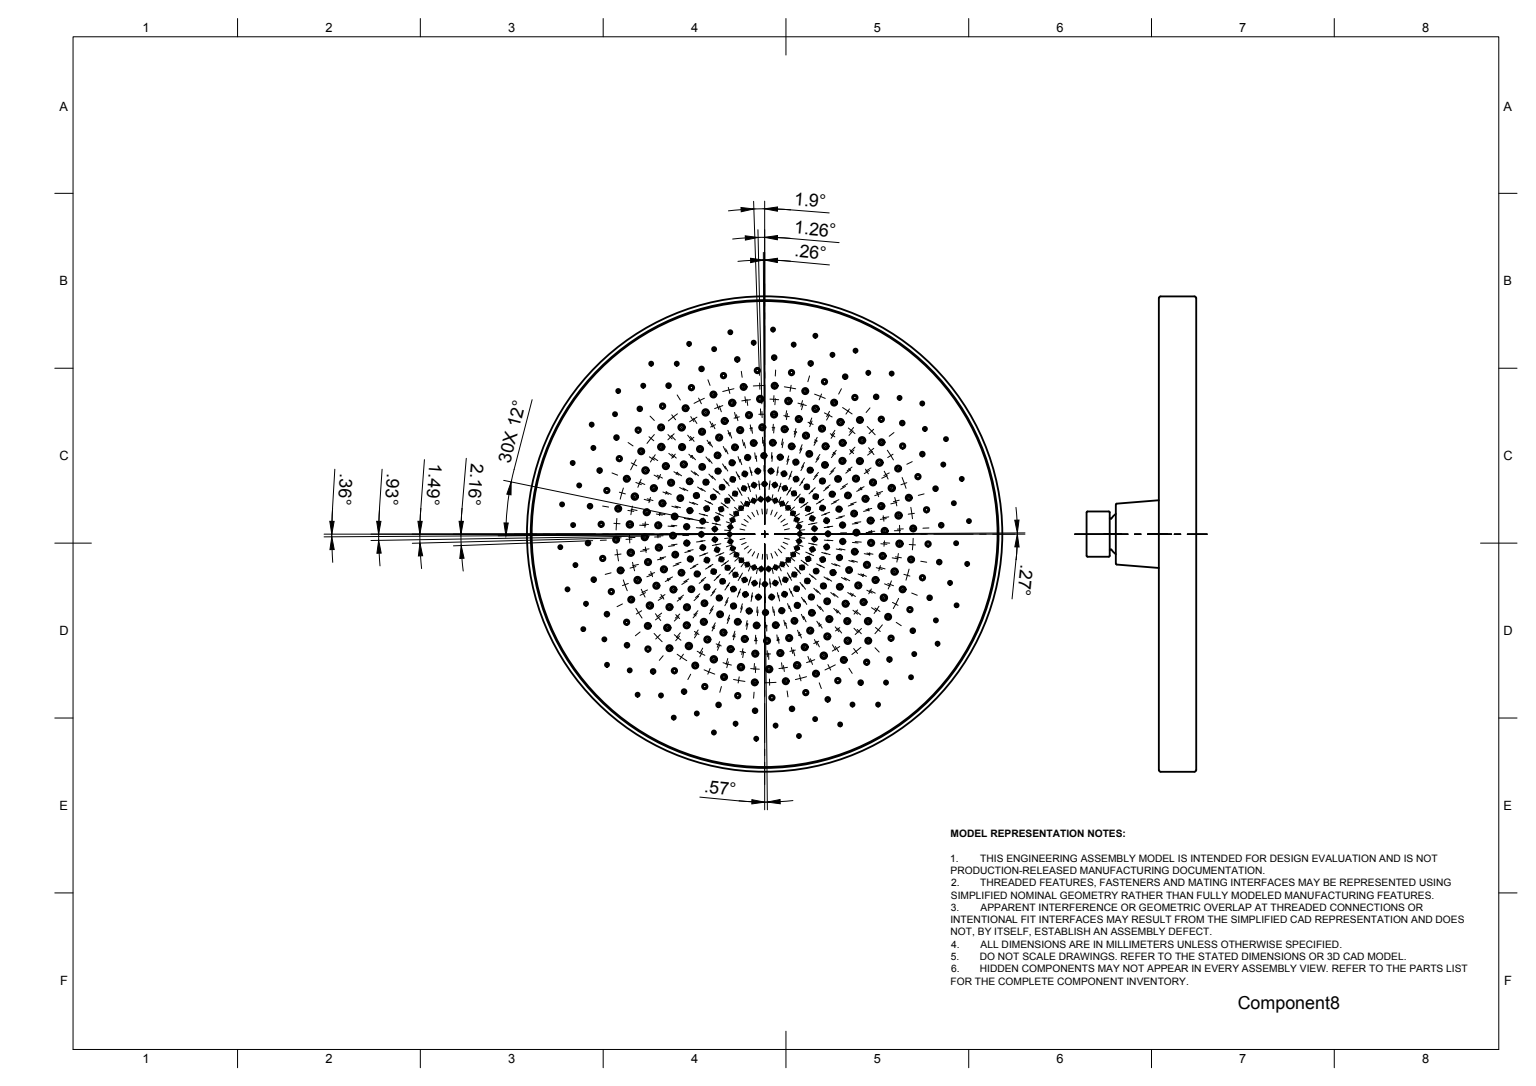
ISO-10303-21;
HEADER;
/* Generated by software containing ST-Developer
 * from STEP Tools, Inc. (www.steptools.com) 
 */

FILE_DESCRIPTION(
/* description */ ('STEP AP214'),
/* implementation_level */ '2;1');

FILE_NAME(
/* name */ 'Component8.step',
/* time_stamp */ '2026-10-06T11:02:40-07:00',
/* author */ (''),
/* organization */ (''),
/* preprocessor_version */ 'ST-DEVELOPER v20.2',
/* originating_system */ 'Autodesk Translation Framework v15.15.0.0',
/* authorisation */ '');

FILE_SCHEMA (('AUTOMOTIVE_DESIGN { 1 0 10303 214 3 1 1 }'));
ENDSEC;

DATA;
#10=MECHANICAL_DESIGN_GEOMETRIC_PRESENTATION_REPRESENTATION('',(#2943),#130910);
#70=SPHERICAL_SURFACE('',#50902,14.1583614602198);
#82=CONICAL_SURFACE('',#50915,18.5103550292801,0.080595262641945);
#732=FACE_BOUND('',#15338,.T.);
#733=FACE_BOUND('',#15339,.T.);
#734=FACE_BOUND('',#15340,.T.);
#735=FACE_BOUND('',#15341,.T.);
#736=FACE_BOUND('',#15342,.T.);
#737=FACE_BOUND('',#15343,.T.);
#738=FACE_BOUND('',#15344,.T.);
#739=FACE_BOUND('',#15345,.T.);
#740=FACE_BOUND('',#15346,.T.);
#741=FACE_BOUND('',#15347,.T.);
#742=FACE_BOUND('',#15348,.T.);
#743=FACE_BOUND('',#15349,.T.);
#744=FACE_BOUND('',#15350,.T.);
#745=FACE_BOUND('',#15351,.T.);
#746=FACE_BOUND('',#15352,.T.);
#747=FACE_BOUND('',#15353,.T.);
#748=FACE_BOUND('',#15354,.T.);
#749=FACE_BOUND('',#15355,.T.);
#750=FACE_BOUND('',#15356,.T.);
#751=FACE_BOUND('',#15357,.T.);
#752=FACE_BOUND('',#15358,.T.);
#753=FACE_BOUND('',#15359,.T.);
#754=FACE_BOUND('',#15360,.T.);
#755=FACE_BOUND('',#15361,.T.);
#756=FACE_BOUND('',#15362,.T.);
#757=FACE_BOUND('',#15363,.T.);
#758=FACE_BOUND('',#15364,.T.);
#759=FACE_BOUND('',#15365,.T.);
#760=FACE_BOUND('',#15366,.T.);
#761=FACE_BOUND('',#15367,.T.);
#762=FACE_BOUND('',#15368,.T.);
#763=FACE_BOUND('',#15369,.T.);
#764=FACE_BOUND('',#15370,.T.);
#765=FACE_BOUND('',#15371,.T.);
#766=FACE_BOUND('',#15372,.T.);
#767=FACE_BOUND('',#15373,.T.);
#768=FACE_BOUND('',#15374,.T.);
#769=FACE_BOUND('',#15375,.T.);
#770=FACE_BOUND('',#15376,.T.);
#771=FACE_BOUND('',#15377,.T.);
#772=FACE_BOUND('',#15378,.T.);
#773=FACE_BOUND('',#15379,.T.);
#774=FACE_BOUND('',#15380,.T.);
#775=FACE_BOUND('',#15381,.T.);
#776=FACE_BOUND('',#15382,.T.);
#777=FACE_BOUND('',#15383,.T.);
#778=FACE_BOUND('',#15384,.T.);
#779=FACE_BOUND('',#15385,.T.);
#780=FACE_BOUND('',#15386,.T.);
#781=FACE_BOUND('',#15387,.T.);
#782=FACE_BOUND('',#15388,.T.);
#783=FACE_BOUND('',#15389,.T.);
#784=FACE_BOUND('',#15390,.T.);
#785=FACE_BOUND('',#15391,.T.);
#786=FACE_BOUND('',#15392,.T.);
#787=FACE_BOUND('',#15393,.T.);
#788=FACE_BOUND('',#15394,.T.);
#789=FACE_BOUND('',#15395,.T.);
#790=FACE_BOUND('',#15396,.T.);
#791=FACE_BOUND('',#15397,.T.);
#792=FACE_BOUND('',#16183,.T.);
#793=FACE_BOUND('',#16193,.T.);
#794=FACE_BOUND('',#16196,.T.);
#795=FACE_BOUND('',#16198,.T.);
#796=FACE_BOUND('',#16200,.T.);
#797=FACE_BOUND('',#16203,.T.);
#798=FACE_BOUND('',#16205,.T.);
#799=FACE_BOUND('',#16206,.T.);
#800=FACE_BOUND('',#16207,.T.);
#801=FACE_BOUND('',#16208,.T.);
#802=FACE_BOUND('',#16209,.T.);
#803=FACE_BOUND('',#16210,.T.);
#804=FACE_BOUND('',#16211,.T.);
#805=FACE_BOUND('',#16212,.T.);
#806=FACE_BOUND('',#16213,.T.);
#807=FACE_BOUND('',#16214,.T.);
#808=FACE_BOUND('',#16215,.T.);
#809=FACE_BOUND('',#16216,.T.);
#810=FACE_BOUND('',#16217,.T.);
#811=FACE_BOUND('',#16218,.T.);
#812=FACE_BOUND('',#16219,.T.);
#813=FACE_BOUND('',#16220,.T.);
#814=FACE_BOUND('',#16221,.T.);
#815=FACE_BOUND('',#16222,.T.);
#816=FACE_BOUND('',#16223,.T.);
#817=FACE_BOUND('',#16224,.T.);
#818=FACE_BOUND('',#16225,.T.);
#819=FACE_BOUND('',#16226,.T.);
#820=FACE_BOUND('',#16227,.T.);
#821=FACE_BOUND('',#16228,.T.);
#822=FACE_BOUND('',#16229,.T.);
#823=FACE_BOUND('',#16230,.T.);
#824=FACE_BOUND('',#16231,.T.);
#825=FACE_BOUND('',#16232,.T.);
#826=FACE_BOUND('',#16233,.T.);
#827=FACE_BOUND('',#16234,.T.);
#828=FACE_BOUND('',#16235,.T.);
#829=FACE_BOUND('',#16236,.T.);
#830=FACE_BOUND('',#16237,.T.);
#831=FACE_BOUND('',#16238,.T.);
#832=FACE_BOUND('',#16239,.T.);
#833=FACE_BOUND('',#16240,.T.);
#834=FACE_BOUND('',#16241,.T.);
#835=FACE_BOUND('',#16242,.T.);
#836=FACE_BOUND('',#16243,.T.);
#837=FACE_BOUND('',#16244,.T.);
#838=FACE_BOUND('',#16245,.T.);
#839=FACE_BOUND('',#16246,.T.);
#840=FACE_BOUND('',#16247,.T.);
#841=FACE_BOUND('',#16248,.T.);
#842=FACE_BOUND('',#16249,.T.);
#843=FACE_BOUND('',#16250,.T.);
#844=FACE_BOUND('',#16251,.T.);
#845=FACE_BOUND('',#16252,.T.);
#846=FACE_BOUND('',#16253,.T.);
#847=FACE_BOUND('',#16254,.T.);
#848=FACE_BOUND('',#16255,.T.);
#849=FACE_BOUND('',#16256,.T.);
#850=FACE_BOUND('',#16257,.T.);
#851=FACE_BOUND('',#16258,.T.);
#852=FACE_BOUND('',#16259,.T.);
#853=FACE_BOUND('',#16260,.T.);
#854=FACE_BOUND('',#16261,.T.);
#855=FACE_BOUND('',#16262,.T.);
#856=FACE_BOUND('',#16263,.T.);
#857=FACE_BOUND('',#16264,.T.);
#858=FACE_BOUND('',#16265,.T.);
#859=FACE_BOUND('',#16266,.T.);
#860=FACE_BOUND('',#16267,.T.);
#861=FACE_BOUND('',#16268,.T.);
#862=FACE_BOUND('',#16269,.T.);
#863=FACE_BOUND('',#16270,.T.);
#864=FACE_BOUND('',#16271,.T.);
#865=FACE_BOUND('',#16272,.T.);
#866=FACE_BOUND('',#16273,.T.);
#867=FACE_BOUND('',#16274,.T.);
#868=FACE_BOUND('',#16275,.T.);
#869=FACE_BOUND('',#16276,.T.);
#870=FACE_BOUND('',#16277,.T.);
#871=FACE_BOUND('',#16278,.T.);
#872=FACE_BOUND('',#16279,.T.);
#873=FACE_BOUND('',#16280,.T.);
#874=FACE_BOUND('',#16281,.T.);
#875=FACE_BOUND('',#16282,.T.);
#876=FACE_BOUND('',#16283,.T.);
#877=FACE_BOUND('',#16284,.T.);
#878=FACE_BOUND('',#16285,.T.);
#879=FACE_BOUND('',#16286,.T.);
#880=FACE_BOUND('',#16287,.T.);
#881=FACE_BOUND('',#16288,.T.);
#882=FACE_BOUND('',#16289,.T.);
#883=FACE_BOUND('',#16290,.T.);
#884=FACE_BOUND('',#16291,.T.);
#885=FACE_BOUND('',#16292,.T.);
#886=FACE_BOUND('',#16293,.T.);
#887=FACE_BOUND('',#16294,.T.);
#888=FACE_BOUND('',#16295,.T.);
#889=FACE_BOUND('',#16296,.T.);
#890=FACE_BOUND('',#16297,.T.);
#891=FACE_BOUND('',#16298,.T.);
#892=FACE_BOUND('',#16299,.T.);
#893=FACE_BOUND('',#16300,.T.);
#894=FACE_BOUND('',#16301,.T.);
#895=FACE_BOUND('',#16302,.T.);
#896=FACE_BOUND('',#16303,.T.);
#897=FACE_BOUND('',#16304,.T.);
#898=FACE_BOUND('',#16305,.T.);
#899=FACE_BOUND('',#16306,.T.);
#900=FACE_BOUND('',#16307,.T.);
#901=FACE_BOUND('',#16308,.T.);
#902=FACE_BOUND('',#16309,.T.);
#903=FACE_BOUND('',#16310,.T.);
#904=FACE_BOUND('',#16311,.T.);
#905=FACE_BOUND('',#16312,.T.);
#906=FACE_BOUND('',#16313,.T.);
#907=FACE_BOUND('',#16314,.T.);
#908=FACE_BOUND('',#16315,.T.);
#909=FACE_BOUND('',#16316,.T.);
#910=FACE_BOUND('',#16317,.T.);
#911=FACE_BOUND('',#16318,.T.);
#912=FACE_BOUND('',#16319,.T.);
#913=FACE_BOUND('',#16320,.T.);
#914=FACE_BOUND('',#16321,.T.);
#915=FACE_BOUND('',#16322,.T.);
#916=FACE_BOUND('',#16323,.T.);
#917=FACE_BOUND('',#16324,.T.);
#918=FACE_BOUND('',#16325,.T.);
#919=FACE_BOUND('',#16326,.T.);
#920=FACE_BOUND('',#16327,.T.);
#921=FACE_BOUND('',#16328,.T.);
#922=FACE_BOUND('',#16329,.T.);
#923=FACE_BOUND('',#16330,.T.);
#924=FACE_BOUND('',#16331,.T.);
#925=FACE_BOUND('',#16332,.T.);
#926=FACE_BOUND('',#16333,.T.);
#927=FACE_BOUND('',#16334,.T.);
#928=FACE_BOUND('',#16335,.T.);
#929=FACE_BOUND('',#16336,.T.);
#930=FACE_BOUND('',#16337,.T.);
#931=FACE_BOUND('',#16338,.T.);
#932=FACE_BOUND('',#16339,.T.);
#933=FACE_BOUND('',#16340,.T.);
#934=FACE_BOUND('',#16341,.T.);
#935=FACE_BOUND('',#16342,.T.);
#936=FACE_BOUND('',#16343,.T.);
#937=FACE_BOUND('',#16344,.T.);
#938=FACE_BOUND('',#16345,.T.);
#939=FACE_BOUND('',#16346,.T.);
#940=FACE_BOUND('',#16347,.T.);
#941=FACE_BOUND('',#16348,.T.);
#942=FACE_BOUND('',#16349,.T.);
#943=FACE_BOUND('',#16350,.T.);
#944=FACE_BOUND('',#16351,.T.);
#945=FACE_BOUND('',#16352,.T.);
#946=FACE_BOUND('',#16353,.T.);
#947=FACE_BOUND('',#16354,.T.);
#948=FACE_BOUND('',#16355,.T.);
#949=FACE_BOUND('',#16356,.T.);
#950=FACE_BOUND('',#16357,.T.);
#951=FACE_BOUND('',#16358,.T.);
#952=FACE_BOUND('',#16359,.T.);
#953=FACE_BOUND('',#16360,.T.);
#954=FACE_BOUND('',#16361,.T.);
#955=FACE_BOUND('',#16362,.T.);
#956=FACE_BOUND('',#16363,.T.);
#957=FACE_BOUND('',#16364,.T.);
#958=FACE_BOUND('',#16365,.T.);
#959=FACE_BOUND('',#16366,.T.);
#960=FACE_BOUND('',#16367,.T.);
#961=FACE_BOUND('',#16368,.T.);
#962=FACE_BOUND('',#16369,.T.);
#963=FACE_BOUND('',#16370,.T.);
#964=FACE_BOUND('',#16371,.T.);
#965=FACE_BOUND('',#16372,.T.);
#966=FACE_BOUND('',#16373,.T.);
#967=FACE_BOUND('',#16374,.T.);
#968=FACE_BOUND('',#16375,.T.);
#969=FACE_BOUND('',#16376,.T.);
#970=FACE_BOUND('',#16377,.T.);
#971=FACE_BOUND('',#16378,.T.);
#972=FACE_BOUND('',#16379,.T.);
#973=FACE_BOUND('',#16380,.T.);
#974=FACE_BOUND('',#16381,.T.);
#975=FACE_BOUND('',#16382,.T.);
#976=FACE_BOUND('',#16383,.T.);
#977=FACE_BOUND('',#16384,.T.);
#978=FACE_BOUND('',#16385,.T.);
#979=FACE_BOUND('',#16386,.T.);
#980=FACE_BOUND('',#16387,.T.);
#981=FACE_BOUND('',#16388,.T.);
#982=FACE_BOUND('',#16389,.T.);
#983=FACE_BOUND('',#16390,.T.);
#984=FACE_BOUND('',#16391,.T.);
#985=FACE_BOUND('',#16392,.T.);
#986=FACE_BOUND('',#16393,.T.);
#987=FACE_BOUND('',#16394,.T.);
#988=FACE_BOUND('',#16395,.T.);
#989=FACE_BOUND('',#16396,.T.);
#990=FACE_BOUND('',#16397,.T.);
#991=FACE_BOUND('',#16398,.T.);
#992=FACE_BOUND('',#16399,.T.);
#993=FACE_BOUND('',#16400,.T.);
#994=FACE_BOUND('',#16401,.T.);
#995=FACE_BOUND('',#16402,.T.);
#996=FACE_BOUND('',#16403,.T.);
#997=FACE_BOUND('',#16404,.T.);
#998=FACE_BOUND('',#16405,.T.);
#999=FACE_BOUND('',#16406,.T.);
#1000=FACE_BOUND('',#16407,.T.);
#1001=FACE_BOUND('',#16408,.T.);
#1002=FACE_BOUND('',#16409,.T.);
#1003=FACE_BOUND('',#16410,.T.);
#1004=FACE_BOUND('',#16411,.T.);
#1005=FACE_BOUND('',#16412,.T.);
#1006=FACE_BOUND('',#16413,.T.);
#1007=FACE_BOUND('',#16414,.T.);
#1008=FACE_BOUND('',#16415,.T.);
#1009=FACE_BOUND('',#16416,.T.);
#1010=FACE_BOUND('',#16417,.T.);
#1011=FACE_BOUND('',#16418,.T.);
#1012=FACE_BOUND('',#16419,.T.);
#1013=FACE_BOUND('',#16420,.T.);
#1014=FACE_BOUND('',#16421,.T.);
#1015=FACE_BOUND('',#16422,.T.);
#1016=FACE_BOUND('',#16423,.T.);
#1017=FACE_BOUND('',#16424,.T.);
#1018=FACE_BOUND('',#16425,.T.);
#1019=FACE_BOUND('',#16426,.T.);
#1020=FACE_BOUND('',#16427,.T.);
#1021=FACE_BOUND('',#16428,.T.);
#1022=FACE_BOUND('',#16429,.T.);
#1023=FACE_BOUND('',#16430,.T.);
#1024=FACE_BOUND('',#16431,.T.);
#1025=FACE_BOUND('',#16432,.T.);
#1026=FACE_BOUND('',#16433,.T.);
#1027=FACE_BOUND('',#16434,.T.);
#1028=FACE_BOUND('',#16435,.T.);
#1029=FACE_BOUND('',#16436,.T.);
#1030=FACE_BOUND('',#16437,.T.);
#1031=FACE_BOUND('',#16438,.T.);
#1032=FACE_BOUND('',#16439,.T.);
#1033=FACE_BOUND('',#16440,.T.);
#1034=FACE_BOUND('',#16441,.T.);
#1035=FACE_BOUND('',#16442,.T.);
#1036=FACE_BOUND('',#16443,.T.);
#1037=FACE_BOUND('',#16444,.T.);
#1038=FACE_BOUND('',#16445,.T.);
#1039=FACE_BOUND('',#16446,.T.);
#1040=FACE_BOUND('',#16447,.T.);
#1041=FACE_BOUND('',#16448,.T.);
#1042=FACE_BOUND('',#16449,.T.);
#1043=FACE_BOUND('',#16450,.T.);
#1044=FACE_BOUND('',#16451,.T.);
#1045=FACE_BOUND('',#16452,.T.);
#1046=FACE_BOUND('',#16453,.T.);
#1047=FACE_BOUND('',#16454,.T.);
#1048=FACE_BOUND('',#16455,.T.);
#1049=FACE_BOUND('',#16456,.T.);
#1050=FACE_BOUND('',#16457,.T.);
#1051=FACE_BOUND('',#16458,.T.);
#1052=FACE_BOUND('',#16459,.T.);
#1053=FACE_BOUND('',#16460,.T.);
#1054=FACE_BOUND('',#16461,.T.);
#1055=FACE_BOUND('',#16462,.T.);
#1056=FACE_BOUND('',#16463,.T.);
#1057=FACE_BOUND('',#16464,.T.);
#1058=FACE_BOUND('',#16465,.T.);
#1059=FACE_BOUND('',#16466,.T.);
#1060=FACE_BOUND('',#16467,.T.);
#1061=FACE_BOUND('',#16468,.T.);
#1062=FACE_BOUND('',#16469,.T.);
#1063=FACE_BOUND('',#16470,.T.);
#1064=FACE_BOUND('',#16471,.T.);
#1065=FACE_BOUND('',#16472,.T.);
#1066=FACE_BOUND('',#16473,.T.);
#1067=FACE_BOUND('',#16474,.T.);
#1068=FACE_BOUND('',#16476,.T.);
#1069=FACE_BOUND('',#16477,.T.);
#1070=FACE_BOUND('',#16478,.T.);
#1071=FACE_BOUND('',#16479,.T.);
#1072=FACE_BOUND('',#16480,.T.);
#1073=FACE_BOUND('',#16481,.T.);
#1074=FACE_BOUND('',#16482,.T.);
#1075=FACE_BOUND('',#16483,.T.);
#1076=FACE_BOUND('',#16484,.T.);
#1077=FACE_BOUND('',#16485,.T.);
#1078=FACE_BOUND('',#16486,.T.);
#1079=FACE_BOUND('',#16487,.T.);
#1080=FACE_BOUND('',#16488,.T.);
#1081=FACE_BOUND('',#16489,.T.);
#1082=FACE_BOUND('',#16490,.T.);
#1083=FACE_BOUND('',#16491,.T.);
#1084=FACE_BOUND('',#16492,.T.);
#1085=FACE_BOUND('',#16493,.T.);
#1086=FACE_BOUND('',#16494,.T.);
#1087=FACE_BOUND('',#16495,.T.);
#1088=FACE_BOUND('',#16496,.T.);
#1089=FACE_BOUND('',#16497,.T.);
#1090=FACE_BOUND('',#16498,.T.);
#1091=FACE_BOUND('',#16499,.T.);
#1092=FACE_BOUND('',#16500,.T.);
#1093=FACE_BOUND('',#16501,.T.);
#1094=FACE_BOUND('',#16502,.T.);
#1095=FACE_BOUND('',#16503,.T.);
#1096=FACE_BOUND('',#16504,.T.);
#1097=FACE_BOUND('',#16505,.T.);
#1098=FACE_BOUND('',#16506,.T.);
#1099=FACE_BOUND('',#16507,.T.);
#1100=FACE_BOUND('',#16508,.T.);
#1101=FACE_BOUND('',#16509,.T.);
#1102=FACE_BOUND('',#16510,.T.);
#1103=FACE_BOUND('',#16511,.T.);
#1104=FACE_BOUND('',#16512,.T.);
#1105=FACE_BOUND('',#16513,.T.);
#1106=FACE_BOUND('',#16514,.T.);
#1107=FACE_BOUND('',#16515,.T.);
#1108=FACE_BOUND('',#16516,.T.);
#1109=FACE_BOUND('',#16517,.T.);
#1110=FACE_BOUND('',#16518,.T.);
#1111=FACE_BOUND('',#16519,.T.);
#1112=FACE_BOUND('',#16520,.T.);
#1113=FACE_BOUND('',#16521,.T.);
#1114=FACE_BOUND('',#16522,.T.);
#1115=FACE_BOUND('',#16523,.T.);
#1116=FACE_BOUND('',#16524,.T.);
#1117=FACE_BOUND('',#16525,.T.);
#1118=FACE_BOUND('',#16526,.T.);
#1119=FACE_BOUND('',#16527,.T.);
#1120=FACE_BOUND('',#16528,.T.);
#1121=FACE_BOUND('',#16529,.T.);
#1122=FACE_BOUND('',#16530,.T.);
#1123=FACE_BOUND('',#16531,.T.);
#1124=FACE_BOUND('',#16532,.T.);
#1125=FACE_BOUND('',#16533,.T.);
#1126=FACE_BOUND('',#16534,.T.);
#1127=FACE_BOUND('',#16535,.T.);
#1128=FACE_BOUND('',#16538,.T.);
#1129=FACE_BOUND('',#16541,.T.);
#1130=FACE_BOUND('',#16544,.T.);
#1131=FACE_BOUND('',#16547,.T.);
#1132=FACE_BOUND('',#16550,.T.);
#1133=FACE_BOUND('',#16553,.T.);
#1134=FACE_BOUND('',#16556,.T.);
#1135=FACE_BOUND('',#16559,.T.);
#1136=FACE_BOUND('',#16562,.T.);
#1137=FACE_BOUND('',#16565,.T.);
#1138=FACE_BOUND('',#16568,.T.);
#1139=FACE_BOUND('',#16571,.T.);
#1140=FACE_BOUND('',#16574,.T.);
#1141=FACE_BOUND('',#16577,.T.);
#1142=FACE_BOUND('',#16580,.T.);
#1143=FACE_BOUND('',#16583,.T.);
#1144=FACE_BOUND('',#16586,.T.);
#1145=FACE_BOUND('',#16589,.T.);
#1146=FACE_BOUND('',#16592,.T.);
#1147=FACE_BOUND('',#16595,.T.);
#1148=FACE_BOUND('',#16598,.T.);
#1149=FACE_BOUND('',#16601,.T.);
#1150=FACE_BOUND('',#16604,.T.);
#1151=FACE_BOUND('',#16607,.T.);
#1152=FACE_BOUND('',#16610,.T.);
#1153=FACE_BOUND('',#16613,.T.);
#1154=FACE_BOUND('',#16616,.T.);
#1155=FACE_BOUND('',#16619,.T.);
#1156=FACE_BOUND('',#16622,.T.);
#1157=FACE_BOUND('',#16625,.T.);
#1158=FACE_BOUND('',#16628,.T.);
#1159=FACE_BOUND('',#16631,.T.);
#1160=FACE_BOUND('',#16634,.T.);
#1161=FACE_BOUND('',#16637,.T.);
#1162=FACE_BOUND('',#16640,.T.);
#1163=FACE_BOUND('',#16643,.T.);
#1164=FACE_BOUND('',#16646,.T.);
#1165=FACE_BOUND('',#16649,.T.);
#1166=FACE_BOUND('',#16652,.T.);
#1167=FACE_BOUND('',#16655,.T.);
#1168=FACE_BOUND('',#16658,.T.);
#1169=FACE_BOUND('',#16661,.T.);
#1170=FACE_BOUND('',#16664,.T.);
#1171=FACE_BOUND('',#16667,.T.);
#1172=FACE_BOUND('',#16670,.T.);
#1173=FACE_BOUND('',#16673,.T.);
#1174=FACE_BOUND('',#16676,.T.);
#1175=FACE_BOUND('',#16679,.T.);
#1176=FACE_BOUND('',#16682,.T.);
#1177=FACE_BOUND('',#16685,.T.);
#1178=FACE_BOUND('',#16688,.T.);
#1179=FACE_BOUND('',#16691,.T.);
#1180=FACE_BOUND('',#16694,.T.);
#1181=FACE_BOUND('',#16697,.T.);
#1182=FACE_BOUND('',#16700,.T.);
#1183=FACE_BOUND('',#16703,.T.);
#1184=FACE_BOUND('',#16706,.T.);
#1185=FACE_BOUND('',#16709,.T.);
#1186=FACE_BOUND('',#16712,.T.);
#1187=FACE_BOUND('',#16715,.T.);
#1188=FACE_BOUND('',#16718,.T.);
#1189=FACE_BOUND('',#16721,.T.);
#1190=FACE_BOUND('',#16724,.T.);
#1191=FACE_BOUND('',#16727,.T.);
#1192=FACE_BOUND('',#16730,.T.);
#1193=FACE_BOUND('',#16733,.T.);
#1194=FACE_BOUND('',#16736,.T.);
#1195=FACE_BOUND('',#16739,.T.);
#1196=FACE_BOUND('',#16742,.T.);
#1197=FACE_BOUND('',#16745,.T.);
#1198=FACE_BOUND('',#16748,.T.);
#1199=FACE_BOUND('',#16751,.T.);
#1200=FACE_BOUND('',#16754,.T.);
#1201=FACE_BOUND('',#16757,.T.);
#1202=FACE_BOUND('',#16760,.T.);
#1203=FACE_BOUND('',#16763,.T.);
#1204=FACE_BOUND('',#16766,.T.);
#1205=FACE_BOUND('',#16769,.T.);
#1206=FACE_BOUND('',#16772,.T.);
#1207=FACE_BOUND('',#16775,.T.);
#1208=FACE_BOUND('',#16778,.T.);
#1209=FACE_BOUND('',#16781,.T.);
#1210=FACE_BOUND('',#16784,.T.);
#1211=FACE_BOUND('',#16787,.T.);
#1212=FACE_BOUND('',#16790,.T.);
#1213=FACE_BOUND('',#16793,.T.);
#1214=FACE_BOUND('',#16796,.T.);
#1215=FACE_BOUND('',#16799,.T.);
#1216=FACE_BOUND('',#16802,.T.);
#1217=FACE_BOUND('',#16805,.T.);
#1218=FACE_BOUND('',#16808,.T.);
#1219=FACE_BOUND('',#16811,.T.);
#1220=FACE_BOUND('',#16814,.T.);
#1221=FACE_BOUND('',#16817,.T.);
#1222=FACE_BOUND('',#16820,.T.);
#1223=FACE_BOUND('',#16823,.T.);
#1224=FACE_BOUND('',#16826,.T.);
#1225=FACE_BOUND('',#16829,.T.);
#1226=FACE_BOUND('',#16832,.T.);
#1227=FACE_BOUND('',#16835,.T.);
#1228=FACE_BOUND('',#16838,.T.);
#1229=FACE_BOUND('',#16841,.T.);
#1230=FACE_BOUND('',#16844,.T.);
#1231=FACE_BOUND('',#16847,.T.);
#1232=FACE_BOUND('',#16850,.T.);
#1233=FACE_BOUND('',#16853,.T.);
#1234=FACE_BOUND('',#16856,.T.);
#1235=FACE_BOUND('',#16859,.T.);
#1236=FACE_BOUND('',#16862,.T.);
#1237=FACE_BOUND('',#16865,.T.);
#1238=FACE_BOUND('',#16868,.T.);
#1239=FACE_BOUND('',#16871,.T.);
#1240=FACE_BOUND('',#16874,.T.);
#1241=FACE_BOUND('',#16877,.T.);
#1242=FACE_BOUND('',#16880,.T.);
#1243=FACE_BOUND('',#16883,.T.);
#1244=FACE_BOUND('',#16886,.T.);
#1245=FACE_BOUND('',#16889,.T.);
#1246=FACE_BOUND('',#16892,.T.);
#1247=FACE_BOUND('',#16895,.T.);
#1248=FACE_BOUND('',#16898,.T.);
#1249=FACE_BOUND('',#16901,.T.);
#1250=FACE_BOUND('',#16904,.T.);
#1251=FACE_BOUND('',#16907,.T.);
#1252=FACE_BOUND('',#16910,.T.);
#1253=FACE_BOUND('',#16913,.T.);
#1254=FACE_BOUND('',#16916,.T.);
#1255=FACE_BOUND('',#16919,.T.);
#1256=FACE_BOUND('',#16922,.T.);
#1257=FACE_BOUND('',#16925,.T.);
#1258=FACE_BOUND('',#16928,.T.);
#1259=FACE_BOUND('',#16931,.T.);
#1260=FACE_BOUND('',#16934,.T.);
#1261=FACE_BOUND('',#16937,.T.);
#1262=FACE_BOUND('',#16940,.T.);
#1263=FACE_BOUND('',#16943,.T.);
#1264=FACE_BOUND('',#16946,.T.);
#1265=FACE_BOUND('',#16949,.T.);
#1266=FACE_BOUND('',#16952,.T.);
#1267=FACE_BOUND('',#16955,.T.);
#1268=FACE_BOUND('',#16958,.T.);
#1269=FACE_BOUND('',#16961,.T.);
#1270=FACE_BOUND('',#16964,.T.);
#1271=FACE_BOUND('',#16967,.T.);
#1272=FACE_BOUND('',#16970,.T.);
#1273=FACE_BOUND('',#16973,.T.);
#1274=FACE_BOUND('',#16976,.T.);
#1275=FACE_BOUND('',#16979,.T.);
#1276=FACE_BOUND('',#16982,.T.);
#1277=FACE_BOUND('',#16985,.T.);
#1278=FACE_BOUND('',#16988,.T.);
#1279=FACE_BOUND('',#16991,.T.);
#1280=FACE_BOUND('',#16994,.T.);
#1281=FACE_BOUND('',#16997,.T.);
#1282=FACE_BOUND('',#17000,.T.);
#1283=FACE_BOUND('',#17003,.T.);
#1284=FACE_BOUND('',#17006,.T.);
#1285=FACE_BOUND('',#17009,.T.);
#1286=FACE_BOUND('',#17012,.T.);
#1287=FACE_BOUND('',#17015,.T.);
#1288=FACE_BOUND('',#17018,.T.);
#1289=FACE_BOUND('',#17021,.T.);
#1290=FACE_BOUND('',#17024,.T.);
#1291=FACE_BOUND('',#17027,.T.);
#1292=FACE_BOUND('',#17030,.T.);
#1293=FACE_BOUND('',#17033,.T.);
#1294=FACE_BOUND('',#17036,.T.);
#1295=FACE_BOUND('',#17039,.T.);
#1296=FACE_BOUND('',#17042,.T.);
#1297=FACE_BOUND('',#17045,.T.);
#1298=FACE_BOUND('',#17048,.T.);
#1299=FACE_BOUND('',#17051,.T.);
#1300=FACE_BOUND('',#17054,.T.);
#1301=FACE_BOUND('',#17057,.T.);
#1302=FACE_BOUND('',#17060,.T.);
#1303=FACE_BOUND('',#17063,.T.);
#1304=FACE_BOUND('',#17066,.T.);
#1305=FACE_BOUND('',#17069,.T.);
#1306=FACE_BOUND('',#17072,.T.);
#1307=FACE_BOUND('',#17075,.T.);
#1308=FACE_BOUND('',#17078,.T.);
#1309=FACE_BOUND('',#17081,.T.);
#1310=FACE_BOUND('',#17084,.T.);
#1311=FACE_BOUND('',#17087,.T.);
#1312=FACE_BOUND('',#17090,.T.);
#1313=FACE_BOUND('',#17093,.T.);
#1314=FACE_BOUND('',#17096,.T.);
#1315=FACE_BOUND('',#17099,.T.);
#1316=FACE_BOUND('',#17102,.T.);
#1317=FACE_BOUND('',#17105,.T.);
#1318=FACE_BOUND('',#17108,.T.);
#1319=FACE_BOUND('',#17111,.T.);
#1320=FACE_BOUND('',#17114,.T.);
#1321=FACE_BOUND('',#17117,.T.);
#1322=FACE_BOUND('',#17120,.T.);
#1323=FACE_BOUND('',#17123,.T.);
#1324=FACE_BOUND('',#17126,.T.);
#1325=FACE_BOUND('',#17129,.T.);
#1326=FACE_BOUND('',#17132,.T.);
#1327=FACE_BOUND('',#17135,.T.);
#1328=FACE_BOUND('',#17138,.T.);
#1329=FACE_BOUND('',#17141,.T.);
#1330=FACE_BOUND('',#17144,.T.);
#1331=FACE_BOUND('',#17147,.T.);
#1332=FACE_BOUND('',#17150,.T.);
#1333=FACE_BOUND('',#17153,.T.);
#1334=FACE_BOUND('',#17156,.T.);
#1335=FACE_BOUND('',#17159,.T.);
#1336=FACE_BOUND('',#17162,.T.);
#1337=FACE_BOUND('',#17165,.T.);
#1338=FACE_BOUND('',#17168,.T.);
#1339=FACE_BOUND('',#17171,.T.);
#1340=FACE_BOUND('',#17174,.T.);
#1341=FACE_BOUND('',#17177,.T.);
#1342=FACE_BOUND('',#17180,.T.);
#1343=FACE_BOUND('',#17183,.T.);
#1344=FACE_BOUND('',#17186,.T.);
#1345=FACE_BOUND('',#17189,.T.);
#1346=FACE_BOUND('',#17192,.T.);
#1347=FACE_BOUND('',#17195,.T.);
#1348=FACE_BOUND('',#17198,.T.);
#1349=FACE_BOUND('',#17201,.T.);
#1350=FACE_BOUND('',#17204,.T.);
#1351=FACE_BOUND('',#17207,.T.);
#1352=FACE_BOUND('',#17210,.T.);
#1353=FACE_BOUND('',#17213,.T.);
#1354=FACE_BOUND('',#17216,.T.);
#1355=FACE_BOUND('',#17219,.T.);
#1356=FACE_BOUND('',#17222,.T.);
#1357=FACE_BOUND('',#17225,.T.);
#1358=FACE_BOUND('',#17228,.T.);
#1359=FACE_BOUND('',#17231,.T.);
#1360=FACE_BOUND('',#17234,.T.);
#1361=FACE_BOUND('',#17237,.T.);
#1362=FACE_BOUND('',#17240,.T.);
#1363=FACE_BOUND('',#17243,.T.);
#1364=FACE_BOUND('',#17246,.T.);
#1365=FACE_BOUND('',#17249,.T.);
#1366=FACE_BOUND('',#17252,.T.);
#1367=FACE_BOUND('',#17255,.T.);
#1368=FACE_BOUND('',#17258,.T.);
#1369=FACE_BOUND('',#17261,.T.);
#1370=FACE_BOUND('',#17264,.T.);
#1371=FACE_BOUND('',#17267,.T.);
#1372=FACE_BOUND('',#17270,.T.);
#1373=FACE_BOUND('',#17273,.T.);
#1374=FACE_BOUND('',#17276,.T.);
#1375=FACE_BOUND('',#17279,.T.);
#1376=FACE_BOUND('',#17282,.T.);
#1377=FACE_BOUND('',#17285,.T.);
#1378=FACE_BOUND('',#17288,.T.);
#1379=FACE_BOUND('',#17291,.T.);
#1380=FACE_BOUND('',#17294,.T.);
#1381=FACE_BOUND('',#17297,.T.);
#1382=FACE_BOUND('',#17300,.T.);
#1383=FACE_BOUND('',#17303,.T.);
#1384=FACE_BOUND('',#17306,.T.);
#1385=FACE_BOUND('',#17309,.T.);
#1386=FACE_BOUND('',#17312,.T.);
#1387=FACE_BOUND('',#17315,.T.);
#1388=FACE_BOUND('',#17318,.T.);
#1389=FACE_BOUND('',#17321,.T.);
#1390=FACE_BOUND('',#17324,.T.);
#1391=FACE_BOUND('',#17327,.T.);
#1392=FACE_BOUND('',#17330,.T.);
#1393=FACE_BOUND('',#17333,.T.);
#1394=FACE_BOUND('',#17336,.T.);
#1395=FACE_BOUND('',#17339,.T.);
#1396=FACE_BOUND('',#17342,.T.);
#1397=FACE_BOUND('',#17345,.T.);
#1398=FACE_BOUND('',#17348,.T.);
#1399=FACE_BOUND('',#17351,.T.);
#1400=FACE_BOUND('',#17354,.T.);
#1401=FACE_BOUND('',#17357,.T.);
#1402=FACE_BOUND('',#17360,.T.);
#1403=FACE_BOUND('',#17363,.T.);
#1404=FACE_BOUND('',#17366,.T.);
#1405=FACE_BOUND('',#17369,.T.);
#1406=FACE_BOUND('',#17372,.T.);
#1407=FACE_BOUND('',#17375,.T.);
#1408=FACE_BOUND('',#17378,.T.);
#1409=FACE_BOUND('',#17381,.T.);
#1410=FACE_BOUND('',#17384,.T.);
#1411=FACE_BOUND('',#17387,.T.);
#1412=FACE_BOUND('',#17390,.T.);
#1413=FACE_BOUND('',#17393,.T.);
#1414=FACE_BOUND('',#17396,.T.);
#1415=FACE_BOUND('',#17399,.T.);
#1416=FACE_BOUND('',#17402,.T.);
#1417=FACE_BOUND('',#17405,.T.);
#1418=FACE_BOUND('',#17408,.T.);
#1419=FACE_BOUND('',#17411,.T.);
#1420=FACE_BOUND('',#17414,.T.);
#1421=FACE_BOUND('',#17417,.T.);
#1422=FACE_BOUND('',#17420,.T.);
#1423=FACE_BOUND('',#17423,.T.);
#1424=FACE_BOUND('',#17426,.T.);
#1425=FACE_BOUND('',#17429,.T.);
#1426=FACE_BOUND('',#17432,.T.);
#1427=FACE_BOUND('',#17435,.T.);
#1428=FACE_BOUND('',#17438,.T.);
#1429=FACE_BOUND('',#17441,.T.);
#1430=FACE_BOUND('',#17444,.T.);
#1431=FACE_BOUND('',#17447,.T.);
#1432=FACE_BOUND('',#17450,.T.);
#1433=FACE_BOUND('',#17453,.T.);
#1434=FACE_BOUND('',#17456,.T.);
#1435=FACE_BOUND('',#17459,.T.);
#1436=FACE_BOUND('',#17462,.T.);
#1437=FACE_BOUND('',#17465,.T.);
#1438=FACE_BOUND('',#17468,.T.);
#1439=FACE_BOUND('',#17471,.T.);
#1440=FACE_BOUND('',#17474,.T.);
#1441=FACE_BOUND('',#17477,.T.);
#1442=FACE_BOUND('',#17480,.T.);
#1443=FACE_BOUND('',#17483,.T.);
#1444=FACE_BOUND('',#17486,.T.);
#1445=FACE_BOUND('',#17489,.T.);
#1446=FACE_BOUND('',#17492,.T.);
#1447=FACE_BOUND('',#17495,.T.);
#1448=FACE_BOUND('',#17498,.T.);
#1449=FACE_BOUND('',#17501,.T.);
#1450=FACE_BOUND('',#17504,.T.);
#1451=FACE_BOUND('',#17507,.T.);
#1452=FACE_BOUND('',#17510,.T.);
#1453=FACE_BOUND('',#17513,.T.);
#1454=FACE_BOUND('',#17516,.T.);
#1455=FACE_BOUND('',#17519,.T.);
#1456=FACE_BOUND('',#17522,.T.);
#1457=FACE_BOUND('',#17525,.T.);
#1458=FACE_BOUND('',#17528,.T.);
#1459=FACE_BOUND('',#17531,.T.);
#1460=FACE_BOUND('',#17534,.T.);
#1461=FACE_BOUND('',#17537,.T.);
#1462=FACE_BOUND('',#17540,.T.);
#1463=FACE_BOUND('',#17543,.T.);
#1464=FACE_BOUND('',#17546,.T.);
#1465=FACE_BOUND('',#17549,.T.);
#1466=FACE_BOUND('',#17552,.T.);
#1467=FACE_BOUND('',#17555,.T.);
#1468=FACE_BOUND('',#17558,.T.);
#1469=FACE_BOUND('',#17561,.T.);
#1470=FACE_BOUND('',#17564,.T.);
#1471=FACE_BOUND('',#17567,.T.);
#1472=FACE_BOUND('',#17570,.T.);
#1473=FACE_BOUND('',#17573,.T.);
#1474=FACE_BOUND('',#17576,.T.);
#1475=FACE_BOUND('',#17579,.T.);
#1476=FACE_BOUND('',#17582,.T.);
#1477=FACE_BOUND('',#17585,.T.);
#1478=FACE_BOUND('',#17588,.T.);
#1479=FACE_BOUND('',#17591,.T.);
#1480=FACE_BOUND('',#17594,.T.);
#1481=FACE_BOUND('',#17597,.T.);
#1482=FACE_BOUND('',#17600,.T.);
#1483=FACE_BOUND('',#17603,.T.);
#1484=FACE_BOUND('',#17606,.T.);
#1485=FACE_BOUND('',#17609,.T.);
#1486=FACE_BOUND('',#17612,.T.);
#1487=FACE_BOUND('',#17615,.T.);
#1488=FACE_BOUND('',#17618,.T.);
#1489=FACE_BOUND('',#17621,.T.);
#1490=FACE_BOUND('',#17624,.T.);
#1491=FACE_BOUND('',#17627,.T.);
#1492=FACE_BOUND('',#17630,.T.);
#1493=FACE_BOUND('',#17633,.T.);
#1494=FACE_BOUND('',#17636,.T.);
#1495=FACE_BOUND('',#17639,.T.);
#1496=FACE_BOUND('',#17642,.T.);
#1497=FACE_BOUND('',#17645,.T.);
#1498=FACE_BOUND('',#17648,.T.);
#1499=FACE_BOUND('',#17651,.T.);
#1500=FACE_BOUND('',#17654,.T.);
#1501=FACE_BOUND('',#17657,.T.);
#1502=FACE_BOUND('',#17660,.T.);
#1503=FACE_BOUND('',#17663,.T.);
#1504=FACE_BOUND('',#17666,.T.);
#1505=FACE_BOUND('',#17669,.T.);
#1506=FACE_BOUND('',#17672,.T.);
#1507=FACE_BOUND('',#17675,.T.);
#1508=FACE_BOUND('',#17678,.T.);
#1509=FACE_BOUND('',#17681,.T.);
#1510=FACE_BOUND('',#17684,.T.);
#1511=FACE_BOUND('',#17687,.T.);
#1512=FACE_BOUND('',#17690,.T.);
#1513=FACE_BOUND('',#17693,.T.);
#1514=FACE_BOUND('',#17696,.T.);
#1515=FACE_BOUND('',#17699,.T.);
#1516=FACE_BOUND('',#17702,.T.);
#1686=(
BOUNDED_SURFACE()
B_SPLINE_SURFACE(2,3,((#106592,#106593,#106594,#106595),(#106596,#106597,
#106598,#106599),(#106600,#106601,#106602,#106603)),.UNSPECIFIED.,.F.,.F.,
 .F.)
B_SPLINE_SURFACE_WITH_KNOTS((3,3),(4,4),(0.,0.976475345222878),(0.,1.),
 .UNSPECIFIED.)
GEOMETRIC_REPRESENTATION_ITEM()
RATIONAL_B_SPLINE_SURFACE(((1.,0.333333333333333,0.333333333333333,1.),
(1.,0.333333333333333,0.333333333333333,1.),(1.,0.333333333333333,0.333333333333333,
1.)))
REPRESENTATION_ITEM('')
SURFACE()
);
#1687=(
BOUNDED_SURFACE()
B_SPLINE_SURFACE(3,3,((#128284,#128285,#128286,#128287),(#128288,#128289,
#128290,#128291),(#128292,#128293,#128294,#128295),(#128296,#128297,#128298,
#128299)),.UNSPECIFIED.,.F.,.F.,.F.)
B_SPLINE_SURFACE_WITH_KNOTS((4,4),(4,4),(0.847987177476328,0.924268857153948),
(0.,1.),.UNSPECIFIED.)
GEOMETRIC_REPRESENTATION_ITEM()
RATIONAL_B_SPLINE_SURFACE(((1.,0.999906698612453,0.999906698612453,1.),
(1.,0.999906698612453,0.999906698612453,1.),(1.,0.999906698612453,0.999906698612453,
1.),(1.,0.999906698612453,0.999906698612453,1.)))
REPRESENTATION_ITEM('')
SURFACE()
);
#1688=(
BOUNDED_SURFACE()
B_SPLINE_SURFACE(2,3,((#128308,#128309,#128310,#128311),(#128312,#128313,
#128314,#128315),(#128316,#128317,#128318,#128319)),.UNSPECIFIED.,.F.,.F.,
 .F.)
B_SPLINE_SURFACE_WITH_KNOTS((3,3),(4,4),(0.,0.976475345222877),(0.,1.),
 .UNSPECIFIED.)
GEOMETRIC_REPRESENTATION_ITEM()
RATIONAL_B_SPLINE_SURFACE(((1.,0.333333333333333,0.333333333333333,1.),
(1.,0.333333333333333,0.333333333333333,1.),(1.,0.333333333333333,0.333333333333333,
1.)))
REPRESENTATION_ITEM('')
SURFACE()
);
#1689=(
BOUNDED_SURFACE()
B_SPLINE_SURFACE(3,3,((#128861,#128862,#128863,#128864),(#128865,#128866,
#128867,#128868),(#128869,#128870,#128871,#128872),(#128873,#128874,#128875,
#128876)),.UNSPECIFIED.,.F.,.F.,.F.)
B_SPLINE_SURFACE_WITH_KNOTS((4,4),(4,4),(0.485044458534508,0.53777950288349),
(0.,1.),.UNSPECIFIED.)
GEOMETRIC_REPRESENTATION_ITEM()
RATIONAL_B_SPLINE_SURFACE(((1.,0.999962226576742,0.999962226576742,1.),
(1.,0.999962226576742,0.999962226576742,1.),(1.,0.999962226576742,0.999962226576742,
1.),(1.,0.999962226576742,0.999962226576742,1.)))
REPRESENTATION_ITEM('')
SURFACE()
);
#1690=(
BOUNDED_SURFACE()
B_SPLINE_SURFACE(3,3,((#128878,#128879,#128880,#128881),(#128882,#128883,
#128884,#128885),(#128886,#128887,#128888,#128889),(#128890,#128891,#128892,
#128893)),.UNSPECIFIED.,.F.,.F.,.F.)
B_SPLINE_SURFACE_WITH_KNOTS((4,4),(4,4),(0.320611406771219,0.371419418548152),
(0.,1.),.UNSPECIFIED.)
GEOMETRIC_REPRESENTATION_ITEM()
RATIONAL_B_SPLINE_SURFACE(((1.,0.999967235134602,0.999967235134602,1.),
(1.,0.999967235134602,0.999967235134602,1.),(1.,0.999967235134602,0.999967235134602,
1.),(1.,0.999967235134602,0.999967235134602,1.)))
REPRESENTATION_ITEM('')
SURFACE()
);
#1691=(
BOUNDED_SURFACE()
B_SPLINE_SURFACE(3,3,((#128895,#128896,#128897,#128898),(#128899,#128900,
#128901,#128902),(#128903,#128904,#128905,#128906),(#128907,#128908,#128909,
#128910)),.UNSPECIFIED.,.F.,.F.,.F.)
B_SPLINE_SURFACE_WITH_KNOTS((4,4),(4,4),(0.675456663809549,0.739075881246651),
(0.,1.),.UNSPECIFIED.)
GEOMETRIC_REPRESENTATION_ITEM()
RATIONAL_B_SPLINE_SURFACE(((1.,0.999940066556315,0.999940066556315,1.),
(1.,0.999940066556315,0.999940066556315,1.),(1.,0.999940066556315,0.999940066556315,
1.),(1.,0.999940066556315,0.999940066556315,1.)))
REPRESENTATION_ITEM('')
SURFACE()
);
#1692=(
BOUNDED_SURFACE()
B_SPLINE_SURFACE(3,3,((#128912,#128913,#128914,#128915),(#128916,#128917,
#128918,#128919),(#128920,#128921,#128922,#128923),(#128924,#128925,#128926,
#128927)),.UNSPECIFIED.,.F.,.F.,.F.)
B_SPLINE_SURFACE_WITH_KNOTS((4,4),(4,4),(0.848056712870581,0.924286002747189),
(0.,1.),.UNSPECIFIED.)
GEOMETRIC_REPRESENTATION_ITEM()
RATIONAL_B_SPLINE_SURFACE(((1.,0.999906141303136,0.999906141303136,1.),
(1.,0.999906141303136,0.999906141303136,1.),(1.,0.999906141303136,0.999906141303136,
1.),(1.,0.999906141303136,0.999906141303136,1.)))
REPRESENTATION_ITEM('')
SURFACE()
);
#1693=(
BOUNDED_SURFACE()
B_SPLINE_SURFACE(3,3,((#128929,#128930,#128931,#128932),(#128933,#128934,
#128935,#128936),(#128937,#128938,#128939,#128940),(#128941,#128942,#128943,
#128944)),.UNSPECIFIED.,.F.,.F.,.F.)
B_SPLINE_SURFACE_WITH_KNOTS((4,4),(4,4),(0.320500925502344,0.371279762151148),
(0.,1.),.UNSPECIFIED.)
GEOMETRIC_REPRESENTATION_ITEM()
RATIONAL_B_SPLINE_SURFACE(((1.,0.999967409032415,0.999967409032415,1.),
(1.,0.999967409032415,0.999967409032415,1.),(1.,0.999967409032415,0.999967409032415,
1.),(1.,0.999967409032415,0.999967409032415,1.)))
REPRESENTATION_ITEM('')
SURFACE()
);
#1694=(
BOUNDED_SURFACE()
B_SPLINE_SURFACE(3,3,((#128946,#128947,#128948,#128949),(#128950,#128951,
#128952,#128953),(#128954,#128955,#128956,#128957),(#128958,#128959,#128960,
#128961)),.UNSPECIFIED.,.F.,.F.,.F.)
B_SPLINE_SURFACE_WITH_KNOTS((4,4),(4,4),(0.485038746158877,0.537899824885899),
(0.,1.),.UNSPECIFIED.)
GEOMETRIC_REPRESENTATION_ITEM()
RATIONAL_B_SPLINE_SURFACE(((1.,0.999962208905504,0.999962208905504,1.),
(1.,0.999962208905504,0.999962208905504,1.),(1.,0.999962208905504,0.999962208905504,
1.),(1.,0.999962208905504,0.999962208905504,1.)))
REPRESENTATION_ITEM('')
SURFACE()
);
#1695=(
BOUNDED_SURFACE()
B_SPLINE_SURFACE(3,3,((#128963,#128964,#128965,#128966),(#128967,#128968,
#128969,#128970),(#128971,#128972,#128973,#128974),(#128975,#128976,#128977,
#128978)),.UNSPECIFIED.,.F.,.F.,.F.)
B_SPLINE_SURFACE_WITH_KNOTS((4,4),(4,4),(0.675591945838646,0.739081108319602),
(0.,1.),.UNSPECIFIED.)
GEOMETRIC_REPRESENTATION_ITEM()
RATIONAL_B_SPLINE_SURFACE(((1.,0.999939919244887,0.999939919244887,1.),
(1.,0.999939919244887,0.999939919244887,1.),(1.,0.999939919244887,0.999939919244887,
1.),(1.,0.999939919244887,0.999939919244887,1.)))
REPRESENTATION_ITEM('')
SURFACE()
);
#1696=(
BOUNDED_SURFACE()
B_SPLINE_SURFACE(3,3,((#128980,#128981,#128982,#128983),(#128984,#128985,
#128986,#128987),(#128988,#128989,#128990,#128991),(#128992,#128993,#128994,
#128995)),.UNSPECIFIED.,.F.,.F.,.F.)
B_SPLINE_SURFACE_WITH_KNOTS((4,4),(4,4),(0.847948073492975,0.924101847380027),
(0.,1.),.UNSPECIFIED.)
GEOMETRIC_REPRESENTATION_ITEM()
RATIONAL_B_SPLINE_SURFACE(((1.,0.999906397449935,0.999906397449935,1.),
(1.,0.999906397449935,0.999906397449935,1.),(1.,0.999906397449935,0.999906397449935,
1.),(1.,0.999906397449935,0.999906397449935,1.)))
REPRESENTATION_ITEM('')
SURFACE()
);
#1697=(
BOUNDED_SURFACE()
B_SPLINE_SURFACE(3,3,((#128997,#128998,#128999,#129000),(#129001,#129002,
#129003,#129004),(#129005,#129006,#129007,#129008),(#129009,#129010,#129011,
#129012)),.UNSPECIFIED.,.F.,.F.,.F.)
B_SPLINE_SURFACE_WITH_KNOTS((4,4),(4,4),(0.320502373890073,0.371416725883164),
(0.,1.),.UNSPECIFIED.)
GEOMETRIC_REPRESENTATION_ITEM()
RATIONAL_B_SPLINE_SURFACE(((1.,0.999967412958646,0.999967412958646,1.),
(1.,0.999967412958646,0.999967412958646,1.),(1.,0.999967412958646,0.999967412958646,
1.),(1.,0.999967412958646,0.999967412958646,1.)))
REPRESENTATION_ITEM('')
SURFACE()
);
#1698=(
BOUNDED_SURFACE()
B_SPLINE_SURFACE(3,3,((#129014,#129015,#129016,#129017),(#129018,#129019,
#129020,#129021),(#129022,#129023,#129024,#129025),(#129026,#129027,#129028,
#129029)),.UNSPECIFIED.,.F.,.F.,.F.)
B_SPLINE_SURFACE_WITH_KNOTS((4,4),(4,4),(0.485176572716987,0.537896306928668),
(0.,1.),.UNSPECIFIED.)
GEOMETRIC_REPRESENTATION_ITEM()
RATIONAL_B_SPLINE_SURFACE(((1.,0.999962047914293,0.999962047914293,1.),
(1.,0.999962047914293,0.999962047914293,1.),(1.,0.999962047914293,0.999962047914293,
1.),(1.,0.999962047914293,0.999962047914293,1.)))
REPRESENTATION_ITEM('')
SURFACE()
);
#1699=(
BOUNDED_SURFACE()
B_SPLINE_SURFACE(3,3,((#129031,#129032,#129033,#129034),(#129035,#129036,
#129037,#129038),(#129039,#129040,#129041,#129042),(#129043,#129044,#129045,
#129046)),.UNSPECIFIED.,.F.,.F.,.F.)
B_SPLINE_SURFACE_WITH_KNOTS((4,4),(4,4),(0.675443757413942,0.738914540526937),
(0.,1.),.UNSPECIFIED.)
GEOMETRIC_REPRESENTATION_ITEM()
RATIONAL_B_SPLINE_SURFACE(((1.,0.999940218802441,0.999940218802441,1.),
(1.,0.999940218802441,0.999940218802441,1.),(1.,0.999940218802441,0.999940218802441,
1.),(1.,0.999940218802441,0.999940218802441,1.)))
REPRESENTATION_ITEM('')
SURFACE()
);
#1700=(
BOUNDED_SURFACE()
B_SPLINE_SURFACE(3,3,((#129048,#129049,#129050,#129051),(#129052,#129053,
#129054,#129055),(#129056,#129057,#129058,#129059),(#129060,#129061,#129062,
#129063)),.UNSPECIFIED.,.F.,.F.,.F.)
B_SPLINE_SURFACE_WITH_KNOTS((4,4),(4,4),(0.847942166937427,0.924299897199325),
(0.,1.),.UNSPECIFIED.)
GEOMETRIC_REPRESENTATION_ITEM()
RATIONAL_B_SPLINE_SURFACE(((1.,0.999906256993129,0.999906256993129,1.),
(1.,0.999906256993129,0.999906256993129,1.),(1.,0.999906256993129,0.999906256993129,
1.),(1.,0.999906256993129,0.999906256993129,1.)))
REPRESENTATION_ITEM('')
SURFACE()
);
#1701=(
BOUNDED_SURFACE()
B_SPLINE_SURFACE(3,3,((#129065,#129066,#129067,#129068),(#129069,#129070,
#129071,#129072),(#129073,#129074,#129075,#129076),(#129077,#129078,#129079,
#129080)),.UNSPECIFIED.,.F.,.F.,.F.)
B_SPLINE_SURFACE_WITH_KNOTS((4,4),(4,4),(0.320591553275913,0.371408509515467),
(0.,1.),.UNSPECIFIED.)
GEOMETRIC_REPRESENTATION_ITEM()
RATIONAL_B_SPLINE_SURFACE(((1.,0.999967222717093,0.999967222717093,1.),
(1.,0.999967222717093,0.999967222717093,1.),(1.,0.999967222717093,0.999967222717093,
1.),(1.,0.999967222717093,0.999967222717093,1.)))
REPRESENTATION_ITEM('')
SURFACE()
);
#1702=(
BOUNDED_SURFACE()
B_SPLINE_SURFACE(3,3,((#129082,#129083,#129084,#129085),(#129086,#129087,
#129088,#129089),(#129090,#129091,#129092,#129093),(#129094,#129095,#129096,
#129097)),.UNSPECIFIED.,.F.,.F.,.F.)
B_SPLINE_SURFACE_WITH_KNOTS((4,4),(4,4),(0.485044526648914,0.537808799135296),
(0.,1.),.UNSPECIFIED.)
GEOMETRIC_REPRESENTATION_ITEM()
RATIONAL_B_SPLINE_SURFACE(((1.,0.999962197880072,0.999962197880072,1.),
(1.,0.999962197880072,0.999962197880072,1.),(1.,0.999962197880072,0.999962197880072,
1.),(1.,0.999962197880072,0.999962197880072,1.)))
REPRESENTATION_ITEM('')
SURFACE()
);
#1703=(
BOUNDED_SURFACE()
B_SPLINE_SURFACE(3,3,((#129099,#129100,#129101,#129102),(#129103,#129104,
#129105,#129106),(#129107,#129108,#129109,#129110),(#129111,#129112,#129113,
#129114)),.UNSPECIFIED.,.F.,.F.,.F.)
B_SPLINE_SURFACE_WITH_KNOTS((4,4),(4,4),(0.675446956850003,0.739072743686735),
(0.,1.),.UNSPECIFIED.)
GEOMETRIC_REPRESENTATION_ITEM()
RATIONAL_B_SPLINE_SURFACE(((1.,0.999940262362188,0.999940262362188,1.),
(1.,0.999940262362188,0.999940262362188,1.),(1.,0.999940262362188,0.999940262362188,
1.),(1.,0.999940262362188,0.999940262362188,1.)))
REPRESENTATION_ITEM('')
SURFACE()
);
#1704=(
BOUNDED_SURFACE()
B_SPLINE_SURFACE(3,3,((#129116,#129117,#129118,#129119),(#129120,#129121,
#129122,#129123),(#129124,#129125,#129126,#129127),(#129128,#129129,#129130,
#129131)),.UNSPECIFIED.,.F.,.F.,.F.)
B_SPLINE_SURFACE_WITH_KNOTS((4,4),(4,4),(0.848119490523076,0.924292153421624),
(0.,1.),.UNSPECIFIED.)
GEOMETRIC_REPRESENTATION_ITEM()
RATIONAL_B_SPLINE_SURFACE(((1.,0.999905838370628,0.999905838370628,1.),
(1.,0.999905838370628,0.999905838370628,1.),(1.,0.999905838370628,0.999905838370628,
1.),(1.,0.999905838370628,0.999905838370628,1.)))
REPRESENTATION_ITEM('')
SURFACE()
);
#1705=(
BOUNDED_SURFACE()
B_SPLINE_SURFACE(3,3,((#129133,#129134,#129135,#129136),(#129137,#129138,
#129139,#129140),(#129141,#129142,#129143,#129144),(#129145,#129146,#129147,
#129148)),.UNSPECIFIED.,.F.,.F.,.F.)
B_SPLINE_SURFACE_WITH_KNOTS((4,4),(4,4),(0.320518889190736,0.371365428236457),
(0.,1.),.UNSPECIFIED.)
GEOMETRIC_REPRESENTATION_ITEM()
RATIONAL_B_SPLINE_SURFACE(((1.,0.999967318979484,0.999967318979484,1.),
(1.,0.999967318979484,0.999967318979484,1.),(1.,0.999967318979484,0.999967318979484,
1.),(1.,0.999967318979484,0.999967318979484,1.)))
REPRESENTATION_ITEM('')
SURFACE()
);
#1706=(
BOUNDED_SURFACE()
B_SPLINE_SURFACE(3,3,((#129150,#129151,#129152,#129153),(#129154,#129155,
#129156,#129157),(#129158,#129159,#129160,#129161),(#129162,#129163,#129164,
#129165)),.UNSPECIFIED.,.F.,.F.,.F.)
B_SPLINE_SURFACE_WITH_KNOTS((4,4),(4,4),(0.485053151926106,0.537874785203655),
(0.,1.),.UNSPECIFIED.)
GEOMETRIC_REPRESENTATION_ITEM()
RATIONAL_B_SPLINE_SURFACE(((1.,0.999962225139893,0.999962225139893,1.),
(1.,0.999962225139893,0.999962225139893,1.),(1.,0.999962225139893,0.999962225139893,
1.),(1.,0.999962225139893,0.999962225139893,1.)))
REPRESENTATION_ITEM('')
SURFACE()
);
#1707=(
BOUNDED_SURFACE()
B_SPLINE_SURFACE(3,3,((#129167,#129168,#129169,#129170),(#129171,#129172,
#129173,#129174),(#129175,#129176,#129177,#129178),(#129179,#129180,#129181,
#129182)),.UNSPECIFIED.,.F.,.F.,.F.)
B_SPLINE_SURFACE_WITH_KNOTS((4,4),(4,4),(0.675540106157524,0.739058970060862),
(0.,1.),.UNSPECIFIED.)
GEOMETRIC_REPRESENTATION_ITEM()
RATIONAL_B_SPLINE_SURFACE(((1.,0.999939959405442,0.999939959405442,1.),
(1.,0.999939959405442,0.999939959405442,1.),(1.,0.999939959405442,0.999939959405442,
1.),(1.,0.999939959405442,0.999939959405442,1.)))
REPRESENTATION_ITEM('')
SURFACE()
);
#1708=(
BOUNDED_SURFACE()
B_SPLINE_SURFACE(3,3,((#129184,#129185,#129186,#129187),(#129188,#129189,
#129190,#129191),(#129192,#129193,#129194,#129195),(#129196,#129197,#129198,
#129199)),.UNSPECIFIED.,.F.,.F.,.F.)
B_SPLINE_SURFACE_WITH_KNOTS((4,4),(4,4),(0.847959162456777,0.924189890634277),
(0.,1.),.UNSPECIFIED.)
GEOMETRIC_REPRESENTATION_ITEM()
RATIONAL_B_SPLINE_SURFACE(((1.,0.999906054677511,0.999906054677511,1.),
(1.,0.999906054677511,0.999906054677511,1.),(1.,0.999906054677511,0.999906054677511,
1.),(1.,0.999906054677511,0.999906054677511,1.)))
REPRESENTATION_ITEM('')
SURFACE()
);
#1709=(
BOUNDED_SURFACE()
B_SPLINE_SURFACE(3,3,((#129201,#129202,#129203,#129204),(#129205,#129206,
#129207,#129208),(#129209,#129210,#129211,#129212),(#129213,#129214,#129215,
#129216)),.UNSPECIFIED.,.F.,.F.,.F.)
B_SPLINE_SURFACE_WITH_KNOTS((4,4),(4,4),(0.320639964684793,0.371314507617759),
(0.,1.),.UNSPECIFIED.)
GEOMETRIC_REPRESENTATION_ITEM()
RATIONAL_B_SPLINE_SURFACE(((1.,0.999967350702174,0.999967350702174,1.),
(1.,0.999967350702174,0.999967350702174,1.),(1.,0.999967350702174,0.999967350702174,
1.),(1.,0.999967350702174,0.999967350702174,1.)))
REPRESENTATION_ITEM('')
SURFACE()
);
#1710=(
BOUNDED_SURFACE()
B_SPLINE_SURFACE(3,3,((#129218,#129219,#129220,#129221),(#129222,#129223,
#129224,#129225),(#129226,#129227,#129228,#129229),(#129230,#129231,#129232,
#129233)),.UNSPECIFIED.,.F.,.F.,.F.)
B_SPLINE_SURFACE_WITH_KNOTS((4,4),(4,4),(0.485088192372813,0.537796433966225),
(0.,1.),.UNSPECIFIED.)
GEOMETRIC_REPRESENTATION_ITEM()
RATIONAL_B_SPLINE_SURFACE(((1.,0.999962120409815,0.999962120409815,1.),
(1.,0.999962120409815,0.999962120409815,1.),(1.,0.999962120409815,0.999962120409815,
1.),(1.,0.999962120409815,0.999962120409815,1.)))
REPRESENTATION_ITEM('')
SURFACE()
);
#1711=(
BOUNDED_SURFACE()
B_SPLINE_SURFACE(3,3,((#129235,#129236,#129237,#129238),(#129239,#129240,
#129241,#129242),(#129243,#129244,#129245,#129246),(#129247,#129248,#129249,
#129250)),.UNSPECIFIED.,.F.,.F.,.F.)
B_SPLINE_SURFACE_WITH_KNOTS((4,4),(4,4),(0.675478450031988,0.739029557635334),
(0.,1.),.UNSPECIFIED.)
GEOMETRIC_REPRESENTATION_ITEM()
RATIONAL_B_SPLINE_SURFACE(((1.,0.999940036715462,0.999940036715462,1.),
(1.,0.999940036715462,0.999940036715462,1.),(1.,0.999940036715462,0.999940036715462,
1.),(1.,0.999940036715462,0.999940036715462,1.)))
REPRESENTATION_ITEM('')
SURFACE()
);
#1712=(
BOUNDED_SURFACE()
B_SPLINE_SURFACE(3,3,((#129252,#129253,#129254,#129255),(#129256,#129257,
#129258,#129259),(#129260,#129261,#129262,#129263),(#129264,#129265,#129266,
#129267)),.UNSPECIFIED.,.F.,.F.,.F.)
B_SPLINE_SURFACE_WITH_KNOTS((4,4),(4,4),(0.847977146575099,0.924247070973153),
(0.,1.),.UNSPECIFIED.)
GEOMETRIC_REPRESENTATION_ITEM()
RATIONAL_B_SPLINE_SURFACE(((1.,0.9999062633542,0.9999062633542,1.),(1.,
0.9999062633542,0.9999062633542,1.),(1.,0.9999062633542,0.9999062633542,
1.),(1.,0.9999062633542,0.9999062633542,1.)))
REPRESENTATION_ITEM('')
SURFACE()
);
#1713=(
BOUNDED_SURFACE()
B_SPLINE_SURFACE(3,3,((#129269,#129270,#129271,#129272),(#129273,#129274,
#129275,#129276),(#129277,#129278,#129279,#129280),(#129281,#129282,#129283,
#129284)),.UNSPECIFIED.,.F.,.F.,.F.)
B_SPLINE_SURFACE_WITH_KNOTS((4,4),(4,4),(0.320583334123496,0.371380663507137),
(0.,1.),.UNSPECIFIED.)
GEOMETRIC_REPRESENTATION_ITEM()
RATIONAL_B_SPLINE_SURFACE(((1.,0.99996730938274,0.99996730938274,1.),(1.,
0.99996730938274,0.99996730938274,1.),(1.,0.99996730938274,0.99996730938274,
1.),(1.,0.99996730938274,0.99996730938274,1.)))
REPRESENTATION_ITEM('')
SURFACE()
);
#1714=(
BOUNDED_SURFACE()
B_SPLINE_SURFACE(3,3,((#129286,#129287,#129288,#129289),(#129290,#129291,
#129292,#129293),(#129294,#129295,#129296,#129297),(#129298,#129299,#129300,
#129301)),.UNSPECIFIED.,.F.,.F.,.F.)
B_SPLINE_SURFACE_WITH_KNOTS((4,4),(4,4),(0.485126102700377,0.537860300944991),
(0.,1.),.UNSPECIFIED.)
GEOMETRIC_REPRESENTATION_ITEM()
RATIONAL_B_SPLINE_SURFACE(((1.,0.999962137299808,0.999962137299808,1.),
(1.,0.999962137299808,0.999962137299808,1.),(1.,0.999962137299808,0.999962137299808,
1.),(1.,0.999962137299808,0.999962137299808,1.)))
REPRESENTATION_ITEM('')
SURFACE()
);
#1715=(
BOUNDED_SURFACE()
B_SPLINE_SURFACE(3,3,((#129303,#129304,#129305,#129306),(#129307,#129308,
#129309,#129310),(#129311,#129312,#129313,#129314),(#129315,#129316,#129317,
#129318)),.UNSPECIFIED.,.F.,.F.,.F.)
B_SPLINE_SURFACE_WITH_KNOTS((4,4),(4,4),(0.675620555481706,0.738956525898373),
(0.,1.),.UNSPECIFIED.)
GEOMETRIC_REPRESENTATION_ITEM()
RATIONAL_B_SPLINE_SURFACE(((1.,0.999940072974474,0.999940072974474,1.),
(1.,0.999940072974474,0.999940072974474,1.),(1.,0.999940072974474,0.999940072974474,
1.),(1.,0.999940072974474,0.999940072974474,1.)))
REPRESENTATION_ITEM('')
SURFACE()
);
#1716=(
BOUNDED_SURFACE()
B_SPLINE_SURFACE(3,3,((#129320,#129321,#129322,#129323),(#129324,#129325,
#129326,#129327),(#129328,#129329,#129330,#129331),(#129332,#129333,#129334,
#129335)),.UNSPECIFIED.,.F.,.F.,.F.)
B_SPLINE_SURFACE_WITH_KNOTS((4,4),(4,4),(0.84799244392776,0.924142505922786),
(0.,1.),.UNSPECIFIED.)
GEOMETRIC_REPRESENTATION_ITEM()
RATIONAL_B_SPLINE_SURFACE(((1.,0.999906153501141,0.999906153501141,1.),
(1.,0.999906153501141,0.999906153501141,1.),(1.,0.999906153501141,0.999906153501141,
1.),(1.,0.999906153501141,0.999906153501141,1.)))
REPRESENTATION_ITEM('')
SURFACE()
);
#1717=(
BOUNDED_SURFACE()
B_SPLINE_SURFACE(3,3,((#129337,#129338,#129339,#129340),(#129341,#129342,
#129343,#129344),(#129345,#129346,#129347,#129348),(#129349,#129350,#129351,
#129352)),.UNSPECIFIED.,.F.,.F.,.F.)
B_SPLINE_SURFACE_WITH_KNOTS((4,4),(4,4),(0.320518100436019,0.371362835533565),
(0.,1.),.UNSPECIFIED.)
GEOMETRIC_REPRESENTATION_ITEM()
RATIONAL_B_SPLINE_SURFACE(((1.,0.999967298407033,0.999967298407033,1.),
(1.,0.999967298407033,0.999967298407033,1.),(1.,0.999967298407033,0.999967298407033,
1.),(1.,0.999967298407033,0.999967298407033,1.)))
REPRESENTATION_ITEM('')
SURFACE()
);
#1718=(
BOUNDED_SURFACE()
B_SPLINE_SURFACE(3,3,((#129354,#129355,#129356,#129357),(#129358,#129359,
#129360,#129361),(#129362,#129363,#129364,#129365),(#129366,#129367,#129368,
#129369)),.UNSPECIFIED.,.F.,.F.,.F.)
B_SPLINE_SURFACE_WITH_KNOTS((4,4),(4,4),(0.485111695336929,0.537875420193652),
(0.,1.),.UNSPECIFIED.)
GEOMETRIC_REPRESENTATION_ITEM()
RATIONAL_B_SPLINE_SURFACE(((1.,0.999962111917502,0.999962111917502,1.),
(1.,0.999962111917502,0.999962111917502,1.),(1.,0.999962111917502,0.999962111917502,
1.),(1.,0.999962111917502,0.999962111917502,1.)))
REPRESENTATION_ITEM('')
SURFACE()
);
#1719=(
BOUNDED_SURFACE()
B_SPLINE_SURFACE(3,3,((#129371,#129372,#129373,#129374),(#129375,#129376,
#129377,#129378),(#129379,#129380,#129381,#129382),(#129383,#129384,#129385,
#129386)),.UNSPECIFIED.,.F.,.F.,.F.)
B_SPLINE_SURFACE_WITH_KNOTS((4,4),(4,4),(0.67554330969252,0.739050792335592),
(0.,1.),.UNSPECIFIED.)
GEOMETRIC_REPRESENTATION_ITEM()
RATIONAL_B_SPLINE_SURFACE(((1.,0.999940183216014,0.999940183216014,1.),
(1.,0.999940183216014,0.999940183216014,1.),(1.,0.999940183216014,0.999940183216014,
1.),(1.,0.999940183216014,0.999940183216014,1.)))
REPRESENTATION_ITEM('')
SURFACE()
);
#1720=(
BOUNDED_SURFACE()
B_SPLINE_SURFACE(3,3,((#129388,#129389,#129390,#129391),(#129392,#129393,
#129394,#129395),(#129396,#129397,#129398,#129399),(#129400,#129401,#129402,
#129403)),.UNSPECIFIED.,.F.,.F.,.F.)
B_SPLINE_SURFACE_WITH_KNOTS((4,4),(4,4),(0.848082295900864,0.924212909944339),
(0.,1.),.UNSPECIFIED.)
GEOMETRIC_REPRESENTATION_ITEM()
RATIONAL_B_SPLINE_SURFACE(((1.,0.999906015094081,0.999906015094081,1.),
(1.,0.999906015094081,0.999906015094081,1.),(1.,0.999906015094081,0.999906015094081,
1.),(1.,0.999906015094081,0.999906015094081,1.)))
REPRESENTATION_ITEM('')
SURFACE()
);
#1721=(
BOUNDED_SURFACE()
B_SPLINE_SURFACE(3,3,((#129405,#129406,#129407,#129408),(#129409,#129410,
#129411,#129412),(#129413,#129414,#129415,#129416),(#129417,#129418,#129419,
#129420)),.UNSPECIFIED.,.F.,.F.,.F.)
B_SPLINE_SURFACE_WITH_KNOTS((4,4),(4,4),(0.320600960423681,0.371411458072819),
(0.,1.),.UNSPECIFIED.)
GEOMETRIC_REPRESENTATION_ITEM()
RATIONAL_B_SPLINE_SURFACE(((1.,0.999967243891018,0.999967243891018,1.),
(1.,0.999967243891018,0.999967243891018,1.),(1.,0.999967243891018,0.999967243891018,
1.),(1.,0.999967243891018,0.999967243891018,1.)))
REPRESENTATION_ITEM('')
SURFACE()
);
#1722=(
BOUNDED_SURFACE()
B_SPLINE_SURFACE(3,3,((#129422,#129423,#129424,#129425),(#129426,#129427,
#129428,#129429),(#129430,#129431,#129432,#129433),(#129434,#129435,#129436,
#129437)),.UNSPECIFIED.,.F.,.F.,.F.)
B_SPLINE_SURFACE_WITH_KNOTS((4,4),(4,4),(0.48504256867854,0.537887934754555),
(0.,1.),.UNSPECIFIED.)
GEOMETRIC_REPRESENTATION_ITEM()
RATIONAL_B_SPLINE_SURFACE(((1.,0.999962231855016,0.999962231855016,1.),
(1.,0.999962231855016,0.999962231855016,1.),(1.,0.999962231855016,0.999962231855016,
1.),(1.,0.999962231855016,0.999962231855016,1.)))
REPRESENTATION_ITEM('')
SURFACE()
);
#1723=(
BOUNDED_SURFACE()
B_SPLINE_SURFACE(3,3,((#129439,#129440,#129441,#129442),(#129443,#129444,
#129445,#129446),(#129447,#129448,#129449,#129450),(#129451,#129452,#129453,
#129454)),.UNSPECIFIED.,.F.,.F.,.F.)
B_SPLINE_SURFACE_WITH_KNOTS((4,4),(4,4),(0.675450724081424,0.73897092350891),
(0.,1.),.UNSPECIFIED.)
GEOMETRIC_REPRESENTATION_ITEM()
RATIONAL_B_SPLINE_SURFACE(((1.,0.99994009649207,0.99994009649207,1.),(1.,
0.99994009649207,0.99994009649207,1.),(1.,0.99994009649207,0.99994009649207,
1.),(1.,0.99994009649207,0.99994009649207,1.)))
REPRESENTATION_ITEM('')
SURFACE()
);
#1724=(
BOUNDED_SURFACE()
B_SPLINE_SURFACE(3,3,((#129456,#129457,#129458,#129459),(#129460,#129461,
#129462,#129463),(#129464,#129465,#129466,#129467),(#129468,#129469,#129470,
#129471)),.UNSPECIFIED.,.F.,.F.,.F.)
B_SPLINE_SURFACE_WITH_KNOTS((4,4),(4,4),(0.848090733102027,0.924284397580542),
(0.,1.),.UNSPECIFIED.)
GEOMETRIC_REPRESENTATION_ITEM()
RATIONAL_B_SPLINE_SURFACE(((1.,0.999905868674041,0.999905868674041,1.),
(1.,0.999905868674041,0.999905868674041,1.),(1.,0.999905868674041,0.999905868674041,
1.),(1.,0.999905868674041,0.999905868674041,1.)))
REPRESENTATION_ITEM('')
SURFACE()
);
#1725=(
BOUNDED_SURFACE()
B_SPLINE_SURFACE(3,3,((#129473,#129474,#129475,#129476),(#129477,#129478,
#129479,#129480),(#129481,#129482,#129483,#129484),(#129485,#129486,#129487,
#129488)),.UNSPECIFIED.,.F.,.F.,.F.)
B_SPLINE_SURFACE_WITH_KNOTS((4,4),(4,4),(0.320500281417297,0.37141920772819),
(0.,1.),.UNSPECIFIED.)
GEOMETRIC_REPRESENTATION_ITEM()
RATIONAL_B_SPLINE_SURFACE(((1.,0.999967398958956,0.999967398958956,1.),
(1.,0.999967398958956,0.999967398958956,1.),(1.,0.999967398958956,0.999967398958956,
1.),(1.,0.999967398958956,0.999967398958956,1.)))
REPRESENTATION_ITEM('')
SURFACE()
);
#1726=(
BOUNDED_SURFACE()
B_SPLINE_SURFACE(3,3,((#129490,#129491,#129492,#129493),(#129494,#129495,
#129496,#129497),(#129498,#129499,#129500,#129501),(#129502,#129503,#129504,
#129505)),.UNSPECIFIED.,.F.,.F.,.F.)
B_SPLINE_SURFACE_WITH_KNOTS((4,4),(4,4),(0.485039113478553,0.537770836541586),
(0.,1.),.UNSPECIFIED.)
GEOMETRIC_REPRESENTATION_ITEM()
RATIONAL_B_SPLINE_SURFACE(((1.,0.999962216400084,0.999962216400084,1.),
(1.,0.999962216400084,0.999962216400084,1.),(1.,0.999962216400084,0.999962216400084,
1.),(1.,0.999962216400084,0.999962216400084,1.)))
REPRESENTATION_ITEM('')
SURFACE()
);
#1727=(
BOUNDED_SURFACE()
B_SPLINE_SURFACE(3,3,((#129507,#129508,#129509,#129510),(#129511,#129512,
#129513,#129514),(#129515,#129516,#129517,#129518),(#129519,#129520,#129521,
#129522)),.UNSPECIFIED.,.F.,.F.,.F.)
B_SPLINE_SURFACE_WITH_KNOTS((4,4),(4,4),(0.675616885244456,0.739079678101414),
(0.,1.),.UNSPECIFIED.)
GEOMETRIC_REPRESENTATION_ITEM()
RATIONAL_B_SPLINE_SURFACE(((1.,0.999939908563371,0.999939908563371,1.),
(1.,0.999939908563371,0.999939908563371,1.),(1.,0.999939908563371,0.999939908563371,
1.),(1.,0.999939908563371,0.999939908563371,1.)))
REPRESENTATION_ITEM('')
SURFACE()
);
#1728=(
BOUNDED_SURFACE()
B_SPLINE_SURFACE(3,3,((#129524,#129525,#129526,#129527),(#129528,#129529,
#129530,#129531),(#129532,#129533,#129534,#129535),(#129536,#129537,#129538,
#129539)),.UNSPECIFIED.,.F.,.F.,.F.)
B_SPLINE_SURFACE_WITH_KNOTS((4,4),(4,4),(0.847942523738152,0.924296420006828),
(0.,1.),.UNSPECIFIED.)
GEOMETRIC_REPRESENTATION_ITEM()
RATIONAL_B_SPLINE_SURFACE(((1.,0.999906356251184,0.999906356251184,1.),
(1.,0.999906356251184,0.999906356251184,1.),(1.,0.999906356251184,0.999906356251184,
1.),(1.,0.999906356251184,0.999906356251184,1.)))
REPRESENTATION_ITEM('')
SURFACE()
);
#1729=(
BOUNDED_SURFACE()
B_SPLINE_SURFACE(3,3,((#129541,#129542,#129543,#129544),(#129545,#129546,
#129547,#129548),(#129549,#129550,#129551,#129552),(#129553,#129554,#129555,
#129556)),.UNSPECIFIED.,.F.,.F.,.F.)
B_SPLINE_SURFACE_WITH_KNOTS((4,4),(4,4),(0.320503220290746,0.371278341845292),
(0.,1.),.UNSPECIFIED.)
GEOMETRIC_REPRESENTATION_ITEM()
RATIONAL_B_SPLINE_SURFACE(((1.,0.999967413248699,0.999967413248699,1.),
(1.,0.999967413248699,0.999967413248699,1.),(1.,0.999967413248699,0.999967413248699,
1.),(1.,0.999967413248699,0.999967413248699,1.)))
REPRESENTATION_ITEM('')
SURFACE()
);
#1730=(
BOUNDED_SURFACE()
B_SPLINE_SURFACE(3,3,((#129558,#129559,#129560,#129561),(#129562,#129563,
#129564,#129565),(#129566,#129567,#129568,#129569),(#129570,#129571,#129572,
#129573)),.UNSPECIFIED.,.F.,.F.,.F.)
B_SPLINE_SURFACE_WITH_KNOTS((4,4),(4,4),(0.485167461585208,0.537898795794421),
(0.,1.),.UNSPECIFIED.)
GEOMETRIC_REPRESENTATION_ITEM()
RATIONAL_B_SPLINE_SURFACE(((1.,0.999962048910248,0.999962048910248,1.),
(1.,0.999962048910248,0.999962048910248,1.),(1.,0.999962048910248,0.999962048910248,
1.),(1.,0.999962048910248,0.999962048910248,1.)))
REPRESENTATION_ITEM('')
SURFACE()
);
#1731=(
BOUNDED_SURFACE()
B_SPLINE_SURFACE(3,3,((#129575,#129576,#129577,#129578),(#129579,#129580,
#129581,#129582),(#129583,#129584,#129585,#129586),(#129587,#129588,#129589,
#129590)),.UNSPECIFIED.,.F.,.F.,.F.)
B_SPLINE_SURFACE_WITH_KNOTS((4,4),(4,4),(0.675444558331159,0.739082790885492),
(0.,1.),.UNSPECIFIED.)
GEOMETRIC_REPRESENTATION_ITEM()
RATIONAL_B_SPLINE_SURFACE(((1.,0.999940167892219,0.999940167892219,1.),
(1.,0.999940167892219,0.999940167892219,1.),(1.,0.999940167892219,0.999940167892219,
1.),(1.,0.999940167892219,0.999940167892219,1.)))
REPRESENTATION_ITEM('')
SURFACE()
);
#1732=(
BOUNDED_SURFACE()
B_SPLINE_SURFACE(3,3,((#129592,#129593,#129594,#129595),(#129596,#129597,
#129598,#129599),(#129600,#129601,#129602,#129603),(#129604,#129605,#129606,
#129607)),.UNSPECIFIED.,.F.,.F.,.F.)
B_SPLINE_SURFACE_WITH_KNOTS((4,4),(4,4),(0.847944615083763,0.924067134683459),
(0.,1.),.UNSPECIFIED.)
GEOMETRIC_REPRESENTATION_ITEM()
RATIONAL_B_SPLINE_SURFACE(((1.,0.999906379098947,0.999906379098947,1.),
(1.,0.999906379098947,0.999906379098947,1.),(1.,0.999906379098947,0.999906379098947,
1.),(1.,0.999906379098947,0.999906379098947,1.)))
REPRESENTATION_ITEM('')
SURFACE()
);
#1733=(
BOUNDED_SURFACE()
B_SPLINE_SURFACE(3,3,((#129609,#129610,#129611,#129612),(#129613,#129614,
#129615,#129616),(#129617,#129618,#129619,#129620),(#129621,#129622,#129623,
#129624)),.UNSPECIFIED.,.F.,.F.,.F.)
B_SPLINE_SURFACE_WITH_KNOTS((4,4),(4,4),(0.320579981379885,0.371413971104649),
(0.,1.),.UNSPECIFIED.)
GEOMETRIC_REPRESENTATION_ITEM()
RATIONAL_B_SPLINE_SURFACE(((1.,0.999967229881466,0.999967229881466,1.),
(1.,0.999967229881466,0.999967229881466,1.),(1.,0.999967229881466,0.999967229881466,
1.),(1.,0.999967229881466,0.999967229881466,1.)))
REPRESENTATION_ITEM('')
SURFACE()
);
#1734=(
BOUNDED_SURFACE()
B_SPLINE_SURFACE(3,3,((#129626,#129627,#129628,#129629),(#129630,#129631,
#129632,#129633),(#129634,#129635,#129636,#129637),(#129638,#129639,#129640,
#129641)),.UNSPECIFIED.,.F.,.F.,.F.)
B_SPLINE_SURFACE_WITH_KNOTS((4,4),(4,4),(0.485048076032685,0.537894489611572),
(0.,1.),.UNSPECIFIED.)
GEOMETRIC_REPRESENTATION_ITEM()
RATIONAL_B_SPLINE_SURFACE(((1.,0.999962180624942,0.999962180624942,1.),
(1.,0.999962180624942,0.999962180624942,1.),(1.,0.999962180624942,0.999962180624942,
1.),(1.,0.999962180624942,0.999962180624942,1.)))
REPRESENTATION_ITEM('')
SURFACE()
);
#1735=(
BOUNDED_SURFACE()
B_SPLINE_SURFACE(3,3,((#129643,#129644,#129645,#129646),(#129647,#129648,
#129649,#129650),(#129651,#129652,#129653,#129654),(#129655,#129656,#129657,
#129658)),.UNSPECIFIED.,.F.,.F.,.F.)
B_SPLINE_SURFACE_WITH_KNOTS((4,4),(4,4),(0.675453398131279,0.738944677678275),
(0.,1.),.UNSPECIFIED.)
GEOMETRIC_REPRESENTATION_ITEM()
RATIONAL_B_SPLINE_SURFACE(((1.,0.9999402244459,0.9999402244459,1.),(1.,
0.9999402244459,0.9999402244459,1.),(1.,0.9999402244459,0.9999402244459,
1.),(1.,0.9999402244459,0.9999402244459,1.)))
REPRESENTATION_ITEM('')
SURFACE()
);
#1736=(
BOUNDED_SURFACE()
B_SPLINE_SURFACE(3,3,((#129660,#129661,#129662,#129663),(#129664,#129665,
#129666,#129667),(#129668,#129669,#129670,#129671),(#129672,#129673,#129674,
#129675)),.UNSPECIFIED.,.F.,.F.,.F.)
B_SPLINE_SURFACE_WITH_KNOTS((4,4),(4,4),(0.848081923661779,0.924293307560431),
(0.,1.),.UNSPECIFIED.)
GEOMETRIC_REPRESENTATION_ITEM()
RATIONAL_B_SPLINE_SURFACE(((1.,0.999905876932681,0.999905876932681,1.),
(1.,0.999905876932681,0.999905876932681,1.),(1.,0.999905876932681,0.999905876932681,
1.),(1.,0.999905876932681,0.999905876932681,1.)))
REPRESENTATION_ITEM('')
SURFACE()
);
#1737=(
BOUNDED_SURFACE()
B_SPLINE_SURFACE(3,3,((#129677,#129678,#129679,#129680),(#129681,#129682,
#129683,#129684),(#129685,#129686,#129687,#129688),(#129689,#129690,#129691,
#129692)),.UNSPECIFIED.,.F.,.F.,.F.)
B_SPLINE_SURFACE_WITH_KNOTS((4,4),(4,4),(0.320532095739598,0.371399682963038),
(0.,1.),.UNSPECIFIED.)
GEOMETRIC_REPRESENTATION_ITEM()
RATIONAL_B_SPLINE_SURFACE(((1.,0.999967407141921,0.999967407141921,1.),
(1.,0.999967407141921,0.999967407141921,1.),(1.,0.999967407141921,0.999967407141921,
1.),(1.,0.999967407141921,0.999967407141921,1.)))
REPRESENTATION_ITEM('')
SURFACE()
);
#1738=(
BOUNDED_SURFACE()
B_SPLINE_SURFACE(3,3,((#129694,#129695,#129696,#129697),(#129698,#129699,
#129700,#129701),(#129702,#129703,#129704,#129705),(#129706,#129707,#129708,
#129709)),.UNSPECIFIED.,.F.,.F.,.F.)
B_SPLINE_SURFACE_WITH_KNOTS((4,4),(4,4),(0.485063242836078,0.537827571850851),
(0.,1.),.UNSPECIFIED.)
GEOMETRIC_REPRESENTATION_ITEM()
RATIONAL_B_SPLINE_SURFACE(((1.,0.999962210107628,0.999962210107628,1.),
(1.,0.999962210107628,0.999962210107628,1.),(1.,0.999962210107628,0.999962210107628,
1.),(1.,0.999962210107628,0.999962210107628,1.)))
REPRESENTATION_ITEM('')
SURFACE()
);
#1739=(
BOUNDED_SURFACE()
B_SPLINE_SURFACE(3,3,((#129711,#129712,#129713,#129714),(#129715,#129716,
#129717,#129718),(#129719,#129720,#129721,#129722),(#129723,#129724,#129725,
#129726)),.UNSPECIFIED.,.F.,.F.,.F.)
B_SPLINE_SURFACE_WITH_KNOTS((4,4),(4,4),(0.675517041172354,0.739061923565337),
(0.,1.),.UNSPECIFIED.)
GEOMETRIC_REPRESENTATION_ITEM()
RATIONAL_B_SPLINE_SURFACE(((1.,0.999940001666099,0.999940001666099,1.),
(1.,0.999940001666099,0.999940001666099,1.),(1.,0.999940001666099,0.999940001666099,
1.),(1.,0.999940001666099,0.999940001666099,1.)))
REPRESENTATION_ITEM('')
SURFACE()
);
#1740=(
BOUNDED_SURFACE()
B_SPLINE_SURFACE(3,3,((#129728,#129729,#129730,#129731),(#129732,#129733,
#129734,#129735),(#129736,#129737,#129738,#129739),(#129740,#129741,#129742,
#129743)),.UNSPECIFIED.,.F.,.F.,.F.)
B_SPLINE_SURFACE_WITH_KNOTS((4,4),(4,4),(0.847973179754561,0.924280871374564),
(0.,1.),.UNSPECIFIED.)
GEOMETRIC_REPRESENTATION_ITEM()
RATIONAL_B_SPLINE_SURFACE(((1.,0.999906008444178,0.999906008444178,1.),
(1.,0.999906008444178,0.999906008444178,1.),(1.,0.999906008444178,0.999906008444178,
1.),(1.,0.999906008444178,0.999906008444178,1.)))
REPRESENTATION_ITEM('')
SURFACE()
);
#1741=(
BOUNDED_SURFACE()
B_SPLINE_SURFACE(3,3,((#129745,#129746,#129747,#129748),(#129749,#129750,
#129751,#129752),(#129753,#129754,#129755,#129756),(#129757,#129758,#129759,
#129760)),.UNSPECIFIED.,.F.,.F.,.F.)
B_SPLINE_SURFACE_WITH_KNOTS((4,4),(4,4),(0.320557075856707,0.371389535077562),
(0.,1.),.UNSPECIFIED.)
GEOMETRIC_REPRESENTATION_ITEM()
RATIONAL_B_SPLINE_SURFACE(((1.,0.999967354745893,0.999967354745893,1.),
(1.,0.999967354745893,0.999967354745893,1.),(1.,0.999967354745893,0.999967354745893,
1.),(1.,0.999967354745893,0.999967354745893,1.)))
REPRESENTATION_ITEM('')
SURFACE()
);
#1742=(
BOUNDED_SURFACE()
B_SPLINE_SURFACE(3,3,((#129762,#129763,#129764,#129765),(#129766,#129767,
#129768,#129769),(#129770,#129771,#129772,#129773),(#129774,#129775,#129776,
#129777)),.UNSPECIFIED.,.F.,.F.,.F.)
B_SPLINE_SURFACE_WITH_KNOTS((4,4),(4,4),(0.485068338493211,0.537857806791834),
(0.,1.),.UNSPECIFIED.)
GEOMETRIC_REPRESENTATION_ITEM()
RATIONAL_B_SPLINE_SURFACE(((1.,0.999962427563455,0.999962427563455,1.),
(1.,0.999962427563455,0.999962427563455,1.),(1.,0.999962427563455,0.999962427563455,
1.),(1.,0.999962427563455,0.999962427563455,1.)))
REPRESENTATION_ITEM('')
SURFACE()
);
#1743=(
BOUNDED_SURFACE()
B_SPLINE_SURFACE(3,3,((#129779,#129780,#129781,#129782),(#129783,#129784,
#129785,#129786),(#129787,#129788,#129789,#129790),(#129791,#129792,#129793,
#129794)),.UNSPECIFIED.,.F.,.F.,.F.)
B_SPLINE_SURFACE_WITH_KNOTS((4,4),(4,4),(0.675489981246965,0.739042440925566),
(0.,1.),.UNSPECIFIED.)
GEOMETRIC_REPRESENTATION_ITEM()
RATIONAL_B_SPLINE_SURFACE(((1.,0.999940192796421,0.999940192796421,1.),
(1.,0.999940192796421,0.999940192796421,1.),(1.,0.999940192796421,0.999940192796421,
1.),(1.,0.999940192796421,0.999940192796421,1.)))
REPRESENTATION_ITEM('')
SURFACE()
);
#1744=(
BOUNDED_SURFACE()
B_SPLINE_SURFACE(3,3,((#129796,#129797,#129798,#129799),(#129800,#129801,
#129802,#129803),(#129804,#129805,#129806,#129807),(#129808,#129809,#129810,
#129811)),.UNSPECIFIED.,.F.,.F.,.F.)
B_SPLINE_SURFACE_WITH_KNOTS((4,4),(4,4),(0.847997664137825,0.924222883197149),
(0.,1.),.UNSPECIFIED.)
GEOMETRIC_REPRESENTATION_ITEM()
RATIONAL_B_SPLINE_SURFACE(((1.,0.999906130607457,0.999906130607457,1.),
(1.,0.999906130607457,0.999906130607457,1.),(1.,0.999906130607457,0.999906130607457,
1.),(1.,0.999906130607457,0.999906130607457,1.)))
REPRESENTATION_ITEM('')
SURFACE()
);
#1745=(
BOUNDED_SURFACE()
B_SPLINE_SURFACE(3,3,((#129813,#129814,#129815,#129816),(#129817,#129818,
#129819,#129820),(#129821,#129822,#129823,#129824),(#129825,#129826,#129827,
#129828)),.UNSPECIFIED.,.F.,.F.,.F.)
B_SPLINE_SURFACE_WITH_KNOTS((4,4),(4,4),(0.320507814263771,0.371406373023686),
(0.,1.),.UNSPECIFIED.)
GEOMETRIC_REPRESENTATION_ITEM()
RATIONAL_B_SPLINE_SURFACE(((1.,0.999967375144329,0.999967375144329,1.),
(1.,0.999967375144329,0.999967375144329,1.),(1.,0.999967375144329,0.999967375144329,
1.),(1.,0.999967375144329,0.999967375144329,1.)))
REPRESENTATION_ITEM('')
SURFACE()
);
#1746=(
BOUNDED_SURFACE()
B_SPLINE_SURFACE(3,3,((#129830,#129831,#129832,#129833),(#129834,#129835,
#129836,#129837),(#129838,#129839,#129840,#129841),(#129842,#129843,#129844,
#129845)),.UNSPECIFIED.,.F.,.F.,.F.)
B_SPLINE_SURFACE_WITH_KNOTS((4,4),(4,4),(0.485052737431369,0.53783191570572),
(0.,1.),.UNSPECIFIED.)
GEOMETRIC_REPRESENTATION_ITEM()
RATIONAL_B_SPLINE_SURFACE(((1.,0.999962226594182,0.999962226594182,1.),
(1.,0.999962226594182,0.999962226594182,1.),(1.,0.999962226594182,0.999962226594182,
1.),(1.,0.999962226594182,0.999962226594182,1.)))
REPRESENTATION_ITEM('')
SURFACE()
);
#1747=(
BOUNDED_SURFACE()
B_SPLINE_SURFACE(3,3,((#129847,#129848,#129849,#129850),(#129851,#129852,
#129853,#129854),(#129855,#129856,#129857,#129858),(#129859,#129860,#129861,
#129862)),.UNSPECIFIED.,.F.,.F.,.F.)
B_SPLINE_SURFACE_WITH_KNOTS((4,4),(4,4),(0.675526759490361,0.739051034903929),
(0.,1.),.UNSPECIFIED.)
GEOMETRIC_REPRESENTATION_ITEM()
RATIONAL_B_SPLINE_SURFACE(((1.,0.999940214293996,0.999940214293996,1.),
(1.,0.999940214293996,0.999940214293996,1.),(1.,0.999940214293996,0.999940214293996,
1.),(1.,0.999940214293996,0.999940214293996,1.)))
REPRESENTATION_ITEM('')
SURFACE()
);
#1748=(
BOUNDED_SURFACE()
B_SPLINE_SURFACE(3,3,((#129864,#129865,#129866,#129867),(#129868,#129869,
#129870,#129871),(#129872,#129873,#129874,#129875),(#129876,#129877,#129878,
#129879)),.UNSPECIFIED.,.F.,.F.,.F.)
B_SPLINE_SURFACE_WITH_KNOTS((4,4),(4,4),(0.847972351420996,0.924252627795196),
(0.,1.),.UNSPECIFIED.)
GEOMETRIC_REPRESENTATION_ITEM()
RATIONAL_B_SPLINE_SURFACE(((1.,0.999906726046663,0.999906726046663,1.),
(1.,0.999906726046663,0.999906726046663,1.),(1.,0.999906726046663,0.999906726046663,
1.),(1.,0.999906726046663,0.999906726046663,1.)))
REPRESENTATION_ITEM('')
SURFACE()
);
#1749=(
BOUNDED_SURFACE()
B_SPLINE_SURFACE(3,3,((#129881,#129882,#129883,#129884),(#129885,#129886,
#129887,#129888),(#129889,#129890,#129891,#129892),(#129893,#129894,#129895,
#129896)),.UNSPECIFIED.,.F.,.F.,.F.)
B_SPLINE_SURFACE_WITH_KNOTS((4,4),(4,4),(0.320502655600432,0.371307521287429),
(0.,1.),.UNSPECIFIED.)
GEOMETRIC_REPRESENTATION_ITEM()
RATIONAL_B_SPLINE_SURFACE(((1.,0.999967242859915,0.999967242859915,1.),
(1.,0.999967242859915,0.999967242859915,1.),(1.,0.999967242859915,0.999967242859915,
1.),(1.,0.999967242859915,0.999967242859915,1.)))
REPRESENTATION_ITEM('')
SURFACE()
);
#1750=(
BOUNDED_SURFACE()
B_SPLINE_SURFACE(3,3,((#129898,#129899,#129900,#129901),(#129902,#129903,
#129904,#129905),(#129906,#129907,#129908,#129909),(#129910,#129911,#129912,
#129913)),.UNSPECIFIED.,.F.,.F.,.F.)
B_SPLINE_SURFACE_WITH_KNOTS((4,4),(4,4),(0.485155008733541,0.537892550151409),
(0.,1.),.UNSPECIFIED.)
GEOMETRIC_REPRESENTATION_ITEM()
RATIONAL_B_SPLINE_SURFACE(((1.,0.999962141529141,0.999962141529141,1.),
(1.,0.999962141529141,0.999962141529141,1.),(1.,0.999962141529141,0.999962141529141,
1.),(1.,0.999962141529141,0.999962141529141,1.)))
REPRESENTATION_ITEM('')
SURFACE()
);
#1751=(
BOUNDED_SURFACE()
B_SPLINE_SURFACE(3,3,((#129915,#129916,#129917,#129918),(#129919,#129920,
#129921,#129922),(#129923,#129924,#129925,#129926),(#129927,#129928,#129929,
#129930)),.UNSPECIFIED.,.F.,.F.,.F.)
B_SPLINE_SURFACE_WITH_KNOTS((4,4),(4,4),(0.675449354058364,0.739068188298896),
(0.,1.),.UNSPECIFIED.)
GEOMETRIC_REPRESENTATION_ITEM()
RATIONAL_B_SPLINE_SURFACE(((1.,0.999940252055417,0.999940252055417,1.),
(1.,0.999940252055417,0.999940252055417,1.),(1.,0.999940252055417,0.999940252055417,
1.),(1.,0.999940252055417,0.999940252055417,1.)))
REPRESENTATION_ITEM('')
SURFACE()
);
#1752=(
BOUNDED_SURFACE()
B_SPLINE_SURFACE(3,3,((#129932,#129933,#129934,#129935),(#129936,#129937,
#129938,#129939),(#129940,#129941,#129942,#129943),(#129944,#129945,#129946,
#129947)),.UNSPECIFIED.,.F.,.F.,.F.)
B_SPLINE_SURFACE_WITH_KNOTS((4,4),(4,4),(0.847955892602436,0.924180945781555),
(0.,1.),.UNSPECIFIED.)
GEOMETRIC_REPRESENTATION_ITEM()
RATIONAL_B_SPLINE_SURFACE(((1.,0.999906284659141,0.999906284659141,1.),
(1.,0.999906284659141,0.999906284659141,1.),(1.,0.999906284659141,0.999906284659141,
1.),(1.,0.999906284659141,0.999906284659141,1.)))
REPRESENTATION_ITEM('')
SURFACE()
);
#1753=(
BOUNDED_SURFACE()
B_SPLINE_SURFACE(3,3,((#129949,#129950,#129951,#129952),(#129953,#129954,
#129955,#129956),(#129957,#129958,#129959,#129960),(#129961,#129962,#129963,
#129964)),.UNSPECIFIED.,.F.,.F.,.F.)
B_SPLINE_SURFACE_WITH_KNOTS((4,4),(4,4),(0.320636407294544,0.371421293305274),
(0.,1.),.UNSPECIFIED.)
GEOMETRIC_REPRESENTATION_ITEM()
RATIONAL_B_SPLINE_SURFACE(((1.,0.999967341957925,0.999967341957925,1.),
(1.,0.999967341957925,0.999967341957925,1.),(1.,0.999967341957925,0.999967341957925,
1.),(1.,0.999967341957925,0.999967341957925,1.)))
REPRESENTATION_ITEM('')
SURFACE()
);
#1754=(
BOUNDED_SURFACE()
B_SPLINE_SURFACE(3,3,((#129966,#129967,#129968,#129969),(#129970,#129971,
#129972,#129973),(#129974,#129975,#129976,#129977),(#129978,#129979,#129980,
#129981)),.UNSPECIFIED.,.F.,.F.,.F.)
B_SPLINE_SURFACE_WITH_KNOTS((4,4),(4,4),(0.485037430561784,0.537898553504801),
(0.,1.),.UNSPECIFIED.)
GEOMETRIC_REPRESENTATION_ITEM()
RATIONAL_B_SPLINE_SURFACE(((1.,0.999962289386236,0.999962289386236,1.),
(1.,0.999962289386236,0.999962289386236,1.),(1.,0.999962289386236,0.999962289386236,
1.),(1.,0.999962289386236,0.999962289386236,1.)))
REPRESENTATION_ITEM('')
SURFACE()
);
#1755=(
BOUNDED_SURFACE()
B_SPLINE_SURFACE(3,3,((#129983,#129984,#129985,#129986),(#129987,#129988,
#129989,#129990),(#129991,#129992,#129993,#129994),(#129995,#129996,#129997,
#129998)),.UNSPECIFIED.,.F.,.F.,.F.)
B_SPLINE_SURFACE_WITH_KNOTS((4,4),(4,4),(0.675444462502036,0.738927835629777),
(0.,1.),.UNSPECIFIED.)
GEOMETRIC_REPRESENTATION_ITEM()
RATIONAL_B_SPLINE_SURFACE(((1.,0.999939938463589,0.999939938463589,1.),
(1.,0.999939938463589,0.999939938463589,1.),(1.,0.999939938463589,0.999939938463589,
1.),(1.,0.999939938463589,0.999939938463589,1.)))
REPRESENTATION_ITEM('')
SURFACE()
);
#1756=(
BOUNDED_SURFACE()
B_SPLINE_SURFACE(3,3,((#130000,#130001,#130002,#130003),(#130004,#130005,
#130006,#130007),(#130008,#130009,#130010,#130011),(#130012,#130013,#130014,
#130015)),.UNSPECIFIED.,.F.,.F.,.F.)
B_SPLINE_SURFACE_WITH_KNOTS((4,4),(4,4),(0.848132173016768,0.924294320658525),
(0.,1.),.UNSPECIFIED.)
GEOMETRIC_REPRESENTATION_ITEM()
RATIONAL_B_SPLINE_SURFACE(((1.,0.999906066464898,0.999906066464898,1.),
(1.,0.999906066464898,0.999906066464898,1.),(1.,0.999906066464898,0.999906066464898,
1.),(1.,0.999906066464898,0.999906066464898,1.)))
REPRESENTATION_ITEM('')
SURFACE()
);
#1757=(
BOUNDED_SURFACE()
B_SPLINE_SURFACE(3,3,((#130017,#130018,#130019,#130020),(#130021,#130022,
#130023,#130024),(#130025,#130026,#130027,#130028),(#130029,#130030,#130031,
#130032)),.UNSPECIFIED.,.F.,.F.,.F.)
B_SPLINE_SURFACE_WITH_KNOTS((4,4),(4,4),(0.320505725021218,0.371419722674487),
(0.,1.),.UNSPECIFIED.)
GEOMETRIC_REPRESENTATION_ITEM()
RATIONAL_B_SPLINE_SURFACE(((1.,0.999967360975282,0.999967360975282,1.),
(1.,0.999967360975282,0.999967360975282,1.),(1.,0.999967360975282,0.999967360975282,
1.),(1.,0.999967360975282,0.999967360975282,1.)))
REPRESENTATION_ITEM('')
SURFACE()
);
#1758=(
BOUNDED_SURFACE()
B_SPLINE_SURFACE(3,3,((#130034,#130035,#130036,#130037),(#130038,#130039,
#130040,#130041),(#130042,#130043,#130044,#130045),(#130046,#130047,#130048,
#130049)),.UNSPECIFIED.,.F.,.F.,.F.)
B_SPLINE_SURFACE_WITH_KNOTS((4,4),(4,4),(0.485041236272929,0.537757161067977),
(0.,1.),.UNSPECIFIED.)
GEOMETRIC_REPRESENTATION_ITEM()
RATIONAL_B_SPLINE_SURFACE(((1.,0.999962057900831,0.999962057900831,1.),
(1.,0.999962057900831,0.999962057900831,1.),(1.,0.999962057900831,0.999962057900831,
1.),(1.,0.999962057900831,0.999962057900831,1.)))
REPRESENTATION_ITEM('')
SURFACE()
);
#1759=(
BOUNDED_SURFACE()
B_SPLINE_SURFACE(3,3,((#130051,#130052,#130053,#130054),(#130055,#130056,
#130057,#130058),(#130059,#130060,#130061,#130062),(#130063,#130064,#130065,
#130066)),.UNSPECIFIED.,.F.,.F.,.F.)
B_SPLINE_SURFACE_WITH_KNOTS((4,4),(4,4),(0.675602722634434,0.739081859127056),
(0.,1.),.UNSPECIFIED.)
GEOMETRIC_REPRESENTATION_ITEM()
RATIONAL_B_SPLINE_SURFACE(((1.,0.99994018156245,0.99994018156245,1.),(1.,
0.99994018156245,0.99994018156245,1.),(1.,0.99994018156245,0.99994018156245,
1.),(1.,0.99994018156245,0.99994018156245,1.)))
REPRESENTATION_ITEM('')
SURFACE()
);
#1760=(
BOUNDED_SURFACE()
B_SPLINE_SURFACE(3,3,((#130068,#130069,#130070,#130071),(#130072,#130073,
#130074,#130075),(#130076,#130077,#130078,#130079),(#130080,#130081,#130082,
#130083)),.UNSPECIFIED.,.F.,.F.,.F.)
B_SPLINE_SURFACE_WITH_KNOTS((4,4),(4,4),(0.847942716817777,0.924300472680093),
(0.,1.),.UNSPECIFIED.)
GEOMETRIC_REPRESENTATION_ITEM()
RATIONAL_B_SPLINE_SURFACE(((1.,0.99990624222844,0.99990624222844,1.),(1.,
0.99990624222844,0.99990624222844,1.),(1.,0.99990624222844,0.99990624222844,
1.),(1.,0.99990624222844,0.99990624222844,1.)))
REPRESENTATION_ITEM('')
SURFACE()
);
#1761=(
BOUNDED_SURFACE()
B_SPLINE_SURFACE(3,3,((#130085,#130086,#130087,#130088),(#130089,#130090,
#130091,#130092),(#130093,#130094,#130095,#130096),(#130097,#130098,#130099,
#130100)),.UNSPECIFIED.,.F.,.F.,.F.)
B_SPLINE_SURFACE_WITH_KNOTS((4,4),(4,4),(0.320514009564598,0.371328550441877),
(0.,1.),.UNSPECIFIED.)
GEOMETRIC_REPRESENTATION_ITEM()
RATIONAL_B_SPLINE_SURFACE(((1.,0.999967231313903,0.999967231313903,1.),
(1.,0.999967231313903,0.999967231313903,1.),(1.,0.999967231313903,0.999967231313903,
1.),(1.,0.999967231313903,0.999967231313903,1.)))
REPRESENTATION_ITEM('')
SURFACE()
);
#1762=(
BOUNDED_SURFACE()
B_SPLINE_SURFACE(3,3,((#130102,#130103,#130104,#130105),(#130106,#130107,
#130108,#130109),(#130110,#130111,#130112,#130113),(#130114,#130115,#130116,
#130117)),.UNSPECIFIED.,.F.,.F.,.F.)
B_SPLINE_SURFACE_WITH_KNOTS((4,4),(4,4),(0.48512402908949,0.537892318607367),
(0.,1.),.UNSPECIFIED.)
GEOMETRIC_REPRESENTATION_ITEM()
RATIONAL_B_SPLINE_SURFACE(((1.,0.999962289571751,0.999962289571751,1.),
(1.,0.999962289571751,0.999962289571751,1.),(1.,0.999962289571751,0.999962289571751,
1.),(1.,0.999962289571751,0.999962289571751,1.)))
REPRESENTATION_ITEM('')
SURFACE()
);
#1763=(
BOUNDED_SURFACE()
B_SPLINE_SURFACE(3,3,((#130119,#130120,#130121,#130122),(#130123,#130124,
#130125,#130126),(#130127,#130128,#130129,#130130),(#130131,#130132,#130133,
#130134)),.UNSPECIFIED.,.F.,.F.,.F.)
B_SPLINE_SURFACE_WITH_KNOTS((4,4),(4,4),(0.675452991908006,0.739078420574732),
(0.,1.),.UNSPECIFIED.)
GEOMETRIC_REPRESENTATION_ITEM()
RATIONAL_B_SPLINE_SURFACE(((1.,0.999940089902897,0.999940089902897,1.),
(1.,0.999940089902897,0.999940089902897,1.),(1.,0.999940089902897,0.999940089902897,
1.),(1.,0.999940089902897,0.999940089902897,1.)))
REPRESENTATION_ITEM('')
SURFACE()
);
#1764=(
BOUNDED_SURFACE()
B_SPLINE_SURFACE(3,3,((#130136,#130137,#130138,#130139),(#130140,#130141,
#130142,#130143),(#130144,#130145,#130146,#130147),(#130148,#130149,#130150,
#130151)),.UNSPECIFIED.,.F.,.F.,.F.)
B_SPLINE_SURFACE_WITH_KNOTS((4,4),(4,4),(0.847950520319574,0.924115043194035),
(0.,1.),.UNSPECIFIED.)
GEOMETRIC_REPRESENTATION_ITEM()
RATIONAL_B_SPLINE_SURFACE(((1.,0.999905876767882,0.999905876767882,1.),
(1.,0.999905876767882,0.999905876767882,1.),(1.,0.999905876767882,0.999905876767882,
1.),(1.,0.999905876767882,0.999905876767882,1.)))
REPRESENTATION_ITEM('')
SURFACE()
);
#1765=(
BOUNDED_SURFACE()
B_SPLINE_SURFACE(3,3,((#130153,#130154,#130155,#130156),(#130157,#130158,
#130159,#130160),(#130161,#130162,#130163,#130164),(#130165,#130166,#130167,
#130168)),.UNSPECIFIED.,.F.,.F.,.F.)
B_SPLINE_SURFACE_WITH_KNOTS((4,4),(4,4),(0.320554317164351,0.371402703199328),
(0.,1.),.UNSPECIFIED.)
GEOMETRIC_REPRESENTATION_ITEM()
RATIONAL_B_SPLINE_SURFACE(((1.,0.999967393810812,0.999967393810812,1.),
(1.,0.999967393810812,0.999967393810812,1.),(1.,0.999967393810812,0.999967393810812,
1.),(1.,0.999967393810812,0.999967393810812,1.)))
REPRESENTATION_ITEM('')
SURFACE()
);
#1766=(
BOUNDED_SURFACE()
B_SPLINE_SURFACE(3,3,((#130170,#130171,#130172,#130173),(#130174,#130175,
#130176,#130177),(#130178,#130179,#130180,#130181),(#130182,#130183,#130184,
#130185)),.UNSPECIFIED.,.F.,.F.,.F.)
B_SPLINE_SURFACE_WITH_KNOTS((4,4),(4,4),(0.485062342489115,0.537883560988347),
(0.,1.),.UNSPECIFIED.)
GEOMETRIC_REPRESENTATION_ITEM()
RATIONAL_B_SPLINE_SURFACE(((1.,0.999962138574809,0.999962138574809,1.),
(1.,0.999962138574809,0.999962138574809,1.),(1.,0.999962138574809,0.999962138574809,
1.),(1.,0.999962138574809,0.999962138574809,1.)))
REPRESENTATION_ITEM('')
SURFACE()
);
#1767=(
BOUNDED_SURFACE()
B_SPLINE_SURFACE(3,3,((#130187,#130188,#130189,#130190),(#130191,#130192,
#130193,#130194),(#130195,#130196,#130197,#130198),(#130199,#130200,#130201,
#130202)),.UNSPECIFIED.,.F.,.F.,.F.)
B_SPLINE_SURFACE_WITH_KNOTS((4,4),(4,4),(0.675466656549766,0.738982296165968),
(0.,1.),.UNSPECIFIED.)
GEOMETRIC_REPRESENTATION_ITEM()
RATIONAL_B_SPLINE_SURFACE(((1.,0.999939980433748,0.999939980433748,1.),
(1.,0.999939980433748,0.999939980433748,1.),(1.,0.999939980433748,0.999939980433748,
1.),(1.,0.999939980433748,0.999939980433748,1.)))
REPRESENTATION_ITEM('')
SURFACE()
);
#1768=(
BOUNDED_SURFACE()
B_SPLINE_SURFACE(3,3,((#130204,#130205,#130206,#130207),(#130208,#130209,
#130210,#130211),(#130212,#130213,#130214,#130215),(#130216,#130217,#130218,
#130219)),.UNSPECIFIED.,.F.,.F.,.F.)
B_SPLINE_SURFACE_WITH_KNOTS((4,4),(4,4),(0.84804648712844,0.924282372382723),
(0.,1.),.UNSPECIFIED.)
GEOMETRIC_REPRESENTATION_ITEM()
RATIONAL_B_SPLINE_SURFACE(((1.,0.999906415714148,0.999906415714148,1.),
(1.,0.999906415714148,0.999906415714148,1.),(1.,0.999906415714148,0.999906415714148,
1.),(1.,0.999906415714148,0.999906415714148,1.)))
REPRESENTATION_ITEM('')
SURFACE()
);
#1769=(
BOUNDED_SURFACE()
B_SPLINE_SURFACE(3,3,((#130221,#130222,#130223,#130224),(#130225,#130226,
#130227,#130228),(#130229,#130230,#130231,#130232),(#130233,#130234,#130235,
#130236)),.UNSPECIFIED.,.F.,.F.,.F.)
B_SPLINE_SURFACE_WITH_KNOTS((4,4),(4,4),(0.320604734130633,0.371278297272317),
(0.,1.),.UNSPECIFIED.)
GEOMETRIC_REPRESENTATION_ITEM()
RATIONAL_B_SPLINE_SURFACE(((1.,0.999967281636602,0.999967281636602,1.),
(1.,0.999967281636602,0.999967281636602,1.),(1.,0.999967281636602,0.999967281636602,
1.),(1.,0.999967281636602,0.999967281636602,1.)))
REPRESENTATION_ITEM('')
SURFACE()
);
#1770=(
BOUNDED_SURFACE()
B_SPLINE_SURFACE(3,3,((#130238,#130239,#130240,#130241),(#130242,#130243,
#130244,#130245),(#130246,#130247,#130248,#130249),(#130250,#130251,#130252,
#130253)),.UNSPECIFIED.,.F.,.F.,.F.)
B_SPLINE_SURFACE_WITH_KNOTS((4,4),(4,4),(0.485137973433402,0.537847298674517),
(0.,1.),.UNSPECIFIED.)
GEOMETRIC_REPRESENTATION_ITEM()
RATIONAL_B_SPLINE_SURFACE(((1.,0.99996212094789,0.99996212094789,1.),(1.,
0.99996212094789,0.99996212094789,1.),(1.,0.99996212094789,0.99996212094789,
1.),(1.,0.99996212094789,0.99996212094789,1.)))
REPRESENTATION_ITEM('')
SURFACE()
);
#1771=(
BOUNDED_SURFACE()
B_SPLINE_SURFACE(3,3,((#130255,#130256,#130257,#130258),(#130259,#130260,
#130261,#130262),(#130263,#130264,#130265,#130266),(#130267,#130268,#130269,
#130270)),.UNSPECIFIED.,.F.,.F.,.F.)
B_SPLINE_SURFACE_WITH_KNOTS((4,4),(4,4),(0.675493277798674,0.739045612587958),
(0.,1.),.UNSPECIFIED.)
GEOMETRIC_REPRESENTATION_ITEM()
RATIONAL_B_SPLINE_SURFACE(((1.,0.999940222070666,0.999940222070666,1.),
(1.,0.999940222070666,0.999940222070666,1.),(1.,0.999940222070666,0.999940222070666,
1.),(1.,0.999940222070666,0.999940222070666,1.)))
REPRESENTATION_ITEM('')
SURFACE()
);
#1772=(
BOUNDED_SURFACE()
B_SPLINE_SURFACE(3,3,((#130272,#130273,#130274,#130275),(#130276,#130277,
#130278,#130279),(#130280,#130281,#130282,#130283),(#130284,#130285,#130286,
#130287)),.UNSPECIFIED.,.F.,.F.,.F.)
B_SPLINE_SURFACE_WITH_KNOTS((4,4),(4,4),(0.84799348482738,0.92426372810007),
(0.,1.),.UNSPECIFIED.)
GEOMETRIC_REPRESENTATION_ITEM()
RATIONAL_B_SPLINE_SURFACE(((1.,0.999905944721945,0.999905944721945,1.),
(1.,0.999905944721945,0.999905944721945,1.),(1.,0.999905944721945,0.999905944721945,
1.),(1.,0.999905944721945,0.999905944721945,1.)))
REPRESENTATION_ITEM('')
SURFACE()
);
#1773=(
BOUNDED_SURFACE()
B_SPLINE_SURFACE(3,3,((#130289,#130290,#130291,#130292),(#130293,#130294,
#130295,#130296),(#130297,#130298,#130299,#130300),(#130301,#130302,#130303,
#130304)),.UNSPECIFIED.,.F.,.F.,.F.)
B_SPLINE_SURFACE_WITH_KNOTS((4,4),(4,4),(0.3205402280231,0.371335872514157),
(0.,1.),.UNSPECIFIED.)
GEOMETRIC_REPRESENTATION_ITEM()
RATIONAL_B_SPLINE_SURFACE(((1.,0.99996727377962,0.99996727377962,1.),(1.,
0.99996727377962,0.99996727377962,1.),(1.,0.99996727377962,0.99996727377962,
1.),(1.,0.99996727377962,0.99996727377962,1.)))
REPRESENTATION_ITEM('')
SURFACE()
);
#1774=(
BOUNDED_SURFACE()
B_SPLINE_SURFACE(3,3,((#130306,#130307,#130308,#130309),(#130310,#130311,
#130312,#130313),(#130314,#130315,#130316,#130317),(#130318,#130319,#130320,
#130321)),.UNSPECIFIED.,.F.,.F.,.F.)
B_SPLINE_SURFACE_WITH_KNOTS((4,4),(4,4),(0.485075837246189,0.537808186355769),
(0.,1.),.UNSPECIFIED.)
GEOMETRIC_REPRESENTATION_ITEM()
RATIONAL_B_SPLINE_SURFACE(((1.,0.999962230795869,0.999962230795869,1.),
(1.,0.999962230795869,0.999962230795869,1.),(1.,0.999962230795869,0.999962230795869,
1.),(1.,0.999962230795869,0.999962230795869,1.)))
REPRESENTATION_ITEM('')
SURFACE()
);
#1775=(
BOUNDED_SURFACE()
B_SPLINE_SURFACE(3,3,((#130323,#130324,#130325,#130326),(#130327,#130328,
#130329,#130330),(#130331,#130332,#130333,#130334),(#130335,#130336,#130337,
#130338)),.UNSPECIFIED.,.F.,.F.,.F.)
B_SPLINE_SURFACE_WITH_KNOTS((4,4),(4,4),(0.675564486464684,0.738898139890546),
(0.,1.),.UNSPECIFIED.)
GEOMETRIC_REPRESENTATION_ITEM()
RATIONAL_B_SPLINE_SURFACE(((1.,0.999939996666824,0.999939996666824,1.),
(1.,0.999939996666824,0.999939996666824,1.),(1.,0.999939996666824,0.999939996666824,
1.),(1.,0.999939996666824,0.999939996666824,1.)))
REPRESENTATION_ITEM('')
SURFACE()
);
#1776=(
BOUNDED_SURFACE()
B_SPLINE_SURFACE(3,3,((#130340,#130341,#130342,#130343),(#130344,#130345,
#130346,#130347),(#130348,#130349,#130350,#130351),(#130352,#130353,#130354,
#130355)),.UNSPECIFIED.,.F.,.F.,.F.)
B_SPLINE_SURFACE_WITH_KNOTS((4,4),(4,4),(0.84809304582895,0.924247716835722),
(0.,1.),.UNSPECIFIED.)
GEOMETRIC_REPRESENTATION_ITEM()
RATIONAL_B_SPLINE_SURFACE(((1.,0.999905933509504,0.999905933509504,1.),
(1.,0.999905933509504,0.999905933509504,1.),(1.,0.999905933509504,0.999905933509504,
1.),(1.,0.999905933509504,0.999905933509504,1.)))
REPRESENTATION_ITEM('')
SURFACE()
);
#1777=(
BOUNDED_SURFACE()
B_SPLINE_SURFACE(3,3,((#130357,#130358,#130359,#130360),(#130361,#130362,
#130363,#130364),(#130365,#130366,#130367,#130368),(#130369,#130370,#130371,
#130372)),.UNSPECIFIED.,.F.,.F.,.F.)
B_SPLINE_SURFACE_WITH_KNOTS((4,4),(4,4),(0.320557294445702,0.371402834588606),
(0.,1.),.UNSPECIFIED.)
GEOMETRIC_REPRESENTATION_ITEM()
RATIONAL_B_SPLINE_SURFACE(((1.,0.999967373265669,0.999967373265669,1.),
(1.,0.999967373265669,0.999967373265669,1.),(1.,0.999967373265669,0.999967373265669,
1.),(1.,0.999967373265669,0.999967373265669,1.)))
REPRESENTATION_ITEM('')
SURFACE()
);
#1778=(
BOUNDED_SURFACE()
B_SPLINE_SURFACE(3,3,((#130374,#130375,#130376,#130377),(#130378,#130379,
#130380,#130381),(#130382,#130383,#130384,#130385),(#130386,#130387,#130388,
#130389)),.UNSPECIFIED.,.F.,.F.,.F.)
B_SPLINE_SURFACE_WITH_KNOTS((4,4),(4,4),(0.485061470768506,0.537824685725865),
(0.,1.),.UNSPECIFIED.)
GEOMETRIC_REPRESENTATION_ITEM()
RATIONAL_B_SPLINE_SURFACE(((1.,0.999962123207486,0.999962123207486,1.),
(1.,0.999962123207486,0.999962123207486,1.),(1.,0.999962123207486,0.999962123207486,
1.),(1.,0.999962123207486,0.999962123207486,1.)))
REPRESENTATION_ITEM('')
SURFACE()
);
#1779=(
BOUNDED_SURFACE()
B_SPLINE_SURFACE(3,3,((#130391,#130392,#130393,#130394),(#130395,#130396,
#130397,#130398),(#130399,#130400,#130401,#130402),(#130403,#130404,#130405,
#130406)),.UNSPECIFIED.,.F.,.F.,.F.)
B_SPLINE_SURFACE_WITH_KNOTS((4,4),(4,4),(0.675473799809187,0.738977929617164),
(0.,1.),.UNSPECIFIED.)
GEOMETRIC_REPRESENTATION_ITEM()
RATIONAL_B_SPLINE_SURFACE(((1.,0.999940012441812,0.999940012441812,1.),
(1.,0.999940012441812,0.999940012441812,1.),(1.,0.999940012441812,0.999940012441812,
1.),(1.,0.999940012441812,0.999940012441812,1.)))
REPRESENTATION_ITEM('')
SURFACE()
);
#1780=(
BOUNDED_SURFACE()
B_SPLINE_SURFACE(3,3,((#130408,#130409,#130410,#130411),(#130412,#130413,
#130414,#130415),(#130416,#130417,#130418,#130419),(#130420,#130421,#130422,
#130423)),.UNSPECIFIED.,.F.,.F.,.F.)
B_SPLINE_SURFACE_WITH_KNOTS((4,4),(4,4),(0.848025753359781,0.924153418178438),
(0.,1.),.UNSPECIFIED.)
GEOMETRIC_REPRESENTATION_ITEM()
RATIONAL_B_SPLINE_SURFACE(((1.,0.99990637728161,0.99990637728161,1.),(1.,
0.99990637728161,0.99990637728161,1.),(1.,0.99990637728161,0.99990637728161,
1.),(1.,0.99990637728161,0.99990637728161,1.)))
REPRESENTATION_ITEM('')
SURFACE()
);
#1781=(
BOUNDED_SURFACE()
B_SPLINE_SURFACE(3,3,((#130425,#130426,#130427,#130428),(#130429,#130430,
#130431,#130432),(#130433,#130434,#130435,#130436),(#130437,#130438,#130439,
#130440)),.UNSPECIFIED.,.F.,.F.,.F.)
B_SPLINE_SURFACE_WITH_KNOTS((4,4),(4,4),(0.320510703809115,0.371320148131838),
(0.,1.),.UNSPECIFIED.)
GEOMETRIC_REPRESENTATION_ITEM()
RATIONAL_B_SPLINE_SURFACE(((1.,0.999967253008905,0.999967253008905,1.),
(1.,0.999967253008905,0.999967253008905,1.),(1.,0.999967253008905,0.999967253008905,
1.),(1.,0.999967253008905,0.999967253008905,1.)))
REPRESENTATION_ITEM('')
SURFACE()
);
#1782=(
BOUNDED_SURFACE()
B_SPLINE_SURFACE(3,3,((#130442,#130443,#130444,#130445),(#130446,#130447,
#130448,#130449),(#130450,#130451,#130452,#130453),(#130454,#130455,#130456,
#130457)),.UNSPECIFIED.,.F.,.F.,.F.)
B_SPLINE_SURFACE_WITH_KNOTS((4,4),(4,4),(0.485049233505636,0.537894115044618),
(0.,1.),.UNSPECIFIED.)
GEOMETRIC_REPRESENTATION_ITEM()
RATIONAL_B_SPLINE_SURFACE(((1.,0.999962145144179,0.999962145144179,1.),
(1.,0.999962145144179,0.999962145144179,1.),(1.,0.999962145144179,0.999962145144179,
1.),(1.,0.999962145144179,0.999962145144179,1.)))
REPRESENTATION_ITEM('')
SURFACE()
);
#1783=(
BOUNDED_SURFACE()
B_SPLINE_SURFACE(3,3,((#130459,#130460,#130461,#130462),(#130463,#130464,
#130465,#130466),(#130467,#130468,#130469,#130470),(#130471,#130472,#130473,
#130474)),.UNSPECIFIED.,.F.,.F.,.F.)
B_SPLINE_SURFACE_WITH_KNOTS((4,4),(4,4),(0.67554993384203,0.739074174432657),
(0.,1.),.UNSPECIFIED.)
GEOMETRIC_REPRESENTATION_ITEM()
RATIONAL_B_SPLINE_SURFACE(((1.,0.999940279534679,0.999940279534679,1.),
(1.,0.999940279534679,0.999940279534679,1.),(1.,0.999940279534679,0.999940279534679,
1.),(1.,0.999940279534679,0.999940279534679,1.)))
REPRESENTATION_ITEM('')
SURFACE()
);
#1784=(
BOUNDED_SURFACE()
B_SPLINE_SURFACE(3,3,((#130476,#130477,#130478,#130479),(#130480,#130481,
#130482,#130483),(#130484,#130485,#130486,#130487),(#130488,#130489,#130490,
#130491)),.UNSPECIFIED.,.F.,.F.,.F.)
B_SPLINE_SURFACE_WITH_KNOTS((4,4),(4,4),(0.847957765543921,0.924145861363742),
(0.,1.),.UNSPECIFIED.)
GEOMETRIC_REPRESENTATION_ITEM()
RATIONAL_B_SPLINE_SURFACE(((1.,0.9999059073186,0.9999059073186,1.),(1.,
0.9999059073186,0.9999059073186,1.),(1.,0.9999059073186,0.9999059073186,
1.),(1.,0.9999059073186,0.9999059073186,1.)))
REPRESENTATION_ITEM('')
SURFACE()
);
#1785=(
BOUNDED_SURFACE()
B_SPLINE_SURFACE(3,3,((#130493,#130494,#130495,#130496),(#130497,#130498,
#130499,#130500),(#130501,#130502,#130503,#130504),(#130505,#130506,#130507,
#130508)),.UNSPECIFIED.,.F.,.F.,.F.)
B_SPLINE_SURFACE_WITH_KNOTS((4,4),(4,4),(0.320502991162247,0.371421831902603),
(0.,1.),.UNSPECIFIED.)
GEOMETRIC_REPRESENTATION_ITEM()
RATIONAL_B_SPLINE_SURFACE(((1.,0.999967329307079,0.999967329307079,1.),
(1.,0.999967329307079,0.999967329307079,1.),(1.,0.999967329307079,0.999967329307079,
1.),(1.,0.999967329307079,0.999967329307079,1.)))
REPRESENTATION_ITEM('')
SURFACE()
);
#1786=(
BOUNDED_SURFACE()
B_SPLINE_SURFACE(3,3,((#130510,#130511,#130512,#130513),(#130514,#130515,
#130516,#130517),(#130518,#130519,#130520,#130521),(#130522,#130523,#130524,
#130525)),.UNSPECIFIED.,.F.,.F.,.F.)
B_SPLINE_SURFACE_WITH_KNOTS((4,4),(4,4),(0.485162005966803,0.537898074092653),
(0.,1.),.UNSPECIFIED.)
GEOMETRIC_REPRESENTATION_ITEM()
RATIONAL_B_SPLINE_SURFACE(((1.,0.999962283120094,0.999962283120094,1.),
(1.,0.999962283120094,0.999962283120094,1.),(1.,0.999962283120094,0.999962283120094,
1.),(1.,0.999962283120094,0.999962283120094,1.)))
REPRESENTATION_ITEM('')
SURFACE()
);
#1787=(
BOUNDED_SURFACE()
B_SPLINE_SURFACE(3,3,((#130527,#130528,#130529,#130530),(#130531,#130532,
#130533,#130534),(#130535,#130536,#130537,#130538),(#130539,#130540,#130541,
#130542)),.UNSPECIFIED.,.F.,.F.,.F.)
B_SPLINE_SURFACE_WITH_KNOTS((4,4),(4,4),(0.675446019028147,0.738904200659153),
(0.,1.),.UNSPECIFIED.)
GEOMETRIC_REPRESENTATION_ITEM()
RATIONAL_B_SPLINE_SURFACE(((1.,0.999939928462316,0.999939928462316,1.),
(1.,0.999939928462316,0.999939928462316,1.),(1.,0.999939928462316,0.999939928462316,
1.),(1.,0.999939928462316,0.999939928462316,1.)))
REPRESENTATION_ITEM('')
SURFACE()
);
#1788=(
BOUNDED_SURFACE()
B_SPLINE_SURFACE(3,3,((#130544,#130545,#130546,#130547),(#130548,#130549,
#130550,#130551),(#130552,#130553,#130554,#130555),(#130556,#130557,#130558,
#130559)),.UNSPECIFIED.,.F.,.F.,.F.)
B_SPLINE_SURFACE_WITH_KNOTS((4,4),(4,4),(0.847946092181821,0.924299972364549),
(0.,1.),.UNSPECIFIED.)
GEOMETRIC_REPRESENTATION_ITEM()
RATIONAL_B_SPLINE_SURFACE(((1.,0.999906151714093,0.999906151714093,1.),
(1.,0.999906151714093,0.999906151714093,1.),(1.,0.999906151714093,0.999906151714093,
1.),(1.,0.999906151714093,0.999906151714093,1.)))
REPRESENTATION_ITEM('')
SURFACE()
);
#1789=(
BOUNDED_SURFACE()
B_SPLINE_SURFACE(3,3,((#130561,#130562,#130563,#130564),(#130565,#130566,
#130567,#130568),(#130569,#130570,#130571,#130572),(#130573,#130574,#130575,
#130576)),.UNSPECIFIED.,.F.,.F.,.F.)
B_SPLINE_SURFACE_WITH_KNOTS((4,4),(4,4),(0.320639346010966,0.371419107445367),
(0.,1.),.UNSPECIFIED.)
GEOMETRIC_REPRESENTATION_ITEM()
RATIONAL_B_SPLINE_SURFACE(((1.,0.999967363082376,0.999967363082376,1.),
(1.,0.999967363082376,0.999967363082376,1.),(1.,0.999967363082376,0.999967363082376,
1.),(1.,0.999967363082376,0.999967363082376,1.)))
REPRESENTATION_ITEM('')
SURFACE()
);
#1790=(
BOUNDED_SURFACE()
B_SPLINE_SURFACE(3,3,((#130578,#130579,#130580,#130581),(#130582,#130583,
#130584,#130585),(#130586,#130587,#130588,#130589),(#130590,#130591,#130592,
#130593)),.UNSPECIFIED.,.F.,.F.,.F.)
B_SPLINE_SURFACE_WITH_KNOTS((4,4),(4,4),(0.485038469133326,0.53776448421819),
(0.,1.),.UNSPECIFIED.)
GEOMETRIC_REPRESENTATION_ITEM()
RATIONAL_B_SPLINE_SURFACE(((1.,0.999962058707067,0.999962058707067,1.),
(1.,0.999962058707067,0.999962058707067,1.),(1.,0.999962058707067,0.999962058707067,
1.),(1.,0.999962058707067,0.999962058707067,1.)))
REPRESENTATION_ITEM('')
SURFACE()
);
#1791=(
BOUNDED_SURFACE()
B_SPLINE_SURFACE(3,3,((#130595,#130596,#130597,#130598),(#130599,#130600,
#130601,#130602),(#130603,#130604,#130605,#130606),(#130607,#130608,#130609,
#130610)),.UNSPECIFIED.,.F.,.F.,.F.)
B_SPLINE_SURFACE_WITH_KNOTS((4,4),(4,4),(0.675442877290701,0.739081132522842),
(0.,1.),.UNSPECIFIED.)
GEOMETRIC_REPRESENTATION_ITEM()
RATIONAL_B_SPLINE_SURFACE(((1.,0.999940234359194,0.999940234359194,1.),
(1.,0.999940234359194,0.999940234359194,1.),(1.,0.999940234359194,0.999940234359194,
1.),(1.,0.999940234359194,0.999940234359194,1.)))
REPRESENTATION_ITEM('')
SURFACE()
);
#1792=(
BOUNDED_SURFACE()
B_SPLINE_SURFACE(3,3,((#130612,#130613,#130614,#130615),(#130616,#130617,
#130618,#130619),(#130620,#130621,#130622,#130623),(#130624,#130625,#130626,
#130627)),.UNSPECIFIED.,.F.,.F.,.F.)
B_SPLINE_SURFACE_WITH_KNOTS((4,4),(4,4),(0.848165051389747,0.924298160543409),
(0.,1.),.UNSPECIFIED.)
GEOMETRIC_REPRESENTATION_ITEM()
RATIONAL_B_SPLINE_SURFACE(((1.,0.999906139404426,0.999906139404426,1.),
(1.,0.999906139404426,0.999906139404426,1.),(1.,0.999906139404426,0.999906139404426,
1.),(1.,0.999906139404426,0.999906139404426,1.)))
REPRESENTATION_ITEM('')
SURFACE()
);
#1793=(
BOUNDED_SURFACE()
B_SPLINE_SURFACE(3,3,((#130629,#130630,#130631,#130632),(#130633,#130634,
#130635,#130636),(#130637,#130638,#130639,#130640),(#130641,#130642,#130643,
#130644)),.UNSPECIFIED.,.F.,.F.,.F.)
B_SPLINE_SURFACE_WITH_KNOTS((4,4),(4,4),(0.32050822714455,0.371339675656775),
(0.,1.),.UNSPECIFIED.)
GEOMETRIC_REPRESENTATION_ITEM()
RATIONAL_B_SPLINE_SURFACE(((1.,0.999967238121568,0.999967238121568,1.),
(1.,0.999967238121568,0.999967238121568,1.),(1.,0.999967238121568,0.999967238121568,
1.),(1.,0.999967238121568,0.999967238121568,1.)))
REPRESENTATION_ITEM('')
SURFACE()
);
#1794=(
BOUNDED_SURFACE()
B_SPLINE_SURFACE(3,3,((#130646,#130647,#130648,#130649),(#130650,#130651,
#130652,#130653),(#130654,#130655,#130656,#130657),(#130658,#130659,#130660,
#130661)),.UNSPECIFIED.,.F.,.F.,.F.)
B_SPLINE_SURFACE_WITH_KNOTS((4,4),(4,4),(0.48504281620503,0.537888955734494),
(0.,1.),.UNSPECIFIED.)
GEOMETRIC_REPRESENTATION_ITEM()
RATIONAL_B_SPLINE_SURFACE(((1.,0.999962273981182,0.999962273981182,1.),
(1.,0.999962273981182,0.999962273981182,1.),(1.,0.999962273981182,0.999962273981182,
1.),(1.,0.999962273981182,0.999962273981182,1.)))
REPRESENTATION_ITEM('')
SURFACE()
);
#1795=(
BOUNDED_SURFACE()
B_SPLINE_SURFACE(3,3,((#130663,#130664,#130665,#130666),(#130667,#130668,
#130669,#130670),(#130671,#130672,#130673,#130674),(#130675,#130676,#130677,
#130678)),.UNSPECIFIED.,.F.,.F.,.F.)
B_SPLINE_SURFACE_WITH_KNOTS((4,4),(4,4),(0.675575393990298,0.739072202256826),
(0.,1.),.UNSPECIFIED.)
GEOMETRIC_REPRESENTATION_ITEM()
RATIONAL_B_SPLINE_SURFACE(((1.,0.999940054601015,0.999940054601015,1.),
(1.,0.999940054601015,0.999940054601015,1.),(1.,0.999940054601015,0.999940054601015,
1.),(1.,0.999940054601015,0.999940054601015,1.)))
REPRESENTATION_ITEM('')
SURFACE()
);
#1796=(
BOUNDED_SURFACE()
B_SPLINE_SURFACE(3,3,((#130680,#130681,#130682,#130683),(#130684,#130685,
#130686,#130687),(#130688,#130689,#130690,#130691),(#130692,#130693,#130694,
#130695)),.UNSPECIFIED.,.F.,.F.,.F.)
B_SPLINE_SURFACE_WITH_KNOTS((4,4),(4,4),(0.847948974964019,0.924153056993776),
(0.,1.),.UNSPECIFIED.)
GEOMETRIC_REPRESENTATION_ITEM()
RATIONAL_B_SPLINE_SURFACE(((1.,0.999905914043422,0.999905914043422,1.),
(1.,0.999905914043422,0.999905914043422,1.),(1.,0.999905914043422,0.999905914043422,
1.),(1.,0.999905914043422,0.999905914043422,1.)))
REPRESENTATION_ITEM('')
SURFACE()
);
#1797=(
BOUNDED_SURFACE()
B_SPLINE_SURFACE(3,3,((#130697,#130698,#130699,#130700),(#130701,#130702,
#130703,#130704),(#130705,#130706,#130707,#130708),(#130709,#130710,#130711,
#130712)),.UNSPECIFIED.,.F.,.F.,.F.)
B_SPLINE_SURFACE_WITH_KNOTS((4,4),(4,4),(0.320522498194537,0.37138906164921),
(0.,1.),.UNSPECIFIED.)
GEOMETRIC_REPRESENTATION_ITEM()
RATIONAL_B_SPLINE_SURFACE(((1.,0.999967455651376,0.999967455651376,1.),
(1.,0.999967455651376,0.999967455651376,1.),(1.,0.999967455651376,0.999967455651376,
1.),(1.,0.999967455651376,0.999967455651376,1.)))
REPRESENTATION_ITEM('')
SURFACE()
);
#1798=(
BOUNDED_SURFACE()
B_SPLINE_SURFACE(3,3,((#130714,#130715,#130716,#130717),(#130718,#130719,
#130720,#130721),(#130722,#130723,#130724,#130725),(#130726,#130727,#130728,
#130729)),.UNSPECIFIED.,.F.,.F.,.F.)
B_SPLINE_SURFACE_WITH_KNOTS((4,4),(4,4),(0.485106664599375,0.537873353821538),
(0.,1.),.UNSPECIFIED.)
GEOMETRIC_REPRESENTATION_ITEM()
RATIONAL_B_SPLINE_SURFACE(((1.,0.999962124007028,0.999962124007028,1.),
(1.,0.999962124007028,0.999962124007028,1.),(1.,0.999962124007028,0.999962124007028,
1.),(1.,0.999962124007028,0.999962124007028,1.)))
REPRESENTATION_ITEM('')
SURFACE()
);
#1799=(
BOUNDED_SURFACE()
B_SPLINE_SURFACE(3,3,((#130731,#130732,#130733,#130734),(#130735,#130736,
#130737,#130738),(#130739,#130740,#130741,#130742),(#130743,#130744,#130745,
#130746)),.UNSPECIFIED.,.F.,.F.,.F.)
B_SPLINE_SURFACE_WITH_KNOTS((4,4),(4,4),(0.675463196603712,0.739005452081438),
(0.,1.),.UNSPECIFIED.)
GEOMETRIC_REPRESENTATION_ITEM()
RATIONAL_B_SPLINE_SURFACE(((1.,0.999940012325831,0.999940012325831,1.),
(1.,0.999940012325831,0.999940012325831,1.),(1.,0.999940012325831,0.999940012325831,
1.),(1.,0.999940012325831,0.999940012325831,1.)))
REPRESENTATION_ITEM('')
SURFACE()
);
#1800=(
BOUNDED_SURFACE()
B_SPLINE_SURFACE(3,3,((#130748,#130749,#130750,#130751),(#130752,#130753,
#130754,#130755),(#130756,#130757,#130758,#130759),(#130760,#130761,#130762,
#130763)),.UNSPECIFIED.,.F.,.F.,.F.)
B_SPLINE_SURFACE_WITH_KNOTS((4,4),(4,4),(0.847961069051777,0.924267936729202),
(0.,1.),.UNSPECIFIED.)
GEOMETRIC_REPRESENTATION_ITEM()
RATIONAL_B_SPLINE_SURFACE(((1.,0.999906371282588,0.999906371282588,1.),
(1.,0.999906371282588,0.999906371282588,1.),(1.,0.999906371282588,0.999906371282588,
1.),(1.,0.999906371282588,0.999906371282588,1.)))
REPRESENTATION_ITEM('')
SURFACE()
);
#1801=(
BOUNDED_SURFACE()
B_SPLINE_SURFACE(3,3,((#130765,#130766,#130767,#130768),(#130769,#130770,
#130771,#130772),(#130773,#130774,#130775,#130776),(#130777,#130778,#130779,
#130780)),.UNSPECIFIED.,.F.,.F.,.F.)
B_SPLINE_SURFACE_WITH_KNOTS((4,4),(4,4),(0.320531188332224,0.371363614789913),
(0.,1.),.UNSPECIFIED.)
GEOMETRIC_REPRESENTATION_ITEM()
RATIONAL_B_SPLINE_SURFACE(((1.,0.999967376576078,0.999967376576078,1.),
(1.,0.999967376576078,0.999967376576078,1.),(1.,0.999967376576078,0.999967376576078,
1.),(1.,0.999967376576078,0.999967376576078,1.)))
REPRESENTATION_ITEM('')
SURFACE()
);
#1802=(
BOUNDED_SURFACE()
B_SPLINE_SURFACE(3,3,((#130782,#130783,#130784,#130785),(#130786,#130787,
#130788,#130789),(#130790,#130791,#130792,#130793),(#130794,#130795,#130796,
#130797)),.UNSPECIFIED.,.F.,.F.,.F.)
B_SPLINE_SURFACE_WITH_KNOTS((4,4),(4,4),(0.485078772666084,0.537867979489318),
(0.,1.),.UNSPECIFIED.)
GEOMETRIC_REPRESENTATION_ITEM()
RATIONAL_B_SPLINE_SURFACE(((1.,0.999962406883938,0.999962406883938,1.),
(1.,0.999962406883938,0.999962406883938,1.),(1.,0.999962406883938,0.999962406883938,
1.),(1.,0.999962406883938,0.999962406883938,1.)))
REPRESENTATION_ITEM('')
SURFACE()
);
#1803=(
BOUNDED_SURFACE()
B_SPLINE_SURFACE(3,3,((#130799,#130800,#130801,#130802),(#130803,#130804,
#130805,#130806),(#130807,#130808,#130809,#130810),(#130811,#130812,#130813,
#130814)),.UNSPECIFIED.,.F.,.F.,.F.)
B_SPLINE_SURFACE_WITH_KNOTS((4,4),(4,4),(0.675482427883467,0.739033730461373),
(0.,1.),.UNSPECIFIED.)
GEOMETRIC_REPRESENTATION_ITEM()
RATIONAL_B_SPLINE_SURFACE(((1.,0.999940312318114,0.999940312318114,1.),
(1.,0.999940312318114,0.999940312318114,1.),(1.,0.999940312318114,0.999940312318114,
1.),(1.,0.999940312318114,0.999940312318114,1.)))
REPRESENTATION_ITEM('')
SURFACE()
);
#1804=(
BOUNDED_SURFACE()
B_SPLINE_SURFACE(3,3,((#130816,#130817,#130818,#130819),(#130820,#130821,
#130822,#130823),(#130824,#130825,#130826,#130827),(#130828,#130829,#130830,
#130831)),.UNSPECIFIED.,.F.,.F.,.F.)
B_SPLINE_SURFACE_WITH_KNOTS((4,4),(4,4),(0.848015663369457,0.924242408791934),
(0.,1.),.UNSPECIFIED.)
GEOMETRIC_REPRESENTATION_ITEM()
RATIONAL_B_SPLINE_SURFACE(((1.,0.999905933188592,0.999905933188592,1.),
(1.,0.999905933188592,0.999905933188592,1.),(1.,0.999905933188592,0.999905933188592,
1.),(1.,0.999905933188592,0.999905933188592,1.)))
REPRESENTATION_ITEM('')
SURFACE()
);
#1805=(
BOUNDED_SURFACE()
B_SPLINE_SURFACE(3,3,((#130833,#130834,#130835,#130836),(#130837,#130838,
#130839,#130840),(#130841,#130842,#130843,#130844),(#130845,#130846,#130847,
#130848)),.UNSPECIFIED.,.F.,.F.,.F.)
B_SPLINE_SURFACE_WITH_KNOTS((4,4),(4,4),(0.320515186267197,0.371414001692915),
(0.,1.),.UNSPECIFIED.)
GEOMETRIC_REPRESENTATION_ITEM()
RATIONAL_B_SPLINE_SURFACE(((1.,0.999967299513002,0.999967299513002,1.),
(1.,0.999967299513002,0.999967299513002,1.),(1.,0.999967299513002,0.999967299513002,
1.),(1.,0.999967299513002,0.999967299513002,1.)))
REPRESENTATION_ITEM('')
SURFACE()
);
#1806=(
BOUNDED_SURFACE()
B_SPLINE_SURFACE(3,3,((#130850,#130851,#130852,#130853),(#130854,#130855,
#130856,#130857),(#130858,#130859,#130860,#130861),(#130862,#130863,#130864,
#130865)),.UNSPECIFIED.,.F.,.F.,.F.)
B_SPLINE_SURFACE_WITH_KNOTS((4,4),(4,4),(0.485104001865671,0.537883970557087),
(0.,1.),.UNSPECIFIED.)
GEOMETRIC_REPRESENTATION_ITEM()
RATIONAL_B_SPLINE_SURFACE(((1.,0.999962204175861,0.999962204175861,1.),
(1.,0.999962204175861,0.999962204175861,1.),(1.,0.999962204175861,0.999962204175861,
1.),(1.,0.999962204175861,0.999962204175861,1.)))
REPRESENTATION_ITEM('')
SURFACE()
);
#1807=(
BOUNDED_SURFACE()
B_SPLINE_SURFACE(3,3,((#130867,#130868,#130869,#130870),(#130871,#130872,
#130873,#130874),(#130875,#130876,#130877,#130878),(#130879,#130880,#130881,
#130882)),.UNSPECIFIED.,.F.,.F.,.F.)
B_SPLINE_SURFACE_WITH_KNOTS((4,4),(4,4),(0.675472893615401,0.738995723881163),
(0.,1.),.UNSPECIFIED.)
GEOMETRIC_REPRESENTATION_ITEM()
RATIONAL_B_SPLINE_SURFACE(((1.,0.999940268417788,0.999940268417788,1.),
(1.,0.999940268417788,0.999940268417788,1.),(1.,0.999940268417788,0.999940268417788,
1.),(1.,0.999940268417788,0.999940268417788,1.)))
REPRESENTATION_ITEM('')
SURFACE()
);
#2361=B_SPLINE_CURVE_WITH_KNOTS('',2,(#106608,#106609,#106610),
 .UNSPECIFIED.,.F.,.F.,(3,3),(0.,0.976475345222877),.UNSPECIFIED.);
#2362=B_SPLINE_CURVE_WITH_KNOTS('',2,(#106613,#106614,#106615),
 .UNSPECIFIED.,.F.,.F.,(3,3),(0.,0.976475345222875),.UNSPECIFIED.);
#2363=B_SPLINE_CURVE_WITH_KNOTS('',3,(#106618,#106619,#106620,#106621,#106622,
#106623,#106624,#106625,#106626,#106627,#106628,#106629,#106630,#106631,
#106632,#106633,#106634,#106635,#106636,#106637,#106638,#106639,#106640,
#106641,#106642,#106643,#106644,#106645,#106646,#106647),.UNSPECIFIED.,
 .F.,.F.,(4,2,2,2,2,2,2,2,2,2,2,2,2,2,4),(0.344961523665507,0.345864796648895,
0.383397870327102,0.424095939866412,0.467988143099323,0.511077186362632,
0.54898968974865,0.584500295299886,0.594525424662999,0.600320181695393,
0.604744384514621,0.610406509282569,0.620117456540854,0.65644704575773,
0.689892766641171),.UNSPECIFIED.);
#2364=B_SPLINE_CURVE_WITH_KNOTS('',3,(#106648,#106649,#106650,#106651,#106652,
#106653,#106654,#106655,#106656,#106657,#106658,#106659,#106660,#106661,
#106662,#106663,#106664,#106665,#106666,#106667,#106668,#106669,#106670,
#106671,#106672,#106673,#106674,#106675,#106676,#106677,#106678),
 .UNSPECIFIED.,.F.,.F.,(4,3,2,2,2,2,2,2,2,2,2,2,2,2,4),(0.689892766641171,
0.689896902267116,0.727453888182981,0.768250651128135,0.812331190066408,
0.855408230286001,0.893310548156423,0.92927077257846,0.939389872106851,
0.945235691660359,0.949698027562582,0.955408685939896,0.965204348659296,
1.00190831825778,1.03485842593262),.UNSPECIFIED.);
#2365=B_SPLINE_CURVE_WITH_KNOTS('',3,(#106681,#106682,#106683,#106684,#106685,
#106686,#106687,#106688,#106689,#106690,#106691,#106692,#106693,#106694,
#106695,#106696,#106697,#106698,#106699,#106700,#106701,#106702,#106703,
#106704,#106705,#106706,#106707,#106708,#106709,#106710),.UNSPECIFIED.,
 .F.,.F.,(4,2,2,2,2,2,2,2,2,2,2,2,2,2,4),(0.345009231853205,0.378244613783399,
0.420328023332794,0.464149227428814,0.506016437255813,0.543856281234535,
0.565813314722034,0.573688761513894,0.578687760592208,0.583312543899507,
0.589347859881529,0.601974028845171,0.645360854368571,0.669727951332881,
0.689924578750462),.UNSPECIFIED.);
#2366=B_SPLINE_CURVE_WITH_KNOTS('',3,(#106711,#106712,#106713,#106714,#106715,
#106716,#106717,#106718,#106719,#106720,#106721,#106722,#106723,#106724,
#106725,#106726,#106727,#106728,#106729,#106730,#106731,#106732,#106733,
#106734,#106735,#106736,#106737,#106738,#106739,#106740,#106741,#106742,
#106743),.UNSPECIFIED.,.F.,.F.,(4,3,2,2,2,2,2,2,2,2,2,2,2,2,2,4),(0.689924578750462,
0.68993991408243,0.729536128270215,0.772335318064264,0.815994793172523,
0.857023119234385,0.897080615078242,0.913006093260828,0.919873093228367,
0.924198675336843,0.928927860867944,0.935400644318752,0.950143092826215,
0.993632031191612,1.02921319219025,1.03494914593564),.UNSPECIFIED.);
#2367=B_SPLINE_CURVE_WITH_KNOTS('',3,(#106746,#106747,#106748,#106749,#106750,
#106751,#106752,#106753,#106754,#106755,#106756,#106757,#106758,#106759,
#106760,#106761,#106762,#106763,#106764,#106765,#106766,#106767,#106768,
#106769,#106770,#106771,#106772,#106773,#106774,#106775),.UNSPECIFIED.,
 .F.,.F.,(4,2,2,2,2,2,2,2,2,2,2,2,2,2,4),(0.346938551924172,0.378440651179373,
0.421240632795595,0.464958543144959,0.506100204098339,0.54769824656266,
0.561705730881516,0.567440855372351,0.572216908670401,0.577088174639597,
0.584110215881562,0.601759745786392,0.645470178035154,0.67174709596461,
0.693868053317107),.UNSPECIFIED.);
#2368=B_SPLINE_CURVE_WITH_KNOTS('',3,(#106776,#106777,#106778,#106779,#106780,
#106781,#106782,#106783,#106784,#106785,#106786,#106787,#106788,#106789,
#106790,#106791,#106792,#106793,#106794,#106795,#106796,#106797,#106798,
#106799,#106800,#106801,#106802,#106803,#106804,#106805,#106806,#106807,
#106808),.UNSPECIFIED.,.F.,.F.,(4,3,2,2,2,2,2,2,2,2,2,2,2,2,2,4),(0.693868053317107,
0.693886488938521,0.734477998053822,0.778249159437278,0.82165549791726,
0.860952275386496,0.900557922887624,0.9098397687485,0.915807211744923,0.920529512902708,
0.925787413564647,0.934409438144411,0.963342903225506,0.99595895476539,
1.03255538373466,1.04082504086269),.UNSPECIFIED.);
#2369=B_SPLINE_CURVE_WITH_KNOTS('',3,(#106811,#106812,#106813,#106814,#106815,
#106816,#106817,#106818,#106819,#106820,#106821,#106822,#106823,#106824,
#106825,#106826,#106827,#106828,#106829,#106830,#106831,#106832,#106833,
#106834,#106835,#106836,#106837,#106838,#106839,#106840),.UNSPECIFIED.,
 .F.,.F.,(4,2,2,2,2,2,2,2,2,2,2,2,2,2,4),(0.40209989847735,0.40660288487618,
0.45450907004254,0.50530634558164,0.554814904564047,0.59717232465397,0.631280174008838,
0.641914587848182,0.648218209580416,0.653710157873207,0.660536877518756,
0.673512975029444,0.724577287352579,0.76556777577582,0.80412687291917),
 .UNSPECIFIED.);
#2370=B_SPLINE_CURVE_WITH_KNOTS('',3,(#106841,#106842,#106843,#106844,#106845,
#106846,#106847,#106848,#106849,#106850,#106851,#106852,#106853,#106854,
#106855,#106856,#106857,#106858,#106859,#106860,#106861,#106862,#106863,
#106864,#106865,#106866,#106867,#106868,#106869,#106870,#106871),
 .UNSPECIFIED.,.F.,.F.,(4,3,2,2,2,2,2,2,2,2,2,2,2,2,4),(0.80412687291917,
0.804148773323481,0.852022764489678,0.902845917375077,0.952486292226827,
0.993805484048557,1.03219252264168,1.04331428445352,1.04983910175525,1.0553827665417,
1.06210101783198,1.07437911638428,1.12547022180492,1.16619918742605,1.20624867180083),
 .UNSPECIFIED.);
#2371=B_SPLINE_CURVE_WITH_KNOTS('',3,(#106874,#106875,#106876,#106877,#106878,
#106879,#106880,#106881,#106882,#106883,#106884,#106885,#106886,#106887,
#106888,#106889,#106890,#106891,#106892,#106893,#106894,#106895,#106896,
#106897,#106898,#106899,#106900,#106901,#106902,#106903),.UNSPECIFIED.,
 .F.,.F.,(4,2,2,2,2,2,2,2,2,2,2,2,2,2,4),(0.465633214662796,0.465954622179084,
0.521966589812807,0.580586441169497,0.637296003323887,0.689137640373933,
0.718928717554103,0.730000425807782,0.737142867836688,0.743827353101546,
0.75265656150245,0.771478832925962,0.830418451259722,0.87860301952136,0.931247240689163),
 .UNSPECIFIED.);
#2372=B_SPLINE_CURVE_WITH_KNOTS('',3,(#106904,#106905,#106906,#106907,#106908,
#106909,#106910,#106911,#106912,#106913,#106914,#106915,#106916,#106917,
#106918,#106919,#106920,#106921,#106922,#106923,#106924,#106925,#106926,
#106927,#106928,#106929,#106930,#106931,#106932,#106933,#106934),
 .UNSPECIFIED.,.F.,.F.,(4,3,2,2,2,2,2,2,2,2,2,2,2,2,4),(0.931247240689163,
0.931260314529748,0.987731629074412,1.04629867668198,1.1027854627381,1.15459842582523,
1.18443011275622,1.19558842708719,1.20281567458219,1.20960223615331,1.21860242711111,
1.23793740883115,1.29692637503074,1.34499044045235,1.39689352919254),
 .UNSPECIFIED.);
#2373=B_SPLINE_CURVE_WITH_KNOTS('',3,(#106937,#106938,#106939,#106940,#106941,
#106942,#106943,#106944,#106945,#106946,#106947,#106948,#106949,#106950,
#106951,#106952,#106953,#106954,#106955,#106956,#106957,#106958,#106959,
#106960,#106961,#106962,#106963,#106964,#106965,#106966),.UNSPECIFIED.,
 .F.,.F.,(4,2,2,2,2,2,2,2,2,2,2,2,2,2,4),(0.465633282607765,0.476375394601976,
0.528663123786714,0.584725991294486,0.64333981569091,0.700032605532688,
0.75318841685325,0.780812469598235,0.792201294755606,0.799151250192924,
0.806562525317479,0.816363786652937,0.837233438559275,0.896272823761712,
0.931207257834669),.UNSPECIFIED.);
#2374=B_SPLINE_CURVE_WITH_KNOTS('',3,(#106967,#106968,#106969,#106970,#106971,
#106972,#106973,#106974,#106975,#106976,#106977,#106978,#106979,#106980,
#106981,#106982,#106983,#106984,#106985,#106986,#106987,#106988,#106989,
#106990,#106991,#106992,#106993,#106994,#106995,#106996,#106997),
 .UNSPECIFIED.,.F.,.F.,(4,3,2,2,2,2,2,2,2,2,2,2,2,2,4),(0.931207257834669,
0.931212131173444,0.982986506311894,1.03869641281129,1.09737760956241,1.15460057349639,
1.20473347532919,1.24264303882272,1.25581895302213,1.26401634376283,1.27147456569156,
1.28101576638611,1.3002403817436,1.35942112225154,1.39684541378121),
 .UNSPECIFIED.);
#2375=B_SPLINE_CURVE_WITH_KNOTS('',3,(#107000,#107001,#107002,#107003,#107004,
#107005,#107006,#107007,#107008,#107009,#107010,#107011,#107012,#107013,
#107014,#107015,#107016,#107017,#107018,#107019,#107020,#107021,#107022,
#107023,#107024,#107025,#107026,#107027,#107028,#107029),.UNSPECIFIED.,
 .F.,.F.,(4,2,2,2,2,2,2,2,2,2,2,2,2,2,4),(0.402110712104017,0.41872237939637,
0.463540332761411,0.511693032899096,0.562458220229975,0.611784757547159,
0.655989679395872,0.685075113511474,0.695759884692332,0.702594719239558,
0.708942989788131,0.717248297339878,0.734614608729777,0.757078010388911,
0.804098343149695),.UNSPECIFIED.);
#2376=B_SPLINE_CURVE_WITH_KNOTS('',3,(#107030,#107031,#107032,#107033,#107034,
#107035,#107036,#107037,#107038,#107039,#107040,#107041,#107042,#107043,
#107044,#107045,#107046,#107047,#107048,#107049,#107050,#107051,#107052,
#107053,#107054,#107055,#107056,#107057,#107058,#107059,#107060),
 .UNSPECIFIED.,.F.,.F.,(4,3,2,2,2,2,2,2,2,2,2,2,2,2,4),(0.804098343149695,
0.804102668688614,0.84772337182573,0.894852633655198,0.945590312254206,
0.995686686428953,1.04088233415374,1.08317466217842,1.0957257184503,1.10311305075802,
1.10939434530366,1.11700267358253,1.1308607530412,1.18173687996318,1.20621338079263),
 .UNSPECIFIED.);
#2377=B_SPLINE_CURVE_WITH_KNOTS('',3,(#107063,#107064,#107065,#107066,#107067,
#107068,#107069,#107070,#107071,#107072,#107073,#107074,#107075,#107076,
#107077,#107078,#107079,#107080,#107081,#107082,#107083,#107084,#107085,
#107086,#107087,#107088,#107089,#107090,#107091,#107092),.UNSPECIFIED.,
 .F.,.F.,(4,2,2,2,2,2,2,2,2,2,2,2,2,2,4),(0.346992260168847,0.349530800286321,
0.38627866048027,0.426164077376898,0.469071116498728,0.512754181117553,
0.553769559902602,0.597242326448665,0.60786359204204,0.614714583583491,
0.620138976121923,0.626171706766658,0.636023024924637,0.668251949000156,
0.693906585258332),.UNSPECIFIED.);
#2378=B_SPLINE_CURVE_WITH_KNOTS('',3,(#107093,#107094,#107095,#107096,#107097,
#107098,#107099,#107100,#107101,#107102,#107103,#107104,#107105,#107106,
#107107,#107108,#107109,#107110,#107111,#107112,#107113,#107114,#107115,
#107116,#107117,#107118,#107119,#107120,#107121,#107122,#107123),
 .UNSPECIFIED.,.F.,.F.,(4,3,2,2,2,2,2,2,2,2,2,2,2,2,4),(0.693906585258332,
0.693912249614694,0.730513622803473,0.770348783422489,0.813285096596775,
0.857012732304838,0.898242274447473,0.940578720860681,0.953105519851957,
0.959832426695438,0.965425958564593,0.971115461808322,0.979275907192453,
0.999461241194498,1.04090450978354),.UNSPECIFIED.);
#2379=B_SPLINE_CURVE_WITH_KNOTS('',3,(#107126,#107127,#107128,#107129,#107130,
#107131,#107132,#107133,#107134,#107135,#107136,#107137,#107138,#107139,
#107140,#107141,#107142,#107143,#107144,#107145,#107146,#107147,#107148,
#107149,#107150,#107151,#107152,#107153,#107154,#107155),.UNSPECIFIED.,
 .F.,.F.,(4,2,2,2,2,2,2,2,2,2,2,2,2,2,4),(0.344951413336473,0.351263812252431,
0.387082240635607,0.426231505582015,0.468477015007063,0.512252444209689,
0.553957162909252,0.593842901031732,0.61206567233696,0.620069861726783,
0.62514830287496,0.630721476371493,0.638371191430603,0.655771612190609,
0.689837953066993),.UNSPECIFIED.);
#2380=B_SPLINE_CURVE_WITH_KNOTS('',3,(#107156,#107157,#107158,#107159,#107160,
#107161,#107162,#107163,#107164,#107165,#107166,#107167,#107168,#107169,
#107170,#107171,#107172,#107173,#107174,#107175,#107176,#107177,#107178,
#107179,#107180,#107181,#107182,#107183,#107184,#107185,#107186),
 .UNSPECIFIED.,.F.,.F.,(4,3,2,2,2,2,2,2,2,2,2,2,2,2,4),(0.689837953066993,
0.689842314231483,0.725044567858473,0.763732437183778,0.805601673607611,
0.849510712956202,0.891773097528399,0.92955257745313,0.954274008555207,
0.963486286429678,0.969426005177119,0.974977209335325,0.982290928535058,
0.997772229719781,1.03479372756796),.UNSPECIFIED.);
#2381=B_SPLINE_CURVE_WITH_KNOTS('',3,(#107189,#107190,#107191,#107192,#107193,
#107194,#107195,#107196,#107197,#107198,#107199,#107200,#107201,#107202,
#107203,#107204,#107205,#107206,#107207,#107208,#107209,#107210,#107211,
#107212,#107213,#107214,#107215,#107216,#107217,#107218),.UNSPECIFIED.,
 .F.,.F.,(4,2,2,2,2,2,2,2,2,2,2,2,2,2,4),(0.465611109415691,0.467801168335867,
0.521727320971316,0.579585905539099,0.637746437962676,0.691244410595713,
0.743421186764121,0.756490984203512,0.765054461682126,0.771929024386779,
0.779678856588505,0.792584330974367,0.837109914470849,0.88241247221796,
0.931180169103219),.UNSPECIFIED.);
#2382=B_SPLINE_CURVE_WITH_KNOTS('',3,(#107219,#107220,#107221,#107222,#107223,
#107224,#107225,#107226,#107227,#107228,#107229,#107230,#107231,#107232,
#107233,#107234,#107235,#107236,#107237,#107238,#107239,#107240,#107241,
#107242,#107243,#107244,#107245,#107246,#107247,#107248,#107249),
 .UNSPECIFIED.,.F.,.F.,(4,3,2,2,2,2,2,2,2,2,2,2,2,2,4),(0.931180169103219,
0.931190700960073,0.985359391461488,1.04360629966377,1.1017009783728,1.15517235673943,
1.20857836605825,1.22186490429068,1.23055817840862,1.23753111124902,1.24538769484831,
1.25846672994737,1.30364877307048,1.34893703322522,1.39680181037576),
 .UNSPECIFIED.);
#2383=B_SPLINE_CURVE_WITH_KNOTS('',3,(#107252,#107253,#107254,#107255,#107256,
#107257,#107258,#107259,#107260,#107261,#107262,#107263,#107264,#107265,
#107266,#107267,#107268,#107269,#107270,#107271,#107272,#107273,#107274,
#107275,#107276,#107277,#107278,#107279,#107280,#107281),.UNSPECIFIED.,
 .F.,.F.,(4,2,2,2,2,2,2,2,2,2,2,2,2,2,4),(0.402104921302211,0.40543549785947,
0.451285049701036,0.500507144213953,0.551060081418048,0.599064996386686,
0.647473246556257,0.664439861589408,0.672224467659491,0.678150589012572,
0.684415149542514,0.693989426680647,0.721067191394358,0.757870178076073,
0.804134169471361),.UNSPECIFIED.);
#2384=B_SPLINE_CURVE_WITH_KNOTS('',3,(#107282,#107283,#107284,#107285,#107286,
#107287,#107288,#107289,#107290,#107291,#107292,#107293,#107294,#107295,
#107296,#107297,#107298,#107299,#107300,#107301,#107302,#107303,#107304,
#107305,#107306,#107307,#107308,#107309,#107310,#107311,#107312),
 .UNSPECIFIED.,.F.,.F.,(4,3,2,2,2,2,2,2,2,2,2,2,2,2,4),(0.804134169471361,
0.804148839679616,0.849980894175911,0.899293831723779,0.949871636716832,
0.998054666218493,1.04512970460772,1.06464658368308,1.07326751351405,1.07931411697895,
1.08546450846965,1.09429459053202,1.11625370584153,1.16727831526251,1.20625376098183),
 .UNSPECIFIED.);
#2385=B_SPLINE_CURVE_WITH_KNOTS('',3,(#107315,#107316,#107317,#107318,#107319,
#107320,#107321,#107322,#107323,#107324,#107325,#107326,#107327,#107328,
#107329,#107330,#107331,#107332,#107333,#107334,#107335,#107336,#107337,
#107338,#107339,#107340,#107341,#107342,#107343,#107344,#107345,#107346),
 .UNSPECIFIED.,.F.,.F.,(4,2,2,2,2,2,2,2,2,2,2,2,2,2,2,4),(0.346968393948669,
0.349681440565168,0.38848093502615,0.43028464532601,0.474246146607666,0.516732383605594,
0.554321336137149,0.579626948171219,0.588407112189454,0.593879794000829,
0.598870391068503,0.605276295008421,0.618284444515363,0.634910302035259,
0.666887126081608,0.693786984354256),.UNSPECIFIED.);
#2386=B_SPLINE_CURVE_WITH_KNOTS('',3,(#107347,#107348,#107349,#107350,#107351,
#107352,#107353,#107354,#107355,#107356,#107357,#107358,#107359,#107360,
#107361,#107362,#107363,#107364,#107365,#107366,#107367,#107368,#107369,
#107370,#107371,#107372,#107373,#107374,#107375,#107376,#107377),
 .UNSPECIFIED.,.F.,.F.,(4,3,2,2,2,2,2,2,2,2,2,2,2,2,4),(0.693786984354256,
0.693797831240842,0.732509231161277,0.774310918514032,0.818303801091492,
0.860899596877086,0.89782782159184,0.925658037889556,0.934852364047167,
0.940451300977366,0.945471484446629,0.951800265319109,0.964281244127681,
1.00801838154444,1.04076622518951),.UNSPECIFIED.);
#2387=B_SPLINE_CURVE_WITH_KNOTS('',3,(#107380,#107381,#107382,#107383,#107384,
#107385,#107386,#107387,#107388,#107389,#107390,#107391,#107392,#107393,
#107394,#107395,#107396,#107397,#107398,#107399,#107400,#107401,#107402,
#107403,#107404,#107405,#107406,#107407,#107408,#107409),.UNSPECIFIED.,
 .F.,.F.,(4,2,2,2,2,2,2,2,2,2,2,2,2,2,4),(0.235057050857596,0.292167847167887,
0.348533232507195,0.401524038651083,0.427641552568632,0.43803416448635,
0.444965886579442,0.451624678980447,0.460685531955045,0.481055806932457,
0.540180732620175,0.588617276937645,0.641338245174112,0.698017197142133,
0.700679974573688),.UNSPECIFIED.);
#2388=B_SPLINE_CURVE_WITH_KNOTS('',3,(#107410,#107411,#107412,#107413,#107414,
#107415,#107416,#107417,#107418,#107419,#107420,#107421,#107422,#107423,
#107424,#107425,#107426,#107427,#107428,#107429,#107430,#107431,#107432,
#107433,#107434,#107435,#107436,#107437,#107438,#107439,#107440,#107441,
#107442),.UNSPECIFIED.,.F.,.F.,(4,2,2,2,2,2,2,2,2,3,2,2,2,2,2,4),(0.700679974573688,
0.75654544780487,0.81278852129577,0.865332254711976,0.892716069810879,0.903401685258624,
0.910463492023461,0.917199943822292,0.92629568345056,0.93118074096206,0.964614669288399,
1.00756753716764,1.05596925831,1.1084746812396,1.1647789115579,1.16623779181966),
 .UNSPECIFIED.);
#2389=B_SPLINE_CURVE_WITH_KNOTS('',3,(#107445,#107446,#107447,#107448,#107449,
#107450,#107451,#107452,#107453,#107454,#107455,#107456,#107457,#107458,
#107459,#107460,#107461,#107462,#107463,#107464,#107465,#107466,#107467,
#107468,#107469,#107470,#107471,#107472),.UNSPECIFIED.,.F.,.F.,(4,2,2,2,
2,2,2,2,2,2,2,2,2,4),(0.402076330997609,0.452506126987892,0.501960460596592,
0.544174046662978,0.578024001620107,0.588408509033419,0.594526453801688,
0.599886720261833,0.606484916474157,0.61902420194864,0.670057777031238,
0.710940214646799,0.755738002101945,0.804142170440177),.UNSPECIFIED.);
#2390=B_SPLINE_CURVE_WITH_KNOTS('',3,(#107473,#107474,#107475,#107476,#107477,
#107478,#107479,#107480,#107481,#107482,#107483,#107484,#107485,#107486,
#107487,#107488,#107489,#107490,#107491,#107492,#107493,#107494,#107495,
#107496,#107497,#107498,#107499,#107500,#107501,#107502,#107503,#107504,
#107505),.UNSPECIFIED.,.F.,.F.,(4,3,2,2,2,2,2,2,2,2,2,2,2,2,2,4),(0.804142170440177,
0.80418148149889,0.854955500213731,0.904274720656576,0.946542921138172,
0.980094405895,0.990499100597637,0.996663986623071,1.0020365722695,1.00872009768154,
1.02145302090351,1.07252538866429,1.11332010049143,1.15793086937237,1.20589739254531,
1.2062578124965),.UNSPECIFIED.);
#2391=B_SPLINE_CURVE_WITH_KNOTS('',3,(#107508,#107509,#107510,#107511,#107512,
#107513,#107514,#107515,#107516,#107517,#107518,#107519,#107520,#107521,
#107522,#107523,#107524,#107525,#107526,#107527,#107528,#107529,#107530,
#107531,#107532,#107533,#107534,#107535,#107536,#107537),.UNSPECIFIED.,
 .F.,.F.,(4,2,2,2,2,2,2,2,2,2,2,2,2,2,4),(0.346941605198609,0.373567910257419,
0.417315713383248,0.458600424228201,0.499168359176905,0.514509718036955,
0.521095418591649,0.525235214587882,0.529755122461575,0.535931877421553,
0.549970599447536,0.593803901426271,0.629554481206799,0.663265304325165,
0.693877848521967),.UNSPECIFIED.);
#2392=B_SPLINE_CURVE_WITH_KNOTS('',3,(#107538,#107539,#107540,#107541,#107542,
#107543,#107544,#107545,#107546,#107547,#107548,#107549,#107550,#107551,
#107552,#107553,#107554,#107555,#107556,#107557,#107558,#107559,#107560,
#107561,#107562,#107563,#107564,#107565,#107566,#107567,#107568,#107569,
#107570),.UNSPECIFIED.,.F.,.F.,(4,3,2,2,2,2,2,2,2,2,2,2,2,2,2,4),(0.693877848521967,
0.693902648209849,0.738154480356306,0.781315453318249,0.81887107307235,
0.855429713474733,0.86408961971932,0.869698324340631,0.874166418409527,
0.879174671198948,0.887469616252308,0.916149834072149,0.948595112072686,
0.985080349849095,1.02476161037089,1.04084425340846),.UNSPECIFIED.);
#2393=B_SPLINE_CURVE_WITH_KNOTS('',3,(#107573,#107574,#107575,#107576,#107577,
#107578,#107579,#107580,#107581,#107582,#107583,#107584,#107585,#107586,
#107587,#107588,#107589,#107590,#107591,#107592,#107593,#107594,#107595,
#107596,#107597,#107598,#107599,#107600,#107601,#107602),.UNSPECIFIED.,
 .F.,.F.,(4,2,2,2,2,2,2,2,2,2,2,2,2,2,4),(0.345013218218888,0.376774001203925,
0.42054829328545,0.462160314370201,0.500129576849606,0.520667701551143,
0.52798814139206,0.532626762104135,0.536915397032792,0.542511761139062,
0.554238383666024,0.597657877890008,0.632740518823297,0.662888343785372,
0.689951584416554),.UNSPECIFIED.);
#2394=B_SPLINE_CURVE_WITH_KNOTS('',3,(#107603,#107604,#107605,#107606,#107607,
#107608,#107609,#107610,#107611,#107612,#107613,#107614,#107615,#107616,
#107617,#107618,#107619,#107620,#107621,#107622,#107623,#107624,#107625,
#107626,#107627,#107628,#107629,#107630,#107631,#107632,#107633,#107634,
#107635),.UNSPECIFIED.,.F.,.F.,(4,3,2,2,2,2,2,2,2,2,2,2,2,2,2,4),(0.689951584416554,
0.690031175819254,0.733367493896147,0.77682341922442,0.816779853506336,
0.859352194286298,0.869120219591277,0.874371575626691,0.878753589986668,
0.883235408613554,0.889725075757398,0.906246615748049,0.949592112952706,
0.985377265897947,1.02453248644676,1.03504439403814),.UNSPECIFIED.);
#2395=B_SPLINE_CURVE_WITH_KNOTS('',3,(#107638,#107639,#107640,#107641,#107642,
#107643,#107644,#107645,#107646,#107647,#107648,#107649,#107650,#107651,
#107652,#107653,#107654,#107655,#107656,#107657,#107658,#107659,#107660,
#107661,#107662,#107663,#107664,#107665,#107666,#107667),.UNSPECIFIED.,
 .F.,.F.,(4,2,2,2,2,2,2,2,2,2,2,2,2,2,4),(0.465678353925176,0.47947283256797,
0.538189478865465,0.595588351848854,0.645484311587241,0.685163547761563,
0.697581925416736,0.704952011159827,0.711377663530687,0.719369776764823,
0.734570748252662,0.793813012992343,0.841382671384268,0.888689663004795,
0.931208999842379),.UNSPECIFIED.);
#2396=B_SPLINE_CURVE_WITH_KNOTS('',3,(#107668,#107669,#107670,#107671,#107672,
#107673,#107674,#107675,#107676,#107677,#107678,#107679,#107680,#107681,
#107682,#107683,#107684,#107685,#107686,#107687,#107688,#107689,#107690,
#107691,#107692,#107693,#107694,#107695,#107696,#107697,#107698),
 .UNSPECIFIED.,.F.,.F.,(4,3,2,2,2,2,2,2,2,2,2,2,2,2,4),(0.931208999842379,
0.931226011304187,0.990115852016496,1.04793975658026,1.09935327814772,1.14838855309107,
1.16193535150595,1.16970866979478,1.17627256265779,1.18405220552771,1.19799767304289,
1.25690684108002,1.30400469548165,1.35545656622951,1.39690436522936),
 .UNSPECIFIED.);
#2397=B_SPLINE_CURVE_WITH_KNOTS('',3,(#107701,#107702,#107703,#107704,#107705,
#107706,#107707,#107708,#107709,#107710,#107711,#107712,#107713,#107714,
#107715,#107716,#107717,#107718,#107719,#107720,#107721,#107722,#107723,
#107724,#107725,#107726,#107727,#107728,#107729,#107730),.UNSPECIFIED.,
 .F.,.F.,(4,2,2,2,2,2,2,2,2,2,2,2,2,2,4),(0.345014549679634,0.386080567219748,
0.430067136651455,0.472735539508552,0.507148500076332,0.54032355653713,
0.549335158653087,0.554493138732614,0.558409474651096,0.563401158008921,
0.571922511028402,0.603836011650846,0.636683621167115,0.665362157489524,
0.689861699781107),.UNSPECIFIED.);
#2398=B_SPLINE_CURVE_WITH_KNOTS('',3,(#107731,#107732,#107733,#107734,#107735,
#107736,#107737,#107738,#107739,#107740,#107741,#107742,#107743,#107744,
#107745,#107746,#107747,#107748,#107749,#107750,#107751,#107752,#107753,
#107754,#107755,#107756,#107757,#107758,#107759,#107760,#107761,#107762,
#107763),.UNSPECIFIED.,.F.,.F.,(4,3,2,2,2,2,2,2,2,2,2,2,2,2,2,4),(0.689861699781107,
0.689885375867946,0.731365309643938,0.775350418287857,0.81793713912826,
0.854547668609502,0.885597013512973,0.894397666004993,0.899531658955586,
0.903879917755934,0.909136579589272,0.918721215817642,0.961979632551239,
0.996553294581035,1.0346901002883,1.03489992554758),.UNSPECIFIED.);
#2399=B_SPLINE_CURVE_WITH_KNOTS('',3,(#107766,#107767,#107768,#107769,#107770,
#107771,#107772,#107773,#107774,#107775,#107776,#107777,#107778,#107779,
#107780,#107781,#107782,#107783,#107784,#107785,#107786,#107787,#107788,
#107789,#107790,#107791,#107792,#107793,#107794,#107795),.UNSPECIFIED.,
 .F.,.F.,(4,2,2,2,2,2,2,2,2,2,2,2,2,2,4),(0.346984223850431,0.383731720043479,
0.427698885613696,0.470189395445113,0.506972584188474,0.533779035203666,
0.542258080208027,0.547330337125225,0.551374818695336,0.556768695551526,
0.566676832623525,0.610454623908707,0.645453349283034,0.670975380391931,
0.693877493439465),.UNSPECIFIED.);
#2400=B_SPLINE_CURVE_WITH_KNOTS('',3,(#107796,#107797,#107798,#107799,#107800,
#107801,#107802,#107803,#107804,#107805,#107806,#107807,#107808,#107809,
#107810,#107811,#107812,#107813,#107814,#107815,#107816,#107817,#107818,
#107819,#107820,#107821,#107822,#107823,#107824,#107825,#107826,#107827,
#107828),.UNSPECIFIED.,.F.,.F.,(4,3,2,2,2,2,2,2,2,2,2,2,2,2,2,4),(0.693877493439465,
0.693901141466938,0.73629287301764,0.780170172633046,0.82212462450606,0.860287561330358,
0.882073393862794,0.889866480431594,0.894811040195521,0.899385691506485,
0.905358118387944,0.917873381778568,0.961665207927685,0.997075301414317,
1.03584749510858,1.04088536531737),.UNSPECIFIED.);
#2401=B_SPLINE_CURVE_WITH_KNOTS('',3,(#107831,#107832,#107833,#107834,#107835,
#107836,#107837,#107838,#107839,#107840,#107841,#107842,#107843,#107844,
#107845,#107846,#107847,#107848,#107849,#107850,#107851,#107852,#107853,
#107854,#107855,#107856,#107857,#107858,#107859,#107860),.UNSPECIFIED.,
 .F.,.F.,(4,2,2,2,2,2,2,2,2,2,2,2,2,2,4),(0.402049162873731,0.433559116857739,
0.484300694332918,0.533445518859648,0.576861073004399,0.606036271221772,
0.615810656424386,0.621810686769589,0.627224521241337,0.634098780951983,
0.64782988545491,0.698680764045257,0.739769115378164,0.773562070585536,
0.804032136336491),.UNSPECIFIED.);
#2402=B_SPLINE_CURVE_WITH_KNOTS('',3,(#107861,#107862,#107863,#107864,#107865,
#107866,#107867,#107868,#107869,#107870,#107871,#107872,#107873,#107874,
#107875,#107876,#107877,#107878,#107879,#107880,#107881,#107882,#107883,
#107884,#107885,#107886,#107887,#107888,#107889,#107890,#107891,#107892,
#107893),.UNSPECIFIED.,.F.,.F.,(4,3,2,2,2,2,2,2,2,2,2,2,2,2,2,4),(0.804032136336491,
0.804062641115949,0.85398261454777,0.904386995172918,0.951492381667235,
1.00139949755574,1.01359242137182,1.02087251185226,1.02641430638157,1.03227768692638,
1.04126037251219,1.06694413485489,1.1031299344385,1.14435539546706,1.18931296399841,
1.20611180398968),.UNSPECIFIED.);
#2403=B_SPLINE_CURVE_WITH_KNOTS('',3,(#107896,#107897,#107898,#107899,#107900,
#107901,#107902,#107903,#107904,#107905,#107906,#107907,#107908,#107909,
#107910,#107911,#107912,#107913,#107914,#107915,#107916,#107917,#107918,
#107919,#107920,#107921,#107922,#107923),.UNSPECIFIED.,.F.,.F.,(4,2,2,2,
2,2,2,2,2,2,2,2,2,4),(0.346923834548804,0.347492471562536,0.358682387319118,
0.381656594144265,0.4255057126124,0.463082280883045,0.503624903071197,0.547176174235262,
0.590646242398574,0.630908946566644,0.663727463065525,0.677240358541954,
0.686199062140188,0.693838455970793),.UNSPECIFIED.);
#2404=B_SPLINE_CURVE_WITH_KNOTS('',3,(#107924,#107925,#107926,#107927,#107928,
#107929,#107930,#107931,#107932,#107933,#107934,#107935,#107936,#107937,
#107938,#107939,#107940,#107941,#107942,#107943,#107944,#107945,#107946,
#107947,#107948,#107949),.UNSPECIFIED.,.F.,.F.,(4,2,2,2,2,2,2,2,2,2,2,2,
4),(0.693839419404206,0.704606750411996,0.725889158263226,0.769735770694385,
0.807180923266053,0.847680428772612,0.891263177530282,0.934787064816284,
0.975315507846382,1.00980363380315,1.02369855675641,1.03279737143398,1.0407622905196),
 .UNSPECIFIED.);
#2405=B_SPLINE_CURVE_WITH_KNOTS('',3,(#107952,#107953,#107954,#107955,#107956,
#107957,#107958,#107959,#107960,#107961,#107962,#107963,#107964,#107965,
#107966,#107967,#107968,#107969,#107970,#107971,#107972,#107973,#107974,
#107975,#107976,#107977,#107978,#107979),.UNSPECIFIED.,.F.,.F.,(4,2,2,2,
2,2,2,2,2,2,2,2,2,4),(0.402045801646055,0.426921368863666,0.477783146629179,
0.521019108342606,0.567585276430284,0.617510190643648,0.66788189707345,
0.715127898259456,0.756057910476084,0.771905472506671,0.782049634113368,
0.791401874899713,0.803445023961482,0.804097435867718),.UNSPECIFIED.);
#2406=B_SPLINE_CURVE_WITH_KNOTS('',3,(#107980,#107981,#107982,#107983,#107984,
#107985,#107986,#107987,#107988,#107989,#107990,#107991,#107992,#107993,
#107994,#107995,#107996,#107997,#107998,#107999,#108000,#108001,#108002,
#108003,#108004,#108005,#108006,#108007,#108008,#108009,#108010),
 .UNSPECIFIED.,.F.,.F.,(4,3,2,2,2,2,2,2,2,2,2,2,2,2,4),(0.804097435867718,
0.804103776346135,0.829254561954751,0.880091094347011,0.923508652442152,
0.970360729707258,1.02070692826603,1.07099893487689,1.11789119350307,1.1582226578329,
1.17400850621127,1.18420897271328,1.19368863158308,1.20600944477179,1.20614957799219),
 .UNSPECIFIED.);
#2407=B_SPLINE_CURVE_WITH_KNOTS('',3,(#108013,#108014,#108015,#108016,#108017,
#108018,#108019,#108020,#108021,#108022,#108023,#108024,#108025,#108026,
#108027,#108028,#108029,#108030,#108031,#108032,#108033,#108034,#108035,
#108036,#108037,#108038,#108039,#108040,#108041,#108042,#108043),
 .UNSPECIFIED.,.F.,.F.,(4,2,2,2,2,2,2,2,2,2,2,2,2,3,4),(0.465705745830445,
0.470774723111983,0.52973002499315,0.578949941471191,0.632027677515685,
0.688850530102868,0.747336217373916,0.803360293533464,0.858785062007324,
0.878232653829143,0.889966032860068,0.900224687334042,0.912925016678726,
0.931340862153995,0.931356284564515),.UNSPECIFIED.);
#2408=B_SPLINE_CURVE_WITH_KNOTS('',3,(#108044,#108045,#108046,#108047,#108048,
#108049,#108050,#108051,#108052,#108053,#108054,#108055,#108056,#108057,
#108058,#108059,#108060,#108061,#108062,#108063,#108064,#108065,#108066,
#108067,#108068,#108069),.UNSPECIFIED.,.F.,.F.,(4,2,2,2,2,2,2,2,2,2,2,2,
4),(0.931356284564515,0.99029013163098,1.03925563042585,1.09229320421292,
1.1492159206642,1.20771402926609,1.26396011211653,1.32304991410423,1.34320598478706,
1.35520274265849,1.3656980982517,1.37850099915017,1.39704660798444),
 .UNSPECIFIED.);
#2409=B_SPLINE_CURVE_WITH_KNOTS('',3,(#108072,#108073,#108074,#108075,#108076,
#108077,#108078,#108079,#108080,#108081,#108082,#108083,#108084,#108085,
#108086,#108087,#108088,#108089,#108090,#108091,#108092,#108093,#108094,
#108095,#108096,#108097,#108098,#108099,#108100,#108101,#108102),
 .UNSPECIFIED.,.F.,.F.,(4,2,2,2,2,2,2,2,2,2,2,2,2,3,4),(0.465625642587795,
0.46963582819796,0.486523139143415,0.521324663550571,0.580567805094179,
0.631598103689096,0.68626244179692,0.744842955132037,0.802806095596914,
0.856101750172039,0.894199625898987,0.912116560013009,0.92483196746483,
0.93121746950414,0.931219179268937),.UNSPECIFIED.);
#2410=B_SPLINE_CURVE_WITH_KNOTS('',3,(#108103,#108104,#108105,#108106,#108107,
#108108,#108109,#108110,#108111,#108112,#108113,#108114,#108115,#108116,
#108117,#108118,#108119,#108120,#108121,#108122,#108123,#108124,#108125,
#108126,#108127,#108128),.UNSPECIFIED.,.F.,.F.,(4,2,2,2,2,2,2,2,2,2,2,2,
4),(0.931219179268937,0.945898873169598,0.971610242714637,1.03089218876425,
1.08093500745788,1.13484629914441,1.19265752748803,1.25095610952642,1.30630408366767,
1.3543436424464,1.37459191685001,1.38807682528934,1.39684311209194),
 .UNSPECIFIED.);
#2411=B_SPLINE_CURVE_WITH_KNOTS('',3,(#108131,#108132,#108133,#108134,#108135,
#108136,#108137,#108138,#108139,#108140,#108141,#108142,#108143,#108144,
#108145,#108146,#108147,#108148,#108149,#108150,#108151,#108152,#108153,
#108154,#108155,#108156,#108157,#108158,#108159,#108160),.UNSPECIFIED.,
 .F.,.F.,(4,2,2,2,2,2,2,2,2,2,2,2,2,2,4),(0.344929353748955,0.356066387985214,
0.389855717107168,0.427273389355083,0.46783456176705,0.511548842370844,
0.554747413930576,0.593618559643077,0.627942429506497,0.63944129776671,
0.646393342871627,0.651954413439602,0.659369265155035,0.672885808948647,
0.689779825813832),.UNSPECIFIED.);
#2412=B_SPLINE_CURVE_WITH_KNOTS('',3,(#108161,#108162,#108163,#108164,#108165,
#108166,#108167,#108168,#108169,#108170,#108171,#108172,#108173,#108174,
#108175,#108176,#108177,#108178,#108179,#108180,#108181,#108182,#108183,
#108184,#108185,#108186,#108187,#108188,#108189,#108190,#108191),
 .UNSPECIFIED.,.F.,.F.,(4,3,2,2,2,2,2,2,2,2,2,2,2,2,4),(0.689779825813832,
0.689781272935385,0.722061177204161,0.758341904221671,0.797942076641633,
0.840714760187093,0.884384308283039,0.925587030298816,0.968028390553152,
0.980740789559616,0.988792848857853,0.995059183993389,1.00190661459628,
1.01279771322258,1.03471062668434),.UNSPECIFIED.);
#2413=B_SPLINE_CURVE_WITH_KNOTS('',3,(#108194,#108195,#108196,#108197,#108198,
#108199,#108200,#108201,#108202,#108203,#108204,#108205,#108206,#108207,
#108208,#108209,#108210,#108211,#108212,#108213,#108214,#108215,#108216,
#108217,#108218,#108219,#108220,#108221,#108222,#108223),.UNSPECIFIED.,
 .F.,.F.,(4,2,2,2,2,2,2,2,2,2,2,2,2,2,4),(0.346946091970032,0.362169661154315,
0.397913330429784,0.436911788404973,0.478890702759673,0.522820047512213,
0.565181015061556,0.604959042354894,0.625937529042244,0.635004093110909,
0.640690484113908,0.646869824701532,0.655230741674527,0.673680600425937,
0.693804801232447),.UNSPECIFIED.);
#2414=B_SPLINE_CURVE_WITH_KNOTS('',3,(#108224,#108225,#108226,#108227,#108228,
#108229,#108230,#108231,#108232,#108233,#108234,#108235,#108236,#108237,
#108238,#108239,#108240,#108241,#108242,#108243,#108244,#108245,#108246,
#108247,#108248,#108249,#108250,#108251,#108252,#108253,#108254),
 .UNSPECIFIED.,.F.,.F.,(4,3,2,2,2,2,2,2,2,2,2,2,2,2,4),(0.693804801232447,
0.693806115099353,0.727855665576057,0.765538671741975,0.806334052799794,
0.850308183137197,0.893628499506294,0.932649719620875,0.967659922220942,
0.979166044414383,0.986074731355195,0.991577842716568,0.998889785880524,
1.01215643999181,1.04075220706938),.UNSPECIFIED.);
#2415=B_SPLINE_CURVE_WITH_KNOTS('',3,(#108257,#108258,#108259,#108260,#108261,
#108262,#108263,#108264,#108265,#108266,#108267,#108268,#108269,#108270,
#108271,#108272,#108273,#108274,#108275,#108276,#108277,#108278,#108279,
#108280,#108281,#108282,#108283,#108284,#108285,#108286),.UNSPECIFIED.,
 .F.,.F.,(4,2,2,2,2,2,2,2,2,2,2,2,2,2,4),(0.402056392934123,0.415725541001598,
0.458014623602486,0.503818281659996,0.552968951849433,0.603544598861705,
0.651759339635257,0.701442307487862,0.717795138271998,0.726389516260717,
0.733336281403097,0.741203550532206,0.754346536834056,0.799145653455496,
0.804125925786716),.UNSPECIFIED.);
#2416=B_SPLINE_CURVE_WITH_KNOTS('',3,(#108287,#108288,#108289,#108290,#108291,
#108292,#108293,#108294,#108295,#108296,#108297,#108298,#108299,#108300,
#108301,#108302,#108303,#108304,#108305,#108306,#108307,#108308,#108309,
#108310,#108311,#108312,#108313,#108314,#108315,#108316,#108317),
 .UNSPECIFIED.,.F.,.F.,(4,3,2,2,2,2,2,2,2,2,2,2,2,2,4),(0.804125925786716,
0.804128615238701,0.845155185705043,0.890014570959388,0.93831179499375,
0.989084952746491,1.03844854652443,1.08299792990404,1.11259388513163,1.12407593396706,
1.13161574664347,1.13875379755981,1.14828275904418,1.16884243501129,1.20618500817282),
 .UNSPECIFIED.);
#2417=B_SPLINE_CURVE_WITH_KNOTS('',3,(#108320,#108321,#108322,#108323,#108324,
#108325,#108326,#108327,#108328,#108329,#108330,#108331,#108332,#108333,
#108334,#108335,#108336,#108337,#108338,#108339,#108340,#108341,#108342,
#108343,#108344,#108345,#108346,#108347,#108348,#108349),.UNSPECIFIED.,
 .F.,.F.,(4,2,2,2,2,2,2,2,2,2,2,2,2,2,4),(0.465633555653808,0.48902304098224,
0.539900733776193,0.594559743378545,0.653268263770176,0.711087177306013,
0.762115182186353,0.805365665617788,0.820017835174731,0.828957198199194,
0.836960392683509,0.847007604204608,0.866574886846893,0.891177068870352,
0.931115281912586),.UNSPECIFIED.);
#2418=B_SPLINE_CURVE_WITH_KNOTS('',3,(#108350,#108351,#108352,#108353,#108354,
#108355,#108356,#108357,#108358,#108359,#108360,#108361,#108362,#108363,
#108364,#108365,#108366,#108367,#108368,#108369,#108370,#108371,#108372,
#108373,#108374,#108375,#108376,#108377,#108378,#108379,#108380),
 .UNSPECIFIED.,.F.,.F.,(4,3,2,2,2,2,2,2,2,2,2,2,2,2,4),(0.931115281912586,
0.931118834265423,0.980185404156724,1.03339735797292,1.09056474151636,1.14899276356096,
1.20469552616681,1.26194703525585,1.28158858556552,1.29173091397475,1.29984279634438,
1.30894160242414,1.32394974737251,1.3737045459604,1.39675238991923),
 .UNSPECIFIED.);
#2419=B_SPLINE_CURVE_WITH_KNOTS('',3,(#108383,#108384,#108385,#108386,#108387,
#108388,#108389,#108390,#108391,#108392,#108393,#108394,#108395,#108396,
#108397,#108398,#108399,#108400,#108401,#108402,#108403,#108404,#108405,
#108406,#108407,#108408,#108409,#108410,#108411,#108412,#108413),
 .UNSPECIFIED.,.F.,.F.,(4,2,2,2,2,2,2,2,2,2,2,2,2,3,4),(0.465589681684986,
0.496128546877633,0.544999613356941,0.597826659970873,0.65441740735428,
0.712942957110809,0.769128685328421,0.827041610036713,0.844828954473707,
0.856270447579278,0.865269152346198,0.875183138738762,0.891087651752675,
0.931218391145373,0.931220143022425),.UNSPECIFIED.);
#2420=B_SPLINE_CURVE_WITH_KNOTS('',3,(#108414,#108415,#108416,#108417,#108418,
#108419,#108420,#108421,#108422,#108423,#108424,#108425,#108426,#108427,
#108428,#108429,#108430,#108431,#108432,#108433,#108434,#108435,#108436,
#108437,#108438,#108439,#108440,#108441),.UNSPECIFIED.,.F.,.F.,(4,2,2,2,
2,2,2,2,2,2,2,2,2,4),(0.931220143022425,0.976984089799801,1.02746543549214,
1.08190728792339,1.14042373752107,1.19843917110758,1.25168121512924,1.29873019007383,
1.31517435472236,1.3252999622728,1.33441215374149,1.34589730846604,1.36832488468541,
1.39680807283036),.UNSPECIFIED.);
#2421=B_SPLINE_CURVE_WITH_KNOTS('',3,(#108444,#108445,#108446,#108447,#108448,
#108449,#108450,#108451,#108452,#108453,#108454,#108455,#108456,#108457,
#108458,#108459,#108460,#108461,#108462,#108463,#108464,#108465,#108466,
#108467,#108468,#108469,#108470,#108471),.UNSPECIFIED.,.F.,.F.,(4,2,2,2,
2,2,2,2,2,2,2,2,2,4),(0.402063646876575,0.441646596742676,0.483924716415397,
0.529687053017377,0.578771335705642,0.62936790151733,0.677767564968129,
0.728753561348022,0.744574570083672,0.753834238490205,0.760926103248254,
0.769993393033367,0.785403526963908,0.804156206519059),.UNSPECIFIED.);
#2422=B_SPLINE_CURVE_WITH_KNOTS('',3,(#108472,#108473,#108474,#108475,#108476,
#108477,#108478,#108479,#108480,#108481,#108482,#108483,#108484,#108485,
#108486,#108487,#108488,#108489,#108490,#108491,#108492,#108493,#108494,
#108495,#108496,#108497,#108498,#108499,#108500,#108501,#108502),
 .UNSPECIFIED.,.F.,.F.,(4,3,2,2,2,2,2,2,2,2,2,2,2,2,4),(0.804156206519059,
0.804157258093312,0.854950961196192,0.898407721114375,0.945342475157257,
0.995820010661875,1.0460439587594,1.0923382436039,1.13368877110193,1.14817489104761,
1.15708729909082,1.16509903970329,1.17518134959325,1.19480243396671,1.20622090496989),
 .UNSPECIFIED.);
#2423=B_SPLINE_CURVE_WITH_KNOTS('',3,(#108505,#108506,#108507,#108508,#108509,
#108510,#108511,#108512,#108513,#108514,#108515,#108516,#108517,#108518,
#108519,#108520,#108521,#108522,#108523,#108524,#108525,#108526,#108527,
#108528,#108529,#108530,#108531,#108532),.UNSPECIFIED.,.F.,.F.,(4,2,2,2,
2,2,2,2,2,2,2,2,2,4),(0.346979838988578,0.389336004351652,0.425577187134249,
0.46496713826328,0.507320727156668,0.55117060783772,0.593174276350411,0.635676681418817,
0.651757495702357,0.660344238561706,0.667330683117476,0.675272687128708,
0.688553176936598,0.693939839454841),.UNSPECIFIED.);
#2424=B_SPLINE_CURVE_WITH_KNOTS('',3,(#108533,#108534,#108535,#108536,#108537,
#108538,#108539,#108540,#108541,#108542,#108543,#108544,#108545,#108546,
#108547,#108548,#108549,#108550,#108551,#108552,#108553,#108554,#108555,
#108556,#108557,#108558,#108559,#108560),.UNSPECIFIED.,.F.,.F.,(4,2,2,2,
2,2,2,2,2,2,2,2,2,4),(0.693940241893941,0.737947156937577,0.774444412995097,
0.814135349753758,0.856885167708674,0.900674824035094,0.942337766572511,
0.986246565510725,1.00029536137702,1.0084596027801,1.01549910539396,1.02397712029396,
1.03938606723986,1.04092008088252),.UNSPECIFIED.);
#2425=B_SPLINE_CURVE_WITH_KNOTS('',3,(#108563,#108564,#108565,#108566,#108567,
#108568,#108569,#108570,#108571,#108572,#108573,#108574,#108575,#108576,
#108577,#108578,#108579,#108580,#108581,#108582,#108583,#108584,#108585,
#108586,#108587,#108588,#108589,#108590),.UNSPECIFIED.,.F.,.F.,(4,2,2,2,
2,2,2,2,2,2,2,2,2,4),(0.344885080154984,0.354876053781735,0.398358879728667,
0.434465989334581,0.473802837102125,0.516196923660638,0.55993729649274,
0.601593803249262,0.644356926525559,0.659194193979544,0.667768322580426,
0.674987214089382,0.683465605510929,0.689844673350394),.UNSPECIFIED.);
#2426=B_SPLINE_CURVE_WITH_KNOTS('',3,(#108591,#108592,#108593,#108594,#108595,
#108596,#108597,#108598,#108599,#108600,#108601,#108602,#108603,#108604,
#108605,#108606,#108607,#108608,#108609,#108610,#108611,#108612,#108613,
#108614,#108615,#108616,#108617,#108618,#108619,#108620,#108621),
 .UNSPECIFIED.,.F.,.F.,(4,3,2,2,2,2,2,2,2,2,2,2,2,2,4),(0.689844673350394,
0.689846634861934,0.715465196018713,0.748402202680178,0.785108152470509,
0.825054217672711,0.868162581283261,0.911721478265126,0.952519282856293,
0.99187467863693,1.00547719556773,1.01371135701474,1.02028401069715,1.02900997080457,
1.03473171501692),.UNSPECIFIED.);
#2427=B_SPLINE_CURVE_WITH_KNOTS('',3,(#108624,#108625,#108626,#108627,#108628,
#108629,#108630,#108631,#108632,#108633,#108634,#108635,#108636,#108637,
#108638,#108639,#108640,#108641,#108642,#108643,#108644,#108645,#108646,
#108647,#108648,#108649,#108650,#108651,#108652,#108653),.UNSPECIFIED.,
 .F.,.F.,(4,2,2,2,2,2,2,2,2,2,2,2,2,2,4),(0.23513087161813,0.257665545269238,
0.314319195769947,0.366535179018702,0.395398201653438,0.406406232789782,
0.413600810132003,0.42040112084831,0.429482432095946,0.449207525765485,
0.508236859979792,0.556589804879141,0.609236088900844,0.665834302352657,
0.700744682332408),.UNSPECIFIED.);
#2428=B_SPLINE_CURVE_WITH_KNOTS('',3,(#108654,#108655,#108656,#108657,#108658,
#108659,#108660,#108661,#108662,#108663,#108664,#108665,#108666,#108667,
#108668,#108669,#108670,#108671,#108672,#108673,#108674,#108675,#108676,
#108677,#108678,#108679,#108680,#108681,#108682,#108683,#108684,#108685,
#108686),.UNSPECIFIED.,.F.,.F.,(4,2,2,2,2,2,2,2,2,2,3,2,2,2,2,4),(0.700744682332408,
0.724377815208848,0.780725936511176,0.833217266124318,0.86120641695614,
0.872169246047208,0.879420403240007,0.886340189619999,0.895684963280036,
0.916407130769888,0.931141466796302,0.973719157965918,1.02185187591133,
1.07413019711891,1.13019606874401,1.16627233841443),.UNSPECIFIED.);
#2429=B_SPLINE_CURVE_WITH_KNOTS('',3,(#108689,#108690,#108691,#108692,#108693,
#108694,#108695,#108696,#108697,#108698,#108699,#108700,#108701,#108702,
#108703,#108704,#108705,#108706,#108707,#108708,#108709,#108710,#108711,
#108712,#108713,#108714,#108715,#108716,#108717,#108718),.UNSPECIFIED.,
 .F.,.F.,(4,2,2,2,2,2,2,2,2,2,2,2,2,2,4),(0.402049576064962,0.442924940773306,
0.490985398883326,0.538391239477101,0.556366477228441,0.564315810841895,
0.569899087317611,0.575587236270038,0.583774297354325,0.604278587837761,
0.655331441968366,0.69752209930774,0.743402415341105,0.773581410804251,
0.804039827553986),.UNSPECIFIED.);
#2430=B_SPLINE_CURVE_WITH_KNOTS('',3,(#108719,#108720,#108721,#108722,#108723,
#108724,#108725,#108726,#108727,#108728,#108729,#108730,#108731,#108732,
#108733,#108734,#108735,#108736,#108737,#108738,#108739,#108740,#108741,
#108742,#108743,#108744,#108745,#108746,#108747,#108748,#108749,#108750,
#108751),.UNSPECIFIED.,.F.,.F.,(4,3,2,2,2,2,2,2,2,2,2,2,2,2,2,4),(0.804039827553986,
0.804063550621079,0.854373442811622,0.900881225382939,0.949678790887404,
0.96080284686332,0.967871450737339,0.973410881050953,0.979522490884367,
0.989418941157237,1.02159380938173,1.05923062921021,1.10145952242515,1.14725276098453,
1.19642197418901,1.20611312668604),.UNSPECIFIED.);
#2431=B_SPLINE_CURVE_WITH_KNOTS('',3,(#108754,#108755,#108756,#108757,#108758,
#108759,#108760,#108761,#108762,#108763,#108764,#108765,#108766,#108767,
#108768,#108769,#108770,#108771,#108772,#108773,#108774,#108775,#108776,
#108777,#108778,#108779,#108780,#108781,#108782,#108783),.UNSPECIFIED.,
 .F.,.F.,(4,2,2,2,2,2,2,2,2,2,2,2,2,2,4),(0.346993950805442,0.380996151679775,
0.423508224638363,0.460147398068903,0.487374610716494,0.495858524682818,
0.500900558944594,0.505305062634139,0.51079885501452,0.52131419844937,0.565233428154864,
0.600368372516561,0.638991123740337,0.66668600193962,0.693883548523562),
 .UNSPECIFIED.);
#2432=B_SPLINE_CURVE_WITH_KNOTS('',3,(#108784,#108785,#108786,#108787,#108788,
#108789,#108790,#108791,#108792,#108793,#108794,#108795,#108796,#108797,
#108798,#108799,#108800,#108801,#108802,#108803,#108804,#108805,#108806,
#108807,#108808,#108809,#108810,#108811,#108812,#108813,#108814,#108815,
#108816),.UNSPECIFIED.,.F.,.F.,(4,3,2,2,2,2,2,2,2,2,2,2,2,2,2,4),(0.693883548523562,
0.693911449692292,0.737714685061078,0.779272180174301,0.818589460670165,
0.836942720435357,0.844132912473772,0.848432810651463,0.852961474627973,
0.858870645041464,0.871244658654114,0.915042137758771,0.950422336714534,
0.989171528292634,1.03093524701467,1.04090540049773),.UNSPECIFIED.);
#2433=B_SPLINE_CURVE_WITH_KNOTS('',3,(#108819,#108820,#108821,#108822,#108823,
#108824,#108825,#108826,#108827,#108828,#108829,#108830,#108831,#108832,
#108833,#108834,#108835,#108836,#108837,#108838,#108839,#108840,#108841,
#108842,#108843,#108844,#108845,#108846,#108847,#108848),.UNSPECIFIED.,
 .F.,.F.,(4,2,2,2,2,2,2,2,2,2,2,2,2,2,4),(0.3449473234351,0.383972379609475,
0.426630739903034,0.463495506028656,0.49478654096451,0.503410679492906,
0.508385006664272,0.512183429878956,0.517050806941317,0.525433985800617,
0.557706502535248,0.590555291519674,0.627396944749139,0.659553333722666,
0.68982195704123),.UNSPECIFIED.);
#2434=B_SPLINE_CURVE_WITH_KNOTS('',3,(#108849,#108850,#108851,#108852,#108853,
#108854,#108855,#108856,#108857,#108858,#108859,#108860,#108861,#108862,
#108863,#108864,#108865,#108866,#108867,#108868,#108869,#108870,#108871,
#108872,#108873,#108874,#108875,#108876,#108877,#108878,#108879,#108880,
#108881),.UNSPECIFIED.,.F.,.F.,(4,3,2,2,2,2,2,2,2,2,2,2,2,2,2,4),(0.68982195704123,
0.689915857735377,0.733838749870872,0.776100520611407,0.811923867201258,
0.840265609412777,0.848576158635835,0.853501218510488,0.857761720827947,
0.862941916004609,0.872615795928119,0.915883691423952,0.950464809790433,
0.988612423914805,1.02990109317486,1.03486318117048),.UNSPECIFIED.);
#2435=B_SPLINE_CURVE_WITH_KNOTS('',3,(#108884,#108885,#108886,#108887,#108888,
#108889,#108890,#108891,#108892,#108893,#108894,#108895,#108896,#108897,
#108898,#108899,#108900,#108901,#108902,#108903,#108904,#108905,#108906,
#108907,#108908,#108909,#108910,#108911,#108912,#108913,#108914),
 .UNSPECIFIED.,.F.,.F.,(4,2,2,2,2,2,2,2,2,2,2,2,2,3,4),(0.344948818872903,
0.34648558610318,0.35379420124694,0.363486809549799,0.380807029707963,0.424289830006885,
0.460871612859494,0.500666448418649,0.543589083599318,0.587222639540401,
0.628438882135512,0.668029692054682,0.682703378839969,0.689884357221945,
0.689885383506442),.UNSPECIFIED.);
#2436=B_SPLINE_CURVE_WITH_KNOTS('',3,(#108915,#108916,#108917,#108918,#108919,
#108920,#108921,#108922,#108923,#108924,#108925,#108926,#108927,#108928,
#108929,#108930,#108931,#108932,#108933,#108934,#108935,#108936,#108937,
#108938,#108939,#108940),.UNSPECIFIED.,.F.,.F.,(4,2,2,2,2,2,2,2,2,2,2,2,
4),(0.689885383506442,0.698053478442917,0.707526032156531,0.723721892194936,
0.767089663931964,0.803365942675116,0.842817653261609,0.885307866396609,
0.929024686839016,0.970639482202589,1.01223872953034,1.02722931611229,1.03483317609485),
 .UNSPECIFIED.);
#2437=B_SPLINE_CURVE_WITH_KNOTS('',3,(#108943,#108944,#108945,#108946,#108947,
#108948,#108949,#108950,#108951,#108952,#108953,#108954,#108955,#108956,
#108957,#108958,#108959,#108960,#108961,#108962,#108963,#108964,#108965,
#108966,#108967,#108968,#108969,#108970),.UNSPECIFIED.,.F.,.F.,(4,2,2,2,
2,2,2,2,2,2,2,2,2,4),(0.344882043626189,0.352989105107807,0.363926627501424,
0.3711716185643,0.378060236624948,0.387276828919064,0.407094714992322,0.450659584359954,
0.487474857318371,0.527535978355668,0.570775578744059,0.614277204715927,
0.65477324729973,0.689797023258215),.UNSPECIFIED.);
#2438=B_SPLINE_CURVE_WITH_KNOTS('',3,(#108971,#108972,#108973,#108974,#108975,
#108976,#108977,#108978,#108979,#108980,#108981,#108982,#108983,#108984,
#108985,#108986,#108987,#108988,#108989,#108990,#108991,#108992,#108993,
#108994,#108995,#108996,#108997,#108998),.UNSPECIFIED.,.F.,.F.,(4,2,2,2,
2,2,2,2,2,2,2,2,2,4),(0.689797333961378,0.703450158460547,0.71220221069754,
0.719066574503029,0.726610076636724,0.738671816952097,0.775294349047951,
0.80986862415414,0.847901887648394,0.889027092265501,0.933366718957538,
0.976197876803047,1.01535724395698,1.0346790668844),.UNSPECIFIED.);
#2439=B_SPLINE_CURVE_WITH_KNOTS('',3,(#109001,#109002,#109003,#109004,#109005,
#109006,#109007,#109008,#109009,#109010,#109011,#109012,#109013,#109014,
#109015,#109016,#109017,#109018,#109019,#109020,#109021,#109022,#109023,
#109024,#109025,#109026,#109027,#109028),.UNSPECIFIED.,.F.,.F.,(4,2,2,2,
2,2,2,2,2,2,2,2,2,4),(0.346869666639179,0.354370653515026,0.362541062299255,
0.370355651574061,0.38085124734922,0.403385681755292,0.447233199907815,
0.484762146264627,0.52536318975603,0.569075144213089,0.612537491684678,
0.652657149294534,0.687070443946799,0.693791313456527),.UNSPECIFIED.);
#2440=B_SPLINE_CURVE_WITH_KNOTS('',3,(#109029,#109030,#109031,#109032,#109033,
#109034,#109035,#109036,#109037,#109038,#109039,#109040,#109041,#109042,
#109043,#109044,#109045,#109046,#109047,#109048,#109049,#109050,#109051,
#109052,#109053,#109054,#109055,#109056,#109057,#109058,#109059),
 .UNSPECIFIED.,.F.,.F.,(4,3,2,2,2,2,2,2,2,2,2,2,2,2,4),(0.693791313456527,
0.693794119363892,0.704023311866356,0.711876653713803,0.720190462252714,
0.732808907987192,0.766691935276412,0.80138404315909,0.839422665010973,
0.880425923133339,0.924528249546443,0.967721377887932,1.00633946370428,
1.03596310622201,1.04066378600307),.UNSPECIFIED.);
#2441=B_SPLINE_CURVE_WITH_KNOTS('',3,(#109062,#109063,#109064,#109065,#109066,
#109067,#109068,#109069,#109070,#109071,#109072,#109073,#109074,#109075,
#109076,#109077,#109078,#109079,#109080,#109081,#109082,#109083,#109084,
#109085,#109086,#109087,#109088,#109089,#109090,#109091,#109092),
 .UNSPECIFIED.,.F.,.F.,(4,2,2,2,2,2,2,2,2,2,2,2,2,3,4),(0.402095295909212,
0.405579891764716,0.415766170466332,0.4284730590739,0.45249443113515,0.503327000412256,
0.546700481715136,0.593473225181061,0.643696040678488,0.694046096415582,
0.741373026361261,0.781608430858166,0.798286582163595,0.804144678533662,
0.804146349058566),.UNSPECIFIED.);
#2442=B_SPLINE_CURVE_WITH_KNOTS('',3,(#109093,#109094,#109095,#109096,#109097,
#109098,#109099,#109100,#109101,#109102,#109103,#109104,#109105,#109106,
#109107,#109108,#109109,#109110,#109111,#109112,#109113,#109114,#109115,
#109116,#109117,#109118),.UNSPECIFIED.,.F.,.F.,(4,2,2,2,2,2,2,2,2,2,2,2,
4),(0.804146349058566,0.814450657715169,0.825919625880521,0.844245346091432,
0.89509135649372,0.937392406014544,0.983081672039519,1.03202864527732,1.0826698233326,
1.13145421224722,1.18006724600391,1.19837326252841,1.20623997444287),
 .UNSPECIFIED.);
#2443=B_SPLINE_CURVE_WITH_KNOTS('',3,(#109121,#109122,#109123,#109124,#109125,
#109126,#109127,#109128,#109129,#109130,#109131,#109132,#109133,#109134,
#109135,#109136,#109137,#109138,#109139,#109140,#109141,#109142,#109143,
#109144,#109145,#109146,#109147,#109148,#109149,#109150),.UNSPECIFIED.,
 .F.,.F.,(4,2,2,2,2,2,2,2,2,2,2,2,2,2,4),(0.465630957639009,0.481933210616303,
0.535242614313078,0.563024946110058,0.574648402499332,0.581809656529143,
0.589496546094033,0.599743139456495,0.621829787220229,0.680864997484433,
0.729716870256327,0.782756962199145,0.83974870019235,0.881827618684303,
0.931138912205881),.UNSPECIFIED.);
#2444=B_SPLINE_CURVE_WITH_KNOTS('',3,(#109151,#109152,#109153,#109154,#109155,
#109156,#109157,#109158,#109159,#109160,#109161,#109162,#109163,#109164,
#109165,#109166,#109167,#109168,#109169,#109170,#109171,#109172,#109173,
#109174,#109175,#109176,#109177,#109178,#109179,#109180,#109181),
 .UNSPECIFIED.,.F.,.F.,(4,3,2,2,2,2,2,2,2,2,2,2,2,2,4),(0.931138912205881,
0.931141638331543,0.980504007870222,1.02323155336671,1.0374278068647,1.0460417539728,
1.05373254085545,1.06337028302394,1.08213318737524,1.14131516052482,1.18943829620451,
1.24168287524649,1.29769743121417,1.35631949893545,1.39677259597055),
 .UNSPECIFIED.);
#2445=B_SPLINE_CURVE_WITH_KNOTS('',3,(#109184,#109185,#109186,#109187,#109188,
#109189,#109190,#109191,#109192,#109193,#109194,#109195,#109196,#109197,
#109198,#109199,#109200,#109201,#109202,#109203,#109204,#109205,#109206,
#109207,#109208,#109209,#109210,#109211,#109212,#109213),.UNSPECIFIED.,
 .F.,.F.,(4,2,2,2,2,2,2,2,2,2,2,2,2,2,4),(0.402124309272361,0.421627341777243,
0.464872714227461,0.496765510113577,0.507624575968613,0.514319250314185,
0.520371390461007,0.528062884199748,0.543405344995164,0.594209088483205,
0.635662749000266,0.680906583862294,0.729607600766311,0.764590820032904,
0.804073160672369),.UNSPECIFIED.);
#2446=B_SPLINE_CURVE_WITH_KNOTS('',3,(#109214,#109215,#109216,#109217,#109218,
#109219,#109220,#109221,#109222,#109223,#109224,#109225,#109226,#109227,
#109228,#109229,#109230,#109231,#109232,#109233,#109234,#109235,#109236,
#109237,#109238,#109239,#109240,#109241,#109242,#109243,#109244),
 .UNSPECIFIED.,.F.,.F.,(4,3,2,2,2,2,2,2,2,2,2,2,2,2,4),(0.804073160672369,
0.804085254144401,0.850050308649933,0.895243952982647,0.907843732340252,
0.915061602581693,0.921143593411249,0.928331556329836,0.94114401239225,
0.991985862136534,1.0328415254673,1.0774801344348,1.12546183964273,1.17625016754876,
1.20620956341676),.UNSPECIFIED.);
#2447=B_SPLINE_CURVE_WITH_KNOTS('',3,(#109247,#109248,#109249,#109250,#109251,
#109252,#109253,#109254,#109255,#109256,#109257,#109258,#109259,#109260,
#109261,#109262,#109263,#109264,#109265,#109266,#109267,#109268,#109269,
#109270,#109271,#109272,#109273,#109274,#109275,#109276),.UNSPECIFIED.,
 .F.,.F.,(4,2,2,2,2,2,2,2,2,2,2,2,2,2,4),(0.346994532186391,0.382164652532166,
0.420784033011186,0.442103361704628,0.45010253341702,0.455291674197675,
0.460170465296368,0.466649939984645,0.480606624884645,0.524360787319406,
0.560151349727645,0.599306476742075,0.64155218827536,0.666590950965648,
0.693872421523419),.UNSPECIFIED.);
#2448=B_SPLINE_CURVE_WITH_KNOTS('',3,(#109277,#109278,#109279,#109280,#109281,
#109282,#109283,#109284,#109285,#109286,#109287,#109288,#109289,#109290,
#109291,#109292,#109293,#109294,#109295,#109296,#109297,#109298,#109299,
#109300,#109301,#109302,#109303,#109304,#109305,#109306,#109307,#109308,
#109309),.UNSPECIFIED.,.F.,.F.,(4,3,2,2,2,2,2,2,2,2,2,2,2,2,2,4),(0.693872421523419,
0.693884091081668,0.7351695103979,0.776128574475123,0.791745968454944,0.797891390586484,
0.802453862835923,0.807407685914084,0.814124184856907,0.829141438103611,
0.872882271954203,0.908751433499746,0.947896971802218,0.990049089273971,
1.03394297490375,1.04087862326806),.UNSPECIFIED.);
#2449=B_SPLINE_CURVE_WITH_KNOTS('',3,(#109312,#109313,#109314,#109315,#109316,
#109317,#109318,#109319,#109320,#109321,#109322,#109323,#109324,#109325,
#109326,#109327,#109328,#109329,#109330,#109331,#109332,#109333,#109334,
#109335,#109336,#109337,#109338,#109339,#109340,#109341),.UNSPECIFIED.,
 .F.,.F.,(4,2,2,2,2,2,2,2,2,2,2,2,2,2,4),(0.344999942815522,0.381943582058605,
0.418154029345294,0.44831722446467,0.45712008470837,0.462312727341851,0.46678675019175,
0.472201183473186,0.482227764720134,0.525498069008382,0.560258776784043,
0.598611000252602,0.640171561678573,0.664290716544723,0.68990424298228),
 .UNSPECIFIED.);
#2450=B_SPLINE_CURVE_WITH_KNOTS('',3,(#109342,#109343,#109344,#109345,#109346,
#109347,#109348,#109349,#109350,#109351,#109352,#109353,#109354,#109355,
#109356,#109357,#109358,#109359,#109360,#109361,#109362,#109363,#109364,
#109365,#109366,#109367,#109368,#109369,#109370,#109371,#109372,#109373,
#109374),.UNSPECIFIED.,.F.,.F.,(4,3,2,2,2,2,2,2,2,2,2,2,2,2,2,4),(0.68990424298228,
0.689921489597089,0.732017271454668,0.768741909879443,0.794320223466152,
0.802659448183967,0.807720878420951,0.811799401099935,0.817294338043404,
0.827565067504058,0.870910623355331,0.90565267068528,0.943924419349473,
0.985327674934479,1.0292961171375,1.03492143241261),.UNSPECIFIED.);
#2451=B_SPLINE_CURVE_WITH_KNOTS('',3,(#109377,#109378,#109379,#109380,#109381,
#109382,#109383,#109384,#109385,#109386,#109387,#109388,#109389,#109390,
#109391,#109392,#109393,#109394,#109395,#109396,#109397,#109398,#109399,
#109400,#109401,#109402,#109403,#109404,#109405,#109406),.UNSPECIFIED.,
 .F.,.F.,(4,2,2,2,2,2,2,2,2,2,2,2,2,2,4),(0.235147519047353,0.270079203343737,
0.321248161065438,0.360484158913179,0.373462373146903,0.381345721820111,
0.388394617326011,0.397247094673285,0.414563352645265,0.473778780166836,
0.521797219958211,0.574157167267294,0.630455746779035,0.689053581599555,
0.700757096167161),.UNSPECIFIED.);
#2452=B_SPLINE_CURVE_WITH_KNOTS('',3,(#109407,#109408,#109409,#109410,#109411,
#109412,#109413,#109414,#109415,#109416,#109417,#109418,#109419,#109420,
#109421,#109422,#109423,#109424,#109425,#109426,#109427,#109428,#109429,
#109430,#109431,#109432,#109433,#109434,#109435,#109436,#109437),
 .UNSPECIFIED.,.F.,.F.,(4,2,2,2,2,2,2,2,2,3,2,2,2,2,4),(0.700757096167161,
0.74574592571697,0.797562147829136,0.828614623243329,0.840400148080654,
0.848080143967425,0.855320592607384,0.864958909385184,0.885761885582985,
0.931172598139542,0.978100519054367,1.02940050406239,1.0844850950303,1.1437492669342,
1.16632011718689),.UNSPECIFIED.);
#2453=B_SPLINE_CURVE_WITH_KNOTS('',3,(#109440,#109441,#109442,#109443,#109444,
#109445,#109446,#109447,#109448,#109449,#109450,#109451,#109452,#109453,
#109454,#109455,#109456,#109457,#109458,#109459,#109460,#109461,#109462,
#109463,#109464,#109465,#109466,#109467,#109468,#109469),.UNSPECIFIED.,
 .F.,.F.,(4,2,2,2,2,2,2,2,2,2,2,2,2,2,4),(0.402068706671266,0.403065557403745,
0.452265829927698,0.495942952564712,0.525036207784967,0.535088757160506,
0.541344128236347,0.547042238725329,0.554348485704057,0.569162218753928,
0.619983909342393,0.661298627530047,0.706438874571811,0.755042332304185,
0.804117029823683),.UNSPECIFIED.);
#2454=B_SPLINE_CURVE_WITH_KNOTS('',3,(#109470,#109471,#109472,#109473,#109474,
#109475,#109476,#109477,#109478,#109479,#109480,#109481,#109482,#109483,
#109484,#109485,#109486,#109487,#109488,#109489,#109490,#109491,#109492,
#109493,#109494,#109495,#109496,#109497,#109498,#109499,#109500),
 .UNSPECIFIED.,.F.,.F.,(4,3,2,2,2,2,2,2,2,2,2,2,2,2,4),(0.804117029823683,
0.804148478785509,0.853289954180878,0.89669726254831,0.926741624702312,
0.936995948249101,0.943342218262998,0.949101125759267,0.956456433532982,
0.971280891051743,1.02210639107617,1.06328898116581,1.10820381165191,1.15646537383303,
1.20621718545677),.UNSPECIFIED.);
#2455=B_SPLINE_CURVE_WITH_KNOTS('',3,(#109503,#109504,#109505,#109506,#109507,
#109508,#109509,#109510,#109511,#109512,#109513,#109514,#109515,#109516,
#109517,#109518,#109519,#109520,#109521,#109522,#109523,#109524,#109525,
#109526,#109527,#109528,#109529,#109530,#109531,#109532,#109533,#109534),
 .UNSPECIFIED.,.F.,.F.,(4,2,2,2,2,2,2,2,2,2,2,2,2,2,2,4),(0.347000201591407,
0.349957219711082,0.39293291266258,0.428785611965772,0.46239565443992,0.47172731156569,
0.477108289343941,0.481213483526896,0.486467015331691,0.495487378786048,
0.529647560730359,0.56320586320055,0.600581178594504,0.641128658155968,
0.667016278770337,0.69380582230332),.UNSPECIFIED.);
#2456=B_SPLINE_CURVE_WITH_KNOTS('',3,(#109535,#109536,#109537,#109538,#109539,
#109540,#109541,#109542,#109543,#109544,#109545,#109546,#109547,#109548,
#109549,#109550,#109551,#109552,#109553,#109554,#109555,#109556,#109557,
#109558,#109559,#109560,#109561,#109562,#109563,#109564,#109565),
 .UNSPECIFIED.,.F.,.F.,(4,3,2,2,2,2,2,2,2,2,2,2,2,2,4),(0.69380582230332,
0.693823417159995,0.736887921450666,0.77375096897562,0.8088488216942,0.818398781231576,
0.823859998204031,0.828463261660433,0.833911929852199,0.843668681036052,
0.885405269817422,0.920052462661799,0.958204970860161,0.99939121812381,
1.0408236187514),.UNSPECIFIED.);
#2457=B_SPLINE_CURVE_WITH_KNOTS('',3,(#109568,#109569,#109570,#109571,#109572,
#109573,#109574,#109575,#109576,#109577,#109578,#109579,#109580,#109581,
#109582,#109583,#109584,#109585,#109586,#109587,#109588,#109589,#109590,
#109591,#109592,#109593,#109594,#109595,#109596,#109597),.UNSPECIFIED.,
 .F.,.F.,(4,2,2,2,2,2,2,2,2,2,2,2,2,2,4),(0.344994788972036,0.371998850508981,
0.41383828389175,0.451257335147389,0.473742260370782,0.481413353641608,
0.486172059564842,0.490502237936666,0.496054570065859,0.50734469069417,
0.5507443601542,0.585751946465345,0.624314672083482,0.657180388120093,0.689930754578743),
 .UNSPECIFIED.);
#2458=B_SPLINE_CURVE_WITH_KNOTS('',3,(#109598,#109599,#109600,#109601,#109602,
#109603,#109604,#109605,#109606,#109607,#109608,#109609,#109610,#109611,
#109612,#109613,#109614,#109615,#109616,#109617,#109618,#109619,#109620,
#109621,#109622,#109623,#109624,#109625,#109626,#109627,#109628,#109629,
#109630),.UNSPECIFIED.,.F.,.F.,(4,3,2,2,2,2,2,2,2,2,2,2,2,2,2,4),(0.689930754578743,
0.68995605109708,0.733315175883505,0.772752808703065,0.814476102512377,
0.823487197603381,0.829129592965408,0.833502545720314,0.838281230189835,
0.845927355678044,0.870210369956026,0.901450945282902,0.937040898848585,
0.976028236344697,1.01813254197155,1.03495084006912),.UNSPECIFIED.);
#2459=B_SPLINE_CURVE_WITH_KNOTS('',3,(#109633,#109634,#109635,#109636,#109637,
#109638,#109639,#109640,#109641,#109642,#109643,#109644,#109645,#109646,
#109647,#109648,#109649,#109650,#109651,#109652,#109653,#109654,#109655,
#109656,#109657,#109658,#109659,#109660,#109661,#109662,#109663,#109664),
 .UNSPECIFIED.,.F.,.F.,(4,2,2,2,2,2,2,2,2,2,2,2,2,2,2,4),(0.344971545335952,
0.345545647028644,0.384764681179798,0.40424327008886,0.412309880833698,
0.417253957091865,0.422545454073276,0.429579981909098,0.444717699179436,
0.488060634823621,0.523877930949446,0.563102095839794,0.605510165502449,
0.643225963532927,0.664545274820508,0.689824776316506),.UNSPECIFIED.);
#2460=B_SPLINE_CURVE_WITH_KNOTS('',3,(#109665,#109666,#109667,#109668,#109669,
#109670,#109671,#109672,#109673,#109674,#109675,#109676,#109677,#109678,
#109679,#109680,#109681,#109682,#109683,#109684,#109685,#109686,#109687,
#109688,#109689,#109690,#109691,#109692,#109693,#109694,#109695),
 .UNSPECIFIED.,.F.,.F.,(4,3,2,2,2,2,2,2,2,2,2,2,2,2,4),(0.689824776316506,
0.689830282259499,0.728867836398559,0.74884817389962,0.757049758657684,
0.762048740226498,0.767378328492543,0.77442980694277,0.789487509518511,
0.832830212937649,0.868546979352336,0.907616287512977,0.949786922410696,
0.993585378979441,1.03480182759545),.UNSPECIFIED.);
#2461=B_SPLINE_CURVE_WITH_KNOTS('',3,(#109698,#109699,#109700,#109701,#109702,
#109703,#109704,#109705,#109706,#109707,#109708,#109709,#109710,#109711,
#109712,#109713,#109714,#109715,#109716,#109717,#109718,#109719,#109720,
#109721,#109722,#109723,#109724,#109725,#109726,#109727),.UNSPECIFIED.,
 .F.,.F.,(4,2,2,2,2,2,2,2,2,2,2,2,2,2,4),(0.346991000077703,0.369652304047158,
0.393534285289892,0.402847338016846,0.408986699981362,0.414819000879822,
0.422638624902608,0.439658747555291,0.483358554520194,0.51977654113599,
0.559441391326081,0.602191731812778,0.641992454894118,0.665097906765919,
0.693832015935598),.UNSPECIFIED.);
#2462=B_SPLINE_CURVE_WITH_KNOTS('',3,(#109728,#109729,#109730,#109731,#109732,
#109733,#109734,#109735,#109736,#109737,#109738,#109739,#109740,#109741,
#109742,#109743,#109744,#109745,#109746,#109747,#109748,#109749,#109750,
#109751,#109752,#109753,#109754,#109755,#109756,#109757,#109758),
 .UNSPECIFIED.,.F.,.F.,(4,3,2,2,2,2,2,2,2,2,2,2,2,2,4),(0.693832015935598,
0.693838450061331,0.735157906153247,0.747030826425598,0.753866318900802,
0.759637840977357,0.766464847112779,0.778622940969573,0.82230777596829,
0.857791368445199,0.896584070116107,0.938366691203684,0.982333997742008,
1.02487382026543,1.04082945013903),.UNSPECIFIED.);
#2463=B_SPLINE_CURVE_WITH_KNOTS('',3,(#109761,#109762,#109763,#109764,#109765,
#109766,#109767,#109768,#109769,#109770,#109771,#109772,#109773,#109774,
#109775,#109776,#109777,#109778,#109779,#109780,#109781,#109782,#109783,
#109784,#109785,#109786,#109787,#109788,#109789,#109790),.UNSPECIFIED.,
 .F.,.F.,(4,2,2,2,2,2,2,2,2,2,2,2,2,2,4),(0.402070660444346,0.430721222203059,
0.448436737907617,0.457639121252569,0.465012884527248,0.473287523239665,
0.486915648254195,0.531388130722923,0.571962836637525,0.616435337523612,
0.664342021409311,0.715164441118493,0.752777285105839,0.775342417317356,
0.803996534145188),.UNSPECIFIED.);
#2464=B_SPLINE_CURVE_WITH_KNOTS('',3,(#109791,#109792,#109793,#109794,#109795,
#109796,#109797,#109798,#109799,#109800,#109801,#109802,#109803,#109804,
#109805,#109806,#109807,#109808,#109809,#109810,#109811,#109812,#109813,
#109814,#109815,#109816,#109817,#109818),.UNSPECIFIED.,.F.,.F.,(4,2,2,2,
2,2,2,2,2,2,2,2,2,4),(0.80399666330925,0.840948073023333,0.85411547906342,
0.862340222843209,0.869827285138543,0.879389422933621,0.898503079269372,
0.949541782070688,0.991673901808353,1.03732980012108,1.08631662695951,1.13693275473247,
1.18540913330378,1.20606719458953),.UNSPECIFIED.);
#2465=B_SPLINE_CURVE_WITH_KNOTS('',3,(#109821,#109822,#109823,#109824,#109825,
#109826,#109827,#109828,#109829,#109830,#109831,#109832,#109833,#109834,
#109835,#109836,#109837,#109838,#109839,#109840,#109841,#109842,#109843,
#109844,#109845,#109846,#109847,#109848,#109849,#109850,#109851),
 .UNSPECIFIED.,.F.,.F.,(4,2,2,2,2,2,2,2,2,2,2,2,2,3,4),(0.46556985358348,
0.477882011556651,0.488346204604764,0.499686903254209,0.514866865476111,
0.547047227056689,0.606163109414153,0.656953163861814,0.711606625070641,
0.770301819100196,0.828283906607871,0.881749498431883,0.924288167774753,
0.931164974956878,0.931170439482049),.UNSPECIFIED.);
#2466=B_SPLINE_CURVE_WITH_KNOTS('',3,(#109852,#109853,#109854,#109855,#109856,
#109857,#109858,#109859,#109860,#109861,#109862,#109863,#109864,#109865,
#109866,#109867,#109868,#109869,#109870,#109871,#109872,#109873,#109874,
#109875,#109876,#109877,#109878,#109879),.UNSPECIFIED.,.F.,.F.,(4,2,2,2,
2,2,2,2,2,2,2,2,2,4),(0.931170439482049,0.946077334530951,0.957538186455137,
0.969659736733055,0.987988431122021,1.03634818069539,1.08369048993003,1.13512985187121,
1.19024389724709,1.24943791437987,1.30707512832393,1.36096869048164,1.39504142334864,
1.39673482854036),.UNSPECIFIED.);
#2467=B_SPLINE_CURVE_WITH_KNOTS('',3,(#109882,#109883,#109884,#109885,#109886,
#109887,#109888,#109889,#109890,#109891,#109892,#109893,#109894,#109895,
#109896,#109897,#109898,#109899,#109900,#109901,#109902,#109903,#109904,
#109905,#109906,#109907,#109908,#109909),.UNSPECIFIED.,.F.,.F.,(4,2,2,2,
2,2,2,2,2,2,2,2,2,4),(0.402035858284301,0.415800106188637,0.426509562079159,
0.43449821732174,0.44316499473855,0.454821097473714,0.479978494161069,0.530831774585308,
0.574142313470446,0.620921348665322,0.671202766396292,0.721509774951859,
0.768376054624899,0.804067995108011),.UNSPECIFIED.);
#2468=B_SPLINE_CURVE_WITH_KNOTS('',3,(#109910,#109911,#109912,#109913,#109914,
#109915,#109916,#109917,#109918,#109919,#109920,#109921,#109922,#109923,
#109924,#109925,#109926,#109927,#109928,#109929,#109930,#109931,#109932,
#109933,#109934,#109935,#109936,#109937),.UNSPECIFIED.,.F.,.F.,(4,2,2,2,
2,2,2,2,2,2,2,2,2,4),(0.804068015337196,0.820830037169018,0.831725865127309,
0.840355281596958,0.849911251608451,0.865314090182635,0.912359544350536,
0.953570658305018,0.998400421083362,1.04651355615953,1.09728907212346,1.14674897700792,
1.19347446440925,1.20610385339231),.UNSPECIFIED.);
#2469=B_SPLINE_CURVE_WITH_KNOTS('',3,(#109940,#109941,#109942,#109943,#109944,
#109945,#109946,#109947,#109948,#109949,#109950,#109951,#109952,#109953,
#109954,#109955,#109956,#109957,#109958,#109959,#109960,#109961,#109962,
#109963,#109964,#109965,#109966,#109967,#109968,#109969),.UNSPECIFIED.,
 .F.,.F.,(4,2,2,2,2,2,2,2,2,2,2,2,2,2,4),(0.34693956539501,0.36351871144698,
0.376402246255229,0.383922554697919,0.390434897410649,0.398320444565317,
0.41279772900145,0.456696958114542,0.492818163098098,0.532197319465947,
0.574634286636639,0.61850585479356,0.649183604204981,0.668216244832537,
0.693788573117956),.UNSPECIFIED.);
#2470=B_SPLINE_CURVE_WITH_KNOTS('',3,(#109970,#109971,#109972,#109973,#109974,
#109975,#109976,#109977,#109978,#109979,#109980,#109981,#109982,#109983,
#109984,#109985,#109986,#109987,#109988,#109989,#109990,#109991,#109992,
#109993,#109994,#109995,#109996,#109997),.UNSPECIFIED.,.F.,.F.,(4,2,2,2,
2,2,2,2,2,2,2,2,2,4),(0.693788666223921,0.716636792221272,0.726516620727249,
0.732704302176124,0.739415944795447,0.748466294242799,0.768259990862704,
0.812205377250718,0.849077532443543,0.88904156018983,0.932010512859336,
0.975680172894089,1.01671881686369,1.04072813851297),.UNSPECIFIED.);
#2471=B_SPLINE_CURVE_WITH_KNOTS('',3,(#110000,#110001,#110002,#110003,#110004,
#110005,#110006,#110007,#110008,#110009,#110010,#110011,#110012,#110013,
#110014,#110015,#110016,#110017,#110018,#110019,#110020,#110021,#110022,
#110023,#110024,#110025,#110026,#110027,#110028,#110029),.UNSPECIFIED.,
 .F.,.F.,(4,2,2,2,2,2,2,2,2,2,2,2,2,2,4),(0.344949052494914,0.36277009235622,
0.381467624672727,0.388884092762833,0.394389517740211,0.400354875245585,
0.408399545858477,0.426069166833454,0.469389147836557,0.505710222697627,
0.545356716966147,0.588183386073944,0.630668972094002,0.656032036251321,
0.6898186201039),.UNSPECIFIED.);
#2472=B_SPLINE_CURVE_WITH_KNOTS('',3,(#110030,#110031,#110032,#110033,#110034,
#110035,#110036,#110037,#110038,#110039,#110040,#110041,#110042,#110043,
#110044,#110045,#110046,#110047,#110048,#110049,#110050,#110051,#110052,
#110053,#110054,#110055,#110056,#110057,#110058,#110059,#110060),
 .UNSPECIFIED.,.F.,.F.,(4,3,2,2,2,2,2,2,2,2,2,2,2,2,4),(0.6898186201039,
0.689820287363217,0.720993326898501,0.731680371989911,0.738253283448811,
0.744176013144634,0.751666615512782,0.766445212379684,0.809788249849371,
0.845546547900242,0.884630535928773,0.926803266506532,0.970599772849603,
1.01242230839075,1.03476933985813),.UNSPECIFIED.);
#2473=B_SPLINE_CURVE_WITH_KNOTS('',3,(#110063,#110064,#110065,#110066,#110067,
#110068,#110069,#110070,#110071,#110072,#110073,#110074,#110075,#110076,
#110077,#110078,#110079,#110080,#110081,#110082,#110083,#110084,#110085,
#110086,#110087,#110088,#110089,#110090,#110091,#110092),.UNSPECIFIED.,
 .F.,.F.,(4,2,2,2,2,2,2,2,2,2,2,2,2,2,4),(0.344940008736965,0.378978791644863,
0.42186508520073,0.431590749918263,0.437742985858769,0.442544553022841,
0.44782033022748,0.456311381108014,0.48343211103597,0.515569701577298,0.551845082220461,
0.591482902943101,0.634321511103674,0.660439052235908,0.689822751077019),
 .UNSPECIFIED.);
#2474=B_SPLINE_CURVE_WITH_KNOTS('',3,(#110093,#110094,#110095,#110096,#110097,
#110098,#110099,#110100,#110101,#110102,#110103,#110104,#110105,#110106,
#110107,#110108,#110109,#110110,#110111,#110112,#110113,#110114,#110115,
#110116,#110117,#110118,#110119,#110120,#110121,#110122,#110123,#110124,
#110125),.UNSPECIFIED.,.F.,.F.,(4,3,2,2,2,2,2,2,2,2,2,2,2,2,2,4),(0.689822751077019,
0.689835002982984,0.728744495340446,0.76747936074641,0.776814384144543,
0.782869367749044,0.787694633017288,0.793101248828574,0.802041370620515,
0.832608555074118,0.865362173435765,0.902043132002549,0.941969769687353,
0.985027673395759,1.02852816507098,1.03477501171995),.UNSPECIFIED.);
#2475=B_SPLINE_CURVE_WITH_KNOTS('',3,(#110128,#110129,#110130,#110131,#110132,
#110133,#110134,#110135,#110136,#110137,#110138,#110139,#110140,#110141,
#110142,#110143,#110144,#110145,#110146,#110147,#110148,#110149,#110150,
#110151,#110152,#110153,#110154,#110155,#110156,#110157,#110158,#110159,
#110160),.UNSPECIFIED.,.F.,.F.,(4,2,2,2,2,2,2,2,2,2,2,2,2,2,3,4),(0.347023138138081,
0.354237651152506,0.392088742983375,0.417111712806915,0.426077762137051,
0.43174994473942,0.436977598867684,0.44376256853267,0.45778036032763,0.501521672898848,
0.537374603000262,0.576570640714205,0.618850505784507,0.653291130836709,
0.693855228776299,0.693903487772775),.UNSPECIFIED.);
#2476=B_SPLINE_CURVE_WITH_KNOTS('',3,(#110161,#110162,#110163,#110164,#110165,
#110166,#110167,#110168,#110169,#110170,#110171,#110172,#110173,#110174,
#110175,#110176,#110177,#110178,#110179,#110180,#110181,#110182,#110183,
#110184,#110185,#110186,#110187,#110188),.UNSPECIFIED.,.F.,.F.,(4,2,2,2,
2,2,2,2,2,2,2,2,2,4),(0.693903487772775,0.729687754639204,0.761874414282563,
0.771942093684843,0.777899539963646,0.783079765382483,0.789502118333581,
0.801642899823187,0.845596548586892,0.881045805067327,0.91982886691259,
0.961612807804786,1.00557856818985,1.04087836691438),.UNSPECIFIED.);
#2477=B_SPLINE_CURVE_WITH_KNOTS('',3,(#110191,#110192,#110193,#110194,#110195,
#110196,#110197,#110198,#110199,#110200,#110201,#110202,#110203,#110204,
#110205,#110206,#110207,#110208,#110209,#110210,#110211,#110212,#110213,
#110214,#110215,#110216,#110217,#110218,#110219,#110220),.UNSPECIFIED.,
 .F.,.F.,(4,2,2,2,2,2,2,2,2,2,2,2,2,2,4),(0.402082644734097,0.408816886367671,
0.457317700146456,0.475413758181528,0.484000465094417,0.490648854483846,
0.497776850058018,0.508849809023471,0.540995027585967,0.579223696731807,
0.621922224793676,0.668212867966239,0.718001195146057,0.756613895926381,
0.804035907610257),.UNSPECIFIED.);
#2478=B_SPLINE_CURVE_WITH_KNOTS('',3,(#110221,#110222,#110223,#110224,#110225,
#110226,#110227,#110228,#110229,#110230,#110231,#110232,#110233,#110234,
#110235,#110236,#110237,#110238,#110239,#110240,#110241,#110242,#110243,
#110244,#110245,#110246,#110247,#110248,#110249,#110250,#110251),
 .UNSPECIFIED.,.F.,.F.,(4,3,2,2,2,2,2,2,2,2,2,2,2,2,4),(0.804035907610257,
0.804040984651415,0.850086369432104,0.873922371268176,0.884014085041587,
0.89028098025585,0.897048185533734,0.906140890385097,0.926032251354922,
0.977055761637495,1.0191917936117,1.06487574383506,1.11390884249085,1.16451044494518,
1.20612362938551),.UNSPECIFIED.);
#2479=B_SPLINE_CURVE_WITH_KNOTS('',3,(#110254,#110255,#110256,#110257,#110258,
#110259,#110260,#110261,#110262,#110263,#110264,#110265,#110266,#110267,
#110268,#110269,#110270,#110271,#110272,#110273,#110274,#110275,#110276,
#110277,#110278,#110279,#110280,#110281,#110282,#110283,#110284,#110285,
#110286),.UNSPECIFIED.,.F.,.F.,(4,2,2,2,2,2,2,2,2,2,2,2,2,2,3,4),(0.465697318151285,
0.500096550816189,0.530152083768842,0.542887027000964,0.550777921662509,
0.55927272797757,0.570621274065763,0.595067159352315,0.65402940437608,0.703342238243548,
0.756754657905659,0.814127098826639,0.865095529254773,0.894692705834994,
0.931141236328648,0.931163109251236),.UNSPECIFIED.);
#2480=B_SPLINE_CURVE_WITH_KNOTS('',3,(#110287,#110288,#110289,#110290,#110291,
#110292,#110293,#110294,#110295,#110296,#110297,#110298,#110299,#110300,
#110301,#110302,#110303,#110304,#110305,#110306,#110307,#110308,#110309,
#110310,#110311,#110312,#110313,#110314),.UNSPECIFIED.,.F.,.F.,(4,2,2,2,
2,2,2,2,2,2,2,2,2,4),(0.931163109251236,0.986893757473382,1.00378700412891,
1.01368892697709,1.02129904029214,1.03107558281521,1.04786913337837,1.10678708647645,
1.15462078504369,1.20659986804395,1.26232717177621,1.32099255779553,1.37806644213216,
1.39683855447993),.UNSPECIFIED.);
#2481=B_SPLINE_CURVE_WITH_KNOTS('',3,(#110317,#110318,#110319,#110320,#110321,
#110322,#110323,#110324,#110325,#110326,#110327,#110328,#110329,#110330,
#110331,#110332,#110333,#110334,#110335,#110336,#110337,#110338,#110339,
#110340,#110341,#110342,#110343,#110344),.UNSPECIFIED.,.F.,.F.,(4,2,2,2,
2,2,2,2,2,2,2,2,2,4),(0.4655389112447,0.488133130774159,0.506318884175181,
0.517142152662043,0.526626059065126,0.538230532411421,0.559797581148832,
0.618783918753435,0.667805538713148,0.720924860650082,0.777953615959564,
0.83642444066412,0.875349746240229,0.93113996876562),.UNSPECIFIED.);
#2482=B_SPLINE_CURVE_WITH_KNOTS('',3,(#110345,#110346,#110347,#110348,#110349,
#110350,#110351,#110352,#110353,#110354,#110355,#110356,#110357,#110358,
#110359,#110360,#110361,#110362,#110363,#110364,#110365,#110366,#110367,
#110368,#110369,#110370,#110371,#110372),.UNSPECIFIED.,.F.,.F.,(4,2,2,2,
2,2,2,2,2,2,2,2,2,4),(0.93113999918218,0.963154453507864,0.977016717729584,
0.986854762909184,0.996911582350658,1.01135266092654,1.04654269594155,1.09119591127059,
1.14061195756702,1.19389677378683,1.25097456683904,1.30939222705096,1.3649241947938,
1.39667888001032),.UNSPECIFIED.);
#2483=B_SPLINE_CURVE_WITH_KNOTS('',3,(#110382,#110383,#110384,#110385,#110386,
#110387,#110388,#110389,#110390,#110391,#110392,#110393,#110394,#110395,
#110396,#110397,#110398,#110399,#110400,#110401,#110402,#110403,#110404,
#110405,#110406,#110407,#110408,#110409,#110410,#110411,#110412,#110413,
#110414,#110415,#110416,#110417,#110418,#110419),.UNSPECIFIED.,.T.,.F.,
(4,2,2,2,2,2,2,2,2,2,2,2,2,2,2,2,2,2,4),(0.,0.0253587207966879,0.0757398285085816,
0.126070132097997,0.176266080606921,0.226299383634684,0.276249073740046,
0.326254642699978,0.376402382431699,0.401502370508004,0.426571573512854,
0.477394582349303,0.528028902540467,0.57881116631453,0.629741966063948,
0.68057107151679,0.731217559248426,0.7819629019431,0.804608887664541),
 .UNSPECIFIED.);
#2484=B_SPLINE_CURVE_WITH_KNOTS('',3,(#110423,#110424,#110425,#110426,#110427,
#110428,#110429,#110430,#110431,#110432,#110433,#110434,#110435,#110436,
#110437,#110438,#110439,#110440,#110441,#110442,#110443,#110444,#110445),
 .UNSPECIFIED.,.F.,.F.,(4,2,2,2,2,2,2,2,2,3,4),(0.213085231160066,0.229427465846964,
0.256360845004798,0.282978089057426,0.309527611387396,0.336016212989723,
0.362490334276596,0.389007528718512,0.415593427837248,0.42617576632081,
0.42617835082105),.UNSPECIFIED.);
#2485=B_SPLINE_CURVE_WITH_KNOTS('',3,(#110449,#110450,#110451,#110452,#110453,
#110454,#110455,#110456,#110457,#110458,#110459,#110460,#110461,#110462,
#110463,#110464,#110465,#110466,#110467,#110468),.UNSPECIFIED.,.F.,.F.,
(4,2,2,2,2,2,2,2,2,4),(0.42617835082105,0.439441496185428,0.466455555306613,
0.493421519222728,0.520432879955794,0.547485339174318,0.574506555632534,
0.6014753733821,0.628473697232218,0.639260997480876),.UNSPECIFIED.);
#2486=B_SPLINE_CURVE_WITH_KNOTS('',3,(#110472,#110473,#110474,#110475,#110476,
#110477,#110478,#110479,#110480,#110481,#110482,#110483,#110484,#110485,
#110486,#110487,#110488,#110489,#110490,#110491,#110492,#110493,#110494,
#110495,#110496,#110497,#110498,#110499,#110500,#110501,#110502,#110503,
#110504,#110505,#110506,#110507,#110508,#110509),.UNSPECIFIED.,.T.,.F.,
(4,2,2,2,2,2,2,2,2,2,2,2,2,2,2,2,2,2,4),(0.,0.0215934538029461,0.0661140688763958,
0.109673264959663,0.152976786454784,0.196013449229872,0.238933453610375,
0.281964346413397,0.325260417404302,0.347000989066419,0.368728099328494,
0.412825446316775,0.456665802011567,0.500491031429621,0.544396329252895,
0.587414183713088,0.631225382181991,0.675103653567844,0.694395412341892),
 .UNSPECIFIED.);
#2487=B_SPLINE_CURVE_WITH_KNOTS('',3,(#110513,#110514,#110515,#110516,#110517,
#110518,#110519,#110520,#110521,#110522,#110523,#110524,#110525,#110526,
#110527,#110528,#110529,#110530,#110531,#110532,#110533,#110534),
 .UNSPECIFIED.,.F.,.F.,(4,2,2,2,2,2,2,2,2,2,4),(0.157591377093445,0.158341318200066,
0.16816064064739,0.188318306898892,0.2082429048757,0.227875908952582,0.247403814330963,
0.266900129823757,0.28645832978064,0.306134210260318,0.315207466804691),
 .UNSPECIFIED.);
#2488=B_SPLINE_CURVE_WITH_KNOTS('',3,(#110538,#110539,#110540,#110541,#110542,
#110543,#110544,#110545,#110546,#110547,#110548,#110549,#110550,#110551,
#110552,#110553,#110554,#110555,#110556,#110557,#110558,#110559,#110560),
 .UNSPECIFIED.,.F.,.F.,(4,3,2,2,2,2,2,2,2,2,4),(0.315207466804691,0.315229215381257,
0.325074413465618,0.345142403734454,0.36514541055531,0.385129442882843,
0.404649613884746,0.424165788062158,0.443755125331743,0.463768996929674,
0.472820592474702),.UNSPECIFIED.);
#2489=B_SPLINE_CURVE_WITH_KNOTS('',3,(#110564,#110565,#110566,#110567,#110568,
#110569,#110570,#110571,#110572,#110573,#110574,#110575,#110576,#110577,
#110578,#110579,#110580,#110581,#110582,#110583,#110584,#110585,#110586,
#110587,#110588,#110589,#110590,#110591,#110592,#110593,#110594,#110595,
#110596,#110597,#110598,#110599,#110600,#110601),.UNSPECIFIED.,.T.,.F.,
(4,2,2,2,2,2,2,2,2,2,2,2,2,2,2,2,2,2,4),(0.,0.0214612457013718,0.0430041716204019,
0.0873575122693011,0.130712730392479,0.173621420731722,0.2161633020124,
0.258638327861848,0.301388430216311,0.344585415156887,0.366255653226389,
0.387851313185509,0.431696072327512,0.475306021742627,0.518888272730588,
0.561418888334619,0.604005607771101,0.647584473031916,0.690474393099494),
 .UNSPECIFIED.);
#2490=B_SPLINE_CURVE_WITH_KNOTS('',3,(#110605,#110606,#110607,#110608,#110609,
#110610,#110611,#110612,#110613,#110614,#110615,#110616,#110617,#110618,
#110619,#110620,#110621,#110622,#110623,#110624,#110625,#110626,#110627,
#110628,#110629),.UNSPECIFIED.,.F.,.F.,(4,2,2,2,2,2,2,2,2,2,3,4),(0.155294477826636,
0.155659400125146,0.165338299598688,0.175034361113789,0.194920097606448,
0.214541319872842,0.233821348963659,0.252953941695607,0.272074687541761,
0.29132605951052,0.310584998214978,0.310589086453876),.UNSPECIFIED.);
#2491=B_SPLINE_CURVE_WITH_KNOTS('',3,(#110633,#110634,#110635,#110636,#110637,
#110638,#110639,#110640,#110641,#110642,#110643,#110644,#110645,#110646,
#110647,#110648,#110649,#110650,#110651,#110652),.UNSPECIFIED.,.F.,.F.,
(4,2,2,2,2,2,2,2,2,4),(0.310589086453876,0.320305218454811,0.330010867645859,
0.349792458885214,0.369503570696552,0.388938417010325,0.408070037520553,
0.427213089555852,0.446492546606876,0.465879476041615),.UNSPECIFIED.);
#2492=B_SPLINE_CURVE_WITH_KNOTS('',3,(#110656,#110657,#110658,#110659,#110660,
#110661,#110662,#110663,#110664,#110665,#110666,#110667,#110668,#110669,
#110670,#110671,#110672,#110673,#110674,#110675,#110676,#110677,#110678,
#110679,#110680,#110681,#110682,#110683,#110684,#110685,#110686,#110687,
#110688,#110689,#110690,#110691,#110692,#110693),.UNSPECIFIED.,.T.,.F.,
(4,2,2,2,2,2,2,2,2,2,2,2,2,2,2,2,2,2,4),(0.,0.0582499854078214,0.116522238011401,
0.174719222883445,0.232763101450122,0.290685326407376,0.348596993560137,
0.406576740290978,0.435566714351364,0.494495631365087,0.552987315365781,
0.611558833999642,0.670345355331475,0.729066826381109,0.78756171029075,
0.846156998753239,0.874931172542359,0.903174012205886,0.93172187928848),
 .UNSPECIFIED.);
#2493=B_SPLINE_CURVE_WITH_KNOTS('',3,(#110697,#110698,#110699,#110700,#110701,
#110702,#110703,#110704,#110705,#110706,#110707,#110708,#110709,#110710,
#110711,#110712,#110713,#110714,#110715,#110716,#110717,#110718),
 .UNSPECIFIED.,.F.,.F.,(4,2,2,2,2,2,2,2,2,2,4),(0.276825859161365,0.297043390131478,
0.331626580694953,0.366194217943258,0.400710187129129,0.435170426794847,
0.469611031748545,0.504073425287484,0.521299803107865,0.537372852441424,
0.55357036764084),.UNSPECIFIED.);
#2494=B_SPLINE_CURVE_WITH_KNOTS('',3,(#110722,#110723,#110724,#110725,#110726,
#110727,#110728,#110729,#110730,#110731,#110732,#110733,#110734,#110735,
#110736,#110737,#110738,#110739,#110740,#110741),.UNSPECIFIED.,.F.,.F.,
(4,2,2,2,2,2,2,2,2,4),(0.553570660833043,0.588585516849723,0.623535548686362,
0.658551470263866,0.693596719240443,0.728577625844064,0.763532714810859,
0.798639038192274,0.816043463348951,0.830396226802205),.UNSPECIFIED.);
#2495=B_SPLINE_CURVE_WITH_KNOTS('',3,(#110745,#110746,#110747,#110748,#110749,
#110750,#110751,#110752,#110753,#110754,#110755,#110756,#110757,#110758,
#110759,#110760,#110761,#110762,#110763,#110764,#110765,#110766,#110767,
#110768,#110769,#110770,#110771,#110772,#110773,#110774,#110775,#110776,
#110777,#110778,#110779,#110780),.UNSPECIFIED.,.T.,.F.,(4,2,2,2,2,2,2,2,
2,2,2,2,2,2,2,2,2,4),(0.,0.0503768236674881,0.100697265705858,0.150882364943078,
0.200910039641612,0.250863071799662,0.300878991841609,0.351037208469142,
0.376138911045814,0.401180140933725,0.45196140826745,0.502592407894745,
0.553406592994723,0.60437887729313,0.655232719281932,0.70587844620255,0.756604415957716,
0.804713332817945),.UNSPECIFIED.);
#2496=B_SPLINE_CURVE_WITH_KNOTS('',3,(#110784,#110785,#110786,#110787,#110788,
#110789,#110790,#110791,#110792,#110793,#110794,#110795,#110796,#110797,
#110798,#110799,#110800,#110801,#110802,#110803,#110804,#110805,#110806,
#110807,#110808),.UNSPECIFIED.,.F.,.F.,(4,2,2,2,2,2,2,2,2,2,3,4),(0.213125454324095,
0.215371214439484,0.242304080051861,0.26891712435903,0.295463050658844,
0.321950717827531,0.348427104398956,0.374948460855996,0.401537986608032,
0.413805283512627,0.426168952202461,0.426174000047882),.UNSPECIFIED.);
#2497=B_SPLINE_CURVE_WITH_KNOTS('',3,(#110812,#110813,#110814,#110815,#110816,
#110817,#110818,#110819,#110820,#110821,#110822,#110823,#110824,#110825,
#110826,#110827,#110828,#110829),.UNSPECIFIED.,.F.,.F.,(4,2,2,2,2,2,2,2,
4),(0.426174000047882,0.453163023079439,0.480127907810925,0.507155788480461,
0.533952061349386,0.560478308801999,0.587447628308409,0.614431474663807,
0.639294406526556),.UNSPECIFIED.);
#2498=B_SPLINE_CURVE_WITH_KNOTS('',3,(#110833,#110834,#110835,#110836,#110837,
#110838,#110839,#110840,#110841,#110842,#110843,#110844,#110845,#110846,
#110847,#110848,#110849,#110850,#110851,#110852,#110853,#110854,#110855,
#110856,#110857,#110858,#110859,#110860,#110861,#110862,#110863,#110864,
#110865,#110866,#110867,#110868,#110869,#110870),.UNSPECIFIED.,.T.,.F.,
(4,2,2,2,2,2,2,2,2,2,2,2,2,2,2,2,2,2,4),(0.,0.0444221121400932,0.0879541817963996,
0.131227015999418,0.174246979918824,0.217174048974236,0.260231920457301,
0.303559228338858,0.325306871790306,0.346970541213297,0.390946973288773,
0.434747171355873,0.478633478836622,0.521609326830897,0.564635515872938,
0.608480355472813,0.652299252145619,0.673231330408672,0.694389830450528),
 .UNSPECIFIED.);
#2499=B_SPLINE_CURVE_WITH_KNOTS('',3,(#110874,#110875,#110876,#110877,#110878,
#110879,#110880,#110881,#110882,#110883,#110884,#110885,#110886,#110887,
#110888,#110889,#110890,#110891,#110892,#110893,#110894,#110895),
 .UNSPECIFIED.,.F.,.F.,(4,2,2,2,2,2,2,2,2,2,4),(0.157589267359033,0.158005279271924,
0.178114857305211,0.198037545113508,0.217659078264535,0.237181560870524,
0.256681548189167,0.276250496936562,0.295938152700304,0.305537860047768,
0.315206514186509),.UNSPECIFIED.);
#2500=B_SPLINE_CURVE_WITH_KNOTS('',3,(#110899,#110900,#110901,#110902,#110903,
#110904,#110905,#110906,#110907,#110908,#110909,#110910,#110911,#110912,
#110913,#110914,#110915,#110916,#110917,#110918,#110919,#110920,#110921),
 .UNSPECIFIED.,.F.,.F.,(4,3,2,2,2,2,2,2,2,2,4),(0.315206514186509,0.315228106062157,
0.335243855233202,0.355229872898987,0.375034891987949,0.39454965103334,
0.414070002826143,0.43367079485033,0.453658486096216,0.463440026256045,
0.472817373421189),.UNSPECIFIED.);
#2501=B_SPLINE_CURVE_WITH_KNOTS('',3,(#110925,#110926,#110927,#110928,#110929,
#110930,#110931,#110932,#110933,#110934,#110935,#110936,#110937,#110938,
#110939,#110940,#110941,#110942,#110943,#110944,#110945,#110946,#110947,
#110948,#110949,#110950,#110951,#110952,#110953,#110954,#110955,#110956,
#110957,#110958,#110959,#110960,#110961,#110962),.UNSPECIFIED.,.T.,.F.,
(4,2,2,2,2,2,2,2,2,2,2,2,2,2,2,2,2,2,4),(0.,0.0215520464773449,0.065916778292889,
0.109258524694745,0.152151785274527,0.194685629726144,0.237165327483375,
0.279930295138766,0.323143228583621,0.344811565913954,0.366403507243528,
0.410241083863158,0.453847992476275,0.497429011858637,0.539957033885482,
0.582551741103232,0.626132369502366,0.6698761895927,0.69048940316824),
 .UNSPECIFIED.);
#2502=B_SPLINE_CURVE_WITH_KNOTS('',3,(#110966,#110967,#110968,#110969,#110970,
#110971,#110972,#110973,#110974,#110975,#110976,#110977,#110978,#110979,
#110980,#110981,#110982,#110983,#110984,#110985,#110986,#110987),
 .UNSPECIFIED.,.F.,.F.,(4,2,2,2,2,2,2,2,2,2,4),(0.15527235737458,0.15562510787596,
0.165323609967748,0.185212103287073,0.204826616573261,0.224100586518285,
0.243230509120738,0.26235370154504,0.28161134459152,0.30106539687992,0.31057081404642),
 .UNSPECIFIED.);
#2503=B_SPLINE_CURVE_WITH_KNOTS('',3,(#110991,#110992,#110993,#110994,#110995,
#110996,#110997,#110998,#110999,#111000,#111001,#111002,#111003,#111004,
#111005,#111006,#111007,#111008,#111009,#111010,#111011,#111012,#111013),
 .UNSPECIFIED.,.F.,.F.,(4,3,2,2,2,2,2,2,2,2,4),(0.31057081404642,0.310589850236165,
0.32029547338224,0.340076326550382,0.359786151240218,0.379216021927432,
0.398345929856394,0.417491927740968,0.436777439352559,0.456533677744053,
0.465862207610745),.UNSPECIFIED.);
#2504=B_SPLINE_CURVE_WITH_KNOTS('',3,(#111017,#111018,#111019,#111020,#111021,
#111022,#111023,#111024,#111025,#111026,#111027,#111028,#111029,#111030,
#111031,#111032,#111033,#111034,#111035,#111036,#111037,#111038,#111039,
#111040,#111041,#111042,#111043,#111044,#111045,#111046,#111047,#111048,
#111049,#111050,#111051,#111052,#111053,#111054),.UNSPECIFIED.,.T.,.F.,
(4,2,2,2,2,2,2,2,2,2,2,2,2,2,2,2,2,2,4),(0.,0.0582371853616322,0.116450034307396,
0.174555153981211,0.23253603852723,0.290470301636954,0.348447688277155,
0.377437572006861,0.406430276039093,0.465167898343824,0.523607434262112,
0.582288349171024,0.641268831623812,0.700144809512642,0.758670415181914,
0.817168437078618,0.845875575798632,0.875163161983379,0.931710252415266),
 .UNSPECIFIED.);
#2505=B_SPLINE_CURVE_WITH_KNOTS('',3,(#111058,#111059,#111060,#111061,#111062,
#111063,#111064,#111065,#111066,#111067,#111068,#111069,#111070,#111071,
#111072,#111073,#111074,#111075,#111076,#111077,#111078,#111079,#111080,
#111081,#111082),.UNSPECIFIED.,.F.,.F.,(4,2,2,2,2,2,2,2,2,2,3,4),(0.276799012407407,
0.279373782652995,0.313936794852817,0.348484301688893,0.382991613305011,
0.417459748808092,0.45192017602727,0.48640262407376,0.50363241062791,0.520852093736164,
0.553556515029853,0.55355923315894),.UNSPECIFIED.);
#2506=B_SPLINE_CURVE_WITH_KNOTS('',3,(#111086,#111087,#111088,#111089,#111090,
#111091,#111092,#111093,#111094,#111095,#111096,#111097,#111098,#111099,
#111100,#111101,#111102,#111103,#111104,#111105),.UNSPECIFIED.,.F.,.F.,
(4,2,2,2,2,2,2,2,2,4),(0.55355923315894,0.588486820049772,0.623528572740515,
0.658687237671087,0.693800354600396,0.728770060347164,0.763712953575019,
0.780829430331441,0.798001660236641,0.83035552743726),.UNSPECIFIED.);
#2507=B_SPLINE_CURVE_WITH_KNOTS('',3,(#111109,#111110,#111111,#111112,#111113,
#111114,#111115,#111116,#111117,#111118,#111119,#111120,#111121,#111122,
#111123,#111124,#111125,#111126,#111127,#111128,#111129,#111130,#111131,
#111132,#111133,#111134,#111135,#111136,#111137,#111138,#111139,#111140,
#111141,#111142,#111143,#111144),.UNSPECIFIED.,.T.,.F.,(4,2,2,2,2,2,2,2,
2,2,2,2,2,2,2,2,2,4),(0.,0.0503765293579072,0.100656386784499,0.150767302359921,
0.200734910020674,0.250685919670086,0.300751653603399,0.35095811132866,
0.376056517716232,0.426926457491189,0.477568603688572,0.528302799585843,
0.579143561840979,0.629894549187007,0.680535051806248,0.73136306480552,
0.782694491287284,0.80473018173603),.UNSPECIFIED.);
#2508=B_SPLINE_CURVE_WITH_KNOTS('',3,(#111148,#111149,#111150,#111151,#111152,
#111153,#111154,#111155,#111156,#111157,#111158,#111159,#111160,#111161,
#111162,#111163,#111164,#111165,#111166,#111167),.UNSPECIFIED.,.F.,.F.,
(4,2,2,2,2,2,2,2,2,4),(0.213098726156546,0.215970507757757,0.242617902005601,
0.269207806476468,0.295724361337248,0.322195200337876,0.348679383881839,
0.375225908894206,0.401835845995312,0.426189984379948),.UNSPECIFIED.);
#2509=B_SPLINE_CURVE_WITH_KNOTS('',3,(#111171,#111172,#111173,#111174,#111175,
#111176,#111177,#111178,#111179,#111180,#111181,#111182,#111183,#111184,
#111185,#111186,#111187,#111188,#111189,#111190,#111191),.UNSPECIFIED.,
 .F.,.F.,(4,3,2,2,2,2,2,2,2,4),(0.426189984379948,0.426215668917109,0.453208711882292,
0.480176759933483,0.507173805734186,0.534171874901274,0.561140699681476,
0.588130649676459,0.615239336311902,0.639314395073655),.UNSPECIFIED.);
#2510=B_SPLINE_CURVE_WITH_KNOTS('',3,(#111195,#111196,#111197,#111198,#111199,
#111200,#111201,#111202,#111203,#111204,#111205,#111206,#111207,#111208,
#111209,#111210,#111211,#111212,#111213,#111214,#111215,#111216,#111217,
#111218,#111219,#111220,#111221,#111222,#111223,#111224,#111225,#111226,
#111227,#111228,#111229,#111230,#111231,#111232),.UNSPECIFIED.,.T.,.F.,
(4,2,2,2,2,2,2,2,2,2,2,2,2,2,2,2,2,2,4),(0.,0.0436396354015875,0.0870799379946624,
0.130235175112472,0.173181603494129,0.216128697217889,0.259286147781706,
0.302719831957823,0.324465331746154,0.368595894415476,0.412446137360158,
0.456247245545887,0.500100201234702,0.543937122812399,0.58773303976263,
0.63165494060563,0.653207446330335,0.673701504443971,0.694392975330147),
 .UNSPECIFIED.);
#2511=B_SPLINE_CURVE_WITH_KNOTS('',3,(#111236,#111237,#111238,#111239,#111240,
#111241,#111242,#111243,#111244,#111245,#111246,#111247,#111248,#111249,
#111250,#111251,#111252,#111253,#111254,#111255,#111256,#111257),
 .UNSPECIFIED.,.F.,.F.,(4,2,2,2,2,2,2,2,2,2,4),(0.157608270286503,0.168928237568431,
0.188674330321961,0.208302465762515,0.227826612069672,0.247322672121388,
0.266884223982705,0.286564705052486,0.296430638563966,0.305790479364867,
0.315202716294224),.UNSPECIFIED.);
#2512=B_SPLINE_CURVE_WITH_KNOTS('',3,(#111261,#111262,#111263,#111264,#111265,
#111266,#111267,#111268,#111269,#111270,#111271,#111272,#111273,#111274,
#111275,#111276,#111277,#111278,#111279,#111280,#111281,#111282,#111283),
 .UNSPECIFIED.,.F.,.F.,(4,3,2,2,2,2,2,2,2,2,4),(0.315202716294224,0.315228523372249,
0.335270894652026,0.355254388730732,0.375013449023108,0.394520810149056,
0.414067151678346,0.434066258167069,0.454138928812652,0.463973627677658,
0.472836793658752),.UNSPECIFIED.);
#2513=B_SPLINE_CURVE_WITH_KNOTS('',3,(#111287,#111288,#111289,#111290,#111291,
#111292,#111293,#111294,#111295,#111296,#111297,#111298,#111299,#111300,
#111301,#111302,#111303,#111304,#111305,#111306,#111307,#111308,#111309,
#111310,#111311,#111312,#111313,#111314,#111315,#111316,#111317,#111318,
#111319,#111320,#111321,#111322,#111323,#111324),.UNSPECIFIED.,.T.,.F.,
(4,2,2,2,2,2,2,2,2,2,2,2,2,2,2,2,2,2,4),(0.,0.044308474695846,0.0876221732407881,
0.13048794984384,0.173010584725196,0.215501776298411,0.258294467524509,
0.301535055508773,0.323165493512123,0.34471113614295,0.38847500202065,0.432069843045601,
0.475261647497953,0.517783869440572,0.560390231176503,0.603979847218741,
0.647677207401233,0.668966276445715,0.690485997484513),.UNSPECIFIED.);
#2514=B_SPLINE_CURVE_WITH_KNOTS('',3,(#111328,#111329,#111330,#111331,#111332,
#111333,#111334,#111335,#111336,#111337,#111338,#111339,#111340,#111341,
#111342,#111343,#111344,#111345,#111346,#111347,#111348,#111349),
 .UNSPECIFIED.,.F.,.F.,(4,2,2,2,2,2,2,2,2,2,4),(0.155266549715351,0.155540359583602,
0.175401508132681,0.195010291008741,0.214273102592753,0.233399032217858,
0.252527597849283,0.271796998188979,0.291262445086705,0.300880271086537,
0.310565043388772),.UNSPECIFIED.);
#2515=B_SPLINE_CURVE_WITH_KNOTS('',3,(#111353,#111354,#111355,#111356,#111357,
#111358,#111359,#111360,#111361,#111362,#111363,#111364,#111365,#111366,
#111367,#111368,#111369,#111370,#111371,#111372,#111373,#111374,#111375),
 .UNSPECIFIED.,.F.,.F.,(4,3,2,2,2,2,2,2,2,2,4),(0.310565043388772,0.310589642487775,
0.330339397260518,0.350044366011474,0.369470075015529,0.388596515754746,
0.407748711655326,0.427046686185302,0.446782028837706,0.456448834828453,
0.465856192203126),.UNSPECIFIED.);
#2516=B_SPLINE_CURVE_WITH_KNOTS('',3,(#111379,#111380,#111381,#111382,#111383,
#111384,#111385,#111386,#111387,#111388,#111389,#111390,#111391,#111392,
#111393,#111394,#111395,#111396,#111397,#111398,#111399,#111400,#111401,
#111402,#111403,#111404,#111405,#111406,#111407,#111408,#111409,#111410,
#111411,#111412,#111413,#111414,#111415,#111416),.UNSPECIFIED.,.T.,.F.,
(4,2,2,2,2,2,2,2,2,2,2,2,2,2,2,2,2,2,4),(0.,0.0582746652411334,0.116465563883562,
0.174498657639209,0.232413193768181,0.290323519241188,0.348304847203968,
0.37729479476534,0.436198928686154,0.49468657172654,0.553261258987217,0.612031433556264,
0.670719397047039,0.729201952557845,0.787836578600544,0.816640912143595,
0.845923968771257,0.90415568160122,0.931717558493197),.UNSPECIFIED.);
#2517=B_SPLINE_CURVE_WITH_KNOTS('',3,(#111420,#111421,#111422,#111423,#111424,
#111425,#111426,#111427,#111428,#111429,#111430,#111431,#111432,#111433,
#111434,#111435,#111436,#111437,#111438,#111439,#111440,#111441),
 .UNSPECIFIED.,.F.,.F.,(4,2,2,2,2,2,2,2,2,2,4),(0.276824259036896,0.296611116807084,
0.331178721594792,0.365691854475663,0.400148469904013,0.434586793442788,
0.469048541672308,0.486274882510752,0.503503889308575,0.53860420639192,
0.553568065350035),.UNSPECIFIED.);
#2518=B_SPLINE_CURVE_WITH_KNOTS('',3,(#111445,#111446,#111447,#111448,#111449,
#111450,#111451,#111452,#111453,#111454,#111455,#111456,#111457,#111458,
#111459,#111460,#111461,#111462,#111463,#111464),.UNSPECIFIED.,.F.,.F.,
(4,2,2,2,2,2,2,2,2,4),(0.553568655458047,0.588517511821428,0.623525749772073,
0.658555918364597,0.693525509166112,0.728486932769869,0.763618198128497,
0.781022020612757,0.815594259375338,0.830392914494943),.UNSPECIFIED.);
#2519=B_SPLINE_CURVE_WITH_KNOTS('',3,(#111468,#111469,#111470,#111471,#111472,
#111473,#111474,#111475,#111476,#111477,#111478,#111479,#111480,#111481,
#111482,#111483,#111484,#111485,#111486,#111487,#111488,#111489,#111490,
#111491,#111492,#111493,#111494,#111495,#111496,#111497,#111498,#111499,
#111500,#111501,#111502,#111503),.UNSPECIFIED.,.T.,.F.,(4,2,2,2,2,2,2,2,
2,2,2,2,2,2,2,2,2,4),(0.,0.0503397569852893,0.100535814375046,0.150559311436999,
0.20049644388078,0.250492956056916,0.300635695532588,0.325734796020786,
0.350832855894969,0.401702116132417,0.452343313876895,0.503069511784625,
0.553891621921385,0.60462388767292,0.655263863923187,0.706116496828786,
0.757483229007975,0.804696187913725),.UNSPECIFIED.);
#2520=B_SPLINE_CURVE_WITH_KNOTS('',3,(#111507,#111508,#111509,#111510,#111511,
#111512,#111513,#111514,#111515,#111516,#111517,#111518,#111519,#111520,
#111521,#111522,#111523,#111524,#111525,#111526,#111527,#111528,#111529),
 .UNSPECIFIED.,.F.,.F.,(4,2,2,2,2,2,2,2,2,3,4),(0.213084510884075,0.228781186975439,
0.255371494150004,0.281887710763666,0.308357606751256,0.334840690693978,
0.361386330906224,0.387995767314121,0.41510213099284,0.426162916715676,
0.426168100816612),.UNSPECIFIED.);
#2521=B_SPLINE_CURVE_WITH_KNOTS('',3,(#111533,#111534,#111535,#111536,#111537,
#111538,#111539,#111540,#111541,#111542,#111543,#111544,#111545,#111546,
#111547,#111548,#111549,#111550,#111551,#111552),.UNSPECIFIED.,.F.,.F.,
(4,2,2,2,2,2,2,2,2,4),(0.426168100816612,0.453130885029272,0.480106246397837,
0.507100150030191,0.53407533862366,0.561043554729105,0.588091928815527,
0.601349529885376,0.628296013507661,0.639247427599751),.UNSPECIFIED.);
#2522=B_SPLINE_CURVE_WITH_KNOTS('',3,(#111556,#111557,#111558,#111559,#111560,
#111561,#111562,#111563,#111564,#111565,#111566,#111567,#111568,#111569,
#111570,#111571,#111572,#111573,#111574,#111575,#111576,#111577,#111578,
#111579,#111580,#111581,#111582,#111583,#111584,#111585,#111586,#111587,
#111588,#111589,#111590,#111591,#111592,#111593),.UNSPECIFIED.,.T.,.F.,
(4,2,2,2,2,2,2,2,2,2,2,2,2,2,2,2,2,2,4),(0.,0.0435250099426588,0.0867875676414407,
0.129798831049099,0.172723528677881,0.215785743787518,0.259119343545877,
0.280868720015448,0.302536290796754,0.346522406274042,0.390327377842269,
0.434204529765891,0.477178955585274,0.520208273340797,0.564038055478109,
0.607876492390102,0.6293685607735,0.650934887956273,0.694354039347353),
 .UNSPECIFIED.);
#2523=B_SPLINE_CURVE_WITH_KNOTS('',3,(#111597,#111598,#111599,#111600,#111601,
#111602,#111603,#111604,#111605,#111606,#111607,#111608,#111609,#111610,
#111611,#111612,#111613,#111614,#111615,#111616,#111617,#111618,#111619,
#111620,#111621),.UNSPECIFIED.,.F.,.F.,(4,2,2,2,2,2,2,2,2,2,3,4),(0.157609960982023,
0.158131914212271,0.178047596316255,0.197664157824957,0.21718321769825,
0.236683024193072,0.256254661663229,0.275945553163195,0.2857852745923,0.295605663211171,
0.315211906754256,0.315215197496655),.UNSPECIFIED.);
#2524=B_SPLINE_CURVE_WITH_KNOTS('',3,(#111625,#111626,#111627,#111628,#111629,
#111630,#111631,#111632,#111633,#111634,#111635,#111636,#111637,#111638,
#111639,#111640,#111641,#111642,#111643,#111644),.UNSPECIFIED.,.F.,.F.,
(4,2,2,2,2,2,2,2,2,4),(0.315215197496655,0.335200466876354,0.354999433605467,
0.374512449736718,0.394033699253622,0.413636951394353,0.433631734481444,
0.443418967878,0.453219950155937,0.472821867736279),.UNSPECIFIED.);
#2525=B_SPLINE_CURVE_WITH_KNOTS('',3,(#111648,#111649,#111650,#111651,#111652,
#111653,#111654,#111655,#111656,#111657,#111658,#111659,#111660,#111661,
#111662,#111663,#111664,#111665,#111666,#111667,#111668,#111669,#111670,
#111671,#111672,#111673,#111674,#111675,#111676,#111677,#111678,#111679,
#111680,#111681,#111682,#111683,#111684,#111685),.UNSPECIFIED.,.T.,.F.,
(4,2,2,2,2,2,2,2,2,2,2,2,2,2,2,2,2,2,4),(0.,0.0435158903681535,0.0866337303822979,
0.129311950410083,0.17176772862335,0.214353892471028,0.257343254730134,
0.300752733852546,0.322381697566155,0.366274614380129,0.409883810353136,
0.453406609581401,0.495934191090317,0.538530090897993,0.582105934721859,
0.625923161624818,0.64744336097096,0.66884623605417,0.69046738873967),
 .UNSPECIFIED.);
#2526=B_SPLINE_CURVE_WITH_KNOTS('',3,(#111689,#111690,#111691,#111692,#111693,
#111694,#111695,#111696,#111697,#111698,#111699,#111700,#111701,#111702,
#111703,#111704,#111705,#111706,#111707,#111708,#111709,#111710,#111711,
#111712,#111713),.UNSPECIFIED.,.F.,.F.,(4,2,2,2,2,2,2,2,2,2,3,4),(0.15531487351589,
0.166145970728797,0.185609441146789,0.204874632650298,0.223999607628438,
0.243124535499743,0.262389220003626,0.281850923436399,0.291587450265206,
0.301045446444696,0.310583538395292,0.310587695933181),.UNSPECIFIED.);
#2527=B_SPLINE_CURVE_WITH_KNOTS('',3,(#111717,#111718,#111719,#111720,#111721,
#111722,#111723,#111724,#111725,#111726,#111727,#111728,#111729,#111730,
#111731,#111732,#111733,#111734,#111735,#111736),.UNSPECIFIED.,.F.,.F.,
(4,2,2,2,2,2,2,2,2,4),(0.310587695933181,0.330338548490155,0.35001160002629,
0.36918336873163,0.388303018538272,0.407509226017143,0.427247589363119,
0.447088430248727,0.456810155929384,0.465898411911182),.UNSPECIFIED.);
#2528=B_SPLINE_CURVE_WITH_KNOTS('',3,(#111740,#111741,#111742,#111743,#111744,
#111745,#111746,#111747,#111748,#111749,#111750,#111751,#111752,#111753,
#111754,#111755,#111756,#111757,#111758,#111759,#111760,#111761,#111762,
#111763,#111764,#111765,#111766,#111767,#111768,#111769,#111770,#111771,
#111772,#111773,#111774,#111775,#111776,#111777),.UNSPECIFIED.,.T.,.F.,
(4,2,2,2,2,2,2,2,2,2,2,2,2,2,2,2,2,2,4),(0.,0.0579456402909644,0.0869299048751541,
0.115920063309306,0.174806990420041,0.233290522899272,0.291875001059739,
0.350660758745357,0.409359852180272,0.467844120994597,0.526472280441444,
0.555272349874393,0.584555610575361,0.642786260517934,0.701059261140235,
0.759300709458156,0.817409370762721,0.875368479051853,0.931707159703552),
 .UNSPECIFIED.);
#2529=B_SPLINE_CURVE_WITH_KNOTS('',3,(#111781,#111782,#111783,#111784,#111785,
#111786,#111787,#111788,#111789,#111790,#111791,#111792,#111793,#111794,
#111795,#111796,#111797,#111798,#111799,#111800),.UNSPECIFIED.,.F.,.F.,
(4,2,2,2,2,2,2,2,2,4),(1.00000028111068E-6,0.0347832075796592,0.0692716651495764,
0.103819772803296,0.13840130343469,0.172863389577014,0.190089620355572,
0.207318502211029,0.242417063886181,0.276778761880576),.UNSPECIFIED.);
#2530=B_SPLINE_CURVE_WITH_KNOTS('',3,(#111804,#111805,#111806,#111807,#111808,
#111809,#111810,#111811,#111812,#111813,#111814,#111815,#111816,#111817,
#111818,#111819,#111820,#111821,#111822,#111823,#111824,#111825,#111826,
#111827,#111828,#111829,#111830,#111831,#111832,#111833,#111834,#111835,
#111836,#111837,#111838,#111839,#111840,#111841,#111842,#111843,#111844,
#111845,#111846,#111847,#111848,#111849,#111850,#111851,#111852,#111853,
#111854,#111855,#111856,#111857,#111858,#111859,#111860,#111861,#111862,
#111863,#111864,#111865,#111866,#111867,#111868,#111869,#111870,#111871,
#111872,#111873,#111874,#111875,#111876,#111877,#111878,#111879,#111880,
#111881,#111882),.UNSPECIFIED.,.F.,.F.,(4,3,3,3,3,3,3,3,3,3,3,3,3,3,3,3,
3,3,3,3,3,3,3,3,3,3,4),(0.00274647550789723,0.00284764836235053,0.00294876159984055,
0.00304994614202459,0.00308970325655458,0.00318942908487613,0.00328907626887442,
0.00338877449852303,0.00343293100521208,0.00354315533571446,0.00365327844248592,
0.00376338004483701,0.00377615875386958,0.0039686408465685,0.00411938650252707,
0.00426424510927638,0.00441595944867224,0.00446261425118457,0.00458541711012655,
0.00470860724668196,0.00480584199984207,0.00493281230714532,0.00505965424824699,
0.00518600265972549,0.00531190386550827,0.00543695346148025,0.00549229749715719),
 .UNSPECIFIED.);
#2531=B_SPLINE_CURVE_WITH_KNOTS('',3,(#111886,#111887,#111888,#111889,#111890,
#111891,#111892,#111893,#111894,#111895,#111896,#111897,#111898,#111899,
#111900,#111901,#111902,#111903,#111904,#111905,#111906,#111907,#111908,
#111909,#111910,#111911,#111912,#111913,#111914,#111915,#111916,#111917,
#111918,#111919,#111920,#111921),.UNSPECIFIED.,.T.,.F.,(4,2,2,2,2,2,2,2,
2,2,2,2,2,2,2,2,2,4),(0.,0.050238053143519,0.100318703593234,0.150284930734814,
0.200263745526201,0.250367992087392,0.30059723478709,0.351510110444586,
0.402132532931605,0.452865784267353,0.503834596479786,0.554795405381783,
0.605516639507723,0.656143227180573,0.680951395143589,0.705853156657982,
0.756739251203461,0.804680497302985),.UNSPECIFIED.);
#2532=B_SPLINE_CURVE_WITH_KNOTS('',3,(#111925,#111926,#111927,#111928,#111929,
#111930,#111931,#111932,#111933,#111934,#111935,#111936,#111937,#111938,
#111939,#111940,#111941,#111942,#111943,#111944,#111945,#111946,#111947),
 .UNSPECIFIED.,.F.,.F.,(4,2,2,2,2,2,2,2,2,3,4),(0.2131238921346,0.214468422234068,
0.241041142260569,0.267548108379182,0.294021969529815,0.320519566555282,
0.347081755444668,0.373699970899426,0.400716003372662,0.426139175217478,
0.426214998931696),.UNSPECIFIED.);
#2533=B_SPLINE_CURVE_WITH_KNOTS('',3,(#111951,#111952,#111953,#111954,#111955,
#111956,#111957,#111958,#111959,#111960,#111961,#111962,#111963,#111964,
#111965,#111966,#111967,#111968,#111969,#111970),.UNSPECIFIED.,.F.,.F.,
(4,2,2,2,2,2,2,2,2,4),(0.426214998931696,0.453141486117911,0.479941628222141,
0.506446749253699,0.533446181809698,0.560399835109198,0.573588277851575,
0.586799440471832,0.61397554918602,0.639263067352078),.UNSPECIFIED.);
#2534=B_SPLINE_CURVE_WITH_KNOTS('',3,(#111974,#111975,#111976,#111977,#111978,
#111979,#111980,#111981,#111982,#111983,#111984,#111985,#111986,#111987,
#111988,#111989,#111990,#111991,#111992,#111993,#111994,#111995,#111996,
#111997,#111998,#111999,#112000,#112001,#112002,#112003,#112004,#112005,
#112006,#112007,#112008,#112009,#112010,#112011),.UNSPECIFIED.,.T.,.F.,
(4,2,2,2,2,2,2,2,2,2,2,2,2,2,2,2,2,2,4),(0.,0.0434332594561585,0.0865773364499496,
0.129513968405876,0.17245727714254,0.215616554324647,0.259052653928386,
0.280820020239544,0.324985455094301,0.368839855016106,0.412603610869772,
0.456387211561026,0.500159730990598,0.543941426909056,0.587917004107691,
0.609507132339805,0.631194826658406,0.675273884169567,0.694350838467621),
 .UNSPECIFIED.);
#2535=B_SPLINE_CURVE_WITH_KNOTS('',3,(#112015,#112016,#112017,#112018,#112019,
#112020,#112021,#112022,#112023,#112024,#112025,#112026,#112027,#112028,
#112029,#112030,#112031,#112032,#112033,#112034,#112035,#112036),
 .UNSPECIFIED.,.F.,.F.,(4,2,2,2,2,2,2,2,2,2,4),(0.157597789128493,0.169083802496607,
0.18870673517436,0.208226233094476,0.227720441582404,0.247283245699002,
0.266966206820028,0.276841811354643,0.286707833757665,0.306807298818768,
0.315181555765077),.UNSPECIFIED.);
#2536=B_SPLINE_CURVE_WITH_KNOTS('',3,(#112040,#112041,#112042,#112043,#112044,
#112045,#112046,#112047,#112048,#112049,#112050,#112051,#112052,#112053,
#112054,#112055,#112056,#112057,#112058,#112059,#112060,#112061,#112062),
 .UNSPECIFIED.,.F.,.F.,(4,3,2,2,2,2,2,2,2,2,4),(0.315181555765077,0.315211081404571,
0.335185778257555,0.355123769487627,0.374629687959294,0.394580515763128,
0.414589339174075,0.43469511893165,0.44454832600833,0.46455224696731,0.472808870533064),
 .UNSPECIFIED.);
#2537=B_SPLINE_CURVE_WITH_KNOTS('',3,(#112066,#112067,#112068,#112069,#112070,
#112071,#112072,#112073,#112074,#112075,#112076,#112077,#112078,#112079,
#112080,#112081,#112082,#112083,#112084,#112085,#112086,#112087,#112088,
#112089,#112090,#112091,#112092,#112093,#112094,#112095,#112096,#112097,
#112098,#112099,#112100,#112101),.UNSPECIFIED.,.T.,.F.,(4,2,2,2,2,2,2,2,
2,2,2,2,2,2,2,2,2,4),(0.,0.0433164111904613,0.0861802904256355,0.128695730684266,
0.17117710467452,0.213959992111218,0.257192364442634,0.278872188929985,
0.300475215881829,0.344325448282991,0.387923981596494,0.43146876574843,
0.473989434020882,0.516592272710811,0.560170910964625,0.603968557707506,
0.648131236112833,0.690514011068081),.UNSPECIFIED.);
#2538=B_SPLINE_CURVE_WITH_KNOTS('',3,(#112105,#112106,#112107,#112108,#112109,
#112110,#112111,#112112,#112113,#112114,#112115,#112116,#112117,#112118,
#112119,#112120,#112121,#112122,#112123,#112124,#112125,#112126),
 .UNSPECIFIED.,.F.,.F.,(4,2,2,2,2,2,2,2,2,2,4),(0.155287089809751,0.156239702321605,
0.175693722579379,0.194950054784518,0.214071007842835,0.233198182186066,
0.252469243668368,0.271936827701031,0.281664497015936,0.291376767571409,
0.310561645694942),.UNSPECIFIED.);
#2539=B_SPLINE_CURVE_WITH_KNOTS('',3,(#112130,#112131,#112132,#112133,#112134,
#112135,#112136,#112137,#112138,#112139,#112140,#112141,#112142,#112143,
#112144,#112145,#112146,#112147,#112148,#112149,#112150),.UNSPECIFIED.,
 .F.,.F.,(4,3,2,2,2,2,2,2,2,4),(0.310561645694942,0.310600891687435,0.330305486834909,
0.349720687016697,0.368845270661463,0.387995078999074,0.40729029280085,
0.427067810869433,0.446935487204266,0.465887981497185),.UNSPECIFIED.);
#2540=B_SPLINE_CURVE_WITH_KNOTS('',3,(#112154,#112155,#112156,#112157,#112158,
#112159,#112160,#112161,#112162,#112163,#112164,#112165,#112166,#112167,
#112168,#112169,#112170,#112171,#112172,#112173,#112174,#112175,#112176,
#112177,#112178,#112179,#112180,#112181,#112182,#112183,#112184,#112185,
#112186,#112187,#112188,#112189,#112190,#112191),.UNSPECIFIED.,.T.,.F.,
(4,2,2,2,2,2,2,2,2,2,2,2,2,2,2,2,2,2,4),(0.,0.0580082234967378,0.0870003549736756,
0.145722824454584,0.204170932747089,0.262860983195594,0.32181813325465,
0.380645368506535,0.439147647867318,0.497686767907287,0.526427549115819,
0.555714243195097,0.61393184666816,0.672175661372658,0.730386137666084,
0.78847933364516,0.846448163441301,0.904377989258386,0.93172076410077),
 .UNSPECIFIED.);
#2541=B_SPLINE_CURVE_WITH_KNOTS('',3,(#112195,#112196,#112197,#112198,#112199,
#112200,#112201,#112202,#112203,#112204,#112205,#112206,#112207,#112208,
#112209,#112210,#112211,#112212,#112213,#112214,#112215,#112216),
 .UNSPECIFIED.,.F.,.F.,(4,2,2,2,2,2,2,2,2,2,4),(0.276825419382499,0.296324142535683,
0.330827915139416,0.365291806459535,0.399749802742698,0.434231353821986,
0.451460874855943,0.468676585515715,0.503676193620126,0.538615895182268,
0.553565879266481),.UNSPECIFIED.);
#2542=B_SPLINE_CURVE_WITH_KNOTS('',3,(#112220,#112221,#112222,#112223,#112224,
#112225,#112226,#112227,#112228,#112229,#112230,#112231,#112232,#112233,
#112234,#112235,#112236,#112237,#112238,#112239),.UNSPECIFIED.,.F.,.F.,
(4,2,2,2,2,2,2,2,2,4),(0.553566629579059,0.588673847195773,0.623808685061497,
0.658827117911204,0.693760556057172,0.728808292162389,0.74621422278564,
0.780776959390752,0.815342636920125,0.830391298648981),.UNSPECIFIED.);
#2543=B_SPLINE_CURVE_WITH_KNOTS('',3,(#112243,#112244,#112245,#112246,#112247,
#112248,#112249,#112250,#112251,#112252,#112253,#112254,#112255,#112256,
#112257,#112258,#112259,#112260,#112261,#112262,#112263,#112264,#112265,
#112266,#112267,#112268,#112269,#112270,#112271,#112272,#112273,#112274,
#112275,#112276,#112277,#112278),.UNSPECIFIED.,.T.,.F.,(4,2,2,2,2,2,2,2,
2,2,2,2,2,2,2,2,2,4),(0.,0.0501941079062752,0.100208029985453,0.150133961016788,
0.200122562975031,0.250261040409613,0.300503454318807,0.351402927886362,
0.402040021073659,0.452714837694694,0.503452587635481,0.55411839025828,
0.604764231782756,0.655704733278668,0.681060469351491,0.731450356759017,
0.781833273489143,0.804680564507272),.UNSPECIFIED.);
#2544=B_SPLINE_CURVE_WITH_KNOTS('',3,(#112282,#112283,#112284,#112285,#112286,
#112287,#112288,#112289,#112290,#112291,#112292,#112293,#112294,#112295,
#112296,#112297,#112298,#112299,#112300,#112301,#112302,#112303,#112304,
#112305,#112306),.UNSPECIFIED.,.F.,.F.,(4,2,2,2,2,2,2,2,2,2,3,4),(0.213115940430313,
0.228240783603859,0.25475654265634,0.281222254477514,0.307699372237131,
0.334239639354176,0.347526280393058,0.360821523860804,0.387448044952019,
0.41444762115626,0.42607809063124,0.426122798621427),.UNSPECIFIED.);
#2545=B_SPLINE_CURVE_WITH_KNOTS('',3,(#112310,#112311,#112312,#112313,#112314,
#112315,#112316,#112317,#112318,#112319,#112320,#112321,#112322,#112323,
#112324,#112325,#112326,#112327,#112328,#112329),.UNSPECIFIED.,.F.,.F.,
(4,2,2,2,2,2,2,2,2,4),(0.426122798621427,0.453022011122751,0.479971032167598,
0.506914688870937,0.533886525204312,0.560974013753547,0.574405821463177,
0.601073035300724,0.627725348855489,0.639194031061553),.UNSPECIFIED.);
#2546=B_SPLINE_CURVE_WITH_KNOTS('',3,(#112333,#112334,#112335,#112336,#112337,
#112338,#112339,#112340,#112341,#112342,#112343,#112344,#112345,#112346,
#112347,#112348,#112349,#112350,#112351,#112352,#112353,#112354,#112355,
#112356,#112357,#112358,#112359,#112360,#112361,#112362,#112363,#112364,
#112365,#112366,#112367,#112368,#112369,#112370),.UNSPECIFIED.,.T.,.F.,
(4,2,2,2,2,2,2,2,2,2,2,2,2,2,2,2,2,2,4),(0.,0.0432546244612286,0.086255807439944,
0.129173083664551,0.172232566355353,0.215565601873972,0.23731502413423,
0.259009358276642,0.30304397619408,0.346860989813651,0.390696968675583,
0.434168192850255,0.477198720502358,0.521002216775895,0.564898011457953,
0.586432590869027,0.608052372281735,0.652125519462753,0.694293106594506),
 .UNSPECIFIED.);
#2547=B_SPLINE_CURVE_WITH_KNOTS('',3,(#112374,#112375,#112376,#112377,#112378,
#112379,#112380,#112381,#112382,#112383,#112384,#112385,#112386,#112387,
#112388,#112389,#112390,#112391,#112392,#112393,#112394,#112395),
 .UNSPECIFIED.,.F.,.F.,(4,2,2,2,2,2,2,2,2,2,4),(0.157571090181139,0.158533388827235,
0.178145141731992,0.197659871594592,0.217157670328134,0.236729740971422,
0.256421770612226,0.266273321120224,0.276108275501286,0.296155698892633,
0.315156398956201),.UNSPECIFIED.);
#2548=B_SPLINE_CURVE_WITH_KNOTS('',3,(#112399,#112400,#112401,#112402,#112403,
#112404,#112405,#112406,#112407,#112408,#112409,#112410,#112411,#112412,
#112413,#112414,#112415,#112416,#112417,#112418,#112419,#112420,#112421),
 .UNSPECIFIED.,.F.,.F.,(4,3,2,2,2,2,2,2,2,2,4),(0.315156398956201,0.315184248085558,
0.33516826884962,0.354679961794265,0.37420007938843,0.394184451236293,0.414202323850884,
0.4240062685368,0.433828109433089,0.453986817846637,0.472755338266697),
 .UNSPECIFIED.);
#2549=B_SPLINE_CURVE_WITH_KNOTS('',3,(#112425,#112426,#112427,#112428,#112429,
#112430,#112431,#112432,#112433,#112434,#112435,#112436,#112437,#112438,
#112439,#112440,#112441,#112442,#112443,#112444,#112445,#112446,#112447,
#112448,#112449,#112450,#112451,#112452,#112453,#112454,#112455,#112456,
#112457,#112458,#112459,#112460),.UNSPECIFIED.,.T.,.F.,(4,2,2,2,2,2,2,2,
2,2,2,2,2,2,2,2,2,4),(0.,0.0430585199525399,0.0856946946073311,0.128146367850984,
0.170765293674358,0.21380192121876,0.258059130523452,0.279602698825103,
0.32336245007672,0.366948239185581,0.41010425798879,0.452616352668395,0.495235832149333,
0.53881891492568,0.582560673493689,0.626639303656973,0.670992351859876,
0.690486283458249),.UNSPECIFIED.);
#2550=B_SPLINE_CURVE_WITH_KNOTS('',3,(#112464,#112465,#112466,#112467,#112468,
#112469,#112470,#112471,#112472,#112473,#112474,#112475,#112476,#112477,
#112478,#112479,#112480,#112481,#112482,#112483,#112484,#112485,#112486),
 .UNSPECIFIED.,.F.,.F.,(4,2,2,2,2,2,2,2,2,3,4),(0.15531757295188,0.156219469888912,
0.175559071474778,0.194724030140012,0.21382905049678,0.233024066023952,
0.252406525118312,0.272263835569533,0.292052092223187,0.310621714473832,
0.310623433033234),.UNSPECIFIED.);
#2551=B_SPLINE_CURVE_WITH_KNOTS('',3,(#112490,#112491,#112492,#112493,#112494,
#112495,#112496,#112497,#112498,#112499,#112500,#112501,#112502,#112503,
#112504,#112505,#112506,#112507),.UNSPECIFIED.,.F.,.F.,(4,2,2,2,2,2,2,2,
4),(0.310623433033234,0.330112775227974,0.349270594235827,0.36839029551999,
0.387608771293272,0.407326728692038,0.42711301933763,0.446969017839007,
0.465939287425712),.UNSPECIFIED.);
#2552=B_SPLINE_CURVE_WITH_KNOTS('',3,(#112511,#112512,#112513,#112514,#112515,
#112516,#112517,#112518,#112519,#112520,#112521,#112522,#112523,#112524,
#112525,#112526,#112527,#112528,#112529,#112530,#112531,#112532,#112533,
#112534,#112535,#112536,#112537,#112538,#112539,#112540,#112541,#112542,
#112543,#112544,#112545,#112546),.UNSPECIFIED.,.T.,.F.,(4,2,2,2,2,2,2,2,
2,2,2,2,2,2,2,2,2,4),(0.,0.0580987417317566,0.116047179752343,0.173942504194012,
0.231890034901526,0.260874895236775,0.289864886177479,0.348715623176785,
0.40719421054338,0.465783055157053,0.524545288006566,0.583199724794616,
0.641672766601171,0.700361462609497,0.759142645252055,0.817380642606661,
0.875659937599892,0.931838431390136),.UNSPECIFIED.);
#2553=B_SPLINE_CURVE_WITH_KNOTS('',3,(#112550,#112551,#112552,#112553,#112554,
#112555,#112556,#112557,#112558,#112559,#112560,#112561,#112562,#112563,
#112564,#112565,#112566,#112567,#112568,#112569,#112570,#112571),
 .UNSPECIFIED.,.F.,.F.,(4,2,2,2,2,2,2,2,2,2,4),(0.139807847310764,0.172892344288993,
0.207349020107777,0.241786047442339,0.276246202522754,0.293472315492746,
0.31070131942903,0.345811547283687,0.380767382220101,0.41573982156058,0.416591164797455),
 .UNSPECIFIED.);
#2554=B_SPLINE_CURVE_WITH_KNOTS('',3,(#112575,#112576,#112577,#112578,#112579,
#112580,#112581,#112582,#112583,#112584,#112585,#112586,#112587,#112588,
#112589,#112590,#112591,#112592,#112593,#112594,#112595,#112596,#112597),
 .UNSPECIFIED.,.F.,.F.,(4,2,2,2,3,2,2,2,2,2,4),(0.416591164797455,0.450764532772226,
0.485758661251731,0.52070521808968,0.553554982405065,0.570960064057211,
0.588202925424454,0.622775829172639,0.657363001084429,0.691932699501471,
0.69336282971583),.UNSPECIFIED.);
#2555=B_SPLINE_CURVE_WITH_KNOTS('',3,(#112601,#112602,#112603,#112604,#112605,
#112606,#112607,#112608,#112609,#112610,#112611,#112612,#112613,#112614,
#112615,#112616,#112617,#112618,#112619,#112620,#112621,#112622,#112623,
#112624,#112625,#112626,#112627,#112628,#112629,#112630,#112631,#112632,
#112633,#112634,#112635,#112636),.UNSPECIFIED.,.T.,.F.,(4,2,2,2,2,2,2,2,
2,2,2,2,2,2,2,2,2,4),(0.,0.0500751837172648,0.100032835755184,0.150004622813311,
0.200104477996478,0.250330155712872,0.301275718890895,0.351916973449905,
0.402634777221146,0.453544462099944,0.504429457760046,0.555113620900938,
0.605779259382996,0.630621781652347,0.655571265702426,0.706455348933985,
0.756802298634988,0.804652792367142),.UNSPECIFIED.);
#2556=B_SPLINE_CURVE_WITH_KNOTS('',3,(#112640,#112641,#112642,#112643,#112644,
#112645,#112646,#112647,#112648,#112649,#112650,#112651,#112652,#112653,
#112654,#112655,#112656,#112657,#112658,#112659,#112660,#112661,#112662,
#112663,#112664),.UNSPECIFIED.,.F.,.F.,(4,2,2,2,2,2,2,2,2,2,3,4),(0.213076432906529,
0.214625312887961,0.241130224916482,0.267600798364176,0.294095401469753,
0.320655354479264,0.333945803383919,0.347229432506566,0.374268970490067,
0.401233145512626,0.426062397290551,0.426094069355307),.UNSPECIFIED.);
#2557=B_SPLINE_CURVE_WITH_KNOTS('',3,(#112668,#112669,#112670,#112671,#112672,
#112673,#112674,#112675,#112676,#112677,#112678,#112679,#112680,#112681,
#112682,#112683,#112684,#112685,#112686,#112687),.UNSPECIFIED.,.F.,.F.,
(4,2,2,2,2,2,2,2,2,4),(0.426094069355307,0.453108809523285,0.480148392673564,
0.507128954570031,0.534100718191605,0.547305148979544,0.560538665060336,
0.58748104776454,0.614114710291041,0.63913883019708),.UNSPECIFIED.);
#2558=B_SPLINE_CURVE_WITH_KNOTS('',3,(#112691,#112692,#112693,#112694,#112695,
#112696,#112697,#112698,#112699,#112700,#112701,#112702,#112703,#112704,
#112705,#112706,#112707,#112708,#112709,#112710,#112711,#112712,#112713,
#112714,#112715,#112716,#112717,#112718,#112719,#112720,#112721,#112722,
#112723,#112724,#112725,#112726,#112727,#112728),.UNSPECIFIED.,.T.,.F.,
(4,2,2,2,2,2,2,2,2,2,2,2,2,2,2,2,2,2,4),(0.,0.0431036505402475,0.086030227698429,
0.12899757453654,0.172198322896197,0.215665127366231,0.237347439199144,
0.28136115483838,0.325171935923412,0.369015030741623,0.412483731024054,
0.455518305292952,0.499321306509743,0.54321713079997,0.564752036213917,
0.58637219462266,0.63043986218883,0.673944869558154,0.694276631667984),
 .UNSPECIFIED.);
#2559=B_SPLINE_CURVE_WITH_KNOTS('',3,(#112732,#112733,#112734,#112735,#112736,
#112737,#112738,#112739,#112740,#112741,#112742,#112743,#112744,#112745,
#112746,#112747,#112748,#112749,#112750,#112751,#112752,#112753),
 .UNSPECIFIED.,.F.,.F.,(4,2,2,2,2,2,2,2,2,2,4),(0.157610394168263,0.167948182018796,
0.187461103302467,0.206959039117144,0.226532732494941,0.246226517887538,
0.256075595964361,0.265907492794962,0.285949702319035,0.305941086537169,
0.315175721481595),.UNSPECIFIED.);
#2560=B_SPLINE_CURVE_WITH_KNOTS('',3,(#112757,#112758,#112759,#112760,#112761,
#112762,#112763,#112764,#112765,#112766,#112767,#112768,#112769,#112770,
#112771,#112772,#112773,#112774,#112775,#112776),.UNSPECIFIED.,.F.,.F.,
(4,2,2,2,2,2,2,2,2,4),(0.315176131159691,0.334712905302903,0.354217365440266,
0.373772274158537,0.393765409621518,0.413813284197024,0.423632882046344,
0.443787520663527,0.46351526610713,0.472786115649858),.UNSPECIFIED.);
#2561=B_SPLINE_CURVE_WITH_KNOTS('',3,(#112780,#112781,#112782,#112783,#112784,
#112785,#112786,#112787,#112788,#112789,#112790,#112791,#112792,#112793,
#112794,#112795,#112796,#112797,#112798,#112799,#112800,#112801,#112802,
#112803,#112804,#112805,#112806,#112807,#112808,#112809,#112810,#112811,
#112812,#112813,#112814,#112815,#112816,#112817),.UNSPECIFIED.,.T.,.F.,
(4,2,2,2,2,2,2,2,2,2,2,2,2,2,2,2,2,2,4),(0.,0.0428352656493673,0.0853323262706088,
0.12781305629003,0.170609089855836,0.213855236814163,0.23554467169079,0.257156357809307,
0.301012526245623,0.344596881047352,0.388103409972812,0.43061567105667,
0.473223348968646,0.51680383210501,0.56065107298488,0.582188244212754,0.626563562308793,
0.67003492597377,0.69032599641099),.UNSPECIFIED.);
#2562=B_SPLINE_CURVE_WITH_KNOTS('',3,(#112821,#112822,#112823,#112824,#112825,
#112826,#112827,#112828,#112829,#112830,#112831,#112832,#112833,#112834,
#112835,#112836,#112837,#112838,#112839,#112840),.UNSPECIFIED.,.F.,.F.,
(4,2,2,2,2,2,2,2,2,4),(0.155279913630204,0.16580783098891,0.184973337282856,
0.204075159603871,0.223264401799693,0.242640837393322,0.262555404900247,
0.282398648796319,0.3021371068126,0.310566010568874),.UNSPECIFIED.);
#2563=B_SPLINE_CURVE_WITH_KNOTS('',3,(#112844,#112845,#112846,#112847,#112848,
#112849,#112850,#112851,#112852,#112853,#112854,#112855,#112856,#112857,
#112858,#112859,#112860,#112861,#112862,#112863),.UNSPECIFIED.,.F.,.F.,
(4,2,2,2,2,2,2,2,2,4),(0.31056680619282,0.329971810180022,0.349091924172357,
0.368241538651675,0.387939228916316,0.407735663979358,0.417440913787486,
0.437356634777529,0.457031325949547,0.465846719823024),.UNSPECIFIED.);
#2564=B_SPLINE_CURVE_WITH_KNOTS('',3,(#112868,#112869,#112870,#112871,#112872,
#112873,#112874,#112875,#112876,#112877,#112878,#112879,#112880,#112881,
#112882,#112883,#112884,#112885,#112886,#112887,#112888,#112889,#112890,
#112891,#112892,#112893,#112894,#112895,#112896,#112897,#112898,#112899,
#112900,#112901,#112902,#112903,#112904,#112905,#112906,#112907,#112908,
#112909,#112910,#112911,#112912,#112913,#112914,#112915,#112916,#112917,
#112918,#112919,#112920,#112921,#112922,#112923,#112924,#112925,#112926,
#112927,#112928,#112929,#112930,#112931,#112932,#112933,#112934,#112935,
#112936,#112937,#112938,#112939,#112940,#112941,#112942,#112943,#112944,
#112945,#112946,#112947,#112948,#112949,#112950,#112951,#112952,#112953,
#112954,#112955,#112956,#112957,#112958,#112959,#112960,#112961,#112962,
#112963,#112964,#112965,#112966,#112967,#112968,#112969,#112970,#112971,
#112972,#112973,#112974,#112975,#112976,#112977,#112978,#112979,#112980,
#112981,#112982,#112983,#112984,#112985,#112986,#112987,#112988,#112989,
#112990,#112991),.UNSPECIFIED.,.F.,.F.,(4,3,3,3,3,3,3,3,3,3,3,3,3,3,3,3,
3,3,3,3,3,3,3,3,3,3,3,3,3,3,3,3,3,3,3,3,3,3,3,3,3,4),(0.,0.000132727827510117,
0.000266773740721149,0.000288916803381741,0.000405384809022413,0.000521742841023505,
0.000577833606763482,0.000712486468141431,0.000847464610128366,0.000866750410145223,
0.000975173680697608,0.00108362607993552,0.00115566721352696,0.00130437632058373,
0.00145300072902973,0.00160173866912145,0.00173350082029021,0.0018816218515353,
0.00202963491476389,0.00217772706204638,0.00231133442705345,0.00242041547284975,
0.0025294417699843,0.00260025123043525,0.0027352309774238,0.00287005073028349,
0.00288916803381705,0.00300322542298272,0.00311737920790335,0.00317808483719885,
0.00331233809713726,0.00344542767765184,0.00346700164058064,0.00367446908522699,
0.00389243458456527,0.00404483524734448,0.00417937562109319,0.00431434174898983,
0.00433375205072634,0.00444167959104199,0.00454961794032719,0.00462266885410819),
 .UNSPECIFIED.);
#2565=B_SPLINE_CURVE_WITH_KNOTS('',3,(#112992,#112993,#112994,#112995,#112996,
#112997,#112998,#112999,#113000,#113001,#113002,#113003,#113004,#113005,
#113006,#113007,#113008,#113009,#113010,#113011,#113012,#113013),
 .UNSPECIFIED.,.F.,.F.,(4,2,2,2,2,2,2,2,2,2,4),(1.00000008493243E-6,0.029653429365995,
0.0602604700157899,0.11533078437385,0.17381113667683,0.232718531946666,
0.29151133439998,0.349760765588745,0.405060944992747,0.435860211986261,
0.465679959802954),.UNSPECIFIED.);
#2566=B_SPLINE_CURVE_WITH_KNOTS('',3,(#113017,#113018,#113019,#113020,#113021,
#113022,#113023,#113024,#113025,#113026,#113027,#113028,#113029,#113030,
#113031,#113032,#113033,#113034,#113035,#113036,#113037,#113038),
 .UNSPECIFIED.,.F.,.F.,(4,2,2,2,2,2,2,2,2,2,4),(0.139778603637599,0.155618232301033,
0.190078361151525,0.224525782933454,0.258996784686075,0.276224747417236,
0.293454286943181,0.328509035327943,0.363455338377977,0.398466352212045,
0.416560896929866),.UNSPECIFIED.);
#2567=B_SPLINE_CURVE_WITH_KNOTS('',3,(#113042,#113043,#113044,#113045,#113046,
#113047,#113048,#113049,#113050,#113051,#113052,#113053,#113054,#113055,
#113056,#113057,#113058,#113059,#113060,#113061,#113062,#113063,#113064),
 .UNSPECIFIED.,.F.,.F.,(4,2,2,2,2,3,2,2,2,2,4),(0.416560896929866,0.433550062973671,
0.468586736901151,0.503537705167099,0.538545078807563,0.553571177289101,
0.5709760822326,0.605544501529132,0.640121440384529,0.674680233623428,0.6933497809267),
 .UNSPECIFIED.);
#2568=B_SPLINE_CURVE_WITH_KNOTS('',3,(#113068,#113069,#113070,#113071,#113072,
#113073,#113074,#113075,#113076,#113077,#113078,#113079,#113080,#113081,
#113082,#113083,#113084,#113085,#113086,#113087,#113088,#113089,#113090,
#113091,#113092,#113093,#113094,#113095,#113096,#113097,#113098,#113099,
#113100,#113101,#113102,#113103),.UNSPECIFIED.,.T.,.F.,(4,2,2,2,2,2,2,2,
2,2,2,2,2,2,2,2,2,4),(0.,0.0500013751008811,0.0999335696666295,0.149942216996394,
0.200099464079681,0.250344942531881,0.301166873531067,0.35180215134918,
0.402535817466994,0.453341707681982,0.504043858657694,0.554688223342568,
0.605603037386339,0.630958857926489,0.681344686655627,0.731710165394641,
0.781959095477368,0.8046581519998),.UNSPECIFIED.);
#2569=B_SPLINE_CURVE_WITH_KNOTS('',3,(#113107,#113108,#113109,#113110,#113111,
#113112,#113113,#113114,#113115,#113116,#113117,#113118,#113119,#113120,
#113121,#113122,#113123,#113124,#113125,#113126,#113127,#113128,#113129,
#113130,#113131),.UNSPECIFIED.,.F.,.F.,(4,2,2,2,2,2,2,2,2,2,3,4),(0.21306639715026,
0.227818517188535,0.254284620692242,0.280769692590348,0.307320004030579,
0.320608781865553,0.333904721980843,0.360999127823795,0.387980630115309,
0.414943709069341,0.426070661041189,0.426071735170524),.UNSPECIFIED.);
#2570=B_SPLINE_CURVE_WITH_KNOTS('',3,(#113135,#113136,#113137,#113138,#113139,
#113140,#113141,#113142,#113143,#113144,#113145,#113146,#113147,#113148,
#113149,#113150,#113151,#113152,#113153,#113154),.UNSPECIFIED.,.F.,.F.,
(4,2,2,2,2,2,2,2,2,4),(0.426071735170524,0.453056419326165,0.480023136717187,
0.506993993658203,0.534059802781662,0.547491641042938,0.574156120741799,
0.600799182590686,0.627381165688696,0.639137058191448),.UNSPECIFIED.);
#2571=B_SPLINE_CURVE_WITH_KNOTS('',3,(#113158,#113159,#113160,#113161,#113162,
#113163,#113164,#113165,#113166,#113167,#113168,#113169,#113170,#113171,
#113172,#113173,#113174,#113175,#113176,#113177,#113178,#113179,#113180,
#113181,#113182,#113183,#113184,#113185,#113186,#113187,#113188,#113189,
#113190,#113191,#113192,#113193,#113194,#113195),.UNSPECIFIED.,.T.,.F.,
(4,2,2,2,2,2,2,2,2,2,2,2,2,2,2,2,2,2,4),(0.,0.0429891853374796,0.0859005999535319,
0.128961697155561,0.172298985504059,0.194049435970534,0.215763342582676,
0.259828801018375,0.30364808584257,0.34744608553005,0.391291350030285,0.435107609405515,
0.478899297207649,0.522858735862178,0.544436771053145,0.566107742248526,
0.610164662353544,0.653665850718197,0.694242334530551),.UNSPECIFIED.);
#2572=B_SPLINE_CURVE_WITH_KNOTS('',3,(#113199,#113200,#113201,#113202,#113203,
#113204,#113205,#113206,#113207,#113208,#113209,#113210,#113211,#113212,
#113213,#113214,#113215,#113216,#113217,#113218,#113219,#113220),
 .UNSPECIFIED.,.F.,.F.,(4,2,2,2,2,2,2,2,2,2,4),(0.157585769628841,0.158225301867115,
0.177736895355939,0.197232454756444,0.216803549637752,0.236495203073658,
0.246357547652047,0.256205161209479,0.276272029703586,0.296265613933276,
0.315159925279468),.UNSPECIFIED.);
#2573=B_SPLINE_CURVE_WITH_KNOTS('',3,(#113224,#113225,#113226,#113227,#113228,
#113229,#113230,#113231,#113232,#113233,#113234,#113235,#113236,#113237,
#113238,#113239,#113240,#113241,#113242,#113243),.UNSPECIFIED.,.F.,.F.,
(4,2,2,2,2,2,2,2,2,4),(0.315160050285981,0.334670430203605,0.354189141254802,
0.374168068425965,0.394206586146733,0.404024624906889,0.413863252447633,
0.434047259293593,0.453776342647583,0.47274569490831),.UNSPECIFIED.);
#2574=B_SPLINE_CURVE_WITH_KNOTS('',3,(#113247,#113248,#113249,#113250,#113251,
#113252,#113253,#113254,#113255,#113256,#113257,#113258,#113259,#113260,
#113261,#113262,#113263,#113264,#113265,#113266,#113267,#113268,#113269,
#113270,#113271,#113272,#113273,#113274,#113275,#113276,#113277,#113278,
#113279,#113280,#113281,#113282),.UNSPECIFIED.,.T.,.F.,(4,2,2,2,2,2,2,2,
2,2,2,2,2,2,2,2,2,4),(0.,0.0426100058611737,0.0850537338212922,0.127683673144397,
0.170738592765703,0.21499975720634,0.258917600876533,0.302551931591063,
0.346114098909498,0.388667892881555,0.431196440879394,0.473979898101083,
0.517628800858337,0.539043319669517,0.560533654325841,0.604811095552307,
0.648250315521968,0.690350009265023),.UNSPECIFIED.);
#2575=B_SPLINE_CURVE_WITH_KNOTS('',3,(#113286,#113287,#113288,#113289,#113290,
#113291,#113292,#113293,#113294,#113295,#113296,#113297,#113298,#113299,
#113300,#113301,#113302,#113303,#113304,#113305),.UNSPECIFIED.,.F.,.F.,
(4,2,2,2,2,2,2,2,2,4),(0.155247189447164,0.15543816107154,0.174597755768616,
0.193700166759114,0.212895298509184,0.232278832018566,0.252145502041954,
0.271941852319901,0.291661619042685,0.310534450795838),.UNSPECIFIED.);
#2576=B_SPLINE_CURVE_WITH_KNOTS('',3,(#113309,#113310,#113311,#113312,#113313,
#113314,#113315,#113316,#113317,#113318,#113319,#113320,#113321,#113322,
#113323,#113324,#113325,#113326,#113327,#113328),.UNSPECIFIED.,.F.,.F.,
(4,2,2,2,2,2,2,2,2,4),(0.310534954456055,0.329684905209518,0.348803441508971,
0.368026285193018,0.387750202801044,0.397415039714546,0.407097339812214,
0.426966474822227,0.446639471435926,0.465781640243002),.UNSPECIFIED.);
#2577=B_SPLINE_CURVE_WITH_KNOTS('',3,(#113331,#113332,#113333,#113334,#113335,
#113336,#113337,#113338,#113339,#113340,#113341,#113342,#113343,#113344,
#113345,#113346,#113347,#113348,#113349,#113350,#113351,#113352,#113353,
#113354,#113355,#113356,#113357,#113358,#113359,#113360,#113361,#113362,
#113363,#113364,#113365,#113366,#113367,#113368,#113369,#113370,#113371,
#113372,#113373,#113374,#113375,#113376,#113377,#113378,#113379,#113380,
#113381,#113382),.UNSPECIFIED.,.T.,.F.,(4,2,2,2,2,2,2,2,2,2,2,2,2,2,2,2,
2,2,2,2,2,2,2,2,2,4),(0.,0.0149121900649762,0.0263730121522091,0.0384946282833061,
0.0568236080976033,0.105185035310543,0.15252757552285,0.203967129899997,
0.259081364502726,0.318275621652717,0.375912708112063,0.429806971717993,
0.463877271061734,0.477882387809619,0.488346463978146,0.499687248960309,
0.514867691809364,0.547050340458692,0.606166413599678,0.656956780260717,
0.711610535401277,0.770306075356335,0.828288024650288,0.881752841068639,
0.924288918494816,0.931164985314503),.UNSPECIFIED.);
#2578=B_SPLINE_CURVE_WITH_KNOTS('',3,(#113385,#113386,#113387,#113388,#113389,
#113390,#113391,#113392,#113393,#113394,#113395,#113396,#113397,#113398,
#113399,#113400,#113401,#113402,#113403,#113404,#113405,#113406,#113407,
#113408,#113409,#113410,#113411,#113412,#113413,#113414,#113415,#113416,
#113417,#113418,#113419,#113420),.UNSPECIFIED.,.T.,.F.,(4,2,2,2,2,2,2,2,
2,2,2,2,2,2,2,2,2,4),(0.,0.0579392178980262,0.115832358242759,0.173782569200263,
0.202768105596445,0.231758126402807,0.290580147948642,0.349055239233202,
0.407648475424486,0.466395965739747,0.525022431850849,0.583492702203568,
0.642227911139218,0.701011634440832,0.759255031074558,0.817537947627413,
0.875769434518001,0.931837689371155),.UNSPECIFIED.);
#2579=B_SPLINE_CURVE_WITH_KNOTS('',3,(#113424,#113425,#113426,#113427,#113428,
#113429,#113430,#113431,#113432,#113433,#113434,#113435,#113436,#113437,
#113438,#113439,#113440,#113441,#113442,#113443,#113444,#113445),
 .UNSPECIFIED.,.F.,.F.,(4,2,2,2,2,2,2,2,2,2,4),(0.139755173621917,0.172696789744073,
0.207132505990929,0.241593382301936,0.258819812106426,0.276048929239917,
0.311151713616841,0.346105311669953,0.381075529717181,0.41609094289428,
0.416542789415429),.UNSPECIFIED.);
#2580=B_SPLINE_CURVE_WITH_KNOTS('',3,(#113449,#113450,#113451,#113452,#113453,
#113454,#113455,#113456,#113457,#113458,#113459,#113460,#113461,#113462,
#113463,#113464,#113465,#113466,#113467,#113468,#113469),.UNSPECIFIED.,
 .F.,.F.,(4,2,2,2,3,2,2,2,2,4),(0.416542789415429,0.451073116937688,0.486019624601739,
0.521078658759031,0.553639441035905,0.588214628645733,0.622803758665613,
0.657372419330951,0.691883255250138,0.693394614657822),.UNSPECIFIED.);
#2581=B_SPLINE_CURVE_WITH_KNOTS('',3,(#113472,#113473,#113474,#113475,#113476,
#113477,#113478,#113479,#113480,#113481,#113482,#113483,#113484,#113485,
#113486,#113487,#113488,#113489,#113490,#113491,#113492,#113493,#113494,
#113495,#113496,#113497,#113498,#113499,#113500,#113501,#113502,#113503,
#113504,#113505,#113506,#113507,#113508,#113509,#113510,#113511,#113512,
#113513,#113514,#113515,#113516,#113517,#113518,#113519,#113520,#113521),
 .UNSPECIFIED.,.T.,.F.,(4,2,2,2,2,2,2,2,2,2,2,2,2,2,2,2,2,2,2,2,2,2,2,2,
4),(0.,0.0103059827755144,0.021774930988132,0.0401005683710028,0.090946545392836,
0.133247576820222,0.17893682677858,0.227883783029288,0.278524964641298,
0.327309372403573,0.37592257094133,0.394228620230764,0.40557993585886,0.415766213194267,
0.428473089004967,0.452494405415434,0.503326975354497,0.546700448497774,
0.593473184390451,0.643695991372201,0.694046049974661,0.741372994330537,
0.781608468235862,0.798286634292714,0.804144679584088),.UNSPECIFIED.);
#2582=B_SPLINE_CURVE_WITH_KNOTS('',3,(#113524,#113525,#113526,#113527,#113528,
#113529,#113530,#113531,#113532,#113533,#113534,#113535,#113536,#113537,
#113538,#113539,#113540,#113541,#113542,#113543,#113544,#113545,#113546,
#113547,#113548,#113549,#113550,#113551,#113552,#113553,#113554,#113555,
#113556,#113557,#113558,#113559,#113560,#113561),.UNSPECIFIED.,.T.,.F.,
(4,2,2,2,2,2,2,2,2,2,2,2,2,2,2,2,2,2,4),(0.,0.0499381989460856,0.0998725123828674,
0.149935465327738,0.175016839438851,0.20011500129057,0.250360066695874,
0.301079010812412,0.351683677823475,0.402342546584077,0.452986451623471,
0.503593628908851,0.55440362747551,0.579355474490794,0.604708961736832,
0.655104047538882,0.705491754668316,0.755762117527372,0.80452176568964),
 .UNSPECIFIED.);
#2583=B_SPLINE_CURVE_WITH_KNOTS('',3,(#113565,#113566,#113567,#113568,#113569,
#113570,#113571,#113572,#113573,#113574,#113575,#113576,#113577,#113578,
#113579,#113580,#113581,#113582,#113583,#113584,#113585,#113586),
 .UNSPECIFIED.,.F.,.F.,(4,2,2,2,2,2,2,2,2,2,4),(0.213036061661774,0.214062815800093,
0.240524020727665,0.266997646133557,0.29353628989623,0.306823019148326,
0.320117997400603,0.346744786261035,0.373746339552302,0.400671850422301,
0.426054641361433),.UNSPECIFIED.);
#2584=B_SPLINE_CURVE_WITH_KNOTS('',3,(#113590,#113591,#113592,#113593,#113594,
#113595,#113596,#113597,#113598,#113599,#113600,#113601,#113602,#113603,
#113604,#113605,#113606,#113607,#113608,#113609),.UNSPECIFIED.,.F.,.F.,
(4,2,2,2,2,2,2,2,2,4),(0.426054687950607,0.452967716227119,0.479908637510472,
0.506954984943613,0.520385011281766,0.533687129977179,0.560356541301992,
0.587011391805014,0.613604928441249,0.639090749612381),.UNSPECIFIED.);
#2585=B_SPLINE_CURVE_WITH_KNOTS('',3,(#113613,#113614,#113615,#113616,#113617,
#113618,#113619,#113620,#113621,#113622,#113623,#113624,#113625,#113626,
#113627,#113628,#113629,#113630,#113631,#113632,#113633,#113634,#113635,
#113636,#113637,#113638,#113639,#113640,#113641,#113642,#113643,#113644,
#113645,#113646,#113647,#113648,#113649,#113650),.UNSPECIFIED.,.T.,.F.,
(4,2,2,2,2,2,2,2,2,2,2,2,2,2,2,2,2,2,4),(0.,0.0429187561003746,0.0858896515884315,
0.129100841751142,0.172575064704186,0.194263906971067,0.238287259078713,
0.282096822611242,0.325917945154874,0.369798678855887,0.413639582963019,
0.457434972396386,0.501380295514906,0.52294868181926,0.544607783282859,
0.588658005732957,0.63214369771093,0.675352452131438,0.694246639445642),
 .UNSPECIFIED.);
#2586=B_SPLINE_CURVE_WITH_KNOTS('',3,(#113654,#113655,#113656,#113657,#113658,
#113659,#113660,#113661,#113662,#113663,#113664,#113665,#113666,#113667,
#113668,#113669,#113670,#113671,#113672,#113673,#113674,#113675),
 .UNSPECIFIED.,.F.,.F.,(4,2,2,2,2,2,2,2,2,2,4),(0.157602878251341,0.167966818930531,
0.187464755105539,0.207042369642738,0.226740593720201,0.236595153449156,
0.246433052495769,0.266483796840619,0.286473869825833,0.306251221539351,
0.31516019215871),.UNSPECIFIED.);
#2587=B_SPLINE_CURVE_WITH_KNOTS('',3,(#113679,#113680,#113681,#113682,#113683,
#113684,#113685,#113686,#113687,#113688,#113689,#113690,#113691,#113692,
#113693,#113694,#113695,#113696,#113697,#113698),.UNSPECIFIED.,.F.,.F.,
(4,2,2,2,2,2,2,2,2,4),(0.315160208779593,0.334664476111517,0.354222134261767,
0.374222014056629,0.394291801029766,0.40412343171917,0.424295177671824,
0.44401709971294,0.463618758444822,0.472763087030934),.UNSPECIFIED.);
#2588=B_SPLINE_CURVE_WITH_KNOTS('',3,(#113702,#113703,#113704,#113705,#113706,
#113707,#113708,#113709,#113710,#113711,#113712,#113713,#113714,#113715,
#113716,#113717,#113718,#113719,#113720,#113721,#113722,#113723,#113724,
#113725,#113726,#113727,#113728,#113729,#113730,#113731,#113732,#113733,
#113734,#113735,#113736,#113737),.UNSPECIFIED.,.T.,.F.,(4,2,2,2,2,2,2,2,
2,2,2,2,2,2,2,2,2,4),(0.,0.0424789666300493,0.0849679774709149,0.127790667162137,
0.171061745642256,0.215259555594848,0.259077282811308,0.302642339527092,
0.346144078161022,0.38864715447244,0.431272128189375,0.474862210112901,
0.518734949851575,0.54028507684164,0.584672370605554,0.628106698383023,
0.671112016502596,0.690344504645899),.UNSPECIFIED.);
#2589=B_SPLINE_CURVE_WITH_KNOTS('',3,(#113741,#113742,#113743,#113744,#113745,
#113746,#113747,#113748,#113749,#113750,#113751,#113752,#113753,#113754,
#113755,#113756,#113757,#113758,#113759,#113760,#113761,#113762),
 .UNSPECIFIED.,.F.,.F.,(4,2,2,2,2,2,2,2,2,2,4),(0.155262427717209,0.165532373530381,
0.184632674841114,0.203829217875136,0.223215778643951,0.232952142141799,
0.24268393600619,0.262519622819918,0.282251093096163,0.301905988234787,
0.310480476684161),.UNSPECIFIED.);
#2590=B_SPLINE_CURVE_WITH_KNOTS('',3,(#113766,#113767,#113768,#113769,#113770,
#113771,#113772,#113773,#113774,#113775,#113776,#113777,#113778,#113779,
#113780,#113781,#113782,#113783,#113784,#113785),.UNSPECIFIED.,.F.,.F.,
(4,2,2,2,2,2,2,2,2,4),(0.310481108556768,0.329596553706086,0.348750568027949,
0.368451085094143,0.388251140444173,0.39795747456272,0.417871174091899,
0.437531059277961,0.456858480786928,0.465742904401369),.UNSPECIFIED.);
#2591=B_SPLINE_CURVE_WITH_KNOTS('',3,(#113788,#113789,#113790,#113791,#113792,
#113793,#113794,#113795,#113796,#113797,#113798,#113799,#113800,#113801,
#113802,#113803,#113804,#113805,#113806,#113807,#113808,#113809,#113810,
#113811,#113812,#113813,#113814,#113815,#113816,#113817,#113818,#113819,
#113820,#113821,#113822,#113823,#113824,#113825,#113826,#113827,#113828,
#113829,#113830,#113831,#113832,#113833,#113834,#113835,#113836,#113837,
#113838,#113839),.UNSPECIFIED.,.T.,.F.,(4,2,2,2,2,2,2,2,2,2,2,2,2,2,2,2,
2,2,2,2,2,2,2,2,2,4),(0.,0.0320144497702016,0.0458767136401181,0.0557147592155635,
0.0657715796145349,0.0802126605367964,0.115402705682847,0.160055925397762,
0.209471976042195,0.262756796732718,0.319834594604882,0.378252258368803,
0.433784228024685,0.488133124396683,0.506318876043764,0.517142144121038,
0.526626050564159,0.538230524464352,0.559797575654237,0.61878391320983,
0.667805533571324,0.720924855856359,0.777953611535871,0.836424436159223,
0.875349742476717,0.931139968817718),.UNSPECIFIED.);
#2592=B_SPLINE_CURVE_WITH_KNOTS('',3,(#113842,#113843,#113844,#113845,#113846,
#113847,#113848,#113849,#113850,#113851,#113852,#113853,#113854,#113855,
#113856,#113857,#113858,#113859,#113860,#113861,#113862,#113863,#113864,
#113865,#113866,#113867,#113868,#113869,#113870,#113871,#113872,#113873,
#113874,#113875,#113876,#113877),.UNSPECIFIED.,.T.,.F.,(4,2,2,2,2,2,2,2,
2,2,2,2,2,2,2,2,2,4),(0.,0.057912290383271,0.115844267345691,0.173845899019275,
0.202836343323089,0.261569328211721,0.320036860000859,0.378698392235191,
0.437537296788471,0.496221105841023,0.554691820018049,0.613381775757485,
0.672164534867042,0.730400175357851,0.788666822605191,0.846880699532441,
0.904953792012004,0.931852649550286),.UNSPECIFIED.);
#2593=B_SPLINE_CURVE_WITH_KNOTS('',3,(#113881,#113882,#113883,#113884,#113885,
#113886,#113887,#113888,#113889,#113890,#113891,#113892,#113893,#113894,
#113895,#113896,#113897,#113898,#113899,#113900),.UNSPECIFIED.,.F.,.F.,
(4,2,2,2,2,2,2,2,2,4),(0.139754715013795,0.172609259421165,0.207064650854054,
0.24155037115346,0.258779798092583,0.293833199650583,0.328780765782036,
0.363788421544044,0.398858105741495,0.416586635623603),.UNSPECIFIED.);
#2594=B_SPLINE_CURVE_WITH_KNOTS('',3,(#113904,#113905,#113906,#113907,#113908,
#113909,#113910,#113911,#113912,#113913,#113914,#113915,#113916,#113917,
#113918,#113919,#113920,#113921,#113922,#113923,#113924,#113925,#113926),
 .UNSPECIFIED.,.F.,.F.,(4,2,2,2,2,3,2,2,2,2,4),(0.416586635623603,0.433877760225201,
0.468826219581986,0.503854463105767,0.538780024933523,0.553655470180159,
0.588232581400899,0.6228064666686,0.657341280871621,0.691819483465528,0.693410185193954),
 .UNSPECIFIED.);
#2595=B_SPLINE_CURVE_WITH_KNOTS('',3,(#113929,#113930,#113931,#113932,#113933,
#113934,#113935,#113936,#113937,#113938,#113939,#113940,#113941,#113942,
#113943,#113944,#113945,#113946,#113947,#113948,#113949,#113950,#113951,
#113952,#113953,#113954,#113955,#113956,#113957,#113958,#113959,#113960,
#113961,#113962,#113963,#113964,#113965,#113966,#113967,#113968,#113969,
#113970,#113971,#113972,#113973,#113974,#113975,#113976,#113977,#113978,
#113979,#113980),.UNSPECIFIED.,.T.,.F.,(4,2,2,2,2,2,2,2,2,2,2,2,2,2,2,2,
2,2,2,2,2,2,2,2,2,4),(0.,0.0167619929348656,0.0276578117894851,0.0362872275608602,
0.0458432035478929,0.061246066336341,0.108291688612086,0.149502826269685,
0.194332609410432,0.242445764956923,0.293221281057508,0.342681173875022,
0.389406729870615,0.415800156239406,0.426509574580191,0.434498220080772,
0.44316500485031,0.454821148519414,0.479978746987761,0.530832024838283,
0.57414259102436,0.620921651218219,0.671203097113141,0.72151009555737,0.768376318472014,
0.804067995997234),.UNSPECIFIED.);
#2596=B_SPLINE_CURVE_WITH_KNOTS('',3,(#113983,#113984,#113985,#113986,#113987,
#113988,#113989,#113990,#113991,#113992,#113993,#113994,#113995,#113996,
#113997,#113998,#113999,#114000,#114001,#114002,#114003,#114004,#114005,
#114006,#114007,#114008,#114009,#114010,#114011,#114012,#114013,#114014,
#114015,#114016,#114017,#114018,#114019,#114020),.UNSPECIFIED.,.T.,.F.,
(4,2,2,2,2,2,2,2,2,2,2,2,2,2,2,2,2,2,4),(0.,0.0499483525656873,0.099989590289901,
0.150174211793659,0.175276943687537,0.226175081735644,0.276808377411066,
0.32754657529046,0.378464849820159,0.429330158496053,0.479996567083159,
0.530683580160234,0.5555461562912,0.580523336179942,0.631403252897784,0.681741873714619,
0.731957307096482,0.782008216404938,0.804543742961689),.UNSPECIFIED.);
#2597=B_SPLINE_CURVE_WITH_KNOTS('',3,(#114024,#114025,#114026,#114027,#114028,
#114029,#114030,#114031,#114032,#114033,#114034,#114035,#114036,#114037,
#114038,#114039,#114040,#114041,#114042,#114043,#114044,#114045),
 .UNSPECIFIED.,.F.,.F.,(4,2,2,2,2,2,2,2,2,2,4),(0.21306486411963,0.227332866823859,
0.253831618810689,0.280397178858473,0.293689043125694,0.306966278490336,
0.33399561376579,0.360958674455788,0.387958258092557,0.415007997854744,
0.426072187027784),.UNSPECIFIED.);
#2598=B_SPLINE_CURVE_WITH_KNOTS('',3,(#114049,#114050,#114051,#114052,#114053,
#114054,#114055,#114056,#114057,#114058,#114059,#114060,#114061,#114062,
#114063,#114064,#114065,#114066,#114067,#114068),.UNSPECIFIED.,.F.,.F.,
(4,2,2,2,2,2,2,2,2,4),(0.426072562334217,0.453077952711787,0.480040917586814,
0.507059803852167,0.520299739781239,0.547239747248079,0.573869121368994,
0.600435778555616,0.62693553674137,0.639137426453847),.UNSPECIFIED.);
#2599=B_SPLINE_CURVE_WITH_KNOTS('',3,(#114071,#114072,#114073,#114074,#114075,
#114076,#114077,#114078,#114079,#114080,#114081,#114082,#114083,#114084,
#114085,#114086,#114087,#114088,#114089,#114090,#114091,#114092,#114093,
#114094,#114095,#114096,#114097,#114098,#114099,#114100,#114101,#114102,
#114103,#114104,#114105,#114106,#114107,#114108,#114109,#114110,#114111,
#114112,#114113,#114114,#114115,#114116,#114117,#114118,#114119,#114120,
#114121,#114122),.UNSPECIFIED.,.T.,.F.,(4,2,2,2,2,2,2,2,2,2,2,2,2,2,2,2,
2,2,2,2,2,2,2,2,2,4),(0.,0.0102292473935223,0.018082598833696,0.0263963859846061,
0.0390147385032582,0.0728971977507561,0.107589219061119,0.145627768693997,
0.186630958119302,0.230733204186149,0.273926375893012,0.312544707081939,
0.342168896043744,0.354370671563563,0.362541105016026,0.370355680991137,
0.380851202731197,0.403385275933281,0.447232798198564,0.484761694810815,
0.525362691985882,0.569074594761023,0.612536964225629,0.652656732784191,
0.687070434853681,0.693794119617982),.UNSPECIFIED.);
#2600=B_SPLINE_CURVE_WITH_KNOTS('',3,(#114125,#114126,#114127,#114128,#114129,
#114130,#114131,#114132,#114133,#114134,#114135,#114136,#114137,#114138,
#114139,#114140,#114141,#114142,#114143,#114144,#114145,#114146,#114147,
#114148,#114149,#114150,#114151,#114152,#114153,#114154,#114155,#114156,
#114157,#114158,#114159,#114160),.UNSPECIFIED.,.T.,.F.,(4,2,2,2,2,2,2,2,
2,2,2,2,2,2,2,2,2,4),(0.,0.0429106502366654,0.0859817598443145,0.129331618969271,
0.151085232625045,0.172807852044397,0.21688288321358,0.260697808811353,
0.304470070080087,0.348270726520065,0.392048555605167,0.435841729163604,
0.479853272526997,0.524250865104275,0.567905223640583,0.611392741401498,
0.654598658582422,0.694333300491708),.UNSPECIFIED.);
#2601=B_SPLINE_CURVE_WITH_KNOTS('',3,(#114164,#114165,#114166,#114167,#114168,
#114169,#114170,#114171,#114172,#114173,#114174,#114175,#114176,#114177,
#114178,#114179,#114180,#114181,#114182,#114183,#114184,#114185),
 .UNSPECIFIED.,.F.,.F.,(4,2,2,2,2,2,2,2,2,2,4),(0.157555629279167,0.158070011383171,
0.177565895247574,0.197140695879063,0.216836715527659,0.226706323780034,
0.236561509314436,0.256637830271492,0.276629064151961,0.296577893477034,
0.315128960060253),.UNSPECIFIED.);
#2602=B_SPLINE_CURVE_WITH_KNOTS('',3,(#114189,#114190,#114191,#114192,#114193,
#114194,#114195,#114196,#114197,#114198,#114199,#114200,#114201,#114202,
#114203,#114204,#114205,#114206,#114207,#114208,#114209,#114210,#114211),
 .UNSPECIFIED.,.F.,.F.,(4,3,2,2,2,2,2,2,2,2,4),(0.315128960060253,0.31515595446884,
0.334676647783077,0.354656565529836,0.374714656610475,0.384544781031409,
0.394396710796161,0.41438903597914,0.434114151291953,0.453717853798424,
0.472711583748007),.UNSPECIFIED.);
#2603=B_SPLINE_CURVE_WITH_KNOTS('',3,(#114214,#114215,#114216,#114217,#114218,
#114219,#114220,#114221,#114222,#114223,#114224,#114225,#114226,#114227,
#114228,#114229,#114230,#114231,#114232,#114233,#114234,#114235,#114236,
#114237,#114238,#114239,#114240,#114241,#114242,#114243,#114244,#114245,
#114246,#114247,#114248,#114249,#114250,#114251,#114252,#114253,#114254,
#114255,#114256,#114257,#114258,#114259,#114260,#114261,#114262,#114263),
 .UNSPECIFIED.,.T.,.F.,(4,2,2,2,2,2,2,2,2,2,2,2,2,2,2,2,2,2,2,2,2,2,2,2,
4),(0.,0.00816912193231024,0.0176416594614524,0.0338374510674327,0.0772052149196674,
0.113481480317982,0.152933178844101,0.195423379618985,0.239140203807657,
0.28075501503573,0.3223543759762,0.3373449838732,0.346485616157516,0.353794230672201,
0.363486832242064,0.380807023601717,0.424289821313145,0.460871598877258,
0.500666429588826,0.54358905970758,0.587222617397712,0.628438867274253,
0.668029721109657,0.682703416332507,0.689884358287045),.UNSPECIFIED.);
#2604=B_SPLINE_CURVE_WITH_KNOTS('',3,(#114266,#114267,#114268,#114269,#114270,
#114271,#114272,#114273,#114274,#114275,#114276,#114277,#114278,#114279,
#114280,#114281,#114282,#114283,#114284,#114285,#114286,#114287,#114288,
#114289,#114290,#114291,#114292,#114293,#114294,#114295,#114296,#114297,
#114298,#114299,#114300,#114301,#114302,#114303),.UNSPECIFIED.,.T.,.F.,
(4,2,2,2,2,2,2,2,2,2,2,2,2,2,2,2,2,2,4),(0.,0.0424329954915689,0.0850548921633571,
0.128105489804561,0.149803496669879,0.171520604045967,0.215603286957798,
0.259291508388645,0.302760327587543,0.3461701106744,0.388697344372228,0.432199116431131,
0.47596752314268,0.497471190734652,0.519075683971176,0.563108028735137,
0.606545409681133,0.649549890723535,0.690224907908624),.UNSPECIFIED.);
#2605=B_SPLINE_CURVE_WITH_KNOTS('',3,(#114307,#114308,#114309,#114310,#114311,
#114312,#114313,#114314,#114315,#114316,#114317,#114318,#114319,#114320,
#114321,#114322,#114323,#114324,#114325,#114326,#114327,#114328),
 .UNSPECIFIED.,.F.,.F.,(4,2,2,2,2,2,2,2,2,2,4),(0.155239472480513,0.155629710387306,
0.174728016684647,0.193920885494023,0.213303831703006,0.223055692389348,
0.23280748114644,0.252679804558889,0.272421255492315,0.292053011218848,
0.310471145323146),.UNSPECIFIED.);
#2606=B_SPLINE_CURVE_WITH_KNOTS('',3,(#114332,#114333,#114334,#114335,#114336,
#114337,#114338,#114339,#114340,#114341,#114342,#114343,#114344,#114345,
#114346,#114347,#114348,#114349,#114350,#114351),.UNSPECIFIED.,.F.,.F.,
(4,2,2,2,2,2,2,2,2,4),(0.310471318769338,0.329587743034597,0.348807224721795,
0.368577426857687,0.378277472762051,0.388005564817206,0.407959259227537,
0.427615216256153,0.44694589841925,0.465710791249851),.UNSPECIFIED.);
#2607=B_SPLINE_CURVE_WITH_KNOTS('',3,(#114354,#114355,#114356,#114357,#114358,
#114359,#114360,#114361,#114362,#114363,#114364,#114365,#114366,#114367,
#114368,#114369,#114370,#114371,#114372,#114373,#114374,#114375,#114376,
#114377,#114378,#114379,#114380,#114381,#114382,#114383,#114384,#114385,
#114386,#114387,#114388,#114389,#114390,#114391,#114392,#114393,#114394,
#114395,#114396,#114397,#114398,#114399,#114400,#114401,#114402,#114403,
#114404,#114405),.UNSPECIFIED.,.T.,.F.,(4,2,2,2,2,2,2,2,2,2,2,2,2,2,2,2,
2,2,2,2,2,2,2,2,2,4),(0.,0.0525083345848551,0.108779286030152,0.167362101081689,
0.223884663346406,0.279431074018823,0.303364169525237,0.314486881214728,
0.322976133922097,0.331946667594864,0.345595995515426,0.383174082493277,
0.427903989648404,0.477632626158776,0.531410548614856,0.589183859623761,
0.647452074973242,0.702210239020413,0.756794536135306,0.773516436584552,
0.783377035922492,0.791753189623331,0.801870707780898,0.820156312424674,
0.879246497783655,0.931260216792454),.UNSPECIFIED.);
#2608=B_SPLINE_CURVE_WITH_KNOTS('',3,(#114408,#114409,#114410,#114411,#114412,
#114413,#114414,#114415,#114416,#114417,#114418,#114419,#114420,#114421,
#114422,#114423,#114424,#114425,#114426,#114427,#114428,#114429,#114430,
#114431,#114432,#114433,#114434,#114435,#114436,#114437,#114438,#114439,
#114440,#114441),.UNSPECIFIED.,.T.,.F.,(4,2,2,2,2,2,2,2,2,2,2,2,2,2,2,2,
4),(0.,0.0579319231973149,0.115920382400655,0.17394883011719,0.232575230845978,
0.29104002295107,0.349793697557817,0.408751929036138,0.467508142527154,
0.525973906050046,0.58459684254218,0.643901563943303,0.702126116460104,
0.760371269954299,0.818562878710026,0.876625675277847,0.931980461253038),
 .UNSPECIFIED.);
#2609=B_SPLINE_CURVE_WITH_KNOTS('',3,(#114445,#114446,#114447,#114448,#114449,
#114450,#114451,#114452,#114453,#114454,#114455,#114456,#114457,#114458,
#114459,#114460,#114461,#114462,#114463,#114464),.UNSPECIFIED.,.F.,.F.,
(4,2,2,2,2,2,2,2,2,4),(0.139799730781408,0.172534688541551,0.20701737584227,
0.224247110424717,0.241456599860779,0.27645017850127,0.311393660872747,
0.346452033300128,0.381592642182531,0.416592031663367),.UNSPECIFIED.);
#2610=B_SPLINE_CURVE_WITH_KNOTS('',3,(#114468,#114469,#114470,#114471,#114472,
#114473,#114474,#114475,#114476,#114477,#114478,#114479,#114480,#114481,
#114482,#114483,#114484,#114485,#114486,#114487,#114488,#114489,#114490),
 .UNSPECIFIED.,.F.,.F.,(4,2,2,2,2,3,2,2,2,2,4),(0.416592031663367,0.416659563180101,
0.451607079053152,0.486590699737675,0.521807059609053,0.553638721576443,
0.588205308843122,0.62275164209292,0.657252949664438,0.691715150272187,
0.693438452357851),.UNSPECIFIED.);
#2611=B_SPLINE_CURVE_WITH_KNOTS('',3,(#114493,#114494,#114495,#114496,#114497,
#114498,#114499,#114500,#114501,#114502,#114503,#114504,#114505,#114506,
#114507,#114508,#114509,#114510,#114511,#114512,#114513,#114514,#114515,
#114516,#114517,#114518,#114519,#114520,#114521,#114522,#114523,#114524,
#114525,#114526,#114527,#114528,#114529,#114530,#114531,#114532,#114533,
#114534,#114535,#114536,#114537,#114538,#114539,#114540,#114541,#114542,
#114543,#114544,#114545,#114546),.UNSPECIFIED.,.T.,.F.,(4,2,2,2,2,2,2,2,
2,2,2,2,2,2,2,2,2,2,2,2,2,2,2,2,2,2,4),(0.,0.0369491160369705,0.0501161427537167,
0.0583408003539779,0.0658278867613358,0.0753901969450591,0.0945046567240877,
0.145543352718396,0.187675607865597,0.233331625629896,0.282318578506677,
0.332934697685839,0.381410945852096,0.430720162800404,0.448434472729937,
0.45763659248232,0.465010329741499,0.473285136007353,0.486913981469558,
0.531392119941888,0.57196763051739,0.616440783205194,0.66434809866151,0.715170452984358,
0.752780603211039,0.775344267167268,0.803996562106116),.UNSPECIFIED.);
#2612=B_SPLINE_CURVE_WITH_KNOTS('',3,(#114549,#114550,#114551,#114552,#114553,
#114554,#114555,#114556,#114557,#114558,#114559,#114560,#114561,#114562,
#114563,#114564,#114565,#114566,#114567,#114568,#114569,#114570,#114571,
#114572,#114573,#114574,#114575,#114576,#114577,#114578,#114579,#114580,
#114581,#114582,#114583,#114584,#114585,#114586),.UNSPECIFIED.,.T.,.F.,
(4,2,2,2,2,2,2,2,2,2,2,2,2,2,2,2,2,2,4),(0.,0.0499637560937677,0.100062844084125,
0.125152294272686,0.150253945446171,0.201248481135741,0.251911968622351,
0.30259118437123,0.353387136819273,0.404139339396542,0.454777727746519,
0.505547296964785,0.530469187635523,0.555824699095162,0.606213141707336,
0.656572148122596,0.706804639103619,0.75685973914386,0.804538060714784),
 .UNSPECIFIED.);
#2613=B_SPLINE_CURVE_WITH_KNOTS('',3,(#114590,#114591,#114592,#114593,#114594,
#114595,#114596,#114597,#114598,#114599,#114600,#114601,#114602,#114603,
#114604,#114605,#114606,#114607,#114608,#114609,#114610,#114611),
 .UNSPECIFIED.,.F.,.F.,(4,2,2,2,2,2,2,2,2,2,4),(0.213035334055591,0.213498058337152,
0.239986509786572,0.266541736009027,0.279831953885245,0.293128400800926,
0.320214748878366,0.347192802047242,0.374155977515257,0.401138870741644,
0.42606188797298),.UNSPECIFIED.);
#2614=B_SPLINE_CURVE_WITH_KNOTS('',3,(#114615,#114616,#114617,#114618,#114619,
#114620,#114621,#114622,#114623,#114624,#114625,#114626,#114627,#114628,
#114629,#114630,#114631,#114632,#114633,#114634),.UNSPECIFIED.,.F.,.F.,
(4,2,2,2,2,2,2,2,2,4),(0.42606268775071,0.453023220919234,0.480038654483965,
0.493275670389338,0.506707490462197,0.533372517385062,0.560013344973749,
0.586590984961471,0.613095139159837,0.639098021806301),.UNSPECIFIED.);
#2615=B_SPLINE_CURVE_WITH_KNOTS('',3,(#114637,#114638,#114639,#114640,#114641,
#114642,#114643,#114644,#114645,#114646,#114647,#114648,#114649,#114650,
#114651,#114652,#114653,#114654,#114655,#114656,#114657,#114658,#114659,
#114660,#114661,#114662,#114663,#114664,#114665,#114666,#114667,#114668,
#114669,#114670,#114671,#114672,#114673,#114674,#114675,#114676,#114677,
#114678,#114679,#114680,#114681,#114682,#114683,#114684,#114685,#114686,
#114687,#114688,#114689,#114690),.UNSPECIFIED.,.T.,.F.,(4,2,2,2,2,2,2,2,
2,2,2,2,2,2,2,2,2,2,2,2,2,2,2,2,2,2,4),(0.,0.0228480468435155,0.0327278613357826,
0.0389155412692941,0.0456271880868092,0.0546775533820688,0.0744713233992156,
0.118416720185575,0.155288894882617,0.195252941934963,0.238221915332059,
0.281891583999893,0.322930222568161,0.363518611295154,0.3764021328255,0.383922438192359,
0.390434781093071,0.398320332011738,0.412797633133752,0.456696864945195,
0.492818073211253,0.532197232422632,0.574634202506513,0.618505769963775,
0.64918353719598,0.668216196324756,0.693788572706354),.UNSPECIFIED.);
#2616=B_SPLINE_CURVE_WITH_KNOTS('',3,(#114693,#114694,#114695,#114696,#114697,
#114698,#114699,#114700,#114701,#114702,#114703,#114704,#114705,#114706,
#114707,#114708,#114709,#114710,#114711,#114712,#114713,#114714,#114715,
#114716,#114717,#114718,#114719,#114720,#114721,#114722,#114723,#114724,
#114725,#114726,#114727,#114728),.UNSPECIFIED.,.T.,.F.,(4,2,2,2,2,2,2,2,
2,2,2,2,2,2,2,2,2,4),(0.,0.0429881271999506,0.0862259450153807,0.12971880175422,
0.151383394484505,0.195368245878792,0.239171549410387,0.283012428053759,
0.32647532705118,0.370326496748914,0.414125196034328,0.458075699664007,
0.502382022531898,0.546417694371204,0.589878387317715,0.633059308295633,
0.676015445526238,0.694361023560929),.UNSPECIFIED.);
#2617=B_SPLINE_CURVE_WITH_KNOTS('',3,(#114732,#114733,#114734,#114735,#114736,
#114737,#114738,#114739,#114740,#114741,#114742,#114743,#114744,#114745,
#114746,#114747,#114748,#114749,#114750,#114751,#114752,#114753),
 .UNSPECIFIED.,.F.,.F.,(4,2,2,2,2,2,2,2,2,2,4),(0.157606273259384,0.167943647681616,
0.187531534785128,0.207239841218768,0.217088558581301,0.226918881348354,
0.246957240578774,0.266944508893794,0.286716039025147,0.306221084842367,
0.315164770989864),.UNSPECIFIED.);
#2618=B_SPLINE_CURVE_WITH_KNOTS('',3,(#114757,#114758,#114759,#114760,#114761,
#114762,#114763,#114764,#114765,#114766,#114767,#114768,#114769,#114770,
#114771,#114772,#114773,#114774,#114775,#114776),.UNSPECIFIED.,.F.,.F.,
(4,2,2,2,2,2,2,2,2,4),(0.315165008584859,0.33473120703126,0.354732300285761,
0.374800531585434,0.384630520973591,0.404797893462523,0.42451030767009,
0.444102244164262,0.463606440620998,0.472771281844243),.UNSPECIFIED.);
#2619=B_SPLINE_CURVE_WITH_KNOTS('',3,(#114779,#114780,#114781,#114782,#114783,
#114784,#114785,#114786,#114787,#114788,#114789,#114790,#114791,#114792,
#114793,#114794,#114795,#114796,#114797,#114798,#114799,#114800,#114801,
#114802,#114803,#114804,#114805,#114806,#114807,#114808,#114809,#114810,
#114811,#114812,#114813,#114814,#114815,#114816,#114817,#114818,#114819,
#114820,#114821,#114822,#114823,#114824,#114825,#114826,#114827,#114828,
#114829,#114830),.UNSPECIFIED.,.T.,.F.,(4,2,2,2,2,2,2,2,2,2,2,2,2,2,2,2,
2,2,2,2,2,2,2,2,2,4),(0.,0.0136527846687363,0.0224048280718145,0.0292691959298057,
0.0368127137003927,0.0488745028759635,0.085497339849254,0.12007168662968,
0.158105018498429,0.199230292707366,0.243569997033518,0.286401168138391,
0.325560442066355,0.352989103119234,0.363926580530411,0.371171561415239,
0.378060184528038,0.387276805864347,0.407094836053811,0.450659703174363,
0.487474997610149,0.527536138269538,0.570775759477264,0.614277377050491,
0.654773380862052,0.689797023507),.UNSPECIFIED.);
#2620=B_SPLINE_CURVE_WITH_KNOTS('',3,(#114833,#114834,#114835,#114836,#114837,
#114838,#114839,#114840,#114841,#114842,#114843,#114844,#114845,#114846,
#114847,#114848,#114849,#114850,#114851,#114852,#114853,#114854,#114855,
#114856,#114857,#114858,#114859,#114860,#114861,#114862,#114863,#114864,
#114865,#114866,#114867,#114868,#114869,#114870),.UNSPECIFIED.,.T.,.F.,
(4,2,2,2,2,2,2,2,2,2,2,2,2,2,2,2,2,2,4),(0.,0.0425200356386948,0.0854005081350503,
0.128721173636264,0.150328968556923,0.194198532515018,0.237811372563917,
0.281382187239665,0.323917849204456,0.36645979650346,0.41002400041801,0.45368714777466,
0.475110659146658,0.496611135342448,0.540900250276031,0.584295227160176,
0.627255306982154,0.669821335667285,0.690233235741649),.UNSPECIFIED.);
#2621=B_SPLINE_CURVE_WITH_KNOTS('',3,(#114874,#114875,#114876,#114877,#114878,
#114879,#114880,#114881,#114882,#114883,#114884,#114885,#114886,#114887,
#114888,#114889,#114890,#114891,#114892,#114893,#114894,#114895),
 .UNSPECIFIED.,.F.,.F.,(4,2,2,2,2,2,2,2,2,2,4),(0.155262278701396,0.165381853607852,
0.184598949561035,0.204009403841683,0.213725435380747,0.223428918096119,
0.243208588599942,0.262918832679783,0.282370974502219,0.301506216814708,
0.310476735734228),.UNSPECIFIED.);
#2622=B_SPLINE_CURVE_WITH_KNOTS('',3,(#114899,#114900,#114901,#114902,#114903,
#114904,#114905,#114906,#114907,#114908,#114909,#114910,#114911,#114912,
#114913,#114914,#114915,#114916,#114917,#114918),.UNSPECIFIED.,.F.,.F.,
(4,2,2,2,2,2,2,2,2,4),(0.310476868687956,0.329646504529723,0.349347797550038,
0.369112205680196,0.378795195849324,0.3986619979492,0.418308071473111,0.437611587488503,
0.456753059132737,0.465739147389351),.UNSPECIFIED.);
#2623=B_SPLINE_CURVE_WITH_KNOTS('',3,(#114921,#114922,#114923,#114924,#114925,
#114926,#114927,#114928,#114929,#114930,#114931,#114932,#114933,#114934,
#114935,#114936,#114937,#114938,#114939,#114940,#114941,#114942,#114943,
#114944,#114945,#114946,#114947,#114948,#114949,#114950,#114951,#114952,
#114953,#114954,#114955,#114956,#114957,#114958,#114959,#114960,#114961,
#114962,#114963,#114964,#114965,#114966,#114967,#114968,#114969,#114970,
#114971,#114972,#114973,#114974),.UNSPECIFIED.,.T.,.F.,(4,2,2,2,2,2,2,2,
2,2,2,2,2,2,2,2,2,2,2,2,2,2,2,2,2,2,4),(0.,0.0493622911687678,0.0920897389128855,
0.106285977716751,0.114899921438983,0.122590708880221,0.132228456506715,
0.150991386280156,0.210173358576881,0.25829649839813,0.310541080858129,
0.366555640333151,0.425177707499093,0.481933053819406,0.535242472646899,
0.563024761787985,0.574648209252878,0.581809461553343,0.589496352209351,
0.59974295206476,0.621829632667757,0.680864842162272,0.729716719843076,
0.782756815964081,0.839748558376594,0.881827529122477,0.931141638313032),
 .UNSPECIFIED.);
#2624=B_SPLINE_CURVE_WITH_KNOTS('',3,(#114977,#114978,#114979,#114980,#114981,
#114982,#114983,#114984,#114985,#114986,#114987,#114988,#114989,#114990,
#114991,#114992,#114993,#114994,#114995,#114996,#114997,#114998,#114999,
#115000,#115001,#115002,#115003,#115004,#115005,#115006,#115007,#115008,
#115009,#115010,#115011,#115012),.UNSPECIFIED.,.T.,.F.,(4,2,2,2,2,2,2,2,
2,2,2,2,2,2,2,2,2,4),(0.,0.0579192164299872,0.115915121999537,0.173939752951927,
0.232491074358606,0.290999738521068,0.349702831816148,0.408399067865895,
0.466900664533333,0.525466259798678,0.554212336114783,0.612999379812414,
0.671249213282526,0.729534399890861,0.787757602555752,0.845825377259922,
0.903751470504909,0.931850859346782),.UNSPECIFIED.);
#2625=B_SPLINE_CURVE_WITH_KNOTS('',3,(#115016,#115017,#115018,#115019,#115020,
#115021,#115022,#115023,#115024,#115025,#115026,#115027,#115028,#115029,
#115030,#115031,#115032,#115033,#115034,#115035),.UNSPECIFIED.,.F.,.F.,
(4,2,2,2,2,2,2,2,2,4),(0.139799547746219,0.172474352311618,0.206955199528419,
0.241453517992284,0.276447794358104,0.311395446051869,0.346393507325481,
0.381392485264966,0.416340784159462,0.416668190260015),.UNSPECIFIED.);
#2626=B_SPLINE_CURVE_WITH_KNOTS('',3,(#115039,#115040,#115041,#115042,#115043,
#115044,#115045,#115046,#115047,#115048,#115049,#115050,#115051,#115052,
#115053,#115054,#115055,#115056,#115057,#115058,#115059),.UNSPECIFIED.,
 .F.,.F.,(4,2,2,2,3,2,2,2,2,4),(0.416668190260015,0.451332143736155,0.486542632424401,
0.521110864132053,0.553717878818723,0.588300910930042,0.622838001130257,
0.657310553681014,0.691745956896247,0.693517426564942),.UNSPECIFIED.);
#2627=B_SPLINE_CURVE_WITH_KNOTS('',3,(#115062,#115063,#115064,#115065,#115066,
#115067,#115068,#115069,#115070,#115071,#115072,#115073,#115074,#115075,
#115076,#115077,#115078,#115079,#115080,#115081,#115082,#115083,#115084,
#115085,#115086,#115087,#115088,#115089,#115090,#115091,#115092,#115093,
#115094,#115095,#115096,#115097,#115098,#115099,#115100,#115101,#115102,
#115103,#115104,#115105,#115106,#115107,#115108,#115109,#115110,#115111,
#115112,#115113,#115114,#115115),.UNSPECIFIED.,.T.,.F.,(4,2,2,2,2,2,2,2,
2,2,2,2,2,2,2,2,2,2,2,2,2,2,2,2,2,2,4),(0.,0.0460454477309475,0.0698812709915654,
0.0799729491598215,0.0862398375617845,0.0930070476114817,0.102099779915382,
0.12199128194129,0.173014803100763,0.21515085683549,0.260834825677685,0.309867943965691,
0.360469541845697,0.408816940310194,0.457317861799748,0.475413690833949,
0.484000351732,0.490648733697361,0.497776749178407,0.508849795549764,0.540995625074898,
0.579224411541502,0.621923026586917,0.668213746346409,0.718002156860292,
0.756614424716887,0.804040984351295),.UNSPECIFIED.);
#2628=B_SPLINE_CURVE_WITH_KNOTS('',3,(#115118,#115119,#115120,#115121,#115122,
#115123,#115124,#115125,#115126,#115127,#115128,#115129,#115130,#115131,
#115132,#115133,#115134,#115135,#115136,#115137,#115138,#115139,#115140,
#115141,#115142,#115143,#115144,#115145,#115146,#115147,#115148,#115149,
#115150,#115151,#115152,#115153,#115154,#115155),.UNSPECIFIED.,.T.,.F.,
(4,2,2,2,2,2,2,2,2,2,2,2,2,2,2,2,2,2,4),(0.,0.0500536302415826,0.100248886721465,
0.125348489355815,0.176214379653189,0.226845565123319,0.277601849505133,
0.328529501083987,0.379384828230058,0.430042925474586,0.480747127831807,
0.505624113439625,0.530982199089092,0.581360554251538,0.631694084279792,
0.681899084709615,0.731940525776284,0.781889300824048,0.804562731596483),
 .UNSPECIFIED.);
#2629=B_SPLINE_CURVE_WITH_KNOTS('',3,(#115159,#115160,#115161,#115162,#115163,
#115164,#115165,#115166,#115167,#115168,#115169,#115170,#115171,#115172,
#115173,#115174,#115175,#115176,#115177,#115178,#115179,#115180),
 .UNSPECIFIED.,.F.,.F.,(4,2,2,2,2,2,2,2,2,2,4),(0.21303360006203,0.226832685951809,
0.253402905279486,0.266696066155347,0.279968866775037,0.306991635605764,
0.333954950569698,0.360959243335334,0.388011844627178,0.415040640294028,
0.426047300578329),.UNSPECIFIED.);
#2630=B_SPLINE_CURVE_WITH_KNOTS('',3,(#115184,#115185,#115186,#115187,#115188,
#115189,#115190,#115191,#115192,#115193,#115194,#115195,#115196,#115197,
#115198,#115199,#115200,#115201,#115202,#115203,#115204,#115205,#115206),
 .UNSPECIFIED.,.F.,.F.,(4,3,2,2,2,2,2,2,2,2,4),(0.426047300578329,0.426084033079102,
0.453047560010972,0.4800723465664,0.493315909525459,0.520255179816914,0.5468823927282,
0.573445726460533,0.599943230326549,0.626413995982194,0.639117633141133),
 .UNSPECIFIED.);
#2631=B_SPLINE_CURVE_WITH_KNOTS('',3,(#115209,#115210,#115211,#115212,#115213,
#115214,#115215,#115216,#115217,#115218,#115219,#115220,#115221,#115222,
#115223,#115224,#115225,#115226,#115227,#115228,#115229,#115230,#115231,
#115232,#115233,#115234,#115235,#115236,#115237,#115238,#115239,#115240,
#115241,#115242,#115243,#115244,#115245,#115246,#115247,#115248,#115249,
#115250,#115251,#115252,#115253,#115254,#115255,#115256,#115257,#115258,
#115259,#115260,#115261,#115262),.UNSPECIFIED.,.T.,.F.,(4,2,2,2,2,2,2,2,
2,2,2,2,2,2,2,2,2,2,2,2,2,2,2,2,2,2,4),(0.,0.0413227067380907,0.0531960655412227,
0.060031662678502,0.0658031849778232,0.07263008717472,0.0847877219638444,
0.128472435213838,0.163955924831537,0.202748540799982,0.24453107733556,
0.288498399386162,0.331038302481138,0.369654939117629,0.393537949750696,
0.40285118334134,0.408990585916016,0.414822866875922,0.422642375189097,
0.439661907426131,0.483361718793369,0.519779614744175,0.559444385853513,
0.602194643829491,0.641994578407272,0.665099346451145,0.693838467012807),
 .UNSPECIFIED.);
#2632=B_SPLINE_CURVE_WITH_KNOTS('',3,(#115265,#115266,#115267,#115268,#115269,
#115270,#115271,#115272,#115273,#115274,#115275,#115276,#115277,#115278,
#115279,#115280,#115281,#115282,#115283,#115284,#115285,#115286,#115287,
#115288,#115289,#115290,#115291,#115292,#115293,#115294,#115295,#115296,
#115297,#115298,#115299,#115300),.UNSPECIFIED.,.T.,.F.,(4,2,2,2,2,2,2,2,
2,2,2,2,2,2,2,2,2,4),(0.,0.0431187333258002,0.0865147403830464,0.108243472874369,
0.12987976773851,0.173823473750012,0.217625265484648,0.261500895168154,
0.30446942925918,0.347533682276283,0.391335394292735,0.435259987839497,
0.479528027047697,0.523564188295094,0.567017611697541,0.610192543513944,
0.65314862373146,0.69437312784443),.UNSPECIFIED.);
#2633=B_SPLINE_CURVE_WITH_KNOTS('',3,(#115304,#115305,#115306,#115307,#115308,
#115309,#115310,#115311,#115312,#115313,#115314,#115315,#115316,#115317,
#115318,#115319,#115320,#115321,#115322,#115323,#115324,#115325,#115326),
 .UNSPECIFIED.,.F.,.F.,(4,2,2,2,2,2,2,2,2,3,4),(0.157667239710267,0.158554027511542,
0.17815254113598,0.1978706695312,0.217965348217132,0.237985776857621,0.257972625908517,
0.277739830800538,0.297244191330894,0.315264873286815,0.315290356393478),
 .UNSPECIFIED.);
#2634=B_SPLINE_CURVE_WITH_KNOTS('',3,(#115330,#115331,#115332,#115333,#115334,
#115335,#115336,#115337,#115338,#115339,#115340,#115341,#115342,#115343,
#115344,#115345,#115346,#115347),.UNSPECIFIED.,.F.,.F.,(4,2,2,2,2,2,2,2,
4),(0.315290356393478,0.335251799150366,0.35527186304086,0.37536599132469,
0.395521932534894,0.415225521851564,0.434809279024896,0.454311174901168,
0.472932112997082),.UNSPECIFIED.);
#2635=B_SPLINE_CURVE_WITH_KNOTS('',3,(#115350,#115351,#115352,#115353,#115354,
#115355,#115356,#115357,#115358,#115359,#115360,#115361,#115362,#115363,
#115364,#115365,#115366,#115367,#115368,#115369,#115370,#115371,#115372,
#115373,#115374,#115375,#115376,#115377,#115378,#115379,#115380,#115381,
#115382,#115383,#115384,#115385,#115386,#115387,#115388,#115389,#115390,
#115391,#115392,#115393,#115394,#115395,#115396,#115397,#115398,#115399,
#115400,#115401,#115402,#115403),.UNSPECIFIED.,.T.,.F.,(4,2,2,2,2,2,2,2,
2,2,2,2,2,2,2,2,2,2,2,2,2,2,2,2,2,2,4),(0.,0.0311731506870284,0.0418602132086393,
0.048433128696634,0.0543558575881586,0.0618464529327373,0.0766250168557595,
0.119968052551404,0.155726344679955,0.19481032757455,0.236983053010675,
0.280779560740691,0.322602102638611,0.362770152170366,0.381467742535013,
0.388884220477945,0.394389648003183,0.400355003625582,0.408399663589159,
0.426069229886513,0.469389210961475,0.505710277303957,0.545356763992023,
0.588183425258028,0.630669016411542,0.656032073470706,0.689820287540479),
 .UNSPECIFIED.);
#2636=B_SPLINE_CURVE_WITH_KNOTS('',3,(#115406,#115407,#115408,#115409,#115410,
#115411,#115412,#115413,#115414,#115415,#115416,#115417,#115418,#115419,
#115420,#115421,#115422,#115423,#115424,#115425,#115426,#115427,#115428,
#115429,#115430,#115431,#115432,#115433,#115434,#115435,#115436,#115437,
#115438,#115439,#115440,#115441,#115442,#115443),.UNSPECIFIED.,.T.,.F.,
(4,2,2,2,2,2,2,2,2,2,2,2,2,2,2,2,2,2,4),(0.,0.0426685344635419,0.0857754965458324,
0.107489611928664,0.129156562111911,0.173132822929053,0.216777258109929,
0.260284069552824,0.303288551242756,0.345834109097685,0.389370602799947,
0.433121652565274,0.454607365601712,0.476184832899817,0.520605100709639,
0.564002866904102,0.606959572147738,0.649520039161279,0.690276797053979),
 .UNSPECIFIED.);
#2637=B_SPLINE_CURVE_WITH_KNOTS('',3,(#115447,#115448,#115449,#115450,#115451,
#115452,#115453,#115454,#115455,#115456,#115457,#115458,#115459,#115460,
#115461,#115462,#115463,#115464,#115465,#115466,#115467,#115468,#115469,
#115470,#115471),.UNSPECIFIED.,.F.,.F.,(4,2,2,2,2,2,2,2,2,2,3,4),(0.155275981907625,
0.155530727882454,0.174743293281782,0.194149185772797,0.203888255648882,
0.213620765996803,0.233452450372135,0.253177159350054,0.272625126802198,
0.29176374553163,0.310495193130836,0.310519740065872),.UNSPECIFIED.);
#2638=B_SPLINE_CURVE_WITH_KNOTS('',3,(#115475,#115476,#115477,#115478,#115479,
#115480,#115481,#115482,#115483,#115484,#115485,#115486,#115487,#115488,
#115489,#115490,#115491,#115492,#115493,#115494),.UNSPECIFIED.,.F.,.F.,
(4,2,2,2,2,2,2,2,2,4),(0.310519740065872,0.329735065471992,0.349497188529111,
0.359187916628613,0.368901622450452,0.388823108609513,0.408466318982931,
0.427776988505657,0.446921682939557,0.465771175038461),.UNSPECIFIED.);
#2639=B_SPLINE_CURVE_WITH_KNOTS('',3,(#115497,#115498,#115499,#115500,#115501,
#115502,#115503,#115504,#115505,#115506,#115507,#115508,#115509,#115510,
#115511,#115512,#115513,#115514,#115515,#115516,#115517,#115518,#115519,
#115520,#115521,#115522,#115523,#115524,#115525,#115526,#115527,#115528,
#115529,#115530,#115531,#115532,#115533,#115534,#115535,#115536,#115537,
#115538,#115539,#115540,#115541,#115542,#115543,#115544,#115545,#115546,
#115547,#115548,#115549,#115550,#115551,#115552),.UNSPECIFIED.,.T.,.F.,
(4,2,2,2,2,2,2,2,2,2,2,2,2,2,2,2,2,2,2,2,2,2,2,2,2,2,2,4),(0.,0.0556753555883514,
0.111295357417788,0.132652566908597,0.14142414914753,0.1487293705942,0.156174104643047,
0.166882176783822,0.193563212831233,0.2306943281175,0.277656076892647,0.328982761782772,
0.384093225685445,0.443390367350251,0.500873838595757,0.551867915029868,
0.590932224647382,0.603885289668247,0.611762893866178,0.618812845921861,
0.627674925944102,0.645036014643981,0.704250219211749,0.752276706881969,
0.804643362721499,0.860948773120595,0.894503008286371,0.931042954406025),
 .UNSPECIFIED.);
#2640=B_SPLINE_CURVE_WITH_KNOTS('',3,(#115555,#115556,#115557,#115558,#115559,
#115560,#115561,#115562,#115563,#115564,#115565,#115566,#115567,#115568,
#115569,#115570,#115571,#115572,#115573,#115574,#115575,#115576,#115577,
#115578,#115579,#115580,#115581,#115582,#115583,#115584,#115585,#115586,
#115587,#115588,#115589,#115590),.UNSPECIFIED.,.T.,.F.,(4,2,2,2,2,2,2,2,
2,2,2,2,2,2,2,2,2,4),(0.,0.0579994311336097,0.116029404790947,0.174596164903087,
0.233073341184589,0.291880997534754,0.350877078588918,0.409632811124117,
0.468086866237769,0.526716683879389,0.555532242001599,0.614327126259762,
0.672562416696001,0.730782847087877,0.788903549501615,0.84689624499945,
0.904830147920778,0.931861761959869),.UNSPECIFIED.);
#2641=B_SPLINE_CURVE_WITH_KNOTS('',3,(#115594,#115595,#115596,#115597,#115598,
#115599,#115600,#115601,#115602,#115603,#115604,#115605,#115606,#115607,
#115608,#115609,#115610,#115611),.UNSPECIFIED.,.F.,.F.,(4,2,2,2,2,2,2,2,
4),(0.139799327221814,0.172451176872989,0.206950960902435,0.241917535014109,
0.276864920489073,0.311948417753927,0.347111913059652,0.382185271834272,
0.416673693505186),.UNSPECIFIED.);
#2642=B_SPLINE_CURVE_WITH_KNOTS('',3,(#115615,#115616,#115617,#115618,#115619,
#115620,#115621,#115622,#115623,#115624,#115625,#115626,#115627,#115628,
#115629,#115630,#115631,#115632,#115633,#115634,#115635,#115636,#115637,
#115638,#115639),.UNSPECIFIED.,.F.,.F.,(4,2,2,2,2,2,3,2,2,2,2,4),(0.416673693505186,
0.417127062322145,0.452103545097567,0.469249909212646,0.504177842204279,
0.538741036337965,0.553651070766805,0.588191271421502,0.622688360343799,
0.657151199404152,0.691614448294263,0.693450397988619),.UNSPECIFIED.);
#2643=B_SPLINE_CURVE_WITH_KNOTS('',3,(#115642,#115643,#115644,#115645,#115646,
#115647,#115648,#115649,#115650,#115651,#115652,#115653,#115654,#115655,
#115656,#115657,#115658,#115659,#115660,#115661,#115662,#115663,#115664,
#115665,#115666,#115667,#115668,#115669,#115670,#115671,#115672,#115673,
#115674,#115675,#115676,#115677,#115678,#115679,#115680,#115681,#115682,
#115683,#115684,#115685,#115686,#115687,#115688,#115689,#115690,#115691,
#115692,#115693,#115694,#115695),.UNSPECIFIED.,.T.,.F.,(4,2,2,2,2,2,2,2,
2,2,2,2,2,2,2,2,2,2,2,2,2,2,2,2,2,2,4),(0.,0.0459650663680729,0.0911587487632471,
0.103758532892469,0.11097640426392,0.117058395098765,0.124246356906787,
0.137058808038479,0.187900652546287,0.228756314324871,0.273394922041315,
0.32137662602244,0.372164954082387,0.421627383459268,0.464872751605755,
0.4967655638021,0.507624632110352,0.514319307018795,0.520371447043926,0.528062939766105,
0.543405395719753,0.594209139288907,0.635662798972432,0.680906633143842,
0.729607649348098,0.764590848895352,0.804085254219191),.UNSPECIFIED.);
#2644=B_SPLINE_CURVE_WITH_KNOTS('',3,(#115698,#115699,#115700,#115701,#115702,
#115703,#115704,#115705,#115706,#115707,#115708,#115709,#115710,#115711,
#115712,#115713,#115714,#115715,#115716,#115717,#115718,#115719,#115720,
#115721,#115722,#115723,#115724,#115725,#115726,#115727,#115728,#115729,
#115730,#115731,#115732,#115733,#115734,#115735),.UNSPECIFIED.,.T.,.F.,
(4,2,2,2,2,2,2,2,2,2,2,2,2,2,2,2,2,2,4),(0.,0.050121484155583,0.075216166844529,
0.100319777381396,0.151235204038981,0.20188109216132,0.252602851798492,
0.30345847426458,0.3542470207301,0.404892138611418,0.455654054509687,0.480571332706012,
0.505928132668391,0.556314256329173,0.606659368692688,0.656872239708216,
0.706914001750365,0.756857068749588,0.804567373387168),.UNSPECIFIED.);
#2645=B_SPLINE_CURVE_WITH_KNOTS('',3,(#115739,#115740,#115741,#115742,#115743,
#115744,#115745,#115746,#115747,#115748,#115749,#115750,#115751,#115752,
#115753,#115754,#115755,#115756,#115757,#115758,#115759,#115760),
 .UNSPECIFIED.,.F.,.F.,(4,2,2,2,2,2,2,2,2,2,4),(0.213043644044945,0.213108864360279,
0.23967407776299,0.252966657113423,0.266258274056565,0.293313125821752,
0.320284000338968,0.347266237832029,0.374279444703112,0.401275655429572,
0.426078427446025),.UNSPECIFIED.);
#2646=B_SPLINE_CURVE_WITH_KNOTS('',3,(#115764,#115765,#115766,#115767,#115768,
#115769,#115770,#115771,#115772,#115773,#115774,#115775,#115776,#115777,
#115778,#115779,#115780,#115781,#115782,#115783),.UNSPECIFIED.,.F.,.F.,
(4,2,2,2,2,2,2,2,2,4),(0.426078993093609,0.453084151464664,0.466313597304974,
0.479578787641244,0.506518893015236,0.533152886075883,0.559722291205634,
0.586222004888706,0.612690373328852,0.639122637138555),.UNSPECIFIED.);
#2647=B_SPLINE_CURVE_WITH_KNOTS('',3,(#115786,#115787,#115788,#115789,#115790,
#115791,#115792,#115793,#115794,#115795,#115796,#115797,#115798,#115799,
#115800,#115801,#115802,#115803,#115804,#115805,#115806,#115807,#115808,
#115809,#115810,#115811,#115812,#115813,#115814,#115815,#115816,#115817,
#115818,#115819,#115820,#115821,#115822,#115823,#115824,#115825,#115826,
#115827,#115828,#115829,#115830,#115831,#115832,#115833,#115834,#115835,
#115836,#115837,#115838,#115839),.UNSPECIFIED.,.T.,.F.,(4,2,2,2,2,2,2,2,
2,2,2,2,2,2,2,2,2,2,2,2,2,2,2,2,2,2,4),(0.,0.0358323773236018,0.0680188975168841,
0.0780865576065245,0.0840439994585673,0.0892242253478545,0.0956465843966478,
0.107787393851632,0.151741050997288,0.187190313612102,0.225973380531026,
0.267757326418516,0.311723085858284,0.354237392706437,0.392088501575104,
0.417111408422495,0.426077447776635,0.431749628100514,0.436977282925462,
0.443762257478613,0.457780073244758,0.501521385415829,0.537374319538356,
0.576570360647237,0.618850229147283,0.653290957580071,0.693855228535154),
 .UNSPECIFIED.);
#2648=B_SPLINE_CURVE_WITH_KNOTS('',3,(#115842,#115843,#115844,#115845,#115846,
#115847,#115848,#115849,#115850,#115851,#115852,#115853,#115854,#115855,
#115856,#115857,#115858,#115859,#115860,#115861,#115862,#115863,#115864,
#115865,#115866,#115867,#115868,#115869,#115870,#115871,#115872,#115873,
#115874,#115875,#115876,#115877),.UNSPECIFIED.,.T.,.F.,(4,2,2,2,2,2,2,2,
2,2,2,2,2,2,2,2,2,4),(0.,0.0432393772392339,0.0867357606147896,0.108454670231706,
0.152516802376092,0.196322221380555,0.240080495751704,0.283855323105076,
0.327612995695394,0.371423848910237,0.415499999521694,0.437148924076865,
0.481248840441568,0.524832181184604,0.568165199922297,0.611217062785529,
0.654126345857691,0.694403285213169),.UNSPECIFIED.);
#2649=B_SPLINE_CURVE_WITH_KNOTS('',3,(#115881,#115882,#115883,#115884,#115885,
#115886,#115887,#115888,#115889,#115890,#115891,#115892,#115893,#115894,
#115895,#115896,#115897,#115898,#115899,#115900),.UNSPECIFIED.,.F.,.F.,
(4,2,2,2,2,2,2,2,2,4),(0.157626892744907,0.158356648238268,0.178006478909925,
0.197765608415954,0.217893227495238,0.237918399467858,0.257873965262179,
0.277802919510397,0.297312155754085,0.315258042050784),.UNSPECIFIED.);
#2650=B_SPLINE_CURVE_WITH_KNOTS('',3,(#115904,#115905,#115906,#115907,#115908,
#115909,#115910,#115911,#115912,#115913,#115914,#115915,#115916,#115917,
#115918,#115919,#115920,#115921,#115922,#115923,#115924),.UNSPECIFIED.,
 .F.,.F.,(4,3,2,2,2,2,2,2,2,4),(0.315258042050784,0.315279326727019,0.335308798957692,
0.35544106154069,0.375647730314253,0.395414743460894,0.415069475378914,
0.434609381924642,0.454099654500455,0.472906219471926),.UNSPECIFIED.);
#2651=B_SPLINE_CURVE_WITH_KNOTS('',3,(#115927,#115928,#115929,#115930,#115931,
#115932,#115933,#115934,#115935,#115936,#115937,#115938,#115939,#115940,
#115941,#115942,#115943,#115944,#115945,#115946,#115947,#115948,#115949,
#115950,#115951,#115952,#115953,#115954,#115955,#115956,#115957,#115958,
#115959,#115960,#115961,#115962,#115963,#115964,#115965,#115966,#115967,
#115968,#115969,#115970,#115971,#115972,#115973,#115974,#115975,#115976,
#115977,#115978,#115979,#115980,#115981,#115982),.UNSPECIFIED.,.T.,.F.,
(4,2,2,2,2,2,2,2,2,2,2,2,2,2,2,2,2,2,2,2,2,2,2,2,2,2,2,4),(0.,0.0390375792045744,
0.0590178458522155,0.0672194166711689,0.0722183955160815,0.0775479853100994,
0.0845994732587413,0.0996572237805605,0.14299992688214,0.178716701234394,
0.217786016234129,0.259956657972089,0.303755112722266,0.345545654433592,
0.38476471673647,0.404243229009083,0.412309823986064,0.417253897181447,
0.422545396002088,0.429579934992201,0.444717708915258,0.488060644137423,
0.523877949673102,0.563102122736068,0.605510200655335,0.643225976330391,
0.664545279498856,0.689830282636683),.UNSPECIFIED.);
#2652=B_SPLINE_CURVE_WITH_KNOTS('',3,(#115985,#115986,#115987,#115988,#115989,
#115990,#115991,#115992,#115993,#115994,#115995,#115996,#115997,#115998,
#115999,#116000,#116001,#116002,#116003,#116004,#116005,#116006,#116007,
#116008,#116009,#116010,#116011,#116012,#116013,#116014,#116015,#116016,
#116017,#116018,#116019,#116020,#116021,#116022),.UNSPECIFIED.,.T.,.F.,
(4,2,2,2,2,2,2,2,2,2,2,2,2,2,2,2,2,2,4),(0.,0.0429286760162795,0.0862893470429538,
0.107869956323031,0.15168893150141,0.195288381210701,0.238885645590843,
0.281412823568044,0.323975646504692,0.367552260777747,0.411219341914282,
0.432643267861024,0.454142634616226,0.498425946874695,0.541789855901478,
0.584712513093188,0.627258856393838,0.669718871101792,0.69031086887045),
 .UNSPECIFIED.);
#2653=B_SPLINE_CURVE_WITH_KNOTS('',3,(#116026,#116027,#116028,#116029,#116030,
#116031,#116032,#116033,#116034,#116035,#116036,#116037,#116038,#116039,
#116040,#116041,#116042,#116043,#116044,#116045,#116046,#116047),
 .UNSPECIFIED.,.F.,.F.,(4,2,2,2,2,2,2,2,2,2,4),(0.155281525707715,0.165407413678005,
0.184837154921267,0.194547083649518,0.204241569791125,0.224004541735763,
0.243710040103625,0.263152667016854,0.282283166620068,0.301416643807714,
0.310510623695354),.UNSPECIFIED.);
#2654=B_SPLINE_CURVE_WITH_KNOTS('',3,(#116051,#116052,#116053,#116054,#116055,
#116056,#116057,#116058,#116059,#116060,#116061,#116062,#116063,#116064,
#116065,#116066,#116067,#116068,#116069,#116070),.UNSPECIFIED.,.F.,.F.,
(4,2,2,2,2,2,2,2,2,4),(0.310510783932394,0.33021534549801,0.349975556798286,
0.359654748676357,0.37951365110717,0.399147572564983,0.418436153684863,
0.43757097487398,0.456683395879265,0.465792149403069),.UNSPECIFIED.);
#2655=B_SPLINE_CURVE_WITH_KNOTS('',3,(#116073,#116074,#116075,#116076,#116077,
#116078,#116079,#116080,#116081,#116082,#116083,#116084,#116085,#116086,
#116087,#116088,#116089,#116090,#116091,#116092,#116093,#116094,#116095,
#116096,#116097,#116098,#116099,#116100,#116101,#116102,#116103,#116104,
#116105,#116106,#116107,#116108,#116109,#116110,#116111,#116112,#116113,
#116114,#116115,#116116,#116117,#116118,#116119,#116120,#116121,#116122,
#116123,#116124,#116125,#116126),.UNSPECIFIED.,.T.,.F.,(4,2,2,2,2,2,2,2,
2,2,2,2,2,2,2,2,2,2,2,2,2,2,2,2,2,2,4),(0.,0.0577066589623385,0.108220241511108,
0.155025064619134,0.168566924488323,0.176486388257448,0.183196502035754,
0.19130287220519,0.206035894029007,0.26494305616825,0.312215986498219,0.36379987608317,
0.419167761629723,0.477871964115765,0.535180527979754,0.584787120836968,
0.622981568939877,0.63542970577016,0.642952510898312,0.648987621127709,
0.657075914044929,0.672025070963926,0.731047633253834,0.778568461524894,
0.83053501913079,0.880505757758383,0.931203521812045),.UNSPECIFIED.);
#2656=B_SPLINE_CURVE_WITH_KNOTS('',3,(#116129,#116130,#116131,#116132,#116133,
#116134,#116135,#116136,#116137,#116138,#116139,#116140,#116141,#116142,
#116143,#116144,#116145,#116146,#116147,#116148,#116149,#116150,#116151,
#116152,#116153,#116154,#116155,#116156,#116157,#116158,#116159,#116160,
#116161,#116162,#116163,#116164),.UNSPECIFIED.,.T.,.F.,(4,2,2,2,2,2,2,2,
2,2,2,2,2,2,2,2,2,4),(0.,0.0580062210999761,0.116027500581797,0.174539501268387,
0.233085095091822,0.291851800270691,0.350586183609165,0.4090941168664,0.467658902805053,
0.496406714569538,0.525691391466127,0.583914495393509,0.642183460479962,
0.700438611055605,0.758574908135443,0.816555683924175,0.874457701625133,
0.931848830026075),.UNSPECIFIED.);
#2657=B_SPLINE_CURVE_WITH_KNOTS('',3,(#116168,#116169,#116170,#116171,#116172,
#116173,#116174,#116175,#116176,#116177,#116178,#116179,#116180,#116181,
#116182,#116183,#116184,#116185),.UNSPECIFIED.,.F.,.F.,(4,2,2,2,2,2,2,2,
4),(0.139756359393238,0.172379146205813,0.206875888117782,0.241848498189916,
0.276811650419912,0.311843728956546,0.346869648108179,0.381826442196638,
0.416625798777337),.UNSPECIFIED.);
#2658=B_SPLINE_CURVE_WITH_KNOTS('',3,(#116189,#116190,#116191,#116192,#116193,
#116194,#116195,#116196,#116197,#116198,#116199,#116200,#116201,#116202,
#116203,#116204,#116205,#116206,#116207,#116208,#116209,#116210,#116211,
#116212,#116213),.UNSPECIFIED.,.F.,.F.,(4,2,2,2,2,2,3,2,2,2,2,4),(0.416625798777337,
0.416811988200141,0.433955298027859,0.4513600485358,0.48592734829649,0.520509887106317,
0.553630915158508,0.588160307888751,0.622630239726201,0.657069905215908,
0.69152400979313,0.693387274551746),.UNSPECIFIED.);
#2659=B_SPLINE_CURVE_WITH_KNOTS('',3,(#116216,#116217,#116218,#116219,#116220,
#116221,#116222,#116223,#116224,#116225,#116226,#116227,#116228,#116229,
#116230,#116231,#116232,#116233,#116234,#116235,#116236,#116237,#116238,
#116239,#116240,#116241,#116242,#116243,#116244,#116245,#116246,#116247,
#116248,#116249,#116250,#116251,#116252,#116253,#116254,#116255,#116256,
#116257,#116258,#116259,#116260,#116261,#116262,#116263,#116264,#116265,
#116266,#116267,#116268,#116269),.UNSPECIFIED.,.T.,.F.,(4,2,2,2,2,2,2,2,
2,2,2,2,2,2,2,2,2,2,2,2,2,2,2,2,2,2,4),(0.,0.0491414753089632,0.0925487839832437,
0.122593144975948,0.132847468349746,0.139193738324383,0.14495264583004,
0.152307953678182,0.167132411558137,0.217957911591671,0.25914050175531,
0.304055332305895,0.35231689455287,0.403065556918838,0.452265829412814,
0.495942952242087,0.525036206824292,0.535088756106163,0.54134412715987,
0.547042237653256,0.554348484673671,0.56916221793295,0.619983908515213,
0.661298626737727,0.706438873808049,0.755042331569686,0.804148478915545),
 .UNSPECIFIED.);
#2660=B_SPLINE_CURVE_WITH_KNOTS('',3,(#116272,#116273,#116274,#116275,#116276,
#116277,#116278,#116279,#116280,#116281,#116282,#116283,#116284,#116285,
#116286,#116287,#116288,#116289,#116290,#116291,#116292,#116293,#116294,
#116295,#116296,#116297,#116298,#116299,#116300,#116301,#116302,#116303,
#116304,#116305,#116306,#116307,#116308,#116309),.UNSPECIFIED.,.T.,.F.,
(4,2,2,2,2,2,2,2,2,2,2,2,2,2,2,2,2,2,4),(0.,0.0501833807776728,0.0752864723656921,
0.12626759651476,0.176927418053835,0.227597522568229,0.278358481987529,
0.329065980432407,0.379699791417318,0.430534861965737,0.455501787095014,
0.480856165965872,0.531251764035078,0.581611739513776,0.63183513372458,
0.681877255988317,0.731811481032622,0.781785602018675,0.804591288052395),
 .UNSPECIFIED.);
#2661=B_SPLINE_CURVE_WITH_KNOTS('',3,(#116313,#116314,#116315,#116316,#116317,
#116318,#116319,#116320,#116321,#116322,#116323,#116324,#116325,#116326,
#116327,#116328,#116329,#116330,#116331,#116332,#116333,#116334),
 .UNSPECIFIED.,.F.,.F.,(4,2,2,2,2,2,2,2,2,2,4),(0.213057265421291,0.226444841366151,
0.239736816501714,0.253034106200005,0.280126668221598,0.3071042938041,0.334056714793563,
0.36101913045305,0.387974252130544,0.414936420729693,0.42607613571615),
 .UNSPECIFIED.);
#2662=B_SPLINE_CURVE_WITH_KNOTS('',3,(#116338,#116339,#116340,#116341,#116342,
#116343,#116344,#116345,#116346,#116347,#116348,#116349,#116350,#116351,
#116352,#116353,#116354,#116355,#116356,#116357,#116358,#116359,#116360),
 .UNSPECIFIED.,.F.,.F.,(4,3,2,2,2,2,2,2,2,2,4),(0.42607613571615,0.426097060646127,
0.453209656703842,0.466641094363468,0.493308893322814,0.519950454049193,
0.546525916596096,0.57302682164241,0.599491300460783,0.625982272547063,
0.639154326067418),.UNSPECIFIED.);
#2663=B_SPLINE_CURVE_WITH_KNOTS('',3,(#116363,#116364,#116365,#116366,#116367,
#116368,#116369,#116370,#116371,#116372,#116373,#116374,#116375,#116376,
#116377,#116378,#116379,#116380,#116381,#116382,#116383,#116384,#116385,
#116386,#116387,#116388,#116389,#116390,#116391,#116392,#116393,#116394,
#116395,#116396,#116397,#116398,#116399,#116400,#116401,#116402,#116403,
#116404,#116405,#116406,#116407,#116408,#116409,#116410,#116411,#116412,
#116413,#116414,#116415,#116416,#116417,#116418),.UNSPECIFIED.,.T.,.F.,
(4,2,2,2,2,2,2,2,2,2,2,2,2,2,2,2,2,2,2,2,2,2,2,2,2,2,2,4),(0.,0.041285253628399,
0.0822448660680709,0.0978610724808867,0.10400629769675,0.108568719624014,
0.113522581485496,0.120239297953382,0.13525770505281,0.178998524482636,
0.214867867279051,0.254013558218206,0.296165829644769,0.340059680648694,
0.382165264453309,0.420785265606447,0.442102674108075,0.450101530221598,
0.455290600040355,0.460169421252104,0.466649080514575,0.480606708590981,
0.524360856110365,0.560151574991358,0.599306833792761,0.6415526782016,0.666591170965427,
0.693884097625634),.UNSPECIFIED.);
#2664=B_SPLINE_CURVE_WITH_KNOTS('',3,(#116421,#116422,#116423,#116424,#116425,
#116426,#116427,#116428,#116429,#116430,#116431,#116432,#116433,#116434,
#116435,#116436,#116437,#116438,#116439,#116440,#116441,#116442,#116443,
#116444,#116445,#116446,#116447,#116448,#116449,#116450,#116451,#116452,
#116453,#116454,#116455,#116456),.UNSPECIFIED.,.T.,.F.,(4,2,2,2,2,2,2,2,
2,2,2,2,2,2,2,2,2,4),(0.,0.043430317645468,0.0876189818453222,0.131490406017855,
0.17529842262449,0.219243734427261,0.262215746345614,0.305308136875401,
0.34910933896524,0.393004507675874,0.414540236113842,0.45894962553968,0.502489821198032,
0.545774652003282,0.588801627501863,0.63172385035613,0.674765513237447,
0.694442278112711),.UNSPECIFIED.);
#2665=B_SPLINE_CURVE_WITH_KNOTS('',3,(#116460,#116461,#116462,#116463,#116464,
#116465,#116466,#116467,#116468,#116469,#116470,#116471,#116472,#116473,
#116474,#116475,#116476,#116477,#116478,#116479),.UNSPECIFIED.,.F.,.F.,
(4,2,2,2,2,2,2,2,2,4),(0.157627193529841,0.167716827321412,0.187814282331985,
0.207836144110288,0.227821673078062,0.247827083298905,0.267342985260238,
0.28685856777808,0.306450487286998,0.315250728700652),.UNSPECIFIED.);
#2666=B_SPLINE_CURVE_WITH_KNOTS('',3,(#116483,#116484,#116485,#116486,#116487,
#116488,#116489,#116490,#116491,#116492,#116493,#116494,#116495,#116496,
#116497,#116498,#116499,#116500,#116501,#116502,#116503,#116504,#116505),
 .UNSPECIFIED.,.F.,.F.,(4,3,2,2,2,2,2,2,2,2,4),(0.315250728700652,0.315252659637721,
0.335252771579398,0.345044128740003,0.365147854527748,0.385081661646758,
0.404715888785962,0.424245396326341,0.443741595607751,0.463297264804012,
0.472879853167562),.UNSPECIFIED.);
#2667=B_SPLINE_CURVE_WITH_KNOTS('',3,(#116508,#116509,#116510,#116511,#116512,
#116513,#116514,#116515,#116516,#116517,#116518,#116519,#116520,#116521,
#116522,#116523,#116524,#116525,#116526,#116527,#116528,#116529,#116530,
#116531,#116532,#116533,#116534,#116535,#116536,#116537,#116538,#116539,
#116540,#116541,#116542,#116543,#116544,#116545,#116546,#116547,#116548,
#116549,#116550,#116551,#116552,#116553,#116554,#116555,#116556,#116557,
#116558,#116559,#116560,#116561,#116562,#116563),.UNSPECIFIED.,.T.,.F.,
(4,2,2,2,2,2,2,2,2,2,2,2,2,2,2,2,2,2,2,2,2,2,2,2,2,2,2,4),(0.,0.0389094768208776,
0.077644299909024,0.0869793188239608,0.0930343010064621,0.0978595661268027,
0.103266182813461,0.112206308441846,0.142773526660472,0.175527151159333,
0.212208114415353,0.252134756286138,0.29519266441111,0.338693154248625,
0.378978774214529,0.421865026269376,0.431590686763012,0.437742921379179,
0.442544488371915,0.447820266261681,0.456311320145132,0.483432074234788,
0.51556966970483,0.551845054032032,0.591482878005452,0.63432148952688,0.660439037839305,
0.689835002387049),.UNSPECIFIED.);
#2668=B_SPLINE_CURVE_WITH_KNOTS('',3,(#116566,#116567,#116568,#116569,#116570,
#116571,#116572,#116573,#116574,#116575,#116576,#116577,#116578,#116579,
#116580,#116581,#116582,#116583,#116584,#116585,#116586,#116587,#116588,
#116589,#116590,#116591,#116592,#116593,#116594,#116595,#116596,#116597,
#116598,#116599,#116600,#116601,#116602,#116603),.UNSPECIFIED.,.T.,.F.,
(4,2,2,2,2,2,2,2,2,2,2,2,2,2,2,2,2,2,4),(0.,0.0431561762404372,0.0648561590452176,
0.0864916690642867,0.130405697248895,0.174030302676733,0.217566990876258,
0.260102189498512,0.302668301258938,0.346227368299971,0.389977906413364,
0.411459041889591,0.433027647489369,0.477425144947406,0.520797890347173,
0.563724989172446,0.606272249689026,0.648733187794411,0.690383069014513),
 .UNSPECIFIED.);
#2669=B_SPLINE_CURVE_WITH_KNOTS('',3,(#116607,#116608,#116609,#116610,#116611,
#116612,#116613,#116614,#116615,#116616,#116617,#116618,#116619,#116620,
#116621,#116622,#116623,#116624,#116625,#116626,#116627,#116628),
 .UNSPECIFIED.,.F.,.F.,(4,2,2,2,2,2,2,2,2,2,4),(0.155275319539932,0.155472519940377,
0.174899463638446,0.184631482355954,0.194352939394403,0.214162137141302,
0.233879076545751,0.253319079372333,0.272453534450712,0.291587356219028,
0.310541455171113),.UNSPECIFIED.);
#2670=B_SPLINE_CURVE_WITH_KNOTS('',3,(#116632,#116633,#116634,#116635,#116636,
#116637,#116638,#116639,#116640,#116641,#116642,#116643,#116644,#116645,
#116646,#116647,#116648,#116649,#116650,#116651,#116652,#116653,#116654),
 .UNSPECIFIED.,.F.,.F.,(4,3,2,2,2,2,2,2,2,2,4),(0.310541455171113,0.310542742432682,
0.330303977577274,0.339991361015711,0.349699012642844,0.369606133275464,
0.389237991660081,0.408533484226866,0.42767172155954,0.446783628648094,
0.465818061972614),.UNSPECIFIED.);
#2671=B_SPLINE_CURVE_WITH_KNOTS('',3,(#116657,#116658,#116659,#116660,#116661,
#116662,#116663,#116664,#116665,#116666,#116667,#116668,#116669,#116670,
#116671,#116672,#116673,#116674,#116675,#116676,#116677,#116678,#116679,
#116680,#116681,#116682,#116683,#116684,#116685,#116686,#116687,#116688,
#116689,#116690,#116691,#116692,#116693,#116694,#116695,#116696,#116697,
#116698,#116699,#116700,#116701,#116702,#116703,#116704,#116705,#116706,
#116707,#116708,#116709,#116710,#116711,#116712),.UNSPECIFIED.,.T.,.F.,
(4,2,2,2,2,2,2,2,2,2,2,2,2,2,2,2,2,2,2,2,2,2,2,2,2,2,2,4),(0.,0.0584891512695919,
0.114492542178861,0.167895255153171,0.192926962144756,0.203201312515091,
0.209475661727826,0.216178889385321,0.225078797588162,0.244244249149783,
0.303228610481566,0.351253205348421,0.40344779802583,0.459430920400994,
0.518055048404651,0.574790904207356,0.626379818080268,0.656739046234691,
0.667820528375868,0.674906502512356,0.681494594812286,0.690134018443859,
0.708330275060749,0.767556059783576,0.81565597509107,0.86809846809008,0.89975349026725,
0.931147159319543),.UNSPECIFIED.);
#2672=B_SPLINE_CURVE_WITH_KNOTS('',3,(#116715,#116716,#116717,#116718,#116719,
#116720,#116721,#116722,#116723,#116724,#116725,#116726,#116727,#116728,
#116729,#116730,#116731,#116732,#116733,#116734,#116735,#116736,#116737,
#116738,#116739,#116740,#116741,#116742,#116743,#116744,#116745,#116746,
#116747,#116748,#116749,#116750),.UNSPECIFIED.,.T.,.F.,(4,2,2,2,2,2,2,2,
2,2,2,2,2,2,2,2,2,4),(0.,0.0580273876658578,0.116624709778379,0.175109980248094,
0.233875067237791,0.292781005354475,0.351458258505243,0.409917402953638,
0.468652301333266,0.497938514908916,0.556156374039708,0.614407784487279,
0.672639310224047,0.730758072220705,0.788738683692563,0.846658543028034,
0.904617546167748,0.931861050654944),.UNSPECIFIED.);
#2673=B_SPLINE_CURVE_WITH_KNOTS('',3,(#116754,#116755,#116756,#116757,#116758,
#116759,#116760,#116761,#116762,#116763,#116764,#116765,#116766,#116767,
#116768,#116769,#116770,#116771),.UNSPECIFIED.,.F.,.F.,(4,2,2,2,2,2,2,2,
4),(0.13975667624528,0.172385107747455,0.207377997148642,0.242328900489864,
0.277382835898854,0.312493359299448,0.347523544103189,0.382466335247368,
0.416631398225218),.UNSPECIFIED.);
#2674=B_SPLINE_CURVE_WITH_KNOTS('',3,(#116775,#116776,#116777,#116778,#116779,
#116780,#116781,#116782,#116783,#116784,#116785,#116786,#116787,#116788,
#116789,#116790,#116791,#116792,#116793,#116794,#116795,#116796,#116797,
#116798,#116799),.UNSPECIFIED.,.F.,.F.,(4,2,2,2,2,2,3,2,2,2,2,4),(0.416631398225218,
0.417494170154389,0.434899729575189,0.469463645133473,0.504035272545212,
0.538595601414024,0.55364530802227,0.588140235067004,0.6225958952251,0.657050905834583,
0.691532621286376,0.69340198426755),.UNSPECIFIED.);
#2675=B_SPLINE_CURVE_WITH_KNOTS('',3,(#116802,#116803,#116804,#116805,#116806,
#116807,#116808,#116809,#116810,#116811,#116812,#116813,#116814,#116815,
#116816,#116817,#116818,#116819,#116820,#116821,#116822,#116823,#116824,
#116825,#116826,#116827,#116828,#116829,#116830,#116831,#116832,#116833,
#116834,#116835,#116836,#116837,#116838,#116839,#116840,#116841,#116842,
#116843,#116844,#116845,#116846,#116847,#116848,#116849,#116850,#116851,
#116852,#116853,#116854,#116855,#116856,#116857),.UNSPECIFIED.,.T.,.F.,
(4,2,2,2,2,2,2,2,2,2,2,2,2,2,2,2,2,2,2,2,2,2,2,2,2,2,2,4),(0.,0.050309885077182,
0.0968176213990348,0.14561500811571,0.156739046106578,0.163807644338246,
0.16934707395481,0.175458686824546,0.185355150398173,0.217530128519313,
0.25516696991148,0.297395878474636,0.343189130145614,0.392358357282366,
0.442924870955592,0.490985306930195,0.538391227704406,0.55636629273847,
0.564315592840812,0.569898862718201,0.575587019218597,0.583774116525507,
0.604278624054994,0.655331471969062,0.697522159209062,0.743402500798943,
0.773581445154641,0.804063549998697),.UNSPECIFIED.);
#2676=B_SPLINE_CURVE_WITH_KNOTS('',3,(#116860,#116861,#116862,#116863,#116864,
#116865,#116866,#116867,#116868,#116869,#116870,#116871,#116872,#116873,
#116874,#116875,#116876,#116877,#116878,#116879,#116880,#116881,#116882,
#116883,#116884,#116885,#116886,#116887,#116888,#116889,#116890,#116891,
#116892,#116893,#116894,#116895),.UNSPECIFIED.,.T.,.F.,(4,2,2,2,2,2,2,2,
2,2,2,2,2,2,2,2,2,4),(0.,0.0251012805543509,0.0501415752591219,0.100917082239335,
0.151542035486755,0.202362336623636,0.253360602597951,0.304245574169001,
0.354898572509294,0.405593370032142,0.45672129467809,0.507094850947286,
0.557408623612551,0.607586772950294,0.657611039698548,0.707566257516175,
0.757588498528219,0.804710998356802),.UNSPECIFIED.);
#2677=B_SPLINE_CURVE_WITH_KNOTS('',3,(#116899,#116900,#116901,#116902,#116903,
#116904,#116905,#116906,#116907,#116908,#116909,#116910,#116911,#116912,
#116913,#116914,#116915,#116916,#116917,#116918),.UNSPECIFIED.,.F.,.F.,
(4,2,2,2,2,2,2,2,2,4),(0.213045309439027,0.225903171160768,0.23915487036106,
0.266145051380448,0.293105692945154,0.320136249990941,0.34662148809123,
0.373143786348127,0.400118964953456,0.426087518215633),.UNSPECIFIED.);
#2678=B_SPLINE_CURVE_WITH_KNOTS('',3,(#116922,#116923,#116924,#116925,#116926,
#116927,#116928,#116929,#116930,#116931,#116932,#116933,#116934,#116935,
#116936,#116937,#116938,#116939,#116940,#116941,#116942,#116943,#116944,
#116945,#116946),.UNSPECIFIED.,.F.,.F.,(4,3,2,2,2,2,2,2,2,2,2,4),(0.426087518215633,
0.426092043059227,0.439294541944362,0.452527327986773,0.479465410345481,
0.506084663851214,0.532639176079408,0.559132814855581,0.58560811112673,
0.612122033742717,0.638703850902336,0.639137352498254),.UNSPECIFIED.);
#2679=B_SPLINE_CURVE_WITH_KNOTS('',3,(#116949,#116950,#116951,#116952,#116953,
#116954,#116955,#116956,#116957,#116958,#116959,#116960,#116961,#116962,
#116963,#116964,#116965,#116966,#116967,#116968,#116969,#116970,#116971,
#116972,#116973,#116974,#116975,#116976,#116977,#116978,#116979,#116980,
#116981,#116982,#116983,#116984,#116985,#116986,#116987,#116988,#116989,
#116990,#116991,#116992,#116993,#116994,#116995,#116996,#116997,#116998,
#116999,#117000,#117001,#117002,#117003,#117004),.UNSPECIFIED.,.T.,.F.,
(4,2,2,2,2,2,2,2,2,2,2,2,2,2,2,2,2,2,2,2,2,2,2,2,2,2,2,4),(0.,0.04306450588528,
0.0799275659781319,0.115025434929688,0.124575396355486,0.130036613772263,
0.134639877230734,0.140088544983391,0.149845294197815,0.191581859546887,
0.22622904912325,0.264381554721172,0.305567799522646,0.349957215317373,
0.392932910186313,0.428785627015779,0.462395684866412,0.471727343819009,
0.477108322028563,0.481213516207419,0.486467047619745,0.495487409345996,
0.529647573843035,0.563205873397388,0.600581186566829,0.641128664104466,
0.667016282704079,0.693823417143794),.UNSPECIFIED.);
#2680=B_SPLINE_CURVE_WITH_KNOTS('',3,(#117007,#117008,#117009,#117010,#117011,
#117012,#117013,#117014,#117015,#117016,#117017,#117018,#117019,#117020,
#117021,#117022,#117023,#117024,#117025,#117026,#117027,#117028,#117029,
#117030,#117031,#117032,#117033,#117034,#117035,#117036,#117037,#117038,
#117039,#117040,#117041,#117042),.UNSPECIFIED.,.T.,.F.,(4,2,2,2,2,2,2,2,
2,2,2,2,2,2,2,2,2,4),(0.,0.0435201388237783,0.0876896865062443,0.131556050902525,
0.175347888012368,0.219184263957841,0.263011932322101,0.306802442037427,
0.350712621875749,0.372257866489833,0.393892414057866,0.437988072782709,
0.481550707432859,0.524854944245018,0.567888576652302,0.610803761428183,
0.653830385515191,0.69446576879133),.UNSPECIFIED.);
#2681=B_SPLINE_CURVE_WITH_KNOTS('',3,(#117046,#117047,#117048,#117049,#117050,
#117051,#117052,#117053,#117054,#117055,#117056,#117057,#117058,#117059,
#117060,#117061,#117062,#117063,#117064,#117065,#117066),.UNSPECIFIED.,
 .F.,.F.,(4,2,2,2,2,2,2,2,3,4),(0.157656823790096,0.177236697355346,0.197336849182283,
0.217351967607823,0.237321518579206,0.256846128436631,0.276358786518457,
0.296332744546969,0.315265150459455,0.315307705902751),.UNSPECIFIED.);
#2682=B_SPLINE_CURVE_WITH_KNOTS('',3,(#117070,#117071,#117072,#117073,#117074,
#117075,#117076,#117077,#117078,#117079,#117080,#117081,#117082,#117083,
#117084,#117085,#117086,#117087,#117088,#117089,#117090,#117091),
 .UNSPECIFIED.,.F.,.F.,(4,2,2,2,2,2,2,2,2,2,4),(0.315307705902751,0.325075072158519,
0.33490628806666,0.355089026447615,0.374851285877192,0.394499906238306,
0.4140370791025,0.433530763726022,0.453075863775059,0.472735940924408,0.472921974249551),
 .UNSPECIFIED.);
#2683=B_SPLINE_CURVE_WITH_KNOTS('',3,(#117094,#117095,#117096,#117097,#117098,
#117099,#117100,#117101,#117102,#117103,#117104,#117105,#117106,#117107,
#117108,#117109,#117110,#117111,#117112,#117113,#117114,#117115,#117116,
#117117,#117118,#117119,#117120,#117121,#117122,#117123,#117124,#117125,
#117126,#117127,#117128,#117129,#117130,#117131,#117132,#117133,#117134,
#117135,#117136,#117137,#117138,#117139,#117140,#117141,#117142,#117143,
#117144,#117145,#117146,#117147,#117148,#117149),.UNSPECIFIED.,.T.,.F.,
(4,2,2,2,2,2,2,2,2,2,2,2,2,2,2,2,2,2,2,2,2,2,2,2,2,2,2,4),(0.,0.0420957482556104,
0.0788204825590171,0.10439842115468,0.112737593521854,0.117799011810767,
0.121877536406845,0.127372490945778,0.137643300991004,0.180988892763695,
0.215730960955723,0.25400272679975,0.295405998843111,0.339374438240802,
0.381943378576841,0.418153695727972,0.448316824505312,0.457119676510764,
0.462312317182371,0.466786340130831,0.472200775743362,0.482227367612323,
0.525497676632813,0.560258387201869,0.598610612973799,0.640171176621586,
0.664290506141458,0.689921488883007),.UNSPECIFIED.);
#2684=B_SPLINE_CURVE_WITH_KNOTS('',3,(#117152,#117153,#117154,#117155,#117156,
#117157,#117158,#117159,#117160,#117161,#117162,#117163,#117164,#117165,
#117166,#117167,#117168,#117169,#117170,#117171,#117172,#117173,#117174,
#117175,#117176,#117177,#117178,#117179,#117180,#117181,#117182,#117183,
#117184,#117185,#117186,#117187,#117188,#117189),.UNSPECIFIED.,.T.,.F.,
(4,2,2,2,2,2,2,2,2,2,2,2,2,2,2,2,2,2,4),(0.,0.0433710488880423,0.0650253824547739,
0.108968254486875,0.152596643322638,0.196107206689574,0.238642946636128,
0.281214225978943,0.32477135649117,0.368564045409551,0.390072545346376,
0.411672777792178,0.455677790431156,0.499049066862304,0.541971910087472,
0.584515751159163,0.626977488416304,0.669703944754416,0.690418361534604),
 .UNSPECIFIED.);
#2685=B_SPLINE_CURVE_WITH_KNOTS('',3,(#117193,#117194,#117195,#117196,#117197,
#117198,#117199,#117200,#117201,#117202,#117203,#117204,#117205,#117206,
#117207,#117208,#117209,#117210,#117211,#117212,#117213,#117214),
 .UNSPECIFIED.,.F.,.F.,(4,2,2,2,2,2,2,2,2,2,4),(0.155304109067118,0.165313690891263,
0.175054466501976,0.184785723582231,0.204609586111903,0.224327485013603,
0.243761651045815,0.262895169247043,0.282030889979258,0.301296683977728,
0.310555525369536),.UNSPECIFIED.);
#2686=B_SPLINE_CURVE_WITH_KNOTS('',3,(#117218,#117219,#117220,#117221,#117222,
#117223,#117224,#117225,#117226,#117227,#117228,#117229,#117230,#117231,
#117232,#117233,#117234,#117235,#117236,#117237,#117238,#117239,#117240),
 .UNSPECIFIED.,.F.,.F.,(4,3,2,2,2,2,2,2,2,2,4),(0.310555525369536,0.31055833948538,
0.330390740094614,0.340111031893878,0.360037161153345,0.37966238872268,
0.398954774450647,0.418091310700888,0.437204580349564,0.456440316485847,
0.465862448552498),.UNSPECIFIED.);
#2687=B_SPLINE_CURVE_WITH_KNOTS('',3,(#117243,#117244,#117245,#117246,#117247,
#117248,#117249,#117250,#117251,#117252,#117253,#117254,#117255,#117256,
#117257,#117258,#117259,#117260,#117261,#117262,#117263,#117264,#117265,
#117266,#117267,#117268,#117269,#117270,#117271,#117272,#117273,#117274,
#117275,#117276,#117277,#117278,#117279,#117280,#117281,#117282,#117283,
#117284,#117285,#117286,#117287,#117288,#117289,#117290,#117291,#117292,
#117293,#117294,#117295,#117296),.UNSPECIFIED.,.T.,.F.,(4,2,2,2,2,2,2,2,
2,2,2,2,2,2,2,2,2,2,2,2,2,2,2,2,2,2,4),(0.,0.0588899148675681,0.116713784598351,
0.168127032983557,0.217161756198921,0.230708488164785,0.238481790712691,
0.245045683531671,0.252825342057254,0.266770879667179,0.325680310196297,
0.372778207213426,0.424230111324823,0.479472421391073,0.538189063657707,
0.59558791103362,0.645483611950939,0.685162679203097,0.697581033759298,
0.704951114140878,0.711376767007497,0.719368887500008,0.734569892864707,
0.793812168199268,0.841381833347496,0.888689256421084,0.931225999577531),
 .UNSPECIFIED.);
#2688=B_SPLINE_CURVE_WITH_KNOTS('',3,(#117299,#117300,#117301,#117302,#117303,
#117304,#117305,#117306,#117307,#117308,#117309,#117310,#117311,#117312,
#117313,#117314,#117315,#117316,#117317,#117318,#117319,#117320,#117321,
#117322,#117323,#117324,#117325,#117326,#117327,#117328,#117329,#117330,
#117331,#117332,#117333,#117334,#117335,#117336),.UNSPECIFIED.,.T.,.F.,
(4,2,2,2,2,2,2,2,2,2,2,2,2,2,2,2,2,2,4),(0.,0.0586869128804075,0.117101756083158,
0.175809300555675,0.234870079029752,0.293836105351144,0.352394127952532,
0.410832470887651,0.439493106921451,0.468301655288093,0.527096860275995,
0.585318822752492,0.643517734326523,0.701618600084167,0.759606971398693,
0.817555987879628,0.875547839400924,0.903528726059672,0.931729138475359),
 .UNSPECIFIED.);
#2689=B_SPLINE_CURVE_WITH_KNOTS('',3,(#117340,#117341,#117342,#117343,#117344,
#117345,#117346,#117347,#117348,#117349,#117350,#117351,#117352,#117353,
#117354,#117355,#117356,#117357,#117358,#117359),.UNSPECIFIED.,.F.,.F.,
(4,2,2,2,2,2,2,2,2,4),(0.139842570142282,0.172920078696101,0.207831273050215,
0.242880597158898,0.278083844108549,0.3132558378693,0.348251982782376,0.383159208999535,
0.400246012749396,0.416635718978169),.UNSPECIFIED.);
#2690=B_SPLINE_CURVE_WITH_KNOTS('',3,(#117363,#117364,#117365,#117366,#117367,
#117368,#117369,#117370,#117371,#117372,#117373,#117374,#117375,#117376,
#117377,#117378,#117379,#117380,#117381,#117382,#117383,#117384,#117385),
 .UNSPECIFIED.,.F.,.F.,(4,2,2,2,2,3,2,2,2,2,4),(0.416635718978169,0.417378505027386,
0.45230554511966,0.486859439730073,0.521400572944025,0.553633145844837,
0.588108965928037,0.622576103225218,0.657062747984201,0.691566133172587,
0.69347571598712),.UNSPECIFIED.);
#2691=B_SPLINE_CURVE_WITH_KNOTS('',3,(#117388,#117389,#117390,#117391,#117392,
#117393,#117394,#117395,#117396,#117397,#117398,#117399,#117400,#117401,
#117402,#117403,#117404,#117405,#117406,#117407,#117408,#117409,#117410,
#117411,#117412,#117413,#117414,#117415,#117416,#117417,#117418,#117419,
#117420,#117421,#117422,#117423,#117424,#117425,#117426,#117427,#117428,
#117429,#117430,#117431,#117432,#117433,#117434,#117435,#117436,#117437,
#117438,#117439,#117440,#117441),.UNSPECIFIED.,.T.,.F.,(4,2,2,2,2,2,2,2,
2,2,2,2,2,2,2,2,2,2,2,2,2,2,2,2,2,2,4),(0.,0.0507741420462431,0.100094123453666,
0.142359412560989,0.175922593461849,0.186328843425225,0.19249408395989,
0.197866628454765,0.204549652896258,0.217280256032914,0.268351707683292,
0.309145879302129,0.353756216170168,0.401722317023322,0.45251258636343,
0.501967269874822,0.544179399225482,0.578035171108809,0.588420444970115,
0.594538564389574,0.599898813169662,0.60649676894749,0.619034943707488,
0.670068082662381,0.710950255764047,0.755747830094524,0.804181423392594),
 .UNSPECIFIED.);
#2692=B_SPLINE_CURVE_WITH_KNOTS('',3,(#117444,#117445,#117446,#117447,#117448,
#117449,#117450,#117451,#117452,#117453,#117454,#117455,#117456,#117457,
#117458,#117459,#117460,#117461,#117462,#117463,#117464,#117465,#117466,
#117467,#117468,#117469,#117470,#117471,#117472,#117473,#117474,#117475,
#117476,#117477,#117478,#117479),.UNSPECIFIED.,.T.,.F.,(4,2,2,2,2,2,2,2,
2,2,2,2,2,2,2,2,2,4),(0.,0.0250756242963306,0.0759095369482803,0.126546430158223,
0.177318372769854,0.228228295543835,0.279038395635305,0.329682630992297,
0.380447242003444,0.431684110304875,0.482066275987924,0.532392855418118,
0.582579304112608,0.632602831630785,0.68254973102261,0.73256082187328,0.782716074484924,
0.804734027170493),.UNSPECIFIED.);
#2693=B_SPLINE_CURVE_WITH_KNOTS('',3,(#117483,#117484,#117485,#117486,#117487,
#117488,#117489,#117490,#117491,#117492,#117493,#117494,#117495,#117496,
#117497,#117498,#117499,#117500,#117501,#117502),.UNSPECIFIED.,.F.,.F.,
(4,2,2,2,2,2,2,2,2,4),(0.213048682846188,0.226000664813719,0.253024885755239,
0.279991915565222,0.306995259686518,0.334036256070164,0.361049651624042,
0.388018253154667,0.415023294971757,0.426106451248178),.UNSPECIFIED.);
#2694=B_SPLINE_CURVE_WITH_KNOTS('',3,(#117506,#117507,#117508,#117509,#117510,
#117511,#117512,#117513,#117514,#117515,#117516,#117517,#117518,#117519,
#117520,#117521,#117522,#117523,#117524,#117525,#117526,#117527,#117528,
#117529,#117530),.UNSPECIFIED.,.F.,.F.,(4,3,2,2,2,2,2,2,2,2,2,4),(0.426106451248178,
0.426109299341064,0.43936868528645,0.466306397762246,0.492932086443071,
0.519491619644926,0.545986019938596,0.57245772480979,0.598965803631853,
0.625542456621915,0.638837591160798,0.639157982187252),.UNSPECIFIED.);
#2695=B_SPLINE_CURVE_WITH_KNOTS('',3,(#117533,#117534,#117535,#117536,#117537,
#117538,#117539,#117540,#117541,#117542,#117543,#117544,#117545,#117546,
#117547,#117548,#117549,#117550,#117551,#117552,#117553,#117554,#117555,
#117556,#117557,#117558,#117559,#117560,#117561,#117562,#117563,#117564,
#117565,#117566,#117567,#117568,#117569,#117570,#117571,#117572,#117573,
#117574,#117575,#117576,#117577,#117578,#117579,#117580,#117581,#117582,
#117583,#117584,#117585,#117586,#117587,#117588),.UNSPECIFIED.,.T.,.F.,
(4,2,2,2,2,2,2,2,2,2,2,2,2,2,2,2,2,2,2,2,2,2,2,2,2,2,2,4),(0.,0.0438032399281999,
0.0853607593781,0.124677963323405,0.143031430545011,0.150221652844284,0.154521557014495,
0.159050218307573,0.16495937041696,0.17733329248977,0.221130773605562,0.256510956710958,
0.295260135268376,0.337023841203116,0.380996197810603,0.423508283158955,
0.460147416455634,0.487374794940251,0.495858730912228,0.500900770187446,
0.505305273252891,0.510799058391344,0.521314368148725,0.565233583186423,
0.600368519153137,0.638991263532745,0.66668607501751,0.693911448956519),
 .UNSPECIFIED.);
#2696=B_SPLINE_CURVE_WITH_KNOTS('',3,(#117591,#117592,#117593,#117594,#117595,
#117596,#117597,#117598,#117599,#117600,#117601,#117602,#117603,#117604,
#117605,#117606,#117607,#117608,#117609,#117610,#117611,#117612,#117613,
#117614,#117615,#117616,#117617,#117618,#117619,#117620,#117621,#117622,
#117623,#117624,#117625,#117626,#117627,#117628),.UNSPECIFIED.,.T.,.F.,
(4,2,2,2,2,2,2,2,2,2,2,2,2,2,2,2,2,2,4),(0.,0.021720404281955,0.0658046663067377,
0.109640478743245,0.153471770102935,0.196955906477114,0.239974074579092,
0.283788922227855,0.327660640057054,0.349176397554091,0.370772527384884,
0.415295853168791,0.458843328684095,0.502130984362252,0.545156609874512,
0.588077379151349,0.631120466938282,0.674432102515339,0.694392108277034),
 .UNSPECIFIED.);
#2697=B_SPLINE_CURVE_WITH_KNOTS('',3,(#117632,#117633,#117634,#117635,#117636,
#117637,#117638,#117639,#117640,#117641,#117642,#117643,#117644,#117645,
#117646,#117647,#117648,#117649,#117650,#117651,#117652,#117653,#117654,
#117655,#117656),.UNSPECIFIED.,.F.,.F.,(4,2,2,2,2,2,2,2,2,2,3,4),(0.157639235373943,
0.157642233535094,0.167484880448895,0.187547965451918,0.207549295069419,
0.227535872366622,0.24705560360124,0.266571987452983,0.286162045201152,
0.306173181062702,0.315228898222867,0.315250512378167),.UNSPECIFIED.);
#2698=B_SPLINE_CURVE_WITH_KNOTS('',3,(#117660,#117661,#117662,#117663,#117664,
#117665,#117666,#117667,#117668,#117669,#117670,#117671,#117672,#117673,
#117674,#117675,#117676,#117677,#117678,#117679),.UNSPECIFIED.,.F.,.F.,
(4,2,2,2,2,2,2,2,2,4),(0.315250512378167,0.325044189685063,0.345194921525286,
0.365124037617517,0.38476096157514,0.404291501464033,0.423787526395124,
0.443342675224153,0.463014699867811,0.47286813359681),.UNSPECIFIED.);
#2699=B_SPLINE_CURVE_WITH_KNOTS('',3,(#117682,#117683,#117684,#117685,#117686,
#117687,#117688,#117689,#117690,#117691,#117692,#117693,#117694,#117695,
#117696,#117697,#117698,#117699,#117700,#117701,#117702,#117703,#117704,
#117705,#117706,#117707,#117708,#117709,#117710,#117711,#117712,#117713,
#117714,#117715,#117716,#117717,#117718,#117719,#117720,#117721,#117722,
#117723,#117724,#117725,#117726,#117727,#117728,#117729,#117730,#117731,
#117732,#117733,#117734,#117735,#117736,#117737),.UNSPECIFIED.,.T.,.F.,
(4,2,2,2,2,2,2,2,2,2,2,2,2,2,2,2,2,2,2,2,2,2,2,2,2,2,2,4),(0.,0.043359114946712,
0.0827966930249876,0.124519807183276,0.133530885608685,0.139173275794822,
0.143546227845922,0.14832491485639,0.155971051546056,0.180254156404085,
0.211494752418665,0.247084720750642,0.286072070810718,0.328176388927468,
0.371998745260341,0.413838162940434,0.451257260030457,0.473742030125035,
0.481413100726095,0.486171801486404,0.490501981131898,0.496054323204978,
0.5073444923318,0.550744168012344,0.585751764291186,0.624314498227347,0.65718029277283,
0.689956049972293),.UNSPECIFIED.);
#2700=B_SPLINE_CURVE_WITH_KNOTS('',3,(#117740,#117741,#117742,#117743,#117744,
#117745,#117746,#117747,#117748,#117749,#117750,#117751,#117752,#117753,
#117754,#117755,#117756,#117757,#117758,#117759,#117760,#117761,#117762,
#117763,#117764,#117765,#117766,#117767,#117768,#117769,#117770,#117771,
#117772,#117773,#117774,#117775,#117776,#117777),.UNSPECIFIED.,.T.,.F.,
(4,2,2,2,2,2,2,2,2,2,2,2,2,2,2,2,2,2,4),(0.,0.0216485531474219,0.0432173037461375,
0.0870175786107822,0.130618682039334,0.174231294254911,0.216757996492257,
0.259351610024986,0.30293769448103,0.34664050390938,0.368085861126179,0.389609200257064,
0.433928919817407,0.477263108896134,0.520150204902444,0.562682206963715,
0.605164701416418,0.64793524162617,0.690474681070088),.UNSPECIFIED.);
#2701=B_SPLINE_CURVE_WITH_KNOTS('',3,(#117781,#117782,#117783,#117784,#117785,
#117786,#117787,#117788,#117789,#117790,#117791,#117792,#117793,#117794,
#117795,#117796,#117797,#117798,#117799,#117800),.UNSPECIFIED.,.F.,.F.,
(4,2,2,2,2,2,2,2,2,4),(0.155292405987498,0.164791612401374,0.174486676683334,
0.194251067647735,0.213959456186071,0.233396530522292,0.252527635537242,
0.271671379434195,0.290952375222479,0.310581312971656),.UNSPECIFIED.);
#2702=B_SPLINE_CURVE_WITH_KNOTS('',3,(#117804,#117805,#117806,#117807,#117808,
#117809,#117810,#117811,#117812,#117813,#117814,#117815,#117816,#117817,
#117818,#117819,#117820,#117821,#117822,#117823,#117824,#117825,#117826,
#117827,#117828),.UNSPECIFIED.,.F.,.F.,(4,3,2,2,2,2,2,2,2,2,2,4),(0.310581312971656,
0.310585453103689,0.320254584528652,0.329939011021033,0.349806464126837,
0.369431787280329,0.38871220797298,0.407845471371859,0.426966696725866,
0.446218186332258,0.465665653817226,0.465877859091187),.UNSPECIFIED.);
#2703=B_SPLINE_CURVE_WITH_KNOTS('',3,(#117831,#117832,#117833,#117834,#117835,
#117836,#117837,#117838,#117839,#117840,#117841,#117842,#117843,#117844,
#117845,#117846,#117847,#117848,#117849,#117850,#117851,#117852,#117853,
#117854,#117855,#117856,#117857,#117858,#117859,#117860,#117861,#117862,
#117863,#117864,#117865,#117866,#117867,#117868,#117869,#117870,#117871,
#117872,#117873,#117874,#117875,#117876,#117877,#117878,#117879,#117880,
#117881,#117882,#117883,#117884),.UNSPECIFIED.,.T.,.F.,(4,2,2,2,2,2,2,2,
2,2,2,2,2,2,2,2,2,2,2,2,2,2,2,2,2,2,4),(0.,0.0564712967416743,0.115038347531717,
0.171525153227716,0.223338045127873,0.253169957371529,0.264328308664071,
0.271555564478627,0.278342122584976,0.287342292159235,0.306677164918464,
0.365666117627072,0.413730164621536,0.465954645778289,0.521966597945684,
0.580586451721482,0.637296030517189,0.689137603931885,0.718928884525764,
0.730000625988998,0.737143075518541,0.743827557819252,0.752656747560013,
0.771478924689879,0.830418531004859,0.878603082634546,0.931260313331436),
 .UNSPECIFIED.);
#2704=B_SPLINE_CURVE_WITH_KNOTS('',3,(#117888,#117889,#117890,#117891,#117892,
#117893,#117894,#117895,#117896,#117897,#117898,#117899,#117900,#117901,
#117902,#117903,#117904,#117905,#117906,#117907,#117908,#117909,#117910,
#117911,#117912,#117913,#117914,#117915,#117916,#117917,#117918,#117919,
#117920,#117921,#117922,#117923,#117924,#117925,#117926,#117927,#117928,
#117929,#117930,#117931,#117932,#117933,#117934,#117935,#117936,#117937,
#117938,#117939,#117940,#117941,#117942,#117943,#117944,#117945,#117946,
#117947,#117948,#117949,#117950,#117951,#117952,#117953,#117954,#117955,
#117956,#117957,#117958,#117959,#117960,#117961,#117962,#117963,#117964,
#117965,#117966,#117967,#117968,#117969,#117970,#117971,#117972,#117973,
#117974,#117975,#117976,#117977,#117978,#117979,#117980,#117981,#117982,
#117983,#117984,#117985,#117986,#117987,#117988,#117989,#117990,#117991,
#117992,#117993,#117994,#117995,#117996,#117997,#117998,#117999,#118000,
#118001,#118002,#118003,#118004,#118005,#118006,#118007,#118008,#118009,
#118010,#118011),.UNSPECIFIED.,.F.,.F.,(4,3,3,3,3,3,3,3,3,3,3,3,3,3,3,3,
3,3,3,3,3,3,3,3,3,3,3,3,3,3,3,3,3,3,3,3,3,3,3,3,3,4),(0.,0.000132780866822235,
0.000266873743469484,0.000288904340061033,0.000405509517205523,0.000522002177348785,
0.000577808680122067,0.000712482869108472,0.00084747631154527,0.0008667130201831,
0.000975050275463839,0.00108341287396082,0.00115561736024413,0.00130428113167908,
0.00145285915006363,0.00160154905450121,0.00173342604036622,0.00188138755364419,
0.00202924107209608,0.00217717427357142,0.00231123472048831,0.00242030735385376,
0.0025293260926867,0.00260013906054927,0.00273508332987814,0.00286987804292202,
0.00288904340061024,0.00300313603185183,0.0031173273659021,0.0031779477406712,
0.00331220596338911,0.00344530795511321,0.00346685208073216,0.00367373680256345,
0.00389128296162316,0.004044660760854,0.00417924015261657,0.00431424687026292,
0.00433356510091496,0.00444155537662282,0.00454955744617284,0.00462246944097592),
 .UNSPECIFIED.);
#2705=B_SPLINE_CURVE_WITH_KNOTS('',3,(#118012,#118013,#118014,#118015,#118016,
#118017,#118018,#118019,#118020,#118021,#118022,#118023,#118024,#118025,
#118026,#118027,#118028,#118029,#118030,#118031),.UNSPECIFIED.,.F.,.F.,
(4,2,2,2,2,2,2,2,2,4),(1.00000017144998E-6,0.0589091086023463,0.116821182098481,
0.174782248585886,0.232882215848222,0.290811365541089,0.348733625156973,
0.406721474339845,0.436820554289351,0.465866613116424),.UNSPECIFIED.);
#2706=B_SPLINE_CURVE_WITH_KNOTS('',3,(#118035,#118036,#118037,#118038,#118039,
#118040,#118041,#118042,#118043,#118044,#118045,#118046,#118047,#118048,
#118049,#118050,#118051,#118052,#118053,#118054,#118055,#118056),
 .UNSPECIFIED.,.F.,.F.,(4,2,2,2,2,2,2,2,2,2,4),(0.139811245314732,0.155709821294679,
0.1906606447556,0.225651069631098,0.260726976222177,0.295779710904132,0.330740401449915,
0.365720622817098,0.38286162399923,0.4002666603197,0.416590733425148),
 .UNSPECIFIED.);
#2707=B_SPLINE_CURVE_WITH_KNOTS('',3,(#118060,#118061,#118062,#118063,#118064,
#118065,#118066,#118067,#118068,#118069,#118070,#118071,#118072,#118073,
#118074,#118075,#118076,#118077,#118078,#118079,#118080,#118081,#118082),
 .UNSPECIFIED.,.F.,.F.,(4,2,2,2,2,3,2,2,2,2,4),(0.416590733425148,0.434833062902334,
0.469409572199181,0.503972722175614,0.538489176242052,0.553563397262184,
0.588014339663571,0.62246556895172,0.656945200368898,0.674174237448786,
0.693374642576916),.UNSPECIFIED.);
#2708=B_SPLINE_CURVE_WITH_KNOTS('',3,(#118085,#118086,#118087,#118088,#118089,
#118090,#118091,#118092,#118093,#118094,#118095,#118096,#118097,#118098,
#118099,#118100,#118101,#118102,#118103,#118104,#118105,#118106,#118107,
#118108,#118109,#118110,#118111,#118112,#118113,#118114,#118115,#118116,
#118117,#118118,#118119,#118120,#118121,#118122,#118123,#118124,#118125,
#118126,#118127,#118128,#118129,#118130,#118131,#118132,#118133,#118134,
#118135,#118136,#118137,#118138,#118139,#118140),.UNSPECIFIED.,.T.,.F.,
(4,2,2,2,2,2,2,2,2,2,2,2,2,2,2,2,2,2,2,2,2,2,2,2,2,2,2,4),(0.,0.0499191511799086,
0.100323798483693,0.147430853941386,0.19733219387334,0.209533422841237,
0.21681600564989,0.222358234196958,0.228220671789085,0.23719913857369,0.262853256702964,
0.299031751002697,0.340252278981359,0.385205828086949,0.433510601774857,
0.484252817009215,0.533401629552871,0.576802914325161,0.606031391015876,
0.615813482963946,0.621815274859459,0.627228741894021,0.63409986671774,
0.647815955990171,0.69869320668563,0.739781768645123,0.773567944088127,
0.804062709433453),.UNSPECIFIED.);
#2709=B_SPLINE_CURVE_WITH_KNOTS('',3,(#118143,#118144,#118145,#118146,#118147,
#118148,#118149,#118150,#118151,#118152,#118153,#118154,#118155,#118156,
#118157,#118158,#118159,#118160,#118161,#118162,#118163,#118164,#118165,
#118166,#118167,#118168,#118169,#118170,#118171,#118172,#118173,#118174,
#118175,#118176,#118177,#118178),.UNSPECIFIED.,.T.,.F.,(4,2,2,2,2,2,2,2,
2,2,2,2,2,2,2,2,2,4),(0.,0.0508102428370469,0.101446446049902,0.15223400388986,
0.203157794195011,0.253970631498262,0.304612808351331,0.355379759922047,
0.406622741889554,0.45700292782468,0.507323471911212,0.557501934458369,
0.607520193736365,0.657468271381405,0.707486102342854,0.75764833283291,
0.781103021944058,0.80473316872163),.UNSPECIFIED.);
#2710=B_SPLINE_CURVE_WITH_KNOTS('',3,(#118182,#118183,#118184,#118185,#118186,
#118187,#118188,#118189,#118190,#118191,#118192,#118193,#118194,#118195,
#118196,#118197,#118198,#118199,#118200,#118201,#118202),.UNSPECIFIED.,
 .F.,.F.,(4,2,2,2,2,2,2,2,3,4),(0.213076350460928,0.239748662991589,0.266715218453498,
0.293725024577096,0.32077322414254,0.347789969932072,0.37475820239879,0.401761549963476,
0.426157396856437,0.426182397841807),.UNSPECIFIED.);
#2711=B_SPLINE_CURVE_WITH_KNOTS('',3,(#118206,#118207,#118208,#118209,#118210,
#118211,#118212,#118213,#118214,#118215,#118216,#118217,#118218,#118219,
#118220,#118221,#118222,#118223,#118224,#118225,#118226,#118227),
 .UNSPECIFIED.,.F.,.F.,(4,2,2,2,2,2,2,2,2,2,4),(0.426182397841807,0.453093828382958,
0.479716429177484,0.506272416039609,0.532764847505401,0.559237494928504,
0.585748871646683,0.612328914248202,0.625624663661876,0.638890854983996,
0.639233747317365),.UNSPECIFIED.);
#2712=B_SPLINE_CURVE_WITH_KNOTS('',3,(#118230,#118231,#118232,#118233,#118234,
#118235,#118236,#118237,#118238,#118239,#118240,#118241,#118242,#118243,
#118244,#118245,#118246,#118247,#118248,#118249,#118250,#118251,#118252,
#118253,#118254,#118255,#118256,#118257,#118258,#118259,#118260,#118261,
#118262,#118263,#118264,#118265,#118266,#118267,#118268,#118269,#118270,
#118271,#118272,#118273,#118274,#118275,#118276,#118277,#118278,#118279,
#118280,#118281,#118282,#118283,#118284,#118285),.UNSPECIFIED.,.T.,.F.,
(4,2,2,2,2,2,2,2,2,2,2,2,2,2,2,2,2,2,2,2,2,2,2,2,2,2,2,4),(0.,0.0442480422944534,
0.0874111550741445,0.124982769447723,0.161567305412722,0.17022981975583,
0.175839348378204,0.18030752670857,0.185315270085969,0.193607980645255,
0.222268058354423,0.254709421019499,0.291191815675512,0.330870616067579,
0.373576985297977,0.417325574307142,0.458614686770495,0.499167985772272,
0.514540802408916,0.521132469232114,0.525273371147843,0.529792346622681,
0.535963995927171,0.549975098997772,0.593804620572848,0.629550277964284,
0.663265595848305,0.693902648410645),.UNSPECIFIED.);
#2713=B_SPLINE_CURVE_WITH_KNOTS('',3,(#118288,#118289,#118290,#118291,#118292,
#118293,#118294,#118295,#118296,#118297,#118298,#118299,#118300,#118301,
#118302,#118303,#118304,#118305,#118306,#118307,#118308,#118309,#118310,
#118311,#118312,#118313,#118314,#118315,#118316,#118317,#118318,#118319,
#118320,#118321,#118322,#118323,#118324,#118325),.UNSPECIFIED.,.T.,.F.,
(4,2,2,2,2,2,2,2,2,2,2,2,2,2,2,2,2,2,4),(0.,0.0439639503368589,0.0877604826916409,
0.131653516194325,0.174628164548689,0.217655865061386,0.261503244306837,
0.305316782533662,0.326788961668223,0.348329007627559,0.39274923929494,
0.436273490381119,0.479536625012623,0.522550458846832,0.565478794845261,
0.608544620564116,0.651881382844738,0.673041580934267,0.69438925335854),
 .UNSPECIFIED.);
#2714=B_SPLINE_CURVE_WITH_KNOTS('',3,(#118329,#118330,#118331,#118332,#118333,
#118334,#118335,#118336,#118337,#118338,#118339,#118340,#118341,#118342,
#118343,#118344,#118345,#118346,#118347,#118348),.UNSPECIFIED.,.F.,.F.,
(4,2,2,2,2,2,2,2,2,4),(0.157613569881594,0.177590621004305,0.197575064366368,
0.21738044374067,0.236894863818513,0.256415359500327,0.276016696532489,
0.296001655089685,0.305565247158479,0.315223462967867),.UNSPECIFIED.);
#2715=B_SPLINE_CURVE_WITH_KNOTS('',3,(#118352,#118353,#118354,#118355,#118356,
#118357,#118358,#118359,#118360,#118361,#118362,#118363,#118364,#118365,
#118366,#118367,#118368,#118369,#118370,#118371,#118372,#118373,#118374,
#118375,#118376),.UNSPECIFIED.,.F.,.F.,(4,3,2,2,2,2,2,2,2,2,2,4),(0.315223462967867,
0.315228090781128,0.335331383930744,0.355256493204118,0.374879646147263,
0.394403179322639,0.413902980207927,0.433470625988996,0.453156745636569,
0.462992521725115,0.472807666153366,0.472841660662722),.UNSPECIFIED.);
#2716=B_SPLINE_CURVE_WITH_KNOTS('',3,(#118379,#118380,#118381,#118382,#118383,
#118384,#118385,#118386,#118387,#118388,#118389,#118390,#118391,#118392,
#118393,#118394,#118395,#118396,#118397,#118398,#118399,#118400,#118401,
#118402,#118403,#118404,#118405,#118406,#118407,#118408,#118409,#118410,
#118411,#118412,#118413,#118414,#118415,#118416,#118417,#118418,#118419,
#118420,#118421,#118422,#118423,#118424,#118425,#118426,#118427,#118428,
#118429,#118430,#118431,#118432,#118433,#118434),.UNSPECIFIED.,.T.,.F.,
(4,2,2,2,2,2,2,2,2,2,2,2,2,2,2,2,2,2,2,2,2,2,2,2,2,2,2,4),(0.,0.0439238371863919,
0.0861902321541546,0.122000766940326,0.150399248999695,0.158716774702034,
0.16364349810409,0.167903904328712,0.173082066416487,0.182746594055837,
0.22600984128997,0.260588517680107,0.298734181935875,0.340021026144596,
0.384008664161648,0.426668835524534,0.460906519679387,0.494393680768921,
0.502475247123739,0.507752815267995,0.511987106073311,0.516766095538759,
0.524760138175885,0.553180307333632,0.585302647338573,0.621597531052235,
0.656973501569907,0.689916370643902),.UNSPECIFIED.);
#2717=B_SPLINE_CURVE_WITH_KNOTS('',3,(#118437,#118438,#118439,#118440,#118441,
#118442,#118443,#118444,#118445,#118446,#118447,#118448,#118449,#118450,
#118451,#118452,#118453,#118454,#118455,#118456,#118457,#118458,#118459,
#118460,#118461,#118462,#118463,#118464,#118465,#118466,#118467,#118468,
#118469,#118470,#118471,#118472,#118473,#118474),.UNSPECIFIED.,.T.,.F.,
(4,2,2,2,2,2,2,2,2,2,2,2,2,2,2,2,2,2,4),(0.,0.0215971103688694,0.0654425307483053,
0.109049877051987,0.152622345814217,0.195150110292293,0.237745904043596,
0.28132562175596,0.325081612743124,0.346562119435945,0.368126525189833,
0.412507376679562,0.455838675269931,0.498719845806797,0.54124703606024,
0.583729631416507,0.626505135491807,0.669729282213455,0.690488132151514),
 .UNSPECIFIED.);
#2718=B_SPLINE_CURVE_WITH_KNOTS('',3,(#118478,#118479,#118480,#118481,#118482,
#118483,#118484,#118485,#118486,#118487,#118488,#118489,#118490,#118491,
#118492,#118493,#118494,#118495,#118496,#118497,#118498,#118499,#118500),
 .UNSPECIFIED.,.F.,.F.,(4,2,2,2,2,2,2,2,2,3,4),(0.155318197570125,0.164879844339497,
0.184666529440326,0.204377543531482,0.223808485417644,0.242939179394705,
0.262083926601905,0.281366837067981,0.301126438334268,0.310590172209869,
0.310609150032715),.UNSPECIFIED.);
#2719=B_SPLINE_CURVE_WITH_KNOTS('',3,(#118504,#118505,#118506,#118507,#118508,
#118509,#118510,#118511,#118512,#118513,#118514,#118515,#118516,#118517,
#118518,#118519,#118520,#118521,#118522,#118523,#118524,#118525),
 .UNSPECIFIED.,.F.,.F.,(4,2,2,2,2,2,2,2,2,2,4),(0.310609150032715,0.320291308615886,
0.340184624148909,0.359802870962863,0.379081454733931,0.398213338810906,
0.417334739031231,0.436587884463708,0.456037397362742,0.46576085708419,
0.465908369779994),.UNSPECIFIED.);
#2720=B_SPLINE_CURVE_WITH_KNOTS('',3,(#118528,#118529,#118530,#118531,#118532,
#118533,#118534,#118535,#118536,#118537,#118538,#118539,#118540,#118541,
#118542,#118543,#118544,#118545,#118546,#118547,#118548,#118549,#118550,
#118551,#118552,#118553,#118554,#118555,#118556,#118557,#118558,#118559,
#118560,#118561,#118562,#118563,#118564,#118565,#118566,#118567,#118568,
#118569,#118570,#118571,#118572,#118573,#118574,#118575,#118576,#118577,
#118578,#118579,#118580,#118581),.UNSPECIFIED.,.T.,.F.,(4,2,2,2,2,2,2,2,
2,2,2,2,2,2,2,2,2,2,2,2,2,2,2,2,2,2,4),(0.,0.0541686820922835,0.112415580690374,
0.170510262941422,0.223981665771125,0.277387759445974,0.290674307093365,
0.299367584212841,0.306340517334599,0.31419709898001,0.327276125557507,
0.372458093488531,0.417746341578146,0.467801168688974,0.521727313250452,
0.579585888464177,0.637746424232553,0.691244422142438,0.743421281273534,
0.756491088086435,0.765054568557719,0.771929131539263,0.77967896178005,
0.792584427627161,0.837109936091434,0.882412481374293,0.931190701269262),
 .UNSPECIFIED.);
#2721=B_SPLINE_CURVE_WITH_KNOTS('',3,(#118585,#118586,#118587,#118588,#118589,
#118590,#118591,#118592,#118593,#118594,#118595,#118596,#118597,#118598,
#118599,#118600,#118601,#118602,#118603,#118604,#118605,#118606,#118607,
#118608,#118609,#118610,#118611,#118612,#118613,#118614,#118615,#118616,
#118617,#118618,#118619,#118620,#118621,#118622,#118623,#118624,#118625,
#118626,#118627,#118628,#118629,#118630,#118631,#118632,#118633,#118634,
#118635,#118636,#118637,#118638,#118639,#118640,#118641,#118642,#118643,
#118644,#118645,#118646,#118647,#118648,#118649,#118650,#118651,#118652,
#118653,#118654,#118655,#118656,#118657,#118658,#118659,#118660,#118661,
#118662,#118663,#118664,#118665,#118666,#118667,#118668,#118669,#118670,
#118671,#118672,#118673,#118674,#118675,#118676,#118677,#118678,#118679,
#118680,#118681,#118682,#118683,#118684,#118685,#118686,#118687,#118688,
#118689,#118690,#118691,#118692,#118693,#118694,#118695,#118696,#118697,
#118698,#118699,#118700,#118701,#118702,#118703,#118704,#118705,#118706,
#118707,#118708),.UNSPECIFIED.,.F.,.F.,(4,3,3,3,3,3,3,3,3,3,3,3,3,3,3,3,
3,3,3,3,3,3,3,3,3,3,3,3,3,3,3,3,3,3,3,3,3,3,3,3,3,4),(0.,0.00013277251793653,
0.000266857202581178,0.000288907094292459,0.000405479252460701,0.000521939192059059,
0.000577814188584917,0.000712479190419921,0.000847463317123744,0.000866721282877376,
0.00097506874242616,0.00108344212283471,0.00115562837716983,0.00130427764647303,
0.00145284128808089,0.00160151709564146,0.00173344256575487,0.00188142671647943,
0.00202930303207845,0.00217725917594754,0.0023112567543399,0.00242030890240509,
0.00252930785338822,0.00260016384863234,0.0027351175251363,0.00286991989522071,
0.00288907094292478,0.00300323587270697,0.00311750014522043,0.00317797803721722,
0.00331224152428824,0.00344534695923621,0.00346688513150965,0.00367342646213443,
0.00389049440139844,0.00404469932009453,0.00417928189170992,0.00431428786646436,
0.00433360641438694,0.00444159423475505,0.00454959321591867,0.00462251350867935),
 .UNSPECIFIED.);
#2722=B_SPLINE_CURVE_WITH_KNOTS('',3,(#118709,#118710,#118711,#118712,#118713,
#118714,#118715,#118716,#118717,#118718,#118719,#118720,#118721,#118722,
#118723,#118724,#118725,#118726,#118727,#118728),.UNSPECIFIED.,.F.,.F.,
(4,2,2,2,2,2,2,2,2,4),(1.0000001659162E-6,0.0587516845672802,0.116678515181389,
0.174707853111328,0.232881544735254,0.29079726537627,0.3487559236141,0.377742355197926,
0.423463627058049,0.465815224763171),.UNSPECIFIED.);
#2723=B_SPLINE_CURVE_WITH_KNOTS('',3,(#118732,#118733,#118734,#118735,#118736,
#118737,#118738,#118739,#118740,#118741,#118742,#118743,#118744,#118745,
#118746,#118747,#118748,#118749,#118750,#118751),.UNSPECIFIED.,.F.,.F.,
(4,2,2,2,2,2,2,2,2,4),(0.139779656786197,0.173396151004641,0.208397696003322,
0.243489615098716,0.27855188804276,0.313513313892874,0.348489752671695,
0.365628705522415,0.383033972564603,0.416570719226277),.UNSPECIFIED.);
#2724=B_SPLINE_CURVE_WITH_KNOTS('',3,(#118755,#118756,#118757,#118758,#118759,
#118760,#118761,#118762,#118763,#118764,#118765,#118766,#118767,#118768,
#118769,#118770,#118771,#118772,#118773,#118774,#118775,#118776,#118777,
#118778,#118779),.UNSPECIFIED.,.F.,.F.,(4,2,2,2,2,3,2,2,2,2,2,4),(0.416570719226277,
0.417599765181018,0.45217391626731,0.486733498952397,0.521247003328364,
0.553550457873372,0.587998762871438,0.622466686453937,0.639693726684147,
0.656923100441351,0.692000901398468,0.69333011465957),.UNSPECIFIED.);
#2725=B_SPLINE_CURVE_WITH_KNOTS('',3,(#118782,#118783,#118784,#118785,#118786,
#118787,#118788,#118789,#118790,#118791,#118792,#118793,#118794,#118795,
#118796,#118797,#118798,#118799,#118800,#118801,#118802,#118803,#118804,
#118805,#118806,#118807,#118808,#118809,#118810,#118811,#118812,#118813,
#118814,#118815,#118816,#118817,#118818,#118819,#118820,#118821,#118822,
#118823,#118824,#118825,#118826,#118827,#118828,#118829,#118830,#118831,
#118832,#118833,#118834,#118835),.UNSPECIFIED.,.T.,.F.,(4,2,2,2,2,2,2,2,
2,2,2,2,2,2,2,2,2,2,2,2,2,2,2,2,2,2,4),(0.,0.0478739945692769,0.0986971471010809,
0.148337519565137,0.189656688812435,0.228043708382913,0.239165467815064,
0.245690284550349,0.251233949360227,0.25795220129384,0.270230302745385,
0.321321411721412,0.362050378315662,0.406602849867675,0.454509035792872,
0.505306311247286,0.554814869634011,0.597172283297015,0.631280129484872,
0.641914542897276,0.648218164531197,0.653710112834502,0.660536832617733,
0.673512930764169,0.724577243318909,0.765567731891649,0.804148773373606),
 .UNSPECIFIED.);
#2726=B_SPLINE_CURVE_WITH_KNOTS('',3,(#118838,#118839,#118840,#118841,#118842,
#118843,#118844,#118845,#118846,#118847,#118848,#118849,#118850,#118851,
#118852,#118853,#118854,#118855,#118856,#118857,#118858,#118859,#118860,
#118861,#118862,#118863,#118864,#118865,#118866,#118867,#118868,#118869,
#118870,#118871),.UNSPECIFIED.,.T.,.F.,(4,2,2,2,2,2,2,2,2,2,2,2,2,2,2,2,
4),(0.,0.0507036982380927,0.101367967769165,0.15217435009708,0.202988254858527,
0.253660615022253,0.304349675621658,0.355417624755026,0.406309245550189,
0.456681959570615,0.506950514497502,0.557047627860013,0.607008171588907,
0.65696367342519,0.707040719162867,0.757254767928788,0.80482271556345),
 .UNSPECIFIED.);
#2727=B_SPLINE_CURVE_WITH_KNOTS('',3,(#118875,#118876,#118877,#118878,#118879,
#118880,#118881,#118882,#118883,#118884,#118885,#118886,#118887,#118888,
#118889,#118890,#118891,#118892,#118893,#118894,#118895,#118896,#118897),
 .UNSPECIFIED.,.F.,.F.,(4,2,2,2,2,2,2,2,2,3,4),(0.213107054482159,0.226203862898588,
0.253173118245501,0.28015352143344,0.307156285370326,0.334139138956564,
0.361106824850293,0.38814457612529,0.415330879616146,0.42617130555841,0.426197129198138),
 .UNSPECIFIED.);
#2728=B_SPLINE_CURVE_WITH_KNOTS('',3,(#118901,#118902,#118903,#118904,#118905,
#118906,#118907,#118908,#118909,#118910,#118911,#118912,#118913,#118914,
#118915,#118916,#118917,#118918,#118919,#118920),.UNSPECIFIED.,.F.,.F.,
(4,2,2,2,2,2,2,2,2,4),(0.426197129198138,0.452822943590338,0.479420811937044,
0.505945019640447,0.532418265293895,0.558897919334064,0.58543642024838,
0.612041061741514,0.625328210873673,0.639278360040569),.UNSPECIFIED.);
#2729=B_SPLINE_CURVE_WITH_KNOTS('',3,(#118923,#118924,#118925,#118926,#118927,
#118928,#118929,#118930,#118931,#118932,#118933,#118934,#118935,#118936,
#118937,#118938,#118939,#118940,#118941,#118942,#118943,#118944,#118945,
#118946,#118947,#118948,#118949,#118950,#118951,#118952,#118953,#118954,
#118955,#118956,#118957,#118958,#118959,#118960,#118961,#118962,#118963,
#118964,#118965,#118966,#118967,#118968,#118969,#118970,#118971,#118972,
#118973,#118974,#118975,#118976,#118977,#118978),.UNSPECIFIED.,.T.,.F.,
(4,2,2,2,2,2,2,2,2,2,2,2,2,2,2,2,2,2,2,2,2,2,2,2,2,2,2,4),(0.,0.0423917071008588,
0.0862690124816813,0.128223494874909,0.166386336836243,0.188172470137429,
0.195965603192946,0.200910173484711,0.205484821318604,0.211457224587722,
0.223972369869265,0.267764198510775,0.303174271614316,0.341946448532938,
0.383731798431802,0.42769896692924,0.470189492903271,0.506972629115825,
0.533779293250024,0.542258367054284,0.547330630539367,0.55137511128395,
0.556768979326987,0.566677076478627,0.610454812685682,0.645453523164812,
0.670975464062507,0.69390114019026),.UNSPECIFIED.);
#2730=B_SPLINE_CURVE_WITH_KNOTS('',3,(#118981,#118982,#118983,#118984,#118985,
#118986,#118987,#118988,#118989,#118990,#118991,#118992,#118993,#118994,
#118995,#118996,#118997,#118998,#118999,#119000,#119001,#119002,#119003,
#119004,#119005,#119006,#119007,#119008,#119009,#119010,#119011,#119012,
#119013,#119014,#119015,#119016,#119017,#119018),.UNSPECIFIED.,.T.,.F.,
(4,2,2,2,2,2,2,2,2,2,2,2,2,2,2,2,2,2,4),(0.,0.0439285969839785,0.0877338055835913,
0.131600288228661,0.174581723094377,0.218417405783077,0.262237812383161,
0.306273059701853,0.327893564393435,0.371979478856129,0.415515580695926,
0.458786565242884,0.501799585059231,0.544720010296071,0.587775168317762,
0.631102572848802,0.652852121001093,0.673538591001646,0.694388197397481),
 .UNSPECIFIED.);
#2731=B_SPLINE_CURVE_WITH_KNOTS('',3,(#119022,#119023,#119024,#119025,#119026,
#119027,#119028,#119029,#119030,#119031,#119032,#119033,#119034,#119035,
#119036,#119037,#119038,#119039,#119040,#119041,#119042,#119043,#119044,
#119045,#119046),.UNSPECIFIED.,.F.,.F.,(4,2,2,2,2,2,2,2,2,2,3,4),(0.157664314186863,
0.167520999539812,0.187522964929857,0.207504733138004,0.227022893262324,
0.246540738053684,0.266134356212337,0.286153085842429,0.295957890558149,
0.30554520497725,0.315225351986019,0.315251153228398),.UNSPECIFIED.);
#2732=B_SPLINE_CURVE_WITH_KNOTS('',3,(#119050,#119051,#119052,#119053,#119054,
#119055,#119056,#119057,#119058,#119059,#119060,#119061,#119062,#119063,
#119064,#119065,#119066,#119067,#119068,#119069),.UNSPECIFIED.,.F.,.F.,
(4,2,2,2,2,2,2,2,2,4),(0.315251153228398,0.335201080329252,0.354894727899546,
0.374468684471932,0.393968635000947,0.413485447868118,0.433100328931788,
0.452833383067246,0.462678741523263,0.472889666172882),.UNSPECIFIED.);
#2733=B_SPLINE_CURVE_WITH_KNOTS('',3,(#119072,#119073,#119074,#119075,#119076,
#119077,#119078,#119079,#119080,#119081,#119082,#119083,#119084,#119085,
#119086,#119087,#119088,#119089,#119090,#119091,#119092,#119093,#119094,
#119095,#119096,#119097,#119098,#119099,#119100,#119101,#119102,#119103,
#119104,#119105,#119106,#119107,#119108,#119109,#119110,#119111,#119112,
#119113,#119114,#119115,#119116,#119117,#119118,#119119,#119120,#119121,
#119122,#119123,#119124,#119125,#119126,#119127),.UNSPECIFIED.,.T.,.F.,
(4,2,2,2,2,2,2,2,2,2,2,2,2,2,2,2,2,2,2,2,2,2,2,2,2,2,2,4),(0.,0.0433357033279547,
0.0867918942096803,0.12674974376004,0.169317740075874,0.179091766390012,
0.184344749294548,0.188727191507819,0.193208494521891,0.199695700510524,
0.216202111608105,0.259547133084174,0.295329969828243,0.334483203156315,
0.376753899026277,0.420528758464677,0.462143525407209,0.500104687054551,
0.520667413014844,0.527991625556146,0.532631100199553,0.536919456730402,
0.542513918627149,0.554231014573357,0.597650721490353,0.632731625953485,
0.662884793490238,0.690031112817339),.UNSPECIFIED.);
#2734=B_SPLINE_CURVE_WITH_KNOTS('',3,(#119130,#119131,#119132,#119133,#119134,
#119135,#119136,#119137,#119138,#119139,#119140,#119141,#119142,#119143,
#119144,#119145,#119146,#119147,#119148,#119149,#119150,#119151,#119152,
#119153,#119154,#119155,#119156,#119157,#119158,#119159,#119160,#119161,
#119162,#119163,#119164,#119165,#119166,#119167),.UNSPECIFIED.,.T.,.F.,
(4,2,2,2,2,2,2,2,2,2,2,2,2,2,2,2,2,2,4),(0.,0.0437846598539115,0.0873818383118426,
0.130569174600926,0.173091910935896,0.215698254859366,0.25928498636956,
0.303005395562776,0.324461683296978,0.345997226871332,0.390332486539213,
0.433644313592107,0.476506969627738,0.519027119267212,0.561518089693932,
0.604312670966229,0.647555474893121,0.668924190877181,0.690483896486725),
 .UNSPECIFIED.);
#2735=B_SPLINE_CURVE_WITH_KNOTS('',3,(#119171,#119172,#119173,#119174,#119175,
#119176,#119177,#119178,#119179,#119180,#119181,#119182,#119183,#119184,
#119185,#119186,#119187,#119188,#119189,#119190,#119191,#119192,#119193),
 .UNSPECIFIED.,.F.,.F.,(4,2,2,2,2,2,2,2,2,3,4),(0.155323839065176,0.174895282975292,
0.194601807476139,0.214028772431744,0.233156373086578,0.252306343141429,
0.271599920800694,0.291343602566944,0.300917682052659,0.310590124203141,
0.310614889159676),.UNSPECIFIED.);
#2736=B_SPLINE_CURVE_WITH_KNOTS('',3,(#119197,#119198,#119199,#119200,#119201,
#119202,#119203,#119204,#119205,#119206,#119207,#119208,#119209,#119210,
#119211,#119212,#119213,#119214,#119215,#119216,#119217,#119218),
 .UNSPECIFIED.,.F.,.F.,(4,2,2,2,2,2,2,2,2,2,4),(0.310614889159676,0.330461615882692,
0.350073356350718,0.369341148381857,0.38846889618466,0.407595133318853,
0.426859384772424,0.446319865203601,0.45603054018867,0.465724013336885,
0.465913963268316),.UNSPECIFIED.);
#2737=B_SPLINE_CURVE_WITH_KNOTS('',3,(#119222,#119223,#119224,#119225,#119226,
#119227,#119228,#119229,#119230,#119231,#119232,#119233,#119234,#119235,
#119236,#119237,#119238,#119239,#119240,#119241,#119242,#119243,#119244,
#119245,#119246,#119247,#119248,#119249,#119250,#119251),.UNSPECIFIED.,
 .F.,.F.,(4,2,2,2,2,2,2,2,2,2,2,2,2,2,4),(1.00000010940975E-6,0.0384609387804645,
0.0726049480932644,0.12998621409426,0.183385238805886,0.232646795046144,
0.285302749131523,0.314403553947751,0.326074174045375,0.333858467758951,
0.341326316436165,0.351457949388285,0.37402026617642,0.433053304401173,
0.465421514323042),.UNSPECIFIED.);
#2738=B_SPLINE_CURVE_WITH_KNOTS('',3,(#119255,#119256,#119257,#119258,#119259,
#119260,#119261,#119262,#119263,#119264,#119265,#119266,#119267,#119268,
#119269,#119270,#119271,#119272,#119273,#119274,#119275,#119276,#119277,
#119278,#119279,#119280,#119281,#119282,#119283,#119284,#119285,#119286,
#119287,#119288,#119289,#119290,#119291,#119292,#119293,#119294,#119295,
#119296,#119297,#119298,#119299,#119300,#119301,#119302,#119303,#119304,
#119305,#119306,#119307,#119308,#119309,#119310,#119311,#119312,#119313,
#119314,#119315,#119316,#119317,#119318,#119319,#119320,#119321,#119322,
#119323,#119324,#119325,#119326,#119327,#119328,#119329,#119330,#119331,
#119332,#119333,#119334,#119335,#119336,#119337,#119338,#119339,#119340,
#119341,#119342,#119343,#119344,#119345,#119346,#119347,#119348,#119349,
#119350,#119351,#119352,#119353,#119354,#119355,#119356,#119357,#119358,
#119359,#119360,#119361,#119362,#119363,#119364,#119365,#119366,#119367,
#119368,#119369,#119370,#119371,#119372,#119373,#119374,#119375,#119376,
#119377,#119378),.UNSPECIFIED.,.F.,.F.,(4,3,3,3,3,3,3,3,3,3,3,3,3,3,3,3,
3,3,3,3,3,3,3,3,3,3,3,3,3,3,3,3,3,3,3,3,3,3,3,3,3,4),(0.,0.00013276129913434,
0.000266835524831858,0.000288910361442746,0.00040545879614334,0.000521895356260907,
0.000577820722885491,0.00071247778923503,0.000847454257176977,0.000866731084328237,
0.000975087715605292,0.00108347076913653,0.00115564144577098,0.00130428008995543,
0.00145283323966009,0.00160149883572666,0.00173346216865647,0.00188146410637275,
0.00202935838489384,0.00217733269970768,0.00231128289154197,0.00242032515157694,
0.00252931477079484,0.00260019325298471,0.00273515651973894,0.00286996752096618,
0.00288910361442745,0.0030033190459749,0.00311763416070541,0.00317801397587019,
0.00331228109060909,0.00344538869240954,0.00346692433731293,0.00367323273482719,
0.00388991397652125,0.00404474506019841,0.00417932605144588,0.00431432738910213,
0.00433365542164112,0.00444162789512621,0.0045496106988975,0.00462256578308383),
 .UNSPECIFIED.);
#2739=B_SPLINE_CURVE_WITH_KNOTS('',3,(#119379,#119380,#119381,#119382,#119383,
#119384,#119385,#119386,#119387,#119388,#119389,#119390,#119391,#119392,
#119393,#119394,#119395,#119396,#119397,#119398),.UNSPECIFIED.,.F.,.F.,
(4,2,2,2,2,2,2,2,2,4),(1.00000016868767E-6,0.0585541366944336,0.116515904932218,
0.174631749418359,0.232879705095392,0.290789101013029,0.348769985500845,
0.377759774398062,0.42345230050058,0.465809052198513),.UNSPECIFIED.);
#2740=B_SPLINE_CURVE_WITH_KNOTS('',3,(#119399,#119400,#119401,#119402,#119403,
#119404,#119405,#119406,#119407,#119408,#119409,#119410,#119411,#119412,
#119413,#119414,#119415,#119416,#119417,#119418,#119419,#119420,#119421,
#119422,#119423,#119424,#119425,#119426,#119427,#119428,#119429,#119430,
#119431,#119432,#119433,#119434,#119435,#119436,#119437,#119438,#119439,
#119440,#119441,#119442,#119443,#119444,#119445,#119446,#119447,#119448,
#119449,#119450,#119451,#119452,#119453,#119454,#119455,#119456,#119457,
#119458,#119459,#119460,#119461,#119462,#119463,#119464,#119465,#119466,
#119467,#119468,#119469,#119470,#119471,#119472,#119473,#119474,#119475,
#119476,#119477,#119478,#119479,#119480,#119481,#119482,#119483,#119484,
#119485,#119486,#119487,#119488,#119489,#119490,#119491,#119492,#119493,
#119494,#119495,#119496,#119497,#119498,#119499,#119500,#119501,#119502,
#119503,#119504,#119505,#119506,#119507,#119508,#119509,#119510,#119511,
#119512,#119513,#119514,#119515,#119516,#119517,#119518,#119519,#119520,
#119521,#119522),.UNSPECIFIED.,.F.,.F.,(4,3,3,3,3,3,3,3,3,3,3,3,3,3,3,3,
3,3,3,3,3,3,3,3,3,3,3,3,3,3,3,3,3,3,3,3,3,3,3,3,3,4),(0.,0.000132745935003127,
0.000266814935045813,0.000288919615584892,0.000405543240980673,0.00052205660558132,
0.000577839231169785,0.000712522167078833,0.000847534928045407,0.000866758846754677,
0.00097514847331441,0.00108356503212164,0.00115567846233957,0.00130446679715503,
0.00145316983239142,0.00160198502321772,0.00173351769350932,0.00188149019865714,
0.00202935391483387,0.0021772961594043,0.00231135692467908,0.00242052512897724,
0.00252963569872571,0.00260027654026395,0.00273521641874506,0.00287000951803308,
0.00288919615584882,0.00300295417106767,0.00311680707883515,0.00317811577143369,
0.00331235835362441,0.00344545082104483,0.00346703538701856,0.003675605881335,
0.0038952874317491,0.0040448746181883,0.00417940787509396,0.00431437880260212,
0.00433379423377317,0.0044417693386194,0.00454975693031286,0.00462271384935804),
 .UNSPECIFIED.);
#2741=B_SPLINE_CURVE_WITH_KNOTS('',3,(#119526,#119527,#119528,#119529,#119530,
#119531,#119532,#119533,#119534,#119535,#119536,#119537,#119538,#119539,
#119540,#119541,#119542,#119543,#119544,#119545,#119546,#119547),
 .UNSPECIFIED.,.F.,.F.,(4,2,2,2,2,2,2,2,2,2,4),(0.139827597716775,0.156235126594654,
0.191204336808387,0.226231673968276,0.261235307761556,0.296182933144171,
0.33120275340376,0.34837260812873,0.365776511367808,0.400348110030799,0.41660864742562),
 .UNSPECIFIED.);
#2742=B_SPLINE_CURVE_WITH_KNOTS('',3,(#119551,#119552,#119553,#119554,#119555,
#119556,#119557,#119558,#119559,#119560,#119561,#119562,#119563,#119564,
#119565,#119566,#119567,#119568,#119569,#119570,#119571,#119572,#119573),
 .UNSPECIFIED.,.F.,.F.,(4,2,2,2,2,3,2,2,2,2,4),(0.41660864742562,0.434934002630221,
0.469503712280229,0.504019646860705,0.538477704551985,0.553565728510636,
0.588009075052285,0.622483929180438,0.639712551567059,0.67484049808458,
0.69339332622741),.UNSPECIFIED.);
#2743=B_SPLINE_CURVE_WITH_KNOTS('',3,(#119576,#119577,#119578,#119579,#119580,
#119581,#119582,#119583,#119584,#119585,#119586,#119587,#119588,#119589,
#119590,#119591,#119592,#119593,#119594,#119595,#119596,#119597,#119598,
#119599,#119600,#119601,#119602,#119603,#119604,#119605,#119606,#119607,
#119608,#119609,#119610,#119611,#119612,#119613,#119614,#119615,#119616,
#119617,#119618,#119619,#119620,#119621,#119622,#119623,#119624,#119625,
#119626,#119627,#119628,#119629),.UNSPECIFIED.,.T.,.F.,(4,2,2,2,2,2,2,2,
2,2,2,2,2,2,2,2,2,2,2,2,2,2,2,2,2,2,4),(0.,0.0458320233936563,0.0951449281800662,
0.145722741215669,0.193905817750798,0.24098068927026,0.260497956547193,
0.269118961822078,0.275165580221845,0.281315954994347,0.290145956654934,
0.312104595695031,0.36312921663319,0.405435175946239,0.451284673710212,
0.500506710518771,0.551059662709869,0.599064670783345,0.647472573581018,
0.664439886250511,0.672224627284561,0.67815077226323,0.684415281967539,
0.693989332263362,0.721065537010137,0.757868161553381,0.80414884601772),
 .UNSPECIFIED.);
#2744=B_SPLINE_CURVE_WITH_KNOTS('',3,(#119632,#119633,#119634,#119635,#119636,
#119637,#119638,#119639,#119640,#119641,#119642,#119643,#119644,#119645,
#119646,#119647,#119648,#119649,#119650,#119651,#119652,#119653,#119654,
#119655,#119656,#119657,#119658,#119659,#119660,#119661,#119662,#119663,
#119664,#119665,#119666,#119667),.UNSPECIFIED.,.T.,.F.,(4,2,2,2,2,2,2,2,
2,2,2,2,2,2,2,2,2,4),(0.,0.0506382155192934,0.101412301739861,0.152300545666833,
0.203076346321417,0.253714832497476,0.304525318114152,0.329477947350912,
0.380367701352928,0.430730790890535,0.480986961082011,0.531075489416336,
0.581036229250358,0.631000474534633,0.681089122694047,0.731309856554222,
0.782321329423195,0.804714418336591),.UNSPECIFIED.);
#2745=B_SPLINE_CURVE_WITH_KNOTS('',3,(#119671,#119672,#119673,#119674,#119675,
#119676,#119677,#119678,#119679,#119680,#119681,#119682,#119683,#119684,
#119685,#119686,#119687,#119688,#119689,#119690),.UNSPECIFIED.,.F.,.F.,
(4,2,2,2,2,2,2,2,2,4),(0.213039430164029,0.239784499091426,0.266784297866583,
0.29381362797788,0.320813732727093,0.347781018775311,0.374802890367102,
0.388043853196362,0.414989929726265,0.426095694247663),.UNSPECIFIED.);
#2746=B_SPLINE_CURVE_WITH_KNOTS('',3,(#119694,#119695,#119696,#119697,#119698,
#119699,#119700,#119701,#119702,#119703,#119704,#119705,#119706,#119707,
#119708,#119709,#119710,#119711,#119712,#119713,#119714,#119715,#119716,
#119717,#119718),.UNSPECIFIED.,.F.,.F.,(4,3,2,2,2,2,2,2,2,2,2,4),(0.426095694247663,
0.426100860962362,0.452722929227169,0.479276968030936,0.505766829860246,
0.532237790565919,0.55874892707621,0.585329286001983,0.59862501203735,0.611895650008454,
0.638918112912157,0.639140291126391),.UNSPECIFIED.);
#2747=B_SPLINE_CURVE_WITH_KNOTS('',3,(#119721,#119722,#119723,#119724,#119725,
#119726,#119727,#119728,#119729,#119730,#119731,#119732,#119733,#119734,
#119735,#119736,#119737,#119738,#119739,#119740,#119741,#119742,#119743,
#119744,#119745,#119746,#119747,#119748,#119749,#119750,#119751,#119752,
#119753,#119754,#119755,#119756,#119757,#119758,#119759,#119760,#119761,
#119762,#119763,#119764,#119765,#119766,#119767,#119768,#119769,#119770,
#119771,#119772,#119773,#119774,#119775,#119776),.UNSPECIFIED.,.T.,.F.,
(4,2,2,2,2,2,2,2,2,2,2,2,2,2,2,2,2,2,2,2,2,2,2,2,2,2,2,4),(0.,0.0405914926291309,
0.0843626355691103,0.127768982513206,0.167065813577391,0.206671614216115,
0.215953475712915,0.221920923639481,0.226643225345449,0.231901123126324,
0.240523135098381,0.269456491599303,0.302072522394008,0.338668936139127,
0.378440679256369,0.421240646865564,0.46495856166125,0.50610024767708,0.547698204088174,
0.561705855753858,0.567441009098402,0.572217070056482,0.577088327121725,
0.584110325732133,0.60175959891513,0.645470033107342,0.671747046627922,
0.693886489051851),.UNSPECIFIED.);
#2748=B_SPLINE_CURVE_WITH_KNOTS('',3,(#119779,#119780,#119781,#119782,#119783,
#119784,#119785,#119786,#119787,#119788,#119789,#119790,#119791,#119792,
#119793,#119794,#119795,#119796,#119797,#119798,#119799,#119800,#119801,
#119802,#119803,#119804,#119805,#119806,#119807,#119808,#119809,#119810,
#119811,#119812,#119813,#119814,#119815,#119816),.UNSPECIFIED.,.T.,.F.,
(4,2,2,2,2,2,2,2,2,2,2,2,2,2,2,2,2,2,4),(0.,0.0438175087151928,0.0876691144818819,
0.131147129449532,0.174176486018958,0.217992008349161,0.261863242175615,
0.283379432303044,0.304976216118143,0.349059089995391,0.392583706563762,
0.435842850089949,0.478849630518895,0.52177211286288,0.564835596442599,
0.608171918261097,0.629922691866238,0.651607491185624,0.694352304660229),
 .UNSPECIFIED.);
#2749=B_SPLINE_CURVE_WITH_KNOTS('',3,(#119820,#119821,#119822,#119823,#119824,
#119825,#119826,#119827,#119828,#119829,#119830,#119831,#119832,#119833,
#119834,#119835,#119836,#119837,#119838,#119839),.UNSPECIFIED.,.F.,.F.,
(4,2,2,2,2,2,2,2,2,4),(0.157606167153757,0.177533160499949,0.197526249232083,
0.21704082507597,0.236560887844295,0.256160878575661,0.27616865652419,0.285965370433475,
0.29577830412786,0.315209094655922),.UNSPECIFIED.);
#2750=B_SPLINE_CURVE_WITH_KNOTS('',3,(#119843,#119844,#119845,#119846,#119847,
#119848,#119849,#119850,#119851,#119852,#119853,#119854,#119855,#119856,
#119857,#119858,#119859,#119860,#119861,#119862,#119863,#119864,#119865,
#119866,#119867),.UNSPECIFIED.,.F.,.F.,(4,3,2,2,2,2,2,2,2,2,2,4),(0.315209094655922,
0.315212335396961,0.335131144657127,0.354754972246871,0.374277570779983,
0.39377515829634,0.413340082716485,0.433023708581587,0.442873251294654,
0.452706286471694,0.472750995875536,0.472818502550718),.UNSPECIFIED.);
#2751=B_SPLINE_CURVE_WITH_KNOTS('',3,(#119870,#119871,#119872,#119873,#119874,
#119875,#119876,#119877,#119878,#119879,#119880,#119881,#119882,#119883,
#119884,#119885,#119886,#119887,#119888,#119889,#119890,#119891,#119892,
#119893,#119894,#119895,#119896,#119897,#119898,#119899,#119900,#119901,
#119902,#119903,#119904,#119905,#119906,#119907,#119908,#119909,#119910,
#119911,#119912,#119913,#119914,#119915,#119916,#119917,#119918,#119919,
#119920,#119921,#119922,#119923,#119924,#119925),.UNSPECIFIED.,.T.,.F.,
(4,2,2,2,2,2,2,2,2,2,2,2,2,2,2,2,2,2,2,2,2,2,2,2,2,2,2,4),(0.,0.0414795115022862,
0.0854646868492746,0.128051759118891,0.164665226970607,0.195716497055745,
0.204517379482455,0.209651426874716,0.213999683797992,0.219256285248534,
0.228840648703378,0.272097887192487,0.306671347087566,0.344807987469752,
0.386083672854091,0.430070266056682,0.472738795403928,0.507152959663538,
0.540328694973379,0.549340374995075,0.554498373378035,0.558414709258595,
0.563406376511839,0.571927658782594,0.603840451269834,0.636687933284218,
0.665364108131361,0.689885376340169),.UNSPECIFIED.);
#2752=B_SPLINE_CURVE_WITH_KNOTS('',3,(#119928,#119929,#119930,#119931,#119932,
#119933,#119934,#119935,#119936,#119937,#119938,#119939,#119940,#119941,
#119942,#119943,#119944,#119945,#119946,#119947,#119948,#119949,#119950,
#119951,#119952,#119953,#119954,#119955,#119956,#119957,#119958,#119959,
#119960,#119961,#119962,#119963),.UNSPECIFIED.,.T.,.F.,(4,2,2,2,2,2,2,2,
2,2,2,2,2,2,2,2,2,4),(0.,0.0437203941025976,0.0872619187212367,0.130314443853127,
0.172840099632362,0.216371752952188,0.260051472953626,0.304070571832068,
0.348437356049367,0.39193122891185,0.435014940311694,0.477666783665775,
0.520120318579686,0.562730177846754,0.605754886603923,0.649188896287545,
0.669804552140718,0.690576832826956),.UNSPECIFIED.);
#2753=B_SPLINE_CURVE_WITH_KNOTS('',3,(#119967,#119968,#119969,#119970,#119971,
#119972,#119973,#119974,#119975,#119976,#119977,#119978,#119979,#119980,
#119981,#119982,#119983,#119984,#119985,#119986),.UNSPECIFIED.,.F.,.F.,
(4,2,2,2,2,2,2,2,2,4),(0.155313790581586,0.165349433967049,0.185058166819829,
0.204477450512361,0.223605464026358,0.242753401686118,0.262450452504133,
0.282242587220628,0.302131095225523,0.310630462500323),.UNSPECIFIED.);
#2754=B_SPLINE_CURVE_WITH_KNOTS('',3,(#119990,#119991,#119992,#119993,#119994,
#119995,#119996,#119997,#119998,#119999,#120000,#120001,#120002,#120003,
#120004,#120005,#120006,#120007,#120008,#120009,#120010,#120011,#120012),
 .UNSPECIFIED.,.F.,.F.,(4,3,2,2,2,2,2,2,2,2,4),(0.310630462500323,0.310634616707648,
0.330337216979212,0.349710864965688,0.368898762124798,0.388004166232081,
0.407178443301545,0.426532516796507,0.446452164049864,0.4561765436671,0.465948407289234),
 .UNSPECIFIED.);
#2755=B_SPLINE_CURVE_WITH_KNOTS('',3,(#120015,#120016,#120017,#120018,#120019,
#120020,#120021,#120022,#120023,#120024,#120025,#120026,#120027,#120028,
#120029,#120030,#120031,#120032,#120033,#120034,#120035,#120036,#120037,
#120038,#120039,#120040,#120041,#120042,#120043,#120044,#120045,#120046,
#120047,#120048,#120049,#120050,#120051,#120052,#120053,#120054,#120055,
#120056,#120057,#120058,#120059,#120060,#120061,#120062,#120063,#120064,
#120065,#120066,#120067,#120068),.UNSPECIFIED.,.T.,.F.,(4,2,2,2,2,2,2,2,
2,2,2,2,2,2,2,2,2,2,2,2,2,2,2,2,2,2,4),(0.,0.0540423596745269,0.106458768986388,
0.122382214139942,0.131786992503092,0.139792246283686,0.149487906352155,
0.167103867927491,0.226190960021578,0.274156863496862,0.326257305107725,
0.382114137371328,0.440761445270956,0.497701345644869,0.55092190315513,
0.580002255699023,0.59223296424121,0.599783921991879,0.607895871128139,
0.6187122561808,0.641990799106262,0.70098574657611,0.750074000444414,0.803304704986148,
0.860492178265741,0.893904470056555,0.931148964406098),.UNSPECIFIED.);
#2756=B_SPLINE_CURVE_WITH_KNOTS('',3,(#120071,#120072,#120073,#120074,#120075,
#120076,#120077,#120078,#120079,#120080,#120081,#120082,#120083,#120084,
#120085,#120086,#120087,#120088,#120089,#120090,#120091,#120092,#120093,
#120094,#120095,#120096,#120097,#120098,#120099,#120100,#120101,#120102,
#120103,#120104,#120105,#120106,#120107,#120108),.UNSPECIFIED.,.T.,.F.,
(4,2,2,2,2,2,2,2,2,2,2,2,2,2,2,2,2,2,4),(0.,0.0586300084882738,0.117483040973624,
0.17622629878783,0.234715123518207,0.293318069965833,0.322102318538047,
0.351386546001824,0.409612976636273,0.467874879536276,0.526102208109452,
0.584201159872194,0.642161284355705,0.700072909012953,0.758033873788971,
0.787020936942943,0.816011821099062,0.874804862256184,0.931703358703855),
 .UNSPECIFIED.);
#2757=B_SPLINE_CURVE_WITH_KNOTS('',3,(#120112,#120113,#120114,#120115,#120116,
#120117,#120118,#120119,#120120,#120121,#120122,#120123,#120124,#120125,
#120126,#120127,#120128,#120129,#120130,#120131),.UNSPECIFIED.,.F.,.F.,
(4,2,2,2,2,2,2,2,2,4),(0.139767201099283,0.173948087346139,0.209027502769792,
0.244070694700763,0.279025309570312,0.31402030403869,0.331173399059848,
0.348578268416969,0.38314632638829,0.416559483837296),.UNSPECIFIED.);
#2758=B_SPLINE_CURVE_WITH_KNOTS('',3,(#120135,#120136,#120137,#120138,#120139,
#120140,#120141,#120142,#120143,#120144,#120145,#120146,#120147,#120148,
#120149,#120150,#120151,#120152,#120153,#120154,#120155,#120156,#120157,
#120158,#120159),.UNSPECIFIED.,.F.,.F.,(4,2,2,2,2,3,2,2,2,2,2,4),(0.416559483837296,
0.417723433981753,0.452283374405963,0.486794062508417,0.521254824770743,
0.553553763071154,0.588021449246394,0.605248660316662,0.622478045168663,
0.657553404742335,0.692501114966837,0.693320964170437),.UNSPECIFIED.);
#2759=B_SPLINE_CURVE_WITH_KNOTS('',3,(#120162,#120163,#120164,#120165,#120166,
#120167,#120168,#120169,#120170,#120171,#120172,#120173,#120174,#120175,
#120176,#120177,#120178,#120179,#120180,#120181,#120182,#120183,#120184,
#120185,#120186,#120187,#120188,#120189,#120190,#120191,#120192,#120193,
#120194,#120195,#120196,#120197,#120198,#120199,#120200,#120201,#120202,
#120203,#120204,#120205,#120206,#120207,#120208,#120209,#120210,#120211,
#120212,#120213,#120214,#120215),.UNSPECIFIED.,.T.,.F.,(4,2,2,2,2,2,2,2,
2,2,2,2,2,2,2,2,2,2,2,2,2,2,2,2,2,2,4),(0.,0.0436206699491311,0.090749901183791,
0.14148754427114,0.191583934327092,0.236779691637168,0.279072297635201,
0.291623391075206,0.299010732283145,0.305292026455287,0.312900344618033,
0.326758378813266,0.377634492790539,0.418722650965157,0.463540596216931,
0.511693288303611,0.562458476750911,0.611785021190842,0.655989914646358,
0.685075451837005,0.695760239918773,0.702595078313781,0.70894334751278,
0.717248646167864,0.734614913634257,0.7570782451133,0.804102668187989),
 .UNSPECIFIED.);
#2760=B_SPLINE_CURVE_WITH_KNOTS('',3,(#120218,#120219,#120220,#120221,#120222,
#120223,#120224,#120225,#120226,#120227,#120228,#120229,#120230,#120231,
#120232,#120233,#120234,#120235,#120236,#120237,#120238,#120239,#120240,
#120241,#120242,#120243,#120244,#120245,#120246,#120247,#120248,#120249,
#120250,#120251,#120252,#120253),.UNSPECIFIED.,.T.,.F.,(4,2,2,2,2,2,2,2,
2,2,2,2,2,2,2,2,2,4),(0.,0.0507228794267668,0.10166597248895,0.1526015226544,
0.20331343587648,0.253951968982878,0.27876966200945,0.303684210636509,0.354570883308706,
0.404917178454264,0.455153400555304,0.505229442536965,0.555191945447311,
0.605170640049558,0.655277164146098,0.705507445865675,0.756424092950211,
0.804681319466827),.UNSPECIFIED.);
#2761=B_SPLINE_CURVE_WITH_KNOTS('',3,(#120257,#120258,#120259,#120260,#120261,
#120262,#120263,#120264,#120265,#120266,#120267,#120268,#120269,#120270,
#120271,#120272,#120273,#120274,#120275,#120276,#120277,#120278),
 .UNSPECIFIED.,.F.,.F.,(4,2,2,2,2,2,2,2,2,2,4),(0.213065565020054,0.2132216265088,
0.240218856302912,0.267018454471732,0.293523298289317,0.320516778459753,
0.34747669940655,0.360670422284557,0.373888860401591,0.401079646648718,
0.426100077448779),.UNSPECIFIED.);
#2762=B_SPLINE_CURVE_WITH_KNOTS('',3,(#120282,#120283,#120284,#120285,#120286,
#120287,#120288,#120289,#120290,#120291,#120292,#120293,#120294,#120295,
#120296,#120297,#120298,#120299,#120300,#120301,#120302),.UNSPECIFIED.,
 .F.,.F.,(4,3,2,2,2,2,2,2,2,4),(0.426100077448779,0.426138379615387,0.452716978378953,
0.479228067467344,0.505701620846424,0.532194452261604,0.558750452815834,
0.585365281292561,0.612400917766107,0.639203944635441),.UNSPECIFIED.);
#2763=B_SPLINE_CURVE_WITH_KNOTS('',3,(#120305,#120306,#120307,#120308,#120309,
#120310,#120311,#120312,#120313,#120314,#120315,#120316,#120317,#120318,
#120319,#120320,#120321,#120322,#120323,#120324,#120325,#120326,#120327,
#120328,#120329,#120330,#120331,#120332,#120333,#120334,#120335,#120336,
#120337,#120338,#120339,#120340,#120341,#120342,#120343,#120344,#120345,
#120346,#120347,#120348,#120349,#120350,#120351,#120352,#120353,#120354,
#120355,#120356,#120357,#120358,#120359,#120360),.UNSPECIFIED.,.T.,.F.,
(4,2,2,2,2,2,2,2,2,2,2,2,2,2,2,2,2,2,2,2,2,2,2,2,2,2,2,4),(0.,0.0387113895615106,
0.0805130667469615,0.124505950972711,0.167101755822628,0.204029948058607,
0.231860291834698,0.241054636366574,0.246653577504196,0.251673760202214,
0.25800253399371,0.270483479280963,0.314220613655029,0.349681497508595,
0.388480986665803,0.430284691736075,0.474246193962455,0.516732436076201,
0.554321371029958,0.579627049069653,0.588407223118832,0.593879907222584,
0.598870503701298,0.605276403150402,0.618284530922307,0.634910354183487,
0.666887166430965,0.693797831079255),.UNSPECIFIED.);
#2764=B_SPLINE_CURVE_WITH_KNOTS('',3,(#120363,#120364,#120365,#120366,#120367,
#120368,#120369,#120370,#120371,#120372,#120373,#120374,#120375,#120376,
#120377,#120378,#120379,#120380,#120381,#120382,#120383,#120384,#120385,
#120386,#120387,#120388,#120389,#120390,#120391,#120392,#120393,#120394,
#120395,#120396,#120397,#120398,#120399,#120400),.UNSPECIFIED.,.T.,.F.,
(4,2,2,2,2,2,2,2,2,2,2,2,2,2,2,2,2,2,4),(0.,0.0437823947455483,0.0875527147869647,
0.131334832842352,0.175097356688018,0.218947594184666,0.263105738677232,
0.284797487459486,0.32887262269309,0.37240987695627,0.415675530898497,0.458678387410487,
0.501589552021586,0.544639998300872,0.587966065552883,0.609716214397085,
0.631470618066917,0.675605980504124,0.694348679609398),.UNSPECIFIED.);
#2765=B_SPLINE_CURVE_WITH_KNOTS('',3,(#120404,#120405,#120406,#120407,#120408,
#120409,#120410,#120411,#120412,#120413,#120414,#120415,#120416,#120417,
#120418,#120419,#120420,#120421,#120422,#120423,#120424,#120425,#120426,
#120427,#120428),.UNSPECIFIED.,.F.,.F.,(4,2,2,2,2,2,2,2,2,2,3,4),(0.157655388235319,
0.167606622324439,0.18755797051286,0.207290121019144,0.226806056807627,
0.246779384867164,0.266832954580611,0.276661997683397,0.286514670215304,
0.30652070403251,0.315210277187737,0.315239843192017),.UNSPECIFIED.);
#2766=B_SPLINE_CURVE_WITH_KNOTS('',3,(#120432,#120433,#120434,#120435,#120436,
#120437,#120438,#120439,#120440,#120441,#120442,#120443,#120444,#120445,
#120446,#120447,#120448,#120449,#120450,#120451),.UNSPECIFIED.,.F.,.F.,
(4,2,2,2,2,2,2,2,2,4),(0.315239843192017,0.334905849086587,0.354479560933382,
0.37397666178475,0.393489039425844,0.413099451365576,0.432829362268491,
0.442698129027635,0.462806348593131,0.472865665423056),.UNSPECIFIED.);
#2767=B_SPLINE_CURVE_WITH_KNOTS('',3,(#120454,#120455,#120456,#120457,#120458,
#120459,#120460,#120461,#120462,#120463,#120464,#120465,#120466,#120467,
#120468,#120469,#120470,#120471,#120472,#120473,#120474,#120475,#120476,
#120477,#120478,#120479,#120480,#120481,#120482,#120483,#120484,#120485,
#120486,#120487,#120488,#120489,#120490,#120491,#120492,#120493,#120494,
#120495,#120496,#120497,#120498,#120499,#120500,#120501,#120502,#120503,
#120504,#120505,#120506,#120507,#120508,#120509),.UNSPECIFIED.,.T.,.F.,
(4,2,2,2,2,2,2,2,2,2,2,2,2,2,2,2,2,2,2,2,2,2,2,2,2,2,2,4),(0.,0.039596158659987,
0.0823952911968967,0.126054785698637,0.167083206104417,0.207140413493102,
0.223066542451077,0.229933665475212,0.234259270307438,0.238988436149959,
0.245461112639432,0.260202981801162,0.303691845955503,0.339272904760605,
0.378244153279671,0.420327476204424,0.464148702486995,0.506016018533843,
0.543855540127323,0.565813628575552,0.573689239620962,0.578688275946453,
0.583313046972282,0.589348279542586,0.601974032650628,0.645360865220518,
0.669727977192671,0.689939909009643),.UNSPECIFIED.);
#2768=B_SPLINE_CURVE_WITH_KNOTS('',3,(#120512,#120513,#120514,#120515,#120516,
#120517,#120518,#120519,#120520,#120521,#120522,#120523,#120524,#120525,
#120526,#120527,#120528,#120529,#120530,#120531,#120532,#120533,#120534,
#120535,#120536,#120537,#120538,#120539,#120540,#120541,#120542,#120543,
#120544,#120545,#120546,#120547),.UNSPECIFIED.,.T.,.F.,(4,2,2,2,2,2,2,2,
2,2,2,2,2,2,2,2,2,4),(0.,0.0435930401462006,0.0871572230823697,0.129674587861441,
0.172285514734114,0.215867409321496,0.259652335979,0.303793851724133,0.347750906264732,
0.391036793565589,0.433869767017643,0.476371911416724,0.518865596090745,
0.561678995218631,0.604941064761695,0.62660055680218,0.648177684239587,
0.690509480107086),.UNSPECIFIED.);
#2769=B_SPLINE_CURVE_WITH_KNOTS('',3,(#120551,#120552,#120553,#120554,#120555,
#120556,#120557,#120558,#120559,#120560,#120561,#120562,#120563,#120564,
#120565,#120566,#120567,#120568,#120569,#120570,#120571,#120572,#120573),
 .UNSPECIFIED.,.F.,.F.,(4,2,2,2,2,2,2,2,2,3,4),(0.15531965076079,0.174754840487143,
0.19417250033404,0.213297327409549,0.232446865721418,0.251741462324811,
0.271508668310458,0.281196368653977,0.290901690065796,0.310557892572504,
0.310597054279583),.UNSPECIFIED.);
#2770=B_SPLINE_CURVE_WITH_KNOTS('',3,(#120577,#120578,#120579,#120580,#120581,
#120582,#120583,#120584,#120585,#120586,#120587,#120588,#120589,#120590,
#120591,#120592,#120593,#120594,#120595,#120596,#120597,#120598),
 .UNSPECIFIED.,.F.,.F.,(4,2,2,2,2,2,2,2,2,2,4),(0.310597054279583,0.330158543285891,
0.349421041224732,0.36854476073145,0.38766961382693,0.406934670947526,0.426396249473789,
0.436119083138285,0.445826468337623,0.465607794634539,0.465877543333294),
 .UNSPECIFIED.);
#2771=B_SPLINE_CURVE_WITH_KNOTS('',3,(#120601,#120602,#120603,#120604,#120605,
#120606,#120607,#120608,#120609,#120610,#120611,#120612,#120613,#120614,
#120615,#120616,#120617,#120618,#120619,#120620,#120621,#120622,#120623,
#120624,#120625,#120626,#120627,#120628,#120629,#120630,#120631,#120632,
#120633,#120634,#120635,#120636,#120637,#120638,#120639,#120640,#120641,
#120642,#120643,#120644,#120645,#120646,#120647,#120648,#120649,#120650,
#120651,#120652),.UNSPECIFIED.,.T.,.F.,(4,2,2,2,2,2,2,2,2,2,2,2,2,2,2,2,
2,2,2,2,2,2,2,2,2,4),(0.,0.0457657280663599,0.0962470966331294,0.150688970124808,
0.209205444217228,0.267220868171189,0.320462850227009,0.367511629141848,
0.383955761133481,0.39408136108263,0.403193554022451,0.414678721773825,
0.437106357996681,0.496128410031509,0.544999485599928,0.597826540018831,
0.654417295736584,0.712942843780337,0.769128561133749,0.827041531221436,
0.84482879582721,0.856270263279855,0.865268964852738,0.875182965117314,
0.891087537723763,0.931218391002395),.UNSPECIFIED.);
#2772=B_SPLINE_CURVE_WITH_KNOTS('',3,(#120655,#120656,#120657,#120658,#120659,
#120660,#120661,#120662,#120663,#120664,#120665,#120666,#120667,#120668,
#120669,#120670,#120671,#120672,#120673,#120674,#120675,#120676,#120677,
#120678,#120679,#120680,#120681,#120682,#120683,#120684,#120685,#120686,
#120687,#120688,#120689,#120690,#120691,#120692),.UNSPECIFIED.,.T.,.F.,
(4,2,2,2,2,2,2,2,2,2,2,2,2,2,2,2,2,2,4),(0.,0.058920779517719,0.117921436837851,
0.176593233578414,0.235023562463093,0.293771351172449,0.323059071245716,
0.381271618805364,0.439504199673013,0.497700513711045,0.555783874858827,
0.613753712690792,0.671694751020526,0.729686214224615,0.758678280096495,
0.787653234155945,0.846285702672291,0.904728850431761,0.931714763997535),
 .UNSPECIFIED.);
#2773=B_SPLINE_CURVE_WITH_KNOTS('',3,(#120696,#120697,#120698,#120699,#120700,
#120701,#120702,#120703,#120704,#120705,#120706,#120707,#120708,#120709,
#120710,#120711,#120712,#120713,#120714,#120715,#120716,#120717),
 .UNSPECIFIED.,.F.,.F.,(4,2,2,2,2,2,2,2,2,2,4),(0.13982808209604,0.156684952645851,
0.191864559984887,0.226983871072615,0.261948168518473,0.296885504504634,
0.314000364276795,0.331172042431347,0.366100387596459,0.400659900140943,
0.416615012156061),.UNSPECIFIED.);
#2774=B_SPLINE_CURVE_WITH_KNOTS('',3,(#120721,#120722,#120723,#120724,#120725,
#120726,#120727,#120728,#120729,#120730,#120731,#120732,#120733,#120734,
#120735,#120736,#120737,#120738,#120739,#120740,#120741,#120742,#120743),
 .UNSPECIFIED.,.F.,.F.,(4,2,2,2,2,3,2,2,2,2,4),(0.416615012156061,0.435202420474221,
0.469705730447166,0.504173728227007,0.53863810543123,0.553572697693693,
0.588069349484204,0.605280113114109,0.640265555971116,0.675195238381487,
0.693400779789733),.UNSPECIFIED.);
#2775=B_SPLINE_CURVE_WITH_KNOTS('',3,(#120746,#120747,#120748,#120749,#120750,
#120751,#120752,#120753,#120754,#120755,#120756,#120757,#120758,#120759,
#120760,#120761,#120762,#120763,#120764,#120765,#120766,#120767,#120768,
#120769,#120770,#120771,#120772,#120773,#120774,#120775,#120776,#120777,
#120778,#120779,#120780,#120781,#120782,#120783,#120784,#120785,#120786,
#120787,#120788,#120789,#120790,#120791,#120792,#120793,#120794,#120795,
#120796,#120797,#120798,#120799),.UNSPECIFIED.,.T.,.F.,(4,2,2,2,2,2,2,2,
2,2,2,2,2,2,2,2,2,2,2,2,2,2,2,2,2,2,4),(0.,0.0410256960338938,0.0858843637209721,
0.134180876844018,0.184954132352005,0.234318315071286,0.278865232377034,
0.308469870893335,0.319953448457986,0.327493605622781,0.334631495158405,
0.344159506408106,0.364714387064434,0.415726230703315,0.458014625617533,
0.503817689631654,0.552967727939839,0.603543528547655,0.651759195827544,
0.701438514782395,0.717798245396003,0.726394137160027,0.733341030655905,
0.741207260526554,0.754345756228916,0.799107153766506,0.804128273467629),
 .UNSPECIFIED.);
#2776=B_SPLINE_CURVE_WITH_KNOTS('',3,(#120802,#120803,#120804,#120805,#120806,
#120807,#120808,#120809,#120810,#120811,#120812,#120813,#120814,#120815,
#120816,#120817,#120818,#120819,#120820,#120821,#120822,#120823,#120824,
#120825,#120826,#120827,#120828,#120829,#120830,#120831,#120832,#120833,
#120834,#120835,#120836,#120837),.UNSPECIFIED.,.T.,.F.,(4,2,2,2,2,2,2,2,
2,2,2,2,2,2,2,2,2,4),(0.,0.050671481475036,0.101404234134367,0.152066263127611,
0.202712434371903,0.253657694987048,0.279013189545143,0.32940308141885,
0.379786196260612,0.430059917310446,0.480151651481399,0.530099594615151,
0.580042077960693,0.630109747347428,0.680318594563881,0.730564119609313,
0.781277800571749,0.80467565281243),.UNSPECIFIED.);
#2777=B_SPLINE_CURVE_WITH_KNOTS('',3,(#120841,#120842,#120843,#120844,#120845,
#120846,#120847,#120848,#120849,#120850,#120851,#120852,#120853,#120854,
#120855,#120856,#120857,#120858,#120859,#120860,#120861,#120862),
 .UNSPECIFIED.,.F.,.F.,(4,2,2,2,2,2,2,2,2,2,4),(0.213054899584985,0.213240549849428,
0.240182910677569,0.267129686203949,0.294071943340295,0.321044789490067,
0.348135746666136,0.361567634376776,0.388235323149757,0.414887993400968,
0.426100610580404),.UNSPECIFIED.);
#2778=B_SPLINE_CURVE_WITH_KNOTS('',3,(#120866,#120867,#120868,#120869,#120870,
#120871,#120872,#120873,#120874,#120875,#120876,#120877,#120878,#120879,
#120880,#120881,#120882,#120883,#120884,#120885,#120886),.UNSPECIFIED.,
 .F.,.F.,(4,3,2,2,2,2,2,2,2,4),(0.426100610580404,0.426145242037738,0.452705254015028,
0.47919324694378,0.505655512683507,0.532155454420269,0.558727065325242,
0.585349496759048,0.612421136299796,0.639200141622723),.UNSPECIFIED.);
#2779=B_SPLINE_CURVE_WITH_KNOTS('',3,(#120889,#120890,#120891,#120892,#120893,
#120894,#120895,#120896,#120897,#120898,#120899,#120900,#120901,#120902,
#120903,#120904,#120905,#120906,#120907,#120908,#120909,#120910,#120911,
#120912,#120913,#120914,#120915,#120916,#120917,#120918,#120919,#120920,
#120921,#120922,#120923,#120924,#120925,#120926,#120927,#120928,#120929,
#120930,#120931,#120932,#120933,#120934,#120935,#120936,#120937,#120938,
#120939,#120940,#120941,#120942),.UNSPECIFIED.,.T.,.F.,(4,2,2,2,2,2,2,2,
2,2,2,2,2,2,2,2,2,2,2,2,2,2,2,2,2,2,4),(0.,0.0366013559564401,0.0764365014300665,
0.119372798610828,0.16310043928206,0.204330007717561,0.246666363043394,
0.259193316849719,0.265920265998224,0.271513809212394,0.277203299739624,
0.285363684119845,0.305548661058766,0.349530477740465,0.38627829019971,
0.426163665012696,0.469070659303587,0.51275373872358,0.553769200036606,
0.597242402126746,0.607863717680535,0.614714725095663,0.620139119416996,
0.626171840821019,0.636023118823449,0.668251715399877,0.693912250555093),
 .UNSPECIFIED.);
#2780=B_SPLINE_CURVE_WITH_KNOTS('',3,(#120945,#120946,#120947,#120948,#120949,
#120950,#120951,#120952,#120953,#120954,#120955,#120956,#120957,#120958,
#120959,#120960,#120961,#120962,#120963,#120964,#120965,#120966,#120967,
#120968,#120969,#120970,#120971,#120972,#120973,#120974,#120975,#120976,
#120977,#120978,#120979,#120980,#120981,#120982),.UNSPECIFIED.,.T.,.F.,
(4,2,2,2,2,2,2,2,2,2,2,2,2,2,2,2,2,2,4),(0.,0.043813290614458,0.0876872070663863,
0.13153218183437,0.175328457737809,0.2192572073628,0.240814554252403,0.26246165039269,
0.306530340064736,0.350044147248009,0.393286106662586,0.43627728806497,
0.479194135759194,0.522262928847021,0.565607803967553,0.587360629268619,
0.609062896535199,0.653109830395691,0.69429306613882),.UNSPECIFIED.);
#2781=B_SPLINE_CURVE_WITH_KNOTS('',3,(#120986,#120987,#120988,#120989,#120990,
#120991,#120992,#120993,#120994,#120995,#120996,#120997,#120998,#120999,
#121000,#121001,#121002,#121003,#121004,#121005,#121006,#121007,#121008,
#121009,#121010),.UNSPECIFIED.,.F.,.F.,(4,2,2,2,2,2,2,2,2,2,3,4),(0.157621952213009,
0.157653184764648,0.17762672741589,0.197139809159047,0.216658658704082,
0.236639750750289,0.256668741552331,0.266480438865674,0.27631172587911,
0.29648603104283,0.31518544605496,0.315213231454912),.UNSPECIFIED.);
#2782=B_SPLINE_CURVE_WITH_KNOTS('',3,(#121014,#121015,#121016,#121017,#121018,
#121019,#121020,#121021,#121022,#121023,#121024,#121025,#121026,#121027,
#121028,#121029,#121030,#121031,#121032,#121033),.UNSPECIFIED.,.F.,.F.,
(4,2,2,2,2,2,2,2,2,4),(0.315213231454912,0.334806435763938,0.354325740797582,
0.373820720858293,0.393384197724592,0.413067020071531,0.422927128560577,
0.432773257208208,0.452840403179137,0.472807398267969),.UNSPECIFIED.);
#2783=B_SPLINE_CURVE_WITH_KNOTS('',3,(#121036,#121037,#121038,#121039,#121040,
#121041,#121042,#121043,#121044,#121045,#121046,#121047,#121048,#121049,
#121050,#121051,#121052,#121053,#121054,#121055,#121056,#121057,#121058,
#121059,#121060,#121061,#121062,#121063,#121064,#121065,#121066,#121067,
#121068,#121069,#121070,#121071,#121072,#121073,#121074,#121075,#121076,
#121077,#121078,#121079,#121080,#121081,#121082,#121083,#121084,#121085,
#121086,#121087,#121088,#121089),.UNSPECIFIED.,.T.,.F.,(4,2,2,2,2,2,2,2,
2,2,2,2,2,2,2,2,2,2,2,2,2,2,2,2,2,2,4),(0.,0.037556946163732,0.078353672010978,
0.122434169468536,0.165511233753611,0.20341370217087,0.239374223192113,
0.249493359317307,0.255339187545231,0.259801523354461,0.265512173804729,
0.275307801757659,0.312011429228339,0.345864756632766,0.383397787727872,
0.424095817779774,0.467987976817719,0.511077045633704,0.548989716122193,
0.584500641602089,0.594525810714392,0.60032057717742,0.604744779895977,
0.610406896041102,0.620117805489341,0.656447023762833,0.689896900949306),
 .UNSPECIFIED.);
#2784=B_SPLINE_CURVE_WITH_KNOTS('',3,(#121092,#121093,#121094,#121095,#121096,
#121097,#121098,#121099,#121100,#121101,#121102,#121103,#121104,#121105,
#121106,#121107,#121108,#121109,#121110,#121111,#121112,#121113,#121114,
#121115,#121116,#121117,#121118,#121119,#121120,#121121,#121122,#121123,
#121124,#121125),.UNSPECIFIED.,.T.,.F.,(4,2,2,2,2,2,2,2,2,2,2,2,2,2,2,2,
4),(0.,0.043596439164069,0.0861642710137229,0.128693297937725,0.171468209427599,
0.2150813225096,0.258933409386575,0.303127744859599,0.346899194209671,0.389933113733483,
0.432552889836591,0.475005878811627,0.517643008156437,0.560703769720036,
0.604908662276928,0.648772568902826,0.690554784558767),.UNSPECIFIED.);
#2785=B_SPLINE_CURVE_WITH_KNOTS('',3,(#121129,#121130,#121131,#121132,#121133,
#121134,#121135,#121136,#121137,#121138,#121139,#121140,#121141,#121142,
#121143,#121144,#121145,#121146,#121147,#121148),.UNSPECIFIED.,.F.,.F.,
(4,2,2,2,2,2,2,2,2,4),(0.15526622356778,0.16514719842404,0.184370089139019,
0.203490683518605,0.222647435046449,0.241956293352432,0.261690989855888,
0.28149517603416,0.301354306664443,0.31055959145846),.UNSPECIFIED.);
#2786=B_SPLINE_CURVE_WITH_KNOTS('',3,(#121152,#121153,#121154,#121155,#121156,
#121157,#121158,#121159,#121160,#121161,#121162,#121163,#121164,#121165,
#121166,#121167,#121168,#121169,#121170,#121171,#121172,#121173,#121174),
 .UNSPECIFIED.,.F.,.F.,(4,3,2,2,2,2,2,2,2,2,4),(0.31055959145846,0.310586625858458,
0.329931516356413,0.349100382910039,0.368205489314063,0.387396736722476,
0.406773990247626,0.426614881078628,0.436294287031581,0.456033588890424,
0.465852849426238),.UNSPECIFIED.);
#2787=B_SPLINE_CURVE_WITH_KNOTS('',3,(#121177,#121178,#121179,#121180,#121181,
#121182,#121183,#121184,#121185,#121186,#121187,#121188,#121189,#121190,
#121191,#121192,#121193,#121194,#121195,#121196,#121197,#121198,#121199,
#121200,#121201,#121202,#121203,#121204,#121205,#121206,#121207,#121208,
#121209,#121210,#121211,#121212,#121213,#121214,#121215,#121216,#121217,
#121218,#121219,#121220,#121221,#121222,#121223,#121224,#121225,#121226),
 .UNSPECIFIED.,.T.,.F.,(4,2,2,2,2,2,2,2,2,2,2,2,2,2,2,2,2,2,2,2,2,2,2,2,
4),(0.,0.0589492574510598,0.107914736457218,0.160952293016516,0.217874991214115,
0.276373103612947,0.332619207687263,0.391709189818869,0.41186529192147,
0.423862057197878,0.434357412140907,0.447160303263547,0.470774846569851,
0.529730149181218,0.578950059106104,0.63202778938777,0.688850635712996,
0.747336324371342,0.803360408965686,0.858785238766215,0.878232841788907,
0.889966223471808,0.900224877634544,0.912925203241937,0.931340863912512),
 .UNSPECIFIED.);
#2788=B_SPLINE_CURVE_WITH_KNOTS('',3,(#121229,#121230,#121231,#121232,#121233,
#121234,#121235,#121236,#121237,#121238,#121239,#121240,#121241,#121242,
#121243,#121244,#121245,#121246,#121247,#121248,#121249,#121250,#121251,
#121252,#121253,#121254,#121255,#121256,#121257,#121258,#121259,#121260,
#121261,#121262,#121263,#121264),.UNSPECIFIED.,.T.,.F.,(4,2,2,2,2,2,2,2,
2,2,2,2,2,2,2,2,2,4),(0.,0.058754774143773,0.117403197632285,0.175875621269893,
0.234569790357621,0.293351237166583,0.351590064970777,0.409870781021814,
0.468108002533021,0.526201151535928,0.584144950061525,0.642039413541678,
0.699988642810973,0.728973944077931,0.75796401140306,0.816798564560837,
0.87527518388624,0.931839180559051),.UNSPECIFIED.);
#2789=B_SPLINE_CURVE_WITH_KNOTS('',3,(#121268,#121269,#121270,#121271,#121272,
#121273,#121274,#121275,#121276,#121277,#121278,#121279,#121280,#121281,
#121282,#121283,#121284,#121285),.UNSPECIFIED.,.F.,.F.,(4,2,2,2,2,2,2,2,
4),(0.139818026634276,0.174512333238167,0.209502003810185,0.244448225294873,
0.279493276844203,0.314418985135482,0.348993948138227,0.383582033172368,
0.416694165602581),.UNSPECIFIED.);
#2790=B_SPLINE_CURVE_WITH_KNOTS('',3,(#121289,#121290,#121291,#121292,#121293,
#121294,#121295,#121296,#121297,#121298,#121299,#121300,#121301,#121302,
#121303,#121304,#121305,#121306,#121307,#121308,#121309,#121310,#121311,
#121312,#121313),.UNSPECIFIED.,.F.,.F.,(4,2,2,2,2,3,2,2,2,2,2,4),(0.416694165602581,
0.418149030337749,0.452658452441695,0.487111215703082,0.521548035500538,
0.55363961027923,0.570865744607261,0.588094764652048,0.6232050832238,0.658160766047363,
0.693131459530335,0.693457636913506),.UNSPECIFIED.);
#2791=B_SPLINE_CURVE_WITH_KNOTS('',3,(#121316,#121317,#121318,#121319,#121320,
#121321,#121322,#121323,#121324,#121325,#121326,#121327,#121328,#121329,
#121330,#121331,#121332,#121333,#121334,#121335,#121336,#121337,#121338,
#121339,#121340,#121341,#121342,#121343,#121344,#121345,#121346,#121347,
#121348,#121349,#121350,#121351,#121352,#121353,#121354,#121355,#121356,
#121357,#121358,#121359,#121360,#121361,#121362,#121363,#121364,#121365,
#121366,#121367),.UNSPECIFIED.,.T.,.F.,(4,2,2,2,2,2,2,2,2,2,2,2,2,2,2,2,
2,2,2,2,2,2,2,2,2,4),(0.,0.0507937034377209,0.0942504582104237,0.141185207519934,
0.191662737622325,0.241886687841347,0.288180985331185,0.32953155683084,
0.344017684193696,0.352930093965412,0.360941834251172,0.371024141212346,
0.390645212147654,0.441646633380299,0.483924750998178,0.529687085817695,
0.578771366615263,0.629367932882979,0.677767598915435,0.728753614508766,
0.744574626260671,0.753834295400635,0.760926160148939,0.769993449257638,
0.785403580290456,0.804157258531139),.UNSPECIFIED.);
#2792=B_SPLINE_CURVE_WITH_KNOTS('',3,(#121370,#121371,#121372,#121373,#121374,
#121375,#121376,#121377,#121378,#121379,#121380,#121381,#121382,#121383,
#121384,#121385,#121386,#121387,#121388,#121389,#121390,#121391,#121392,
#121393,#121394,#121395,#121396,#121397,#121398,#121399,#121400,#121401,
#121402,#121403,#121404,#121405),.UNSPECIFIED.,.T.,.F.,(4,2,2,2,2,2,2,2,
2,2,2,2,2,2,2,2,2,4),(0.,0.050833907134388,0.101649533693549,0.152311708696542,
0.203013209115999,0.227882884844094,0.252867746078267,0.303753702130619,
0.354114469975017,0.404361960576347,0.454437938512487,0.504389486437119,
0.554352331677784,0.604444370792824,0.654665986279593,0.705665420859672,
0.75632877106835,0.804655263691419),.UNSPECIFIED.);
#2793=B_SPLINE_CURVE_WITH_KNOTS('',3,(#121409,#121410,#121411,#121412,#121413,
#121414,#121415,#121416,#121417,#121418,#121419,#121420,#121421,#121422,
#121423,#121424,#121425,#121426,#121427,#121428,#121429,#121430),
 .UNSPECIFIED.,.F.,.F.,(4,2,2,2,2,2,2,2,2,2,4),(0.213066841557169,0.213662545774583,
0.240669569811573,0.267670841941382,0.294638476552452,0.321631963442581,
0.334853033549719,0.348108184038777,0.375050927422802,0.401690612064548,
0.426093389507995),.UNSPECIFIED.);
#2794=B_SPLINE_CURVE_WITH_KNOTS('',3,(#121434,#121435,#121436,#121437,#121438,
#121439,#121440,#121441,#121442,#121443,#121444,#121445,#121446,#121447,
#121448,#121449,#121450,#121451,#121452,#121453,#121454),.UNSPECIFIED.,
 .F.,.F.,(4,3,2,2,2,2,2,2,2,4),(0.426093389507995,0.426125083936875,0.452637149993507,
0.479106168396101,0.505591290010395,0.532139726713557,0.558750010866693,
0.585835324843181,0.612814653428274,0.639191925494045),.UNSPECIFIED.);
#2795=B_SPLINE_CURVE_WITH_KNOTS('',3,(#121457,#121458,#121459,#121460,#121461,
#121462,#121463,#121464,#121465,#121466,#121467,#121468,#121469,#121470,
#121471,#121472,#121473,#121474,#121475,#121476,#121477,#121478,#121479,
#121480,#121481,#121482,#121483,#121484,#121485,#121486,#121487,#121488,
#121489,#121490,#121491,#121492,#121493,#121494,#121495,#121496,#121497,
#121498,#121499,#121500,#121501,#121502,#121503,#121504,#121505,#121506,
#121507,#121508,#121509,#121510),.UNSPECIFIED.,.T.,.F.,(4,2,2,2,2,2,2,2,
2,2,2,2,2,2,2,2,2,2,2,2,2,2,2,2,2,2,4),(0.,0.0340495896964589,0.0717326270132875,
0.11252803704836,0.156502200310784,0.199822500511049,0.238843623221006,
0.273853576148806,0.285359660224145,0.292268338347826,0.297771450755393,
0.305083405497963,0.318350110983871,0.362169458367038,0.397913138379148,
0.436911605435009,0.478890528871826,0.522819871797262,0.565180829903189,
0.6049588927033,0.625937273272207,0.635003816763026,0.640690203873801,0.646869547498752,
0.655230481335403,0.673680426876438,0.693806114392571),.UNSPECIFIED.);
#2796=B_SPLINE_CURVE_WITH_KNOTS('',3,(#121513,#121514,#121515,#121516,#121517,
#121518,#121519,#121520,#121521,#121522,#121523,#121524,#121525,#121526,
#121527,#121528,#121529,#121530,#121531,#121532,#121533,#121534,#121535,
#121536,#121537,#121538,#121539,#121540,#121541,#121542,#121543,#121544,
#121545,#121546,#121547,#121548,#121549,#121550),.UNSPECIFIED.,.T.,.F.,
(4,2,2,2,2,2,2,2,2,2,2,2,2,2,2,2,2,2,4),(0.,0.0439347739032266,0.0869159744428171,
0.13077627881111,0.174581205598091,0.218579365897418,0.240178093592474,
0.284240919487602,0.327731207437498,0.370950319256991,0.413931398391036,
0.456855715235624,0.499944459043748,0.543309401480821,0.565046800844102,
0.586695146990834,0.630653497733593,0.674454613655654,0.694278240948528),
 .UNSPECIFIED.);
#2797=B_SPLINE_CURVE_WITH_KNOTS('',3,(#121554,#121555,#121556,#121557,#121558,
#121559,#121560,#121561,#121562,#121563,#121564,#121565,#121566,#121567,
#121568,#121569,#121570,#121571,#121572,#121573,#121574,#121575),
 .UNSPECIFIED.,.F.,.F.,(4,2,2,2,2,2,2,2,2,2,4),(0.157610631276741,0.167958486015372,
0.187466426098309,0.206990222488691,0.22660072328568,0.246603187530971,
0.256396456163226,0.266205345368447,0.286342556288682,0.306065981237513,
0.315177053872359),.UNSPECIFIED.);
#2798=B_SPLINE_CURVE_WITH_KNOTS('',3,(#121579,#121580,#121581,#121582,#121583,
#121584,#121585,#121586,#121587,#121588,#121589,#121590,#121591,#121592,
#121593,#121594,#121595,#121596,#121597,#121598),.UNSPECIFIED.,.F.,.F.,
(4,2,2,2,2,2,2,2,2,4),(0.315177875652213,0.334731312382099,0.354225127407107,
0.373752029378928,0.393385414052036,0.413517586583673,0.423338460875682,
0.443362292717093,0.463349884707035,0.472788506928953),.UNSPECIFIED.);
#2799=B_SPLINE_CURVE_WITH_KNOTS('',3,(#121601,#121602,#121603,#121604,#121605,
#121606,#121607,#121608,#121609,#121610,#121611,#121612,#121613,#121614,
#121615,#121616,#121617,#121618,#121619,#121620,#121621,#121622,#121623,
#121624,#121625,#121626,#121627,#121628,#121629,#121630,#121631,#121632,
#121633,#121634,#121635,#121636,#121637,#121638,#121639,#121640,#121641,
#121642,#121643,#121644,#121645,#121646,#121647,#121648,#121649,#121650,
#121651,#121652,#121653,#121654),.UNSPECIFIED.,.T.,.F.,(4,2,2,2,2,2,2,2,
2,2,2,2,2,2,2,2,2,2,2,2,2,2,2,2,2,2,4),(0.,0.0352022673375941,0.0738901483084225,
0.1157593961888,0.159668433184647,0.201930806507174,0.239710322409318,0.264431621656874,
0.2736438776145,0.279583591391943,0.285134797469431,0.292448528839575,0.307929890803635,
0.351263787235359,0.387082225605215,0.426231499198338,0.468477017309043,
0.512252444068684,0.553957151412746,0.593842927431791,0.612065599873391,
0.620069770023004,0.625148207635513,0.630721384385979,0.638371116778437,
0.655771630237812,0.689842314476748),.UNSPECIFIED.);
#2800=B_SPLINE_CURVE_WITH_KNOTS('',3,(#121657,#121658,#121659,#121660,#121661,
#121662,#121663,#121664,#121665,#121666,#121667,#121668,#121669,#121670,
#121671,#121672,#121673,#121674,#121675,#121676,#121677,#121678,#121679,
#121680,#121681,#121682,#121683,#121684,#121685,#121686,#121687,#121688,
#121689,#121690,#121691,#121692),.UNSPECIFIED.,.T.,.F.,(4,2,2,2,2,2,2,2,
2,2,2,2,2,2,2,2,2,4),(0.,0.0435016177078772,0.0860121887793504,0.12862128786204,
0.172202755572531,0.216057150084804,0.237598491123779,0.281980320515373,
0.325446999346799,0.368494831481356,0.411117560750869,0.453561023893441,
0.496180500458554,0.539222786240642,0.58266489810085,0.626698842331351,
0.67038314380947,0.690425413549481),.UNSPECIFIED.);
#2801=B_SPLINE_CURVE_WITH_KNOTS('',3,(#121696,#121697,#121698,#121699,#121700,
#121701,#121702,#121703,#121704,#121705,#121706,#121707,#121708,#121709,
#121710,#121711,#121712,#121713,#121714,#121715,#121716,#121717),
 .UNSPECIFIED.,.F.,.F.,(4,2,2,2,2,2,2,2,2,2,4),(0.155304341878299,0.155614346327306,
0.175017713542264,0.194137740808806,0.213289212695199,0.232988751462658,
0.252789069790465,0.262496324252049,0.282415062372032,0.302087245052277,
0.310566042860497),.UNSPECIFIED.);
#2802=B_SPLINE_CURVE_WITH_KNOTS('',3,(#121721,#121722,#121723,#121724,#121725,
#121726,#121727,#121728,#121729,#121730,#121731,#121732,#121733,#121734,
#121735,#121736,#121737,#121738),.UNSPECIFIED.,.F.,.F.,(4,2,2,2,2,2,2,2,
4),(0.310566841812876,0.329820690946879,0.348938270234188,0.368061455771084,
0.38732839010858,0.406792237945073,0.426685381368033,0.446482972279099,
0.465870384738796),.UNSPECIFIED.);
#2803=B_SPLINE_CURVE_WITH_KNOTS('',3,(#121741,#121742,#121743,#121744,#121745,
#121746,#121747,#121748,#121749,#121750,#121751,#121752,#121753,#121754,
#121755,#121756,#121757,#121758,#121759,#121760,#121761,#121762,#121763,
#121764,#121765,#121766,#121767,#121768,#121769,#121770,#121771,#121772,
#121773,#121774,#121775,#121776,#121777,#121778,#121779,#121780,#121781,
#121782,#121783,#121784,#121785,#121786,#121787,#121788,#121789,#121790),
 .UNSPECIFIED.,.T.,.F.,(4,2,2,2,2,2,2,2,2,2,2,2,2,2,2,2,2,2,2,2,2,2,2,2,
4),(0.,0.0146814900877869,0.0403932201823766,0.0996751527325199,0.149718027008705,
0.203629369858852,0.261440655475543,0.319739221183558,0.375087111970191,
0.423126186803048,0.443374355706851,0.456859239591619,0.469635723415156,
0.486523100520705,0.521324927686473,0.580568089427896,0.631598426631969,
0.686262802022563,0.744843360768508,0.802806482356597,0.856102034365298,
0.894199591680106,0.912116451169146,0.924831843263324,0.931217467582355),
 .UNSPECIFIED.);
#2804=B_SPLINE_CURVE_WITH_KNOTS('',3,(#121793,#121794,#121795,#121796,#121797,
#121798,#121799,#121800,#121801,#121802,#121803,#121804,#121805,#121806,
#121807,#121808,#121809,#121810,#121811,#121812,#121813,#121814,#121815,
#121816,#121817,#121818,#121819,#121820,#121821,#121822,#121823,#121824,
#121825,#121826,#121827,#121828),.UNSPECIFIED.,.T.,.F.,(4,2,2,2,2,2,2,2,
2,2,2,2,2,2,2,2,2,4),(0.,0.0587304660413623,0.117261312681522,0.175782378681062,
0.234811396887744,0.293027463812867,0.351294329347738,0.409567101310013,
0.467736885839166,0.525743559075219,0.583645163091547,0.641559649632323,
0.699549298941314,0.728539390326633,0.78735949377363,0.845834430734695,
0.904430972318154,0.93184955269919),.UNSPECIFIED.);
#2805=B_SPLINE_CURVE_WITH_KNOTS('',3,(#121832,#121833,#121834,#121835,#121836,
#121837,#121838,#121839,#121840,#121841,#121842,#121843,#121844,#121845,
#121846,#121847,#121848,#121849,#121850,#121851),.UNSPECIFIED.,.F.,.F.,
(4,2,2,2,2,2,2,2,2,4),(0.139782642488671,0.157277236176017,0.192263350991827,
0.227209833005202,0.262263155174017,0.297189356143265,0.331765243145084,
0.366353631343455,0.40091932638502,0.416650087036247),.UNSPECIFIED.);
#2806=B_SPLINE_CURVE_WITH_KNOTS('',3,(#121855,#121856,#121857,#121858,#121859,
#121860,#121861,#121862,#121863,#121864,#121865,#121866,#121867,#121868,
#121869,#121870,#121871,#121872,#121873,#121874,#121875,#121876,#121877),
 .UNSPECIFIED.,.F.,.F.,(4,2,2,2,2,3,2,2,2,2,4),(0.416650087036247,0.43542645929999,
0.469877637670099,0.504314536277139,0.538777951627268,0.553655749381749,
0.57088485344067,0.605987902900473,0.640941818311758,0.675913700988461,
0.693438391870421),.UNSPECIFIED.);
#2807=B_SPLINE_CURVE_WITH_KNOTS('',3,(#121880,#121881,#121882,#121883,#121884,
#121885,#121886,#121887,#121888,#121889,#121890,#121891,#121892,#121893,
#121894,#121895,#121896,#121897,#121898,#121899,#121900,#121901,#121902,
#121903,#121904,#121905,#121906,#121907,#121908,#121909,#121910,#121911,
#121912,#121913,#121914,#121915,#121916,#121917,#121918,#121919,#121920,
#121921,#121922,#121923,#121924,#121925,#121926,#121927,#121928,#121929,
#121930,#121931),.UNSPECIFIED.,.T.,.F.,(4,2,2,2,2,2,2,2,2,2,2,2,2,2,2,2,
2,2,2,2,2,2,2,2,2,4),(0.,0.0251512584232482,0.0759877853106741,0.119405408870884,
0.16625754672263,0.216603813925032,0.266895795796829,0.313787921137438,
0.354118828253151,0.36990456778704,0.380105008924405,0.389584676639667,
0.401905547614001,0.426921516051744,0.477783291068181,0.521019289601979,
0.567585491492379,0.617510443801545,0.667882138154644,0.715128069050405,
0.756057760669801,0.771905259786264,0.782049406675469,0.791401652048583,
0.803444832488867,0.804103777769588),.UNSPECIFIED.);
#2808=B_SPLINE_CURVE_WITH_KNOTS('',3,(#121934,#121935,#121936,#121937,#121938,
#121939,#121940,#121941,#121942,#121943,#121944,#121945,#121946,#121947,
#121948,#121949,#121950,#121951,#121952,#121953,#121954,#121955,#121956,
#121957,#121958,#121959,#121960,#121961,#121962,#121963,#121964,#121965,
#121966,#121967,#121968,#121969,#121970,#121971),.UNSPECIFIED.,.T.,.F.,
(4,2,2,2,2,2,2,2,2,2,2,2,2,2,2,2,2,2,4),(0.,0.0508792217220559,0.10162781996598,
0.15226341389946,0.203118878795053,0.22810150196294,0.278985025900999,0.329338017561462,
0.379573992903277,0.429640500475744,0.479590456671073,0.529560364764325,
0.579662501253364,0.604751617442169,0.629853487047417,0.680809050484543,
0.731459039231061,0.782167614091922,0.804545530220026),.UNSPECIFIED.);
#2809=B_SPLINE_CURVE_WITH_KNOTS('',3,(#121975,#121976,#121977,#121978,#121979,
#121980,#121981,#121982,#121983,#121984,#121985,#121986,#121987,#121988,
#121989,#121990,#121991,#121992,#121993,#121994,#121995,#121996),
 .UNSPECIFIED.,.F.,.F.,(4,2,2,2,2,2,2,2,2,2,4),(0.213062544082035,0.227396210814127,
0.254408164208183,0.281378412056288,0.308367215720059,0.32158497568968,
0.334835900148672,0.361777221247026,0.388412697486444,0.414986226725616,
0.426072215562033),.UNSPECIFIED.);
#2810=B_SPLINE_CURVE_WITH_KNOTS('',3,(#122000,#122001,#122002,#122003,#122004,
#122005,#122006,#122007,#122008,#122009,#122010,#122011,#122012,#122013,
#122014,#122015,#122016,#122017,#122018,#122019),.UNSPECIFIED.,.F.,.F.,
(4,2,2,2,2,2,2,2,2,4),(0.426073055069735,0.45255530258914,0.479026549487086,
0.50554445216474,0.532131476024713,0.545427554156093,0.572495206369301,
0.599468234270871,0.626448478859957,0.63913559915177),.UNSPECIFIED.);
#2811=B_SPLINE_CURVE_WITH_KNOTS('',3,(#122022,#122023,#122024,#122025,#122026,
#122027,#122028,#122029,#122030,#122031,#122032,#122033,#122034,#122035,
#122036,#122037,#122038,#122039,#122040,#122041,#122042,#122043,#122044,
#122045,#122046,#122047,#122048,#122049,#122050,#122051,#122052,#122053,
#122054,#122055,#122056,#122057,#122058,#122059,#122060,#122061,#122062,
#122063,#122064,#122065,#122066,#122067,#122068,#122069,#122070,#122071,
#122072,#122073),.UNSPECIFIED.,.T.,.F.,(4,2,2,2,2,2,2,2,2,2,2,2,2,2,2,2,
2,2,2,2,2,2,2,2,2,4),(0.,0.0440069107173191,0.0805041598387523,0.120195090458515,
0.162944901989734,0.206734560097777,0.248397511361373,0.29230637149236,
0.306355177191658,0.314519420881693,0.321558923387898,0.3300369356061,0.34544587077815,
0.38933609730284,0.425577319914237,0.464967314809013,0.507320950852571,
0.551170882890177,0.593174602554415,0.635677047601321,0.651757900842182,
0.660344658217508,0.667331111227712,0.675273121184593,0.688553612441433,
0.693940242356045),.UNSPECIFIED.);
#2812=B_SPLINE_CURVE_WITH_KNOTS('',3,(#122076,#122077,#122078,#122079,#122080,
#122081,#122082,#122083,#122084,#122085,#122086,#122087,#122088,#122089,
#122090,#122091,#122092,#122093,#122094,#122095,#122096,#122097,#122098,
#122099,#122100,#122101,#122102,#122103,#122104,#122105,#122106,#122107,
#122108,#122109,#122110,#122111,#122112,#122113),.UNSPECIFIED.,.T.,.F.,
(4,2,2,2,2,2,2,2,2,2,2,2,2,2,2,2,2,2,4),(0.,0.0438389442248891,0.0876506808071734,
0.131441119700838,0.175401927756875,0.196981044998168,0.218653481449126,
0.262711426228952,0.306215256616897,0.349443427925576,0.392423288200706,
0.435336799977891,0.478410083186314,0.521761202550275,0.543514873045346,
0.565221898322078,0.609273798985652,0.65308768053503,0.694240451037776),
 .UNSPECIFIED.);
#2813=B_SPLINE_CURVE_WITH_KNOTS('',3,(#122117,#122118,#122119,#122120,#122121,
#122122,#122123,#122124,#122125,#122126,#122127,#122128,#122129,#122130,
#122131,#122132,#122133,#122134,#122135,#122136,#122137,#122138),
 .UNSPECIFIED.,.F.,.F.,(4,2,2,2,2,2,2,2,2,2,4),(0.157584368232204,0.158006990486079,
0.177516943435242,0.19703668521392,0.217016218832852,0.237058339849597,
0.246878518641527,0.256719439219093,0.276906190297129,0.296633512619878,
0.315161445165693),.UNSPECIFIED.);
#2814=B_SPLINE_CURVE_WITH_KNOTS('',3,(#122142,#122143,#122144,#122145,#122146,
#122147,#122148,#122149,#122150,#122151,#122152,#122153,#122154,#122155,
#122156,#122157,#122158,#122159,#122160,#122161),.UNSPECIFIED.,.F.,.F.,
(4,2,2,2,2,2,2,2,2,4),(0.315161496914806,0.334675383606245,0.35416969963247,
0.373736756484906,0.393424082824057,0.403288169457306,0.413138376950184,
0.433210368829472,0.453206070159705,0.47274586514701),.UNSPECIFIED.);
#2815=B_SPLINE_CURVE_WITH_KNOTS('',3,(#122164,#122165,#122166,#122167,#122168,
#122169,#122170,#122171,#122172,#122173,#122174,#122175,#122176,#122177,
#122178,#122179,#122180,#122181,#122182,#122183,#122184,#122185,#122186,
#122187,#122188,#122189,#122190,#122191,#122192,#122193,#122194,#122195,
#122196,#122197,#122198,#122199,#122200,#122201,#122202,#122203,#122204,
#122205,#122206,#122207,#122208,#122209,#122210,#122211,#122212,#122213,
#122214,#122215,#122216,#122217),.UNSPECIFIED.,.T.,.F.,(4,2,2,2,2,2,2,2,
2,2,2,2,2,2,2,2,2,2,2,2,2,2,2,2,2,2,4),(0.,0.0322798876799803,0.0685606018541347,
0.108160762822184,0.150933434540211,0.194602986518808,0.23580572634401,
0.278247026689384,0.290959529057898,0.299011621102778,0.305277960644338,
0.312125374882226,0.323016402638355,0.356065834727992,0.389855079384049,
0.427272683016013,0.46783379181312,0.511548002156746,0.554746610986197,
0.593617964666262,0.627942371636709,0.639441324513358,0.646393389257674,
0.651954457241392,0.65936928222828,0.672885707450089,0.689781272001862),
 .UNSPECIFIED.);
#2816=B_SPLINE_CURVE_WITH_KNOTS('',3,(#122220,#122221,#122222,#122223,#122224,
#122225,#122226,#122227,#122228,#122229,#122230,#122231,#122232,#122233,
#122234,#122235,#122236,#122237,#122238,#122239,#122240,#122241,#122242,
#122243,#122244,#122245,#122246,#122247,#122248,#122249,#122250,#122251,
#122252,#122253,#122254,#122255),.UNSPECIFIED.,.T.,.F.,(4,2,2,2,2,2,2,2,
2,2,2,2,2,2,2,2,2,4),(0.,0.0430238998492563,0.0855495432772724,0.129093659280037,
0.172765482913272,0.194198251448662,0.215713043540718,0.260038404831785,
0.303483524869659,0.346505583580621,0.38911120796889,0.431553960019549,
0.474187363803603,0.517247893807355,0.560698863378657,0.604659525929812,
0.648310276563095,0.69036198545067),.UNSPECIFIED.);
#2817=B_SPLINE_CURVE_WITH_KNOTS('',3,(#122259,#122260,#122261,#122262,#122263,
#122264,#122265,#122266,#122267,#122268,#122269,#122270,#122271,#122272,
#122273,#122274,#122275,#122276,#122277,#122278,#122279,#122280),
 .UNSPECIFIED.,.F.,.F.,(4,2,2,2,2,2,2,2,2,2,4),(0.155290377429681,0.155736107592449,
0.17488551807521,0.194003788295001,0.213226575722084,0.232961080634223,
0.242634223098727,0.252327558687821,0.272217875481461,0.291885970236276,
0.310528859738257),.UNSPECIFIED.);
#2818=B_SPLINE_CURVE_WITH_KNOTS('',3,(#122284,#122285,#122286,#122287,#122288,
#122289,#122290,#122291,#122292,#122293,#122294,#122295,#122296,#122297,
#122298,#122299,#122300,#122301),.UNSPECIFIED.,.F.,.F.,(4,2,2,2,2,2,2,2,
4),(0.310529493700324,0.329692092162944,0.348793029124575,0.3679828392031,
0.387359973042316,0.407247623417337,0.427064981708464,0.446792783922369,
0.465819871130005),.UNSPECIFIED.);
#2819=B_SPLINE_CURVE_WITH_KNOTS('',3,(#122305,#122306,#122307,#122308,#122309,
#122310,#122311,#122312,#122313,#122314,#122315,#122316,#122317,#122318,
#122319,#122320,#122321,#122322,#122323,#122324,#122325,#122326,#122327,
#122328,#122329,#122330,#122331,#122332,#122333,#122334,#122335,#122336,
#122337,#122338,#122339,#122340),.UNSPECIFIED.,.T.,.F.,(4,2,2,2,2,2,2,2,
2,2,2,2,2,2,2,2,2,4),(0.,0.0586757670894926,0.117148553828277,0.175835299561973,
0.234617343239876,0.292853783791768,0.35112523429996,0.40934790866558,0.467429051180109,
0.525371799214443,0.583276714932037,0.641239111551701,0.670226582819686,
0.699216950303947,0.757975002952515,0.816444247800303,0.875085664577425,
0.931838732230833),.UNSPECIFIED.);
#2820=B_SPLINE_CURVE_WITH_KNOTS('',3,(#122344,#122345,#122346,#122347,#122348,
#122349,#122350,#122351,#122352,#122353,#122354,#122355,#122356,#122357,
#122358,#122359,#122360,#122361,#122362,#122363),.UNSPECIFIED.,.F.,.F.,
(4,2,2,2,2,2,2,2,2,4),(0.139760712682487,0.140067134145623,0.175076082565958,
0.210024263823074,0.245061416664295,0.27998722238202,0.314560327877607,
0.349142502650659,0.383701322132445,0.416632407884874),.UNSPECIFIED.);
#2821=B_SPLINE_CURVE_WITH_KNOTS('',3,(#122367,#122368,#122369,#122370,#122371,
#122372,#122373,#122374,#122375,#122376,#122377,#122378,#122379,#122380,
#122381,#122382,#122383,#122384,#122385,#122386,#122387,#122388,#122389),
 .UNSPECIFIED.,.F.,.F.,(4,2,2,2,2,2,3,2,2,2,4),(0.416632407884874,0.418204784014263,
0.452657939033403,0.487101288526142,0.521571286252258,0.537552757131005,
0.553655480527853,0.588723712999936,0.623672800339298,0.658668999727483,
0.69341619321034),.UNSPECIFIED.);
#2822=B_SPLINE_CURVE_WITH_KNOTS('',3,(#122393,#122394,#122395,#122396,#122397,
#122398,#122399,#122400,#122401,#122402,#122403,#122404,#122405,#122406,
#122407,#122408,#122409,#122410,#122411,#122412,#122413,#122414,#122415,
#122416,#122417,#122418,#122419,#122420,#122421,#122422,#122423,#122424,
#122425,#122426,#122427,#122428,#122429,#122430),.UNSPECIFIED.,.T.,.F.,
(4,2,2,2,2,2,2,2,2,2,2,2,2,2,2,2,2,2,4),(0.,0.050673276883592,0.101289176630062,
0.152081759329459,0.177020645452896,0.202374739783901,0.252767720361165,
0.303150046715415,0.353415021404996,0.403493331193659,0.45343162999718,
0.503373416551825,0.553446254375365,0.578529932675748,0.603629101080887,
0.653871646642357,0.704574133420325,0.75519545932242,0.804523692757691),
 .UNSPECIFIED.);
#2823=B_SPLINE_CURVE_WITH_KNOTS('',3,(#122434,#122435,#122436,#122437,#122438,
#122439,#122440,#122441,#122442,#122443,#122444,#122445,#122446,#122447,
#122448,#122449,#122450,#122451,#122452,#122453,#122454,#122455,#122456,
#122457,#122458),.UNSPECIFIED.,.F.,.F.,(4,2,2,2,2,2,2,2,2,2,3,4),(0.213033721720665,
0.213549478728336,0.24047802645704,0.267424502166104,0.294464476694524,
0.307719796467723,0.321150652985462,0.347819019993753,0.374470148743606,
0.401059222374504,0.426055563255932,0.426056605130622),.UNSPECIFIED.);
#2824=B_SPLINE_CURVE_WITH_KNOTS('',3,(#122462,#122463,#122464,#122465,#122466,
#122467,#122468,#122469,#122470,#122471,#122472,#122473,#122474,#122475,
#122476,#122477,#122478,#122479,#122480,#122481),.UNSPECIFIED.,.F.,.F.,
(4,2,2,2,2,2,2,2,2,4),(0.426056605130622,0.452518691987417,0.478993507171365,
0.50553229834979,0.5188187144497,0.532113581809939,0.5587398015711,0.585740731909802,
0.612676088223349,0.639089284976597),.UNSPECIFIED.);
#2825=B_SPLINE_CURVE_WITH_KNOTS('',3,(#122484,#122485,#122486,#122487,#122488,
#122489,#122490,#122491,#122492,#122493,#122494,#122495,#122496,#122497,
#122498,#122499,#122500,#122501,#122502,#122503,#122504,#122505,#122506,
#122507,#122508,#122509,#122510,#122511,#122512,#122513,#122514,#122515,
#122516,#122517,#122518,#122519,#122520,#122521,#122522,#122523,#122524,
#122525,#122526,#122527,#122528,#122529,#122530,#122531,#122532,#122533),
 .UNSPECIFIED.,.T.,.F.,(4,2,2,2,2,2,2,2,2,2,2,2,2,2,2,2,2,2,2,2,2,2,2,2,
4),(0.,0.0107674088208145,0.032050092364627,0.0758968238756297,0.113342112075795,
0.153841759557963,0.197424662011024,0.24094865716672,0.281477151458961,
0.315965112974783,0.329860021699639,0.338958849354584,0.347492432482236,
0.358682378546163,0.381656726340758,0.425505843569457,0.463082431170076,
0.503625071404071,0.547176362783087,0.590646422407844,0.630909084266853,
0.663727441955104,0.677240304474487,0.686199000451462,0.693838454416704),
 .UNSPECIFIED.);
#2826=B_SPLINE_CURVE_WITH_KNOTS('',3,(#122536,#122537,#122538,#122539,#122540,
#122541,#122542,#122543,#122544,#122545,#122546,#122547,#122548,#122549,
#122550,#122551,#122552,#122553,#122554,#122555,#122556,#122557,#122558,
#122559,#122560,#122561,#122562,#122563,#122564,#122565,#122566,#122567,
#122568,#122569,#122570,#122571,#122572,#122573),.UNSPECIFIED.,.T.,.F.,
(4,2,2,2,2,2,2,2,2,2,2,2,2,2,2,2,2,2,4),(0.,0.0438243930740146,0.0876062081298315,
0.131457732547539,0.175607022982147,0.197291180384503,0.241342381381052,
0.284837958123228,0.328055583488919,0.371028367060835,0.413942440611152,
0.457022969056832,0.500382292840913,0.522137595971807,0.543841887873517,
0.587887555125371,0.631697460152709,0.675489393505295,0.694245519838248),
 .UNSPECIFIED.);
#2827=B_SPLINE_CURVE_WITH_KNOTS('',3,(#122577,#122578,#122579,#122580,#122581,
#122582,#122583,#122584,#122585,#122586,#122587,#122588,#122589,#122590,
#122591,#122592,#122593,#122594,#122595,#122596,#122597,#122598),
 .UNSPECIFIED.,.F.,.F.,(4,2,2,2,2,2,2,2,2,2,4),(0.157602387106129,0.167770702836318,
0.187291656000666,0.207271901672337,0.227319605740903,0.237143104959657,
0.246987541016024,0.267178023530022,0.286901794386752,0.306504569661967,
0.315162938093162),.UNSPECIFIED.);
#2828=B_SPLINE_CURVE_WITH_KNOTS('',3,(#122602,#122603,#122604,#122605,#122606,
#122607,#122608,#122609,#122610,#122611,#122612,#122613,#122614,#122615,
#122616,#122617,#122618,#122619,#122620,#122621),.UNSPECIFIED.,.F.,.F.,
(4,2,2,2,2,2,2,2,2,4),(0.315162961924269,0.334653864296084,0.354176529092422,
0.373805857336121,0.393549777338162,0.403400597304252,0.423472399890395,
0.443466235193495,0.463424991039942,0.472765325199292),.UNSPECIFIED.);
#2829=B_SPLINE_CURVE_WITH_KNOTS('',3,(#122624,#122625,#122626,#122627,#122628,
#122629,#122630,#122631,#122632,#122633,#122634,#122635,#122636,#122637,
#122638,#122639,#122640,#122641,#122642,#122643,#122644,#122645,#122646,
#122647,#122648,#122649,#122650,#122651,#122652,#122653,#122654,#122655,
#122656,#122657,#122658,#122659,#122660,#122661,#122662,#122663,#122664,
#122665,#122666,#122667,#122668,#122669,#122670,#122671,#122672,#122673,
#122674,#122675),.UNSPECIFIED.,.T.,.F.,(4,2,2,2,2,2,2,2,2,2,2,2,2,2,2,2,
2,2,2,2,2,2,2,2,2,4),(0.,0.0256189301624599,0.0585560093974178,0.0952620183024296,
0.135208137493268,0.178316557997087,0.221875433422912,0.262673142368552,
0.302028045604151,0.315630477424899,0.323864618891318,0.33043727500203,
0.3391632615135,0.354876094361664,0.398358935388055,0.434466067107987,0.473802934543292,
0.516197041102924,0.559937408000424,0.601593888860772,0.644357103880208,
0.659194186873084,0.667768270573467,0.674987161506823,0.683465595734622,
0.689846633560524),.UNSPECIFIED.);
#2830=B_SPLINE_CURVE_WITH_KNOTS('',3,(#122678,#122679,#122680,#122681,#122682,
#122683,#122684,#122685,#122686,#122687,#122688,#122689,#122690,#122691,
#122692,#122693,#122694,#122695,#122696,#122697,#122698,#122699,#122700,
#122701,#122702,#122703,#122704,#122705,#122706,#122707,#122708,#122709,
#122710,#122711,#122712,#122713,#122714,#122715),.UNSPECIFIED.,.T.,.F.,
(4,2,2,2,2,2,2,2,2,2,2,2,2,2,2,2,2,2,4),(0.,0.0425025968360725,0.0851241096660763,
0.128708281636964,0.17255349411788,0.19408748717439,0.238446766102907,0.281883879757632,
0.324894484406876,0.367490323725331,0.409929583877134,0.452566309918705,
0.495632893687133,0.517333643790689,0.538995930030127,0.58297389480917,
0.626627855561898,0.670154211137559,0.690235808572164),.UNSPECIFIED.);
#2831=B_SPLINE_CURVE_WITH_KNOTS('',3,(#122719,#122720,#122721,#122722,#122723,
#122724,#122725,#122726,#122727,#122728,#122729,#122730,#122731,#122732,
#122733,#122734,#122735,#122736,#122737,#122738,#122739,#122740),
 .UNSPECIFIED.,.F.,.F.,(4,2,2,2,2,2,2,2,2,2,4),(0.155260120941377,0.165093014777806,
0.184211383687861,0.203435996037152,0.223178890816999,0.232858171175101,
0.242559308220261,0.262463457205943,0.282125538253841,0.301453343875752,
0.31047848171439),.UNSPECIFIED.);
#2832=B_SPLINE_CURVE_WITH_KNOTS('',3,(#122744,#122745,#122746,#122747,#122748,
#122749,#122750,#122751,#122752,#122753,#122754,#122755,#122756,#122757,
#122758,#122759,#122760,#122761,#122762,#122763),.UNSPECIFIED.,.F.,.F.,
(4,2,2,2,2,2,2,2,2,4),(0.310479060901921,0.329589414222322,0.348718434799171,
0.367999675413274,0.387476460125835,0.39720372215973,0.417032430741726,
0.436763267001542,0.456424627637958,0.465739181843299),.UNSPECIFIED.);
#2833=B_SPLINE_CURVE_WITH_KNOTS('',3,(#122767,#122768,#122769,#122770,#122771,
#122772,#122773,#122774,#122775,#122776,#122777,#122778,#122779,#122780,
#122781,#122782,#122783,#122784,#122785,#122786,#122787,#122788,#122789,
#122790,#122791,#122792,#122793,#122794,#122795,#122796,#122797,#122798,
#122799,#122800),.UNSPECIFIED.,.T.,.F.,(4,2,2,2,2,2,2,2,2,2,2,2,2,2,2,2,
4),(0.,0.0585926765660801,0.117060852770377,0.175963863544342,0.234757324802159,
0.292998945417122,0.351235837265488,0.409377235300801,0.467380436815063,
0.525306461368404,0.583257580760452,0.641271299034342,0.700216836299,0.75869435519625,
0.817268571442382,0.876149337626487,0.931978006137413),.UNSPECIFIED.);
#2834=B_SPLINE_CURVE_WITH_KNOTS('',3,(#122804,#122805,#122806,#122807,#122808,
#122809,#122810,#122811,#122812,#122813,#122814,#122815,#122816,#122817,
#122818,#122819,#122820,#122821,#122822,#122823),.UNSPECIFIED.,.F.,.F.,
(4,2,2,2,2,2,2,2,2,4),(0.139772579008333,0.140146289744173,0.17514281240646,
0.210084776298185,0.245174835201649,0.28010335525236,0.314672240383326,
0.34923361254127,0.383757569691577,0.416643770851934),.UNSPECIFIED.);
#2835=B_SPLINE_CURVE_WITH_KNOTS('',3,(#122827,#122828,#122829,#122830,#122831,
#122832,#122833,#122834,#122835,#122836,#122837,#122838,#122839,#122840,
#122841,#122842,#122843,#122844,#122845,#122846,#122847),.UNSPECIFIED.,
 .F.,.F.,(4,2,2,2,2,3,2,2,2,4),(0.416643770851934,0.418233336826679,0.452686571599011,
0.487154891484257,0.521648920350911,0.553720957181638,0.588667950785789,
0.623652766915587,0.658756034818722,0.693493536189971),.UNSPECIFIED.);
#2836=B_SPLINE_CURVE_WITH_KNOTS('',3,(#122851,#122852,#122853,#122854,#122855,
#122856,#122857,#122858,#122859,#122860,#122861,#122862,#122863,#122864,
#122865,#122866,#122867,#122868,#122869,#122870,#122871,#122872,#122873,
#122874,#122875,#122876,#122877,#122878,#122879,#122880,#122881,#122882,
#122883,#122884,#122885,#122886,#122887,#122888),.UNSPECIFIED.,.T.,.F.,
(4,2,2,2,2,2,2,2,2,2,2,2,2,2,2,2,2,2,4),(0.,0.0507229383181265,0.101364562659594,
0.152264741697718,0.177621136402009,0.228004403729544,0.278358115075993,
0.328590359266365,0.378650356083607,0.428595870888352,0.478566224724603,
0.528671625350514,0.553761862420612,0.578863709834058,0.62981803707715,
0.680469487571423,0.731173027366969,0.782017463135863,0.804541332944367),
 .UNSPECIFIED.);
#2837=B_SPLINE_CURVE_WITH_KNOTS('',3,(#122892,#122893,#122894,#122895,#122896,
#122897,#122898,#122899,#122900,#122901,#122902,#122903,#122904,#122905,
#122906,#122907,#122908,#122909,#122910,#122911,#122912,#122913,#122914,
#122915,#122916),.UNSPECIFIED.,.F.,.F.,(4,2,2,2,2,2,2,2,2,2,3,4),(0.213066867406632,
0.227903691482098,0.254869439722097,0.28187163635418,0.295099259249335,
0.308362448361286,0.335302105137811,0.361936581907251,0.38850722497422,
0.415007489812642,0.426072923770395,0.426074041187361),.UNSPECIFIED.);
#2838=B_SPLINE_CURVE_WITH_KNOTS('',3,(#122920,#122921,#122922,#122923,#122924,
#122925,#122926,#122927,#122928,#122929,#122930,#122931,#122932,#122933,
#122934,#122935,#122936,#122937,#122938,#122939),.UNSPECIFIED.,.F.,.F.,
(4,2,2,2,2,2,2,2,2,4),(0.426074041187361,0.452544161682515,0.479064421758956,
0.505653908774553,0.51895026828597,0.546020643171311,0.572994766851648,
0.599970746744037,0.626979273531269,0.639139791177027),.UNSPECIFIED.);
#2839=B_SPLINE_CURVE_WITH_KNOTS('',3,(#122943,#122944,#122945,#122946,#122947,
#122948,#122949,#122950,#122951,#122952,#122953,#122954,#122955,#122956,
#122957,#122958,#122959,#122960,#122961,#122962,#122963,#122964,#122965,
#122966,#122967,#122968,#122969,#122970,#122971,#122972,#122973,#122974,
#122975,#122976,#122977,#122978,#122979,#122980),.UNSPECIFIED.,.T.,.F.,
(4,2,2,2,2,2,2,2,2,2,2,2,2,2,2,2,2,2,4),(0.,0.0437776276195715,0.0875679900144141,
0.131571445742023,0.153177954178476,0.175159227728739,0.218816832071539,
0.262314817569206,0.305533297393407,0.348505149880481,0.39141745318968,
0.43449638406335,0.477854755514743,0.499610120533722,0.52132723824042,0.565391550289609,
0.609202037344911,0.652974164254737,0.694228661865369),.UNSPECIFIED.);
#2840=B_SPLINE_CURVE_WITH_KNOTS('',3,(#122984,#122985,#122986,#122987,#122988,
#122989,#122990,#122991,#122992,#122993,#122994,#122995,#122996,#122997,
#122998,#122999,#123000,#123001,#123002,#123003,#123004,#123005),
 .UNSPECIFIED.,.F.,.F.,(4,2,2,2,2,2,2,2,2,2,4),(0.157582047532889,0.158016502864322,
0.177538316893226,0.197519409217786,0.217579884773166,0.227411236627675,
0.237264279446347,0.257255031976338,0.276977952611641,0.296579243132181,
0.315156893082293),.UNSPECIFIED.);
#2841=B_SPLINE_CURVE_WITH_KNOTS('',3,(#123009,#123010,#123011,#123012,#123013,
#123014,#123015,#123016,#123017,#123018,#123019,#123020,#123021,#123022,
#123023,#123024,#123025,#123026,#123027,#123028),.UNSPECIFIED.,.F.,.F.,
(4,2,2,2,2,2,2,2,2,4),(0.315157288501979,0.334652252907642,0.354224086191744,
0.373916998640349,0.383787341684051,0.393643851193707,0.413723260089021,
0.433716344820741,0.453665515143594,0.472739336034868),.UNSPECIFIED.);
#2842=B_SPLINE_CURVE_WITH_KNOTS('',3,(#123032,#123033,#123034,#123035,#123036,
#123037,#123038,#123039,#123040,#123041,#123042,#123043,#123044,#123045,
#123046,#123047,#123048,#123049,#123050,#123051,#123052,#123053,#123054,
#123055,#123056,#123057,#123058,#123059,#123060,#123061,#123062,#123063,
#123064,#123065,#123066,#123067,#123068,#123069),.UNSPECIFIED.,.T.,.F.,
(4,2,2,2,2,2,2,2,2,2,2,2,2,2,2,2,2,2,4),(0.,0.0425264858563654,0.0860379263816963,
0.129775411807249,0.151257181847517,0.172834633622422,0.217270439947479,
0.26070584185836,0.303710158081262,0.346298776724129,0.388734672817207,
0.431373528152147,0.474445047486068,0.496148628393663,0.517840489242917,
0.561870047910052,0.60553584876945,0.649023088411614,0.690222497519466),
 .UNSPECIFIED.);
#2843=B_SPLINE_CURVE_WITH_KNOTS('',3,(#123073,#123074,#123075,#123076,#123077,
#123078,#123079,#123080,#123081,#123082,#123083,#123084,#123085,#123086,
#123087,#123088,#123089,#123090,#123091,#123092,#123093,#123094),
 .UNSPECIFIED.,.F.,.F.,(4,2,2,2,2,2,2,2,2,2,4),(0.155239240071724,0.155545159095705,
0.174663418665415,0.193888856365997,0.213651467942332,0.223344964073576,
0.233063963677857,0.252999263159233,0.272652527427125,0.291976817994604,
0.310472561331592),.UNSPECIFIED.);
#2844=B_SPLINE_CURVE_WITH_KNOTS('',3,(#123098,#123099,#123100,#123101,#123102,
#123103,#123104,#123105,#123106,#123107,#123108,#123109,#123110,#123111,
#123112,#123113,#123114,#123115,#123116,#123117),.UNSPECIFIED.,.F.,.F.,
(4,2,2,2,2,2,2,2,2,4),(0.310472731789002,0.329571781965114,0.348764795900237,
0.368147384944638,0.377891730151636,0.387634194863333,0.407490285800687,
0.427228176729605,0.4468714803911,0.465711801403316),.UNSPECIFIED.);
#2845=B_SPLINE_CURVE_WITH_KNOTS('',3,(#123121,#123122,#123123,#123124,#123125,
#123126,#123127,#123128,#123129,#123130,#123131,#123132,#123133,#123134,
#123135,#123136,#123137,#123138,#123139,#123140,#123141,#123142,#123143,
#123144,#123145,#123146,#123147,#123148,#123149,#123150,#123151,#123152,
#123153,#123154),.UNSPECIFIED.,.T.,.F.,(4,2,2,2,2,2,2,2,2,2,2,2,2,2,2,2,
4),(0.,0.0584699775520228,0.117165575370348,0.175948938510645,0.234185086571246,
0.292451210877633,0.350662965265276,0.408733587688452,0.466673944838772,
0.524585872842989,0.582557670909233,0.640581469672834,0.699285196519633,
0.757754370947284,0.816432379354141,0.875275608146019,0.931978925642126),
 .UNSPECIFIED.);
#2846=B_SPLINE_CURVE_WITH_KNOTS('',3,(#123158,#123159,#123160,#123161,#123162,
#123163,#123164,#123165,#123166,#123167,#123168,#123169,#123170,#123171,
#123172,#123173,#123174,#123175,#123176,#123177),.UNSPECIFIED.,.F.,.F.,
(4,2,2,2,2,2,2,2,2,4),(0.139770748206514,0.140049608785387,0.174997299730298,
0.210031400032424,0.244957219954342,0.279529040299516,0.314107503356081,
0.348661078446231,0.383160589516241,0.416637496476957),.UNSPECIFIED.);
#2847=B_SPLINE_CURVE_WITH_KNOTS('',3,(#123181,#123182,#123183,#123184,#123185,
#123186,#123187,#123188,#123189,#123190,#123191,#123192,#123193,#123194,
#123195,#123196,#123197,#123198,#123199,#123200,#123201),.UNSPECIFIED.,
 .F.,.F.,(4,2,2,2,2,3,2,2,2,4),(0.416637496476957,0.417613792200944,0.452061028986347,
0.486535436540338,0.521032083188937,0.553718729366543,0.588666002789255,
0.623678907144246,0.658750981999921,0.693489477573057),.UNSPECIFIED.);
#2848=B_SPLINE_CURVE_WITH_KNOTS('',3,(#123205,#123206,#123207,#123208,#123209,
#123210,#123211,#123212,#123213,#123214,#123215,#123216,#123217,#123218,
#123219,#123220,#123221,#123222,#123223,#123224,#123225,#123226,#123227,
#123228,#123229,#123230,#123231,#123232,#123233,#123234,#123235,#123236,
#123237,#123238,#123239,#123240,#123241,#123242),.UNSPECIFIED.,.T.,.F.,
(4,2,2,2,2,2,2,2,2,2,2,2,2,2,2,2,2,2,4),(0.,0.050638733810621,0.101400253214682,
0.12631607681873,0.151671805389745,0.202060284621524,0.252423238238989,
0.302663024997971,0.352724854939833,0.402666384079521,0.452629817735602,
0.502729034043684,0.52781857736665,0.552920189788985,0.603916159489469,
0.654579944565998,0.705256808810519,0.7560470808032,0.804537568823649),
 .UNSPECIFIED.);
#2849=B_SPLINE_CURVE_WITH_KNOTS('',3,(#123246,#123247,#123248,#123249,#123250,
#123251,#123252,#123253,#123254,#123255,#123256,#123257,#123258,#123259,
#123260,#123261,#123262,#123263,#123264,#123265,#123266,#123267),
 .UNSPECIFIED.,.F.,.F.,(4,2,2,2,2,2,2,2,2,2,4),(0.213045628511085,0.214611385801652,
0.241571963452503,0.268595658943336,0.281838232681206,0.29526966423576,
0.321934713953309,0.348573294216842,0.375146966582712,0.401647612531603,
0.426064000816764),.UNSPECIFIED.);
#2850=B_SPLINE_CURVE_WITH_KNOTS('',3,(#123271,#123272,#123273,#123274,#123275,
#123276,#123277,#123278,#123279,#123280,#123281,#123282,#123283,#123284,
#123285,#123286,#123287,#123288,#123289,#123290),.UNSPECIFIED.,.F.,.F.,
(4,2,2,2,2,2,2,2,2,4),(0.426064655025976,0.452551754020046,0.479105237030249,
0.492395062055931,0.505691423761415,0.532783295767128,0.55976324004501,
0.586724469365241,0.613704084643966,0.639109629327848),.UNSPECIFIED.);
#2851=B_SPLINE_CURVE_WITH_KNOTS('',3,(#123294,#123295,#123296,#123297,#123298,
#123299,#123300,#123301,#123302,#123303,#123304,#123305,#123306,#123307,
#123308,#123309,#123310,#123311,#123312,#123313,#123314,#123315,#123316,
#123317,#123318,#123319,#123320,#123321,#123322,#123323,#123324,#123325,
#123326,#123327,#123328,#123329),.UNSPECIFIED.,.T.,.F.,(4,2,2,2,2,2,2,2,
2,2,2,2,2,2,2,2,2,4),(0.,0.043833939544088,0.0876547626552344,0.13171418373345,
0.176143188576216,0.219711530800857,0.263036228023697,0.306089647100756,
0.349005450632323,0.392008244919775,0.435266561780069,0.478772277691574,
0.500403324464899,0.544338765949995,0.588137875440213,0.63201610258223,
0.674982061745284,0.694353973193238),.UNSPECIFIED.);
#2852=B_SPLINE_CURVE_WITH_KNOTS('',3,(#123333,#123334,#123335,#123336,#123337,
#123338,#123339,#123340,#123341,#123342,#123343,#123344,#123345,#123346,
#123347,#123348,#123349,#123350,#123351,#123352),.UNSPECIFIED.,.F.,.F.,
(4,2,2,2,2,2,2,2,2,4),(0.157606283114567,0.167956263024278,0.18794232221838,
0.20795897095516,0.228048601843927,0.248201222227485,0.26790407483132,0.287487183630145,
0.306988348642051,0.31521639087299),.UNSPECIFIED.);
#2853=B_SPLINE_CURVE_WITH_KNOTS('',3,(#123356,#123357,#123358,#123359,#123360,
#123361,#123362,#123363,#123364,#123365,#123366,#123367,#123368,#123369,
#123370,#123371,#123372,#123373,#123374,#123375),.UNSPECIFIED.,.F.,.F.,
(4,2,2,2,2,2,2,2,2,4),(0.315216519374046,0.334753816642054,0.354403128902944,
0.374535263751892,0.384354671581488,0.404377048151514,0.424363772031088,
0.444136761249955,0.463641311616163,0.472822673987557),.UNSPECIFIED.);
#2854=B_SPLINE_CURVE_WITH_KNOTS('',3,(#123379,#123380,#123381,#123382,#123383,
#123384,#123385,#123386,#123387,#123388,#123389,#123390,#123391,#123392,
#123393,#123394,#123395,#123396,#123397,#123398,#123399,#123400,#123401,
#123402,#123403,#123404,#123405,#123406,#123407,#123408,#123409,#123410,
#123411,#123412,#123413,#123414,#123415,#123416),.UNSPECIFIED.,.T.,.F.,
(4,2,2,2,2,2,2,2,2,2,2,2,2,2,2,2,2,2,4),(0.,0.0426485590853426,0.0862402884782325,
0.130075390184566,0.151600424496342,0.195934123792694,0.239336229067572,
0.282303133840975,0.324871762696591,0.367316422243404,0.409987876619906,
0.453097218074252,0.474786527840847,0.496414747803411,0.540321419594795,
0.583944828411629,0.62749138901914,0.670027574651375,0.69023199317909),
 .UNSPECIFIED.);
#2855=B_SPLINE_CURVE_WITH_KNOTS('',3,(#123420,#123421,#123422,#123423,#123424,
#123425,#123426,#123427,#123428,#123429,#123430,#123431,#123432,#123433,
#123434,#123435,#123436,#123437,#123438,#123439,#123440,#123441),
 .UNSPECIFIED.,.F.,.F.,(4,2,2,2,2,2,2,2,2,2,4),(0.155261651907409,0.16527671528697,
0.184519016768904,0.204259152541559,0.213934192699869,0.223628296706432,
0.24351518419013,0.263160537961134,0.282467130496838,0.301609884756148,
0.310478261413411),.UNSPECIFIED.);
#2856=B_SPLINE_CURVE_WITH_KNOTS('',3,(#123445,#123446,#123447,#123448,#123449,
#123450,#123451,#123452,#123453,#123454,#123455,#123456,#123457,#123458,
#123459,#123460,#123461,#123462,#123463,#123464),.UNSPECIFIED.,.F.,.F.,
(4,2,2,2,2,2,2,2,2,4),(0.310478282765048,0.329618019148117,0.348918877254669,
0.368809358815657,0.378523932330328,0.398324219984893,0.418040807624495,
0.43749361537484,0.456631081663014,0.46573991332082),.UNSPECIFIED.);
#2857=B_SPLINE_CURVE_WITH_KNOTS('',3,(#123468,#123469,#123470,#123471,#123472,
#123473,#123474,#123475,#123476,#123477,#123478,#123479,#123480,#123481,
#123482,#123483,#123484,#123485,#123486,#123487,#123488,#123489,#123490,
#123491,#123492,#123493,#123494,#123495,#123496,#123497,#123498,#123499,
#123500,#123501),.UNSPECIFIED.,.T.,.F.,(4,2,2,2,2,2,2,2,2,2,2,2,2,2,2,2,
4),(0.,0.058563364489267,0.117704649598256,0.175927357335253,0.234203267650359,
0.29247366123109,0.350626680658072,0.408614250475086,0.466507970326649,
0.524426802488493,0.582422733706092,0.640447373658858,0.698997907681633,
0.757505974204621,0.816205252734419,0.874894888625525,0.931980995563416),
 .UNSPECIFIED.);
#2858=B_SPLINE_CURVE_WITH_KNOTS('',3,(#123505,#123506,#123507,#123508,#123509,
#123510,#123511,#123512,#123513,#123514,#123515,#123516,#123517,#123518,
#123519,#123520,#123521,#123522,#123523,#123524),.UNSPECIFIED.,.F.,.F.,
(4,2,2,2,2,2,2,2,2,4),(0.139768652132161,0.139884269762596,0.174878693268074,
0.2100959056963,0.244664521169186,0.279252724422164,0.313834457306522,0.348367398742558,
0.382835795250566,0.416634411007083),.UNSPECIFIED.);
#2859=B_SPLINE_CURVE_WITH_KNOTS('',3,(#123528,#123529,#123530,#123531,#123532,
#123533,#123534,#123535,#123536,#123537,#123538,#123539,#123540,#123541,
#123542,#123543,#123544,#123545,#123546,#123547,#123548),.UNSPECIFIED.,
 .F.,.F.,(4,2,2,2,2,3,2,2,2,4),(0.416634411007083,0.417269899088962,0.451717700829539,
0.48620037123172,0.520698761065574,0.55371684967054,0.588663626154184,0.623659124796111,
0.658654452558276,0.693485501802701),.UNSPECIFIED.);
#2860=B_SPLINE_CURVE_WITH_KNOTS('',3,(#123552,#123553,#123554,#123555,#123556,
#123557,#123558,#123559,#123560,#123561,#123562,#123563,#123564,#123565,
#123566,#123567,#123568,#123569,#123570,#123571,#123572,#123573,#123574,
#123575,#123576,#123577,#123578,#123579,#123580,#123581,#123582,#123583,
#123584,#123585,#123586,#123587,#123588,#123589),.UNSPECIFIED.,.T.,.F.,
(4,2,2,2,2,2,2,2,2,2,2,2,2,2,2,2,2,2,4),(0.,0.0506163528267545,0.101414878043581,
0.126365601401302,0.177244213141222,0.227568438122892,0.277767225411541,
0.327809330368101,0.377764479210017,0.427767296504768,0.477908463703247,
0.503005947479194,0.52806740581208,0.578867942145032,0.62948374284351,0.680281858769973,
0.73128102309058,0.782192581946867,0.804565921037956),.UNSPECIFIED.);
#2861=B_SPLINE_CURVE_WITH_KNOTS('',3,(#123593,#123594,#123595,#123596,#123597,
#123598,#123599,#123600,#123601,#123602,#123603,#123604,#123605,#123606,
#123607,#123608,#123609,#123610,#123611,#123612,#123613,#123614,#123615,
#123616,#123617),.UNSPECIFIED.,.F.,.F.,(4,2,2,2,2,2,2,2,2,2,3,4),(0.213105558873963,
0.227668433906905,0.254627533146885,0.267825149105576,0.281051705768159,
0.307989464834126,0.334608596622551,0.36116368773351,0.387657442427522,
0.414131180745578,0.426078364283007,0.426115006982538),.UNSPECIFIED.);
#2862=B_SPLINE_CURVE_WITH_KNOTS('',3,(#123621,#123622,#123623,#123624,#123625,
#123626,#123627,#123628,#123629,#123630,#123631,#123632,#123633,#123634,
#123635,#123636,#123637,#123638,#123639,#123640),.UNSPECIFIED.,.F.,.F.,
(4,2,2,2,2,2,2,2,2,4),(0.426115006982538,0.452619111505283,0.479224276888074,
0.492480316918045,0.51947355541356,0.546429257856091,0.573453669608358,
0.600249948544724,0.626767102937182,0.63918392315697),.UNSPECIFIED.);
#2863=B_SPLINE_CURVE_WITH_KNOTS('',3,(#123644,#123645,#123646,#123647,#123648,
#123649,#123650,#123651,#123652,#123653,#123654,#123655,#123656,#123657,
#123658,#123659,#123660,#123661,#123662,#123663,#123664,#123665,#123666,
#123667,#123668,#123669,#123670,#123671,#123672,#123673,#123674,#123675,
#123676,#123677,#123678,#123679),.UNSPECIFIED.,.T.,.F.,(4,2,2,2,2,2,2,2,
2,2,2,2,2,2,2,2,2,4),(0.,0.0438004959938472,0.0877618839639682,0.132083039219552,
0.176121014722894,0.219586138844758,0.262771060863382,0.305729705032781,
0.348658957103483,0.391776284984157,0.435171792857276,0.456919677130482,
0.478577335014969,0.522551998360091,0.566354050965616,0.610193917091003,
0.654085372794423,0.694370484526123),.UNSPECIFIED.);
#2864=B_SPLINE_CURVE_WITH_KNOTS('',3,(#123683,#123684,#123685,#123686,#123687,
#123688,#123689,#123690,#123691,#123692,#123693,#123694,#123695,#123696,
#123697,#123698,#123699,#123700,#123701,#123702),.UNSPECIFIED.,.F.,.F.,
(4,2,2,2,2,2,2,2,2,4),(0.157563609058178,0.15782359728517,0.17781025817529,
0.197849116873822,0.217969925178253,0.238143964435893,0.257850129783055,
0.277435616699145,0.296937498491984,0.315195637226173),.UNSPECIFIED.);
#2865=B_SPLINE_CURVE_WITH_KNOTS('',3,(#123706,#123707,#123708,#123709,#123710,
#123711,#123712,#123713,#123714,#123715,#123716,#123717,#123718,#123719,
#123720,#123721,#123722,#123723,#123724,#123725,#123726,#123727,#123728),
 .UNSPECIFIED.,.F.,.F.,(4,3,2,2,2,2,2,2,2,2,4),(0.315195637226173,0.315221189479864,
0.334810208300643,0.354519738182407,0.364371264592903,0.374204660308851,
0.394247715670578,0.414236021170778,0.434007786695688,0.453513973251726,
0.472784798538042),.UNSPECIFIED.);
#2866=B_SPLINE_CURVE_WITH_KNOTS('',3,(#123732,#123733,#123734,#123735,#123736,
#123737,#123738,#123739,#123740,#123741,#123742,#123743,#123744,#123745,
#123746,#123747,#123748,#123749,#123750,#123751,#123752,#123753,#123754,
#123755,#123756,#123757,#123758,#123759,#123760,#123761,#123762,#123763,
#123764,#123765,#123766,#123767,#123768,#123769),.UNSPECIFIED.,.T.,.F.,
(4,2,2,2,2,2,2,2,2,2,2,2,2,2,2,2,2,2,4),(0.,0.0435335379564071,0.0872805418243845,
0.10876424930064,0.130340015627335,0.1747602629752,0.218165610708909,0.261131650700908,
0.3036977785209,0.346142301938299,0.38881760853067,0.431932992538991,0.453649473472543,
0.475314817814312,0.519285676559382,0.562925631864407,0.606429094795108,
0.649431149953087,0.69027309180811),.UNSPECIFIED.);
#2867=B_SPLINE_CURVE_WITH_KNOTS('',3,(#123773,#123774,#123775,#123776,#123777,
#123778,#123779,#123780,#123781,#123782,#123783,#123784,#123785,#123786,
#123787,#123788,#123789,#123790,#123791,#123792,#123793,#123794),
 .UNSPECIFIED.,.F.,.F.,(4,2,2,2,2,2,2,2,2,2,4),(0.155223965039871,0.155362142301834,
0.174603165145324,0.194367025915675,0.204058790757966,0.213773625392455,
0.233696561634035,0.253338083772129,0.272647283209335,0.291791090103793,
0.31047162775744),.UNSPECIFIED.);
#2868=B_SPLINE_CURVE_WITH_KNOTS('',3,(#123798,#123799,#123800,#123801,#123802,
#123803,#123804,#123805,#123806,#123807,#123808,#123809,#123810,#123811,
#123812,#123813,#123814,#123815,#123816,#123817,#123818,#123819,#123820),
 .UNSPECIFIED.,.F.,.F.,(4,3,2,2,2,2,2,2,2,2,4),(0.31047162775744,0.310496225533347,
0.329706636164436,0.349109981103316,0.358849708851866,0.368583376798189,
0.38841786259702,0.408144271063843,0.427594276693172,0.446734179455907,
0.465720190573218),.UNSPECIFIED.);
#2869=B_SPLINE_CURVE_WITH_KNOTS('',3,(#123824,#123825,#123826,#123827,#123828,
#123829,#123830,#123831,#123832,#123833,#123834,#123835,#123836,#123837,
#123838,#123839,#123840,#123841,#123842,#123843,#123844,#123845,#123846,
#123847,#123848,#123849,#123850,#123851,#123852,#123853,#123854,#123855,
#123856,#123857,#123858,#123859),.UNSPECIFIED.,.T.,.F.,(4,2,2,2,2,2,2,2,
2,2,2,2,2,2,2,2,2,4),(0.,0.0586079814967797,0.0874078554054557,0.146201962571134,
0.204435711225752,0.262657544525573,0.320782955246569,0.378780112689523,
0.436715022410588,0.494682759830729,0.552706578295632,0.611539730354419,
0.669983012530477,0.728607350829478,0.787564378993769,0.846487759981544,
0.905061888398866,0.931862013437082),.UNSPECIFIED.);
#2870=B_SPLINE_CURVE_WITH_KNOTS('',3,(#123863,#123864,#123865,#123866,#123867,
#123868,#123869,#123870,#123871,#123872,#123873,#123874,#123875,#123876,
#123877,#123878,#123879,#123880,#123881,#123882,#123883,#123884),
 .UNSPECIFIED.,.F.,.F.,(4,2,2,2,2,2,2,2,2,2,4),(0.139816053457858,0.140268245540218,
0.175242647417502,0.192387726565067,0.227315557315772,0.261878269111605,
0.29643087927095,0.330947507666127,0.365421949126044,0.399880936816061,
0.416635497165623),.UNSPECIFIED.);
#2871=B_SPLINE_CURVE_WITH_KNOTS('',3,(#123888,#123889,#123890,#123891,#123892,
#123893,#123894,#123895,#123896,#123897,#123898,#123899,#123900,#123901,
#123902,#123903,#123904,#123905,#123906,#123907,#123908),.UNSPECIFIED.,
 .F.,.F.,(4,2,2,2,2,3,2,2,2,4),(0.416635497165623,0.434357841681837,0.468856471627119,
0.503897324003799,0.53882431509626,0.553651505064719,0.588736869748285,
0.623903021104051,0.658978159339036,0.693467558522578),.UNSPECIFIED.);
#2872=B_SPLINE_CURVE_WITH_KNOTS('',3,(#123912,#123913,#123914,#123915,#123916,
#123917,#123918,#123919,#123920,#123921,#123922,#123923,#123924,#123925,
#123926,#123927,#123928,#123929,#123930,#123931,#123932,#123933,#123934,
#123935,#123936,#123937,#123938,#123939,#123940,#123941,#123942,#123943,
#123944,#123945,#123946,#123947,#123948,#123949),.UNSPECIFIED.,.T.,.F.,
(4,2,2,2,2,2,2,2,2,2,2,2,2,2,2,2,2,2,4),(0.,0.0507410411059291,0.0756428906135374,
0.101000376964068,0.151385667510921,0.201733650877737,0.251953710970444,
0.302003032346441,0.35194855798103,0.401931246270778,0.452052993923605,
0.477147607318242,0.502251198424077,0.553162007043944,0.603806479049535,
0.6545319614579,0.705395871704498,0.756192455948636,0.804565083083937),
 .UNSPECIFIED.);
#2873=B_SPLINE_CURVE_WITH_KNOTS('',3,(#123953,#123954,#123955,#123956,#123957,
#123958,#123959,#123960,#123961,#123962,#123963,#123964,#123965,#123966,
#123967,#123968,#123969,#123970,#123971,#123972,#123973,#123974),
 .UNSPECIFIED.,.F.,.F.,(4,2,2,2,2,2,2,2,2,2,4),(0.213054244451595,0.215140827835265,
0.242150406659373,0.25538302799454,0.268815218273894,0.295477383870316,
0.322106682092898,0.348669736568472,0.375165012920701,0.401633838738512,
0.426079206306101),.UNSPECIFIED.);
#2874=B_SPLINE_CURVE_WITH_KNOTS('',3,(#123978,#123979,#123980,#123981,#123982,
#123983,#123984,#123985,#123986,#123987,#123988,#123989,#123990,#123991,
#123992,#123993,#123994,#123995,#123996,#123997),.UNSPECIFIED.,.F.,.F.,
(4,2,2,2,2,2,2,2,2,4),(0.426079625809021,0.452645595099671,0.465938337013661,
0.479227879223233,0.506279278725265,0.533249557531349,0.560234630804096,
0.587252678468645,0.614252916234622,0.639133450757696),.UNSPECIFIED.);
#2875=B_SPLINE_CURVE_WITH_KNOTS('',3,(#124001,#124002,#124003,#124004,#124005,
#124006,#124007,#124008,#124009,#124010,#124011,#124012,#124013,#124014,
#124015,#124016,#124017,#124018,#124019,#124020,#124021,#124022,#124023,
#124024,#124025,#124026,#124027,#124028,#124029,#124030,#124031,#124032,
#124033,#124034,#124035,#124036),.UNSPECIFIED.,.T.,.F.,(4,2,2,2,2,2,2,2,
2,2,2,2,2,2,2,2,2,4),(0.,0.0439031127094954,0.065447765592922,0.109902791721661,
0.153561484989613,0.19704719047054,0.240247824587854,0.28320987925128,0.326130003594881,
0.369231772635403,0.412614437139118,0.456180877068987,0.500239656278008,
0.544042664929523,0.587798556171279,0.631569949867552,0.67532475002012,
0.694414801328956),.UNSPECIFIED.);
#2876=B_SPLINE_CURVE_WITH_KNOTS('',3,(#124040,#124041,#124042,#124043,#124044,
#124045,#124046,#124047,#124048,#124049,#124050,#124051,#124052,#124053,
#124054,#124055,#124056,#124057,#124058,#124059,#124060,#124061,#124062,
#124063,#124064),.UNSPECIFIED.,.F.,.F.,(4,2,2,2,2,2,2,2,2,2,3,4),(0.157670270859278,
0.158917049885251,0.178952570765188,0.188772784740277,0.198617965338202,
0.218827169194992,0.238590756353538,0.258240538801305,0.277776837156618,
0.29726705640842,0.315235161822161,0.315256462625511),.UNSPECIFIED.);
#2877=B_SPLINE_CURVE_WITH_KNOTS('',3,(#124068,#124069,#124070,#124071,#124072,
#124073,#124074,#124075,#124076,#124077,#124078,#124079,#124080,#124081,
#124082,#124083,#124084,#124085),.UNSPECIFIED.,.F.,.F.,(4,2,2,2,2,2,2,2,
4),(0.315256462625511,0.334880195493556,0.354636232285665,0.374768960524188,
0.394798226033378,0.414755231257366,0.434683621715996,0.454191919873264,
0.472905432681439),.UNSPECIFIED.);
#2878=B_SPLINE_CURVE_WITH_KNOTS('',3,(#124089,#124090,#124091,#124092,#124093,
#124094,#124095,#124096,#124097,#124098,#124099,#124100,#124101,#124102,
#124103,#124104,#124105,#124106,#124107,#124108,#124109,#124110,#124111,
#124112,#124113,#124114,#124115,#124116,#124117,#124118,#124119,#124120,
#124121,#124122,#124123,#124124,#124125,#124126),.UNSPECIFIED.,.T.,.F.,
(4,2,2,2,2,2,2,2,2,2,2,2,2,2,2,2,2,2,4),(0.,0.0435871080099574,0.0873540036482257,
0.108835854513303,0.153089303041548,0.196450323283551,0.239370816524269,
0.281917126448144,0.324379281818892,0.367100824058561,0.410266027335005,
0.431906304365628,0.453468385800544,0.497254546642128,0.540844614594443,
0.584460030183684,0.626983036772123,0.669548662465944,0.690304813988971),
 .UNSPECIFIED.);
#2879=B_SPLINE_CURVE_WITH_KNOTS('',3,(#124130,#124131,#124132,#124133,#124134,
#124135,#124136,#124137,#124138,#124139,#124140,#124141,#124142,#124143,
#124144,#124145,#124146,#124147,#124148,#124149,#124150,#124151),
 .UNSPECIFIED.,.F.,.F.,(4,2,2,2,2,2,2,2,2,2,4),(0.155277913628404,0.165292665851862,
0.185011545100367,0.19466938884267,0.204340835104207,0.224186417404708,
0.24382080194478,0.263107290942695,0.282241250383083,0.301354342848805,
0.31051158851085),.UNSPECIFIED.);
#2880=B_SPLINE_CURVE_WITH_KNOTS('',3,(#124155,#124156,#124157,#124158,#124159,
#124160,#124161,#124162,#124163,#124164,#124165,#124166,#124167,#124168,
#124169,#124170,#124171,#124172,#124173,#124174),.UNSPECIFIED.,.F.,.F.,
(4,2,2,2,2,2,2,2,2,4),(0.310511631495674,0.329840353193037,0.349688712066573,
0.359376076106975,0.37912670235507,0.398829574981945,0.418273867256278,
0.437404148789155,0.4565385186502,0.465789545124077),.UNSPECIFIED.);
#2881=B_SPLINE_CURVE_WITH_KNOTS('',3,(#124178,#124179,#124180,#124181,#124182,
#124183,#124184,#124185,#124186,#124187,#124188,#124189,#124190,#124191,
#124192,#124193,#124194,#124195,#124196,#124197,#124198,#124199,#124200,
#124201,#124202,#124203,#124204,#124205,#124206,#124207,#124208,#124209,
#124210,#124211,#124212,#124213),.UNSPECIFIED.,.T.,.F.,(4,2,2,2,2,2,2,2,
2,2,2,2,2,2,2,2,2,4),(0.,0.0287048976197577,0.0579909299519489,0.116207370107013,
0.174459798915435,0.232700244737173,0.290833045742682,0.348822778718614,
0.406740374765474,0.46469012417934,0.522704198390246,0.581625693995376,
0.640106014433827,0.698690856835086,0.757547003621423,0.816366942407726,
0.874903135177207,0.931848802228483),.UNSPECIFIED.);
#2882=B_SPLINE_CURVE_WITH_KNOTS('',3,(#124217,#124218,#124219,#124220,#124221,
#124222,#124223,#124224,#124225,#124226,#124227,#124228,#124229,#124230,
#124231,#124232,#124233,#124234,#124235,#124236,#124237,#124238),
 .UNSPECIFIED.,.F.,.F.,(4,2,2,2,2,2,2,2,2,2,4),(0.276840898672623,0.279628334212692,
0.296758473080632,0.314164071599323,0.348729292078658,0.38330329595071,
0.41786548372865,0.452383753230674,0.486851783291951,0.521300673093516,
0.55360078593496),.UNSPECIFIED.);
#2883=B_SPLINE_CURVE_WITH_KNOTS('',3,(#124242,#124243,#124244,#124245,#124246,
#124247,#124248,#124249,#124250,#124251,#124252,#124253,#124254,#124255,
#124256,#124257,#124258,#124259,#124260,#124261,#124262),.UNSPECIFIED.,
 .F.,.F.,(4,3,2,2,2,2,2,2,2,4),(0.55360078593496,0.55363816449267,0.588131209987963,
0.623227027140864,0.658175347111053,0.693169329612643,0.728259424581328,
0.763330988935877,0.798299689355572,0.830479063165293),.UNSPECIFIED.);
#2884=B_SPLINE_CURVE_WITH_KNOTS('',3,(#124266,#124267,#124268,#124269,#124270,
#124271,#124272,#124273,#124274,#124275,#124276,#124277,#124278,#124279,
#124280,#124281,#124282,#124283,#124284,#124285,#124286,#124287,#124288,
#124289,#124290,#124291,#124292,#124293,#124294,#124295,#124296,#124297,
#124298,#124299,#124300,#124301,#124302,#124303),.UNSPECIFIED.,.T.,.F.,
(4,2,2,2,2,2,2,2,2,2,2,2,2,2,2,2,2,2,4),(0.,0.0510429338667782,0.076397917131576,
0.126793391862614,0.177157527703175,0.227388740140887,0.277437957066358,
0.327373639274449,0.377342839915421,0.427453608676605,0.452546874856284,
0.477649776776157,0.528631836304232,0.579291425945068,0.6299594819957,0.68071679986447,
0.731420932397828,0.78205413142032,0.80458996698247),.UNSPECIFIED.);
#2885=B_SPLINE_CURVE_WITH_KNOTS('',3,(#124307,#124308,#124309,#124310,#124311,
#124312,#124313,#124314,#124315,#124316,#124317,#124318,#124319,#124320,
#124321,#124322,#124323,#124324,#124325,#124326,#124327,#124328,#124329,
#124330,#124331),.UNSPECIFIED.,.F.,.F.,(4,2,2,2,2,2,2,2,2,2,3,4),(0.213098728070289,
0.228843062715118,0.242103271971766,0.255533998221794,0.282201549216426,
0.308839793496936,0.335409925514743,0.361906495950229,0.3883705405282,0.414865169494334,
0.42609769849922,0.426118424467579),.UNSPECIFIED.);
#2886=B_SPLINE_CURVE_WITH_KNOTS('',3,(#124335,#124336,#124337,#124338,#124339,
#124340,#124341,#124342,#124343,#124344,#124345,#124346,#124347,#124348,
#124349,#124350,#124351,#124352,#124353,#124354),.UNSPECIFIED.,.F.,.F.,
(4,2,2,2,2,2,2,2,2,4),(0.426118424467579,0.452690856909965,0.465988190892994,
0.493083182685766,0.520061578949307,0.547013033000589,0.573973789465176,
0.600927728790317,0.627889696575217,0.639196426569509),.UNSPECIFIED.);
#2887=B_SPLINE_CURVE_WITH_KNOTS('',3,(#124358,#124359,#124360,#124361,#124362,
#124363,#124364,#124365,#124366,#124367,#124368,#124369,#124370,#124371,
#124372,#124373,#124374,#124375,#124376,#124377,#124378,#124379,#124380,
#124381,#124382,#124383,#124384,#124385,#124386,#124387,#124388,#124389,
#124390,#124391,#124392,#124393),.UNSPECIFIED.,.T.,.F.,(4,2,2,2,2,2,2,2,
2,2,2,2,2,2,2,2,2,4),(0.,0.0439191898210743,0.0654694974190781,0.109907007449981,
0.153463834912755,0.196769506044468,0.239810145530631,0.282730920257517,
0.325757072673901,0.369045496294376,0.412571123326874,0.45662283646866,
0.500442890777996,0.544288582176787,0.587775210315516,0.63078465200412,
0.674618447999147,0.694439725374071),.UNSPECIFIED.);
#2888=B_SPLINE_CURVE_WITH_KNOTS('',3,(#124397,#124398,#124399,#124400,#124401,
#124402,#124403,#124404,#124405,#124406,#124407,#124408,#124409,#124410,
#124411,#124412,#124413,#124414,#124415,#124416,#124417,#124418,#124419,
#124420,#124421),.UNSPECIFIED.,.F.,.F.,(4,2,2,2,2,2,2,2,2,2,3,4),(0.157675809345969,
0.158611419670666,0.178629032205577,0.188431328274174,0.208556988599352,
0.228485012656645,0.248116540522748,0.267643763056576,0.287139442297717,
0.306696505525884,0.315254903066365,0.315278867342973),.UNSPECIFIED.);
#2889=B_SPLINE_CURVE_WITH_KNOTS('',3,(#124425,#124426,#124427,#124428,#124429,
#124430,#124431,#124432,#124433,#124434,#124435,#124436,#124437,#124438,
#124439,#124440,#124441,#124442),.UNSPECIFIED.,.F.,.F.,(4,2,2,2,2,2,2,2,
4),(0.315278867342973,0.334979822168361,0.355060989011452,0.375072649078575,
0.395061815886258,0.414829311844664,0.43433498391426,0.453877529419646,
0.472930712412335),.UNSPECIFIED.);
#2890=B_SPLINE_CURVE_WITH_KNOTS('',3,(#124446,#124447,#124448,#124449,#124450,
#124451,#124452,#124453,#124454,#124455,#124456,#124457,#124458,#124459,
#124460,#124461,#124462,#124463,#124464,#124465,#124466,#124467,#124468,
#124469,#124470,#124471,#124472,#124473,#124474,#124475,#124476,#124477,
#124478,#124479,#124480,#124481,#124482,#124483),.UNSPECIFIED.,.T.,.F.,
(4,2,2,2,2,2,2,2,2,2,2,2,2,2,2,2,2,2,4),(0.,0.0437215782121247,0.0651830243893058,
0.0867281067522949,0.131089093155095,0.174465295391611,0.217398166083778,
0.259950071597516,0.302411478707208,0.345128929837316,0.38829073955286,
0.409975559561997,0.43159220439922,0.475473805177582,0.5190906858709,0.562648790415719,
0.605181447805459,0.647749615983058,0.690381534302931),.UNSPECIFIED.);
#2891=B_SPLINE_CURVE_WITH_KNOTS('',3,(#124487,#124488,#124489,#124490,#124491,
#124492,#124493,#124494,#124495,#124496,#124497,#124498,#124499,#124500,
#124501,#124502,#124503,#124504,#124505,#124506,#124507,#124508,#124509,
#124510,#124511),.UNSPECIFIED.,.F.,.F.,(4,2,2,2,2,2,2,2,2,2,3,4),(0.155271413259303,
0.155351020020443,0.175102755092281,0.184783290700741,0.194482425574497,
0.21437504374942,0.2340065060019,0.253298723705622,0.272435688303237,0.291548990163982,
0.31054439799597,0.310545731557595),.UNSPECIFIED.);
#2892=B_SPLINE_CURVE_WITH_KNOTS('',3,(#124515,#124516,#124517,#124518,#124519,
#124520,#124521,#124522,#124523,#124524,#124525,#124526,#124527,#124528,
#124529,#124530,#124531,#124532,#124533,#124534),.UNSPECIFIED.,.F.,.F.,
(4,2,2,2,2,2,2,2,2,4),(0.310545731557595,0.329972473025655,0.339697811404467,
0.349411125640383,0.369206800889191,0.388921424958359,0.408363687262648,
0.427498048467781,0.446632485253342,0.465815811255273),.UNSPECIFIED.);
#2893=B_SPLINE_CURVE_WITH_KNOTS('',3,(#124538,#124539,#124540,#124541,#124542,
#124543,#124544,#124545,#124546,#124547,#124548,#124549,#124550,#124551,
#124552,#124553,#124554,#124555,#124556,#124557,#124558,#124559,#124560,
#124561,#124562,#124563,#124564,#124565,#124566,#124567,#124568,#124569,
#124570,#124571,#124572,#124573),.UNSPECIFIED.,.T.,.F.,(4,2,2,2,2,2,2,2,
2,2,2,2,2,2,2,2,2,4),(0.,0.0292857032011709,0.0875046671306897,0.145761743962781,
0.204003525537326,0.262132469964737,0.320116278552626,0.378029949376738,
0.435978624454139,0.493992508043103,0.552906912724376,0.611388834361421,
0.669975114270796,0.728816779746512,0.787608935744797,0.846130493044841,
0.904669723525998,0.931860524916837),.UNSPECIFIED.);
#2894=B_SPLINE_CURVE_WITH_KNOTS('',3,(#124577,#124578,#124579,#124580,#124581,
#124582,#124583,#124584,#124585,#124586,#124587,#124588,#124589,#124590,
#124591,#124592,#124593,#124594,#124595,#124596,#124597,#124598),
 .UNSPECIFIED.,.F.,.F.,(4,2,2,2,2,2,2,2,2,2,4),(0.276760272839279,0.279486310257967,
0.296891678680277,0.331458165558293,0.366034485059258,0.400597852950089,
0.43511518918133,0.469581034947741,0.504027951985929,0.538494797944952,
0.553534858849661),.UNSPECIFIED.);
#2895=B_SPLINE_CURVE_WITH_KNOTS('',3,(#124602,#124603,#124604,#124605,#124606,
#124607,#124608,#124609,#124610,#124611,#124612,#124613,#124614,#124615,
#124616,#124617,#124618,#124619,#124620,#124621,#124622,#124623,#124624),
 .UNSPECIFIED.,.F.,.F.,(4,3,2,2,2,2,2,2,2,2,4),(0.553534858849661,0.553571407556779,
0.57080071510399,0.605899668347728,0.640850429205566,0.675842030038425,
0.710921555264802,0.745979016681533,0.780941869360024,0.815919166540209,
0.830331680396058),.UNSPECIFIED.);
#2896=B_SPLINE_CURVE_WITH_KNOTS('',3,(#124628,#124629,#124630,#124631,#124632,
#124633,#124634,#124635,#124636,#124637,#124638,#124639,#124640,#124641,
#124642,#124643,#124644,#124645,#124646,#124647,#124648,#124649,#124650,
#124651,#124652,#124653,#124654,#124655,#124656,#124657,#124658,#124659,
#124660,#124661,#124662,#124663,#124664,#124665),.UNSPECIFIED.,.T.,.F.,
(4,2,2,2,2,2,2,2,2,2,2,2,2,2,2,2,2,2,4),(0.,0.0248933932359958,0.0502522570920565,
0.100634389368853,0.150969557978298,0.201172913172633,0.251211890868952,
0.301161391274955,0.351160968415509,0.401301682580004,0.42640034086851,
0.451484147713581,0.502328460810631,0.552963491530814,0.603732474844502,
0.654653180071778,0.705482878991501,0.756131972743015,0.804589874132826),
 .UNSPECIFIED.);
#2897=B_SPLINE_CURVE_WITH_KNOTS('',3,(#124669,#124670,#124671,#124672,#124673,
#124674,#124675,#124676,#124677,#124678,#124679,#124680,#124681,#124682,
#124683,#124684,#124685,#124686,#124687,#124688,#124689,#124690,#124691),
 .UNSPECIFIED.,.F.,.F.,(4,2,2,2,2,2,2,2,2,3,4),(0.213062242779274,0.215594286347048,
0.242723114912628,0.26965769329563,0.296277525050163,0.322829978657394,
0.349320058762837,0.375793067010212,0.402307147515523,0.42615612595573,
0.426158064897884),.UNSPECIFIED.);
#2898=B_SPLINE_CURVE_WITH_KNOTS('',3,(#124695,#124696,#124697,#124698,#124699,
#124700,#124701,#124702,#124703,#124704,#124705,#124706,#124707,#124708,
#124709,#124710,#124711,#124712,#124713,#124714),.UNSPECIFIED.,.F.,.F.,
(4,2,2,2,2,2,2,2,2,4),(0.426158064897884,0.439451111668312,0.452721748725907,
0.479742872920943,0.50670905019566,0.533715458489057,0.56076305839436,0.587782693638629,
0.614752016947225,0.639218368735004),.UNSPECIFIED.);
#2899=B_SPLINE_CURVE_WITH_KNOTS('',3,(#124718,#124719,#124720,#124721,#124722,
#124723,#124724,#124725,#124726,#124727,#124728,#124729,#124730,#124731,
#124732,#124733,#124734,#124735,#124736,#124737,#124738,#124739,#124740,
#124741,#124742,#124743,#124744,#124745,#124746,#124747,#124748,#124749,
#124750,#124751,#124752,#124753,#124754,#124755),.UNSPECIFIED.,.T.,.F.,
(4,2,2,2,2,2,2,2,2,2,2,2,2,2,2,2,2,2,4),(0.,0.0439678896202485,0.0655655029275496,
0.110009025062157,0.15338644656328,0.196316281992617,0.238864267606157,
0.281325189401524,0.324046767682901,0.36721469666785,0.388931797762863,
0.410585946819287,0.454527722035373,0.498154390781355,0.54166243443166,
0.584196741622454,0.62676799340196,0.670324587180314,0.690419290830314),
 .UNSPECIFIED.);
#2900=B_SPLINE_CURVE_WITH_KNOTS('',3,(#124759,#124760,#124761,#124762,#124763,
#124764,#124765,#124766,#124767,#124768,#124769,#124770,#124771,#124772,
#124773,#124774,#124775,#124776,#124777,#124778,#124779,#124780,#124781,
#124782,#124783),.UNSPECIFIED.,.F.,.F.,(4,2,2,2,2,2,2,2,2,2,3,4),(0.155303368541285,
0.165953518380685,0.175653526394182,0.185375252576559,0.20530184599077,
0.224787768869467,0.24407598561316,0.263210264313593,0.282324346612549,
0.301563317562167,0.310561428945123,0.310564213819402),.UNSPECIFIED.);
#2901=B_SPLINE_CURVE_WITH_KNOTS('',3,(#124787,#124788,#124789,#124790,#124791,
#124792,#124793,#124794,#124795,#124796,#124797,#124798,#124799,#124800,
#124801,#124802,#124803,#124804,#124805,#124806),.UNSPECIFIED.,.F.,.F.,
(4,2,2,2,2,2,2,2,2,4),(0.310564213819402,0.330488585935209,0.340220314466039,
0.360044613831472,0.379762342175092,0.399195717228921,0.41832915217723,
0.437465757350788,0.456733128657656,0.465864797486408),.UNSPECIFIED.);
#2902=B_SPLINE_CURVE_WITH_KNOTS('',3,(#124810,#124811,#124812,#124813,#124814,
#124815,#124816,#124817,#124818,#124819,#124820,#124821,#124822,#124823,
#124824,#124825,#124826,#124827,#124828,#124829,#124830,#124831,#124832,
#124833,#124834,#124835,#124836,#124837,#124838,#124839,#124840,#124841,
#124842,#124843,#124844,#124845),.UNSPECIFIED.,.T.,.F.,(4,2,2,2,2,2,2,2,
2,2,2,2,2,2,2,2,2,4),(0.,0.0215162851055023,0.0431138208697561,0.0876446091306586,
0.131214824931109,0.174533219411644,0.217580020450594,0.260498958605342,
0.303517942761,0.346798698928251,0.390321256126534,0.434453407875001,0.478306337336134,
0.522117779247078,0.565997578097342,0.60900882863582,0.65281351297531,0.694470762403534),
 .UNSPECIFIED.);
#2903=B_SPLINE_CURVE_WITH_KNOTS('',3,(#124849,#124850,#124851,#124852,#124853,
#124854,#124855,#124856,#124857,#124858,#124859,#124860,#124861,#124862,
#124863,#124864,#124865,#124866,#124867,#124868,#124869,#124870),
 .UNSPECIFIED.,.F.,.F.,(4,2,2,2,2,2,2,2,2,2,4),(0.157596843449002,0.158418367788362,
0.168222589374335,0.178045702719235,0.198211232858027,0.217965980314702,
0.237605523059871,0.2571371745784,0.276632033627272,0.296184226993561,0.315204316067632),
 .UNSPECIFIED.);
#2904=B_SPLINE_CURVE_WITH_KNOTS('',3,(#124874,#124875,#124876,#124877,#124878,
#124879,#124880,#124881,#124882,#124883,#124884,#124885,#124886,#124887,
#124888,#124889,#124890,#124891,#124892,#124893,#124894,#124895,#124896),
 .UNSPECIFIED.,.F.,.F.,(4,3,2,2,2,2,2,2,2,2,4),(0.315204316067632,0.315219848506788,
0.325082339394274,0.33493357406727,0.355013881071206,0.375021647425745,
0.395000614069428,0.41452308079024,0.434037261815992,0.45362137049485,0.47281669195579),
 .UNSPECIFIED.);
#2905=B_SPLINE_CURVE_WITH_KNOTS('',3,(#128198,#128199,#128200,#128201,#128202,
#128203,#128204,#128205,#128206,#128207,#128208,#128209,#128210,#128211,
#128212,#128213,#128214,#128215,#128216,#128217,#128218,#128219),
 .UNSPECIFIED.,.F.,.F.,(4,2,2,2,2,2,2,2,2,2,4),(0.276798234884123,0.279451999398466,
0.314379791973188,0.348934706381492,0.383475726766096,0.417982346714956,
0.45245551940928,0.486923657573857,0.521413018577935,0.537430969346281,
0.553574548070559),.UNSPECIFIED.);
#2906=B_SPLINE_CURVE_WITH_KNOTS('',3,(#128223,#128224,#128225,#128226,#128227,
#128228,#128229,#128230,#128231,#128232,#128233,#128234,#128235,#128236,
#128237,#128238,#128239,#128240,#128241,#128242),.UNSPECIFIED.,.F.,.F.,
(4,2,2,2,2,2,2,2,2,4),(0.553575400065736,0.58855639024539,0.623472209566331,
0.658530105742964,0.693733478557596,0.728894593312329,0.763880944627597,
0.798792653463988,0.815885151458029,0.830372782954682),.UNSPECIFIED.);
#2907=B_SPLINE_CURVE_WITH_KNOTS('',3,(#128246,#128247,#128248,#128249,#128250,
#128251,#128252,#128253,#128254,#128255,#128256,#128257,#128258,#128259,
#128260,#128261,#128262,#128263,#128264,#128265,#128266,#128267,#128268,
#128269,#128270,#128271,#128272,#128273,#128274,#128275,#128276,#128277,
#128278,#128279,#128280,#128281,#128282,#128283),.UNSPECIFIED.,.T.,.F.,
(4,2,2,2,2,2,2,2,2,2,2,2,2,2,2,2,2,2,4),(0.,0.0587946924940988,0.117017440565929,
0.175220198207046,0.233326761370365,0.29131841207302,0.349265888456903,
0.40725387524115,0.436245732062709,0.465239839112465,0.523939722158812,
0.582356104658916,0.641055278220904,0.700106923889623,0.75907025217679,
0.817630646713495,0.876070888006275,0.903750502884322,0.931728974146718),
 .UNSPECIFIED.);
#2927=SHAPE_REPRESENTATION_RELATIONSHIP('SRR','None',#130949,#2935);
#2935=ADVANCED_BREP_SHAPE_REPRESENTATION('',(#2949),#130909);
#2943=STYLED_ITEM('',(#130991),#2949);
#2949=MANIFOLD_SOLID_BREP('Body1',#45459);
#3646=PLANE('',#50926);
#3647=PLANE('',#50927);
#3648=PLANE('',#50928);
#3649=PLANE('',#50929);
#3650=PLANE('',#50930);
#3651=PLANE('',#50931);
#3652=PLANE('',#50932);
#3653=PLANE('',#50934);
#3654=PLANE('',#50935);
#3655=PLANE('',#50936);
#3656=PLANE('',#50937);
#3657=PLANE('',#50938);
#3658=PLANE('',#50939);
#3659=PLANE('',#50940);
#3660=PLANE('',#50941);
#3661=PLANE('',#50942);
#3662=PLANE('',#50943);
#3663=PLANE('',#50944);
#3664=PLANE('',#50945);
#3665=PLANE('',#50946);
#3666=PLANE('',#50947);
#3667=PLANE('',#50948);
#3668=PLANE('',#50949);
#3669=PLANE('',#50950);
#3670=PLANE('',#50951);
#3671=PLANE('',#50952);
#3672=PLANE('',#50953);
#3673=PLANE('',#50954);
#3674=PLANE('',#50955);
#3675=PLANE('',#50956);
#3676=PLANE('',#50957);
#3677=PLANE('',#50958);
#3678=PLANE('',#50959);
#3679=PLANE('',#50960);
#3680=PLANE('',#50961);
#3681=PLANE('',#50962);
#3682=PLANE('',#50963);
#3683=PLANE('',#50964);
#3684=PLANE('',#50965);
#3685=PLANE('',#50966);
#3686=PLANE('',#50967);
#3687=PLANE('',#50968);
#3688=PLANE('',#50969);
#3689=PLANE('',#50970);
#3690=PLANE('',#50971);
#3691=PLANE('',#50972);
#3692=PLANE('',#50973);
#3693=PLANE('',#50974);
#3694=PLANE('',#50975);
#3695=PLANE('',#50976);
#3696=PLANE('',#50977);
#3697=PLANE('',#50978);
#3698=PLANE('',#50979);
#3699=PLANE('',#50980);
#3700=PLANE('',#50981);
#3701=PLANE('',#50982);
#3702=PLANE('',#50983);
#3703=PLANE('',#50984);
#3704=PLANE('',#50985);
#3705=PLANE('',#50986);
#3706=PLANE('',#50987);
#3707=PLANE('',#50988);
#3708=PLANE('',#50989);
#3709=PLANE('',#50990);
#3710=PLANE('',#50991);
#3711=PLANE('',#50992);
#3712=PLANE('',#50993);
#3713=PLANE('',#50994);
#3714=PLANE('',#50995);
#3715=PLANE('',#50996);
#3716=PLANE('',#50997);
#3717=PLANE('',#50998);
#3718=PLANE('',#50999);
#3719=PLANE('',#51000);
#3720=PLANE('',#51001);
#3721=PLANE('',#51002);
#3722=PLANE('',#51003);
#3723=PLANE('',#51004);
#3724=PLANE('',#51005);
#3725=PLANE('',#51006);
#3726=PLANE('',#51007);
#3727=PLANE('',#51008);
#3728=PLANE('',#51009);
#3729=PLANE('',#51010);
#3730=PLANE('',#51011);
#3731=PLANE('',#51012);
#3732=PLANE('',#51013);
#3733=PLANE('',#51014);
#3734=PLANE('',#51015);
#3735=PLANE('',#51016);
#3736=PLANE('',#51017);
#3737=PLANE('',#51018);
#3738=PLANE('',#51019);
#3739=PLANE('',#51020);
#3740=PLANE('',#51021);
#3741=PLANE('',#51022);
#3742=PLANE('',#51023);
#3743=PLANE('',#51024);
#3744=PLANE('',#51025);
#3745=PLANE('',#51026);
#3746=PLANE('',#51027);
#3747=PLANE('',#51028);
#3748=PLANE('',#51029);
#3749=PLANE('',#51030);
#3750=PLANE('',#51031);
#3751=PLANE('',#51032);
#3752=PLANE('',#51033);
#3753=PLANE('',#51034);
#3754=PLANE('',#51035);
#3755=PLANE('',#51036);
#3756=PLANE('',#51037);
#3757=PLANE('',#51038);
#3758=PLANE('',#51039);
#3759=PLANE('',#51040);
#3760=PLANE('',#51041);
#3761=PLANE('',#51042);
#3762=PLANE('',#51043);
#3763=PLANE('',#51044);
#3764=PLANE('',#51045);
#3765=PLANE('',#51046);
#3766=PLANE('',#51047);
#3767=PLANE('',#51048);
#3768=PLANE('',#51049);
#3769=PLANE('',#51050);
#3770=PLANE('',#51051);
#3771=PLANE('',#51052);
#3772=PLANE('',#51053);
#3773=PLANE('',#51054);
#3774=PLANE('',#51055);
#3775=PLANE('',#51056);
#3776=PLANE('',#51057);
#3777=PLANE('',#51058);
#3778=PLANE('',#51059);
#3779=PLANE('',#51060);
#3780=PLANE('',#51061);
#3781=PLANE('',#51062);
#3782=PLANE('',#51063);
#3783=PLANE('',#51064);
#3784=PLANE('',#51065);
#3785=PLANE('',#51066);
#3786=PLANE('',#51067);
#3787=PLANE('',#51068);
#3788=PLANE('',#51069);
#3789=PLANE('',#51070);
#3790=PLANE('',#51071);
#3791=PLANE('',#51072);
#3792=PLANE('',#51073);
#3793=PLANE('',#51074);
#3794=PLANE('',#51075);
#3795=PLANE('',#51076);
#3796=PLANE('',#51077);
#3797=PLANE('',#51078);
#3798=PLANE('',#51079);
#3799=PLANE('',#51080);
#3800=PLANE('',#51081);
#3801=PLANE('',#51082);
#3802=PLANE('',#51083);
#3803=PLANE('',#51084);
#3804=PLANE('',#51085);
#3805=PLANE('',#51086);
#3806=PLANE('',#51087);
#3807=PLANE('',#51088);
#3808=PLANE('',#51089);
#3809=PLANE('',#51090);
#3810=PLANE('',#51091);
#3811=PLANE('',#51092);
#3812=PLANE('',#51093);
#3813=PLANE('',#51094);
#3814=PLANE('',#51095);
#3815=PLANE('',#51096);
#3816=PLANE('',#51097);
#3817=PLANE('',#51098);
#3818=PLANE('',#51099);
#3819=PLANE('',#51100);
#3820=PLANE('',#51101);
#3821=PLANE('',#51102);
#3822=PLANE('',#51103);
#3823=PLANE('',#51104);
#3824=PLANE('',#51105);
#3825=PLANE('',#51106);
#3826=PLANE('',#51107);
#3827=PLANE('',#51108);
#3828=PLANE('',#51109);
#3829=PLANE('',#51110);
#3830=PLANE('',#51111);
#3831=PLANE('',#51112);
#3832=PLANE('',#51113);
#3833=PLANE('',#51114);
#3834=PLANE('',#51115);
#3835=PLANE('',#51116);
#3836=PLANE('',#51117);
#3837=PLANE('',#51118);
#3838=PLANE('',#51119);
#3839=PLANE('',#51120);
#3840=PLANE('',#51121);
#3841=PLANE('',#51122);
#3842=PLANE('',#51123);
#3843=PLANE('',#51124);
#3844=PLANE('',#51125);
#3845=PLANE('',#51126);
#3846=PLANE('',#51127);
#3847=PLANE('',#51128);
#3848=PLANE('',#51129);
#3849=PLANE('',#51130);
#3850=PLANE('',#51131);
#3851=PLANE('',#51132);
#3852=PLANE('',#51133);
#3853=PLANE('',#51134);
#3854=PLANE('',#51135);
#3855=PLANE('',#51136);
#3856=PLANE('',#51137);
#3857=PLANE('',#51138);
#3858=PLANE('',#51139);
#3859=PLANE('',#51140);
#3860=PLANE('',#51141);
#3861=PLANE('',#51142);
#3862=PLANE('',#51143);
#3863=PLANE('',#51144);
#3864=PLANE('',#51145);
#3865=PLANE('',#51146);
#3866=PLANE('',#51147);
#3867=PLANE('',#51148);
#3868=PLANE('',#51149);
#3869=PLANE('',#51150);
#3870=PLANE('',#51151);
#3871=PLANE('',#51152);
#3872=PLANE('',#51153);
#3873=PLANE('',#51154);
#3874=PLANE('',#51155);
#3875=PLANE('',#51156);
#3876=PLANE('',#51157);
#3877=PLANE('',#51158);
#3878=PLANE('',#51159);
#3879=PLANE('',#51160);
#3880=PLANE('',#51161);
#3881=PLANE('',#51162);
#3882=PLANE('',#51163);
#3883=PLANE('',#51164);
#3884=PLANE('',#51165);
#3885=PLANE('',#51166);
#3886=PLANE('',#51167);
#3887=PLANE('',#51168);
#3888=PLANE('',#51169);
#3889=PLANE('',#51170);
#3890=PLANE('',#51171);
#3891=PLANE('',#51172);
#3892=PLANE('',#51173);
#3893=PLANE('',#51174);
#3894=PLANE('',#51175);
#3895=PLANE('',#51176);
#3896=PLANE('',#51177);
#3897=PLANE('',#51178);
#3898=PLANE('',#51179);
#3899=PLANE('',#51180);
#3900=PLANE('',#51181);
#3901=PLANE('',#51182);
#3902=PLANE('',#51183);
#3903=PLANE('',#51184);
#3904=PLANE('',#51185);
#3905=PLANE('',#51186);
#3906=PLANE('',#51187);
#3907=PLANE('',#51188);
#3908=PLANE('',#51189);
#3909=PLANE('',#51190);
#3910=PLANE('',#51191);
#3911=PLANE('',#51192);
#3912=PLANE('',#51193);
#3913=PLANE('',#51194);
#3914=PLANE('',#51195);
#3915=PLANE('',#51196);
#3916=PLANE('',#51197);
#3917=PLANE('',#51198);
#3918=PLANE('',#51199);
#3919=PLANE('',#51200);
#3920=PLANE('',#51201);
#3921=PLANE('',#51202);
#3922=PLANE('',#51203);
#3923=PLANE('',#51204);
#3924=PLANE('',#51205);
#3925=PLANE('',#51206);
#3926=PLANE('',#51207);
#3927=PLANE('',#51208);
#3928=PLANE('',#51209);
#3929=PLANE('',#51210);
#3930=PLANE('',#51211);
#3931=PLANE('',#51212);
#3932=PLANE('',#51213);
#3933=PLANE('',#51214);
#3934=PLANE('',#51215);
#3935=PLANE('',#51216);
#3936=PLANE('',#51217);
#3937=PLANE('',#51218);
#3938=PLANE('',#51219);
#3939=PLANE('',#51220);
#3940=PLANE('',#51221);
#3941=PLANE('',#51222);
#3942=PLANE('',#51223);
#3943=PLANE('',#51224);
#3944=PLANE('',#51225);
#3945=PLANE('',#51226);
#3946=PLANE('',#51227);
#3947=PLANE('',#51228);
#3948=PLANE('',#51229);
#3949=PLANE('',#51230);
#3950=PLANE('',#51231);
#3951=PLANE('',#51232);
#3952=PLANE('',#51233);
#3953=PLANE('',#51234);
#3954=PLANE('',#51235);
#3955=PLANE('',#51236);
#3956=PLANE('',#51237);
#3957=PLANE('',#51238);
#3958=PLANE('',#51239);
#3959=PLANE('',#51240);
#3960=PLANE('',#51241);
#3961=PLANE('',#51242);
#3962=PLANE('',#51243);
#3963=PLANE('',#51244);
#3964=PLANE('',#51245);
#3965=PLANE('',#51246);
#3966=PLANE('',#51247);
#3967=PLANE('',#51248);
#3968=PLANE('',#51249);
#3969=PLANE('',#51250);
#3970=PLANE('',#51251);
#3971=PLANE('',#51252);
#3972=PLANE('',#51253);
#3973=PLANE('',#51254);
#3974=PLANE('',#51255);
#3975=PLANE('',#51256);
#3976=PLANE('',#51257);
#3977=PLANE('',#51258);
#3978=PLANE('',#51259);
#3979=PLANE('',#51260);
#3980=PLANE('',#51261);
#3981=PLANE('',#51262);
#3982=PLANE('',#51263);
#3983=PLANE('',#51264);
#3984=PLANE('',#51265);
#3985=PLANE('',#51266);
#3986=PLANE('',#51267);
#3987=PLANE('',#51268);
#3988=PLANE('',#51269);
#3989=PLANE('',#51270);
#3990=PLANE('',#51271);
#3991=PLANE('',#51272);
#3992=PLANE('',#51273);
#3993=PLANE('',#51274);
#3994=PLANE('',#51275);
#3995=PLANE('',#51276);
#3996=PLANE('',#51277);
#3997=PLANE('',#51278);
#3998=PLANE('',#51279);
#3999=PLANE('',#51280);
#4000=PLANE('',#51281);
#4001=PLANE('',#51282);
#4002=PLANE('',#51283);
#4003=PLANE('',#51284);
#4004=PLANE('',#51285);
#4005=PLANE('',#51286);
#4006=PLANE('',#51287);
#4007=PLANE('',#51288);
#4008=PLANE('',#51289);
#4009=PLANE('',#51290);
#4010=PLANE('',#51291);
#4011=PLANE('',#51292);
#4012=PLANE('',#51293);
#4013=PLANE('',#51294);
#4014=PLANE('',#51295);
#4015=PLANE('',#51296);
#4016=PLANE('',#51297);
#4017=PLANE('',#51298);
#4018=PLANE('',#51299);
#4019=PLANE('',#51300);
#4020=PLANE('',#51301);
#4021=PLANE('',#51302);
#4022=PLANE('',#51303);
#4023=PLANE('',#51304);
#4024=PLANE('',#51305);
#4025=PLANE('',#51306);
#4026=PLANE('',#51307);
#4027=PLANE('',#51308);
#4028=PLANE('',#51309);
#4029=PLANE('',#51310);
#4030=PLANE('',#51311);
#4031=PLANE('',#51312);
#4032=PLANE('',#51313);
#4033=PLANE('',#51314);
#4034=PLANE('',#51315);
#4035=PLANE('',#51316);
#4036=PLANE('',#51317);
#4037=PLANE('',#51318);
#4038=PLANE('',#51319);
#4039=PLANE('',#51320);
#4040=PLANE('',#51321);
#4041=PLANE('',#51322);
#4042=PLANE('',#51323);
#4043=PLANE('',#51324);
#4044=PLANE('',#51325);
#4045=PLANE('',#51326);
#4046=PLANE('',#51327);
#4047=PLANE('',#51328);
#4048=PLANE('',#51329);
#4049=PLANE('',#51330);
#4050=PLANE('',#51331);
#4051=PLANE('',#51332);
#4052=PLANE('',#51333);
#4053=PLANE('',#51334);
#4054=PLANE('',#51335);
#4055=PLANE('',#51336);
#4056=PLANE('',#51337);
#4057=PLANE('',#51338);
#4058=PLANE('',#51339);
#4059=PLANE('',#51340);
#4060=PLANE('',#51341);
#4061=PLANE('',#51342);
#4062=PLANE('',#51343);
#4063=PLANE('',#51344);
#4064=PLANE('',#51345);
#4065=PLANE('',#51346);
#4066=PLANE('',#51347);
#4067=PLANE('',#51348);
#4068=PLANE('',#51349);
#4069=PLANE('',#51350);
#4070=PLANE('',#51351);
#4071=PLANE('',#51352);
#4072=PLANE('',#51353);
#4073=PLANE('',#51354);
#4074=PLANE('',#51355);
#4075=PLANE('',#51356);
#4076=PLANE('',#51357);
#4077=PLANE('',#51358);
#4078=PLANE('',#51359);
#4079=PLANE('',#51360);
#4080=PLANE('',#51361);
#4081=PLANE('',#51362);
#4082=PLANE('',#51363);
#4083=PLANE('',#51364);
#4084=PLANE('',#51365);
#4085=PLANE('',#51366);
#4086=PLANE('',#51367);
#4087=PLANE('',#51368);
#4088=PLANE('',#51369);
#4089=PLANE('',#51370);
#4090=PLANE('',#51371);
#4091=PLANE('',#51372);
#4092=PLANE('',#51373);
#4093=PLANE('',#51374);
#4094=PLANE('',#51375);
#4095=PLANE('',#51376);
#4096=PLANE('',#51377);
#4097=PLANE('',#51378);
#4098=PLANE('',#51379);
#4099=PLANE('',#51380);
#4100=PLANE('',#51381);
#4101=PLANE('',#51382);
#4102=PLANE('',#51383);
#4103=PLANE('',#51384);
#4104=PLANE('',#51385);
#4105=PLANE('',#51386);
#4106=PLANE('',#51387);
#4107=PLANE('',#51388);
#4108=PLANE('',#51389);
#4109=PLANE('',#51390);
#4110=PLANE('',#51391);
#4111=PLANE('',#51392);
#4112=PLANE('',#51393);
#4113=PLANE('',#51394);
#4114=PLANE('',#51395);
#4115=PLANE('',#51396);
#4116=PLANE('',#51397);
#4117=PLANE('',#51398);
#4118=PLANE('',#51399);
#4119=PLANE('',#51400);
#4120=PLANE('',#51401);
#4121=PLANE('',#51402);
#4122=PLANE('',#51403);
#4123=PLANE('',#51404);
#4124=PLANE('',#51405);
#4125=PLANE('',#51406);
#4126=PLANE('',#51407);
#4127=PLANE('',#51408);
#4128=PLANE('',#51409);
#4129=PLANE('',#51410);
#4130=PLANE('',#51411);
#4131=PLANE('',#51412);
#4132=PLANE('',#51413);
#4133=PLANE('',#51414);
#4134=PLANE('',#51415);
#4135=PLANE('',#51416);
#4136=PLANE('',#51417);
#4137=PLANE('',#51418);
#4138=PLANE('',#51419);
#4139=PLANE('',#51420);
#4140=PLANE('',#51421);
#4141=PLANE('',#51422);
#4142=PLANE('',#51423);
#4143=PLANE('',#51424);
#4144=PLANE('',#51425);
#4145=PLANE('',#51426);
#4146=PLANE('',#51427);
#4147=PLANE('',#51428);
#4148=PLANE('',#51429);
#4149=PLANE('',#51430);
#4150=PLANE('',#51431);
#4151=PLANE('',#51432);
#4152=PLANE('',#51433);
#4153=PLANE('',#51434);
#4154=PLANE('',#51435);
#4155=PLANE('',#51436);
#4156=PLANE('',#51437);
#4157=PLANE('',#51438);
#4158=PLANE('',#51439);
#4159=PLANE('',#51440);
#4160=PLANE('',#51441);
#4161=PLANE('',#51442);
#4162=PLANE('',#51443);
#4163=PLANE('',#51444);
#4164=PLANE('',#51445);
#4165=PLANE('',#51446);
#4166=PLANE('',#51447);
#4167=PLANE('',#51448);
#4168=PLANE('',#51449);
#4169=PLANE('',#51450);
#4170=PLANE('',#51451);
#4171=PLANE('',#51452);
#4172=PLANE('',#51453);
#4173=PLANE('',#51454);
#4174=PLANE('',#51455);
#4175=PLANE('',#51456);
#4176=PLANE('',#51457);
#4177=PLANE('',#51458);
#4178=PLANE('',#51459);
#4179=PLANE('',#51460);
#4180=PLANE('',#51461);
#4181=PLANE('',#51462);
#4182=PLANE('',#51463);
#4183=PLANE('',#51464);
#4184=PLANE('',#51465);
#4185=PLANE('',#51466);
#4186=PLANE('',#51467);
#4187=PLANE('',#51468);
#4188=PLANE('',#51469);
#4189=PLANE('',#51470);
#4190=PLANE('',#51471);
#4191=PLANE('',#51472);
#4192=PLANE('',#51473);
#4193=PLANE('',#51474);
#4194=PLANE('',#51475);
#4195=PLANE('',#51476);
#4196=PLANE('',#51477);
#4197=PLANE('',#51478);
#4198=PLANE('',#51479);
#4199=PLANE('',#51480);
#4200=PLANE('',#51481);
#4201=PLANE('',#51482);
#4202=PLANE('',#51483);
#4203=PLANE('',#51484);
#4204=PLANE('',#51485);
#4205=PLANE('',#51486);
#4206=PLANE('',#51487);
#4207=PLANE('',#51488);
#4208=PLANE('',#51489);
#4209=PLANE('',#51490);
#4210=PLANE('',#51491);
#4211=PLANE('',#51492);
#4212=PLANE('',#51493);
#4213=PLANE('',#51494);
#4214=PLANE('',#51495);
#4215=PLANE('',#51496);
#4216=PLANE('',#51497);
#4217=PLANE('',#51498);
#4218=PLANE('',#51499);
#4219=PLANE('',#51500);
#4220=PLANE('',#51501);
#4221=PLANE('',#51502);
#4222=PLANE('',#51503);
#4223=PLANE('',#51504);
#4224=PLANE('',#51505);
#4225=PLANE('',#51506);
#4226=PLANE('',#51507);
#4227=PLANE('',#51508);
#4228=PLANE('',#51509);
#4229=PLANE('',#51510);
#4230=PLANE('',#51511);
#4231=PLANE('',#51512);
#4232=PLANE('',#51513);
#4233=PLANE('',#51514);
#4234=PLANE('',#51515);
#4235=PLANE('',#51516);
#4236=PLANE('',#51517);
#4237=PLANE('',#51518);
#4238=PLANE('',#51519);
#4239=PLANE('',#51520);
#4240=PLANE('',#51521);
#4241=PLANE('',#51522);
#4242=PLANE('',#51523);
#4243=PLANE('',#51524);
#4244=PLANE('',#51525);
#4245=PLANE('',#51526);
#4246=PLANE('',#51527);
#4247=PLANE('',#51528);
#4248=PLANE('',#51529);
#4249=PLANE('',#51530);
#4250=PLANE('',#51531);
#4251=PLANE('',#51532);
#4252=PLANE('',#51533);
#4253=PLANE('',#51534);
#4254=PLANE('',#51535);
#4255=PLANE('',#51536);
#4256=PLANE('',#51537);
#4257=PLANE('',#51538);
#4258=PLANE('',#51539);
#4259=PLANE('',#51540);
#4260=PLANE('',#51541);
#4261=PLANE('',#51542);
#4262=PLANE('',#51543);
#4263=PLANE('',#51544);
#4264=PLANE('',#51545);
#4265=PLANE('',#51546);
#4266=PLANE('',#51547);
#4267=PLANE('',#51548);
#4268=PLANE('',#51549);
#4269=PLANE('',#51550);
#4270=PLANE('',#51551);
#4271=PLANE('',#51552);
#4272=PLANE('',#51553);
#4273=PLANE('',#51554);
#4274=PLANE('',#51555);
#4275=PLANE('',#51556);
#4276=PLANE('',#51557);
#4277=PLANE('',#51558);
#4278=PLANE('',#51559);
#4279=PLANE('',#51560);
#4280=PLANE('',#51561);
#4281=PLANE('',#51562);
#4282=PLANE('',#51563);
#4283=PLANE('',#51564);
#4284=PLANE('',#51565);
#4285=PLANE('',#51566);
#4286=PLANE('',#51567);
#4287=PLANE('',#51568);
#4288=PLANE('',#51569);
#4289=PLANE('',#51570);
#4290=PLANE('',#51571);
#4291=PLANE('',#51572);
#4292=PLANE('',#51573);
#4293=PLANE('',#51574);
#4294=PLANE('',#51575);
#4295=PLANE('',#51576);
#4296=PLANE('',#51577);
#4297=PLANE('',#51578);
#4298=PLANE('',#51579);
#4299=PLANE('',#51580);
#4300=PLANE('',#51581);
#4301=PLANE('',#51582);
#4302=PLANE('',#51583);
#4303=PLANE('',#51584);
#4304=PLANE('',#51585);
#4305=PLANE('',#51586);
#4306=PLANE('',#51587);
#4307=PLANE('',#51588);
#4308=PLANE('',#51589);
#4309=PLANE('',#51590);
#4310=PLANE('',#51591);
#4311=PLANE('',#51592);
#5302=LINE('',#110381,#7076);
#5303=LINE('',#110447,#7077);
#5304=LINE('',#110471,#7078);
#5305=LINE('',#110536,#7079);
#5306=LINE('',#110563,#7080);
#5307=LINE('',#110631,#7081);
#5308=LINE('',#110655,#7082);
#5309=LINE('',#110720,#7083);
#5310=LINE('',#110744,#7084);
#5311=LINE('',#110810,#7085);
#5312=LINE('',#110832,#7086);
#5313=LINE('',#110897,#7087);
#5314=LINE('',#110924,#7088);
#5315=LINE('',#110989,#7089);
#5316=LINE('',#111016,#7090);
#5317=LINE('',#111084,#7091);
#5318=LINE('',#111108,#7092);
#5319=LINE('',#111169,#7093);
#5320=LINE('',#111194,#7094);
#5321=LINE('',#111259,#7095);
#5322=LINE('',#111286,#7096);
#5323=LINE('',#111351,#7097);
#5324=LINE('',#111378,#7098);
#5325=LINE('',#111443,#7099);
#5326=LINE('',#111467,#7100);
#5327=LINE('',#111531,#7101);
#5328=LINE('',#111555,#7102);
#5329=LINE('',#111623,#7103);
#5330=LINE('',#111647,#7104);
#5331=LINE('',#111715,#7105);
#5332=LINE('',#111739,#7106);
#5333=LINE('',#111802,#7107);
#5334=LINE('',#111885,#7108);
#5335=LINE('',#111949,#7109);
#5336=LINE('',#111973,#7110);
#5337=LINE('',#112038,#7111);
#5338=LINE('',#112065,#7112);
#5339=LINE('',#112128,#7113);
#5340=LINE('',#112153,#7114);
#5341=LINE('',#112218,#7115);
#5342=LINE('',#112242,#7116);
#5343=LINE('',#112308,#7117);
#5344=LINE('',#112332,#7118);
#5345=LINE('',#112397,#7119);
#5346=LINE('',#112424,#7120);
#5347=LINE('',#112488,#7121);
#5348=LINE('',#112510,#7122);
#5349=LINE('',#112573,#7123);
#5350=LINE('',#112600,#7124);
#5351=LINE('',#112666,#7125);
#5352=LINE('',#112690,#7126);
#5353=LINE('',#112755,#7127);
#5354=LINE('',#112779,#7128);
#5355=LINE('',#112842,#7129);
#5356=LINE('',#112866,#7130);
#5357=LINE('',#113040,#7131);
#5358=LINE('',#113067,#7132);
#5359=LINE('',#113133,#7133);
#5360=LINE('',#113157,#7134);
#5361=LINE('',#113222,#7135);
#5362=LINE('',#113246,#7136);
#5363=LINE('',#113307,#7137);
#5364=LINE('',#113384,#7138);
#5365=LINE('',#113447,#7139);
#5366=LINE('',#113523,#7140);
#5367=LINE('',#113588,#7141);
#5368=LINE('',#113612,#7142);
#5369=LINE('',#113677,#7143);
#5370=LINE('',#113701,#7144);
#5371=LINE('',#113764,#7145);
#5372=LINE('',#113841,#7146);
#5373=LINE('',#113902,#7147);
#5374=LINE('',#113982,#7148);
#5375=LINE('',#114047,#7149);
#5376=LINE('',#114124,#7150);
#5377=LINE('',#114187,#7151);
#5378=LINE('',#114265,#7152);
#5379=LINE('',#114330,#7153);
#5380=LINE('',#114407,#7154);
#5381=LINE('',#114466,#7155);
#5382=LINE('',#114548,#7156);
#5383=LINE('',#114613,#7157);
#5384=LINE('',#114692,#7158);
#5385=LINE('',#114755,#7159);
#5386=LINE('',#114832,#7160);
#5387=LINE('',#114897,#7161);
#5388=LINE('',#114976,#7162);
#5389=LINE('',#115037,#7163);
#5390=LINE('',#115117,#7164);
#5391=LINE('',#115182,#7165);
#5392=LINE('',#115264,#7166);
#5393=LINE('',#115328,#7167);
#5394=LINE('',#115405,#7168);
#5395=LINE('',#115473,#7169);
#5396=LINE('',#115554,#7170);
#5397=LINE('',#115613,#7171);
#5398=LINE('',#115697,#7172);
#5399=LINE('',#115762,#7173);
#5400=LINE('',#115841,#7174);
#5401=LINE('',#115902,#7175);
#5402=LINE('',#115984,#7176);
#5403=LINE('',#116049,#7177);
#5404=LINE('',#116128,#7178);
#5405=LINE('',#116187,#7179);
#5406=LINE('',#116271,#7180);
#5407=LINE('',#116336,#7181);
#5408=LINE('',#116420,#7182);
#5409=LINE('',#116481,#7183);
#5410=LINE('',#116565,#7184);
#5411=LINE('',#116630,#7185);
#5412=LINE('',#116714,#7186);
#5413=LINE('',#116773,#7187);
#5414=LINE('',#116859,#7188);
#5415=LINE('',#116920,#7189);
#5416=LINE('',#117006,#7190);
#5417=LINE('',#117068,#7191);
#5418=LINE('',#117151,#7192);
#5419=LINE('',#117216,#7193);
#5420=LINE('',#117298,#7194);
#5421=LINE('',#117361,#7195);
#5422=LINE('',#117443,#7196);
#5423=LINE('',#117504,#7197);
#5424=LINE('',#117590,#7198);
#5425=LINE('',#117658,#7199);
#5426=LINE('',#117739,#7200);
#5427=LINE('',#117802,#7201);
#5428=LINE('',#117886,#7202);
#5429=LINE('',#118058,#7203);
#5430=LINE('',#118142,#7204);
#5431=LINE('',#118204,#7205);
#5432=LINE('',#118287,#7206);
#5433=LINE('',#118350,#7207);
#5434=LINE('',#118436,#7208);
#5435=LINE('',#118502,#7209);
#5436=LINE('',#118583,#7210);
#5437=LINE('',#118753,#7211);
#5438=LINE('',#118837,#7212);
#5439=LINE('',#118899,#7213);
#5440=LINE('',#118980,#7214);
#5441=LINE('',#119048,#7215);
#5442=LINE('',#119129,#7216);
#5443=LINE('',#119195,#7217);
#5444=LINE('',#119253,#7218);
#5445=LINE('',#119549,#7219);
#5446=LINE('',#119631,#7220);
#5447=LINE('',#119692,#7221);
#5448=LINE('',#119778,#7222);
#5449=LINE('',#119841,#7223);
#5450=LINE('',#119927,#7224);
#5451=LINE('',#119988,#7225);
#5452=LINE('',#120070,#7226);
#5453=LINE('',#120133,#7227);
#5454=LINE('',#120217,#7228);
#5455=LINE('',#120280,#7229);
#5456=LINE('',#120362,#7230);
#5457=LINE('',#120430,#7231);
#5458=LINE('',#120511,#7232);
#5459=LINE('',#120575,#7233);
#5460=LINE('',#120654,#7234);
#5461=LINE('',#120719,#7235);
#5462=LINE('',#120801,#7236);
#5463=LINE('',#120864,#7237);
#5464=LINE('',#120944,#7238);
#5465=LINE('',#121012,#7239);
#5466=LINE('',#121091,#7240);
#5467=LINE('',#121150,#7241);
#5468=LINE('',#121228,#7242);
#5469=LINE('',#121287,#7243);
#5470=LINE('',#121369,#7244);
#5471=LINE('',#121432,#7245);
#5472=LINE('',#121512,#7246);
#5473=LINE('',#121577,#7247);
#5474=LINE('',#121656,#7248);
#5475=LINE('',#121719,#7249);
#5476=LINE('',#121792,#7250);
#5477=LINE('',#121853,#7251);
#5478=LINE('',#121933,#7252);
#5479=LINE('',#121998,#7253);
#5480=LINE('',#122075,#7254);
#5481=LINE('',#122140,#7255);
#5482=LINE('',#122219,#7256);
#5483=LINE('',#122282,#7257);
#5484=LINE('',#122304,#7258);
#5485=LINE('',#122365,#7259);
#5486=LINE('',#122392,#7260);
#5487=LINE('',#122460,#7261);
#5488=LINE('',#122535,#7262);
#5489=LINE('',#122600,#7263);
#5490=LINE('',#122677,#7264);
#5491=LINE('',#122742,#7265);
#5492=LINE('',#122766,#7266);
#5493=LINE('',#122825,#7267);
#5494=LINE('',#122850,#7268);
#5495=LINE('',#122918,#7269);
#5496=LINE('',#122942,#7270);
#5497=LINE('',#123007,#7271);
#5498=LINE('',#123031,#7272);
#5499=LINE('',#123096,#7273);
#5500=LINE('',#123120,#7274);
#5501=LINE('',#123179,#7275);
#5502=LINE('',#123204,#7276);
#5503=LINE('',#123269,#7277);
#5504=LINE('',#123293,#7278);
#5505=LINE('',#123354,#7279);
#5506=LINE('',#123378,#7280);
#5507=LINE('',#123443,#7281);
#5508=LINE('',#123467,#7282);
#5509=LINE('',#123526,#7283);
#5510=LINE('',#123551,#7284);
#5511=LINE('',#123619,#7285);
#5512=LINE('',#123643,#7286);
#5513=LINE('',#123704,#7287);
#5514=LINE('',#123731,#7288);
#5515=LINE('',#123796,#7289);
#5516=LINE('',#123823,#7290);
#5517=LINE('',#123886,#7291);
#5518=LINE('',#123911,#7292);
#5519=LINE('',#123976,#7293);
#5520=LINE('',#124000,#7294);
#5521=LINE('',#124066,#7295);
#5522=LINE('',#124088,#7296);
#5523=LINE('',#124153,#7297);
#5524=LINE('',#124177,#7298);
#5525=LINE('',#124240,#7299);
#5526=LINE('',#124265,#7300);
#5527=LINE('',#124333,#7301);
#5528=LINE('',#124357,#7302);
#5529=LINE('',#124423,#7303);
#5530=LINE('',#124445,#7304);
#5531=LINE('',#124513,#7305);
#5532=LINE('',#124537,#7306);
#5533=LINE('',#124600,#7307);
#5534=LINE('',#124627,#7308);
#5535=LINE('',#124693,#7309);
#5536=LINE('',#124717,#7310);
#5537=LINE('',#124785,#7311);
#5538=LINE('',#124809,#7312);
#5539=LINE('',#124872,#7313);
#5540=LINE('',#124901,#7314);
#5541=LINE('',#124907,#7315);
#5542=LINE('',#124913,#7316);
#5543=LINE('',#124919,#7317);
#5544=LINE('',#124925,#7318);
#5545=LINE('',#124931,#7319);
#5546=LINE('',#124937,#7320);
#5547=LINE('',#124943,#7321);
#5548=LINE('',#124949,#7322);
#5549=LINE('',#124955,#7323);
#5550=LINE('',#124961,#7324);
#5551=LINE('',#124967,#7325);
#5552=LINE('',#124973,#7326);
#5553=LINE('',#124979,#7327);
#5554=LINE('',#124985,#7328);
#5555=LINE('',#124991,#7329);
#5556=LINE('',#124997,#7330);
#5557=LINE('',#125003,#7331);
#5558=LINE('',#125009,#7332);
#5559=LINE('',#125015,#7333);
#5560=LINE('',#125021,#7334);
#5561=LINE('',#125027,#7335);
#5562=LINE('',#125033,#7336);
#5563=LINE('',#125039,#7337);
#5564=LINE('',#125045,#7338);
#5565=LINE('',#125051,#7339);
#5566=LINE('',#125057,#7340);
#5567=LINE('',#125063,#7341);
#5568=LINE('',#125069,#7342);
#5569=LINE('',#125075,#7343);
#5570=LINE('',#125081,#7344);
#5571=LINE('',#125087,#7345);
#5572=LINE('',#125093,#7346);
#5573=LINE('',#125099,#7347);
#5574=LINE('',#125105,#7348);
#5575=LINE('',#125111,#7349);
#5576=LINE('',#125117,#7350);
#5577=LINE('',#125123,#7351);
#5578=LINE('',#125129,#7352);
#5579=LINE('',#125135,#7353);
#5580=LINE('',#125141,#7354);
#5581=LINE('',#125147,#7355);
#5582=LINE('',#125153,#7356);
#5583=LINE('',#125159,#7357);
#5584=LINE('',#125165,#7358);
#5585=LINE('',#125171,#7359);
#5586=LINE('',#125177,#7360);
#5587=LINE('',#125183,#7361);
#5588=LINE('',#125189,#7362);
#5589=LINE('',#125195,#7363);
#5590=LINE('',#125201,#7364);
#5591=LINE('',#125207,#7365);
#5592=LINE('',#125213,#7366);
#5593=LINE('',#125219,#7367);
#5594=LINE('',#125225,#7368);
#5595=LINE('',#125231,#7369);
#5596=LINE('',#125237,#7370);
#5597=LINE('',#125243,#7371);
#5598=LINE('',#125249,#7372);
#5599=LINE('',#125255,#7373);
#5600=LINE('',#125261,#7374);
#5601=LINE('',#125267,#7375);
#5602=LINE('',#125273,#7376);
#5603=LINE('',#125279,#7377);
#5604=LINE('',#125285,#7378);
#5605=LINE('',#125291,#7379);
#5606=LINE('',#125297,#7380);
#5607=LINE('',#125303,#7381);
#5608=LINE('',#125309,#7382);
#5609=LINE('',#125315,#7383);
#5610=LINE('',#125321,#7384);
#5611=LINE('',#125327,#7385);
#5612=LINE('',#125333,#7386);
#5613=LINE('',#125339,#7387);
#5614=LINE('',#125345,#7388);
#5615=LINE('',#125351,#7389);
#5616=LINE('',#125357,#7390);
#5617=LINE('',#125363,#7391);
#5618=LINE('',#125369,#7392);
#5619=LINE('',#125375,#7393);
#5620=LINE('',#125381,#7394);
#5621=LINE('',#125387,#7395);
#5622=LINE('',#125393,#7396);
#5623=LINE('',#125399,#7397);
#5624=LINE('',#125405,#7398);
#5625=LINE('',#125411,#7399);
#5626=LINE('',#125417,#7400);
#5627=LINE('',#125423,#7401);
#5628=LINE('',#125429,#7402);
#5629=LINE('',#125435,#7403);
#5630=LINE('',#125441,#7404);
#5631=LINE('',#125447,#7405);
#5632=LINE('',#125453,#7406);
#5633=LINE('',#125459,#7407);
#5634=LINE('',#125465,#7408);
#5635=LINE('',#125471,#7409);
#5636=LINE('',#125477,#7410);
#5637=LINE('',#125483,#7411);
#5638=LINE('',#125489,#7412);
#5639=LINE('',#125495,#7413);
#5640=LINE('',#125501,#7414);
#5641=LINE('',#125507,#7415);
#5642=LINE('',#125513,#7416);
#5643=LINE('',#125519,#7417);
#5644=LINE('',#125525,#7418);
#5645=LINE('',#125531,#7419);
#5646=LINE('',#125537,#7420);
#5647=LINE('',#125543,#7421);
#5648=LINE('',#125549,#7422);
#5649=LINE('',#125555,#7423);
#5650=LINE('',#125561,#7424);
#5651=LINE('',#125567,#7425);
#5652=LINE('',#125573,#7426);
#5653=LINE('',#125579,#7427);
#5654=LINE('',#125585,#7428);
#5655=LINE('',#125591,#7429);
#5656=LINE('',#125597,#7430);
#5657=LINE('',#125603,#7431);
#5658=LINE('',#125609,#7432);
#5659=LINE('',#125615,#7433);
#5660=LINE('',#125621,#7434);
#5661=LINE('',#125627,#7435);
#5662=LINE('',#125633,#7436);
#5663=LINE('',#125639,#7437);
#5664=LINE('',#125645,#7438);
#5665=LINE('',#125651,#7439);
#5666=LINE('',#125657,#7440);
#5667=LINE('',#125663,#7441);
#5668=LINE('',#125669,#7442);
#5669=LINE('',#125675,#7443);
#5670=LINE('',#125681,#7444);
#5671=LINE('',#125687,#7445);
#5672=LINE('',#125693,#7446);
#5673=LINE('',#125699,#7447);
#5674=LINE('',#125705,#7448);
#5675=LINE('',#125711,#7449);
#5676=LINE('',#125717,#7450);
#5677=LINE('',#125723,#7451);
#5678=LINE('',#125729,#7452);
#5679=LINE('',#125735,#7453);
#5680=LINE('',#125741,#7454);
#5681=LINE('',#125747,#7455);
#5682=LINE('',#125753,#7456);
#5683=LINE('',#125759,#7457);
#5684=LINE('',#125765,#7458);
#5685=LINE('',#125771,#7459);
#5686=LINE('',#125777,#7460);
#5687=LINE('',#125783,#7461);
#5688=LINE('',#125789,#7462);
#5689=LINE('',#125795,#7463);
#5690=LINE('',#125801,#7464);
#5691=LINE('',#125807,#7465);
#5692=LINE('',#125813,#7466);
#5693=LINE('',#125819,#7467);
#5694=LINE('',#125825,#7468);
#5695=LINE('',#125831,#7469);
#5696=LINE('',#125837,#7470);
#5697=LINE('',#125843,#7471);
#5698=LINE('',#125849,#7472);
#5699=LINE('',#125855,#7473);
#5700=LINE('',#125861,#7474);
#5701=LINE('',#125867,#7475);
#5702=LINE('',#125873,#7476);
#5703=LINE('',#125879,#7477);
#5704=LINE('',#125885,#7478);
#5705=LINE('',#125891,#7479);
#5706=LINE('',#125897,#7480);
#5707=LINE('',#125903,#7481);
#5708=LINE('',#125909,#7482);
#5709=LINE('',#125915,#7483);
#5710=LINE('',#125921,#7484);
#5711=LINE('',#125927,#7485);
#5712=LINE('',#125933,#7486);
#5713=LINE('',#125939,#7487);
#5714=LINE('',#125945,#7488);
#5715=LINE('',#125951,#7489);
#5716=LINE('',#125957,#7490);
#5717=LINE('',#125963,#7491);
#5718=LINE('',#125969,#7492);
#5719=LINE('',#125975,#7493);
#5720=LINE('',#125981,#7494);
#5721=LINE('',#125987,#7495);
#5722=LINE('',#125993,#7496);
#5723=LINE('',#125999,#7497);
#5724=LINE('',#126005,#7498);
#5725=LINE('',#126011,#7499);
#5726=LINE('',#126017,#7500);
#5727=LINE('',#126023,#7501);
#5728=LINE('',#126029,#7502);
#5729=LINE('',#126035,#7503);
#5730=LINE('',#126041,#7504);
#5731=LINE('',#126047,#7505);
#5732=LINE('',#126053,#7506);
#5733=LINE('',#126059,#7507);
#5734=LINE('',#126065,#7508);
#5735=LINE('',#126071,#7509);
#5736=LINE('',#126077,#7510);
#5737=LINE('',#126083,#7511);
#5738=LINE('',#126089,#7512);
#5739=LINE('',#126095,#7513);
#5740=LINE('',#126101,#7514);
#5741=LINE('',#126107,#7515);
#5742=LINE('',#126113,#7516);
#5743=LINE('',#126119,#7517);
#5744=LINE('',#126125,#7518);
#5745=LINE('',#126131,#7519);
#5746=LINE('',#126137,#7520);
#5747=LINE('',#126143,#7521);
#5748=LINE('',#126149,#7522);
#5749=LINE('',#126155,#7523);
#5750=LINE('',#126161,#7524);
#5751=LINE('',#126167,#7525);
#5752=LINE('',#126173,#7526);
#5753=LINE('',#126179,#7527);
#5754=LINE('',#126185,#7528);
#5755=LINE('',#126191,#7529);
#5756=LINE('',#126197,#7530);
#5757=LINE('',#126203,#7531);
#5758=LINE('',#126209,#7532);
#5759=LINE('',#126215,#7533);
#5760=LINE('',#126221,#7534);
#5761=LINE('',#126227,#7535);
#5762=LINE('',#126233,#7536);
#5763=LINE('',#126239,#7537);
#5764=LINE('',#126245,#7538);
#5765=LINE('',#126251,#7539);
#5766=LINE('',#126257,#7540);
#5767=LINE('',#126263,#7541);
#5768=LINE('',#126269,#7542);
#5769=LINE('',#126275,#7543);
#5770=LINE('',#126281,#7544);
#5771=LINE('',#126287,#7545);
#5772=LINE('',#126293,#7546);
#5773=LINE('',#126299,#7547);
#5774=LINE('',#126305,#7548);
#5775=LINE('',#126311,#7549);
#5776=LINE('',#126317,#7550);
#5777=LINE('',#126323,#7551);
#5778=LINE('',#126329,#7552);
#5779=LINE('',#126335,#7553);
#5780=LINE('',#126341,#7554);
#5781=LINE('',#126347,#7555);
#5782=LINE('',#126353,#7556);
#5783=LINE('',#126359,#7557);
#5784=LINE('',#126365,#7558);
#5785=LINE('',#126371,#7559);
#5786=LINE('',#126377,#7560);
#5787=LINE('',#126383,#7561);
#5788=LINE('',#126389,#7562);
#5789=LINE('',#126395,#7563);
#5790=LINE('',#126401,#7564);
#5791=LINE('',#126407,#7565);
#5792=LINE('',#126413,#7566);
#5793=LINE('',#126419,#7567);
#5794=LINE('',#126425,#7568);
#5795=LINE('',#126431,#7569);
#5796=LINE('',#126437,#7570);
#5797=LINE('',#126443,#7571);
#5798=LINE('',#126449,#7572);
#5799=LINE('',#126455,#7573);
#5800=LINE('',#126461,#7574);
#5801=LINE('',#126467,#7575);
#5802=LINE('',#126473,#7576);
#5803=LINE('',#126479,#7577);
#5804=LINE('',#126485,#7578);
#5805=LINE('',#126491,#7579);
#5806=LINE('',#126497,#7580);
#5807=LINE('',#126503,#7581);
#5808=LINE('',#126509,#7582);
#5809=LINE('',#126515,#7583);
#5810=LINE('',#126521,#7584);
#5811=LINE('',#126527,#7585);
#5812=LINE('',#126533,#7586);
#5813=LINE('',#126539,#7587);
#5814=LINE('',#126545,#7588);
#5815=LINE('',#126551,#7589);
#5816=LINE('',#126557,#7590);
#5817=LINE('',#126563,#7591);
#5818=LINE('',#126569,#7592);
#5819=LINE('',#126575,#7593);
#5820=LINE('',#126581,#7594);
#5821=LINE('',#126587,#7595);
#5822=LINE('',#126593,#7596);
#5823=LINE('',#126599,#7597);
#5824=LINE('',#126605,#7598);
#5825=LINE('',#126611,#7599);
#5826=LINE('',#126617,#7600);
#5827=LINE('',#126623,#7601);
#5828=LINE('',#126629,#7602);
#5829=LINE('',#126635,#7603);
#5830=LINE('',#126641,#7604);
#5831=LINE('',#126647,#7605);
#5832=LINE('',#126653,#7606);
#5833=LINE('',#126659,#7607);
#5834=LINE('',#126665,#7608);
#5835=LINE('',#126671,#7609);
#5836=LINE('',#126677,#7610);
#5837=LINE('',#126683,#7611);
#5838=LINE('',#126689,#7612);
#5839=LINE('',#126695,#7613);
#5840=LINE('',#126701,#7614);
#5841=LINE('',#126707,#7615);
#5842=LINE('',#126713,#7616);
#5843=LINE('',#126719,#7617);
#5844=LINE('',#126725,#7618);
#5845=LINE('',#126731,#7619);
#5846=LINE('',#126737,#7620);
#5847=LINE('',#126743,#7621);
#5848=LINE('',#126749,#7622);
#5849=LINE('',#126755,#7623);
#5850=LINE('',#126761,#7624);
#5851=LINE('',#126767,#7625);
#5852=LINE('',#126773,#7626);
#5853=LINE('',#126779,#7627);
#5854=LINE('',#126785,#7628);
#5855=LINE('',#126791,#7629);
#5856=LINE('',#126797,#7630);
#5857=LINE('',#126803,#7631);
#5858=LINE('',#126809,#7632);
#5859=LINE('',#126815,#7633);
#5860=LINE('',#126821,#7634);
#5861=LINE('',#126827,#7635);
#5862=LINE('',#126833,#7636);
#5863=LINE('',#126839,#7637);
#5864=LINE('',#126845,#7638);
#5865=LINE('',#126851,#7639);
#5866=LINE('',#126857,#7640);
#5867=LINE('',#126863,#7641);
#5868=LINE('',#126869,#7642);
#5869=LINE('',#126875,#7643);
#5870=LINE('',#126881,#7644);
#5871=LINE('',#126887,#7645);
#5872=LINE('',#126893,#7646);
#5873=LINE('',#126899,#7647);
#5874=LINE('',#126905,#7648);
#5875=LINE('',#126911,#7649);
#5876=LINE('',#126917,#7650);
#5877=LINE('',#126923,#7651);
#5878=LINE('',#126929,#7652);
#5879=LINE('',#126935,#7653);
#5880=LINE('',#126941,#7654);
#5881=LINE('',#126947,#7655);
#5882=LINE('',#126953,#7656);
#5883=LINE('',#126959,#7657);
#5884=LINE('',#126965,#7658);
#5885=LINE('',#126971,#7659);
#5886=LINE('',#126977,#7660);
#5887=LINE('',#126983,#7661);
#5888=LINE('',#126989,#7662);
#5889=LINE('',#126995,#7663);
#5890=LINE('',#127001,#7664);
#5891=LINE('',#127007,#7665);
#5892=LINE('',#127013,#7666);
#5893=LINE('',#127019,#7667);
#5894=LINE('',#127025,#7668);
#5895=LINE('',#127031,#7669);
#5896=LINE('',#127037,#7670);
#5897=LINE('',#127043,#7671);
#5898=LINE('',#127049,#7672);
#5899=LINE('',#127055,#7673);
#5900=LINE('',#127061,#7674);
#5901=LINE('',#127067,#7675);
#5902=LINE('',#127073,#7676);
#5903=LINE('',#127079,#7677);
#5904=LINE('',#127085,#7678);
#5905=LINE('',#127091,#7679);
#5906=LINE('',#127097,#7680);
#5907=LINE('',#127103,#7681);
#5908=LINE('',#127109,#7682);
#5909=LINE('',#127115,#7683);
#5910=LINE('',#127121,#7684);
#5911=LINE('',#127127,#7685);
#5912=LINE('',#127133,#7686);
#5913=LINE('',#127139,#7687);
#5914=LINE('',#127145,#7688);
#5915=LINE('',#127151,#7689);
#5916=LINE('',#127157,#7690);
#5917=LINE('',#127163,#7691);
#5918=LINE('',#127169,#7692);
#5919=LINE('',#127175,#7693);
#5920=LINE('',#127181,#7694);
#5921=LINE('',#127187,#7695);
#5922=LINE('',#127193,#7696);
#5923=LINE('',#127199,#7697);
#5924=LINE('',#127205,#7698);
#5925=LINE('',#127211,#7699);
#5926=LINE('',#127217,#7700);
#5927=LINE('',#127223,#7701);
#5928=LINE('',#127229,#7702);
#5929=LINE('',#127235,#7703);
#5930=LINE('',#127241,#7704);
#5931=LINE('',#127247,#7705);
#5932=LINE('',#127253,#7706);
#5933=LINE('',#127259,#7707);
#5934=LINE('',#127265,#7708);
#5935=LINE('',#127271,#7709);
#5936=LINE('',#127277,#7710);
#5937=LINE('',#127283,#7711);
#5938=LINE('',#127289,#7712);
#5939=LINE('',#127295,#7713);
#5940=LINE('',#127301,#7714);
#5941=LINE('',#127307,#7715);
#5942=LINE('',#127313,#7716);
#5943=LINE('',#127319,#7717);
#5944=LINE('',#127325,#7718);
#5945=LINE('',#127331,#7719);
#5946=LINE('',#127337,#7720);
#5947=LINE('',#127343,#7721);
#5948=LINE('',#127349,#7722);
#5949=LINE('',#127355,#7723);
#5950=LINE('',#127361,#7724);
#5951=LINE('',#127367,#7725);
#5952=LINE('',#127373,#7726);
#5953=LINE('',#127379,#7727);
#5954=LINE('',#127385,#7728);
#5955=LINE('',#127391,#7729);
#5956=LINE('',#127397,#7730);
#5957=LINE('',#127403,#7731);
#5958=LINE('',#127409,#7732);
#5959=LINE('',#127415,#7733);
#5960=LINE('',#127421,#7734);
#5961=LINE('',#127427,#7735);
#5962=LINE('',#127433,#7736);
#5963=LINE('',#127439,#7737);
#5964=LINE('',#127445,#7738);
#5965=LINE('',#127451,#7739);
#5966=LINE('',#127457,#7740);
#5967=LINE('',#127463,#7741);
#5968=LINE('',#127469,#7742);
#5969=LINE('',#127475,#7743);
#5970=LINE('',#127481,#7744);
#5971=LINE('',#127487,#7745);
#5972=LINE('',#127493,#7746);
#5973=LINE('',#127499,#7747);
#5974=LINE('',#127505,#7748);
#5975=LINE('',#127511,#7749);
#5976=LINE('',#127517,#7750);
#5977=LINE('',#127523,#7751);
#5978=LINE('',#127529,#7752);
#5979=LINE('',#127535,#7753);
#5980=LINE('',#127541,#7754);
#5981=LINE('',#127547,#7755);
#5982=LINE('',#127553,#7756);
#5983=LINE('',#127559,#7757);
#5984=LINE('',#127565,#7758);
#5985=LINE('',#127571,#7759);
#5986=LINE('',#127577,#7760);
#5987=LINE('',#127583,#7761);
#5988=LINE('',#127589,#7762);
#5989=LINE('',#127595,#7763);
#5990=LINE('',#127601,#7764);
#5991=LINE('',#127607,#7765);
#5992=LINE('',#127613,#7766);
#5993=LINE('',#127619,#7767);
#5994=LINE('',#127625,#7768);
#5995=LINE('',#127631,#7769);
#5996=LINE('',#127637,#7770);
#5997=LINE('',#127643,#7771);
#5998=LINE('',#127649,#7772);
#5999=LINE('',#127655,#7773);
#6000=LINE('',#127661,#7774);
#6001=LINE('',#127667,#7775);
#6002=LINE('',#127673,#7776);
#6003=LINE('',#127679,#7777);
#6004=LINE('',#127685,#7778);
#6005=LINE('',#127691,#7779);
#6006=LINE('',#127697,#7780);
#6007=LINE('',#127703,#7781);
#6008=LINE('',#127709,#7782);
#6009=LINE('',#127715,#7783);
#6010=LINE('',#127721,#7784);
#6011=LINE('',#127727,#7785);
#6012=LINE('',#127733,#7786);
#6013=LINE('',#127739,#7787);
#6014=LINE('',#127745,#7788);
#6015=LINE('',#127751,#7789);
#6016=LINE('',#127757,#7790);
#6017=LINE('',#127763,#7791);
#6018=LINE('',#127769,#7792);
#6019=LINE('',#127775,#7793);
#6020=LINE('',#127781,#7794);
#6021=LINE('',#127787,#7795);
#6022=LINE('',#127793,#7796);
#6023=LINE('',#127799,#7797);
#6024=LINE('',#127805,#7798);
#6025=LINE('',#127811,#7799);
#6026=LINE('',#127817,#7800);
#6027=LINE('',#127823,#7801);
#6028=LINE('',#127829,#7802);
#6029=LINE('',#127835,#7803);
#6030=LINE('',#127841,#7804);
#6031=LINE('',#127847,#7805);
#6032=LINE('',#127853,#7806);
#6033=LINE('',#127859,#7807);
#6034=LINE('',#127865,#7808);
#6035=LINE('',#127871,#7809);
#6036=LINE('',#127877,#7810);
#6037=LINE('',#127883,#7811);
#6038=LINE('',#127889,#7812);
#6039=LINE('',#127895,#7813);
#6040=LINE('',#127901,#7814);
#6041=LINE('',#127907,#7815);
#6042=LINE('',#127913,#7816);
#6043=LINE('',#127919,#7817);
#6044=LINE('',#127925,#7818);
#6045=LINE('',#127931,#7819);
#6046=LINE('',#127937,#7820);
#6047=LINE('',#127943,#7821);
#6048=LINE('',#127949,#7822);
#6049=LINE('',#127955,#7823);
#6050=LINE('',#127961,#7824);
#6051=LINE('',#127967,#7825);
#6052=LINE('',#127973,#7826);
#6053=LINE('',#127979,#7827);
#6054=LINE('',#127985,#7828);
#6055=LINE('',#127991,#7829);
#6056=LINE('',#127997,#7830);
#6057=LINE('',#128003,#7831);
#6058=LINE('',#128009,#7832);
#6059=LINE('',#128015,#7833);
#6060=LINE('',#128021,#7834);
#6061=LINE('',#128027,#7835);
#6062=LINE('',#128033,#7836);
#6063=LINE('',#128039,#7837);
#6064=LINE('',#128045,#7838);
#6065=LINE('',#128051,#7839);
#6066=LINE('',#128057,#7840);
#6067=LINE('',#128063,#7841);
#6068=LINE('',#128069,#7842);
#6069=LINE('',#128075,#7843);
#6070=LINE('',#128081,#7844);
#6071=LINE('',#128087,#7845);
#6072=LINE('',#128093,#7846);
#6073=LINE('',#128099,#7847);
#6074=LINE('',#128105,#7848);
#6075=LINE('',#128111,#7849);
#6076=LINE('',#128117,#7850);
#6077=LINE('',#128123,#7851);
#6078=LINE('',#128129,#7852);
#6079=LINE('',#128135,#7853);
#6080=LINE('',#128144,#7854);
#6081=LINE('',#128161,#7855);
#6082=LINE('',#128184,#7856);
#6083=LINE('',#128194,#7857);
#6084=LINE('',#128221,#7858);
#6085=LINE('',#128245,#7859);
#7076=VECTOR('',#59313,1.27544412113617);
#7077=VECTOR('',#59316,0.675444121136126);
#7078=VECTOR('',#59321,1.09883113599246);
#7079=VECTOR('',#59324,0.498831135992472);
#7080=VECTOR('',#59329,1.09054074872833);
#7081=VECTOR('',#59332,0.490540748728341);
#7082=VECTOR('',#59337,1.47830313219327);
#7083=VECTOR('',#59340,0.878303132193281);
#7084=VECTOR('',#59345,1.27544412113612);
#7085=VECTOR('',#59348,0.675444121136182);
#7086=VECTOR('',#59353,1.09883113599246);
#7087=VECTOR('',#59356,0.498831135992472);
#7088=VECTOR('',#59361,1.09054074872833);
#7089=VECTOR('',#59364,0.490540748728341);
#7090=VECTOR('',#59369,1.47830313219333);
#7091=VECTOR('',#59372,0.878303132193337);
#7092=VECTOR('',#59377,1.27544412113617);
#7093=VECTOR('',#59380,0.675444121136126);
#7094=VECTOR('',#59385,1.09883113599246);
#7095=VECTOR('',#59388,0.498831135992472);
#7096=VECTOR('',#59393,1.09054074872833);
#7097=VECTOR('',#59396,0.490540748728341);
#7098=VECTOR('',#59401,1.47830313219327);
#7099=VECTOR('',#59404,0.878303132193281);
#7100=VECTOR('',#59409,1.27544412113617);
#7101=VECTOR('',#59412,0.675444121136126);
#7102=VECTOR('',#59417,1.09883113599246);
#7103=VECTOR('',#59420,0.498831135992472);
#7104=VECTOR('',#59425,1.09054074872833);
#7105=VECTOR('',#59428,0.490540748728285);
#7106=VECTOR('',#59433,1.47830313219327);
#7107=VECTOR('',#59436,0.878303132193226);
#7108=VECTOR('',#59441,1.27544412113617);
#7109=VECTOR('',#59444,0.675444121136182);
#7110=VECTOR('',#59449,1.09883113599246);
#7111=VECTOR('',#59452,0.498831135992472);
#7112=VECTOR('',#59457,1.09054074872833);
#7113=VECTOR('',#59460,0.490540748728341);
#7114=VECTOR('',#59465,1.47830313219333);
#7115=VECTOR('',#59468,0.878303132193281);
#7116=VECTOR('',#59473,1.27544412113612);
#7117=VECTOR('',#59476,0.675444121136182);
#7118=VECTOR('',#59481,1.09883113599241);
#7119=VECTOR('',#59484,0.498831135992472);
#7120=VECTOR('',#59489,1.09054074872839);
#7121=VECTOR('',#59492,0.490540748728341);
#7122=VECTOR('',#59497,1.47830313219333);
#7123=VECTOR('',#59500,0.878303132193281);
#7124=VECTOR('',#59505,1.27544412113612);
#7125=VECTOR('',#59508,0.675444121136182);
#7126=VECTOR('',#59513,1.09883113599252);
#7127=VECTOR('',#59516,0.498831135992583);
#7128=VECTOR('',#59521,1.09054074872827);
#7129=VECTOR('',#59524,0.490540748728341);
#7130=VECTOR('',#59529,1.47830313219321);
#7131=VECTOR('',#59532,0.87830313219317);
#7132=VECTOR('',#59537,1.27544412113612);
#7133=VECTOR('',#59540,0.675444121136071);
#7134=VECTOR('',#59545,1.09883113599252);
#7135=VECTOR('',#59548,0.498831135992472);
#7136=VECTOR('',#59553,1.09054074872839);
#7137=VECTOR('',#59556,0.490540748728341);
#7138=VECTOR('',#59561,1.47830313219321);
#7139=VECTOR('',#59564,0.87830313219317);
#7140=VECTOR('',#59569,1.27544412113612);
#7141=VECTOR('',#59572,0.675444121136071);
#7142=VECTOR('',#59577,1.09883113599241);
#7143=VECTOR('',#59580,0.498831135992361);
#7144=VECTOR('',#59585,1.09054074872839);
#7145=VECTOR('',#59588,0.490540748728341);
#7146=VECTOR('',#59593,1.47830313219333);
#7147=VECTOR('',#59596,0.878303132193281);
#7148=VECTOR('',#59601,1.27544412113612);
#7149=VECTOR('',#59604,0.675444121136182);
#7150=VECTOR('',#59609,1.09883113599252);
#7151=VECTOR('',#59612,0.498831135992472);
#7152=VECTOR('',#59617,1.09054074872827);
#7153=VECTOR('',#59620,0.49054074872823);
#7154=VECTOR('',#59625,1.47830313219333);
#7155=VECTOR('',#59628,0.878303132193281);
#7156=VECTOR('',#59633,1.27544412113623);
#7157=VECTOR('',#59636,0.675444121136182);
#7158=VECTOR('',#59641,1.09883113599252);
#7159=VECTOR('',#59644,0.498831135992472);
#7160=VECTOR('',#59649,1.09054074872827);
#7161=VECTOR('',#59652,0.490540748728341);
#7162=VECTOR('',#59657,1.47830313219333);
#7163=VECTOR('',#59660,0.878303132193281);
#7164=VECTOR('',#59665,1.27544412113617);
#7165=VECTOR('',#59668,0.675444121136126);
#7166=VECTOR('',#59673,1.09883113599252);
#7167=VECTOR('',#59676,0.498831135992472);
#7168=VECTOR('',#59681,1.09054074872839);
#7169=VECTOR('',#59684,0.490540748728341);
#7170=VECTOR('',#59689,1.47830313219327);
#7171=VECTOR('',#59692,0.878303132193281);
#7172=VECTOR('',#59697,1.27544412113617);
#7173=VECTOR('',#59700,0.675444121136182);
#7174=VECTOR('',#59705,1.09883113599246);
#7175=VECTOR('',#59708,0.498831135992417);
#7176=VECTOR('',#59713,1.09054074872827);
#7177=VECTOR('',#59716,0.490540748728341);
#7178=VECTOR('',#59721,1.47830313219327);
#7179=VECTOR('',#59724,0.878303132193281);
#7180=VECTOR('',#59729,1.27544412113612);
#7181=VECTOR('',#59732,0.675444121136126);
#7182=VECTOR('',#59737,1.09883113599241);
#7183=VECTOR('',#59740,0.498831135992417);
#7184=VECTOR('',#59745,1.09054074872839);
#7185=VECTOR('',#59748,0.490540748728341);
#7186=VECTOR('',#59753,1.47830313219333);
#7187=VECTOR('',#59756,0.878303132193337);
#7188=VECTOR('',#59761,1.27544412113617);
#7189=VECTOR('',#59764,0.675444121136182);
#7190=VECTOR('',#59769,1.09883113599246);
#7191=VECTOR('',#59772,0.498831135992417);
#7192=VECTOR('',#59777,1.09054074872833);
#7193=VECTOR('',#59780,0.490540748728341);
#7194=VECTOR('',#59785,1.47830313219333);
#7195=VECTOR('',#59788,0.878303132193337);
#7196=VECTOR('',#59793,1.27544412113617);
#7197=VECTOR('',#59796,0.675444121136126);
#7198=VECTOR('',#59801,1.09883113599246);
#7199=VECTOR('',#59804,0.498831135992472);
#7200=VECTOR('',#59809,1.09054074872833);
#7201=VECTOR('',#59812,0.490540748728341);
#7202=VECTOR('',#59817,1.47830313219333);
#7203=VECTOR('',#59820,0.878303132193281);
#7204=VECTOR('',#59825,1.27544412113617);
#7205=VECTOR('',#59828,0.675444121136182);
#7206=VECTOR('',#59833,1.09883113599246);
#7207=VECTOR('',#59836,0.498831135992472);
#7208=VECTOR('',#59841,1.09054074872833);
#7209=VECTOR('',#59844,0.490540748728341);
#7210=VECTOR('',#59849,1.47830313219333);
#7211=VECTOR('',#59852,0.878303132193281);
#7212=VECTOR('',#59857,1.27544412113617);
#7213=VECTOR('',#59860,0.675444121136182);
#7214=VECTOR('',#59865,1.09883113599246);
#7215=VECTOR('',#59868,0.498831135992472);
#7216=VECTOR('',#59873,1.09054074872833);
#7217=VECTOR('',#59876,0.490540748728341);
#7218=VECTOR('',#59881,1.47830313219333);
#7219=VECTOR('',#59884,0.878303132193281);
#7220=VECTOR('',#59889,1.27544412113612);
#7221=VECTOR('',#59892,0.675444121136126);
#7222=VECTOR('',#59897,1.09883113599252);
#7223=VECTOR('',#59900,0.498831135992472);
#7224=VECTOR('',#59905,1.09054074872833);
#7225=VECTOR('',#59908,0.490540748728341);
#7226=VECTOR('',#59913,1.47830313219333);
#7227=VECTOR('',#59916,0.878303132193337);
#7228=VECTOR('',#59921,1.27544412113617);
#7229=VECTOR('',#59924,0.675444121136126);
#7230=VECTOR('',#59929,1.09883113599246);
#7231=VECTOR('',#59932,0.498831135992472);
#7232=VECTOR('',#59937,1.09054074872833);
#7233=VECTOR('',#59940,0.490540748728341);
#7234=VECTOR('',#59945,1.47830313219327);
#7235=VECTOR('',#59948,0.878303132193281);
#7236=VECTOR('',#59953,1.27544412113617);
#7237=VECTOR('',#59956,0.675444121136182);
#7238=VECTOR('',#59961,1.09883113599246);
#7239=VECTOR('',#59964,0.498831135992472);
#7240=VECTOR('',#59969,1.09054074872827);
#7241=VECTOR('',#59972,0.490540748728341);
#7242=VECTOR('',#59977,1.47830313219327);
#7243=VECTOR('',#59980,0.878303132193281);
#7244=VECTOR('',#59985,1.27544412113617);
#7245=VECTOR('',#59988,0.675444121136126);
#7246=VECTOR('',#59993,1.09883113599241);
#7247=VECTOR('',#59996,0.498831135992472);
#7248=VECTOR('',#60001,1.09054074872827);
#7249=VECTOR('',#60004,0.490540748728341);
#7250=VECTOR('',#60009,1.47830313219327);
#7251=VECTOR('',#60012,0.878303132193281);
#7252=VECTOR('',#60017,1.27544412113617);
#7253=VECTOR('',#60020,0.675444121136126);
#7254=VECTOR('',#60025,1.09883113599252);
#7255=VECTOR('',#60028,0.498831135992472);
#7256=VECTOR('',#60033,1.09054074872839);
#7257=VECTOR('',#60036,0.490540748728396);
#7258=VECTOR('',#60041,1.47830313219327);
#7259=VECTOR('',#60044,0.878303132193281);
#7260=VECTOR('',#60049,1.27544412113612);
#7261=VECTOR('',#60052,0.675444121136126);
#7262=VECTOR('',#60057,1.09883113599241);
#7263=VECTOR('',#60060,0.498831135992417);
#7264=VECTOR('',#60065,1.09054074872833);
#7265=VECTOR('',#60068,0.490540748728341);
#7266=VECTOR('',#60073,1.47830313219327);
#7267=VECTOR('',#60076,0.878303132193281);
#7268=VECTOR('',#60081,1.27544412113617);
#7269=VECTOR('',#60084,0.675444121136126);
#7270=VECTOR('',#60089,1.09883113599241);
#7271=VECTOR('',#60092,0.498831135992472);
#7272=VECTOR('',#60097,1.09054074872839);
#7273=VECTOR('',#60100,0.490540748728396);
#7274=VECTOR('',#60105,1.47830313219327);
#7275=VECTOR('',#60108,0.878303132193281);
#7276=VECTOR('',#60113,1.27544412113617);
#7277=VECTOR('',#60116,0.675444121136182);
#7278=VECTOR('',#60121,1.09883113599246);
#7279=VECTOR('',#60124,0.498831135992528);
#7280=VECTOR('',#60129,1.09054074872833);
#7281=VECTOR('',#60132,0.490540748728341);
#7282=VECTOR('',#60137,1.47830313219333);
#7283=VECTOR('',#60140,0.878303132193337);
#7284=VECTOR('',#60145,1.27544412113617);
#7285=VECTOR('',#60148,0.675444121136126);
#7286=VECTOR('',#60153,1.09883113599246);
#7287=VECTOR('',#60156,0.498831135992472);
#7288=VECTOR('',#60161,1.09054074872839);
#7289=VECTOR('',#60164,0.490540748728285);
#7290=VECTOR('',#60169,1.47830313219327);
#7291=VECTOR('',#60172,0.878303132193281);
#7292=VECTOR('',#60177,1.27544412113617);
#7293=VECTOR('',#60180,0.675444121136126);
#7294=VECTOR('',#60185,1.09883113599246);
#7295=VECTOR('',#60188,0.498831135992528);
#7296=VECTOR('',#60193,1.09054074872833);
#7297=VECTOR('',#60196,0.490540748728341);
#7298=VECTOR('',#60201,1.47830313219333);
#7299=VECTOR('',#60204,0.878303132193337);
#7300=VECTOR('',#60209,1.27544412113617);
#7301=VECTOR('',#60212,0.675444121136182);
#7302=VECTOR('',#60217,1.09883113599246);
#7303=VECTOR('',#60220,0.498831135992472);
#7304=VECTOR('',#60225,1.09054074872833);
#7305=VECTOR('',#60228,0.490540748728285);
#7306=VECTOR('',#60233,1.47830313219327);
#7307=VECTOR('',#60236,0.878303132193281);
#7308=VECTOR('',#60241,1.27544412113617);
#7309=VECTOR('',#60244,0.675444121136126);
#7310=VECTOR('',#60249,1.09054074872833);
#7311=VECTOR('',#60252,0.490540748728341);
#7312=VECTOR('',#60257,1.09883113599252);
#7313=VECTOR('',#60260,0.498831135992472);
#7314=VECTOR('',#60267,1.10035806567471);
#7315=VECTOR('',#60274,0.500358065674722);
#7316=VECTOR('',#60281,1.21403156673711);
#7317=VECTOR('',#60288,0.614031566737117);
#7318=VECTOR('',#60295,1.32880796357332);
#7319=VECTOR('',#60302,0.72880796357333);
#7320=VECTOR('',#60309,1.46111700181689);
#7321=VECTOR('',#60316,0.861117001816902);
#7322=VECTOR('',#60323,1.6204820426246);
#7323=VECTOR('',#60330,1.02048204262462);
#7324=VECTOR('',#60337,1.70100022308284);
#7325=VECTOR('',#60344,1.10100022308285);
#7326=VECTOR('',#60351,1.72127463204352);
#7327=VECTOR('',#60358,1.12127463204348);
#7328=VECTOR('',#60365,1.78199265440493);
#7329=VECTOR('',#60372,1.18199265440494);
#7330=VECTOR('',#60379,1.66088080992077);
#7331=VECTOR('',#60386,1.06088080992078);
#7332=VECTOR('',#60393,1.10035806567471);
#7333=VECTOR('',#60400,0.500358065674722);
#7334=VECTOR('',#60407,1.21403156673716);
#7335=VECTOR('',#60414,0.614031566737117);
#7336=VECTOR('',#60421,1.32880796357332);
#7337=VECTOR('',#60428,0.728807963573275);
#7338=VECTOR('',#60435,1.46111700181689);
#7339=VECTOR('',#60442,0.861117001816902);
#7340=VECTOR('',#60449,1.6204820426246);
#7341=VECTOR('',#60456,1.02048204262462);
#7342=VECTOR('',#60463,1.70100022308284);
#7343=VECTOR('',#60470,1.10100022308285);
#7344=VECTOR('',#60477,1.72127463204347);
#7345=VECTOR('',#60484,1.12127463204348);
#7346=VECTOR('',#60491,1.78199265440493);
#7347=VECTOR('',#60498,1.18199265440494);
#7348=VECTOR('',#60505,1.66088080992077);
#7349=VECTOR('',#60512,1.06088080992078);
#7350=VECTOR('',#60519,1.10035806567471);
#7351=VECTOR('',#60526,0.500358065674722);
#7352=VECTOR('',#60533,1.21403156673716);
#7353=VECTOR('',#60540,0.614031566737117);
#7354=VECTOR('',#60547,1.32880796357326);
#7355=VECTOR('',#60554,0.72880796357333);
#7356=VECTOR('',#60561,1.46111700181689);
#7357=VECTOR('',#60568,0.861117001816902);
#7358=VECTOR('',#60575,1.6204820426246);
#7359=VECTOR('',#60582,1.02048204262456);
#7360=VECTOR('',#60589,1.70100022308284);
#7361=VECTOR('',#60596,1.10100022308285);
#7362=VECTOR('',#60603,1.72127463204347);
#7363=VECTOR('',#60610,1.12127463204348);
#7364=VECTOR('',#60617,1.78199265440493);
#7365=VECTOR('',#60624,1.18199265440494);
#7366=VECTOR('',#60631,1.66088080992077);
#7367=VECTOR('',#60638,1.06088080992078);
#7368=VECTOR('',#60645,1.10035806567471);
#7369=VECTOR('',#60652,0.500358065674666);
#7370=VECTOR('',#60659,1.21403156673711);
#7371=VECTOR('',#60666,0.614031566737172);
#7372=VECTOR('',#60673,1.32880796357332);
#7373=VECTOR('',#60680,0.72880796357333);
#7374=VECTOR('',#60687,1.46111700181689);
#7375=VECTOR('',#60694,0.861117001816847);
#7376=VECTOR('',#60701,1.6204820426246);
#7377=VECTOR('',#60708,1.02048204262462);
#7378=VECTOR('',#60715,1.70100022308284);
#7379=VECTOR('',#60722,1.10100022308285);
#7380=VECTOR('',#60729,1.72127463204347);
#7381=VECTOR('',#60736,1.12127463204353);
#7382=VECTOR('',#60743,1.78199265440498);
#7383=VECTOR('',#60750,1.18199265440494);
#7384=VECTOR('',#60757,1.66088080992083);
#7385=VECTOR('',#60764,1.06088080992078);
#7386=VECTOR('',#60771,1.10035806567477);
#7387=VECTOR('',#60778,0.500358065674777);
#7388=VECTOR('',#60785,1.21403156673711);
#7389=VECTOR('',#60792,0.614031566737172);
#7390=VECTOR('',#60799,1.32880796357326);
#7391=VECTOR('',#60806,0.72880796357333);
#7392=VECTOR('',#60813,1.46111700181684);
#7393=VECTOR('',#60820,0.861117001816847);
#7394=VECTOR('',#60827,1.6204820426246);
#7395=VECTOR('',#60834,1.02048204262462);
#7396=VECTOR('',#60841,1.70100022308278);
#7397=VECTOR('',#60848,1.1010002230829);
#7398=VECTOR('',#60855,1.72127463204347);
#7399=VECTOR('',#60862,1.12127463204342);
#7400=VECTOR('',#60869,1.78199265440487);
#7401=VECTOR('',#60876,1.18199265440488);
#7402=VECTOR('',#60883,1.66088080992077);
#7403=VECTOR('',#60890,1.06088080992078);
#7404=VECTOR('',#60897,1.10035806567466);
#7405=VECTOR('',#60904,0.500358065674722);
#7406=VECTOR('',#60911,1.21403156673716);
#7407=VECTOR('',#60918,0.614031566737117);
#7408=VECTOR('',#60925,1.32880796357326);
#7409=VECTOR('',#60932,0.728807963573275);
#7410=VECTOR('',#60939,1.46111700181684);
#7411=VECTOR('',#60946,0.861117001816847);
#7412=VECTOR('',#60953,1.6204820426246);
#7413=VECTOR('',#60960,1.02048204262456);
#7414=VECTOR('',#60967,1.70100022308284);
#7415=VECTOR('',#60974,1.10100022308279);
#7416=VECTOR('',#60981,1.72127463204347);
#7417=VECTOR('',#60988,1.12127463204348);
#7418=VECTOR('',#60995,1.78199265440493);
#7419=VECTOR('',#61002,1.18199265440494);
#7420=VECTOR('',#61009,1.66088080992088);
#7421=VECTOR('',#61016,1.06088080992084);
#7422=VECTOR('',#61023,1.10035806567466);
#7423=VECTOR('',#61030,0.500358065674666);
#7424=VECTOR('',#61037,1.21403156673716);
#7425=VECTOR('',#61044,0.614031566737172);
#7426=VECTOR('',#61051,1.32880796357332);
#7427=VECTOR('',#61058,0.728807963573275);
#7428=VECTOR('',#61065,1.46111700181689);
#7429=VECTOR('',#61072,0.861117001816847);
#7430=VECTOR('',#61079,1.6204820426246);
#7431=VECTOR('',#61086,1.02048204262456);
#7432=VECTOR('',#61093,1.70100022308284);
#7433=VECTOR('',#61100,1.10100022308285);
#7434=VECTOR('',#61107,1.72127463204352);
#7435=VECTOR('',#61114,1.12127463204348);
#7436=VECTOR('',#61121,1.78199265440493);
#7437=VECTOR('',#61128,1.18199265440494);
#7438=VECTOR('',#61135,1.66088080992077);
#7439=VECTOR('',#61142,1.06088080992073);
#7440=VECTOR('',#61149,1.10035806567471);
#7441=VECTOR('',#61156,0.500358065674722);
#7442=VECTOR('',#61163,1.21403156673716);
#7443=VECTOR('',#61170,0.614031566737117);
#7444=VECTOR('',#61177,1.32880796357332);
#7445=VECTOR('',#61184,0.72880796357333);
#7446=VECTOR('',#61191,1.46111700181689);
#7447=VECTOR('',#61198,0.861117001816902);
#7448=VECTOR('',#61205,1.6204820426246);
#7449=VECTOR('',#61212,1.02048204262456);
#7450=VECTOR('',#61219,1.70100022308278);
#7451=VECTOR('',#61226,1.10100022308285);
#7452=VECTOR('',#61233,1.72127463204347);
#7453=VECTOR('',#61240,1.12127463204348);
#7454=VECTOR('',#61247,1.78199265440493);
#7455=VECTOR('',#61254,1.18199265440494);
#7456=VECTOR('',#61261,1.66088080992077);
#7457=VECTOR('',#61268,1.06088080992073);
#7458=VECTOR('',#61275,1.10035806567471);
#7459=VECTOR('',#61282,0.500358065674722);
#7460=VECTOR('',#61289,1.21403156673711);
#7461=VECTOR('',#61296,0.614031566737117);
#7462=VECTOR('',#61303,1.32880796357332);
#7463=VECTOR('',#61310,0.72880796357333);
#7464=VECTOR('',#61317,1.46111700181689);
#7465=VECTOR('',#61324,0.861117001816902);
#7466=VECTOR('',#61331,1.6204820426246);
#7467=VECTOR('',#61338,1.02048204262456);
#7468=VECTOR('',#61345,1.70100022308284);
#7469=VECTOR('',#61352,1.10100022308285);
#7470=VECTOR('',#61359,1.72127463204352);
#7471=VECTOR('',#61366,1.12127463204348);
#7472=VECTOR('',#61373,1.78199265440487);
#7473=VECTOR('',#61380,1.18199265440488);
#7474=VECTOR('',#61387,1.66088080992088);
#7475=VECTOR('',#61394,1.06088080992073);
#7476=VECTOR('',#61401,1.10035806567471);
#7477=VECTOR('',#61408,0.500358065674666);
#7478=VECTOR('',#61415,1.21403156673716);
#7479=VECTOR('',#61422,0.614031566737172);
#7480=VECTOR('',#61429,1.32880796357338);
#7481=VECTOR('',#61436,0.72880796357333);
#7482=VECTOR('',#61443,1.46111700181689);
#7483=VECTOR('',#61450,0.861117001816902);
#7484=VECTOR('',#61457,1.6204820426246);
#7485=VECTOR('',#61464,1.02048204262456);
#7486=VECTOR('',#61471,1.70100022308284);
#7487=VECTOR('',#61478,1.10100022308285);
#7488=VECTOR('',#61485,1.72127463204352);
#7489=VECTOR('',#61492,1.12127463204348);
#7490=VECTOR('',#61499,1.78199265440498);
#7491=VECTOR('',#61506,1.181992654405);
#7492=VECTOR('',#61513,1.66088080992077);
#7493=VECTOR('',#61520,1.06088080992073);
#7494=VECTOR('',#61527,1.10035806567471);
#7495=VECTOR('',#61534,0.500358065674722);
#7496=VECTOR('',#61541,1.21403156673705);
#7497=VECTOR('',#61548,0.614031566737117);
#7498=VECTOR('',#61555,1.32880796357338);
#7499=VECTOR('',#61562,0.72880796357333);
#7500=VECTOR('',#61569,1.46111700181689);
#7501=VECTOR('',#61576,0.861117001816902);
#7502=VECTOR('',#61583,1.6204820426246);
#7503=VECTOR('',#61590,1.02048204262462);
#7504=VECTOR('',#61597,1.70100022308278);
#7505=VECTOR('',#61604,1.10100022308279);
#7506=VECTOR('',#61611,1.72127463204352);
#7507=VECTOR('',#61618,1.12127463204348);
#7508=VECTOR('',#61625,1.78199265440493);
#7509=VECTOR('',#61632,1.18199265440494);
#7510=VECTOR('',#61639,1.66088080992077);
#7511=VECTOR('',#61646,1.06088080992078);
#7512=VECTOR('',#61653,1.10035806567471);
#7513=VECTOR('',#61660,0.500358065674722);
#7514=VECTOR('',#61667,1.21403156673711);
#7515=VECTOR('',#61674,0.614031566737117);
#7516=VECTOR('',#61681,1.32880796357332);
#7517=VECTOR('',#61688,0.72880796357333);
#7518=VECTOR('',#61695,1.46111700181689);
#7519=VECTOR('',#61702,0.861117001816902);
#7520=VECTOR('',#61709,1.62048204262455);
#7521=VECTOR('',#61716,1.02048204262462);
#7522=VECTOR('',#61723,1.70100022308278);
#7523=VECTOR('',#61730,1.10100022308279);
#7524=VECTOR('',#61737,1.72127463204347);
#7525=VECTOR('',#61744,1.12127463204353);
#7526=VECTOR('',#61751,1.78199265440487);
#7527=VECTOR('',#61758,1.18199265440494);
#7528=VECTOR('',#61765,1.66088080992077);
#7529=VECTOR('',#61772,1.06088080992078);
#7530=VECTOR('',#61779,1.10035806567471);
#7531=VECTOR('',#61786,0.500358065674777);
#7532=VECTOR('',#61793,1.21403156673711);
#7533=VECTOR('',#61800,0.614031566737117);
#7534=VECTOR('',#61807,1.32880796357332);
#7535=VECTOR('',#61814,0.728807963573275);
#7536=VECTOR('',#61821,1.46111700181695);
#7537=VECTOR('',#61828,0.861117001816902);
#7538=VECTOR('',#61835,1.6204820426246);
#7539=VECTOR('',#61842,1.02048204262462);
#7540=VECTOR('',#61849,1.70100022308284);
#7541=VECTOR('',#61856,1.10100022308285);
#7542=VECTOR('',#61863,1.72127463204347);
#7543=VECTOR('',#61870,1.12127463204348);
#7544=VECTOR('',#61877,1.78199265440493);
#7545=VECTOR('',#61884,1.18199265440488);
#7546=VECTOR('',#61891,1.66088080992077);
#7547=VECTOR('',#61898,1.06088080992078);
#7548=VECTOR('',#61905,1.10035806567471);
#7549=VECTOR('',#61912,0.500358065674722);
#7550=VECTOR('',#61919,1.21403156673711);
#7551=VECTOR('',#61926,0.614031566737117);
#7552=VECTOR('',#61933,1.32880796357332);
#7553=VECTOR('',#61940,0.72880796357333);
#7554=VECTOR('',#61947,1.46111700181689);
#7555=VECTOR('',#61954,0.861117001816902);
#7556=VECTOR('',#61961,1.62048204262455);
#7557=VECTOR('',#61968,1.02048204262456);
#7558=VECTOR('',#61975,1.70100022308284);
#7559=VECTOR('',#61982,1.10100022308285);
#7560=VECTOR('',#61989,1.72127463204347);
#7561=VECTOR('',#61996,1.12127463204348);
#7562=VECTOR('',#62003,1.78199265440493);
#7563=VECTOR('',#62010,1.18199265440494);
#7564=VECTOR('',#62017,1.66088080992077);
#7565=VECTOR('',#62024,1.06088080992078);
#7566=VECTOR('',#62031,1.10035806567471);
#7567=VECTOR('',#62038,0.500358065674722);
#7568=VECTOR('',#62045,1.21403156673711);
#7569=VECTOR('',#62052,0.614031566737117);
#7570=VECTOR('',#62059,1.32880796357326);
#7571=VECTOR('',#62066,0.728807963573275);
#7572=VECTOR('',#62073,1.46111700181689);
#7573=VECTOR('',#62080,0.861117001816902);
#7574=VECTOR('',#62087,1.6204820426246);
#7575=VECTOR('',#62094,1.02048204262456);
#7576=VECTOR('',#62101,1.70100022308284);
#7577=VECTOR('',#62108,1.10100022308285);
#7578=VECTOR('',#62115,1.72127463204352);
#7579=VECTOR('',#62122,1.12127463204348);
#7580=VECTOR('',#62129,1.78199265440498);
#7581=VECTOR('',#62136,1.18199265440494);
#7582=VECTOR('',#62143,1.66088080992083);
#7583=VECTOR('',#62150,1.06088080992078);
#7584=VECTOR('',#62157,1.10035806567471);
#7585=VECTOR('',#62164,0.500358065674722);
#7586=VECTOR('',#62171,1.21403156673711);
#7587=VECTOR('',#62178,0.614031566737117);
#7588=VECTOR('',#62185,1.32880796357332);
#7589=VECTOR('',#62192,0.72880796357333);
#7590=VECTOR('',#62199,1.46111700181689);
#7591=VECTOR('',#62206,0.861117001816847);
#7592=VECTOR('',#62213,1.6204820426246);
#7593=VECTOR('',#62220,1.02048204262462);
#7594=VECTOR('',#62227,1.70100022308284);
#7595=VECTOR('',#62234,1.10100022308279);
#7596=VECTOR('',#62241,1.72127463204347);
#7597=VECTOR('',#62248,1.12127463204353);
#7598=VECTOR('',#62255,1.78199265440493);
#7599=VECTOR('',#62262,1.18199265440494);
#7600=VECTOR('',#62269,1.66088080992077);
#7601=VECTOR('',#62276,1.06088080992078);
#7602=VECTOR('',#62283,1.10035806567471);
#7603=VECTOR('',#62290,0.500358065674722);
#7604=VECTOR('',#62297,1.21403156673711);
#7605=VECTOR('',#62304,0.614031566737117);
#7606=VECTOR('',#62311,1.32880796357332);
#7607=VECTOR('',#62318,0.72880796357333);
#7608=VECTOR('',#62325,1.46111700181689);
#7609=VECTOR('',#62332,0.861117001816902);
#7610=VECTOR('',#62339,1.6204820426246);
#7611=VECTOR('',#62346,1.02048204262462);
#7612=VECTOR('',#62353,1.70100022308284);
#7613=VECTOR('',#62360,1.10100022308285);
#7614=VECTOR('',#62367,1.72127463204347);
#7615=VECTOR('',#62374,1.12127463204348);
#7616=VECTOR('',#62381,1.78199265440493);
#7617=VECTOR('',#62388,1.18199265440494);
#7618=VECTOR('',#62395,1.66088080992077);
#7619=VECTOR('',#62402,1.06088080992078);
#7620=VECTOR('',#62409,1.10035806567471);
#7621=VECTOR('',#62416,0.500358065674666);
#7622=VECTOR('',#62423,1.21403156673716);
#7623=VECTOR('',#62430,0.614031566737117);
#7624=VECTOR('',#62437,1.32880796357332);
#7625=VECTOR('',#62444,0.72880796357333);
#7626=VECTOR('',#62451,1.46111700181689);
#7627=VECTOR('',#62458,0.861117001816902);
#7628=VECTOR('',#62465,1.6204820426246);
#7629=VECTOR('',#62472,1.02048204262462);
#7630=VECTOR('',#62479,1.70100022308284);
#7631=VECTOR('',#62486,1.10100022308285);
#7632=VECTOR('',#62493,1.72127463204352);
#7633=VECTOR('',#62500,1.12127463204353);
#7634=VECTOR('',#62507,1.78199265440493);
#7635=VECTOR('',#62514,1.18199265440494);
#7636=VECTOR('',#62521,1.66088080992077);
#7637=VECTOR('',#62528,1.06088080992078);
#7638=VECTOR('',#62535,1.10035806567471);
#7639=VECTOR('',#62542,0.500358065674666);
#7640=VECTOR('',#62549,1.21403156673716);
#7641=VECTOR('',#62556,0.614031566737172);
#7642=VECTOR('',#62563,1.32880796357326);
#7643=VECTOR('',#62570,0.728807963573275);
#7644=VECTOR('',#62577,1.46111700181689);
#7645=VECTOR('',#62584,0.861117001816847);
#7646=VECTOR('',#62591,1.62048204262455);
#7647=VECTOR('',#62598,1.02048204262462);
#7648=VECTOR('',#62605,1.70100022308284);
#7649=VECTOR('',#62612,1.10100022308279);
#7650=VECTOR('',#62619,1.72127463204352);
#7651=VECTOR('',#62626,1.12127463204348);
#7652=VECTOR('',#62633,1.78199265440493);
#7653=VECTOR('',#62640,1.18199265440494);
#7654=VECTOR('',#62647,1.66088080992083);
#7655=VECTOR('',#62654,1.06088080992078);
#7656=VECTOR('',#62661,1.10035806567471);
#7657=VECTOR('',#62668,0.500358065674722);
#7658=VECTOR('',#62675,1.21403156673716);
#7659=VECTOR('',#62682,0.614031566737172);
#7660=VECTOR('',#62689,1.32880796357326);
#7661=VECTOR('',#62696,0.72880796357333);
#7662=VECTOR('',#62703,1.46111700181689);
#7663=VECTOR('',#62710,0.861117001816902);
#7664=VECTOR('',#62717,1.6204820426246);
#7665=VECTOR('',#62724,1.02048204262456);
#7666=VECTOR('',#62731,1.70100022308278);
#7667=VECTOR('',#62738,1.10100022308279);
#7668=VECTOR('',#62745,1.72127463204347);
#7669=VECTOR('',#62752,1.12127463204348);
#7670=VECTOR('',#62759,1.78199265440493);
#7671=VECTOR('',#62766,1.18199265440494);
#7672=VECTOR('',#62773,1.66088080992077);
#7673=VECTOR('',#62780,1.06088080992084);
#7674=VECTOR('',#62787,1.10035806567471);
#7675=VECTOR('',#62794,0.500358065674722);
#7676=VECTOR('',#62801,1.21403156673716);
#7677=VECTOR('',#62808,0.614031566737117);
#7678=VECTOR('',#62815,1.32880796357338);
#7679=VECTOR('',#62822,0.728807963573386);
#7680=VECTOR('',#62829,1.46111700181695);
#7681=VECTOR('',#62836,0.861117001816902);
#7682=VECTOR('',#62843,1.6204820426246);
#7683=VECTOR('',#62850,1.02048204262456);
#7684=VECTOR('',#62857,1.70100022308284);
#7685=VECTOR('',#62864,1.10100022308279);
#7686=VECTOR('',#62871,1.72127463204352);
#7687=VECTOR('',#62878,1.12127463204348);
#7688=VECTOR('',#62885,1.78199265440493);
#7689=VECTOR('',#62892,1.18199265440494);
#7690=VECTOR('',#62899,1.66088080992083);
#7691=VECTOR('',#62906,1.06088080992078);
#7692=VECTOR('',#62913,1.10035806567466);
#7693=VECTOR('',#62920,0.500358065674666);
#7694=VECTOR('',#62927,1.21403156673716);
#7695=VECTOR('',#62934,0.614031566737172);
#7696=VECTOR('',#62941,1.32880796357326);
#7697=VECTOR('',#62948,0.728807963573275);
#7698=VECTOR('',#62955,1.46111700181689);
#7699=VECTOR('',#62962,0.861117001816847);
#7700=VECTOR('',#62969,1.6204820426246);
#7701=VECTOR('',#62976,1.02048204262456);
#7702=VECTOR('',#62983,1.70100022308284);
#7703=VECTOR('',#62990,1.10100022308285);
#7704=VECTOR('',#62997,1.72127463204352);
#7705=VECTOR('',#63004,1.12127463204348);
#7706=VECTOR('',#63011,1.78199265440498);
#7707=VECTOR('',#63018,1.18199265440494);
#7708=VECTOR('',#63025,1.66088080992077);
#7709=VECTOR('',#63032,1.06088080992078);
#7710=VECTOR('',#63039,1.10035806567471);
#7711=VECTOR('',#63046,0.500358065674666);
#7712=VECTOR('',#63053,1.21403156673716);
#7713=VECTOR('',#63060,0.614031566737117);
#7714=VECTOR('',#63067,1.32880796357332);
#7715=VECTOR('',#63074,0.72880796357333);
#7716=VECTOR('',#63081,1.46111700181689);
#7717=VECTOR('',#63088,0.861117001816902);
#7718=VECTOR('',#63095,1.62048204262455);
#7719=VECTOR('',#63102,1.02048204262456);
#7720=VECTOR('',#63109,1.70100022308278);
#7721=VECTOR('',#63116,1.10100022308285);
#7722=VECTOR('',#63123,1.72127463204347);
#7723=VECTOR('',#63130,1.12127463204348);
#7724=VECTOR('',#63137,1.78199265440493);
#7725=VECTOR('',#63144,1.18199265440488);
#7726=VECTOR('',#63151,1.66088080992083);
#7727=VECTOR('',#63158,1.06088080992078);
#7728=VECTOR('',#63165,1.10035806567471);
#7729=VECTOR('',#63172,0.500358065674666);
#7730=VECTOR('',#63179,1.21403156673716);
#7731=VECTOR('',#63186,0.614031566737117);
#7732=VECTOR('',#63193,1.32880796357332);
#7733=VECTOR('',#63200,0.72880796357333);
#7734=VECTOR('',#63207,1.46111700181689);
#7735=VECTOR('',#63214,0.861117001816902);
#7736=VECTOR('',#63221,1.6204820426246);
#7737=VECTOR('',#63228,1.02048204262462);
#7738=VECTOR('',#63235,1.70100022308284);
#7739=VECTOR('',#63242,1.10100022308285);
#7740=VECTOR('',#63249,1.72127463204352);
#7741=VECTOR('',#63256,1.12127463204353);
#7742=VECTOR('',#63263,1.78199265440493);
#7743=VECTOR('',#63270,1.18199265440488);
#7744=VECTOR('',#63277,1.66088080992077);
#7745=VECTOR('',#63284,1.06088080992078);
#7746=VECTOR('',#63291,1.10035806567477);
#7747=VECTOR('',#63298,0.500358065674722);
#7748=VECTOR('',#63305,1.21403156673711);
#7749=VECTOR('',#63312,0.614031566737061);
#7750=VECTOR('',#63319,1.32880796357332);
#7751=VECTOR('',#63326,0.728807963573275);
#7752=VECTOR('',#63333,1.46111700181684);
#7753=VECTOR('',#63340,0.861117001816847);
#7754=VECTOR('',#63347,1.6204820426246);
#7755=VECTOR('',#63354,1.02048204262456);
#7756=VECTOR('',#63361,1.70100022308278);
#7757=VECTOR('',#63368,1.10100022308279);
#7758=VECTOR('',#63375,1.72127463204352);
#7759=VECTOR('',#63382,1.12127463204353);
#7760=VECTOR('',#63389,1.78199265440493);
#7761=VECTOR('',#63396,1.18199265440494);
#7762=VECTOR('',#63403,1.66088080992077);
#7763=VECTOR('',#63410,1.06088080992073);
#7764=VECTOR('',#63417,1.10035806567471);
#7765=VECTOR('',#63424,0.500358065674722);
#7766=VECTOR('',#63431,1.21403156673711);
#7767=VECTOR('',#63438,0.614031566737117);
#7768=VECTOR('',#63445,1.32880796357332);
#7769=VECTOR('',#63452,0.728807963573275);
#7770=VECTOR('',#63459,1.46111700181684);
#7771=VECTOR('',#63466,0.861117001816902);
#7772=VECTOR('',#63473,1.6204820426246);
#7773=VECTOR('',#63480,1.02048204262462);
#7774=VECTOR('',#63487,1.70100022308289);
#7775=VECTOR('',#63494,1.10100022308285);
#7776=VECTOR('',#63501,1.72127463204347);
#7777=VECTOR('',#63508,1.12127463204342);
#7778=VECTOR('',#63515,1.78199265440498);
#7779=VECTOR('',#63522,1.18199265440494);
#7780=VECTOR('',#63529,1.66088080992077);
#7781=VECTOR('',#63536,1.06088080992078);
#7782=VECTOR('',#63543,1.10035806567471);
#7783=VECTOR('',#63550,0.500358065674666);
#7784=VECTOR('',#63557,1.21403156673711);
#7785=VECTOR('',#63564,0.614031566737117);
#7786=VECTOR('',#63571,1.32880796357332);
#7787=VECTOR('',#63578,0.72880796357333);
#7788=VECTOR('',#63585,1.46111700181684);
#7789=VECTOR('',#63592,0.861117001816847);
#7790=VECTOR('',#63599,1.6204820426246);
#7791=VECTOR('',#63606,1.02048204262456);
#7792=VECTOR('',#63613,1.70100022308284);
#7793=VECTOR('',#63620,1.10100022308285);
#7794=VECTOR('',#63627,1.72127463204347);
#7795=VECTOR('',#63634,1.12127463204353);
#7796=VECTOR('',#63641,1.78199265440498);
#7797=VECTOR('',#63648,1.18199265440494);
#7798=VECTOR('',#63655,1.66088080992083);
#7799=VECTOR('',#63662,1.06088080992078);
#7800=VECTOR('',#63669,1.10035806567477);
#7801=VECTOR('',#63676,0.500358065674777);
#7802=VECTOR('',#63683,1.21403156673705);
#7803=VECTOR('',#63690,0.614031566737117);
#7804=VECTOR('',#63697,1.32880796357326);
#7805=VECTOR('',#63704,0.728807963573275);
#7806=VECTOR('',#63711,1.46111700181684);
#7807=VECTOR('',#63718,0.861117001816847);
#7808=VECTOR('',#63725,1.6204820426246);
#7809=VECTOR('',#63732,1.02048204262462);
#7810=VECTOR('',#63739,1.70100022308278);
#7811=VECTOR('',#63746,1.10100022308285);
#7812=VECTOR('',#63753,1.72127463204347);
#7813=VECTOR('',#63760,1.12127463204353);
#7814=VECTOR('',#63767,1.78199265440493);
#7815=VECTOR('',#63774,1.18199265440494);
#7816=VECTOR('',#63781,1.66088080992077);
#7817=VECTOR('',#63788,1.06088080992078);
#7818=VECTOR('',#63795,1.10035806567471);
#7819=VECTOR('',#63802,0.500358065674722);
#7820=VECTOR('',#63809,1.21403156673716);
#7821=VECTOR('',#63816,0.614031566737117);
#7822=VECTOR('',#63823,1.32880796357332);
#7823=VECTOR('',#63830,0.72880796357333);
#7824=VECTOR('',#63837,1.46111700181689);
#7825=VECTOR('',#63844,0.861117001816902);
#7826=VECTOR('',#63851,1.6204820426246);
#7827=VECTOR('',#63858,1.02048204262462);
#7828=VECTOR('',#63865,1.70100022308284);
#7829=VECTOR('',#63872,1.10100022308285);
#7830=VECTOR('',#63879,1.72127463204352);
#7831=VECTOR('',#63886,1.12127463204348);
#7832=VECTOR('',#63893,1.78199265440493);
#7833=VECTOR('',#63900,1.18199265440488);
#7834=VECTOR('',#63907,1.66088080992088);
#7835=VECTOR('',#63914,1.06088080992084);
#7836=VECTOR('',#63921,1.10035806567471);
#7837=VECTOR('',#63928,0.500358065674722);
#7838=VECTOR('',#63935,1.21403156673716);
#7839=VECTOR('',#63942,0.614031566737117);
#7840=VECTOR('',#63949,1.32880796357332);
#7841=VECTOR('',#63956,0.72880796357333);
#7842=VECTOR('',#63963,1.46111700181689);
#7843=VECTOR('',#63970,0.861117001816902);
#7844=VECTOR('',#63977,1.6204820426246);
#7845=VECTOR('',#63984,1.02048204262462);
#7846=VECTOR('',#63991,1.70100022308284);
#7847=VECTOR('',#63998,1.10100022308285);
#7848=VECTOR('',#64005,1.72127463204352);
#7849=VECTOR('',#64012,1.12127463204348);
#7850=VECTOR('',#64019,1.78199265440493);
#7851=VECTOR('',#64026,1.18199265440494);
#7852=VECTOR('',#64033,1.66088080992077);
#7853=VECTOR('',#64040,1.06088080992078);
#7854=VECTOR('',#64053,127.41606204049);
#7855=VECTOR('',#64076,12.3670707361132);
#7856=VECTOR('',#64107,18.5103550292801);
#7857=VECTOR('',#64120,130.);
#7858=VECTOR('',#64123,0.878303132193281);
#7859=VECTOR('',#64128,1.47830313219333);
#8684=CYLINDRICAL_SURFACE('',#48909,1.27544412113617);
#8685=CYLINDRICAL_SURFACE('',#48910,0.675444121136126);
#8686=CYLINDRICAL_SURFACE('',#48912,1.09883113599246);
#8687=CYLINDRICAL_SURFACE('',#48913,0.498831135992472);
#8688=CYLINDRICAL_SURFACE('',#48915,1.09054074872833);
#8689=CYLINDRICAL_SURFACE('',#48916,0.490540748728341);
#8690=CYLINDRICAL_SURFACE('',#48918,1.47830313219327);
#8691=CYLINDRICAL_SURFACE('',#48919,0.878303132193281);
#8692=CYLINDRICAL_SURFACE('',#48921,1.27544412113612);
#8693=CYLINDRICAL_SURFACE('',#48922,0.675444121136182);
#8694=CYLINDRICAL_SURFACE('',#48924,1.09883113599246);
#8695=CYLINDRICAL_SURFACE('',#48925,0.498831135992472);
#8696=CYLINDRICAL_SURFACE('',#48927,1.09054074872833);
#8697=CYLINDRICAL_SURFACE('',#48928,0.490540748728341);
#8698=CYLINDRICAL_SURFACE('',#48930,1.47830313219333);
#8699=CYLINDRICAL_SURFACE('',#48931,0.878303132193337);
#8700=CYLINDRICAL_SURFACE('',#48933,1.27544412113617);
#8701=CYLINDRICAL_SURFACE('',#48934,0.675444121136126);
#8702=CYLINDRICAL_SURFACE('',#48936,1.09883113599246);
#8703=CYLINDRICAL_SURFACE('',#48937,0.498831135992472);
#8704=CYLINDRICAL_SURFACE('',#48939,1.09054074872833);
#8705=CYLINDRICAL_SURFACE('',#48940,0.490540748728341);
#8706=CYLINDRICAL_SURFACE('',#48942,1.47830313219327);
#8707=CYLINDRICAL_SURFACE('',#48943,0.878303132193281);
#8708=CYLINDRICAL_SURFACE('',#48945,1.27544412113617);
#8709=CYLINDRICAL_SURFACE('',#48946,0.675444121136126);
#8710=CYLINDRICAL_SURFACE('',#48948,1.09883113599246);
#8711=CYLINDRICAL_SURFACE('',#48949,0.498831135992472);
#8712=CYLINDRICAL_SURFACE('',#48951,1.09054074872833);
#8713=CYLINDRICAL_SURFACE('',#48952,0.490540748728285);
#8714=CYLINDRICAL_SURFACE('',#48954,1.47830313219327);
#8715=CYLINDRICAL_SURFACE('',#48955,0.878303132193226);
#8716=CYLINDRICAL_SURFACE('',#48957,1.27544412113617);
#8717=CYLINDRICAL_SURFACE('',#48958,0.675444121136182);
#8718=CYLINDRICAL_SURFACE('',#48960,1.09883113599246);
#8719=CYLINDRICAL_SURFACE('',#48961,0.498831135992472);
#8720=CYLINDRICAL_SURFACE('',#48963,1.09054074872833);
#8721=CYLINDRICAL_SURFACE('',#48964,0.490540748728341);
#8722=CYLINDRICAL_SURFACE('',#48966,1.47830313219333);
#8723=CYLINDRICAL_SURFACE('',#48967,0.878303132193281);
#8724=CYLINDRICAL_SURFACE('',#48969,1.27544412113612);
#8725=CYLINDRICAL_SURFACE('',#48970,0.675444121136182);
#8726=CYLINDRICAL_SURFACE('',#48972,1.09883113599241);
#8727=CYLINDRICAL_SURFACE('',#48973,0.498831135992472);
#8728=CYLINDRICAL_SURFACE('',#48975,1.09054074872839);
#8729=CYLINDRICAL_SURFACE('',#48976,0.490540748728341);
#8730=CYLINDRICAL_SURFACE('',#48978,1.47830313219333);
#8731=CYLINDRICAL_SURFACE('',#48979,0.878303132193281);
#8732=CYLINDRICAL_SURFACE('',#48981,1.27544412113612);
#8733=CYLINDRICAL_SURFACE('',#48982,0.675444121136182);
#8734=CYLINDRICAL_SURFACE('',#48984,1.09883113599252);
#8735=CYLINDRICAL_SURFACE('',#48985,0.498831135992583);
#8736=CYLINDRICAL_SURFACE('',#48987,1.09054074872827);
#8737=CYLINDRICAL_SURFACE('',#48988,0.490540748728341);
#8738=CYLINDRICAL_SURFACE('',#48990,1.47830313219321);
#8739=CYLINDRICAL_SURFACE('',#48991,0.87830313219317);
#8740=CYLINDRICAL_SURFACE('',#48993,1.27544412113612);
#8741=CYLINDRICAL_SURFACE('',#48994,0.675444121136071);
#8742=CYLINDRICAL_SURFACE('',#48996,1.09883113599252);
#8743=CYLINDRICAL_SURFACE('',#48997,0.498831135992472);
#8744=CYLINDRICAL_SURFACE('',#48999,1.09054074872839);
#8745=CYLINDRICAL_SURFACE('',#49000,0.490540748728341);
#8746=CYLINDRICAL_SURFACE('',#49002,1.47830313219321);
#8747=CYLINDRICAL_SURFACE('',#49003,0.87830313219317);
#8748=CYLINDRICAL_SURFACE('',#49005,1.27544412113612);
#8749=CYLINDRICAL_SURFACE('',#49006,0.675444121136071);
#8750=CYLINDRICAL_SURFACE('',#49008,1.09883113599241);
#8751=CYLINDRICAL_SURFACE('',#49009,0.498831135992361);
#8752=CYLINDRICAL_SURFACE('',#49011,1.09054074872839);
#8753=CYLINDRICAL_SURFACE('',#49012,0.490540748728341);
#8754=CYLINDRICAL_SURFACE('',#49014,1.47830313219333);
#8755=CYLINDRICAL_SURFACE('',#49015,0.878303132193281);
#8756=CYLINDRICAL_SURFACE('',#49017,1.27544412113612);
#8757=CYLINDRICAL_SURFACE('',#49018,0.675444121136182);
#8758=CYLINDRICAL_SURFACE('',#49020,1.09883113599252);
#8759=CYLINDRICAL_SURFACE('',#49021,0.498831135992472);
#8760=CYLINDRICAL_SURFACE('',#49023,1.09054074872827);
#8761=CYLINDRICAL_SURFACE('',#49024,0.49054074872823);
#8762=CYLINDRICAL_SURFACE('',#49026,1.47830313219333);
#8763=CYLINDRICAL_SURFACE('',#49027,0.878303132193281);
#8764=CYLINDRICAL_SURFACE('',#49029,1.27544412113623);
#8765=CYLINDRICAL_SURFACE('',#49030,0.675444121136182);
#8766=CYLINDRICAL_SURFACE('',#49032,1.09883113599252);
#8767=CYLINDRICAL_SURFACE('',#49033,0.498831135992472);
#8768=CYLINDRICAL_SURFACE('',#49035,1.09054074872827);
#8769=CYLINDRICAL_SURFACE('',#49036,0.490540748728341);
#8770=CYLINDRICAL_SURFACE('',#49038,1.47830313219333);
#8771=CYLINDRICAL_SURFACE('',#49039,0.878303132193281);
#8772=CYLINDRICAL_SURFACE('',#49041,1.27544412113617);
#8773=CYLINDRICAL_SURFACE('',#49042,0.675444121136126);
#8774=CYLINDRICAL_SURFACE('',#49044,1.09883113599252);
#8775=CYLINDRICAL_SURFACE('',#49045,0.498831135992472);
#8776=CYLINDRICAL_SURFACE('',#49047,1.09054074872839);
#8777=CYLINDRICAL_SURFACE('',#49048,0.490540748728341);
#8778=CYLINDRICAL_SURFACE('',#49050,1.47830313219327);
#8779=CYLINDRICAL_SURFACE('',#49051,0.878303132193281);
#8780=CYLINDRICAL_SURFACE('',#49053,1.27544412113617);
#8781=CYLINDRICAL_SURFACE('',#49054,0.675444121136182);
#8782=CYLINDRICAL_SURFACE('',#49056,1.09883113599246);
#8783=CYLINDRICAL_SURFACE('',#49057,0.498831135992417);
#8784=CYLINDRICAL_SURFACE('',#49059,1.09054074872827);
#8785=CYLINDRICAL_SURFACE('',#49060,0.490540748728341);
#8786=CYLINDRICAL_SURFACE('',#49062,1.47830313219327);
#8787=CYLINDRICAL_SURFACE('',#49063,0.878303132193281);
#8788=CYLINDRICAL_SURFACE('',#49065,1.27544412113612);
#8789=CYLINDRICAL_SURFACE('',#49066,0.675444121136126);
#8790=CYLINDRICAL_SURFACE('',#49068,1.09883113599241);
#8791=CYLINDRICAL_SURFACE('',#49069,0.498831135992417);
#8792=CYLINDRICAL_SURFACE('',#49071,1.09054074872839);
#8793=CYLINDRICAL_SURFACE('',#49072,0.490540748728341);
#8794=CYLINDRICAL_SURFACE('',#49074,1.47830313219333);
#8795=CYLINDRICAL_SURFACE('',#49075,0.878303132193337);
#8796=CYLINDRICAL_SURFACE('',#49077,1.27544412113617);
#8797=CYLINDRICAL_SURFACE('',#49078,0.675444121136182);
#8798=CYLINDRICAL_SURFACE('',#49080,1.09883113599246);
#8799=CYLINDRICAL_SURFACE('',#49081,0.498831135992417);
#8800=CYLINDRICAL_SURFACE('',#49083,1.09054074872833);
#8801=CYLINDRICAL_SURFACE('',#49084,0.490540748728341);
#8802=CYLINDRICAL_SURFACE('',#49086,1.47830313219333);
#8803=CYLINDRICAL_SURFACE('',#49087,0.878303132193337);
#8804=CYLINDRICAL_SURFACE('',#49089,1.27544412113617);
#8805=CYLINDRICAL_SURFACE('',#49090,0.675444121136126);
#8806=CYLINDRICAL_SURFACE('',#49092,1.09883113599246);
#8807=CYLINDRICAL_SURFACE('',#49093,0.498831135992472);
#8808=CYLINDRICAL_SURFACE('',#49095,1.09054074872833);
#8809=CYLINDRICAL_SURFACE('',#49096,0.490540748728341);
#8810=CYLINDRICAL_SURFACE('',#49098,1.47830313219333);
#8811=CYLINDRICAL_SURFACE('',#49099,0.878303132193281);
#8812=CYLINDRICAL_SURFACE('',#49101,1.27544412113617);
#8813=CYLINDRICAL_SURFACE('',#49102,0.675444121136182);
#8814=CYLINDRICAL_SURFACE('',#49104,1.09883113599246);
#8815=CYLINDRICAL_SURFACE('',#49105,0.498831135992472);
#8816=CYLINDRICAL_SURFACE('',#49107,1.09054074872833);
#8817=CYLINDRICAL_SURFACE('',#49108,0.490540748728341);
#8818=CYLINDRICAL_SURFACE('',#49110,1.47830313219333);
#8819=CYLINDRICAL_SURFACE('',#49111,0.878303132193281);
#8820=CYLINDRICAL_SURFACE('',#49113,1.27544412113617);
#8821=CYLINDRICAL_SURFACE('',#49114,0.675444121136182);
#8822=CYLINDRICAL_SURFACE('',#49116,1.09883113599246);
#8823=CYLINDRICAL_SURFACE('',#49117,0.498831135992472);
#8824=CYLINDRICAL_SURFACE('',#49119,1.09054074872833);
#8825=CYLINDRICAL_SURFACE('',#49120,0.490540748728341);
#8826=CYLINDRICAL_SURFACE('',#49122,1.47830313219333);
#8827=CYLINDRICAL_SURFACE('',#49123,0.878303132193281);
#8828=CYLINDRICAL_SURFACE('',#49125,1.27544412113612);
#8829=CYLINDRICAL_SURFACE('',#49126,0.675444121136126);
#8830=CYLINDRICAL_SURFACE('',#49128,1.09883113599252);
#8831=CYLINDRICAL_SURFACE('',#49129,0.498831135992472);
#8832=CYLINDRICAL_SURFACE('',#49131,1.09054074872833);
#8833=CYLINDRICAL_SURFACE('',#49132,0.490540748728341);
#8834=CYLINDRICAL_SURFACE('',#49134,1.47830313219333);
#8835=CYLINDRICAL_SURFACE('',#49135,0.878303132193337);
#8836=CYLINDRICAL_SURFACE('',#49137,1.27544412113617);
#8837=CYLINDRICAL_SURFACE('',#49138,0.675444121136126);
#8838=CYLINDRICAL_SURFACE('',#49140,1.09883113599246);
#8839=CYLINDRICAL_SURFACE('',#49141,0.498831135992472);
#8840=CYLINDRICAL_SURFACE('',#49143,1.09054074872833);
#8841=CYLINDRICAL_SURFACE('',#49144,0.490540748728341);
#8842=CYLINDRICAL_SURFACE('',#49146,1.47830313219327);
#8843=CYLINDRICAL_SURFACE('',#49147,0.878303132193281);
#8844=CYLINDRICAL_SURFACE('',#49149,1.27544412113617);
#8845=CYLINDRICAL_SURFACE('',#49150,0.675444121136182);
#8846=CYLINDRICAL_SURFACE('',#49152,1.09883113599246);
#8847=CYLINDRICAL_SURFACE('',#49153,0.498831135992472);
#8848=CYLINDRICAL_SURFACE('',#49155,1.09054074872827);
#8849=CYLINDRICAL_SURFACE('',#49156,0.490540748728341);
#8850=CYLINDRICAL_SURFACE('',#49158,1.47830313219327);
#8851=CYLINDRICAL_SURFACE('',#49159,0.878303132193281);
#8852=CYLINDRICAL_SURFACE('',#49161,1.27544412113617);
#8853=CYLINDRICAL_SURFACE('',#49162,0.675444121136126);
#8854=CYLINDRICAL_SURFACE('',#49164,1.09883113599241);
#8855=CYLINDRICAL_SURFACE('',#49165,0.498831135992472);
#8856=CYLINDRICAL_SURFACE('',#49167,1.09054074872827);
#8857=CYLINDRICAL_SURFACE('',#49168,0.490540748728341);
#8858=CYLINDRICAL_SURFACE('',#49170,1.47830313219327);
#8859=CYLINDRICAL_SURFACE('',#49171,0.878303132193281);
#8860=CYLINDRICAL_SURFACE('',#49173,1.27544412113617);
#8861=CYLINDRICAL_SURFACE('',#49174,0.675444121136126);
#8862=CYLINDRICAL_SURFACE('',#49176,1.09883113599252);
#8863=CYLINDRICAL_SURFACE('',#49177,0.498831135992472);
#8864=CYLINDRICAL_SURFACE('',#49179,1.09054074872839);
#8865=CYLINDRICAL_SURFACE('',#49180,0.490540748728396);
#8866=CYLINDRICAL_SURFACE('',#49182,1.47830313219327);
#8867=CYLINDRICAL_SURFACE('',#49183,0.878303132193281);
#8868=CYLINDRICAL_SURFACE('',#49185,1.27544412113612);
#8869=CYLINDRICAL_SURFACE('',#49186,0.675444121136126);
#8870=CYLINDRICAL_SURFACE('',#49188,1.09883113599241);
#8871=CYLINDRICAL_SURFACE('',#49189,0.498831135992417);
#8872=CYLINDRICAL_SURFACE('',#49191,1.09054074872833);
#8873=CYLINDRICAL_SURFACE('',#49192,0.490540748728341);
#8874=CYLINDRICAL_SURFACE('',#49194,1.47830313219327);
#8875=CYLINDRICAL_SURFACE('',#49195,0.878303132193281);
#8876=CYLINDRICAL_SURFACE('',#49197,1.27544412113617);
#8877=CYLINDRICAL_SURFACE('',#49198,0.675444121136126);
#8878=CYLINDRICAL_SURFACE('',#49200,1.09883113599241);
#8879=CYLINDRICAL_SURFACE('',#49201,0.498831135992472);
#8880=CYLINDRICAL_SURFACE('',#49203,1.09054074872839);
#8881=CYLINDRICAL_SURFACE('',#49204,0.490540748728396);
#8882=CYLINDRICAL_SURFACE('',#49206,1.47830313219327);
#8883=CYLINDRICAL_SURFACE('',#49207,0.878303132193281);
#8884=CYLINDRICAL_SURFACE('',#49209,1.27544412113617);
#8885=CYLINDRICAL_SURFACE('',#49210,0.675444121136182);
#8886=CYLINDRICAL_SURFACE('',#49212,1.09883113599246);
#8887=CYLINDRICAL_SURFACE('',#49213,0.498831135992528);
#8888=CYLINDRICAL_SURFACE('',#49215,1.09054074872833);
#8889=CYLINDRICAL_SURFACE('',#49216,0.490540748728341);
#8890=CYLINDRICAL_SURFACE('',#49218,1.47830313219333);
#8891=CYLINDRICAL_SURFACE('',#49219,0.878303132193337);
#8892=CYLINDRICAL_SURFACE('',#49221,1.27544412113617);
#8893=CYLINDRICAL_SURFACE('',#49222,0.675444121136126);
#8894=CYLINDRICAL_SURFACE('',#49224,1.09883113599246);
#8895=CYLINDRICAL_SURFACE('',#49225,0.498831135992472);
#8896=CYLINDRICAL_SURFACE('',#49227,1.09054074872839);
#8897=CYLINDRICAL_SURFACE('',#49228,0.490540748728285);
#8898=CYLINDRICAL_SURFACE('',#49230,1.47830313219327);
#8899=CYLINDRICAL_SURFACE('',#49231,0.878303132193281);
#8900=CYLINDRICAL_SURFACE('',#49233,1.27544412113617);
#8901=CYLINDRICAL_SURFACE('',#49234,0.675444121136126);
#8902=CYLINDRICAL_SURFACE('',#49236,1.09883113599246);
#8903=CYLINDRICAL_SURFACE('',#49237,0.498831135992528);
#8904=CYLINDRICAL_SURFACE('',#49239,1.09054074872833);
#8905=CYLINDRICAL_SURFACE('',#49240,0.490540748728341);
#8906=CYLINDRICAL_SURFACE('',#49242,1.47830313219333);
#8907=CYLINDRICAL_SURFACE('',#49243,0.878303132193337);
#8908=CYLINDRICAL_SURFACE('',#49245,1.27544412113617);
#8909=CYLINDRICAL_SURFACE('',#49246,0.675444121136182);
#8910=CYLINDRICAL_SURFACE('',#49248,1.09883113599246);
#8911=CYLINDRICAL_SURFACE('',#49249,0.498831135992472);
#8912=CYLINDRICAL_SURFACE('',#49251,1.09054074872833);
#8913=CYLINDRICAL_SURFACE('',#49252,0.490540748728285);
#8914=CYLINDRICAL_SURFACE('',#49254,1.47830313219327);
#8915=CYLINDRICAL_SURFACE('',#49255,0.878303132193281);
#8916=CYLINDRICAL_SURFACE('',#49257,1.27544412113617);
#8917=CYLINDRICAL_SURFACE('',#49258,0.675444121136126);
#8918=CYLINDRICAL_SURFACE('',#49260,1.09054074872833);
#8919=CYLINDRICAL_SURFACE('',#49261,0.490540748728341);
#8920=CYLINDRICAL_SURFACE('',#49263,1.09883113599252);
#8921=CYLINDRICAL_SURFACE('',#49264,0.498831135992472);
#8922=CYLINDRICAL_SURFACE('',#49266,1.10035806567471);
#8923=CYLINDRICAL_SURFACE('',#49269,0.500358065674722);
#8924=CYLINDRICAL_SURFACE('',#49272,1.21403156673711);
#8925=CYLINDRICAL_SURFACE('',#49275,0.614031566737117);
#8926=CYLINDRICAL_SURFACE('',#49278,1.32880796357332);
#8927=CYLINDRICAL_SURFACE('',#49281,0.72880796357333);
#8928=CYLINDRICAL_SURFACE('',#49284,1.46111700181689);
#8929=CYLINDRICAL_SURFACE('',#49287,0.861117001816902);
#8930=CYLINDRICAL_SURFACE('',#49290,1.6204820426246);
#8931=CYLINDRICAL_SURFACE('',#49293,1.02048204262462);
#8932=CYLINDRICAL_SURFACE('',#49296,1.70100022308284);
#8933=CYLINDRICAL_SURFACE('',#49299,1.10100022308285);
#8934=CYLINDRICAL_SURFACE('',#49302,1.72127463204352);
#8935=CYLINDRICAL_SURFACE('',#49305,1.12127463204348);
#8936=CYLINDRICAL_SURFACE('',#49308,1.78199265440493);
#8937=CYLINDRICAL_SURFACE('',#49311,1.18199265440494);
#8938=CYLINDRICAL_SURFACE('',#49314,1.66088080992077);
#8939=CYLINDRICAL_SURFACE('',#49317,1.06088080992078);
#8940=CYLINDRICAL_SURFACE('',#49320,1.10035806567471);
#8941=CYLINDRICAL_SURFACE('',#49323,0.500358065674722);
#8942=CYLINDRICAL_SURFACE('',#49326,1.21403156673716);
#8943=CYLINDRICAL_SURFACE('',#49329,0.614031566737117);
#8944=CYLINDRICAL_SURFACE('',#49332,1.32880796357332);
#8945=CYLINDRICAL_SURFACE('',#49335,0.728807963573275);
#8946=CYLINDRICAL_SURFACE('',#49338,1.46111700181689);
#8947=CYLINDRICAL_SURFACE('',#49341,0.861117001816902);
#8948=CYLINDRICAL_SURFACE('',#49344,1.6204820426246);
#8949=CYLINDRICAL_SURFACE('',#49347,1.02048204262462);
#8950=CYLINDRICAL_SURFACE('',#49350,1.70100022308284);
#8951=CYLINDRICAL_SURFACE('',#49353,1.10100022308285);
#8952=CYLINDRICAL_SURFACE('',#49356,1.72127463204347);
#8953=CYLINDRICAL_SURFACE('',#49359,1.12127463204348);
#8954=CYLINDRICAL_SURFACE('',#49362,1.78199265440493);
#8955=CYLINDRICAL_SURFACE('',#49365,1.18199265440494);
#8956=CYLINDRICAL_SURFACE('',#49368,1.66088080992077);
#8957=CYLINDRICAL_SURFACE('',#49371,1.06088080992078);
#8958=CYLINDRICAL_SURFACE('',#49374,1.10035806567471);
#8959=CYLINDRICAL_SURFACE('',#49377,0.500358065674722);
#8960=CYLINDRICAL_SURFACE('',#49380,1.21403156673716);
#8961=CYLINDRICAL_SURFACE('',#49383,0.614031566737117);
#8962=CYLINDRICAL_SURFACE('',#49386,1.32880796357326);
#8963=CYLINDRICAL_SURFACE('',#49389,0.72880796357333);
#8964=CYLINDRICAL_SURFACE('',#49392,1.46111700181689);
#8965=CYLINDRICAL_SURFACE('',#49395,0.861117001816902);
#8966=CYLINDRICAL_SURFACE('',#49398,1.6204820426246);
#8967=CYLINDRICAL_SURFACE('',#49401,1.02048204262456);
#8968=CYLINDRICAL_SURFACE('',#49404,1.70100022308284);
#8969=CYLINDRICAL_SURFACE('',#49407,1.10100022308285);
#8970=CYLINDRICAL_SURFACE('',#49410,1.72127463204347);
#8971=CYLINDRICAL_SURFACE('',#49413,1.12127463204348);
#8972=CYLINDRICAL_SURFACE('',#49416,1.78199265440493);
#8973=CYLINDRICAL_SURFACE('',#49419,1.18199265440494);
#8974=CYLINDRICAL_SURFACE('',#49422,1.66088080992077);
#8975=CYLINDRICAL_SURFACE('',#49425,1.06088080992078);
#8976=CYLINDRICAL_SURFACE('',#49428,1.10035806567471);
#8977=CYLINDRICAL_SURFACE('',#49431,0.500358065674666);
#8978=CYLINDRICAL_SURFACE('',#49434,1.21403156673711);
#8979=CYLINDRICAL_SURFACE('',#49437,0.614031566737172);
#8980=CYLINDRICAL_SURFACE('',#49440,1.32880796357332);
#8981=CYLINDRICAL_SURFACE('',#49443,0.72880796357333);
#8982=CYLINDRICAL_SURFACE('',#49446,1.46111700181689);
#8983=CYLINDRICAL_SURFACE('',#49449,0.861117001816847);
#8984=CYLINDRICAL_SURFACE('',#49452,1.6204820426246);
#8985=CYLINDRICAL_SURFACE('',#49455,1.02048204262462);
#8986=CYLINDRICAL_SURFACE('',#49458,1.70100022308284);
#8987=CYLINDRICAL_SURFACE('',#49461,1.10100022308285);
#8988=CYLINDRICAL_SURFACE('',#49464,1.72127463204347);
#8989=CYLINDRICAL_SURFACE('',#49467,1.12127463204353);
#8990=CYLINDRICAL_SURFACE('',#49470,1.78199265440498);
#8991=CYLINDRICAL_SURFACE('',#49473,1.18199265440494);
#8992=CYLINDRICAL_SURFACE('',#49476,1.66088080992083);
#8993=CYLINDRICAL_SURFACE('',#49479,1.06088080992078);
#8994=CYLINDRICAL_SURFACE('',#49482,1.10035806567477);
#8995=CYLINDRICAL_SURFACE('',#49485,0.500358065674777);
#8996=CYLINDRICAL_SURFACE('',#49488,1.21403156673711);
#8997=CYLINDRICAL_SURFACE('',#49491,0.614031566737172);
#8998=CYLINDRICAL_SURFACE('',#49494,1.32880796357326);
#8999=CYLINDRICAL_SURFACE('',#49497,0.72880796357333);
#9000=CYLINDRICAL_SURFACE('',#49500,1.46111700181684);
#9001=CYLINDRICAL_SURFACE('',#49503,0.861117001816847);
#9002=CYLINDRICAL_SURFACE('',#49506,1.6204820426246);
#9003=CYLINDRICAL_SURFACE('',#49509,1.02048204262462);
#9004=CYLINDRICAL_SURFACE('',#49512,1.70100022308278);
#9005=CYLINDRICAL_SURFACE('',#49515,1.1010002230829);
#9006=CYLINDRICAL_SURFACE('',#49518,1.72127463204347);
#9007=CYLINDRICAL_SURFACE('',#49521,1.12127463204342);
#9008=CYLINDRICAL_SURFACE('',#49524,1.78199265440487);
#9009=CYLINDRICAL_SURFACE('',#49527,1.18199265440488);
#9010=CYLINDRICAL_SURFACE('',#49530,1.66088080992077);
#9011=CYLINDRICAL_SURFACE('',#49533,1.06088080992078);
#9012=CYLINDRICAL_SURFACE('',#49536,1.10035806567466);
#9013=CYLINDRICAL_SURFACE('',#49539,0.500358065674722);
#9014=CYLINDRICAL_SURFACE('',#49542,1.21403156673716);
#9015=CYLINDRICAL_SURFACE('',#49545,0.614031566737117);
#9016=CYLINDRICAL_SURFACE('',#49548,1.32880796357326);
#9017=CYLINDRICAL_SURFACE('',#49551,0.728807963573275);
#9018=CYLINDRICAL_SURFACE('',#49554,1.46111700181684);
#9019=CYLINDRICAL_SURFACE('',#49557,0.861117001816847);
#9020=CYLINDRICAL_SURFACE('',#49560,1.6204820426246);
#9021=CYLINDRICAL_SURFACE('',#49563,1.02048204262456);
#9022=CYLINDRICAL_SURFACE('',#49566,1.70100022308284);
#9023=CYLINDRICAL_SURFACE('',#49569,1.10100022308279);
#9024=CYLINDRICAL_SURFACE('',#49572,1.72127463204347);
#9025=CYLINDRICAL_SURFACE('',#49575,1.12127463204348);
#9026=CYLINDRICAL_SURFACE('',#49578,1.78199265440493);
#9027=CYLINDRICAL_SURFACE('',#49581,1.18199265440494);
#9028=CYLINDRICAL_SURFACE('',#49584,1.66088080992088);
#9029=CYLINDRICAL_SURFACE('',#49587,1.06088080992084);
#9030=CYLINDRICAL_SURFACE('',#49590,1.10035806567466);
#9031=CYLINDRICAL_SURFACE('',#49593,0.500358065674666);
#9032=CYLINDRICAL_SURFACE('',#49596,1.21403156673716);
#9033=CYLINDRICAL_SURFACE('',#49599,0.614031566737172);
#9034=CYLINDRICAL_SURFACE('',#49602,1.32880796357332);
#9035=CYLINDRICAL_SURFACE('',#49605,0.728807963573275);
#9036=CYLINDRICAL_SURFACE('',#49608,1.46111700181689);
#9037=CYLINDRICAL_SURFACE('',#49611,0.861117001816847);
#9038=CYLINDRICAL_SURFACE('',#49614,1.6204820426246);
#9039=CYLINDRICAL_SURFACE('',#49617,1.02048204262456);
#9040=CYLINDRICAL_SURFACE('',#49620,1.70100022308284);
#9041=CYLINDRICAL_SURFACE('',#49623,1.10100022308285);
#9042=CYLINDRICAL_SURFACE('',#49626,1.72127463204352);
#9043=CYLINDRICAL_SURFACE('',#49629,1.12127463204348);
#9044=CYLINDRICAL_SURFACE('',#49632,1.78199265440493);
#9045=CYLINDRICAL_SURFACE('',#49635,1.18199265440494);
#9046=CYLINDRICAL_SURFACE('',#49638,1.66088080992077);
#9047=CYLINDRICAL_SURFACE('',#49641,1.06088080992073);
#9048=CYLINDRICAL_SURFACE('',#49644,1.10035806567471);
#9049=CYLINDRICAL_SURFACE('',#49647,0.500358065674722);
#9050=CYLINDRICAL_SURFACE('',#49650,1.21403156673716);
#9051=CYLINDRICAL_SURFACE('',#49653,0.614031566737117);
#9052=CYLINDRICAL_SURFACE('',#49656,1.32880796357332);
#9053=CYLINDRICAL_SURFACE('',#49659,0.72880796357333);
#9054=CYLINDRICAL_SURFACE('',#49662,1.46111700181689);
#9055=CYLINDRICAL_SURFACE('',#49665,0.861117001816902);
#9056=CYLINDRICAL_SURFACE('',#49668,1.6204820426246);
#9057=CYLINDRICAL_SURFACE('',#49671,1.02048204262456);
#9058=CYLINDRICAL_SURFACE('',#49674,1.70100022308278);
#9059=CYLINDRICAL_SURFACE('',#49677,1.10100022308285);
#9060=CYLINDRICAL_SURFACE('',#49680,1.72127463204347);
#9061=CYLINDRICAL_SURFACE('',#49683,1.12127463204348);
#9062=CYLINDRICAL_SURFACE('',#49686,1.78199265440493);
#9063=CYLINDRICAL_SURFACE('',#49689,1.18199265440494);
#9064=CYLINDRICAL_SURFACE('',#49692,1.66088080992077);
#9065=CYLINDRICAL_SURFACE('',#49695,1.06088080992073);
#9066=CYLINDRICAL_SURFACE('',#49698,1.10035806567471);
#9067=CYLINDRICAL_SURFACE('',#49701,0.500358065674722);
#9068=CYLINDRICAL_SURFACE('',#49704,1.21403156673711);
#9069=CYLINDRICAL_SURFACE('',#49707,0.614031566737117);
#9070=CYLINDRICAL_SURFACE('',#49710,1.32880796357332);
#9071=CYLINDRICAL_SURFACE('',#49713,0.72880796357333);
#9072=CYLINDRICAL_SURFACE('',#49716,1.46111700181689);
#9073=CYLINDRICAL_SURFACE('',#49719,0.861117001816902);
#9074=CYLINDRICAL_SURFACE('',#49722,1.6204820426246);
#9075=CYLINDRICAL_SURFACE('',#49725,1.02048204262456);
#9076=CYLINDRICAL_SURFACE('',#49728,1.70100022308284);
#9077=CYLINDRICAL_SURFACE('',#49731,1.10100022308285);
#9078=CYLINDRICAL_SURFACE('',#49734,1.72127463204352);
#9079=CYLINDRICAL_SURFACE('',#49737,1.12127463204348);
#9080=CYLINDRICAL_SURFACE('',#49740,1.78199265440487);
#9081=CYLINDRICAL_SURFACE('',#49743,1.18199265440488);
#9082=CYLINDRICAL_SURFACE('',#49746,1.66088080992088);
#9083=CYLINDRICAL_SURFACE('',#49749,1.06088080992073);
#9084=CYLINDRICAL_SURFACE('',#49752,1.10035806567471);
#9085=CYLINDRICAL_SURFACE('',#49755,0.500358065674666);
#9086=CYLINDRICAL_SURFACE('',#49758,1.21403156673716);
#9087=CYLINDRICAL_SURFACE('',#49761,0.614031566737172);
#9088=CYLINDRICAL_SURFACE('',#49764,1.32880796357338);
#9089=CYLINDRICAL_SURFACE('',#49767,0.72880796357333);
#9090=CYLINDRICAL_SURFACE('',#49770,1.46111700181689);
#9091=CYLINDRICAL_SURFACE('',#49773,0.861117001816902);
#9092=CYLINDRICAL_SURFACE('',#49776,1.6204820426246);
#9093=CYLINDRICAL_SURFACE('',#49779,1.02048204262456);
#9094=CYLINDRICAL_SURFACE('',#49782,1.70100022308284);
#9095=CYLINDRICAL_SURFACE('',#49785,1.10100022308285);
#9096=CYLINDRICAL_SURFACE('',#49788,1.72127463204352);
#9097=CYLINDRICAL_SURFACE('',#49791,1.12127463204348);
#9098=CYLINDRICAL_SURFACE('',#49794,1.78199265440498);
#9099=CYLINDRICAL_SURFACE('',#49797,1.181992654405);
#9100=CYLINDRICAL_SURFACE('',#49800,1.66088080992077);
#9101=CYLINDRICAL_SURFACE('',#49803,1.06088080992073);
#9102=CYLINDRICAL_SURFACE('',#49806,1.10035806567471);
#9103=CYLINDRICAL_SURFACE('',#49809,0.500358065674722);
#9104=CYLINDRICAL_SURFACE('',#49812,1.21403156673705);
#9105=CYLINDRICAL_SURFACE('',#49815,0.614031566737117);
#9106=CYLINDRICAL_SURFACE('',#49818,1.32880796357338);
#9107=CYLINDRICAL_SURFACE('',#49821,0.72880796357333);
#9108=CYLINDRICAL_SURFACE('',#49824,1.46111700181689);
#9109=CYLINDRICAL_SURFACE('',#49827,0.861117001816902);
#9110=CYLINDRICAL_SURFACE('',#49830,1.6204820426246);
#9111=CYLINDRICAL_SURFACE('',#49833,1.02048204262462);
#9112=CYLINDRICAL_SURFACE('',#49836,1.70100022308278);
#9113=CYLINDRICAL_SURFACE('',#49839,1.10100022308279);
#9114=CYLINDRICAL_SURFACE('',#49842,1.72127463204352);
#9115=CYLINDRICAL_SURFACE('',#49845,1.12127463204348);
#9116=CYLINDRICAL_SURFACE('',#49848,1.78199265440493);
#9117=CYLINDRICAL_SURFACE('',#49851,1.18199265440494);
#9118=CYLINDRICAL_SURFACE('',#49854,1.66088080992077);
#9119=CYLINDRICAL_SURFACE('',#49857,1.06088080992078);
#9120=CYLINDRICAL_SURFACE('',#49860,1.10035806567471);
#9121=CYLINDRICAL_SURFACE('',#49863,0.500358065674722);
#9122=CYLINDRICAL_SURFACE('',#49866,1.21403156673711);
#9123=CYLINDRICAL_SURFACE('',#49869,0.614031566737117);
#9124=CYLINDRICAL_SURFACE('',#49872,1.32880796357332);
#9125=CYLINDRICAL_SURFACE('',#49875,0.72880796357333);
#9126=CYLINDRICAL_SURFACE('',#49878,1.46111700181689);
#9127=CYLINDRICAL_SURFACE('',#49881,0.861117001816902);
#9128=CYLINDRICAL_SURFACE('',#49884,1.62048204262455);
#9129=CYLINDRICAL_SURFACE('',#49887,1.02048204262462);
#9130=CYLINDRICAL_SURFACE('',#49890,1.70100022308278);
#9131=CYLINDRICAL_SURFACE('',#49893,1.10100022308279);
#9132=CYLINDRICAL_SURFACE('',#49896,1.72127463204347);
#9133=CYLINDRICAL_SURFACE('',#49899,1.12127463204353);
#9134=CYLINDRICAL_SURFACE('',#49902,1.78199265440487);
#9135=CYLINDRICAL_SURFACE('',#49905,1.18199265440494);
#9136=CYLINDRICAL_SURFACE('',#49908,1.66088080992077);
#9137=CYLINDRICAL_SURFACE('',#49911,1.06088080992078);
#9138=CYLINDRICAL_SURFACE('',#49914,1.10035806567471);
#9139=CYLINDRICAL_SURFACE('',#49917,0.500358065674777);
#9140=CYLINDRICAL_SURFACE('',#49920,1.21403156673711);
#9141=CYLINDRICAL_SURFACE('',#49923,0.614031566737117);
#9142=CYLINDRICAL_SURFACE('',#49926,1.32880796357332);
#9143=CYLINDRICAL_SURFACE('',#49929,0.728807963573275);
#9144=CYLINDRICAL_SURFACE('',#49932,1.46111700181695);
#9145=CYLINDRICAL_SURFACE('',#49935,0.861117001816902);
#9146=CYLINDRICAL_SURFACE('',#49938,1.6204820426246);
#9147=CYLINDRICAL_SURFACE('',#49941,1.02048204262462);
#9148=CYLINDRICAL_SURFACE('',#49944,1.70100022308284);
#9149=CYLINDRICAL_SURFACE('',#49947,1.10100022308285);
#9150=CYLINDRICAL_SURFACE('',#49950,1.72127463204347);
#9151=CYLINDRICAL_SURFACE('',#49953,1.12127463204348);
#9152=CYLINDRICAL_SURFACE('',#49956,1.78199265440493);
#9153=CYLINDRICAL_SURFACE('',#49959,1.18199265440488);
#9154=CYLINDRICAL_SURFACE('',#49962,1.66088080992077);
#9155=CYLINDRICAL_SURFACE('',#49965,1.06088080992078);
#9156=CYLINDRICAL_SURFACE('',#49968,1.10035806567471);
#9157=CYLINDRICAL_SURFACE('',#49971,0.500358065674722);
#9158=CYLINDRICAL_SURFACE('',#49974,1.21403156673711);
#9159=CYLINDRICAL_SURFACE('',#49977,0.614031566737117);
#9160=CYLINDRICAL_SURFACE('',#49980,1.32880796357332);
#9161=CYLINDRICAL_SURFACE('',#49983,0.72880796357333);
#9162=CYLINDRICAL_SURFACE('',#49986,1.46111700181689);
#9163=CYLINDRICAL_SURFACE('',#49989,0.861117001816902);
#9164=CYLINDRICAL_SURFACE('',#49992,1.62048204262455);
#9165=CYLINDRICAL_SURFACE('',#49995,1.02048204262456);
#9166=CYLINDRICAL_SURFACE('',#49998,1.70100022308284);
#9167=CYLINDRICAL_SURFACE('',#50001,1.10100022308285);
#9168=CYLINDRICAL_SURFACE('',#50004,1.72127463204347);
#9169=CYLINDRICAL_SURFACE('',#50007,1.12127463204348);
#9170=CYLINDRICAL_SURFACE('',#50010,1.78199265440493);
#9171=CYLINDRICAL_SURFACE('',#50013,1.18199265440494);
#9172=CYLINDRICAL_SURFACE('',#50016,1.66088080992077);
#9173=CYLINDRICAL_SURFACE('',#50019,1.06088080992078);
#9174=CYLINDRICAL_SURFACE('',#50022,1.10035806567471);
#9175=CYLINDRICAL_SURFACE('',#50025,0.500358065674722);
#9176=CYLINDRICAL_SURFACE('',#50028,1.21403156673711);
#9177=CYLINDRICAL_SURFACE('',#50031,0.614031566737117);
#9178=CYLINDRICAL_SURFACE('',#50034,1.32880796357326);
#9179=CYLINDRICAL_SURFACE('',#50037,0.728807963573275);
#9180=CYLINDRICAL_SURFACE('',#50040,1.46111700181689);
#9181=CYLINDRICAL_SURFACE('',#50043,0.861117001816902);
#9182=CYLINDRICAL_SURFACE('',#50046,1.6204820426246);
#9183=CYLINDRICAL_SURFACE('',#50049,1.02048204262456);
#9184=CYLINDRICAL_SURFACE('',#50052,1.70100022308284);
#9185=CYLINDRICAL_SURFACE('',#50055,1.10100022308285);
#9186=CYLINDRICAL_SURFACE('',#50058,1.72127463204352);
#9187=CYLINDRICAL_SURFACE('',#50061,1.12127463204348);
#9188=CYLINDRICAL_SURFACE('',#50064,1.78199265440498);
#9189=CYLINDRICAL_SURFACE('',#50067,1.18199265440494);
#9190=CYLINDRICAL_SURFACE('',#50070,1.66088080992083);
#9191=CYLINDRICAL_SURFACE('',#50073,1.06088080992078);
#9192=CYLINDRICAL_SURFACE('',#50076,1.10035806567471);
#9193=CYLINDRICAL_SURFACE('',#50079,0.500358065674722);
#9194=CYLINDRICAL_SURFACE('',#50082,1.21403156673711);
#9195=CYLINDRICAL_SURFACE('',#50085,0.614031566737117);
#9196=CYLINDRICAL_SURFACE('',#50088,1.32880796357332);
#9197=CYLINDRICAL_SURFACE('',#50091,0.72880796357333);
#9198=CYLINDRICAL_SURFACE('',#50094,1.46111700181689);
#9199=CYLINDRICAL_SURFACE('',#50097,0.861117001816847);
#9200=CYLINDRICAL_SURFACE('',#50100,1.6204820426246);
#9201=CYLINDRICAL_SURFACE('',#50103,1.02048204262462);
#9202=CYLINDRICAL_SURFACE('',#50106,1.70100022308284);
#9203=CYLINDRICAL_SURFACE('',#50109,1.10100022308279);
#9204=CYLINDRICAL_SURFACE('',#50112,1.72127463204347);
#9205=CYLINDRICAL_SURFACE('',#50115,1.12127463204353);
#9206=CYLINDRICAL_SURFACE('',#50118,1.78199265440493);
#9207=CYLINDRICAL_SURFACE('',#50121,1.18199265440494);
#9208=CYLINDRICAL_SURFACE('',#50124,1.66088080992077);
#9209=CYLINDRICAL_SURFACE('',#50127,1.06088080992078);
#9210=CYLINDRICAL_SURFACE('',#50130,1.10035806567471);
#9211=CYLINDRICAL_SURFACE('',#50133,0.500358065674722);
#9212=CYLINDRICAL_SURFACE('',#50136,1.21403156673711);
#9213=CYLINDRICAL_SURFACE('',#50139,0.614031566737117);
#9214=CYLINDRICAL_SURFACE('',#50142,1.32880796357332);
#9215=CYLINDRICAL_SURFACE('',#50145,0.72880796357333);
#9216=CYLINDRICAL_SURFACE('',#50148,1.46111700181689);
#9217=CYLINDRICAL_SURFACE('',#50151,0.861117001816902);
#9218=CYLINDRICAL_SURFACE('',#50154,1.6204820426246);
#9219=CYLINDRICAL_SURFACE('',#50157,1.02048204262462);
#9220=CYLINDRICAL_SURFACE('',#50160,1.70100022308284);
#9221=CYLINDRICAL_SURFACE('',#50163,1.10100022308285);
#9222=CYLINDRICAL_SURFACE('',#50166,1.72127463204347);
#9223=CYLINDRICAL_SURFACE('',#50169,1.12127463204348);
#9224=CYLINDRICAL_SURFACE('',#50172,1.78199265440493);
#9225=CYLINDRICAL_SURFACE('',#50175,1.18199265440494);
#9226=CYLINDRICAL_SURFACE('',#50178,1.66088080992077);
#9227=CYLINDRICAL_SURFACE('',#50181,1.06088080992078);
#9228=CYLINDRICAL_SURFACE('',#50184,1.10035806567471);
#9229=CYLINDRICAL_SURFACE('',#50187,0.500358065674666);
#9230=CYLINDRICAL_SURFACE('',#50190,1.21403156673716);
#9231=CYLINDRICAL_SURFACE('',#50193,0.614031566737117);
#9232=CYLINDRICAL_SURFACE('',#50196,1.32880796357332);
#9233=CYLINDRICAL_SURFACE('',#50199,0.72880796357333);
#9234=CYLINDRICAL_SURFACE('',#50202,1.46111700181689);
#9235=CYLINDRICAL_SURFACE('',#50205,0.861117001816902);
#9236=CYLINDRICAL_SURFACE('',#50208,1.6204820426246);
#9237=CYLINDRICAL_SURFACE('',#50211,1.02048204262462);
#9238=CYLINDRICAL_SURFACE('',#50214,1.70100022308284);
#9239=CYLINDRICAL_SURFACE('',#50217,1.10100022308285);
#9240=CYLINDRICAL_SURFACE('',#50220,1.72127463204352);
#9241=CYLINDRICAL_SURFACE('',#50223,1.12127463204353);
#9242=CYLINDRICAL_SURFACE('',#50226,1.78199265440493);
#9243=CYLINDRICAL_SURFACE('',#50229,1.18199265440494);
#9244=CYLINDRICAL_SURFACE('',#50232,1.66088080992077);
#9245=CYLINDRICAL_SURFACE('',#50235,1.06088080992078);
#9246=CYLINDRICAL_SURFACE('',#50238,1.10035806567471);
#9247=CYLINDRICAL_SURFACE('',#50241,0.500358065674666);
#9248=CYLINDRICAL_SURFACE('',#50244,1.21403156673716);
#9249=CYLINDRICAL_SURFACE('',#50247,0.614031566737172);
#9250=CYLINDRICAL_SURFACE('',#50250,1.32880796357326);
#9251=CYLINDRICAL_SURFACE('',#50253,0.728807963573275);
#9252=CYLINDRICAL_SURFACE('',#50256,1.46111700181689);
#9253=CYLINDRICAL_SURFACE('',#50259,0.861117001816847);
#9254=CYLINDRICAL_SURFACE('',#50262,1.62048204262455);
#9255=CYLINDRICAL_SURFACE('',#50265,1.02048204262462);
#9256=CYLINDRICAL_SURFACE('',#50268,1.70100022308284);
#9257=CYLINDRICAL_SURFACE('',#50271,1.10100022308279);
#9258=CYLINDRICAL_SURFACE('',#50274,1.72127463204352);
#9259=CYLINDRICAL_SURFACE('',#50277,1.12127463204348);
#9260=CYLINDRICAL_SURFACE('',#50280,1.78199265440493);
#9261=CYLINDRICAL_SURFACE('',#50283,1.18199265440494);
#9262=CYLINDRICAL_SURFACE('',#50286,1.66088080992083);
#9263=CYLINDRICAL_SURFACE('',#50289,1.06088080992078);
#9264=CYLINDRICAL_SURFACE('',#50292,1.10035806567471);
#9265=CYLINDRICAL_SURFACE('',#50295,0.500358065674722);
#9266=CYLINDRICAL_SURFACE('',#50298,1.21403156673716);
#9267=CYLINDRICAL_SURFACE('',#50301,0.614031566737172);
#9268=CYLINDRICAL_SURFACE('',#50304,1.32880796357326);
#9269=CYLINDRICAL_SURFACE('',#50307,0.72880796357333);
#9270=CYLINDRICAL_SURFACE('',#50310,1.46111700181689);
#9271=CYLINDRICAL_SURFACE('',#50313,0.861117001816902);
#9272=CYLINDRICAL_SURFACE('',#50316,1.6204820426246);
#9273=CYLINDRICAL_SURFACE('',#50319,1.02048204262456);
#9274=CYLINDRICAL_SURFACE('',#50322,1.70100022308278);
#9275=CYLINDRICAL_SURFACE('',#50325,1.10100022308279);
#9276=CYLINDRICAL_SURFACE('',#50328,1.72127463204347);
#9277=CYLINDRICAL_SURFACE('',#50331,1.12127463204348);
#9278=CYLINDRICAL_SURFACE('',#50334,1.78199265440493);
#9279=CYLINDRICAL_SURFACE('',#50337,1.18199265440494);
#9280=CYLINDRICAL_SURFACE('',#50340,1.66088080992077);
#9281=CYLINDRICAL_SURFACE('',#50343,1.06088080992084);
#9282=CYLINDRICAL_SURFACE('',#50346,1.10035806567471);
#9283=CYLINDRICAL_SURFACE('',#50349,0.500358065674722);
#9284=CYLINDRICAL_SURFACE('',#50352,1.21403156673716);
#9285=CYLINDRICAL_SURFACE('',#50355,0.614031566737117);
#9286=CYLINDRICAL_SURFACE('',#50358,1.32880796357338);
#9287=CYLINDRICAL_SURFACE('',#50361,0.728807963573386);
#9288=CYLINDRICAL_SURFACE('',#50364,1.46111700181695);
#9289=CYLINDRICAL_SURFACE('',#50367,0.861117001816902);
#9290=CYLINDRICAL_SURFACE('',#50370,1.6204820426246);
#9291=CYLINDRICAL_SURFACE('',#50373,1.02048204262456);
#9292=CYLINDRICAL_SURFACE('',#50376,1.70100022308284);
#9293=CYLINDRICAL_SURFACE('',#50379,1.10100022308279);
#9294=CYLINDRICAL_SURFACE('',#50382,1.72127463204352);
#9295=CYLINDRICAL_SURFACE('',#50385,1.12127463204348);
#9296=CYLINDRICAL_SURFACE('',#50388,1.78199265440493);
#9297=CYLINDRICAL_SURFACE('',#50391,1.18199265440494);
#9298=CYLINDRICAL_SURFACE('',#50394,1.66088080992083);
#9299=CYLINDRICAL_SURFACE('',#50397,1.06088080992078);
#9300=CYLINDRICAL_SURFACE('',#50400,1.10035806567466);
#9301=CYLINDRICAL_SURFACE('',#50403,0.500358065674666);
#9302=CYLINDRICAL_SURFACE('',#50406,1.21403156673716);
#9303=CYLINDRICAL_SURFACE('',#50409,0.614031566737172);
#9304=CYLINDRICAL_SURFACE('',#50412,1.32880796357326);
#9305=CYLINDRICAL_SURFACE('',#50415,0.728807963573275);
#9306=CYLINDRICAL_SURFACE('',#50418,1.46111700181689);
#9307=CYLINDRICAL_SURFACE('',#50421,0.861117001816847);
#9308=CYLINDRICAL_SURFACE('',#50424,1.6204820426246);
#9309=CYLINDRICAL_SURFACE('',#50427,1.02048204262456);
#9310=CYLINDRICAL_SURFACE('',#50430,1.70100022308284);
#9311=CYLINDRICAL_SURFACE('',#50433,1.10100022308285);
#9312=CYLINDRICAL_SURFACE('',#50436,1.72127463204352);
#9313=CYLINDRICAL_SURFACE('',#50439,1.12127463204348);
#9314=CYLINDRICAL_SURFACE('',#50442,1.78199265440498);
#9315=CYLINDRICAL_SURFACE('',#50445,1.18199265440494);
#9316=CYLINDRICAL_SURFACE('',#50448,1.66088080992077);
#9317=CYLINDRICAL_SURFACE('',#50451,1.06088080992078);
#9318=CYLINDRICAL_SURFACE('',#50454,1.10035806567471);
#9319=CYLINDRICAL_SURFACE('',#50457,0.500358065674666);
#9320=CYLINDRICAL_SURFACE('',#50460,1.21403156673716);
#9321=CYLINDRICAL_SURFACE('',#50463,0.614031566737117);
#9322=CYLINDRICAL_SURFACE('',#50466,1.32880796357332);
#9323=CYLINDRICAL_SURFACE('',#50469,0.72880796357333);
#9324=CYLINDRICAL_SURFACE('',#50472,1.46111700181689);
#9325=CYLINDRICAL_SURFACE('',#50475,0.861117001816902);
#9326=CYLINDRICAL_SURFACE('',#50478,1.62048204262455);
#9327=CYLINDRICAL_SURFACE('',#50481,1.02048204262456);
#9328=CYLINDRICAL_SURFACE('',#50484,1.70100022308278);
#9329=CYLINDRICAL_SURFACE('',#50487,1.10100022308285);
#9330=CYLINDRICAL_SURFACE('',#50490,1.72127463204347);
#9331=CYLINDRICAL_SURFACE('',#50493,1.12127463204348);
#9332=CYLINDRICAL_SURFACE('',#50496,1.78199265440493);
#9333=CYLINDRICAL_SURFACE('',#50499,1.18199265440488);
#9334=CYLINDRICAL_SURFACE('',#50502,1.66088080992083);
#9335=CYLINDRICAL_SURFACE('',#50505,1.06088080992078);
#9336=CYLINDRICAL_SURFACE('',#50508,1.10035806567471);
#9337=CYLINDRICAL_SURFACE('',#50511,0.500358065674666);
#9338=CYLINDRICAL_SURFACE('',#50514,1.21403156673716);
#9339=CYLINDRICAL_SURFACE('',#50517,0.614031566737117);
#9340=CYLINDRICAL_SURFACE('',#50520,1.32880796357332);
#9341=CYLINDRICAL_SURFACE('',#50523,0.72880796357333);
#9342=CYLINDRICAL_SURFACE('',#50526,1.46111700181689);
#9343=CYLINDRICAL_SURFACE('',#50529,0.861117001816902);
#9344=CYLINDRICAL_SURFACE('',#50532,1.6204820426246);
#9345=CYLINDRICAL_SURFACE('',#50535,1.02048204262462);
#9346=CYLINDRICAL_SURFACE('',#50538,1.70100022308284);
#9347=CYLINDRICAL_SURFACE('',#50541,1.10100022308285);
#9348=CYLINDRICAL_SURFACE('',#50544,1.72127463204352);
#9349=CYLINDRICAL_SURFACE('',#50547,1.12127463204353);
#9350=CYLINDRICAL_SURFACE('',#50550,1.78199265440493);
#9351=CYLINDRICAL_SURFACE('',#50553,1.18199265440488);
#9352=CYLINDRICAL_SURFACE('',#50556,1.66088080992077);
#9353=CYLINDRICAL_SURFACE('',#50559,1.06088080992078);
#9354=CYLINDRICAL_SURFACE('',#50562,1.10035806567477);
#9355=CYLINDRICAL_SURFACE('',#50565,0.500358065674722);
#9356=CYLINDRICAL_SURFACE('',#50568,1.21403156673711);
#9357=CYLINDRICAL_SURFACE('',#50571,0.614031566737061);
#9358=CYLINDRICAL_SURFACE('',#50574,1.32880796357332);
#9359=CYLINDRICAL_SURFACE('',#50577,0.728807963573275);
#9360=CYLINDRICAL_SURFACE('',#50580,1.46111700181684);
#9361=CYLINDRICAL_SURFACE('',#50583,0.861117001816847);
#9362=CYLINDRICAL_SURFACE('',#50586,1.6204820426246);
#9363=CYLINDRICAL_SURFACE('',#50589,1.02048204262456);
#9364=CYLINDRICAL_SURFACE('',#50592,1.70100022308278);
#9365=CYLINDRICAL_SURFACE('',#50595,1.10100022308279);
#9366=CYLINDRICAL_SURFACE('',#50598,1.72127463204352);
#9367=CYLINDRICAL_SURFACE('',#50601,1.12127463204353);
#9368=CYLINDRICAL_SURFACE('',#50604,1.78199265440493);
#9369=CYLINDRICAL_SURFACE('',#50607,1.18199265440494);
#9370=CYLINDRICAL_SURFACE('',#50610,1.66088080992077);
#9371=CYLINDRICAL_SURFACE('',#50613,1.06088080992073);
#9372=CYLINDRICAL_SURFACE('',#50616,1.10035806567471);
#9373=CYLINDRICAL_SURFACE('',#50619,0.500358065674722);
#9374=CYLINDRICAL_SURFACE('',#50622,1.21403156673711);
#9375=CYLINDRICAL_SURFACE('',#50625,0.614031566737117);
#9376=CYLINDRICAL_SURFACE('',#50628,1.32880796357332);
#9377=CYLINDRICAL_SURFACE('',#50631,0.728807963573275);
#9378=CYLINDRICAL_SURFACE('',#50634,1.46111700181684);
#9379=CYLINDRICAL_SURFACE('',#50637,0.861117001816902);
#9380=CYLINDRICAL_SURFACE('',#50640,1.6204820426246);
#9381=CYLINDRICAL_SURFACE('',#50643,1.02048204262462);
#9382=CYLINDRICAL_SURFACE('',#50646,1.70100022308289);
#9383=CYLINDRICAL_SURFACE('',#50649,1.10100022308285);
#9384=CYLINDRICAL_SURFACE('',#50652,1.72127463204347);
#9385=CYLINDRICAL_SURFACE('',#50655,1.12127463204342);
#9386=CYLINDRICAL_SURFACE('',#50658,1.78199265440498);
#9387=CYLINDRICAL_SURFACE('',#50661,1.18199265440494);
#9388=CYLINDRICAL_SURFACE('',#50664,1.66088080992077);
#9389=CYLINDRICAL_SURFACE('',#50667,1.06088080992078);
#9390=CYLINDRICAL_SURFACE('',#50670,1.10035806567471);
#9391=CYLINDRICAL_SURFACE('',#50673,0.500358065674666);
#9392=CYLINDRICAL_SURFACE('',#50676,1.21403156673711);
#9393=CYLINDRICAL_SURFACE('',#50679,0.614031566737117);
#9394=CYLINDRICAL_SURFACE('',#50682,1.32880796357332);
#9395=CYLINDRICAL_SURFACE('',#50685,0.72880796357333);
#9396=CYLINDRICAL_SURFACE('',#50688,1.46111700181684);
#9397=CYLINDRICAL_SURFACE('',#50691,0.861117001816847);
#9398=CYLINDRICAL_SURFACE('',#50694,1.6204820426246);
#9399=CYLINDRICAL_SURFACE('',#50697,1.02048204262456);
#9400=CYLINDRICAL_SURFACE('',#50700,1.70100022308284);
#9401=CYLINDRICAL_SURFACE('',#50703,1.10100022308285);
#9402=CYLINDRICAL_SURFACE('',#50706,1.72127463204347);
#9403=CYLINDRICAL_SURFACE('',#50709,1.12127463204353);
#9404=CYLINDRICAL_SURFACE('',#50712,1.78199265440498);
#9405=CYLINDRICAL_SURFACE('',#50715,1.18199265440494);
#9406=CYLINDRICAL_SURFACE('',#50718,1.66088080992083);
#9407=CYLINDRICAL_SURFACE('',#50721,1.06088080992078);
#9408=CYLINDRICAL_SURFACE('',#50724,1.10035806567477);
#9409=CYLINDRICAL_SURFACE('',#50727,0.500358065674777);
#9410=CYLINDRICAL_SURFACE('',#50730,1.21403156673705);
#9411=CYLINDRICAL_SURFACE('',#50733,0.614031566737117);
#9412=CYLINDRICAL_SURFACE('',#50736,1.32880796357326);
#9413=CYLINDRICAL_SURFACE('',#50739,0.728807963573275);
#9414=CYLINDRICAL_SURFACE('',#50742,1.46111700181684);
#9415=CYLINDRICAL_SURFACE('',#50745,0.861117001816847);
#9416=CYLINDRICAL_SURFACE('',#50748,1.6204820426246);
#9417=CYLINDRICAL_SURFACE('',#50751,1.02048204262462);
#9418=CYLINDRICAL_SURFACE('',#50754,1.70100022308278);
#9419=CYLINDRICAL_SURFACE('',#50757,1.10100022308285);
#9420=CYLINDRICAL_SURFACE('',#50760,1.72127463204347);
#9421=CYLINDRICAL_SURFACE('',#50763,1.12127463204353);
#9422=CYLINDRICAL_SURFACE('',#50766,1.78199265440493);
#9423=CYLINDRICAL_SURFACE('',#50769,1.18199265440494);
#9424=CYLINDRICAL_SURFACE('',#50772,1.66088080992077);
#9425=CYLINDRICAL_SURFACE('',#50775,1.06088080992078);
#9426=CYLINDRICAL_SURFACE('',#50778,1.10035806567471);
#9427=CYLINDRICAL_SURFACE('',#50781,0.500358065674722);
#9428=CYLINDRICAL_SURFACE('',#50784,1.21403156673716);
#9429=CYLINDRICAL_SURFACE('',#50787,0.614031566737117);
#9430=CYLINDRICAL_SURFACE('',#50790,1.32880796357332);
#9431=CYLINDRICAL_SURFACE('',#50793,0.72880796357333);
#9432=CYLINDRICAL_SURFACE('',#50796,1.46111700181689);
#9433=CYLINDRICAL_SURFACE('',#50799,0.861117001816902);
#9434=CYLINDRICAL_SURFACE('',#50802,1.6204820426246);
#9435=CYLINDRICAL_SURFACE('',#50805,1.02048204262462);
#9436=CYLINDRICAL_SURFACE('',#50808,1.70100022308284);
#9437=CYLINDRICAL_SURFACE('',#50811,1.10100022308285);
#9438=CYLINDRICAL_SURFACE('',#50814,1.72127463204352);
#9439=CYLINDRICAL_SURFACE('',#50817,1.12127463204348);
#9440=CYLINDRICAL_SURFACE('',#50820,1.78199265440493);
#9441=CYLINDRICAL_SURFACE('',#50823,1.18199265440488);
#9442=CYLINDRICAL_SURFACE('',#50826,1.66088080992088);
#9443=CYLINDRICAL_SURFACE('',#50829,1.06088080992084);
#9444=CYLINDRICAL_SURFACE('',#50832,1.10035806567471);
#9445=CYLINDRICAL_SURFACE('',#50835,0.500358065674722);
#9446=CYLINDRICAL_SURFACE('',#50838,1.21403156673716);
#9447=CYLINDRICAL_SURFACE('',#50841,0.614031566737117);
#9448=CYLINDRICAL_SURFACE('',#50844,1.32880796357332);
#9449=CYLINDRICAL_SURFACE('',#50847,0.72880796357333);
#9450=CYLINDRICAL_SURFACE('',#50850,1.46111700181689);
#9451=CYLINDRICAL_SURFACE('',#50853,0.861117001816902);
#9452=CYLINDRICAL_SURFACE('',#50856,1.6204820426246);
#9453=CYLINDRICAL_SURFACE('',#50859,1.02048204262462);
#9454=CYLINDRICAL_SURFACE('',#50862,1.70100022308284);
#9455=CYLINDRICAL_SURFACE('',#50865,1.10100022308285);
#9456=CYLINDRICAL_SURFACE('',#50868,1.72127463204352);
#9457=CYLINDRICAL_SURFACE('',#50871,1.12127463204348);
#9458=CYLINDRICAL_SURFACE('',#50874,1.78199265440493);
#9459=CYLINDRICAL_SURFACE('',#50877,1.18199265440494);
#9460=CYLINDRICAL_SURFACE('',#50880,1.66088080992077);
#9461=CYLINDRICAL_SURFACE('',#50883,1.06088080992078);
#9462=CYLINDRICAL_SURFACE('',#50890,127.41606204049);
#9463=CYLINDRICAL_SURFACE('',#50901,12.3670707361132);
#9464=CYLINDRICAL_SURFACE('',#50922,130.);
#9465=CYLINDRICAL_SURFACE('',#50923,0.878303132193281);
#9466=CYLINDRICAL_SURFACE('',#50925,1.47830313219333);
#11287=FACE_OUTER_BOUND('',#15337,.T.);
#11288=FACE_OUTER_BOUND('',#15398,.T.);
#11289=FACE_OUTER_BOUND('',#15399,.T.);
#11290=FACE_OUTER_BOUND('',#15400,.T.);
#11291=FACE_OUTER_BOUND('',#15401,.T.);
#11292=FACE_OUTER_BOUND('',#15402,.T.);
#11293=FACE_OUTER_BOUND('',#15403,.T.);
#11294=FACE_OUTER_BOUND('',#15404,.T.);
#11295=FACE_OUTER_BOUND('',#15405,.T.);
#11296=FACE_OUTER_BOUND('',#15406,.T.);
#11297=FACE_OUTER_BOUND('',#15407,.T.);
#11298=FACE_OUTER_BOUND('',#15408,.T.);
#11299=FACE_OUTER_BOUND('',#15409,.T.);
#11300=FACE_OUTER_BOUND('',#15410,.T.);
#11301=FACE_OUTER_BOUND('',#15411,.T.);
#11302=FACE_OUTER_BOUND('',#15412,.T.);
#11303=FACE_OUTER_BOUND('',#15413,.T.);
#11304=FACE_OUTER_BOUND('',#15414,.T.);
#11305=FACE_OUTER_BOUND('',#15415,.T.);
#11306=FACE_OUTER_BOUND('',#15416,.T.);
#11307=FACE_OUTER_BOUND('',#15417,.T.);
#11308=FACE_OUTER_BOUND('',#15418,.T.);
#11309=FACE_OUTER_BOUND('',#15419,.T.);
#11310=FACE_OUTER_BOUND('',#15420,.T.);
#11311=FACE_OUTER_BOUND('',#15421,.T.);
#11312=FACE_OUTER_BOUND('',#15422,.T.);
#11313=FACE_OUTER_BOUND('',#15423,.T.);
#11314=FACE_OUTER_BOUND('',#15424,.T.);
#11315=FACE_OUTER_BOUND('',#15425,.T.);
#11316=FACE_OUTER_BOUND('',#15426,.T.);
#11317=FACE_OUTER_BOUND('',#15427,.T.);
#11318=FACE_OUTER_BOUND('',#15428,.T.);
#11319=FACE_OUTER_BOUND('',#15429,.T.);
#11320=FACE_OUTER_BOUND('',#15430,.T.);
#11321=FACE_OUTER_BOUND('',#15431,.T.);
#11322=FACE_OUTER_BOUND('',#15432,.T.);
#11323=FACE_OUTER_BOUND('',#15433,.T.);
#11324=FACE_OUTER_BOUND('',#15434,.T.);
#11325=FACE_OUTER_BOUND('',#15435,.T.);
#11326=FACE_OUTER_BOUND('',#15436,.T.);
#11327=FACE_OUTER_BOUND('',#15437,.T.);
#11328=FACE_OUTER_BOUND('',#15438,.T.);
#11329=FACE_OUTER_BOUND('',#15439,.T.);
#11330=FACE_OUTER_BOUND('',#15440,.T.);
#11331=FACE_OUTER_BOUND('',#15441,.T.);
#11332=FACE_OUTER_BOUND('',#15442,.T.);
#11333=FACE_OUTER_BOUND('',#15443,.T.);
#11334=FACE_OUTER_BOUND('',#15444,.T.);
#11335=FACE_OUTER_BOUND('',#15445,.T.);
#11336=FACE_OUTER_BOUND('',#15446,.T.);
#11337=FACE_OUTER_BOUND('',#15447,.T.);
#11338=FACE_OUTER_BOUND('',#15448,.T.);
#11339=FACE_OUTER_BOUND('',#15449,.T.);
#11340=FACE_OUTER_BOUND('',#15450,.T.);
#11341=FACE_OUTER_BOUND('',#15451,.T.);
#11342=FACE_OUTER_BOUND('',#15452,.T.);
#11343=FACE_OUTER_BOUND('',#15453,.T.);
#11344=FACE_OUTER_BOUND('',#15454,.T.);
#11345=FACE_OUTER_BOUND('',#15455,.T.);
#11346=FACE_OUTER_BOUND('',#15456,.T.);
#11347=FACE_OUTER_BOUND('',#15457,.T.);
#11348=FACE_OUTER_BOUND('',#15458,.T.);
#11349=FACE_OUTER_BOUND('',#15459,.T.);
#11350=FACE_OUTER_BOUND('',#15460,.T.);
#11351=FACE_OUTER_BOUND('',#15461,.T.);
#11352=FACE_OUTER_BOUND('',#15462,.T.);
#11353=FACE_OUTER_BOUND('',#15463,.T.);
#11354=FACE_OUTER_BOUND('',#15464,.T.);
#11355=FACE_OUTER_BOUND('',#15465,.T.);
#11356=FACE_OUTER_BOUND('',#15466,.T.);
#11357=FACE_OUTER_BOUND('',#15467,.T.);
#11358=FACE_OUTER_BOUND('',#15468,.T.);
#11359=FACE_OUTER_BOUND('',#15469,.T.);
#11360=FACE_OUTER_BOUND('',#15470,.T.);
#11361=FACE_OUTER_BOUND('',#15471,.T.);
#11362=FACE_OUTER_BOUND('',#15472,.T.);
#11363=FACE_OUTER_BOUND('',#15473,.T.);
#11364=FACE_OUTER_BOUND('',#15474,.T.);
#11365=FACE_OUTER_BOUND('',#15475,.T.);
#11366=FACE_OUTER_BOUND('',#15476,.T.);
#11367=FACE_OUTER_BOUND('',#15477,.T.);
#11368=FACE_OUTER_BOUND('',#15478,.T.);
#11369=FACE_OUTER_BOUND('',#15479,.T.);
#11370=FACE_OUTER_BOUND('',#15480,.T.);
#11371=FACE_OUTER_BOUND('',#15481,.T.);
#11372=FACE_OUTER_BOUND('',#15482,.T.);
#11373=FACE_OUTER_BOUND('',#15483,.T.);
#11374=FACE_OUTER_BOUND('',#15484,.T.);
#11375=FACE_OUTER_BOUND('',#15485,.T.);
#11376=FACE_OUTER_BOUND('',#15486,.T.);
#11377=FACE_OUTER_BOUND('',#15487,.T.);
#11378=FACE_OUTER_BOUND('',#15488,.T.);
#11379=FACE_OUTER_BOUND('',#15489,.T.);
#11380=FACE_OUTER_BOUND('',#15490,.T.);
#11381=FACE_OUTER_BOUND('',#15491,.T.);
#11382=FACE_OUTER_BOUND('',#15492,.T.);
#11383=FACE_OUTER_BOUND('',#15493,.T.);
#11384=FACE_OUTER_BOUND('',#15494,.T.);
#11385=FACE_OUTER_BOUND('',#15495,.T.);
#11386=FACE_OUTER_BOUND('',#15496,.T.);
#11387=FACE_OUTER_BOUND('',#15497,.T.);
#11388=FACE_OUTER_BOUND('',#15498,.T.);
#11389=FACE_OUTER_BOUND('',#15499,.T.);
#11390=FACE_OUTER_BOUND('',#15500,.T.);
#11391=FACE_OUTER_BOUND('',#15501,.T.);
#11392=FACE_OUTER_BOUND('',#15502,.T.);
#11393=FACE_OUTER_BOUND('',#15503,.T.);
#11394=FACE_OUTER_BOUND('',#15504,.T.);
#11395=FACE_OUTER_BOUND('',#15505,.T.);
#11396=FACE_OUTER_BOUND('',#15506,.T.);
#11397=FACE_OUTER_BOUND('',#15507,.T.);
#11398=FACE_OUTER_BOUND('',#15508,.T.);
#11399=FACE_OUTER_BOUND('',#15509,.T.);
#11400=FACE_OUTER_BOUND('',#15510,.T.);
#11401=FACE_OUTER_BOUND('',#15511,.T.);
#11402=FACE_OUTER_BOUND('',#15512,.T.);
#11403=FACE_OUTER_BOUND('',#15513,.T.);
#11404=FACE_OUTER_BOUND('',#15514,.T.);
#11405=FACE_OUTER_BOUND('',#15515,.T.);
#11406=FACE_OUTER_BOUND('',#15516,.T.);
#11407=FACE_OUTER_BOUND('',#15517,.T.);
#11408=FACE_OUTER_BOUND('',#15518,.T.);
#11409=FACE_OUTER_BOUND('',#15519,.T.);
#11410=FACE_OUTER_BOUND('',#15520,.T.);
#11411=FACE_OUTER_BOUND('',#15521,.T.);
#11412=FACE_OUTER_BOUND('',#15522,.T.);
#11413=FACE_OUTER_BOUND('',#15523,.T.);
#11414=FACE_OUTER_BOUND('',#15524,.T.);
#11415=FACE_OUTER_BOUND('',#15525,.T.);
#11416=FACE_OUTER_BOUND('',#15526,.T.);
#11417=FACE_OUTER_BOUND('',#15527,.T.);
#11418=FACE_OUTER_BOUND('',#15528,.T.);
#11419=FACE_OUTER_BOUND('',#15529,.T.);
#11420=FACE_OUTER_BOUND('',#15530,.T.);
#11421=FACE_OUTER_BOUND('',#15531,.T.);
#11422=FACE_OUTER_BOUND('',#15532,.T.);
#11423=FACE_OUTER_BOUND('',#15533,.T.);
#11424=FACE_OUTER_BOUND('',#15534,.T.);
#11425=FACE_OUTER_BOUND('',#15535,.T.);
#11426=FACE_OUTER_BOUND('',#15536,.T.);
#11427=FACE_OUTER_BOUND('',#15537,.T.);
#11428=FACE_OUTER_BOUND('',#15538,.T.);
#11429=FACE_OUTER_BOUND('',#15539,.T.);
#11430=FACE_OUTER_BOUND('',#15540,.T.);
#11431=FACE_OUTER_BOUND('',#15541,.T.);
#11432=FACE_OUTER_BOUND('',#15542,.T.);
#11433=FACE_OUTER_BOUND('',#15543,.T.);
#11434=FACE_OUTER_BOUND('',#15544,.T.);
#11435=FACE_OUTER_BOUND('',#15545,.T.);
#11436=FACE_OUTER_BOUND('',#15546,.T.);
#11437=FACE_OUTER_BOUND('',#15547,.T.);
#11438=FACE_OUTER_BOUND('',#15548,.T.);
#11439=FACE_OUTER_BOUND('',#15549,.T.);
#11440=FACE_OUTER_BOUND('',#15550,.T.);
#11441=FACE_OUTER_BOUND('',#15551,.T.);
#11442=FACE_OUTER_BOUND('',#15552,.T.);
#11443=FACE_OUTER_BOUND('',#15553,.T.);
#11444=FACE_OUTER_BOUND('',#15554,.T.);
#11445=FACE_OUTER_BOUND('',#15555,.T.);
#11446=FACE_OUTER_BOUND('',#15556,.T.);
#11447=FACE_OUTER_BOUND('',#15557,.T.);
#11448=FACE_OUTER_BOUND('',#15558,.T.);
#11449=FACE_OUTER_BOUND('',#15559,.T.);
#11450=FACE_OUTER_BOUND('',#15560,.T.);
#11451=FACE_OUTER_BOUND('',#15561,.T.);
#11452=FACE_OUTER_BOUND('',#15562,.T.);
#11453=FACE_OUTER_BOUND('',#15563,.T.);
#11454=FACE_OUTER_BOUND('',#15564,.T.);
#11455=FACE_OUTER_BOUND('',#15565,.T.);
#11456=FACE_OUTER_BOUND('',#15566,.T.);
#11457=FACE_OUTER_BOUND('',#15567,.T.);
#11458=FACE_OUTER_BOUND('',#15568,.T.);
#11459=FACE_OUTER_BOUND('',#15569,.T.);
#11460=FACE_OUTER_BOUND('',#15570,.T.);
#11461=FACE_OUTER_BOUND('',#15571,.T.);
#11462=FACE_OUTER_BOUND('',#15572,.T.);
#11463=FACE_OUTER_BOUND('',#15573,.T.);
#11464=FACE_OUTER_BOUND('',#15574,.T.);
#11465=FACE_OUTER_BOUND('',#15575,.T.);
#11466=FACE_OUTER_BOUND('',#15576,.T.);
#11467=FACE_OUTER_BOUND('',#15577,.T.);
#11468=FACE_OUTER_BOUND('',#15578,.T.);
#11469=FACE_OUTER_BOUND('',#15579,.T.);
#11470=FACE_OUTER_BOUND('',#15580,.T.);
#11471=FACE_OUTER_BOUND('',#15581,.T.);
#11472=FACE_OUTER_BOUND('',#15582,.T.);
#11473=FACE_OUTER_BOUND('',#15583,.T.);
#11474=FACE_OUTER_BOUND('',#15584,.T.);
#11475=FACE_OUTER_BOUND('',#15585,.T.);
#11476=FACE_OUTER_BOUND('',#15586,.T.);
#11477=FACE_OUTER_BOUND('',#15587,.T.);
#11478=FACE_OUTER_BOUND('',#15588,.T.);
#11479=FACE_OUTER_BOUND('',#15589,.T.);
#11480=FACE_OUTER_BOUND('',#15590,.T.);
#11481=FACE_OUTER_BOUND('',#15591,.T.);
#11482=FACE_OUTER_BOUND('',#15592,.T.);
#11483=FACE_OUTER_BOUND('',#15593,.T.);
#11484=FACE_OUTER_BOUND('',#15594,.T.);
#11485=FACE_OUTER_BOUND('',#15595,.T.);
#11486=FACE_OUTER_BOUND('',#15596,.T.);
#11487=FACE_OUTER_BOUND('',#15597,.T.);
#11488=FACE_OUTER_BOUND('',#15598,.T.);
#11489=FACE_OUTER_BOUND('',#15599,.T.);
#11490=FACE_OUTER_BOUND('',#15600,.T.);
#11491=FACE_OUTER_BOUND('',#15601,.T.);
#11492=FACE_OUTER_BOUND('',#15602,.T.);
#11493=FACE_OUTER_BOUND('',#15603,.T.);
#11494=FACE_OUTER_BOUND('',#15604,.T.);
#11495=FACE_OUTER_BOUND('',#15605,.T.);
#11496=FACE_OUTER_BOUND('',#15606,.T.);
#11497=FACE_OUTER_BOUND('',#15607,.T.);
#11498=FACE_OUTER_BOUND('',#15608,.T.);
#11499=FACE_OUTER_BOUND('',#15609,.T.);
#11500=FACE_OUTER_BOUND('',#15610,.T.);
#11501=FACE_OUTER_BOUND('',#15611,.T.);
#11502=FACE_OUTER_BOUND('',#15612,.T.);
#11503=FACE_OUTER_BOUND('',#15613,.T.);
#11504=FACE_OUTER_BOUND('',#15614,.T.);
#11505=FACE_OUTER_BOUND('',#15615,.T.);
#11506=FACE_OUTER_BOUND('',#15616,.T.);
#11507=FACE_OUTER_BOUND('',#15617,.T.);
#11508=FACE_OUTER_BOUND('',#15618,.T.);
#11509=FACE_OUTER_BOUND('',#15619,.T.);
#11510=FACE_OUTER_BOUND('',#15620,.T.);
#11511=FACE_OUTER_BOUND('',#15621,.T.);
#11512=FACE_OUTER_BOUND('',#15622,.T.);
#11513=FACE_OUTER_BOUND('',#15623,.T.);
#11514=FACE_OUTER_BOUND('',#15624,.T.);
#11515=FACE_OUTER_BOUND('',#15625,.T.);
#11516=FACE_OUTER_BOUND('',#15626,.T.);
#11517=FACE_OUTER_BOUND('',#15627,.T.);
#11518=FACE_OUTER_BOUND('',#15628,.T.);
#11519=FACE_OUTER_BOUND('',#15629,.T.);
#11520=FACE_OUTER_BOUND('',#15630,.T.);
#11521=FACE_OUTER_BOUND('',#15631,.T.);
#11522=FACE_OUTER_BOUND('',#15632,.T.);
#11523=FACE_OUTER_BOUND('',#15633,.T.);
#11524=FACE_OUTER_BOUND('',#15634,.T.);
#11525=FACE_OUTER_BOUND('',#15635,.T.);
#11526=FACE_OUTER_BOUND('',#15636,.T.);
#11527=FACE_OUTER_BOUND('',#15637,.T.);
#11528=FACE_OUTER_BOUND('',#15638,.T.);
#11529=FACE_OUTER_BOUND('',#15639,.T.);
#11530=FACE_OUTER_BOUND('',#15640,.T.);
#11531=FACE_OUTER_BOUND('',#15641,.T.);
#11532=FACE_OUTER_BOUND('',#15642,.T.);
#11533=FACE_OUTER_BOUND('',#15643,.T.);
#11534=FACE_OUTER_BOUND('',#15644,.T.);
#11535=FACE_OUTER_BOUND('',#15645,.T.);
#11536=FACE_OUTER_BOUND('',#15646,.T.);
#11537=FACE_OUTER_BOUND('',#15647,.T.);
#11538=FACE_OUTER_BOUND('',#15648,.T.);
#11539=FACE_OUTER_BOUND('',#15649,.T.);
#11540=FACE_OUTER_BOUND('',#15650,.T.);
#11541=FACE_OUTER_BOUND('',#15651,.T.);
#11542=FACE_OUTER_BOUND('',#15652,.T.);
#11543=FACE_OUTER_BOUND('',#15653,.T.);
#11544=FACE_OUTER_BOUND('',#15654,.T.);
#11545=FACE_OUTER_BOUND('',#15655,.T.);
#11546=FACE_OUTER_BOUND('',#15656,.T.);
#11547=FACE_OUTER_BOUND('',#15657,.T.);
#11548=FACE_OUTER_BOUND('',#15658,.T.);
#11549=FACE_OUTER_BOUND('',#15659,.T.);
#11550=FACE_OUTER_BOUND('',#15660,.T.);
#11551=FACE_OUTER_BOUND('',#15661,.T.);
#11552=FACE_OUTER_BOUND('',#15662,.T.);
#11553=FACE_OUTER_BOUND('',#15663,.T.);
#11554=FACE_OUTER_BOUND('',#15664,.T.);
#11555=FACE_OUTER_BOUND('',#15665,.T.);
#11556=FACE_OUTER_BOUND('',#15666,.T.);
#11557=FACE_OUTER_BOUND('',#15667,.T.);
#11558=FACE_OUTER_BOUND('',#15668,.T.);
#11559=FACE_OUTER_BOUND('',#15669,.T.);
#11560=FACE_OUTER_BOUND('',#15670,.T.);
#11561=FACE_OUTER_BOUND('',#15671,.T.);
#11562=FACE_OUTER_BOUND('',#15672,.T.);
#11563=FACE_OUTER_BOUND('',#15673,.T.);
#11564=FACE_OUTER_BOUND('',#15674,.T.);
#11565=FACE_OUTER_BOUND('',#15675,.T.);
#11566=FACE_OUTER_BOUND('',#15676,.T.);
#11567=FACE_OUTER_BOUND('',#15677,.T.);
#11568=FACE_OUTER_BOUND('',#15678,.T.);
#11569=FACE_OUTER_BOUND('',#15679,.T.);
#11570=FACE_OUTER_BOUND('',#15680,.T.);
#11571=FACE_OUTER_BOUND('',#15681,.T.);
#11572=FACE_OUTER_BOUND('',#15682,.T.);
#11573=FACE_OUTER_BOUND('',#15683,.T.);
#11574=FACE_OUTER_BOUND('',#15684,.T.);
#11575=FACE_OUTER_BOUND('',#15685,.T.);
#11576=FACE_OUTER_BOUND('',#15686,.T.);
#11577=FACE_OUTER_BOUND('',#15687,.T.);
#11578=FACE_OUTER_BOUND('',#15688,.T.);
#11579=FACE_OUTER_BOUND('',#15689,.T.);
#11580=FACE_OUTER_BOUND('',#15690,.T.);
#11581=FACE_OUTER_BOUND('',#15691,.T.);
#11582=FACE_OUTER_BOUND('',#15692,.T.);
#11583=FACE_OUTER_BOUND('',#15693,.T.);
#11584=FACE_OUTER_BOUND('',#15694,.T.);
#11585=FACE_OUTER_BOUND('',#15695,.T.);
#11586=FACE_OUTER_BOUND('',#15696,.T.);
#11587=FACE_OUTER_BOUND('',#15697,.T.);
#11588=FACE_OUTER_BOUND('',#15698,.T.);
#11589=FACE_OUTER_BOUND('',#15699,.T.);
#11590=FACE_OUTER_BOUND('',#15700,.T.);
#11591=FACE_OUTER_BOUND('',#15701,.T.);
#11592=FACE_OUTER_BOUND('',#15702,.T.);
#11593=FACE_OUTER_BOUND('',#15703,.T.);
#11594=FACE_OUTER_BOUND('',#15704,.T.);
#11595=FACE_OUTER_BOUND('',#15705,.T.);
#11596=FACE_OUTER_BOUND('',#15706,.T.);
#11597=FACE_OUTER_BOUND('',#15707,.T.);
#11598=FACE_OUTER_BOUND('',#15708,.T.);
#11599=FACE_OUTER_BOUND('',#15709,.T.);
#11600=FACE_OUTER_BOUND('',#15710,.T.);
#11601=FACE_OUTER_BOUND('',#15711,.T.);
#11602=FACE_OUTER_BOUND('',#15712,.T.);
#11603=FACE_OUTER_BOUND('',#15713,.T.);
#11604=FACE_OUTER_BOUND('',#15714,.T.);
#11605=FACE_OUTER_BOUND('',#15715,.T.);
#11606=FACE_OUTER_BOUND('',#15716,.T.);
#11607=FACE_OUTER_BOUND('',#15717,.T.);
#11608=FACE_OUTER_BOUND('',#15718,.T.);
#11609=FACE_OUTER_BOUND('',#15719,.T.);
#11610=FACE_OUTER_BOUND('',#15720,.T.);
#11611=FACE_OUTER_BOUND('',#15721,.T.);
#11612=FACE_OUTER_BOUND('',#15722,.T.);
#11613=FACE_OUTER_BOUND('',#15723,.T.);
#11614=FACE_OUTER_BOUND('',#15724,.T.);
#11615=FACE_OUTER_BOUND('',#15725,.T.);
#11616=FACE_OUTER_BOUND('',#15726,.T.);
#11617=FACE_OUTER_BOUND('',#15727,.T.);
#11618=FACE_OUTER_BOUND('',#15728,.T.);
#11619=FACE_OUTER_BOUND('',#15729,.T.);
#11620=FACE_OUTER_BOUND('',#15730,.T.);
#11621=FACE_OUTER_BOUND('',#15731,.T.);
#11622=FACE_OUTER_BOUND('',#15732,.T.);
#11623=FACE_OUTER_BOUND('',#15733,.T.);
#11624=FACE_OUTER_BOUND('',#15734,.T.);
#11625=FACE_OUTER_BOUND('',#15735,.T.);
#11626=FACE_OUTER_BOUND('',#15736,.T.);
#11627=FACE_OUTER_BOUND('',#15737,.T.);
#11628=FACE_OUTER_BOUND('',#15738,.T.);
#11629=FACE_OUTER_BOUND('',#15739,.T.);
#11630=FACE_OUTER_BOUND('',#15740,.T.);
#11631=FACE_OUTER_BOUND('',#15741,.T.);
#11632=FACE_OUTER_BOUND('',#15742,.T.);
#11633=FACE_OUTER_BOUND('',#15743,.T.);
#11634=FACE_OUTER_BOUND('',#15744,.T.);
#11635=FACE_OUTER_BOUND('',#15745,.T.);
#11636=FACE_OUTER_BOUND('',#15746,.T.);
#11637=FACE_OUTER_BOUND('',#15747,.T.);
#11638=FACE_OUTER_BOUND('',#15748,.T.);
#11639=FACE_OUTER_BOUND('',#15749,.T.);
#11640=FACE_OUTER_BOUND('',#15750,.T.);
#11641=FACE_OUTER_BOUND('',#15751,.T.);
#11642=FACE_OUTER_BOUND('',#15752,.T.);
#11643=FACE_OUTER_BOUND('',#15753,.T.);
#11644=FACE_OUTER_BOUND('',#15754,.T.);
#11645=FACE_OUTER_BOUND('',#15755,.T.);
#11646=FACE_OUTER_BOUND('',#15756,.T.);
#11647=FACE_OUTER_BOUND('',#15757,.T.);
#11648=FACE_OUTER_BOUND('',#15758,.T.);
#11649=FACE_OUTER_BOUND('',#15759,.T.);
#11650=FACE_OUTER_BOUND('',#15760,.T.);
#11651=FACE_OUTER_BOUND('',#15761,.T.);
#11652=FACE_OUTER_BOUND('',#15762,.T.);
#11653=FACE_OUTER_BOUND('',#15763,.T.);
#11654=FACE_OUTER_BOUND('',#15764,.T.);
#11655=FACE_OUTER_BOUND('',#15765,.T.);
#11656=FACE_OUTER_BOUND('',#15766,.T.);
#11657=FACE_OUTER_BOUND('',#15767,.T.);
#11658=FACE_OUTER_BOUND('',#15768,.T.);
#11659=FACE_OUTER_BOUND('',#15769,.T.);
#11660=FACE_OUTER_BOUND('',#15770,.T.);
#11661=FACE_OUTER_BOUND('',#15771,.T.);
#11662=FACE_OUTER_BOUND('',#15772,.T.);
#11663=FACE_OUTER_BOUND('',#15773,.T.);
#11664=FACE_OUTER_BOUND('',#15774,.T.);
#11665=FACE_OUTER_BOUND('',#15775,.T.);
#11666=FACE_OUTER_BOUND('',#15776,.T.);
#11667=FACE_OUTER_BOUND('',#15777,.T.);
#11668=FACE_OUTER_BOUND('',#15778,.T.);
#11669=FACE_OUTER_BOUND('',#15779,.T.);
#11670=FACE_OUTER_BOUND('',#15780,.T.);
#11671=FACE_OUTER_BOUND('',#15781,.T.);
#11672=FACE_OUTER_BOUND('',#15782,.T.);
#11673=FACE_OUTER_BOUND('',#15783,.T.);
#11674=FACE_OUTER_BOUND('',#15784,.T.);
#11675=FACE_OUTER_BOUND('',#15785,.T.);
#11676=FACE_OUTER_BOUND('',#15786,.T.);
#11677=FACE_OUTER_BOUND('',#15787,.T.);
#11678=FACE_OUTER_BOUND('',#15788,.T.);
#11679=FACE_OUTER_BOUND('',#15789,.T.);
#11680=FACE_OUTER_BOUND('',#15790,.T.);
#11681=FACE_OUTER_BOUND('',#15791,.T.);
#11682=FACE_OUTER_BOUND('',#15792,.T.);
#11683=FACE_OUTER_BOUND('',#15793,.T.);
#11684=FACE_OUTER_BOUND('',#15794,.T.);
#11685=FACE_OUTER_BOUND('',#15795,.T.);
#11686=FACE_OUTER_BOUND('',#15796,.T.);
#11687=FACE_OUTER_BOUND('',#15797,.T.);
#11688=FACE_OUTER_BOUND('',#15798,.T.);
#11689=FACE_OUTER_BOUND('',#15799,.T.);
#11690=FACE_OUTER_BOUND('',#15800,.T.);
#11691=FACE_OUTER_BOUND('',#15801,.T.);
#11692=FACE_OUTER_BOUND('',#15802,.T.);
#11693=FACE_OUTER_BOUND('',#15803,.T.);
#11694=FACE_OUTER_BOUND('',#15804,.T.);
#11695=FACE_OUTER_BOUND('',#15805,.T.);
#11696=FACE_OUTER_BOUND('',#15806,.T.);
#11697=FACE_OUTER_BOUND('',#15807,.T.);
#11698=FACE_OUTER_BOUND('',#15808,.T.);
#11699=FACE_OUTER_BOUND('',#15809,.T.);
#11700=FACE_OUTER_BOUND('',#15810,.T.);
#11701=FACE_OUTER_BOUND('',#15811,.T.);
#11702=FACE_OUTER_BOUND('',#15812,.T.);
#11703=FACE_OUTER_BOUND('',#15813,.T.);
#11704=FACE_OUTER_BOUND('',#15814,.T.);
#11705=FACE_OUTER_BOUND('',#15815,.T.);
#11706=FACE_OUTER_BOUND('',#15816,.T.);
#11707=FACE_OUTER_BOUND('',#15817,.T.);
#11708=FACE_OUTER_BOUND('',#15818,.T.);
#11709=FACE_OUTER_BOUND('',#15819,.T.);
#11710=FACE_OUTER_BOUND('',#15820,.T.);
#11711=FACE_OUTER_BOUND('',#15821,.T.);
#11712=FACE_OUTER_BOUND('',#15822,.T.);
#11713=FACE_OUTER_BOUND('',#15823,.T.);
#11714=FACE_OUTER_BOUND('',#15824,.T.);
#11715=FACE_OUTER_BOUND('',#15825,.T.);
#11716=FACE_OUTER_BOUND('',#15826,.T.);
#11717=FACE_OUTER_BOUND('',#15827,.T.);
#11718=FACE_OUTER_BOUND('',#15828,.T.);
#11719=FACE_OUTER_BOUND('',#15829,.T.);
#11720=FACE_OUTER_BOUND('',#15830,.T.);
#11721=FACE_OUTER_BOUND('',#15831,.T.);
#11722=FACE_OUTER_BOUND('',#15832,.T.);
#11723=FACE_OUTER_BOUND('',#15833,.T.);
#11724=FACE_OUTER_BOUND('',#15834,.T.);
#11725=FACE_OUTER_BOUND('',#15835,.T.);
#11726=FACE_OUTER_BOUND('',#15836,.T.);
#11727=FACE_OUTER_BOUND('',#15837,.T.);
#11728=FACE_OUTER_BOUND('',#15838,.T.);
#11729=FACE_OUTER_BOUND('',#15839,.T.);
#11730=FACE_OUTER_BOUND('',#15840,.T.);
#11731=FACE_OUTER_BOUND('',#15841,.T.);
#11732=FACE_OUTER_BOUND('',#15842,.T.);
#11733=FACE_OUTER_BOUND('',#15843,.T.);
#11734=FACE_OUTER_BOUND('',#15844,.T.);
#11735=FACE_OUTER_BOUND('',#15845,.T.);
#11736=FACE_OUTER_BOUND('',#15846,.T.);
#11737=FACE_OUTER_BOUND('',#15847,.T.);
#11738=FACE_OUTER_BOUND('',#15848,.T.);
#11739=FACE_OUTER_BOUND('',#15849,.T.);
#11740=FACE_OUTER_BOUND('',#15850,.T.);
#11741=FACE_OUTER_BOUND('',#15851,.T.);
#11742=FACE_OUTER_BOUND('',#15852,.T.);
#11743=FACE_OUTER_BOUND('',#15853,.T.);
#11744=FACE_OUTER_BOUND('',#15854,.T.);
#11745=FACE_OUTER_BOUND('',#15855,.T.);
#11746=FACE_OUTER_BOUND('',#15856,.T.);
#11747=FACE_OUTER_BOUND('',#15857,.T.);
#11748=FACE_OUTER_BOUND('',#15858,.T.);
#11749=FACE_OUTER_BOUND('',#15859,.T.);
#11750=FACE_OUTER_BOUND('',#15860,.T.);
#11751=FACE_OUTER_BOUND('',#15861,.T.);
#11752=FACE_OUTER_BOUND('',#15862,.T.);
#11753=FACE_OUTER_BOUND('',#15863,.T.);
#11754=FACE_OUTER_BOUND('',#15864,.T.);
#11755=FACE_OUTER_BOUND('',#15865,.T.);
#11756=FACE_OUTER_BOUND('',#15866,.T.);
#11757=FACE_OUTER_BOUND('',#15867,.T.);
#11758=FACE_OUTER_BOUND('',#15868,.T.);
#11759=FACE_OUTER_BOUND('',#15869,.T.);
#11760=FACE_OUTER_BOUND('',#15870,.T.);
#11761=FACE_OUTER_BOUND('',#15871,.T.);
#11762=FACE_OUTER_BOUND('',#15872,.T.);
#11763=FACE_OUTER_BOUND('',#15873,.T.);
#11764=FACE_OUTER_BOUND('',#15874,.T.);
#11765=FACE_OUTER_BOUND('',#15875,.T.);
#11766=FACE_OUTER_BOUND('',#15876,.T.);
#11767=FACE_OUTER_BOUND('',#15877,.T.);
#11768=FACE_OUTER_BOUND('',#15878,.T.);
#11769=FACE_OUTER_BOUND('',#15879,.T.);
#11770=FACE_OUTER_BOUND('',#15880,.T.);
#11771=FACE_OUTER_BOUND('',#15881,.T.);
#11772=FACE_OUTER_BOUND('',#15882,.T.);
#11773=FACE_OUTER_BOUND('',#15883,.T.);
#11774=FACE_OUTER_BOUND('',#15884,.T.);
#11775=FACE_OUTER_BOUND('',#15885,.T.);
#11776=FACE_OUTER_BOUND('',#15886,.T.);
#11777=FACE_OUTER_BOUND('',#15887,.T.);
#11778=FACE_OUTER_BOUND('',#15888,.T.);
#11779=FACE_OUTER_BOUND('',#15889,.T.);
#11780=FACE_OUTER_BOUND('',#15890,.T.);
#11781=FACE_OUTER_BOUND('',#15891,.T.);
#11782=FACE_OUTER_BOUND('',#15892,.T.);
#11783=FACE_OUTER_BOUND('',#15893,.T.);
#11784=FACE_OUTER_BOUND('',#15894,.T.);
#11785=FACE_OUTER_BOUND('',#15895,.T.);
#11786=FACE_OUTER_BOUND('',#15896,.T.);
#11787=FACE_OUTER_BOUND('',#15897,.T.);
#11788=FACE_OUTER_BOUND('',#15898,.T.);
#11789=FACE_OUTER_BOUND('',#15899,.T.);
#11790=FACE_OUTER_BOUND('',#15900,.T.);
#11791=FACE_OUTER_BOUND('',#15901,.T.);
#11792=FACE_OUTER_BOUND('',#15902,.T.);
#11793=FACE_OUTER_BOUND('',#15903,.T.);
#11794=FACE_OUTER_BOUND('',#15904,.T.);
#11795=FACE_OUTER_BOUND('',#15905,.T.);
#11796=FACE_OUTER_BOUND('',#15906,.T.);
#11797=FACE_OUTER_BOUND('',#15907,.T.);
#11798=FACE_OUTER_BOUND('',#15908,.T.);
#11799=FACE_OUTER_BOUND('',#15909,.T.);
#11800=FACE_OUTER_BOUND('',#15910,.T.);
#11801=FACE_OUTER_BOUND('',#15911,.T.);
#11802=FACE_OUTER_BOUND('',#15912,.T.);
#11803=FACE_OUTER_BOUND('',#15913,.T.);
#11804=FACE_OUTER_BOUND('',#15914,.T.);
#11805=FACE_OUTER_BOUND('',#15915,.T.);
#11806=FACE_OUTER_BOUND('',#15916,.T.);
#11807=FACE_OUTER_BOUND('',#15917,.T.);
#11808=FACE_OUTER_BOUND('',#15918,.T.);
#11809=FACE_OUTER_BOUND('',#15919,.T.);
#11810=FACE_OUTER_BOUND('',#15920,.T.);
#11811=FACE_OUTER_BOUND('',#15921,.T.);
#11812=FACE_OUTER_BOUND('',#15922,.T.);
#11813=FACE_OUTER_BOUND('',#15923,.T.);
#11814=FACE_OUTER_BOUND('',#15924,.T.);
#11815=FACE_OUTER_BOUND('',#15925,.T.);
#11816=FACE_OUTER_BOUND('',#15926,.T.);
#11817=FACE_OUTER_BOUND('',#15927,.T.);
#11818=FACE_OUTER_BOUND('',#15928,.T.);
#11819=FACE_OUTER_BOUND('',#15929,.T.);
#11820=FACE_OUTER_BOUND('',#15930,.T.);
#11821=FACE_OUTER_BOUND('',#15931,.T.);
#11822=FACE_OUTER_BOUND('',#15932,.T.);
#11823=FACE_OUTER_BOUND('',#15933,.T.);
#11824=FACE_OUTER_BOUND('',#15934,.T.);
#11825=FACE_OUTER_BOUND('',#15935,.T.);
#11826=FACE_OUTER_BOUND('',#15936,.T.);
#11827=FACE_OUTER_BOUND('',#15937,.T.);
#11828=FACE_OUTER_BOUND('',#15938,.T.);
#11829=FACE_OUTER_BOUND('',#15939,.T.);
#11830=FACE_OUTER_BOUND('',#15940,.T.);
#11831=FACE_OUTER_BOUND('',#15941,.T.);
#11832=FACE_OUTER_BOUND('',#15942,.T.);
#11833=FACE_OUTER_BOUND('',#15943,.T.);
#11834=FACE_OUTER_BOUND('',#15944,.T.);
#11835=FACE_OUTER_BOUND('',#15945,.T.);
#11836=FACE_OUTER_BOUND('',#15946,.T.);
#11837=FACE_OUTER_BOUND('',#15947,.T.);
#11838=FACE_OUTER_BOUND('',#15948,.T.);
#11839=FACE_OUTER_BOUND('',#15949,.T.);
#11840=FACE_OUTER_BOUND('',#15950,.T.);
#11841=FACE_OUTER_BOUND('',#15951,.T.);
#11842=FACE_OUTER_BOUND('',#15952,.T.);
#11843=FACE_OUTER_BOUND('',#15953,.T.);
#11844=FACE_OUTER_BOUND('',#15954,.T.);
#11845=FACE_OUTER_BOUND('',#15955,.T.);
#11846=FACE_OUTER_BOUND('',#15956,.T.);
#11847=FACE_OUTER_BOUND('',#15957,.T.);
#11848=FACE_OUTER_BOUND('',#15958,.T.);
#11849=FACE_OUTER_BOUND('',#15959,.T.);
#11850=FACE_OUTER_BOUND('',#15960,.T.);
#11851=FACE_OUTER_BOUND('',#15961,.T.);
#11852=FACE_OUTER_BOUND('',#15962,.T.);
#11853=FACE_OUTER_BOUND('',#15963,.T.);
#11854=FACE_OUTER_BOUND('',#15964,.T.);
#11855=FACE_OUTER_BOUND('',#15965,.T.);
#11856=FACE_OUTER_BOUND('',#15966,.T.);
#11857=FACE_OUTER_BOUND('',#15967,.T.);
#11858=FACE_OUTER_BOUND('',#15968,.T.);
#11859=FACE_OUTER_BOUND('',#15969,.T.);
#11860=FACE_OUTER_BOUND('',#15970,.T.);
#11861=FACE_OUTER_BOUND('',#15971,.T.);
#11862=FACE_OUTER_BOUND('',#15972,.T.);
#11863=FACE_OUTER_BOUND('',#15973,.T.);
#11864=FACE_OUTER_BOUND('',#15974,.T.);
#11865=FACE_OUTER_BOUND('',#15975,.T.);
#11866=FACE_OUTER_BOUND('',#15976,.T.);
#11867=FACE_OUTER_BOUND('',#15977,.T.);
#11868=FACE_OUTER_BOUND('',#15978,.T.);
#11869=FACE_OUTER_BOUND('',#15979,.T.);
#11870=FACE_OUTER_BOUND('',#15980,.T.);
#11871=FACE_OUTER_BOUND('',#15981,.T.);
#11872=FACE_OUTER_BOUND('',#15982,.T.);
#11873=FACE_OUTER_BOUND('',#15983,.T.);
#11874=FACE_OUTER_BOUND('',#15984,.T.);
#11875=FACE_OUTER_BOUND('',#15985,.T.);
#11876=FACE_OUTER_BOUND('',#15986,.T.);
#11877=FACE_OUTER_BOUND('',#15987,.T.);
#11878=FACE_OUTER_BOUND('',#15988,.T.);
#11879=FACE_OUTER_BOUND('',#15989,.T.);
#11880=FACE_OUTER_BOUND('',#15990,.T.);
#11881=FACE_OUTER_BOUND('',#15991,.T.);
#11882=FACE_OUTER_BOUND('',#15992,.T.);
#11883=FACE_OUTER_BOUND('',#15993,.T.);
#11884=FACE_OUTER_BOUND('',#15994,.T.);
#11885=FACE_OUTER_BOUND('',#15995,.T.);
#11886=FACE_OUTER_BOUND('',#15996,.T.);
#11887=FACE_OUTER_BOUND('',#15997,.T.);
#11888=FACE_OUTER_BOUND('',#15998,.T.);
#11889=FACE_OUTER_BOUND('',#15999,.T.);
#11890=FACE_OUTER_BOUND('',#16000,.T.);
#11891=FACE_OUTER_BOUND('',#16001,.T.);
#11892=FACE_OUTER_BOUND('',#16002,.T.);
#11893=FACE_OUTER_BOUND('',#16003,.T.);
#11894=FACE_OUTER_BOUND('',#16004,.T.);
#11895=FACE_OUTER_BOUND('',#16005,.T.);
#11896=FACE_OUTER_BOUND('',#16006,.T.);
#11897=FACE_OUTER_BOUND('',#16007,.T.);
#11898=FACE_OUTER_BOUND('',#16008,.T.);
#11899=FACE_OUTER_BOUND('',#16009,.T.);
#11900=FACE_OUTER_BOUND('',#16010,.T.);
#11901=FACE_OUTER_BOUND('',#16011,.T.);
#11902=FACE_OUTER_BOUND('',#16012,.T.);
#11903=FACE_OUTER_BOUND('',#16013,.T.);
#11904=FACE_OUTER_BOUND('',#16014,.T.);
#11905=FACE_OUTER_BOUND('',#16015,.T.);
#11906=FACE_OUTER_BOUND('',#16016,.T.);
#11907=FACE_OUTER_BOUND('',#16017,.T.);
#11908=FACE_OUTER_BOUND('',#16018,.T.);
#11909=FACE_OUTER_BOUND('',#16019,.T.);
#11910=FACE_OUTER_BOUND('',#16020,.T.);
#11911=FACE_OUTER_BOUND('',#16021,.T.);
#11912=FACE_OUTER_BOUND('',#16022,.T.);
#11913=FACE_OUTER_BOUND('',#16023,.T.);
#11914=FACE_OUTER_BOUND('',#16024,.T.);
#11915=FACE_OUTER_BOUND('',#16025,.T.);
#11916=FACE_OUTER_BOUND('',#16026,.T.);
#11917=FACE_OUTER_BOUND('',#16027,.T.);
#11918=FACE_OUTER_BOUND('',#16028,.T.);
#11919=FACE_OUTER_BOUND('',#16029,.T.);
#11920=FACE_OUTER_BOUND('',#16030,.T.);
#11921=FACE_OUTER_BOUND('',#16031,.T.);
#11922=FACE_OUTER_BOUND('',#16032,.T.);
#11923=FACE_OUTER_BOUND('',#16033,.T.);
#11924=FACE_OUTER_BOUND('',#16034,.T.);
#11925=FACE_OUTER_BOUND('',#16035,.T.);
#11926=FACE_OUTER_BOUND('',#16036,.T.);
#11927=FACE_OUTER_BOUND('',#16037,.T.);
#11928=FACE_OUTER_BOUND('',#16038,.T.);
#11929=FACE_OUTER_BOUND('',#16039,.T.);
#11930=FACE_OUTER_BOUND('',#16040,.T.);
#11931=FACE_OUTER_BOUND('',#16041,.T.);
#11932=FACE_OUTER_BOUND('',#16042,.T.);
#11933=FACE_OUTER_BOUND('',#16043,.T.);
#11934=FACE_OUTER_BOUND('',#16044,.T.);
#11935=FACE_OUTER_BOUND('',#16045,.T.);
#11936=FACE_OUTER_BOUND('',#16046,.T.);
#11937=FACE_OUTER_BOUND('',#16047,.T.);
#11938=FACE_OUTER_BOUND('',#16048,.T.);
#11939=FACE_OUTER_BOUND('',#16049,.T.);
#11940=FACE_OUTER_BOUND('',#16050,.T.);
#11941=FACE_OUTER_BOUND('',#16051,.T.);
#11942=FACE_OUTER_BOUND('',#16052,.T.);
#11943=FACE_OUTER_BOUND('',#16053,.T.);
#11944=FACE_OUTER_BOUND('',#16054,.T.);
#11945=FACE_OUTER_BOUND('',#16055,.T.);
#11946=FACE_OUTER_BOUND('',#16056,.T.);
#11947=FACE_OUTER_BOUND('',#16057,.T.);
#11948=FACE_OUTER_BOUND('',#16058,.T.);
#11949=FACE_OUTER_BOUND('',#16059,.T.);
#11950=FACE_OUTER_BOUND('',#16060,.T.);
#11951=FACE_OUTER_BOUND('',#16061,.T.);
#11952=FACE_OUTER_BOUND('',#16062,.T.);
#11953=FACE_OUTER_BOUND('',#16063,.T.);
#11954=FACE_OUTER_BOUND('',#16064,.T.);
#11955=FACE_OUTER_BOUND('',#16065,.T.);
#11956=FACE_OUTER_BOUND('',#16066,.T.);
#11957=FACE_OUTER_BOUND('',#16067,.T.);
#11958=FACE_OUTER_BOUND('',#16068,.T.);
#11959=FACE_OUTER_BOUND('',#16069,.T.);
#11960=FACE_OUTER_BOUND('',#16070,.T.);
#11961=FACE_OUTER_BOUND('',#16071,.T.);
#11962=FACE_OUTER_BOUND('',#16072,.T.);
#11963=FACE_OUTER_BOUND('',#16073,.T.);
#11964=FACE_OUTER_BOUND('',#16074,.T.);
#11965=FACE_OUTER_BOUND('',#16075,.T.);
#11966=FACE_OUTER_BOUND('',#16076,.T.);
#11967=FACE_OUTER_BOUND('',#16077,.T.);
#11968=FACE_OUTER_BOUND('',#16078,.T.);
#11969=FACE_OUTER_BOUND('',#16079,.T.);
#11970=FACE_OUTER_BOUND('',#16080,.T.);
#11971=FACE_OUTER_BOUND('',#16081,.T.);
#11972=FACE_OUTER_BOUND('',#16082,.T.);
#11973=FACE_OUTER_BOUND('',#16083,.T.);
#11974=FACE_OUTER_BOUND('',#16084,.T.);
#11975=FACE_OUTER_BOUND('',#16085,.T.);
#11976=FACE_OUTER_BOUND('',#16086,.T.);
#11977=FACE_OUTER_BOUND('',#16087,.T.);
#11978=FACE_OUTER_BOUND('',#16088,.T.);
#11979=FACE_OUTER_BOUND('',#16089,.T.);
#11980=FACE_OUTER_BOUND('',#16090,.T.);
#11981=FACE_OUTER_BOUND('',#16091,.T.);
#11982=FACE_OUTER_BOUND('',#16092,.T.);
#11983=FACE_OUTER_BOUND('',#16093,.T.);
#11984=FACE_OUTER_BOUND('',#16094,.T.);
#11985=FACE_OUTER_BOUND('',#16095,.T.);
#11986=FACE_OUTER_BOUND('',#16096,.T.);
#11987=FACE_OUTER_BOUND('',#16097,.T.);
#11988=FACE_OUTER_BOUND('',#16098,.T.);
#11989=FACE_OUTER_BOUND('',#16099,.T.);
#11990=FACE_OUTER_BOUND('',#16100,.T.);
#11991=FACE_OUTER_BOUND('',#16101,.T.);
#11992=FACE_OUTER_BOUND('',#16102,.T.);
#11993=FACE_OUTER_BOUND('',#16103,.T.);
#11994=FACE_OUTER_BOUND('',#16104,.T.);
#11995=FACE_OUTER_BOUND('',#16105,.T.);
#11996=FACE_OUTER_BOUND('',#16106,.T.);
#11997=FACE_OUTER_BOUND('',#16107,.T.);
#11998=FACE_OUTER_BOUND('',#16108,.T.);
#11999=FACE_OUTER_BOUND('',#16109,.T.);
#12000=FACE_OUTER_BOUND('',#16110,.T.);
#12001=FACE_OUTER_BOUND('',#16111,.T.);
#12002=FACE_OUTER_BOUND('',#16112,.T.);
#12003=FACE_OUTER_BOUND('',#16113,.T.);
#12004=FACE_OUTER_BOUND('',#16114,.T.);
#12005=FACE_OUTER_BOUND('',#16115,.T.);
#12006=FACE_OUTER_BOUND('',#16116,.T.);
#12007=FACE_OUTER_BOUND('',#16117,.T.);
#12008=FACE_OUTER_BOUND('',#16118,.T.);
#12009=FACE_OUTER_BOUND('',#16119,.T.);
#12010=FACE_OUTER_BOUND('',#16120,.T.);
#12011=FACE_OUTER_BOUND('',#16121,.T.);
#12012=FACE_OUTER_BOUND('',#16122,.T.);
#12013=FACE_OUTER_BOUND('',#16123,.T.);
#12014=FACE_OUTER_BOUND('',#16124,.T.);
#12015=FACE_OUTER_BOUND('',#16125,.T.);
#12016=FACE_OUTER_BOUND('',#16126,.T.);
#12017=FACE_OUTER_BOUND('',#16127,.T.);
#12018=FACE_OUTER_BOUND('',#16128,.T.);
#12019=FACE_OUTER_BOUND('',#16129,.T.);
#12020=FACE_OUTER_BOUND('',#16130,.T.);
#12021=FACE_OUTER_BOUND('',#16131,.T.);
#12022=FACE_OUTER_BOUND('',#16132,.T.);
#12023=FACE_OUTER_BOUND('',#16133,.T.);
#12024=FACE_OUTER_BOUND('',#16134,.T.);
#12025=FACE_OUTER_BOUND('',#16135,.T.);
#12026=FACE_OUTER_BOUND('',#16136,.T.);
#12027=FACE_OUTER_BOUND('',#16137,.T.);
#12028=FACE_OUTER_BOUND('',#16138,.T.);
#12029=FACE_OUTER_BOUND('',#16139,.T.);
#12030=FACE_OUTER_BOUND('',#16140,.T.);
#12031=FACE_OUTER_BOUND('',#16141,.T.);
#12032=FACE_OUTER_BOUND('',#16142,.T.);
#12033=FACE_OUTER_BOUND('',#16143,.T.);
#12034=FACE_OUTER_BOUND('',#16144,.T.);
#12035=FACE_OUTER_BOUND('',#16145,.T.);
#12036=FACE_OUTER_BOUND('',#16146,.T.);
#12037=FACE_OUTER_BOUND('',#16147,.T.);
#12038=FACE_OUTER_BOUND('',#16148,.T.);
#12039=FACE_OUTER_BOUND('',#16149,.T.);
#12040=FACE_OUTER_BOUND('',#16150,.T.);
#12041=FACE_OUTER_BOUND('',#16151,.T.);
#12042=FACE_OUTER_BOUND('',#16152,.T.);
#12043=FACE_OUTER_BOUND('',#16153,.T.);
#12044=FACE_OUTER_BOUND('',#16154,.T.);
#12045=FACE_OUTER_BOUND('',#16155,.T.);
#12046=FACE_OUTER_BOUND('',#16156,.T.);
#12047=FACE_OUTER_BOUND('',#16157,.T.);
#12048=FACE_OUTER_BOUND('',#16158,.T.);
#12049=FACE_OUTER_BOUND('',#16159,.T.);
#12050=FACE_OUTER_BOUND('',#16160,.T.);
#12051=FACE_OUTER_BOUND('',#16161,.T.);
#12052=FACE_OUTER_BOUND('',#16162,.T.);
#12053=FACE_OUTER_BOUND('',#16163,.T.);
#12054=FACE_OUTER_BOUND('',#16164,.T.);
#12055=FACE_OUTER_BOUND('',#16165,.T.);
#12056=FACE_OUTER_BOUND('',#16166,.T.);
#12057=FACE_OUTER_BOUND('',#16167,.T.);
#12058=FACE_OUTER_BOUND('',#16168,.T.);
#12059=FACE_OUTER_BOUND('',#16169,.T.);
#12060=FACE_OUTER_BOUND('',#16170,.T.);
#12061=FACE_OUTER_BOUND('',#16171,.T.);
#12062=FACE_OUTER_BOUND('',#16172,.T.);
#12063=FACE_OUTER_BOUND('',#16173,.T.);
#12064=FACE_OUTER_BOUND('',#16174,.T.);
#12065=FACE_OUTER_BOUND('',#16175,.T.);
#12066=FACE_OUTER_BOUND('',#16176,.T.);
#12067=FACE_OUTER_BOUND('',#16177,.T.);
#12068=FACE_OUTER_BOUND('',#16178,.T.);
#12069=FACE_OUTER_BOUND('',#16179,.T.);
#12070=FACE_OUTER_BOUND('',#16180,.T.);
#12071=FACE_OUTER_BOUND('',#16181,.T.);
#12072=FACE_OUTER_BOUND('',#16182,.T.);
#12073=FACE_OUTER_BOUND('',#16184,.T.);
#12074=FACE_OUTER_BOUND('',#16185,.T.);
#12075=FACE_OUTER_BOUND('',#16186,.T.);
#12076=FACE_OUTER_BOUND('',#16187,.T.);
#12077=FACE_OUTER_BOUND('',#16188,.T.);
#12078=FACE_OUTER_BOUND('',#16189,.T.);
#12079=FACE_OUTER_BOUND('',#16190,.T.);
#12080=FACE_OUTER_BOUND('',#16191,.T.);
#12081=FACE_OUTER_BOUND('',#16192,.T.);
#12082=FACE_OUTER_BOUND('',#16194,.T.);
#12083=FACE_OUTER_BOUND('',#16195,.T.);
#12084=FACE_OUTER_BOUND('',#16197,.T.);
#12085=FACE_OUTER_BOUND('',#16199,.T.);
#12086=FACE_OUTER_BOUND('',#16201,.T.);
#12087=FACE_OUTER_BOUND('',#16202,.T.);
#12088=FACE_OUTER_BOUND('',#16204,.T.);
#12089=FACE_OUTER_BOUND('',#16475,.T.);
#12090=FACE_OUTER_BOUND('',#16536,.T.);
#12091=FACE_OUTER_BOUND('',#16537,.T.);
#12092=FACE_OUTER_BOUND('',#16539,.T.);
#12093=FACE_OUTER_BOUND('',#16540,.T.);
#12094=FACE_OUTER_BOUND('',#16542,.T.);
#12095=FACE_OUTER_BOUND('',#16543,.T.);
#12096=FACE_OUTER_BOUND('',#16545,.T.);
#12097=FACE_OUTER_BOUND('',#16546,.T.);
#12098=FACE_OUTER_BOUND('',#16548,.T.);
#12099=FACE_OUTER_BOUND('',#16549,.T.);
#12100=FACE_OUTER_BOUND('',#16551,.T.);
#12101=FACE_OUTER_BOUND('',#16552,.T.);
#12102=FACE_OUTER_BOUND('',#16554,.T.);
#12103=FACE_OUTER_BOUND('',#16555,.T.);
#12104=FACE_OUTER_BOUND('',#16557,.T.);
#12105=FACE_OUTER_BOUND('',#16558,.T.);
#12106=FACE_OUTER_BOUND('',#16560,.T.);
#12107=FACE_OUTER_BOUND('',#16561,.T.);
#12108=FACE_OUTER_BOUND('',#16563,.T.);
#12109=FACE_OUTER_BOUND('',#16564,.T.);
#12110=FACE_OUTER_BOUND('',#16566,.T.);
#12111=FACE_OUTER_BOUND('',#16567,.T.);
#12112=FACE_OUTER_BOUND('',#16569,.T.);
#12113=FACE_OUTER_BOUND('',#16570,.T.);
#12114=FACE_OUTER_BOUND('',#16572,.T.);
#12115=FACE_OUTER_BOUND('',#16573,.T.);
#12116=FACE_OUTER_BOUND('',#16575,.T.);
#12117=FACE_OUTER_BOUND('',#16576,.T.);
#12118=FACE_OUTER_BOUND('',#16578,.T.);
#12119=FACE_OUTER_BOUND('',#16579,.T.);
#12120=FACE_OUTER_BOUND('',#16581,.T.);
#12121=FACE_OUTER_BOUND('',#16582,.T.);
#12122=FACE_OUTER_BOUND('',#16584,.T.);
#12123=FACE_OUTER_BOUND('',#16585,.T.);
#12124=FACE_OUTER_BOUND('',#16587,.T.);
#12125=FACE_OUTER_BOUND('',#16588,.T.);
#12126=FACE_OUTER_BOUND('',#16590,.T.);
#12127=FACE_OUTER_BOUND('',#16591,.T.);
#12128=FACE_OUTER_BOUND('',#16593,.T.);
#12129=FACE_OUTER_BOUND('',#16594,.T.);
#12130=FACE_OUTER_BOUND('',#16596,.T.);
#12131=FACE_OUTER_BOUND('',#16597,.T.);
#12132=FACE_OUTER_BOUND('',#16599,.T.);
#12133=FACE_OUTER_BOUND('',#16600,.T.);
#12134=FACE_OUTER_BOUND('',#16602,.T.);
#12135=FACE_OUTER_BOUND('',#16603,.T.);
#12136=FACE_OUTER_BOUND('',#16605,.T.);
#12137=FACE_OUTER_BOUND('',#16606,.T.);
#12138=FACE_OUTER_BOUND('',#16608,.T.);
#12139=FACE_OUTER_BOUND('',#16609,.T.);
#12140=FACE_OUTER_BOUND('',#16611,.T.);
#12141=FACE_OUTER_BOUND('',#16612,.T.);
#12142=FACE_OUTER_BOUND('',#16614,.T.);
#12143=FACE_OUTER_BOUND('',#16615,.T.);
#12144=FACE_OUTER_BOUND('',#16617,.T.);
#12145=FACE_OUTER_BOUND('',#16618,.T.);
#12146=FACE_OUTER_BOUND('',#16620,.T.);
#12147=FACE_OUTER_BOUND('',#16621,.T.);
#12148=FACE_OUTER_BOUND('',#16623,.T.);
#12149=FACE_OUTER_BOUND('',#16624,.T.);
#12150=FACE_OUTER_BOUND('',#16626,.T.);
#12151=FACE_OUTER_BOUND('',#16627,.T.);
#12152=FACE_OUTER_BOUND('',#16629,.T.);
#12153=FACE_OUTER_BOUND('',#16630,.T.);
#12154=FACE_OUTER_BOUND('',#16632,.T.);
#12155=FACE_OUTER_BOUND('',#16633,.T.);
#12156=FACE_OUTER_BOUND('',#16635,.T.);
#12157=FACE_OUTER_BOUND('',#16636,.T.);
#12158=FACE_OUTER_BOUND('',#16638,.T.);
#12159=FACE_OUTER_BOUND('',#16639,.T.);
#12160=FACE_OUTER_BOUND('',#16641,.T.);
#12161=FACE_OUTER_BOUND('',#16642,.T.);
#12162=FACE_OUTER_BOUND('',#16644,.T.);
#12163=FACE_OUTER_BOUND('',#16645,.T.);
#12164=FACE_OUTER_BOUND('',#16647,.T.);
#12165=FACE_OUTER_BOUND('',#16648,.T.);
#12166=FACE_OUTER_BOUND('',#16650,.T.);
#12167=FACE_OUTER_BOUND('',#16651,.T.);
#12168=FACE_OUTER_BOUND('',#16653,.T.);
#12169=FACE_OUTER_BOUND('',#16654,.T.);
#12170=FACE_OUTER_BOUND('',#16656,.T.);
#12171=FACE_OUTER_BOUND('',#16657,.T.);
#12172=FACE_OUTER_BOUND('',#16659,.T.);
#12173=FACE_OUTER_BOUND('',#16660,.T.);
#12174=FACE_OUTER_BOUND('',#16662,.T.);
#12175=FACE_OUTER_BOUND('',#16663,.T.);
#12176=FACE_OUTER_BOUND('',#16665,.T.);
#12177=FACE_OUTER_BOUND('',#16666,.T.);
#12178=FACE_OUTER_BOUND('',#16668,.T.);
#12179=FACE_OUTER_BOUND('',#16669,.T.);
#12180=FACE_OUTER_BOUND('',#16671,.T.);
#12181=FACE_OUTER_BOUND('',#16672,.T.);
#12182=FACE_OUTER_BOUND('',#16674,.T.);
#12183=FACE_OUTER_BOUND('',#16675,.T.);
#12184=FACE_OUTER_BOUND('',#16677,.T.);
#12185=FACE_OUTER_BOUND('',#16678,.T.);
#12186=FACE_OUTER_BOUND('',#16680,.T.);
#12187=FACE_OUTER_BOUND('',#16681,.T.);
#12188=FACE_OUTER_BOUND('',#16683,.T.);
#12189=FACE_OUTER_BOUND('',#16684,.T.);
#12190=FACE_OUTER_BOUND('',#16686,.T.);
#12191=FACE_OUTER_BOUND('',#16687,.T.);
#12192=FACE_OUTER_BOUND('',#16689,.T.);
#12193=FACE_OUTER_BOUND('',#16690,.T.);
#12194=FACE_OUTER_BOUND('',#16692,.T.);
#12195=FACE_OUTER_BOUND('',#16693,.T.);
#12196=FACE_OUTER_BOUND('',#16695,.T.);
#12197=FACE_OUTER_BOUND('',#16696,.T.);
#12198=FACE_OUTER_BOUND('',#16698,.T.);
#12199=FACE_OUTER_BOUND('',#16699,.T.);
#12200=FACE_OUTER_BOUND('',#16701,.T.);
#12201=FACE_OUTER_BOUND('',#16702,.T.);
#12202=FACE_OUTER_BOUND('',#16704,.T.);
#12203=FACE_OUTER_BOUND('',#16705,.T.);
#12204=FACE_OUTER_BOUND('',#16707,.T.);
#12205=FACE_OUTER_BOUND('',#16708,.T.);
#12206=FACE_OUTER_BOUND('',#16710,.T.);
#12207=FACE_OUTER_BOUND('',#16711,.T.);
#12208=FACE_OUTER_BOUND('',#16713,.T.);
#12209=FACE_OUTER_BOUND('',#16714,.T.);
#12210=FACE_OUTER_BOUND('',#16716,.T.);
#12211=FACE_OUTER_BOUND('',#16717,.T.);
#12212=FACE_OUTER_BOUND('',#16719,.T.);
#12213=FACE_OUTER_BOUND('',#16720,.T.);
#12214=FACE_OUTER_BOUND('',#16722,.T.);
#12215=FACE_OUTER_BOUND('',#16723,.T.);
#12216=FACE_OUTER_BOUND('',#16725,.T.);
#12217=FACE_OUTER_BOUND('',#16726,.T.);
#12218=FACE_OUTER_BOUND('',#16728,.T.);
#12219=FACE_OUTER_BOUND('',#16729,.T.);
#12220=FACE_OUTER_BOUND('',#16731,.T.);
#12221=FACE_OUTER_BOUND('',#16732,.T.);
#12222=FACE_OUTER_BOUND('',#16734,.T.);
#12223=FACE_OUTER_BOUND('',#16735,.T.);
#12224=FACE_OUTER_BOUND('',#16737,.T.);
#12225=FACE_OUTER_BOUND('',#16738,.T.);
#12226=FACE_OUTER_BOUND('',#16740,.T.);
#12227=FACE_OUTER_BOUND('',#16741,.T.);
#12228=FACE_OUTER_BOUND('',#16743,.T.);
#12229=FACE_OUTER_BOUND('',#16744,.T.);
#12230=FACE_OUTER_BOUND('',#16746,.T.);
#12231=FACE_OUTER_BOUND('',#16747,.T.);
#12232=FACE_OUTER_BOUND('',#16749,.T.);
#12233=FACE_OUTER_BOUND('',#16750,.T.);
#12234=FACE_OUTER_BOUND('',#16752,.T.);
#12235=FACE_OUTER_BOUND('',#16753,.T.);
#12236=FACE_OUTER_BOUND('',#16755,.T.);
#12237=FACE_OUTER_BOUND('',#16756,.T.);
#12238=FACE_OUTER_BOUND('',#16758,.T.);
#12239=FACE_OUTER_BOUND('',#16759,.T.);
#12240=FACE_OUTER_BOUND('',#16761,.T.);
#12241=FACE_OUTER_BOUND('',#16762,.T.);
#12242=FACE_OUTER_BOUND('',#16764,.T.);
#12243=FACE_OUTER_BOUND('',#16765,.T.);
#12244=FACE_OUTER_BOUND('',#16767,.T.);
#12245=FACE_OUTER_BOUND('',#16768,.T.);
#12246=FACE_OUTER_BOUND('',#16770,.T.);
#12247=FACE_OUTER_BOUND('',#16771,.T.);
#12248=FACE_OUTER_BOUND('',#16773,.T.);
#12249=FACE_OUTER_BOUND('',#16774,.T.);
#12250=FACE_OUTER_BOUND('',#16776,.T.);
#12251=FACE_OUTER_BOUND('',#16777,.T.);
#12252=FACE_OUTER_BOUND('',#16779,.T.);
#12253=FACE_OUTER_BOUND('',#16780,.T.);
#12254=FACE_OUTER_BOUND('',#16782,.T.);
#12255=FACE_OUTER_BOUND('',#16783,.T.);
#12256=FACE_OUTER_BOUND('',#16785,.T.);
#12257=FACE_OUTER_BOUND('',#16786,.T.);
#12258=FACE_OUTER_BOUND('',#16788,.T.);
#12259=FACE_OUTER_BOUND('',#16789,.T.);
#12260=FACE_OUTER_BOUND('',#16791,.T.);
#12261=FACE_OUTER_BOUND('',#16792,.T.);
#12262=FACE_OUTER_BOUND('',#16794,.T.);
#12263=FACE_OUTER_BOUND('',#16795,.T.);
#12264=FACE_OUTER_BOUND('',#16797,.T.);
#12265=FACE_OUTER_BOUND('',#16798,.T.);
#12266=FACE_OUTER_BOUND('',#16800,.T.);
#12267=FACE_OUTER_BOUND('',#16801,.T.);
#12268=FACE_OUTER_BOUND('',#16803,.T.);
#12269=FACE_OUTER_BOUND('',#16804,.T.);
#12270=FACE_OUTER_BOUND('',#16806,.T.);
#12271=FACE_OUTER_BOUND('',#16807,.T.);
#12272=FACE_OUTER_BOUND('',#16809,.T.);
#12273=FACE_OUTER_BOUND('',#16810,.T.);
#12274=FACE_OUTER_BOUND('',#16812,.T.);
#12275=FACE_OUTER_BOUND('',#16813,.T.);
#12276=FACE_OUTER_BOUND('',#16815,.T.);
#12277=FACE_OUTER_BOUND('',#16816,.T.);
#12278=FACE_OUTER_BOUND('',#16818,.T.);
#12279=FACE_OUTER_BOUND('',#16819,.T.);
#12280=FACE_OUTER_BOUND('',#16821,.T.);
#12281=FACE_OUTER_BOUND('',#16822,.T.);
#12282=FACE_OUTER_BOUND('',#16824,.T.);
#12283=FACE_OUTER_BOUND('',#16825,.T.);
#12284=FACE_OUTER_BOUND('',#16827,.T.);
#12285=FACE_OUTER_BOUND('',#16828,.T.);
#12286=FACE_OUTER_BOUND('',#16830,.T.);
#12287=FACE_OUTER_BOUND('',#16831,.T.);
#12288=FACE_OUTER_BOUND('',#16833,.T.);
#12289=FACE_OUTER_BOUND('',#16834,.T.);
#12290=FACE_OUTER_BOUND('',#16836,.T.);
#12291=FACE_OUTER_BOUND('',#16837,.T.);
#12292=FACE_OUTER_BOUND('',#16839,.T.);
#12293=FACE_OUTER_BOUND('',#16840,.T.);
#12294=FACE_OUTER_BOUND('',#16842,.T.);
#12295=FACE_OUTER_BOUND('',#16843,.T.);
#12296=FACE_OUTER_BOUND('',#16845,.T.);
#12297=FACE_OUTER_BOUND('',#16846,.T.);
#12298=FACE_OUTER_BOUND('',#16848,.T.);
#12299=FACE_OUTER_BOUND('',#16849,.T.);
#12300=FACE_OUTER_BOUND('',#16851,.T.);
#12301=FACE_OUTER_BOUND('',#16852,.T.);
#12302=FACE_OUTER_BOUND('',#16854,.T.);
#12303=FACE_OUTER_BOUND('',#16855,.T.);
#12304=FACE_OUTER_BOUND('',#16857,.T.);
#12305=FACE_OUTER_BOUND('',#16858,.T.);
#12306=FACE_OUTER_BOUND('',#16860,.T.);
#12307=FACE_OUTER_BOUND('',#16861,.T.);
#12308=FACE_OUTER_BOUND('',#16863,.T.);
#12309=FACE_OUTER_BOUND('',#16864,.T.);
#12310=FACE_OUTER_BOUND('',#16866,.T.);
#12311=FACE_OUTER_BOUND('',#16867,.T.);
#12312=FACE_OUTER_BOUND('',#16869,.T.);
#12313=FACE_OUTER_BOUND('',#16870,.T.);
#12314=FACE_OUTER_BOUND('',#16872,.T.);
#12315=FACE_OUTER_BOUND('',#16873,.T.);
#12316=FACE_OUTER_BOUND('',#16875,.T.);
#12317=FACE_OUTER_BOUND('',#16876,.T.);
#12318=FACE_OUTER_BOUND('',#16878,.T.);
#12319=FACE_OUTER_BOUND('',#16879,.T.);
#12320=FACE_OUTER_BOUND('',#16881,.T.);
#12321=FACE_OUTER_BOUND('',#16882,.T.);
#12322=FACE_OUTER_BOUND('',#16884,.T.);
#12323=FACE_OUTER_BOUND('',#16885,.T.);
#12324=FACE_OUTER_BOUND('',#16887,.T.);
#12325=FACE_OUTER_BOUND('',#16888,.T.);
#12326=FACE_OUTER_BOUND('',#16890,.T.);
#12327=FACE_OUTER_BOUND('',#16891,.T.);
#12328=FACE_OUTER_BOUND('',#16893,.T.);
#12329=FACE_OUTER_BOUND('',#16894,.T.);
#12330=FACE_OUTER_BOUND('',#16896,.T.);
#12331=FACE_OUTER_BOUND('',#16897,.T.);
#12332=FACE_OUTER_BOUND('',#16899,.T.);
#12333=FACE_OUTER_BOUND('',#16900,.T.);
#12334=FACE_OUTER_BOUND('',#16902,.T.);
#12335=FACE_OUTER_BOUND('',#16903,.T.);
#12336=FACE_OUTER_BOUND('',#16905,.T.);
#12337=FACE_OUTER_BOUND('',#16906,.T.);
#12338=FACE_OUTER_BOUND('',#16908,.T.);
#12339=FACE_OUTER_BOUND('',#16909,.T.);
#12340=FACE_OUTER_BOUND('',#16911,.T.);
#12341=FACE_OUTER_BOUND('',#16912,.T.);
#12342=FACE_OUTER_BOUND('',#16914,.T.);
#12343=FACE_OUTER_BOUND('',#16915,.T.);
#12344=FACE_OUTER_BOUND('',#16917,.T.);
#12345=FACE_OUTER_BOUND('',#16918,.T.);
#12346=FACE_OUTER_BOUND('',#16920,.T.);
#12347=FACE_OUTER_BOUND('',#16921,.T.);
#12348=FACE_OUTER_BOUND('',#16923,.T.);
#12349=FACE_OUTER_BOUND('',#16924,.T.);
#12350=FACE_OUTER_BOUND('',#16926,.T.);
#12351=FACE_OUTER_BOUND('',#16927,.T.);
#12352=FACE_OUTER_BOUND('',#16929,.T.);
#12353=FACE_OUTER_BOUND('',#16930,.T.);
#12354=FACE_OUTER_BOUND('',#16932,.T.);
#12355=FACE_OUTER_BOUND('',#16933,.T.);
#12356=FACE_OUTER_BOUND('',#16935,.T.);
#12357=FACE_OUTER_BOUND('',#16936,.T.);
#12358=FACE_OUTER_BOUND('',#16938,.T.);
#12359=FACE_OUTER_BOUND('',#16939,.T.);
#12360=FACE_OUTER_BOUND('',#16941,.T.);
#12361=FACE_OUTER_BOUND('',#16942,.T.);
#12362=FACE_OUTER_BOUND('',#16944,.T.);
#12363=FACE_OUTER_BOUND('',#16945,.T.);
#12364=FACE_OUTER_BOUND('',#16947,.T.);
#12365=FACE_OUTER_BOUND('',#16948,.T.);
#12366=FACE_OUTER_BOUND('',#16950,.T.);
#12367=FACE_OUTER_BOUND('',#16951,.T.);
#12368=FACE_OUTER_BOUND('',#16953,.T.);
#12369=FACE_OUTER_BOUND('',#16954,.T.);
#12370=FACE_OUTER_BOUND('',#16956,.T.);
#12371=FACE_OUTER_BOUND('',#16957,.T.);
#12372=FACE_OUTER_BOUND('',#16959,.T.);
#12373=FACE_OUTER_BOUND('',#16960,.T.);
#12374=FACE_OUTER_BOUND('',#16962,.T.);
#12375=FACE_OUTER_BOUND('',#16963,.T.);
#12376=FACE_OUTER_BOUND('',#16965,.T.);
#12377=FACE_OUTER_BOUND('',#16966,.T.);
#12378=FACE_OUTER_BOUND('',#16968,.T.);
#12379=FACE_OUTER_BOUND('',#16969,.T.);
#12380=FACE_OUTER_BOUND('',#16971,.T.);
#12381=FACE_OUTER_BOUND('',#16972,.T.);
#12382=FACE_OUTER_BOUND('',#16974,.T.);
#12383=FACE_OUTER_BOUND('',#16975,.T.);
#12384=FACE_OUTER_BOUND('',#16977,.T.);
#12385=FACE_OUTER_BOUND('',#16978,.T.);
#12386=FACE_OUTER_BOUND('',#16980,.T.);
#12387=FACE_OUTER_BOUND('',#16981,.T.);
#12388=FACE_OUTER_BOUND('',#16983,.T.);
#12389=FACE_OUTER_BOUND('',#16984,.T.);
#12390=FACE_OUTER_BOUND('',#16986,.T.);
#12391=FACE_OUTER_BOUND('',#16987,.T.);
#12392=FACE_OUTER_BOUND('',#16989,.T.);
#12393=FACE_OUTER_BOUND('',#16990,.T.);
#12394=FACE_OUTER_BOUND('',#16992,.T.);
#12395=FACE_OUTER_BOUND('',#16993,.T.);
#12396=FACE_OUTER_BOUND('',#16995,.T.);
#12397=FACE_OUTER_BOUND('',#16996,.T.);
#12398=FACE_OUTER_BOUND('',#16998,.T.);
#12399=FACE_OUTER_BOUND('',#16999,.T.);
#12400=FACE_OUTER_BOUND('',#17001,.T.);
#12401=FACE_OUTER_BOUND('',#17002,.T.);
#12402=FACE_OUTER_BOUND('',#17004,.T.);
#12403=FACE_OUTER_BOUND('',#17005,.T.);
#12404=FACE_OUTER_BOUND('',#17007,.T.);
#12405=FACE_OUTER_BOUND('',#17008,.T.);
#12406=FACE_OUTER_BOUND('',#17010,.T.);
#12407=FACE_OUTER_BOUND('',#17011,.T.);
#12408=FACE_OUTER_BOUND('',#17013,.T.);
#12409=FACE_OUTER_BOUND('',#17014,.T.);
#12410=FACE_OUTER_BOUND('',#17016,.T.);
#12411=FACE_OUTER_BOUND('',#17017,.T.);
#12412=FACE_OUTER_BOUND('',#17019,.T.);
#12413=FACE_OUTER_BOUND('',#17020,.T.);
#12414=FACE_OUTER_BOUND('',#17022,.T.);
#12415=FACE_OUTER_BOUND('',#17023,.T.);
#12416=FACE_OUTER_BOUND('',#17025,.T.);
#12417=FACE_OUTER_BOUND('',#17026,.T.);
#12418=FACE_OUTER_BOUND('',#17028,.T.);
#12419=FACE_OUTER_BOUND('',#17029,.T.);
#12420=FACE_OUTER_BOUND('',#17031,.T.);
#12421=FACE_OUTER_BOUND('',#17032,.T.);
#12422=FACE_OUTER_BOUND('',#17034,.T.);
#12423=FACE_OUTER_BOUND('',#17035,.T.);
#12424=FACE_OUTER_BOUND('',#17037,.T.);
#12425=FACE_OUTER_BOUND('',#17038,.T.);
#12426=FACE_OUTER_BOUND('',#17040,.T.);
#12427=FACE_OUTER_BOUND('',#17041,.T.);
#12428=FACE_OUTER_BOUND('',#17043,.T.);
#12429=FACE_OUTER_BOUND('',#17044,.T.);
#12430=FACE_OUTER_BOUND('',#17046,.T.);
#12431=FACE_OUTER_BOUND('',#17047,.T.);
#12432=FACE_OUTER_BOUND('',#17049,.T.);
#12433=FACE_OUTER_BOUND('',#17050,.T.);
#12434=FACE_OUTER_BOUND('',#17052,.T.);
#12435=FACE_OUTER_BOUND('',#17053,.T.);
#12436=FACE_OUTER_BOUND('',#17055,.T.);
#12437=FACE_OUTER_BOUND('',#17056,.T.);
#12438=FACE_OUTER_BOUND('',#17058,.T.);
#12439=FACE_OUTER_BOUND('',#17059,.T.);
#12440=FACE_OUTER_BOUND('',#17061,.T.);
#12441=FACE_OUTER_BOUND('',#17062,.T.);
#12442=FACE_OUTER_BOUND('',#17064,.T.);
#12443=FACE_OUTER_BOUND('',#17065,.T.);
#12444=FACE_OUTER_BOUND('',#17067,.T.);
#12445=FACE_OUTER_BOUND('',#17068,.T.);
#12446=FACE_OUTER_BOUND('',#17070,.T.);
#12447=FACE_OUTER_BOUND('',#17071,.T.);
#12448=FACE_OUTER_BOUND('',#17073,.T.);
#12449=FACE_OUTER_BOUND('',#17074,.T.);
#12450=FACE_OUTER_BOUND('',#17076,.T.);
#12451=FACE_OUTER_BOUND('',#17077,.T.);
#12452=FACE_OUTER_BOUND('',#17079,.T.);
#12453=FACE_OUTER_BOUND('',#17080,.T.);
#12454=FACE_OUTER_BOUND('',#17082,.T.);
#12455=FACE_OUTER_BOUND('',#17083,.T.);
#12456=FACE_OUTER_BOUND('',#17085,.T.);
#12457=FACE_OUTER_BOUND('',#17086,.T.);
#12458=FACE_OUTER_BOUND('',#17088,.T.);
#12459=FACE_OUTER_BOUND('',#17089,.T.);
#12460=FACE_OUTER_BOUND('',#17091,.T.);
#12461=FACE_OUTER_BOUND('',#17092,.T.);
#12462=FACE_OUTER_BOUND('',#17094,.T.);
#12463=FACE_OUTER_BOUND('',#17095,.T.);
#12464=FACE_OUTER_BOUND('',#17097,.T.);
#12465=FACE_OUTER_BOUND('',#17098,.T.);
#12466=FACE_OUTER_BOUND('',#17100,.T.);
#12467=FACE_OUTER_BOUND('',#17101,.T.);
#12468=FACE_OUTER_BOUND('',#17103,.T.);
#12469=FACE_OUTER_BOUND('',#17104,.T.);
#12470=FACE_OUTER_BOUND('',#17106,.T.);
#12471=FACE_OUTER_BOUND('',#17107,.T.);
#12472=FACE_OUTER_BOUND('',#17109,.T.);
#12473=FACE_OUTER_BOUND('',#17110,.T.);
#12474=FACE_OUTER_BOUND('',#17112,.T.);
#12475=FACE_OUTER_BOUND('',#17113,.T.);
#12476=FACE_OUTER_BOUND('',#17115,.T.);
#12477=FACE_OUTER_BOUND('',#17116,.T.);
#12478=FACE_OUTER_BOUND('',#17118,.T.);
#12479=FACE_OUTER_BOUND('',#17119,.T.);
#12480=FACE_OUTER_BOUND('',#17121,.T.);
#12481=FACE_OUTER_BOUND('',#17122,.T.);
#12482=FACE_OUTER_BOUND('',#17124,.T.);
#12483=FACE_OUTER_BOUND('',#17125,.T.);
#12484=FACE_OUTER_BOUND('',#17127,.T.);
#12485=FACE_OUTER_BOUND('',#17128,.T.);
#12486=FACE_OUTER_BOUND('',#17130,.T.);
#12487=FACE_OUTER_BOUND('',#17131,.T.);
#12488=FACE_OUTER_BOUND('',#17133,.T.);
#12489=FACE_OUTER_BOUND('',#17134,.T.);
#12490=FACE_OUTER_BOUND('',#17136,.T.);
#12491=FACE_OUTER_BOUND('',#17137,.T.);
#12492=FACE_OUTER_BOUND('',#17139,.T.);
#12493=FACE_OUTER_BOUND('',#17140,.T.);
#12494=FACE_OUTER_BOUND('',#17142,.T.);
#12495=FACE_OUTER_BOUND('',#17143,.T.);
#12496=FACE_OUTER_BOUND('',#17145,.T.);
#12497=FACE_OUTER_BOUND('',#17146,.T.);
#12498=FACE_OUTER_BOUND('',#17148,.T.);
#12499=FACE_OUTER_BOUND('',#17149,.T.);
#12500=FACE_OUTER_BOUND('',#17151,.T.);
#12501=FACE_OUTER_BOUND('',#17152,.T.);
#12502=FACE_OUTER_BOUND('',#17154,.T.);
#12503=FACE_OUTER_BOUND('',#17155,.T.);
#12504=FACE_OUTER_BOUND('',#17157,.T.);
#12505=FACE_OUTER_BOUND('',#17158,.T.);
#12506=FACE_OUTER_BOUND('',#17160,.T.);
#12507=FACE_OUTER_BOUND('',#17161,.T.);
#12508=FACE_OUTER_BOUND('',#17163,.T.);
#12509=FACE_OUTER_BOUND('',#17164,.T.);
#12510=FACE_OUTER_BOUND('',#17166,.T.);
#12511=FACE_OUTER_BOUND('',#17167,.T.);
#12512=FACE_OUTER_BOUND('',#17169,.T.);
#12513=FACE_OUTER_BOUND('',#17170,.T.);
#12514=FACE_OUTER_BOUND('',#17172,.T.);
#12515=FACE_OUTER_BOUND('',#17173,.T.);
#12516=FACE_OUTER_BOUND('',#17175,.T.);
#12517=FACE_OUTER_BOUND('',#17176,.T.);
#12518=FACE_OUTER_BOUND('',#17178,.T.);
#12519=FACE_OUTER_BOUND('',#17179,.T.);
#12520=FACE_OUTER_BOUND('',#17181,.T.);
#12521=FACE_OUTER_BOUND('',#17182,.T.);
#12522=FACE_OUTER_BOUND('',#17184,.T.);
#12523=FACE_OUTER_BOUND('',#17185,.T.);
#12524=FACE_OUTER_BOUND('',#17187,.T.);
#12525=FACE_OUTER_BOUND('',#17188,.T.);
#12526=FACE_OUTER_BOUND('',#17190,.T.);
#12527=FACE_OUTER_BOUND('',#17191,.T.);
#12528=FACE_OUTER_BOUND('',#17193,.T.);
#12529=FACE_OUTER_BOUND('',#17194,.T.);
#12530=FACE_OUTER_BOUND('',#17196,.T.);
#12531=FACE_OUTER_BOUND('',#17197,.T.);
#12532=FACE_OUTER_BOUND('',#17199,.T.);
#12533=FACE_OUTER_BOUND('',#17200,.T.);
#12534=FACE_OUTER_BOUND('',#17202,.T.);
#12535=FACE_OUTER_BOUND('',#17203,.T.);
#12536=FACE_OUTER_BOUND('',#17205,.T.);
#12537=FACE_OUTER_BOUND('',#17206,.T.);
#12538=FACE_OUTER_BOUND('',#17208,.T.);
#12539=FACE_OUTER_BOUND('',#17209,.T.);
#12540=FACE_OUTER_BOUND('',#17211,.T.);
#12541=FACE_OUTER_BOUND('',#17212,.T.);
#12542=FACE_OUTER_BOUND('',#17214,.T.);
#12543=FACE_OUTER_BOUND('',#17215,.T.);
#12544=FACE_OUTER_BOUND('',#17217,.T.);
#12545=FACE_OUTER_BOUND('',#17218,.T.);
#12546=FACE_OUTER_BOUND('',#17220,.T.);
#12547=FACE_OUTER_BOUND('',#17221,.T.);
#12548=FACE_OUTER_BOUND('',#17223,.T.);
#12549=FACE_OUTER_BOUND('',#17224,.T.);
#12550=FACE_OUTER_BOUND('',#17226,.T.);
#12551=FACE_OUTER_BOUND('',#17227,.T.);
#12552=FACE_OUTER_BOUND('',#17229,.T.);
#12553=FACE_OUTER_BOUND('',#17230,.T.);
#12554=FACE_OUTER_BOUND('',#17232,.T.);
#12555=FACE_OUTER_BOUND('',#17233,.T.);
#12556=FACE_OUTER_BOUND('',#17235,.T.);
#12557=FACE_OUTER_BOUND('',#17236,.T.);
#12558=FACE_OUTER_BOUND('',#17238,.T.);
#12559=FACE_OUTER_BOUND('',#17239,.T.);
#12560=FACE_OUTER_BOUND('',#17241,.T.);
#12561=FACE_OUTER_BOUND('',#17242,.T.);
#12562=FACE_OUTER_BOUND('',#17244,.T.);
#12563=FACE_OUTER_BOUND('',#17245,.T.);
#12564=FACE_OUTER_BOUND('',#17247,.T.);
#12565=FACE_OUTER_BOUND('',#17248,.T.);
#12566=FACE_OUTER_BOUND('',#17250,.T.);
#12567=FACE_OUTER_BOUND('',#17251,.T.);
#12568=FACE_OUTER_BOUND('',#17253,.T.);
#12569=FACE_OUTER_BOUND('',#17254,.T.);
#12570=FACE_OUTER_BOUND('',#17256,.T.);
#12571=FACE_OUTER_BOUND('',#17257,.T.);
#12572=FACE_OUTER_BOUND('',#17259,.T.);
#12573=FACE_OUTER_BOUND('',#17260,.T.);
#12574=FACE_OUTER_BOUND('',#17262,.T.);
#12575=FACE_OUTER_BOUND('',#17263,.T.);
#12576=FACE_OUTER_BOUND('',#17265,.T.);
#12577=FACE_OUTER_BOUND('',#17266,.T.);
#12578=FACE_OUTER_BOUND('',#17268,.T.);
#12579=FACE_OUTER_BOUND('',#17269,.T.);
#12580=FACE_OUTER_BOUND('',#17271,.T.);
#12581=FACE_OUTER_BOUND('',#17272,.T.);
#12582=FACE_OUTER_BOUND('',#17274,.T.);
#12583=FACE_OUTER_BOUND('',#17275,.T.);
#12584=FACE_OUTER_BOUND('',#17277,.T.);
#12585=FACE_OUTER_BOUND('',#17278,.T.);
#12586=FACE_OUTER_BOUND('',#17280,.T.);
#12587=FACE_OUTER_BOUND('',#17281,.T.);
#12588=FACE_OUTER_BOUND('',#17283,.T.);
#12589=FACE_OUTER_BOUND('',#17284,.T.);
#12590=FACE_OUTER_BOUND('',#17286,.T.);
#12591=FACE_OUTER_BOUND('',#17287,.T.);
#12592=FACE_OUTER_BOUND('',#17289,.T.);
#12593=FACE_OUTER_BOUND('',#17290,.T.);
#12594=FACE_OUTER_BOUND('',#17292,.T.);
#12595=FACE_OUTER_BOUND('',#17293,.T.);
#12596=FACE_OUTER_BOUND('',#17295,.T.);
#12597=FACE_OUTER_BOUND('',#17296,.T.);
#12598=FACE_OUTER_BOUND('',#17298,.T.);
#12599=FACE_OUTER_BOUND('',#17299,.T.);
#12600=FACE_OUTER_BOUND('',#17301,.T.);
#12601=FACE_OUTER_BOUND('',#17302,.T.);
#12602=FACE_OUTER_BOUND('',#17304,.T.);
#12603=FACE_OUTER_BOUND('',#17305,.T.);
#12604=FACE_OUTER_BOUND('',#17307,.T.);
#12605=FACE_OUTER_BOUND('',#17308,.T.);
#12606=FACE_OUTER_BOUND('',#17310,.T.);
#12607=FACE_OUTER_BOUND('',#17311,.T.);
#12608=FACE_OUTER_BOUND('',#17313,.T.);
#12609=FACE_OUTER_BOUND('',#17314,.T.);
#12610=FACE_OUTER_BOUND('',#17316,.T.);
#12611=FACE_OUTER_BOUND('',#17317,.T.);
#12612=FACE_OUTER_BOUND('',#17319,.T.);
#12613=FACE_OUTER_BOUND('',#17320,.T.);
#12614=FACE_OUTER_BOUND('',#17322,.T.);
#12615=FACE_OUTER_BOUND('',#17323,.T.);
#12616=FACE_OUTER_BOUND('',#17325,.T.);
#12617=FACE_OUTER_BOUND('',#17326,.T.);
#12618=FACE_OUTER_BOUND('',#17328,.T.);
#12619=FACE_OUTER_BOUND('',#17329,.T.);
#12620=FACE_OUTER_BOUND('',#17331,.T.);
#12621=FACE_OUTER_BOUND('',#17332,.T.);
#12622=FACE_OUTER_BOUND('',#17334,.T.);
#12623=FACE_OUTER_BOUND('',#17335,.T.);
#12624=FACE_OUTER_BOUND('',#17337,.T.);
#12625=FACE_OUTER_BOUND('',#17338,.T.);
#12626=FACE_OUTER_BOUND('',#17340,.T.);
#12627=FACE_OUTER_BOUND('',#17341,.T.);
#12628=FACE_OUTER_BOUND('',#17343,.T.);
#12629=FACE_OUTER_BOUND('',#17344,.T.);
#12630=FACE_OUTER_BOUND('',#17346,.T.);
#12631=FACE_OUTER_BOUND('',#17347,.T.);
#12632=FACE_OUTER_BOUND('',#17349,.T.);
#12633=FACE_OUTER_BOUND('',#17350,.T.);
#12634=FACE_OUTER_BOUND('',#17352,.T.);
#12635=FACE_OUTER_BOUND('',#17353,.T.);
#12636=FACE_OUTER_BOUND('',#17355,.T.);
#12637=FACE_OUTER_BOUND('',#17356,.T.);
#12638=FACE_OUTER_BOUND('',#17358,.T.);
#12639=FACE_OUTER_BOUND('',#17359,.T.);
#12640=FACE_OUTER_BOUND('',#17361,.T.);
#12641=FACE_OUTER_BOUND('',#17362,.T.);
#12642=FACE_OUTER_BOUND('',#17364,.T.);
#12643=FACE_OUTER_BOUND('',#17365,.T.);
#12644=FACE_OUTER_BOUND('',#17367,.T.);
#12645=FACE_OUTER_BOUND('',#17368,.T.);
#12646=FACE_OUTER_BOUND('',#17370,.T.);
#12647=FACE_OUTER_BOUND('',#17371,.T.);
#12648=FACE_OUTER_BOUND('',#17373,.T.);
#12649=FACE_OUTER_BOUND('',#17374,.T.);
#12650=FACE_OUTER_BOUND('',#17376,.T.);
#12651=FACE_OUTER_BOUND('',#17377,.T.);
#12652=FACE_OUTER_BOUND('',#17379,.T.);
#12653=FACE_OUTER_BOUND('',#17380,.T.);
#12654=FACE_OUTER_BOUND('',#17382,.T.);
#12655=FACE_OUTER_BOUND('',#17383,.T.);
#12656=FACE_OUTER_BOUND('',#17385,.T.);
#12657=FACE_OUTER_BOUND('',#17386,.T.);
#12658=FACE_OUTER_BOUND('',#17388,.T.);
#12659=FACE_OUTER_BOUND('',#17389,.T.);
#12660=FACE_OUTER_BOUND('',#17391,.T.);
#12661=FACE_OUTER_BOUND('',#17392,.T.);
#12662=FACE_OUTER_BOUND('',#17394,.T.);
#12663=FACE_OUTER_BOUND('',#17395,.T.);
#12664=FACE_OUTER_BOUND('',#17397,.T.);
#12665=FACE_OUTER_BOUND('',#17398,.T.);
#12666=FACE_OUTER_BOUND('',#17400,.T.);
#12667=FACE_OUTER_BOUND('',#17401,.T.);
#12668=FACE_OUTER_BOUND('',#17403,.T.);
#12669=FACE_OUTER_BOUND('',#17404,.T.);
#12670=FACE_OUTER_BOUND('',#17406,.T.);
#12671=FACE_OUTER_BOUND('',#17407,.T.);
#12672=FACE_OUTER_BOUND('',#17409,.T.);
#12673=FACE_OUTER_BOUND('',#17410,.T.);
#12674=FACE_OUTER_BOUND('',#17412,.T.);
#12675=FACE_OUTER_BOUND('',#17413,.T.);
#12676=FACE_OUTER_BOUND('',#17415,.T.);
#12677=FACE_OUTER_BOUND('',#17416,.T.);
#12678=FACE_OUTER_BOUND('',#17418,.T.);
#12679=FACE_OUTER_BOUND('',#17419,.T.);
#12680=FACE_OUTER_BOUND('',#17421,.T.);
#12681=FACE_OUTER_BOUND('',#17422,.T.);
#12682=FACE_OUTER_BOUND('',#17424,.T.);
#12683=FACE_OUTER_BOUND('',#17425,.T.);
#12684=FACE_OUTER_BOUND('',#17427,.T.);
#12685=FACE_OUTER_BOUND('',#17428,.T.);
#12686=FACE_OUTER_BOUND('',#17430,.T.);
#12687=FACE_OUTER_BOUND('',#17431,.T.);
#12688=FACE_OUTER_BOUND('',#17433,.T.);
#12689=FACE_OUTER_BOUND('',#17434,.T.);
#12690=FACE_OUTER_BOUND('',#17436,.T.);
#12691=FACE_OUTER_BOUND('',#17437,.T.);
#12692=FACE_OUTER_BOUND('',#17439,.T.);
#12693=FACE_OUTER_BOUND('',#17440,.T.);
#12694=FACE_OUTER_BOUND('',#17442,.T.);
#12695=FACE_OUTER_BOUND('',#17443,.T.);
#12696=FACE_OUTER_BOUND('',#17445,.T.);
#12697=FACE_OUTER_BOUND('',#17446,.T.);
#12698=FACE_OUTER_BOUND('',#17448,.T.);
#12699=FACE_OUTER_BOUND('',#17449,.T.);
#12700=FACE_OUTER_BOUND('',#17451,.T.);
#12701=FACE_OUTER_BOUND('',#17452,.T.);
#12702=FACE_OUTER_BOUND('',#17454,.T.);
#12703=FACE_OUTER_BOUND('',#17455,.T.);
#12704=FACE_OUTER_BOUND('',#17457,.T.);
#12705=FACE_OUTER_BOUND('',#17458,.T.);
#12706=FACE_OUTER_BOUND('',#17460,.T.);
#12707=FACE_OUTER_BOUND('',#17461,.T.);
#12708=FACE_OUTER_BOUND('',#17463,.T.);
#12709=FACE_OUTER_BOUND('',#17464,.T.);
#12710=FACE_OUTER_BOUND('',#17466,.T.);
#12711=FACE_OUTER_BOUND('',#17467,.T.);
#12712=FACE_OUTER_BOUND('',#17469,.T.);
#12713=FACE_OUTER_BOUND('',#17470,.T.);
#12714=FACE_OUTER_BOUND('',#17472,.T.);
#12715=FACE_OUTER_BOUND('',#17473,.T.);
#12716=FACE_OUTER_BOUND('',#17475,.T.);
#12717=FACE_OUTER_BOUND('',#17476,.T.);
#12718=FACE_OUTER_BOUND('',#17478,.T.);
#12719=FACE_OUTER_BOUND('',#17479,.T.);
#12720=FACE_OUTER_BOUND('',#17481,.T.);
#12721=FACE_OUTER_BOUND('',#17482,.T.);
#12722=FACE_OUTER_BOUND('',#17484,.T.);
#12723=FACE_OUTER_BOUND('',#17485,.T.);
#12724=FACE_OUTER_BOUND('',#17487,.T.);
#12725=FACE_OUTER_BOUND('',#17488,.T.);
#12726=FACE_OUTER_BOUND('',#17490,.T.);
#12727=FACE_OUTER_BOUND('',#17491,.T.);
#12728=FACE_OUTER_BOUND('',#17493,.T.);
#12729=FACE_OUTER_BOUND('',#17494,.T.);
#12730=FACE_OUTER_BOUND('',#17496,.T.);
#12731=FACE_OUTER_BOUND('',#17497,.T.);
#12732=FACE_OUTER_BOUND('',#17499,.T.);
#12733=FACE_OUTER_BOUND('',#17500,.T.);
#12734=FACE_OUTER_BOUND('',#17502,.T.);
#12735=FACE_OUTER_BOUND('',#17503,.T.);
#12736=FACE_OUTER_BOUND('',#17505,.T.);
#12737=FACE_OUTER_BOUND('',#17506,.T.);
#12738=FACE_OUTER_BOUND('',#17508,.T.);
#12739=FACE_OUTER_BOUND('',#17509,.T.);
#12740=FACE_OUTER_BOUND('',#17511,.T.);
#12741=FACE_OUTER_BOUND('',#17512,.T.);
#12742=FACE_OUTER_BOUND('',#17514,.T.);
#12743=FACE_OUTER_BOUND('',#17515,.T.);
#12744=FACE_OUTER_BOUND('',#17517,.T.);
#12745=FACE_OUTER_BOUND('',#17518,.T.);
#12746=FACE_OUTER_BOUND('',#17520,.T.);
#12747=FACE_OUTER_BOUND('',#17521,.T.);
#12748=FACE_OUTER_BOUND('',#17523,.T.);
#12749=FACE_OUTER_BOUND('',#17524,.T.);
#12750=FACE_OUTER_BOUND('',#17526,.T.);
#12751=FACE_OUTER_BOUND('',#17527,.T.);
#12752=FACE_OUTER_BOUND('',#17529,.T.);
#12753=FACE_OUTER_BOUND('',#17530,.T.);
#12754=FACE_OUTER_BOUND('',#17532,.T.);
#12755=FACE_OUTER_BOUND('',#17533,.T.);
#12756=FACE_OUTER_BOUND('',#17535,.T.);
#12757=FACE_OUTER_BOUND('',#17536,.T.);
#12758=FACE_OUTER_BOUND('',#17538,.T.);
#12759=FACE_OUTER_BOUND('',#17539,.T.);
#12760=FACE_OUTER_BOUND('',#17541,.T.);
#12761=FACE_OUTER_BOUND('',#17542,.T.);
#12762=FACE_OUTER_BOUND('',#17544,.T.);
#12763=FACE_OUTER_BOUND('',#17545,.T.);
#12764=FACE_OUTER_BOUND('',#17547,.T.);
#12765=FACE_OUTER_BOUND('',#17548,.T.);
#12766=FACE_OUTER_BOUND('',#17550,.T.);
#12767=FACE_OUTER_BOUND('',#17551,.T.);
#12768=FACE_OUTER_BOUND('',#17553,.T.);
#12769=FACE_OUTER_BOUND('',#17554,.T.);
#12770=FACE_OUTER_BOUND('',#17556,.T.);
#12771=FACE_OUTER_BOUND('',#17557,.T.);
#12772=FACE_OUTER_BOUND('',#17559,.T.);
#12773=FACE_OUTER_BOUND('',#17560,.T.);
#12774=FACE_OUTER_BOUND('',#17562,.T.);
#12775=FACE_OUTER_BOUND('',#17563,.T.);
#12776=FACE_OUTER_BOUND('',#17565,.T.);
#12777=FACE_OUTER_BOUND('',#17566,.T.);
#12778=FACE_OUTER_BOUND('',#17568,.T.);
#12779=FACE_OUTER_BOUND('',#17569,.T.);
#12780=FACE_OUTER_BOUND('',#17571,.T.);
#12781=FACE_OUTER_BOUND('',#17572,.T.);
#12782=FACE_OUTER_BOUND('',#17574,.T.);
#12783=FACE_OUTER_BOUND('',#17575,.T.);
#12784=FACE_OUTER_BOUND('',#17577,.T.);
#12785=FACE_OUTER_BOUND('',#17578,.T.);
#12786=FACE_OUTER_BOUND('',#17580,.T.);
#12787=FACE_OUTER_BOUND('',#17581,.T.);
#12788=FACE_OUTER_BOUND('',#17583,.T.);
#12789=FACE_OUTER_BOUND('',#17584,.T.);
#12790=FACE_OUTER_BOUND('',#17586,.T.);
#12791=FACE_OUTER_BOUND('',#17587,.T.);
#12792=FACE_OUTER_BOUND('',#17589,.T.);
#12793=FACE_OUTER_BOUND('',#17590,.T.);
#12794=FACE_OUTER_BOUND('',#17592,.T.);
#12795=FACE_OUTER_BOUND('',#17593,.T.);
#12796=FACE_OUTER_BOUND('',#17595,.T.);
#12797=FACE_OUTER_BOUND('',#17596,.T.);
#12798=FACE_OUTER_BOUND('',#17598,.T.);
#12799=FACE_OUTER_BOUND('',#17599,.T.);
#12800=FACE_OUTER_BOUND('',#17601,.T.);
#12801=FACE_OUTER_BOUND('',#17602,.T.);
#12802=FACE_OUTER_BOUND('',#17604,.T.);
#12803=FACE_OUTER_BOUND('',#17605,.T.);
#12804=FACE_OUTER_BOUND('',#17607,.T.);
#12805=FACE_OUTER_BOUND('',#17608,.T.);
#12806=FACE_OUTER_BOUND('',#17610,.T.);
#12807=FACE_OUTER_BOUND('',#17611,.T.);
#12808=FACE_OUTER_BOUND('',#17613,.T.);
#12809=FACE_OUTER_BOUND('',#17614,.T.);
#12810=FACE_OUTER_BOUND('',#17616,.T.);
#12811=FACE_OUTER_BOUND('',#17617,.T.);
#12812=FACE_OUTER_BOUND('',#17619,.T.);
#12813=FACE_OUTER_BOUND('',#17620,.T.);
#12814=FACE_OUTER_BOUND('',#17622,.T.);
#12815=FACE_OUTER_BOUND('',#17623,.T.);
#12816=FACE_OUTER_BOUND('',#17625,.T.);
#12817=FACE_OUTER_BOUND('',#17626,.T.);
#12818=FACE_OUTER_BOUND('',#17628,.T.);
#12819=FACE_OUTER_BOUND('',#17629,.T.);
#12820=FACE_OUTER_BOUND('',#17631,.T.);
#12821=FACE_OUTER_BOUND('',#17632,.T.);
#12822=FACE_OUTER_BOUND('',#17634,.T.);
#12823=FACE_OUTER_BOUND('',#17635,.T.);
#12824=FACE_OUTER_BOUND('',#17637,.T.);
#12825=FACE_OUTER_BOUND('',#17638,.T.);
#12826=FACE_OUTER_BOUND('',#17640,.T.);
#12827=FACE_OUTER_BOUND('',#17641,.T.);
#12828=FACE_OUTER_BOUND('',#17643,.T.);
#12829=FACE_OUTER_BOUND('',#17644,.T.);
#12830=FACE_OUTER_BOUND('',#17646,.T.);
#12831=FACE_OUTER_BOUND('',#17647,.T.);
#12832=FACE_OUTER_BOUND('',#17649,.T.);
#12833=FACE_OUTER_BOUND('',#17650,.T.);
#12834=FACE_OUTER_BOUND('',#17652,.T.);
#12835=FACE_OUTER_BOUND('',#17653,.T.);
#12836=FACE_OUTER_BOUND('',#17655,.T.);
#12837=FACE_OUTER_BOUND('',#17656,.T.);
#12838=FACE_OUTER_BOUND('',#17658,.T.);
#12839=FACE_OUTER_BOUND('',#17659,.T.);
#12840=FACE_OUTER_BOUND('',#17661,.T.);
#12841=FACE_OUTER_BOUND('',#17662,.T.);
#12842=FACE_OUTER_BOUND('',#17664,.T.);
#12843=FACE_OUTER_BOUND('',#17665,.T.);
#12844=FACE_OUTER_BOUND('',#17667,.T.);
#12845=FACE_OUTER_BOUND('',#17668,.T.);
#12846=FACE_OUTER_BOUND('',#17670,.T.);
#12847=FACE_OUTER_BOUND('',#17671,.T.);
#12848=FACE_OUTER_BOUND('',#17673,.T.);
#12849=FACE_OUTER_BOUND('',#17674,.T.);
#12850=FACE_OUTER_BOUND('',#17676,.T.);
#12851=FACE_OUTER_BOUND('',#17677,.T.);
#12852=FACE_OUTER_BOUND('',#17679,.T.);
#12853=FACE_OUTER_BOUND('',#17680,.T.);
#12854=FACE_OUTER_BOUND('',#17682,.T.);
#12855=FACE_OUTER_BOUND('',#17683,.T.);
#12856=FACE_OUTER_BOUND('',#17685,.T.);
#12857=FACE_OUTER_BOUND('',#17686,.T.);
#12858=FACE_OUTER_BOUND('',#17688,.T.);
#12859=FACE_OUTER_BOUND('',#17689,.T.);
#12860=FACE_OUTER_BOUND('',#17691,.T.);
#12861=FACE_OUTER_BOUND('',#17692,.T.);
#12862=FACE_OUTER_BOUND('',#17694,.T.);
#12863=FACE_OUTER_BOUND('',#17695,.T.);
#12864=FACE_OUTER_BOUND('',#17697,.T.);
#12865=FACE_OUTER_BOUND('',#17698,.T.);
#12866=FACE_OUTER_BOUND('',#17700,.T.);
#12867=FACE_OUTER_BOUND('',#17701,.T.);
#15337=EDGE_LOOP('',(#36820,#36821,#36822,#36823));
#15338=EDGE_LOOP('',(#36824,#36825));
#15339=EDGE_LOOP('',(#36826,#36827));
#15340=EDGE_LOOP('',(#36828,#36829));
#15341=EDGE_LOOP('',(#36830,#36831));
#15342=EDGE_LOOP('',(#36832,#36833));
#15343=EDGE_LOOP('',(#36834,#36835));
#15344=EDGE_LOOP('',(#36836,#36837));
#15345=EDGE_LOOP('',(#36838,#36839));
#15346=EDGE_LOOP('',(#36840,#36841));
#15347=EDGE_LOOP('',(#36842,#36843));
#15348=EDGE_LOOP('',(#36844,#36845));
#15349=EDGE_LOOP('',(#36846,#36847));
#15350=EDGE_LOOP('',(#36848,#36849));
#15351=EDGE_LOOP('',(#36850,#36851));
#15352=EDGE_LOOP('',(#36852,#36853));
#15353=EDGE_LOOP('',(#36854,#36855));
#15354=EDGE_LOOP('',(#36856,#36857));
#15355=EDGE_LOOP('',(#36858,#36859));
#15356=EDGE_LOOP('',(#36860,#36861));
#15357=EDGE_LOOP('',(#36862,#36863));
#15358=EDGE_LOOP('',(#36864,#36865));
#15359=EDGE_LOOP('',(#36866,#36867));
#15360=EDGE_LOOP('',(#36868,#36869));
#15361=EDGE_LOOP('',(#36870,#36871));
#15362=EDGE_LOOP('',(#36872,#36873));
#15363=EDGE_LOOP('',(#36874,#36875));
#15364=EDGE_LOOP('',(#36876,#36877));
#15365=EDGE_LOOP('',(#36878,#36879));
#15366=EDGE_LOOP('',(#36880,#36881));
#15367=EDGE_LOOP('',(#36882,#36883));
#15368=EDGE_LOOP('',(#36884,#36885));
#15369=EDGE_LOOP('',(#36886,#36887));
#15370=EDGE_LOOP('',(#36888,#36889));
#15371=EDGE_LOOP('',(#36890,#36891));
#15372=EDGE_LOOP('',(#36892,#36893));
#15373=EDGE_LOOP('',(#36894,#36895));
#15374=EDGE_LOOP('',(#36896,#36897));
#15375=EDGE_LOOP('',(#36898,#36899));
#15376=EDGE_LOOP('',(#36900,#36901));
#15377=EDGE_LOOP('',(#36902,#36903));
#15378=EDGE_LOOP('',(#36904,#36905));
#15379=EDGE_LOOP('',(#36906,#36907));
#15380=EDGE_LOOP('',(#36908,#36909));
#15381=EDGE_LOOP('',(#36910,#36911));
#15382=EDGE_LOOP('',(#36912,#36913));
#15383=EDGE_LOOP('',(#36914,#36915));
#15384=EDGE_LOOP('',(#36916,#36917));
#15385=EDGE_LOOP('',(#36918,#36919));
#15386=EDGE_LOOP('',(#36920,#36921));
#15387=EDGE_LOOP('',(#36922,#36923));
#15388=EDGE_LOOP('',(#36924,#36925));
#15389=EDGE_LOOP('',(#36926,#36927));
#15390=EDGE_LOOP('',(#36928,#36929));
#15391=EDGE_LOOP('',(#36930,#36931));
#15392=EDGE_LOOP('',(#36932,#36933));
#15393=EDGE_LOOP('',(#36934,#36935));
#15394=EDGE_LOOP('',(#36936,#36937));
#15395=EDGE_LOOP('',(#36938,#36939));
#15396=EDGE_LOOP('',(#36940,#36941));
#15397=EDGE_LOOP('',(#36942,#36943));
#15398=EDGE_LOOP('',(#36944,#36945,#36946,#36947));
#15399=EDGE_LOOP('',(#36948,#36949,#36950,#36951,#36952));
#15400=EDGE_LOOP('',(#36953,#36954,#36955,#36956,#36957));
#15401=EDGE_LOOP('',(#36958,#36959,#36960,#36961,#36962));
#15402=EDGE_LOOP('',(#36963,#36964,#36965,#36966,#36967));
#15403=EDGE_LOOP('',(#36968,#36969,#36970,#36971,#36972));
#15404=EDGE_LOOP('',(#36973,#36974,#36975,#36976,#36977));
#15405=EDGE_LOOP('',(#36978,#36979,#36980,#36981,#36982));
#15406=EDGE_LOOP('',(#36983,#36984,#36985,#36986,#36987));
#15407=EDGE_LOOP('',(#36988,#36989,#36990,#36991,#36992));
#15408=EDGE_LOOP('',(#36993,#36994,#36995,#36996,#36997));
#15409=EDGE_LOOP('',(#36998,#36999,#37000,#37001,#37002));
#15410=EDGE_LOOP('',(#37003,#37004,#37005,#37006,#37007));
#15411=EDGE_LOOP('',(#37008,#37009,#37010,#37011,#37012));
#15412=EDGE_LOOP('',(#37013,#37014,#37015,#37016,#37017));
#15413=EDGE_LOOP('',(#37018,#37019,#37020,#37021,#37022));
#15414=EDGE_LOOP('',(#37023,#37024,#37025,#37026,#37027));
#15415=EDGE_LOOP('',(#37028,#37029,#37030,#37031,#37032));
#15416=EDGE_LOOP('',(#37033,#37034,#37035,#37036,#37037));
#15417=EDGE_LOOP('',(#37038,#37039,#37040,#37041,#37042));
#15418=EDGE_LOOP('',(#37043,#37044,#37045,#37046,#37047));
#15419=EDGE_LOOP('',(#37048,#37049,#37050,#37051,#37052));
#15420=EDGE_LOOP('',(#37053,#37054,#37055,#37056,#37057));
#15421=EDGE_LOOP('',(#37058,#37059,#37060,#37061,#37062));
#15422=EDGE_LOOP('',(#37063,#37064,#37065,#37066,#37067));
#15423=EDGE_LOOP('',(#37068,#37069,#37070,#37071,#37072));
#15424=EDGE_LOOP('',(#37073,#37074,#37075,#37076,#37077));
#15425=EDGE_LOOP('',(#37078,#37079,#37080,#37081,#37082));
#15426=EDGE_LOOP('',(#37083,#37084,#37085,#37086,#37087));
#15427=EDGE_LOOP('',(#37088,#37089,#37090,#37091,#37092));
#15428=EDGE_LOOP('',(#37093,#37094,#37095,#37096,#37097));
#15429=EDGE_LOOP('',(#37098,#37099,#37100,#37101,#37102));
#15430=EDGE_LOOP('',(#37103,#37104,#37105,#37106,#37107));
#15431=EDGE_LOOP('',(#37108,#37109,#37110,#37111,#37112));
#15432=EDGE_LOOP('',(#37113,#37114,#37115,#37116,#37117));
#15433=EDGE_LOOP('',(#37118,#37119,#37120,#37121,#37122));
#15434=EDGE_LOOP('',(#37123,#37124,#37125,#37126,#37127));
#15435=EDGE_LOOP('',(#37128,#37129,#37130,#37131,#37132));
#15436=EDGE_LOOP('',(#37133,#37134,#37135,#37136,#37137));
#15437=EDGE_LOOP('',(#37138,#37139,#37140,#37141,#37142));
#15438=EDGE_LOOP('',(#37143,#37144,#37145,#37146,#37147));
#15439=EDGE_LOOP('',(#37148,#37149,#37150,#37151,#37152));
#15440=EDGE_LOOP('',(#37153,#37154,#37155,#37156,#37157));
#15441=EDGE_LOOP('',(#37158,#37159,#37160,#37161,#37162));
#15442=EDGE_LOOP('',(#37163,#37164,#37165,#37166,#37167));
#15443=EDGE_LOOP('',(#37168,#37169,#37170,#37171,#37172));
#15444=EDGE_LOOP('',(#37173,#37174,#37175,#37176,#37177));
#15445=EDGE_LOOP('',(#37178,#37179,#37180,#37181,#37182));
#15446=EDGE_LOOP('',(#37183,#37184,#37185,#37186,#37187));
#15447=EDGE_LOOP('',(#37188,#37189,#37190,#37191,#37192));
#15448=EDGE_LOOP('',(#37193,#37194,#37195,#37196,#37197));
#15449=EDGE_LOOP('',(#37198,#37199,#37200,#37201,#37202));
#15450=EDGE_LOOP('',(#37203,#37204,#37205,#37206,#37207));
#15451=EDGE_LOOP('',(#37208,#37209,#37210,#37211,#37212));
#15452=EDGE_LOOP('',(#37213,#37214,#37215,#37216,#37217));
#15453=EDGE_LOOP('',(#37218,#37219,#37220,#37221,#37222,#37223));
#15454=EDGE_LOOP('',(#37224,#37225,#37226,#37227,#37228));
#15455=EDGE_LOOP('',(#37229,#37230,#37231,#37232,#37233));
#15456=EDGE_LOOP('',(#37234,#37235,#37236,#37237,#37238));
#15457=EDGE_LOOP('',(#37239,#37240,#37241,#37242,#37243));
#15458=EDGE_LOOP('',(#37244,#37245,#37246,#37247,#37248));
#15459=EDGE_LOOP('',(#37249,#37250,#37251,#37252,#37253));
#15460=EDGE_LOOP('',(#37254,#37255,#37256,#37257,#37258));
#15461=EDGE_LOOP('',(#37259,#37260,#37261,#37262));
#15462=EDGE_LOOP('',(#37263,#37264,#37265,#37266,#37267));
#15463=EDGE_LOOP('',(#37268,#37269,#37270,#37271));
#15464=EDGE_LOOP('',(#37272,#37273,#37274,#37275,#37276));
#15465=EDGE_LOOP('',(#37277,#37278,#37279,#37280,#37281));
#15466=EDGE_LOOP('',(#37282,#37283,#37284,#37285,#37286));
#15467=EDGE_LOOP('',(#37287,#37288,#37289,#37290,#37291));
#15468=EDGE_LOOP('',(#37292,#37293,#37294,#37295,#37296));
#15469=EDGE_LOOP('',(#37297,#37298,#37299,#37300));
#15470=EDGE_LOOP('',(#37301,#37302,#37303,#37304,#37305));
#15471=EDGE_LOOP('',(#37306,#37307,#37308,#37309));
#15472=EDGE_LOOP('',(#37310,#37311,#37312,#37313,#37314));
#15473=EDGE_LOOP('',(#37315,#37316,#37317,#37318));
#15474=EDGE_LOOP('',(#37319,#37320,#37321,#37322,#37323));
#15475=EDGE_LOOP('',(#37324,#37325,#37326,#37327));
#15476=EDGE_LOOP('',(#37328,#37329,#37330,#37331,#37332));
#15477=EDGE_LOOP('',(#37333,#37334,#37335,#37336));
#15478=EDGE_LOOP('',(#37337,#37338,#37339,#37340,#37341));
#15479=EDGE_LOOP('',(#37342,#37343,#37344,#37345));
#15480=EDGE_LOOP('',(#37346,#37347,#37348,#37349,#37350));
#15481=EDGE_LOOP('',(#37351,#37352,#37353,#37354));
#15482=EDGE_LOOP('',(#37355,#37356,#37357,#37358,#37359));
#15483=EDGE_LOOP('',(#37360,#37361,#37362,#37363));
#15484=EDGE_LOOP('',(#37364,#37365,#37366,#37367,#37368));
#15485=EDGE_LOOP('',(#37369,#37370,#37371,#37372));
#15486=EDGE_LOOP('',(#37373,#37374,#37375,#37376,#37377));
#15487=EDGE_LOOP('',(#37378,#37379,#37380,#37381));
#15488=EDGE_LOOP('',(#37382,#37383,#37384,#37385,#37386));
#15489=EDGE_LOOP('',(#37387,#37388,#37389,#37390));
#15490=EDGE_LOOP('',(#37391,#37392,#37393,#37394,#37395));
#15491=EDGE_LOOP('',(#37396,#37397,#37398,#37399));
#15492=EDGE_LOOP('',(#37400,#37401,#37402,#37403,#37404));
#15493=EDGE_LOOP('',(#37405,#37406,#37407,#37408));
#15494=EDGE_LOOP('',(#37409,#37410,#37411,#37412,#37413));
#15495=EDGE_LOOP('',(#37414,#37415,#37416,#37417));
#15496=EDGE_LOOP('',(#37418,#37419,#37420,#37421,#37422));
#15497=EDGE_LOOP('',(#37423,#37424,#37425,#37426));
#15498=EDGE_LOOP('',(#37427,#37428,#37429,#37430,#37431));
#15499=EDGE_LOOP('',(#37432,#37433,#37434,#37435));
#15500=EDGE_LOOP('',(#37436,#37437,#37438,#37439,#37440));
#15501=EDGE_LOOP('',(#37441,#37442,#37443,#37444));
#15502=EDGE_LOOP('',(#37445,#37446,#37447,#37448,#37449));
#15503=EDGE_LOOP('',(#37450,#37451,#37452,#37453));
#15504=EDGE_LOOP('',(#37454,#37455,#37456,#37457,#37458));
#15505=EDGE_LOOP('',(#37459,#37460,#37461,#37462));
#15506=EDGE_LOOP('',(#37463,#37464,#37465,#37466,#37467));
#15507=EDGE_LOOP('',(#37468,#37469,#37470,#37471));
#15508=EDGE_LOOP('',(#37472,#37473,#37474,#37475,#37476));
#15509=EDGE_LOOP('',(#37477,#37478,#37479,#37480));
#15510=EDGE_LOOP('',(#37481,#37482,#37483,#37484,#37485));
#15511=EDGE_LOOP('',(#37486,#37487,#37488,#37489));
#15512=EDGE_LOOP('',(#37490,#37491,#37492,#37493,#37494));
#15513=EDGE_LOOP('',(#37495,#37496,#37497,#37498));
#15514=EDGE_LOOP('',(#37499,#37500,#37501,#37502,#37503));
#15515=EDGE_LOOP('',(#37504,#37505,#37506,#37507));
#15516=EDGE_LOOP('',(#37508,#37509,#37510,#37511,#37512));
#15517=EDGE_LOOP('',(#37513,#37514,#37515,#37516));
#15518=EDGE_LOOP('',(#37517,#37518,#37519,#37520,#37521));
#15519=EDGE_LOOP('',(#37522,#37523,#37524,#37525));
#15520=EDGE_LOOP('',(#37526,#37527,#37528,#37529,#37530));
#15521=EDGE_LOOP('',(#37531,#37532,#37533,#37534));
#15522=EDGE_LOOP('',(#37535,#37536,#37537,#37538,#37539));
#15523=EDGE_LOOP('',(#37540,#37541,#37542,#37543));
#15524=EDGE_LOOP('',(#37544,#37545,#37546,#37547,#37548));
#15525=EDGE_LOOP('',(#37549,#37550,#37551,#37552,#37553));
#15526=EDGE_LOOP('',(#37554,#37555,#37556,#37557,#37558));
#15527=EDGE_LOOP('',(#37559,#37560,#37561,#37562));
#15528=EDGE_LOOP('',(#37563,#37564,#37565,#37566,#37567));
#15529=EDGE_LOOP('',(#37568,#37569,#37570,#37571));
#15530=EDGE_LOOP('',(#37572,#37573,#37574,#37575,#37576));
#15531=EDGE_LOOP('',(#37577,#37578,#37579,#37580));
#15532=EDGE_LOOP('',(#37581,#37582,#37583,#37584,#37585));
#15533=EDGE_LOOP('',(#37586,#37587,#37588,#37589,#37590));
#15534=EDGE_LOOP('',(#37591,#37592,#37593,#37594,#37595));
#15535=EDGE_LOOP('',(#37596,#37597,#37598,#37599));
#15536=EDGE_LOOP('',(#37600,#37601,#37602,#37603,#37604));
#15537=EDGE_LOOP('',(#37605,#37606,#37607,#37608));
#15538=EDGE_LOOP('',(#37609,#37610,#37611,#37612,#37613));
#15539=EDGE_LOOP('',(#37614,#37615,#37616,#37617));
#15540=EDGE_LOOP('',(#37618,#37619,#37620,#37621,#37622));
#15541=EDGE_LOOP('',(#37623,#37624,#37625,#37626,#37627,#37628));
#15542=EDGE_LOOP('',(#37629,#37630,#37631,#37632,#37633));
#15543=EDGE_LOOP('',(#37634,#37635,#37636,#37637));
#15544=EDGE_LOOP('',(#37638,#37639,#37640,#37641,#37642));
#15545=EDGE_LOOP('',(#37643,#37644,#37645,#37646));
#15546=EDGE_LOOP('',(#37647,#37648,#37649,#37650,#37651));
#15547=EDGE_LOOP('',(#37652,#37653,#37654,#37655));
#15548=EDGE_LOOP('',(#37656,#37657,#37658,#37659,#37660));
#15549=EDGE_LOOP('',(#37661,#37662,#37663,#37664));
#15550=EDGE_LOOP('',(#37665,#37666,#37667,#37668,#37669));
#15551=EDGE_LOOP('',(#37670,#37671,#37672,#37673));
#15552=EDGE_LOOP('',(#37674,#37675,#37676,#37677,#37678));
#15553=EDGE_LOOP('',(#37679,#37680,#37681,#37682));
#15554=EDGE_LOOP('',(#37683,#37684,#37685,#37686,#37687));
#15555=EDGE_LOOP('',(#37688,#37689,#37690,#37691));
#15556=EDGE_LOOP('',(#37692,#37693,#37694,#37695,#37696));
#15557=EDGE_LOOP('',(#37697,#37698,#37699,#37700));
#15558=EDGE_LOOP('',(#37701,#37702,#37703,#37704,#37705));
#15559=EDGE_LOOP('',(#37706,#37707,#37708,#37709));
#15560=EDGE_LOOP('',(#37710,#37711,#37712,#37713,#37714));
#15561=EDGE_LOOP('',(#37715,#37716,#37717,#37718));
#15562=EDGE_LOOP('',(#37719,#37720,#37721,#37722,#37723));
#15563=EDGE_LOOP('',(#37724,#37725,#37726,#37727));
#15564=EDGE_LOOP('',(#37728,#37729,#37730,#37731,#37732));
#15565=EDGE_LOOP('',(#37733,#37734,#37735,#37736));
#15566=EDGE_LOOP('',(#37737,#37738,#37739,#37740,#37741));
#15567=EDGE_LOOP('',(#37742,#37743,#37744,#37745));
#15568=EDGE_LOOP('',(#37746,#37747,#37748,#37749,#37750));
#15569=EDGE_LOOP('',(#37751,#37752,#37753,#37754));
#15570=EDGE_LOOP('',(#37755,#37756,#37757,#37758,#37759));
#15571=EDGE_LOOP('',(#37760,#37761,#37762,#37763));
#15572=EDGE_LOOP('',(#37764,#37765,#37766,#37767,#37768));
#15573=EDGE_LOOP('',(#37769,#37770,#37771,#37772));
#15574=EDGE_LOOP('',(#37773,#37774,#37775,#37776,#37777));
#15575=EDGE_LOOP('',(#37778,#37779,#37780,#37781));
#15576=EDGE_LOOP('',(#37782,#37783,#37784,#37785,#37786));
#15577=EDGE_LOOP('',(#37787,#37788,#37789,#37790));
#15578=EDGE_LOOP('',(#37791,#37792,#37793,#37794,#37795));
#15579=EDGE_LOOP('',(#37796,#37797,#37798,#37799));
#15580=EDGE_LOOP('',(#37800,#37801,#37802,#37803,#37804));
#15581=EDGE_LOOP('',(#37805,#37806,#37807,#37808,#37809));
#15582=EDGE_LOOP('',(#37810,#37811,#37812,#37813,#37814));
#15583=EDGE_LOOP('',(#37815,#37816,#37817,#37818,#37819));
#15584=EDGE_LOOP('',(#37820,#37821,#37822,#37823,#37824));
#15585=EDGE_LOOP('',(#37825,#37826,#37827,#37828));
#15586=EDGE_LOOP('',(#37829,#37830,#37831,#37832,#37833));
#15587=EDGE_LOOP('',(#37834,#37835,#37836,#37837));
#15588=EDGE_LOOP('',(#37838,#37839,#37840,#37841,#37842));
#15589=EDGE_LOOP('',(#37843,#37844,#37845,#37846,#37847));
#15590=EDGE_LOOP('',(#37848,#37849,#37850,#37851,#37852));
#15591=EDGE_LOOP('',(#37853,#37854,#37855,#37856,#37857));
#15592=EDGE_LOOP('',(#37858,#37859,#37860,#37861,#37862));
#15593=EDGE_LOOP('',(#37863,#37864,#37865,#37866,#37867));
#15594=EDGE_LOOP('',(#37868,#37869,#37870,#37871,#37872));
#15595=EDGE_LOOP('',(#37873,#37874,#37875,#37876,#37877));
#15596=EDGE_LOOP('',(#37878,#37879,#37880,#37881,#37882));
#15597=EDGE_LOOP('',(#37883,#37884,#37885,#37886,#37887));
#15598=EDGE_LOOP('',(#37888,#37889,#37890,#37891,#37892));
#15599=EDGE_LOOP('',(#37893,#37894,#37895,#37896,#37897));
#15600=EDGE_LOOP('',(#37898,#37899,#37900,#37901,#37902));
#15601=EDGE_LOOP('',(#37903,#37904,#37905,#37906,#37907));
#15602=EDGE_LOOP('',(#37908,#37909,#37910,#37911,#37912));
#15603=EDGE_LOOP('',(#37913,#37914,#37915,#37916,#37917));
#15604=EDGE_LOOP('',(#37918,#37919,#37920,#37921,#37922));
#15605=EDGE_LOOP('',(#37923,#37924,#37925,#37926,#37927));
#15606=EDGE_LOOP('',(#37928,#37929,#37930,#37931,#37932));
#15607=EDGE_LOOP('',(#37933,#37934,#37935,#37936,#37937));
#15608=EDGE_LOOP('',(#37938,#37939,#37940,#37941,#37942));
#15609=EDGE_LOOP('',(#37943,#37944,#37945,#37946,#37947));
#15610=EDGE_LOOP('',(#37948,#37949,#37950,#37951,#37952));
#15611=EDGE_LOOP('',(#37953,#37954,#37955,#37956,#37957));
#15612=EDGE_LOOP('',(#37958,#37959,#37960,#37961,#37962));
#15613=EDGE_LOOP('',(#37963,#37964,#37965,#37966,#37967));
#15614=EDGE_LOOP('',(#37968,#37969,#37970,#37971,#37972));
#15615=EDGE_LOOP('',(#37973,#37974,#37975,#37976,#37977));
#15616=EDGE_LOOP('',(#37978,#37979,#37980,#37981,#37982));
#15617=EDGE_LOOP('',(#37983,#37984,#37985,#37986,#37987));
#15618=EDGE_LOOP('',(#37988,#37989,#37990,#37991,#37992));
#15619=EDGE_LOOP('',(#37993,#37994,#37995,#37996,#37997));
#15620=EDGE_LOOP('',(#37998,#37999,#38000,#38001,#38002));
#15621=EDGE_LOOP('',(#38003,#38004,#38005,#38006,#38007));
#15622=EDGE_LOOP('',(#38008,#38009,#38010,#38011,#38012));
#15623=EDGE_LOOP('',(#38013,#38014,#38015,#38016,#38017));
#15624=EDGE_LOOP('',(#38018,#38019,#38020,#38021,#38022));
#15625=EDGE_LOOP('',(#38023,#38024,#38025,#38026,#38027));
#15626=EDGE_LOOP('',(#38028,#38029,#38030,#38031,#38032));
#15627=EDGE_LOOP('',(#38033,#38034,#38035,#38036,#38037));
#15628=EDGE_LOOP('',(#38038,#38039,#38040,#38041,#38042));
#15629=EDGE_LOOP('',(#38043,#38044,#38045,#38046,#38047));
#15630=EDGE_LOOP('',(#38048,#38049,#38050,#38051,#38052));
#15631=EDGE_LOOP('',(#38053,#38054,#38055,#38056,#38057));
#15632=EDGE_LOOP('',(#38058,#38059,#38060,#38061,#38062));
#15633=EDGE_LOOP('',(#38063,#38064,#38065,#38066,#38067));
#15634=EDGE_LOOP('',(#38068,#38069,#38070,#38071,#38072));
#15635=EDGE_LOOP('',(#38073,#38074,#38075,#38076,#38077));
#15636=EDGE_LOOP('',(#38078,#38079,#38080,#38081,#38082));
#15637=EDGE_LOOP('',(#38083,#38084,#38085,#38086));
#15638=EDGE_LOOP('',(#38087,#38088,#38089,#38090));
#15639=EDGE_LOOP('',(#38091,#38092,#38093,#38094));
#15640=EDGE_LOOP('',(#38095,#38096,#38097,#38098));
#15641=EDGE_LOOP('',(#38099,#38100,#38101,#38102));
#15642=EDGE_LOOP('',(#38103,#38104,#38105,#38106));
#15643=EDGE_LOOP('',(#38107,#38108,#38109,#38110));
#15644=EDGE_LOOP('',(#38111,#38112,#38113,#38114));
#15645=EDGE_LOOP('',(#38115,#38116,#38117,#38118));
#15646=EDGE_LOOP('',(#38119,#38120,#38121,#38122));
#15647=EDGE_LOOP('',(#38123,#38124,#38125,#38126));
#15648=EDGE_LOOP('',(#38127,#38128,#38129,#38130));
#15649=EDGE_LOOP('',(#38131,#38132,#38133,#38134));
#15650=EDGE_LOOP('',(#38135,#38136,#38137,#38138));
#15651=EDGE_LOOP('',(#38139,#38140,#38141,#38142));
#15652=EDGE_LOOP('',(#38143,#38144,#38145,#38146));
#15653=EDGE_LOOP('',(#38147,#38148,#38149,#38150));
#15654=EDGE_LOOP('',(#38151,#38152,#38153,#38154));
#15655=EDGE_LOOP('',(#38155,#38156,#38157,#38158));
#15656=EDGE_LOOP('',(#38159,#38160,#38161,#38162));
#15657=EDGE_LOOP('',(#38163,#38164,#38165,#38166));
#15658=EDGE_LOOP('',(#38167,#38168,#38169,#38170));
#15659=EDGE_LOOP('',(#38171,#38172,#38173,#38174));
#15660=EDGE_LOOP('',(#38175,#38176,#38177,#38178));
#15661=EDGE_LOOP('',(#38179,#38180,#38181,#38182));
#15662=EDGE_LOOP('',(#38183,#38184,#38185,#38186));
#15663=EDGE_LOOP('',(#38187,#38188,#38189,#38190));
#15664=EDGE_LOOP('',(#38191,#38192,#38193,#38194));
#15665=EDGE_LOOP('',(#38195,#38196,#38197,#38198));
#15666=EDGE_LOOP('',(#38199,#38200,#38201,#38202));
#15667=EDGE_LOOP('',(#38203,#38204,#38205,#38206));
#15668=EDGE_LOOP('',(#38207,#38208,#38209,#38210));
#15669=EDGE_LOOP('',(#38211,#38212,#38213,#38214));
#15670=EDGE_LOOP('',(#38215,#38216,#38217,#38218));
#15671=EDGE_LOOP('',(#38219,#38220,#38221,#38222));
#15672=EDGE_LOOP('',(#38223,#38224,#38225,#38226));
#15673=EDGE_LOOP('',(#38227,#38228,#38229,#38230));
#15674=EDGE_LOOP('',(#38231,#38232,#38233,#38234));
#15675=EDGE_LOOP('',(#38235,#38236,#38237,#38238));
#15676=EDGE_LOOP('',(#38239,#38240,#38241,#38242));
#15677=EDGE_LOOP('',(#38243,#38244,#38245,#38246));
#15678=EDGE_LOOP('',(#38247,#38248,#38249,#38250));
#15679=EDGE_LOOP('',(#38251,#38252,#38253,#38254));
#15680=EDGE_LOOP('',(#38255,#38256,#38257,#38258));
#15681=EDGE_LOOP('',(#38259,#38260,#38261,#38262));
#15682=EDGE_LOOP('',(#38263,#38264,#38265,#38266));
#15683=EDGE_LOOP('',(#38267,#38268,#38269,#38270));
#15684=EDGE_LOOP('',(#38271,#38272,#38273,#38274));
#15685=EDGE_LOOP('',(#38275,#38276,#38277,#38278));
#15686=EDGE_LOOP('',(#38279,#38280,#38281,#38282));
#15687=EDGE_LOOP('',(#38283,#38284,#38285,#38286));
#15688=EDGE_LOOP('',(#38287,#38288,#38289,#38290));
#15689=EDGE_LOOP('',(#38291,#38292,#38293,#38294));
#15690=EDGE_LOOP('',(#38295,#38296,#38297,#38298));
#15691=EDGE_LOOP('',(#38299,#38300,#38301,#38302));
#15692=EDGE_LOOP('',(#38303,#38304,#38305,#38306));
#15693=EDGE_LOOP('',(#38307,#38308,#38309,#38310));
#15694=EDGE_LOOP('',(#38311,#38312,#38313,#38314));
#15695=EDGE_LOOP('',(#38315,#38316,#38317,#38318));
#15696=EDGE_LOOP('',(#38319,#38320,#38321,#38322));
#15697=EDGE_LOOP('',(#38323,#38324,#38325,#38326));
#15698=EDGE_LOOP('',(#38327,#38328,#38329,#38330));
#15699=EDGE_LOOP('',(#38331,#38332,#38333,#38334));
#15700=EDGE_LOOP('',(#38335,#38336,#38337,#38338));
#15701=EDGE_LOOP('',(#38339,#38340,#38341,#38342));
#15702=EDGE_LOOP('',(#38343,#38344,#38345,#38346));
#15703=EDGE_LOOP('',(#38347,#38348,#38349,#38350));
#15704=EDGE_LOOP('',(#38351,#38352,#38353,#38354));
#15705=EDGE_LOOP('',(#38355,#38356,#38357,#38358));
#15706=EDGE_LOOP('',(#38359,#38360,#38361,#38362));
#15707=EDGE_LOOP('',(#38363,#38364,#38365,#38366));
#15708=EDGE_LOOP('',(#38367,#38368,#38369,#38370));
#15709=EDGE_LOOP('',(#38371,#38372,#38373,#38374));
#15710=EDGE_LOOP('',(#38375,#38376,#38377,#38378));
#15711=EDGE_LOOP('',(#38379,#38380,#38381,#38382));
#15712=EDGE_LOOP('',(#38383,#38384,#38385,#38386));
#15713=EDGE_LOOP('',(#38387,#38388,#38389,#38390));
#15714=EDGE_LOOP('',(#38391,#38392,#38393,#38394));
#15715=EDGE_LOOP('',(#38395,#38396,#38397,#38398));
#15716=EDGE_LOOP('',(#38399,#38400,#38401,#38402));
#15717=EDGE_LOOP('',(#38403,#38404,#38405,#38406));
#15718=EDGE_LOOP('',(#38407,#38408,#38409,#38410));
#15719=EDGE_LOOP('',(#38411,#38412,#38413,#38414));
#15720=EDGE_LOOP('',(#38415,#38416,#38417,#38418));
#15721=EDGE_LOOP('',(#38419,#38420,#38421,#38422));
#15722=EDGE_LOOP('',(#38423,#38424,#38425,#38426));
#15723=EDGE_LOOP('',(#38427,#38428,#38429,#38430));
#15724=EDGE_LOOP('',(#38431,#38432,#38433,#38434));
#15725=EDGE_LOOP('',(#38435,#38436,#38437,#38438));
#15726=EDGE_LOOP('',(#38439,#38440,#38441,#38442));
#15727=EDGE_LOOP('',(#38443,#38444,#38445,#38446));
#15728=EDGE_LOOP('',(#38447,#38448,#38449,#38450));
#15729=EDGE_LOOP('',(#38451,#38452,#38453,#38454));
#15730=EDGE_LOOP('',(#38455,#38456,#38457,#38458));
#15731=EDGE_LOOP('',(#38459,#38460,#38461,#38462));
#15732=EDGE_LOOP('',(#38463,#38464,#38465,#38466));
#15733=EDGE_LOOP('',(#38467,#38468,#38469,#38470));
#15734=EDGE_LOOP('',(#38471,#38472,#38473,#38474));
#15735=EDGE_LOOP('',(#38475,#38476,#38477,#38478));
#15736=EDGE_LOOP('',(#38479,#38480,#38481,#38482));
#15737=EDGE_LOOP('',(#38483,#38484,#38485,#38486));
#15738=EDGE_LOOP('',(#38487,#38488,#38489,#38490));
#15739=EDGE_LOOP('',(#38491,#38492,#38493,#38494));
#15740=EDGE_LOOP('',(#38495,#38496,#38497,#38498));
#15741=EDGE_LOOP('',(#38499,#38500,#38501,#38502));
#15742=EDGE_LOOP('',(#38503,#38504,#38505,#38506));
#15743=EDGE_LOOP('',(#38507,#38508,#38509,#38510));
#15744=EDGE_LOOP('',(#38511,#38512,#38513,#38514));
#15745=EDGE_LOOP('',(#38515,#38516,#38517,#38518));
#15746=EDGE_LOOP('',(#38519,#38520,#38521,#38522));
#15747=EDGE_LOOP('',(#38523,#38524,#38525,#38526));
#15748=EDGE_LOOP('',(#38527,#38528,#38529,#38530));
#15749=EDGE_LOOP('',(#38531,#38532,#38533,#38534));
#15750=EDGE_LOOP('',(#38535,#38536,#38537,#38538));
#15751=EDGE_LOOP('',(#38539,#38540,#38541,#38542));
#15752=EDGE_LOOP('',(#38543,#38544,#38545,#38546));
#15753=EDGE_LOOP('',(#38547,#38548,#38549,#38550));
#15754=EDGE_LOOP('',(#38551,#38552,#38553,#38554));
#15755=EDGE_LOOP('',(#38555,#38556,#38557,#38558));
#15756=EDGE_LOOP('',(#38559,#38560,#38561,#38562));
#15757=EDGE_LOOP('',(#38563,#38564,#38565,#38566));
#15758=EDGE_LOOP('',(#38567,#38568,#38569,#38570));
#15759=EDGE_LOOP('',(#38571,#38572,#38573,#38574));
#15760=EDGE_LOOP('',(#38575,#38576,#38577,#38578));
#15761=EDGE_LOOP('',(#38579,#38580,#38581,#38582));
#15762=EDGE_LOOP('',(#38583,#38584,#38585,#38586));
#15763=EDGE_LOOP('',(#38587,#38588,#38589,#38590));
#15764=EDGE_LOOP('',(#38591,#38592,#38593,#38594));
#15765=EDGE_LOOP('',(#38595,#38596,#38597,#38598));
#15766=EDGE_LOOP('',(#38599,#38600,#38601,#38602));
#15767=EDGE_LOOP('',(#38603,#38604,#38605,#38606));
#15768=EDGE_LOOP('',(#38607,#38608,#38609,#38610));
#15769=EDGE_LOOP('',(#38611,#38612,#38613,#38614));
#15770=EDGE_LOOP('',(#38615,#38616,#38617,#38618));
#15771=EDGE_LOOP('',(#38619,#38620,#38621,#38622));
#15772=EDGE_LOOP('',(#38623,#38624,#38625,#38626));
#15773=EDGE_LOOP('',(#38627,#38628,#38629,#38630));
#15774=EDGE_LOOP('',(#38631,#38632,#38633,#38634));
#15775=EDGE_LOOP('',(#38635,#38636,#38637,#38638));
#15776=EDGE_LOOP('',(#38639,#38640,#38641,#38642));
#15777=EDGE_LOOP('',(#38643,#38644,#38645,#38646));
#15778=EDGE_LOOP('',(#38647,#38648,#38649,#38650));
#15779=EDGE_LOOP('',(#38651,#38652,#38653,#38654));
#15780=EDGE_LOOP('',(#38655,#38656,#38657,#38658));
#15781=EDGE_LOOP('',(#38659,#38660,#38661,#38662));
#15782=EDGE_LOOP('',(#38663,#38664,#38665,#38666));
#15783=EDGE_LOOP('',(#38667,#38668,#38669,#38670));
#15784=EDGE_LOOP('',(#38671,#38672,#38673,#38674));
#15785=EDGE_LOOP('',(#38675,#38676,#38677,#38678));
#15786=EDGE_LOOP('',(#38679,#38680,#38681,#38682));
#15787=EDGE_LOOP('',(#38683,#38684,#38685,#38686));
#15788=EDGE_LOOP('',(#38687,#38688,#38689,#38690));
#15789=EDGE_LOOP('',(#38691,#38692,#38693,#38694));
#15790=EDGE_LOOP('',(#38695,#38696,#38697,#38698));
#15791=EDGE_LOOP('',(#38699,#38700,#38701,#38702));
#15792=EDGE_LOOP('',(#38703,#38704,#38705,#38706));
#15793=EDGE_LOOP('',(#38707,#38708,#38709,#38710));
#15794=EDGE_LOOP('',(#38711,#38712,#38713,#38714));
#15795=EDGE_LOOP('',(#38715,#38716,#38717,#38718));
#15796=EDGE_LOOP('',(#38719,#38720,#38721,#38722));
#15797=EDGE_LOOP('',(#38723,#38724,#38725,#38726));
#15798=EDGE_LOOP('',(#38727,#38728,#38729,#38730));
#15799=EDGE_LOOP('',(#38731,#38732,#38733,#38734));
#15800=EDGE_LOOP('',(#38735,#38736,#38737,#38738));
#15801=EDGE_LOOP('',(#38739,#38740,#38741,#38742));
#15802=EDGE_LOOP('',(#38743,#38744,#38745,#38746));
#15803=EDGE_LOOP('',(#38747,#38748,#38749,#38750));
#15804=EDGE_LOOP('',(#38751,#38752,#38753,#38754));
#15805=EDGE_LOOP('',(#38755,#38756,#38757,#38758));
#15806=EDGE_LOOP('',(#38759,#38760,#38761,#38762));
#15807=EDGE_LOOP('',(#38763,#38764,#38765,#38766));
#15808=EDGE_LOOP('',(#38767,#38768,#38769,#38770));
#15809=EDGE_LOOP('',(#38771,#38772,#38773,#38774));
#15810=EDGE_LOOP('',(#38775,#38776,#38777,#38778));
#15811=EDGE_LOOP('',(#38779,#38780,#38781,#38782));
#15812=EDGE_LOOP('',(#38783,#38784,#38785,#38786));
#15813=EDGE_LOOP('',(#38787,#38788,#38789,#38790));
#15814=EDGE_LOOP('',(#38791,#38792,#38793,#38794));
#15815=EDGE_LOOP('',(#38795,#38796,#38797,#38798));
#15816=EDGE_LOOP('',(#38799,#38800,#38801,#38802));
#15817=EDGE_LOOP('',(#38803,#38804,#38805,#38806));
#15818=EDGE_LOOP('',(#38807,#38808,#38809,#38810));
#15819=EDGE_LOOP('',(#38811,#38812,#38813,#38814));
#15820=EDGE_LOOP('',(#38815,#38816,#38817,#38818));
#15821=EDGE_LOOP('',(#38819,#38820,#38821,#38822));
#15822=EDGE_LOOP('',(#38823,#38824,#38825,#38826));
#15823=EDGE_LOOP('',(#38827,#38828,#38829,#38830));
#15824=EDGE_LOOP('',(#38831,#38832,#38833,#38834));
#15825=EDGE_LOOP('',(#38835,#38836,#38837,#38838));
#15826=EDGE_LOOP('',(#38839,#38840,#38841,#38842));
#15827=EDGE_LOOP('',(#38843,#38844,#38845,#38846));
#15828=EDGE_LOOP('',(#38847,#38848,#38849,#38850));
#15829=EDGE_LOOP('',(#38851,#38852,#38853,#38854));
#15830=EDGE_LOOP('',(#38855,#38856,#38857,#38858));
#15831=EDGE_LOOP('',(#38859,#38860,#38861,#38862));
#15832=EDGE_LOOP('',(#38863,#38864,#38865,#38866));
#15833=EDGE_LOOP('',(#38867,#38868,#38869,#38870));
#15834=EDGE_LOOP('',(#38871,#38872,#38873,#38874));
#15835=EDGE_LOOP('',(#38875,#38876,#38877,#38878));
#15836=EDGE_LOOP('',(#38879,#38880,#38881,#38882));
#15837=EDGE_LOOP('',(#38883,#38884,#38885,#38886));
#15838=EDGE_LOOP('',(#38887,#38888,#38889,#38890));
#15839=EDGE_LOOP('',(#38891,#38892,#38893,#38894));
#15840=EDGE_LOOP('',(#38895,#38896,#38897,#38898));
#15841=EDGE_LOOP('',(#38899,#38900,#38901,#38902));
#15842=EDGE_LOOP('',(#38903,#38904,#38905,#38906));
#15843=EDGE_LOOP('',(#38907,#38908,#38909,#38910));
#15844=EDGE_LOOP('',(#38911,#38912,#38913,#38914));
#15845=EDGE_LOOP('',(#38915,#38916,#38917,#38918));
#15846=EDGE_LOOP('',(#38919,#38920,#38921,#38922));
#15847=EDGE_LOOP('',(#38923,#38924,#38925,#38926));
#15848=EDGE_LOOP('',(#38927,#38928,#38929,#38930));
#15849=EDGE_LOOP('',(#38931,#38932,#38933,#38934));
#15850=EDGE_LOOP('',(#38935,#38936,#38937,#38938));
#15851=EDGE_LOOP('',(#38939,#38940,#38941,#38942));
#15852=EDGE_LOOP('',(#38943,#38944,#38945,#38946));
#15853=EDGE_LOOP('',(#38947,#38948,#38949,#38950));
#15854=EDGE_LOOP('',(#38951,#38952,#38953,#38954));
#15855=EDGE_LOOP('',(#38955,#38956,#38957,#38958));
#15856=EDGE_LOOP('',(#38959,#38960,#38961,#38962));
#15857=EDGE_LOOP('',(#38963,#38964,#38965,#38966));
#15858=EDGE_LOOP('',(#38967,#38968,#38969,#38970));
#15859=EDGE_LOOP('',(#38971,#38972,#38973,#38974));
#15860=EDGE_LOOP('',(#38975,#38976,#38977,#38978));
#15861=EDGE_LOOP('',(#38979,#38980,#38981,#38982));
#15862=EDGE_LOOP('',(#38983,#38984,#38985,#38986));
#15863=EDGE_LOOP('',(#38987,#38988,#38989,#38990));
#15864=EDGE_LOOP('',(#38991,#38992,#38993,#38994));
#15865=EDGE_LOOP('',(#38995,#38996,#38997,#38998));
#15866=EDGE_LOOP('',(#38999,#39000,#39001,#39002));
#15867=EDGE_LOOP('',(#39003,#39004,#39005,#39006));
#15868=EDGE_LOOP('',(#39007,#39008,#39009,#39010));
#15869=EDGE_LOOP('',(#39011,#39012,#39013,#39014));
#15870=EDGE_LOOP('',(#39015,#39016,#39017,#39018));
#15871=EDGE_LOOP('',(#39019,#39020,#39021,#39022));
#15872=EDGE_LOOP('',(#39023,#39024,#39025,#39026));
#15873=EDGE_LOOP('',(#39027,#39028,#39029,#39030));
#15874=EDGE_LOOP('',(#39031,#39032,#39033,#39034));
#15875=EDGE_LOOP('',(#39035,#39036,#39037,#39038));
#15876=EDGE_LOOP('',(#39039,#39040,#39041,#39042));
#15877=EDGE_LOOP('',(#39043,#39044,#39045,#39046));
#15878=EDGE_LOOP('',(#39047,#39048,#39049,#39050));
#15879=EDGE_LOOP('',(#39051,#39052,#39053,#39054));
#15880=EDGE_LOOP('',(#39055,#39056,#39057,#39058));
#15881=EDGE_LOOP('',(#39059,#39060,#39061,#39062));
#15882=EDGE_LOOP('',(#39063,#39064,#39065,#39066));
#15883=EDGE_LOOP('',(#39067,#39068,#39069,#39070));
#15884=EDGE_LOOP('',(#39071,#39072,#39073,#39074));
#15885=EDGE_LOOP('',(#39075,#39076,#39077,#39078));
#15886=EDGE_LOOP('',(#39079,#39080,#39081,#39082));
#15887=EDGE_LOOP('',(#39083,#39084,#39085,#39086));
#15888=EDGE_LOOP('',(#39087,#39088,#39089,#39090));
#15889=EDGE_LOOP('',(#39091,#39092,#39093,#39094));
#15890=EDGE_LOOP('',(#39095,#39096,#39097,#39098));
#15891=EDGE_LOOP('',(#39099,#39100,#39101,#39102));
#15892=EDGE_LOOP('',(#39103,#39104,#39105,#39106));
#15893=EDGE_LOOP('',(#39107,#39108,#39109,#39110));
#15894=EDGE_LOOP('',(#39111,#39112,#39113,#39114));
#15895=EDGE_LOOP('',(#39115,#39116,#39117,#39118));
#15896=EDGE_LOOP('',(#39119,#39120,#39121,#39122));
#15897=EDGE_LOOP('',(#39123,#39124,#39125,#39126));
#15898=EDGE_LOOP('',(#39127,#39128,#39129,#39130));
#15899=EDGE_LOOP('',(#39131,#39132,#39133,#39134));
#15900=EDGE_LOOP('',(#39135,#39136,#39137,#39138));
#15901=EDGE_LOOP('',(#39139,#39140,#39141,#39142));
#15902=EDGE_LOOP('',(#39143,#39144,#39145,#39146));
#15903=EDGE_LOOP('',(#39147,#39148,#39149,#39150));
#15904=EDGE_LOOP('',(#39151,#39152,#39153,#39154));
#15905=EDGE_LOOP('',(#39155,#39156,#39157,#39158));
#15906=EDGE_LOOP('',(#39159,#39160,#39161,#39162));
#15907=EDGE_LOOP('',(#39163,#39164,#39165,#39166));
#15908=EDGE_LOOP('',(#39167,#39168,#39169,#39170));
#15909=EDGE_LOOP('',(#39171,#39172,#39173,#39174));
#15910=EDGE_LOOP('',(#39175,#39176,#39177,#39178));
#15911=EDGE_LOOP('',(#39179,#39180,#39181,#39182));
#15912=EDGE_LOOP('',(#39183,#39184,#39185,#39186));
#15913=EDGE_LOOP('',(#39187,#39188,#39189,#39190));
#15914=EDGE_LOOP('',(#39191,#39192,#39193,#39194));
#15915=EDGE_LOOP('',(#39195,#39196,#39197,#39198));
#15916=EDGE_LOOP('',(#39199,#39200,#39201,#39202));
#15917=EDGE_LOOP('',(#39203,#39204,#39205,#39206));
#15918=EDGE_LOOP('',(#39207,#39208,#39209,#39210));
#15919=EDGE_LOOP('',(#39211,#39212,#39213,#39214));
#15920=EDGE_LOOP('',(#39215,#39216,#39217,#39218));
#15921=EDGE_LOOP('',(#39219,#39220,#39221,#39222));
#15922=EDGE_LOOP('',(#39223,#39224,#39225,#39226));
#15923=EDGE_LOOP('',(#39227,#39228,#39229,#39230));
#15924=EDGE_LOOP('',(#39231,#39232,#39233,#39234));
#15925=EDGE_LOOP('',(#39235,#39236,#39237,#39238));
#15926=EDGE_LOOP('',(#39239,#39240,#39241,#39242));
#15927=EDGE_LOOP('',(#39243,#39244,#39245,#39246));
#15928=EDGE_LOOP('',(#39247,#39248,#39249,#39250));
#15929=EDGE_LOOP('',(#39251,#39252,#39253,#39254));
#15930=EDGE_LOOP('',(#39255,#39256,#39257,#39258));
#15931=EDGE_LOOP('',(#39259,#39260,#39261,#39262));
#15932=EDGE_LOOP('',(#39263,#39264,#39265,#39266));
#15933=EDGE_LOOP('',(#39267,#39268,#39269,#39270));
#15934=EDGE_LOOP('',(#39271,#39272,#39273,#39274));
#15935=EDGE_LOOP('',(#39275,#39276,#39277,#39278));
#15936=EDGE_LOOP('',(#39279,#39280,#39281,#39282));
#15937=EDGE_LOOP('',(#39283,#39284,#39285,#39286));
#15938=EDGE_LOOP('',(#39287,#39288,#39289,#39290));
#15939=EDGE_LOOP('',(#39291,#39292,#39293,#39294));
#15940=EDGE_LOOP('',(#39295,#39296,#39297,#39298));
#15941=EDGE_LOOP('',(#39299,#39300,#39301,#39302));
#15942=EDGE_LOOP('',(#39303,#39304,#39305,#39306));
#15943=EDGE_LOOP('',(#39307,#39308,#39309,#39310));
#15944=EDGE_LOOP('',(#39311,#39312,#39313,#39314));
#15945=EDGE_LOOP('',(#39315,#39316,#39317,#39318));
#15946=EDGE_LOOP('',(#39319,#39320,#39321,#39322));
#15947=EDGE_LOOP('',(#39323,#39324,#39325,#39326));
#15948=EDGE_LOOP('',(#39327,#39328,#39329,#39330));
#15949=EDGE_LOOP('',(#39331,#39332,#39333,#39334));
#15950=EDGE_LOOP('',(#39335,#39336,#39337,#39338));
#15951=EDGE_LOOP('',(#39339,#39340,#39341,#39342));
#15952=EDGE_LOOP('',(#39343,#39344,#39345,#39346));
#15953=EDGE_LOOP('',(#39347,#39348,#39349,#39350));
#15954=EDGE_LOOP('',(#39351,#39352,#39353,#39354));
#15955=EDGE_LOOP('',(#39355,#39356,#39357,#39358));
#15956=EDGE_LOOP('',(#39359,#39360,#39361,#39362));
#15957=EDGE_LOOP('',(#39363,#39364,#39365,#39366));
#15958=EDGE_LOOP('',(#39367,#39368,#39369,#39370));
#15959=EDGE_LOOP('',(#39371,#39372,#39373,#39374));
#15960=EDGE_LOOP('',(#39375,#39376,#39377,#39378));
#15961=EDGE_LOOP('',(#39379,#39380,#39381,#39382));
#15962=EDGE_LOOP('',(#39383,#39384,#39385,#39386));
#15963=EDGE_LOOP('',(#39387,#39388,#39389,#39390));
#15964=EDGE_LOOP('',(#39391,#39392,#39393,#39394));
#15965=EDGE_LOOP('',(#39395,#39396,#39397,#39398));
#15966=EDGE_LOOP('',(#39399,#39400,#39401,#39402));
#15967=EDGE_LOOP('',(#39403,#39404,#39405,#39406));
#15968=EDGE_LOOP('',(#39407,#39408,#39409,#39410));
#15969=EDGE_LOOP('',(#39411,#39412,#39413,#39414));
#15970=EDGE_LOOP('',(#39415,#39416,#39417,#39418));
#15971=EDGE_LOOP('',(#39419,#39420,#39421,#39422));
#15972=EDGE_LOOP('',(#39423,#39424,#39425,#39426));
#15973=EDGE_LOOP('',(#39427,#39428,#39429,#39430));
#15974=EDGE_LOOP('',(#39431,#39432,#39433,#39434));
#15975=EDGE_LOOP('',(#39435,#39436,#39437,#39438));
#15976=EDGE_LOOP('',(#39439,#39440,#39441,#39442));
#15977=EDGE_LOOP('',(#39443,#39444,#39445,#39446));
#15978=EDGE_LOOP('',(#39447,#39448,#39449,#39450));
#15979=EDGE_LOOP('',(#39451,#39452,#39453,#39454));
#15980=EDGE_LOOP('',(#39455,#39456,#39457,#39458));
#15981=EDGE_LOOP('',(#39459,#39460,#39461,#39462));
#15982=EDGE_LOOP('',(#39463,#39464,#39465,#39466));
#15983=EDGE_LOOP('',(#39467,#39468,#39469,#39470));
#15984=EDGE_LOOP('',(#39471,#39472,#39473,#39474));
#15985=EDGE_LOOP('',(#39475,#39476,#39477,#39478));
#15986=EDGE_LOOP('',(#39479,#39480,#39481,#39482));
#15987=EDGE_LOOP('',(#39483,#39484,#39485,#39486));
#15988=EDGE_LOOP('',(#39487,#39488,#39489,#39490));
#15989=EDGE_LOOP('',(#39491,#39492,#39493,#39494));
#15990=EDGE_LOOP('',(#39495,#39496,#39497,#39498));
#15991=EDGE_LOOP('',(#39499,#39500,#39501,#39502));
#15992=EDGE_LOOP('',(#39503,#39504,#39505,#39506));
#15993=EDGE_LOOP('',(#39507,#39508,#39509,#39510));
#15994=EDGE_LOOP('',(#39511,#39512,#39513,#39514));
#15995=EDGE_LOOP('',(#39515,#39516,#39517,#39518));
#15996=EDGE_LOOP('',(#39519,#39520,#39521,#39522));
#15997=EDGE_LOOP('',(#39523,#39524,#39525,#39526));
#15998=EDGE_LOOP('',(#39527,#39528,#39529,#39530));
#15999=EDGE_LOOP('',(#39531,#39532,#39533,#39534));
#16000=EDGE_LOOP('',(#39535,#39536,#39537,#39538));
#16001=EDGE_LOOP('',(#39539,#39540,#39541,#39542));
#16002=EDGE_LOOP('',(#39543,#39544,#39545,#39546));
#16003=EDGE_LOOP('',(#39547,#39548,#39549,#39550));
#16004=EDGE_LOOP('',(#39551,#39552,#39553,#39554));
#16005=EDGE_LOOP('',(#39555,#39556,#39557,#39558));
#16006=EDGE_LOOP('',(#39559,#39560,#39561,#39562));
#16007=EDGE_LOOP('',(#39563,#39564,#39565,#39566));
#16008=EDGE_LOOP('',(#39567,#39568,#39569,#39570));
#16009=EDGE_LOOP('',(#39571,#39572,#39573,#39574));
#16010=EDGE_LOOP('',(#39575,#39576,#39577,#39578));
#16011=EDGE_LOOP('',(#39579,#39580,#39581,#39582));
#16012=EDGE_LOOP('',(#39583,#39584,#39585,#39586));
#16013=EDGE_LOOP('',(#39587,#39588,#39589,#39590));
#16014=EDGE_LOOP('',(#39591,#39592,#39593,#39594));
#16015=EDGE_LOOP('',(#39595,#39596,#39597,#39598));
#16016=EDGE_LOOP('',(#39599,#39600,#39601,#39602));
#16017=EDGE_LOOP('',(#39603,#39604,#39605,#39606));
#16018=EDGE_LOOP('',(#39607,#39608,#39609,#39610));
#16019=EDGE_LOOP('',(#39611,#39612,#39613,#39614));
#16020=EDGE_LOOP('',(#39615,#39616,#39617,#39618));
#16021=EDGE_LOOP('',(#39619,#39620,#39621,#39622));
#16022=EDGE_LOOP('',(#39623,#39624,#39625,#39626));
#16023=EDGE_LOOP('',(#39627,#39628,#39629,#39630));
#16024=EDGE_LOOP('',(#39631,#39632,#39633,#39634));
#16025=EDGE_LOOP('',(#39635,#39636,#39637,#39638));
#16026=EDGE_LOOP('',(#39639,#39640,#39641,#39642));
#16027=EDGE_LOOP('',(#39643,#39644,#39645,#39646));
#16028=EDGE_LOOP('',(#39647,#39648,#39649,#39650));
#16029=EDGE_LOOP('',(#39651,#39652,#39653,#39654));
#16030=EDGE_LOOP('',(#39655,#39656,#39657,#39658));
#16031=EDGE_LOOP('',(#39659,#39660,#39661,#39662));
#16032=EDGE_LOOP('',(#39663,#39664,#39665,#39666));
#16033=EDGE_LOOP('',(#39667,#39668,#39669,#39670));
#16034=EDGE_LOOP('',(#39671,#39672,#39673,#39674));
#16035=EDGE_LOOP('',(#39675,#39676,#39677,#39678));
#16036=EDGE_LOOP('',(#39679,#39680,#39681,#39682));
#16037=EDGE_LOOP('',(#39683,#39684,#39685,#39686));
#16038=EDGE_LOOP('',(#39687,#39688,#39689,#39690));
#16039=EDGE_LOOP('',(#39691,#39692,#39693,#39694));
#16040=EDGE_LOOP('',(#39695,#39696,#39697,#39698));
#16041=EDGE_LOOP('',(#39699,#39700,#39701,#39702));
#16042=EDGE_LOOP('',(#39703,#39704,#39705,#39706));
#16043=EDGE_LOOP('',(#39707,#39708,#39709,#39710));
#16044=EDGE_LOOP('',(#39711,#39712,#39713,#39714));
#16045=EDGE_LOOP('',(#39715,#39716,#39717,#39718));
#16046=EDGE_LOOP('',(#39719,#39720,#39721,#39722));
#16047=EDGE_LOOP('',(#39723,#39724,#39725,#39726));
#16048=EDGE_LOOP('',(#39727,#39728,#39729,#39730));
#16049=EDGE_LOOP('',(#39731,#39732,#39733,#39734));
#16050=EDGE_LOOP('',(#39735,#39736,#39737,#39738));
#16051=EDGE_LOOP('',(#39739,#39740,#39741,#39742));
#16052=EDGE_LOOP('',(#39743,#39744,#39745,#39746));
#16053=EDGE_LOOP('',(#39747,#39748,#39749,#39750));
#16054=EDGE_LOOP('',(#39751,#39752,#39753,#39754));
#16055=EDGE_LOOP('',(#39755,#39756,#39757,#39758));
#16056=EDGE_LOOP('',(#39759,#39760,#39761,#39762));
#16057=EDGE_LOOP('',(#39763,#39764,#39765,#39766));
#16058=EDGE_LOOP('',(#39767,#39768,#39769,#39770));
#16059=EDGE_LOOP('',(#39771,#39772,#39773,#39774));
#16060=EDGE_LOOP('',(#39775,#39776,#39777,#39778));
#16061=EDGE_LOOP('',(#39779,#39780,#39781,#39782));
#16062=EDGE_LOOP('',(#39783,#39784,#39785,#39786));
#16063=EDGE_LOOP('',(#39787,#39788,#39789,#39790));
#16064=EDGE_LOOP('',(#39791,#39792,#39793,#39794));
#16065=EDGE_LOOP('',(#39795,#39796,#39797,#39798));
#16066=EDGE_LOOP('',(#39799,#39800,#39801,#39802));
#16067=EDGE_LOOP('',(#39803,#39804,#39805,#39806));
#16068=EDGE_LOOP('',(#39807,#39808,#39809,#39810));
#16069=EDGE_LOOP('',(#39811,#39812,#39813,#39814));
#16070=EDGE_LOOP('',(#39815,#39816,#39817,#39818));
#16071=EDGE_LOOP('',(#39819,#39820,#39821,#39822));
#16072=EDGE_LOOP('',(#39823,#39824,#39825,#39826));
#16073=EDGE_LOOP('',(#39827,#39828,#39829,#39830));
#16074=EDGE_LOOP('',(#39831,#39832,#39833,#39834));
#16075=EDGE_LOOP('',(#39835,#39836,#39837,#39838));
#16076=EDGE_LOOP('',(#39839,#39840,#39841,#39842));
#16077=EDGE_LOOP('',(#39843,#39844,#39845,#39846));
#16078=EDGE_LOOP('',(#39847,#39848,#39849,#39850));
#16079=EDGE_LOOP('',(#39851,#39852,#39853,#39854));
#16080=EDGE_LOOP('',(#39855,#39856,#39857,#39858));
#16081=EDGE_LOOP('',(#39859,#39860,#39861,#39862));
#16082=EDGE_LOOP('',(#39863,#39864,#39865,#39866));
#16083=EDGE_LOOP('',(#39867,#39868,#39869,#39870));
#16084=EDGE_LOOP('',(#39871,#39872,#39873,#39874));
#16085=EDGE_LOOP('',(#39875,#39876,#39877,#39878));
#16086=EDGE_LOOP('',(#39879,#39880,#39881,#39882));
#16087=EDGE_LOOP('',(#39883,#39884,#39885,#39886));
#16088=EDGE_LOOP('',(#39887,#39888,#39889,#39890));
#16089=EDGE_LOOP('',(#39891,#39892,#39893,#39894));
#16090=EDGE_LOOP('',(#39895,#39896,#39897,#39898));
#16091=EDGE_LOOP('',(#39899,#39900,#39901,#39902));
#16092=EDGE_LOOP('',(#39903,#39904,#39905,#39906));
#16093=EDGE_LOOP('',(#39907,#39908,#39909,#39910));
#16094=EDGE_LOOP('',(#39911,#39912,#39913,#39914));
#16095=EDGE_LOOP('',(#39915,#39916,#39917,#39918));
#16096=EDGE_LOOP('',(#39919,#39920,#39921,#39922));
#16097=EDGE_LOOP('',(#39923,#39924,#39925,#39926));
#16098=EDGE_LOOP('',(#39927,#39928,#39929,#39930));
#16099=EDGE_LOOP('',(#39931,#39932,#39933,#39934));
#16100=EDGE_LOOP('',(#39935,#39936,#39937,#39938));
#16101=EDGE_LOOP('',(#39939,#39940,#39941,#39942));
#16102=EDGE_LOOP('',(#39943,#39944,#39945,#39946));
#16103=EDGE_LOOP('',(#39947,#39948,#39949,#39950));
#16104=EDGE_LOOP('',(#39951,#39952,#39953,#39954));
#16105=EDGE_LOOP('',(#39955,#39956,#39957,#39958));
#16106=EDGE_LOOP('',(#39959,#39960,#39961,#39962));
#16107=EDGE_LOOP('',(#39963,#39964,#39965,#39966));
#16108=EDGE_LOOP('',(#39967,#39968,#39969,#39970));
#16109=EDGE_LOOP('',(#39971,#39972,#39973,#39974));
#16110=EDGE_LOOP('',(#39975,#39976,#39977,#39978));
#16111=EDGE_LOOP('',(#39979,#39980,#39981,#39982));
#16112=EDGE_LOOP('',(#39983,#39984,#39985,#39986));
#16113=EDGE_LOOP('',(#39987,#39988,#39989,#39990));
#16114=EDGE_LOOP('',(#39991,#39992,#39993,#39994));
#16115=EDGE_LOOP('',(#39995,#39996,#39997,#39998));
#16116=EDGE_LOOP('',(#39999,#40000,#40001,#40002));
#16117=EDGE_LOOP('',(#40003,#40004,#40005,#40006));
#16118=EDGE_LOOP('',(#40007,#40008,#40009,#40010));
#16119=EDGE_LOOP('',(#40011,#40012,#40013,#40014));
#16120=EDGE_LOOP('',(#40015,#40016,#40017,#40018));
#16121=EDGE_LOOP('',(#40019,#40020,#40021,#40022));
#16122=EDGE_LOOP('',(#40023,#40024,#40025,#40026));
#16123=EDGE_LOOP('',(#40027,#40028,#40029,#40030));
#16124=EDGE_LOOP('',(#40031,#40032,#40033,#40034));
#16125=EDGE_LOOP('',(#40035,#40036,#40037,#40038));
#16126=EDGE_LOOP('',(#40039,#40040,#40041,#40042));
#16127=EDGE_LOOP('',(#40043,#40044,#40045,#40046));
#16128=EDGE_LOOP('',(#40047,#40048,#40049,#40050));
#16129=EDGE_LOOP('',(#40051,#40052,#40053,#40054));
#16130=EDGE_LOOP('',(#40055,#40056,#40057,#40058));
#16131=EDGE_LOOP('',(#40059,#40060,#40061,#40062));
#16132=EDGE_LOOP('',(#40063,#40064,#40065,#40066));
#16133=EDGE_LOOP('',(#40067,#40068,#40069,#40070));
#16134=EDGE_LOOP('',(#40071,#40072,#40073,#40074));
#16135=EDGE_LOOP('',(#40075,#40076,#40077,#40078));
#16136=EDGE_LOOP('',(#40079,#40080,#40081,#40082));
#16137=EDGE_LOOP('',(#40083,#40084,#40085,#40086));
#16138=EDGE_LOOP('',(#40087,#40088,#40089,#40090));
#16139=EDGE_LOOP('',(#40091,#40092,#40093,#40094));
#16140=EDGE_LOOP('',(#40095,#40096,#40097,#40098));
#16141=EDGE_LOOP('',(#40099,#40100,#40101,#40102));
#16142=EDGE_LOOP('',(#40103,#40104,#40105,#40106));
#16143=EDGE_LOOP('',(#40107,#40108,#40109,#40110));
#16144=EDGE_LOOP('',(#40111,#40112,#40113,#40114));
#16145=EDGE_LOOP('',(#40115,#40116,#40117,#40118));
#16146=EDGE_LOOP('',(#40119,#40120,#40121,#40122));
#16147=EDGE_LOOP('',(#40123,#40124,#40125,#40126));
#16148=EDGE_LOOP('',(#40127,#40128,#40129,#40130));
#16149=EDGE_LOOP('',(#40131,#40132,#40133,#40134));
#16150=EDGE_LOOP('',(#40135,#40136,#40137,#40138));
#16151=EDGE_LOOP('',(#40139,#40140,#40141,#40142));
#16152=EDGE_LOOP('',(#40143,#40144,#40145,#40146));
#16153=EDGE_LOOP('',(#40147,#40148,#40149,#40150));
#16154=EDGE_LOOP('',(#40151,#40152,#40153,#40154));
#16155=EDGE_LOOP('',(#40155,#40156,#40157,#40158));
#16156=EDGE_LOOP('',(#40159,#40160,#40161,#40162));
#16157=EDGE_LOOP('',(#40163,#40164,#40165,#40166));
#16158=EDGE_LOOP('',(#40167,#40168,#40169,#40170));
#16159=EDGE_LOOP('',(#40171,#40172,#40173,#40174));
#16160=EDGE_LOOP('',(#40175,#40176,#40177,#40178));
#16161=EDGE_LOOP('',(#40179,#40180,#40181,#40182));
#16162=EDGE_LOOP('',(#40183,#40184,#40185,#40186));
#16163=EDGE_LOOP('',(#40187,#40188,#40189,#40190));
#16164=EDGE_LOOP('',(#40191,#40192,#40193,#40194));
#16165=EDGE_LOOP('',(#40195,#40196,#40197,#40198));
#16166=EDGE_LOOP('',(#40199,#40200,#40201,#40202));
#16167=EDGE_LOOP('',(#40203,#40204,#40205,#40206));
#16168=EDGE_LOOP('',(#40207,#40208,#40209,#40210));
#16169=EDGE_LOOP('',(#40211,#40212,#40213,#40214));
#16170=EDGE_LOOP('',(#40215,#40216,#40217,#40218));
#16171=EDGE_LOOP('',(#40219,#40220,#40221,#40222));
#16172=EDGE_LOOP('',(#40223,#40224,#40225,#40226));
#16173=EDGE_LOOP('',(#40227,#40228,#40229,#40230));
#16174=EDGE_LOOP('',(#40231,#40232,#40233,#40234));
#16175=EDGE_LOOP('',(#40235,#40236,#40237,#40238));
#16176=EDGE_LOOP('',(#40239,#40240,#40241,#40242));
#16177=EDGE_LOOP('',(#40243,#40244,#40245,#40246,#40247));
#16178=EDGE_LOOP('',(#40248,#40249,#40250,#40251));
#16179=EDGE_LOOP('',(#40252,#40253,#40254,#40255,#40256));
#16180=EDGE_LOOP('',(#40257,#40258,#40259,#40260));
#16181=EDGE_LOOP('',(#40261,#40262,#40263,#40264,#40265));
#16182=EDGE_LOOP('',(#40266));
#16183=EDGE_LOOP('',(#40267));
#16184=EDGE_LOOP('',(#40268,#40269,#40270,#40271));
#16185=EDGE_LOOP('',(#40272,#40273,#40274,#40275));
#16186=EDGE_LOOP('',(#40276,#40277,#40278,#40279));
#16187=EDGE_LOOP('',(#40280,#40281,#40282,#40283));
#16188=EDGE_LOOP('',(#40284,#40285,#40286,#40287,#40288));
#16189=EDGE_LOOP('',(#40289,#40290,#40291,#40292,#40293));
#16190=EDGE_LOOP('',(#40294,#40295,#40296,#40297,#40298));
#16191=EDGE_LOOP('',(#40299,#40300,#40301,#40302,#40303));
#16192=EDGE_LOOP('',(#40304));
#16193=EDGE_LOOP('',(#40305,#40306));
#16194=EDGE_LOOP('',(#40307));
#16195=EDGE_LOOP('',(#40308));
#16196=EDGE_LOOP('',(#40309));
#16197=EDGE_LOOP('',(#40310));
#16198=EDGE_LOOP('',(#40311));
#16199=EDGE_LOOP('',(#40312));
#16200=EDGE_LOOP('',(#40313));
#16201=EDGE_LOOP('',(#40314));
#16202=EDGE_LOOP('',(#40315));
#16203=EDGE_LOOP('',(#40316));
#16204=EDGE_LOOP('',(#40317,#40318));
#16205=EDGE_LOOP('',(#40319));
#16206=EDGE_LOOP('',(#40320));
#16207=EDGE_LOOP('',(#40321));
#16208=EDGE_LOOP('',(#40322));
#16209=EDGE_LOOP('',(#40323));
#16210=EDGE_LOOP('',(#40324));
#16211=EDGE_LOOP('',(#40325));
#16212=EDGE_LOOP('',(#40326));
#16213=EDGE_LOOP('',(#40327));
#16214=EDGE_LOOP('',(#40328));
#16215=EDGE_LOOP('',(#40329));
#16216=EDGE_LOOP('',(#40330));
#16217=EDGE_LOOP('',(#40331));
#16218=EDGE_LOOP('',(#40332));
#16219=EDGE_LOOP('',(#40333));
#16220=EDGE_LOOP('',(#40334));
#16221=EDGE_LOOP('',(#40335));
#16222=EDGE_LOOP('',(#40336));
#16223=EDGE_LOOP('',(#40337));
#16224=EDGE_LOOP('',(#40338));
#16225=EDGE_LOOP('',(#40339));
#16226=EDGE_LOOP('',(#40340));
#16227=EDGE_LOOP('',(#40341));
#16228=EDGE_LOOP('',(#40342));
#16229=EDGE_LOOP('',(#40343));
#16230=EDGE_LOOP('',(#40344));
#16231=EDGE_LOOP('',(#40345));
#16232=EDGE_LOOP('',(#40346));
#16233=EDGE_LOOP('',(#40347));
#16234=EDGE_LOOP('',(#40348));
#16235=EDGE_LOOP('',(#40349));
#16236=EDGE_LOOP('',(#40350));
#16237=EDGE_LOOP('',(#40351));
#16238=EDGE_LOOP('',(#40352));
#16239=EDGE_LOOP('',(#40353));
#16240=EDGE_LOOP('',(#40354));
#16241=EDGE_LOOP('',(#40355));
#16242=EDGE_LOOP('',(#40356));
#16243=EDGE_LOOP('',(#40357));
#16244=EDGE_LOOP('',(#40358));
#16245=EDGE_LOOP('',(#40359));
#16246=EDGE_LOOP('',(#40360));
#16247=EDGE_LOOP('',(#40361));
#16248=EDGE_LOOP('',(#40362));
#16249=EDGE_LOOP('',(#40363));
#16250=EDGE_LOOP('',(#40364));
#16251=EDGE_LOOP('',(#40365));
#16252=EDGE_LOOP('',(#40366));
#16253=EDGE_LOOP('',(#40367));
#16254=EDGE_LOOP('',(#40368));
#16255=EDGE_LOOP('',(#40369));
#16256=EDGE_LOOP('',(#40370));
#16257=EDGE_LOOP('',(#40371));
#16258=EDGE_LOOP('',(#40372));
#16259=EDGE_LOOP('',(#40373));
#16260=EDGE_LOOP('',(#40374));
#16261=EDGE_LOOP('',(#40375));
#16262=EDGE_LOOP('',(#40376));
#16263=EDGE_LOOP('',(#40377));
#16264=EDGE_LOOP('',(#40378));
#16265=EDGE_LOOP('',(#40379));
#16266=EDGE_LOOP('',(#40380));
#16267=EDGE_LOOP('',(#40381));
#16268=EDGE_LOOP('',(#40382));
#16269=EDGE_LOOP('',(#40383));
#16270=EDGE_LOOP('',(#40384));
#16271=EDGE_LOOP('',(#40385));
#16272=EDGE_LOOP('',(#40386));
#16273=EDGE_LOOP('',(#40387));
#16274=EDGE_LOOP('',(#40388));
#16275=EDGE_LOOP('',(#40389));
#16276=EDGE_LOOP('',(#40390));
#16277=EDGE_LOOP('',(#40391));
#16278=EDGE_LOOP('',(#40392));
#16279=EDGE_LOOP('',(#40393));
#16280=EDGE_LOOP('',(#40394));
#16281=EDGE_LOOP('',(#40395));
#16282=EDGE_LOOP('',(#40396));
#16283=EDGE_LOOP('',(#40397));
#16284=EDGE_LOOP('',(#40398));
#16285=EDGE_LOOP('',(#40399));
#16286=EDGE_LOOP('',(#40400));
#16287=EDGE_LOOP('',(#40401));
#16288=EDGE_LOOP('',(#40402));
#16289=EDGE_LOOP('',(#40403));
#16290=EDGE_LOOP('',(#40404));
#16291=EDGE_LOOP('',(#40405));
#16292=EDGE_LOOP('',(#40406));
#16293=EDGE_LOOP('',(#40407));
#16294=EDGE_LOOP('',(#40408));
#16295=EDGE_LOOP('',(#40409));
#16296=EDGE_LOOP('',(#40410));
#16297=EDGE_LOOP('',(#40411));
#16298=EDGE_LOOP('',(#40412));
#16299=EDGE_LOOP('',(#40413));
#16300=EDGE_LOOP('',(#40414));
#16301=EDGE_LOOP('',(#40415));
#16302=EDGE_LOOP('',(#40416));
#16303=EDGE_LOOP('',(#40417));
#16304=EDGE_LOOP('',(#40418));
#16305=EDGE_LOOP('',(#40419));
#16306=EDGE_LOOP('',(#40420));
#16307=EDGE_LOOP('',(#40421));
#16308=EDGE_LOOP('',(#40422));
#16309=EDGE_LOOP('',(#40423));
#16310=EDGE_LOOP('',(#40424));
#16311=EDGE_LOOP('',(#40425));
#16312=EDGE_LOOP('',(#40426));
#16313=EDGE_LOOP('',(#40427));
#16314=EDGE_LOOP('',(#40428));
#16315=EDGE_LOOP('',(#40429));
#16316=EDGE_LOOP('',(#40430));
#16317=EDGE_LOOP('',(#40431));
#16318=EDGE_LOOP('',(#40432));
#16319=EDGE_LOOP('',(#40433));
#16320=EDGE_LOOP('',(#40434));
#16321=EDGE_LOOP('',(#40435));
#16322=EDGE_LOOP('',(#40436));
#16323=EDGE_LOOP('',(#40437));
#16324=EDGE_LOOP('',(#40438));
#16325=EDGE_LOOP('',(#40439));
#16326=EDGE_LOOP('',(#40440));
#16327=EDGE_LOOP('',(#40441));
#16328=EDGE_LOOP('',(#40442));
#16329=EDGE_LOOP('',(#40443));
#16330=EDGE_LOOP('',(#40444));
#16331=EDGE_LOOP('',(#40445));
#16332=EDGE_LOOP('',(#40446));
#16333=EDGE_LOOP('',(#40447));
#16334=EDGE_LOOP('',(#40448));
#16335=EDGE_LOOP('',(#40449));
#16336=EDGE_LOOP('',(#40450));
#16337=EDGE_LOOP('',(#40451));
#16338=EDGE_LOOP('',(#40452));
#16339=EDGE_LOOP('',(#40453));
#16340=EDGE_LOOP('',(#40454));
#16341=EDGE_LOOP('',(#40455));
#16342=EDGE_LOOP('',(#40456));
#16343=EDGE_LOOP('',(#40457));
#16344=EDGE_LOOP('',(#40458));
#16345=EDGE_LOOP('',(#40459));
#16346=EDGE_LOOP('',(#40460));
#16347=EDGE_LOOP('',(#40461));
#16348=EDGE_LOOP('',(#40462));
#16349=EDGE_LOOP('',(#40463));
#16350=EDGE_LOOP('',(#40464));
#16351=EDGE_LOOP('',(#40465));
#16352=EDGE_LOOP('',(#40466));
#16353=EDGE_LOOP('',(#40467));
#16354=EDGE_LOOP('',(#40468));
#16355=EDGE_LOOP('',(#40469));
#16356=EDGE_LOOP('',(#40470));
#16357=EDGE_LOOP('',(#40471));
#16358=EDGE_LOOP('',(#40472));
#16359=EDGE_LOOP('',(#40473));
#16360=EDGE_LOOP('',(#40474));
#16361=EDGE_LOOP('',(#40475));
#16362=EDGE_LOOP('',(#40476));
#16363=EDGE_LOOP('',(#40477));
#16364=EDGE_LOOP('',(#40478));
#16365=EDGE_LOOP('',(#40479));
#16366=EDGE_LOOP('',(#40480));
#16367=EDGE_LOOP('',(#40481));
#16368=EDGE_LOOP('',(#40482));
#16369=EDGE_LOOP('',(#40483));
#16370=EDGE_LOOP('',(#40484));
#16371=EDGE_LOOP('',(#40485));
#16372=EDGE_LOOP('',(#40486));
#16373=EDGE_LOOP('',(#40487));
#16374=EDGE_LOOP('',(#40488));
#16375=EDGE_LOOP('',(#40489));
#16376=EDGE_LOOP('',(#40490));
#16377=EDGE_LOOP('',(#40491));
#16378=EDGE_LOOP('',(#40492));
#16379=EDGE_LOOP('',(#40493));
#16380=EDGE_LOOP('',(#40494));
#16381=EDGE_LOOP('',(#40495));
#16382=EDGE_LOOP('',(#40496));
#16383=EDGE_LOOP('',(#40497));
#16384=EDGE_LOOP('',(#40498));
#16385=EDGE_LOOP('',(#40499));
#16386=EDGE_LOOP('',(#40500));
#16387=EDGE_LOOP('',(#40501));
#16388=EDGE_LOOP('',(#40502));
#16389=EDGE_LOOP('',(#40503));
#16390=EDGE_LOOP('',(#40504));
#16391=EDGE_LOOP('',(#40505));
#16392=EDGE_LOOP('',(#40506));
#16393=EDGE_LOOP('',(#40507));
#16394=EDGE_LOOP('',(#40508));
#16395=EDGE_LOOP('',(#40509));
#16396=EDGE_LOOP('',(#40510));
#16397=EDGE_LOOP('',(#40511));
#16398=EDGE_LOOP('',(#40512));
#16399=EDGE_LOOP('',(#40513));
#16400=EDGE_LOOP('',(#40514));
#16401=EDGE_LOOP('',(#40515));
#16402=EDGE_LOOP('',(#40516));
#16403=EDGE_LOOP('',(#40517));
#16404=EDGE_LOOP('',(#40518));
#16405=EDGE_LOOP('',(#40519));
#16406=EDGE_LOOP('',(#40520));
#16407=EDGE_LOOP('',(#40521));
#16408=EDGE_LOOP('',(#40522));
#16409=EDGE_LOOP('',(#40523));
#16410=EDGE_LOOP('',(#40524));
#16411=EDGE_LOOP('',(#40525));
#16412=EDGE_LOOP('',(#40526));
#16413=EDGE_LOOP('',(#40527));
#16414=EDGE_LOOP('',(#40528));
#16415=EDGE_LOOP('',(#40529));
#16416=EDGE_LOOP('',(#40530));
#16417=EDGE_LOOP('',(#40531));
#16418=EDGE_LOOP('',(#40532));
#16419=EDGE_LOOP('',(#40533));
#16420=EDGE_LOOP('',(#40534));
#16421=EDGE_LOOP('',(#40535));
#16422=EDGE_LOOP('',(#40536));
#16423=EDGE_LOOP('',(#40537));
#16424=EDGE_LOOP('',(#40538));
#16425=EDGE_LOOP('',(#40539));
#16426=EDGE_LOOP('',(#40540));
#16427=EDGE_LOOP('',(#40541));
#16428=EDGE_LOOP('',(#40542));
#16429=EDGE_LOOP('',(#40543));
#16430=EDGE_LOOP('',(#40544));
#16431=EDGE_LOOP('',(#40545));
#16432=EDGE_LOOP('',(#40546));
#16433=EDGE_LOOP('',(#40547));
#16434=EDGE_LOOP('',(#40548));
#16435=EDGE_LOOP('',(#40549));
#16436=EDGE_LOOP('',(#40550));
#16437=EDGE_LOOP('',(#40551));
#16438=EDGE_LOOP('',(#40552));
#16439=EDGE_LOOP('',(#40553));
#16440=EDGE_LOOP('',(#40554));
#16441=EDGE_LOOP('',(#40555));
#16442=EDGE_LOOP('',(#40556));
#16443=EDGE_LOOP('',(#40557));
#16444=EDGE_LOOP('',(#40558));
#16445=EDGE_LOOP('',(#40559));
#16446=EDGE_LOOP('',(#40560));
#16447=EDGE_LOOP('',(#40561));
#16448=EDGE_LOOP('',(#40562));
#16449=EDGE_LOOP('',(#40563));
#16450=EDGE_LOOP('',(#40564));
#16451=EDGE_LOOP('',(#40565));
#16452=EDGE_LOOP('',(#40566));
#16453=EDGE_LOOP('',(#40567));
#16454=EDGE_LOOP('',(#40568));
#16455=EDGE_LOOP('',(#40569));
#16456=EDGE_LOOP('',(#40570));
#16457=EDGE_LOOP('',(#40571));
#16458=EDGE_LOOP('',(#40572));
#16459=EDGE_LOOP('',(#40573));
#16460=EDGE_LOOP('',(#40574));
#16461=EDGE_LOOP('',(#40575));
#16462=EDGE_LOOP('',(#40576));
#16463=EDGE_LOOP('',(#40577));
#16464=EDGE_LOOP('',(#40578));
#16465=EDGE_LOOP('',(#40579));
#16466=EDGE_LOOP('',(#40580));
#16467=EDGE_LOOP('',(#40581));
#16468=EDGE_LOOP('',(#40582));
#16469=EDGE_LOOP('',(#40583));
#16470=EDGE_LOOP('',(#40584));
#16471=EDGE_LOOP('',(#40585));
#16472=EDGE_LOOP('',(#40586));
#16473=EDGE_LOOP('',(#40587));
#16474=EDGE_LOOP('',(#40588));
#16475=EDGE_LOOP('',(#40589,#40590,#40591,#40592));
#16476=EDGE_LOOP('',(#40593));
#16477=EDGE_LOOP('',(#40594));
#16478=EDGE_LOOP('',(#40595));
#16479=EDGE_LOOP('',(#40596));
#16480=EDGE_LOOP('',(#40597));
#16481=EDGE_LOOP('',(#40598));
#16482=EDGE_LOOP('',(#40599));
#16483=EDGE_LOOP('',(#40600));
#16484=EDGE_LOOP('',(#40601));
#16485=EDGE_LOOP('',(#40602));
#16486=EDGE_LOOP('',(#40603));
#16487=EDGE_LOOP('',(#40604));
#16488=EDGE_LOOP('',(#40605));
#16489=EDGE_LOOP('',(#40606));
#16490=EDGE_LOOP('',(#40607));
#16491=EDGE_LOOP('',(#40608));
#16492=EDGE_LOOP('',(#40609));
#16493=EDGE_LOOP('',(#40610));
#16494=EDGE_LOOP('',(#40611));
#16495=EDGE_LOOP('',(#40612));
#16496=EDGE_LOOP('',(#40613));
#16497=EDGE_LOOP('',(#40614));
#16498=EDGE_LOOP('',(#40615));
#16499=EDGE_LOOP('',(#40616));
#16500=EDGE_LOOP('',(#40617));
#16501=EDGE_LOOP('',(#40618));
#16502=EDGE_LOOP('',(#40619));
#16503=EDGE_LOOP('',(#40620));
#16504=EDGE_LOOP('',(#40621));
#16505=EDGE_LOOP('',(#40622));
#16506=EDGE_LOOP('',(#40623));
#16507=EDGE_LOOP('',(#40624));
#16508=EDGE_LOOP('',(#40625));
#16509=EDGE_LOOP('',(#40626));
#16510=EDGE_LOOP('',(#40627));
#16511=EDGE_LOOP('',(#40628));
#16512=EDGE_LOOP('',(#40629));
#16513=EDGE_LOOP('',(#40630));
#16514=EDGE_LOOP('',(#40631));
#16515=EDGE_LOOP('',(#40632));
#16516=EDGE_LOOP('',(#40633));
#16517=EDGE_LOOP('',(#40634));
#16518=EDGE_LOOP('',(#40635));
#16519=EDGE_LOOP('',(#40636));
#16520=EDGE_LOOP('',(#40637,#40638));
#16521=EDGE_LOOP('',(#40639));
#16522=EDGE_LOOP('',(#40640));
#16523=EDGE_LOOP('',(#40641));
#16524=EDGE_LOOP('',(#40642));
#16525=EDGE_LOOP('',(#40643));
#16526=EDGE_LOOP('',(#40644));
#16527=EDGE_LOOP('',(#40645));
#16528=EDGE_LOOP('',(#40646));
#16529=EDGE_LOOP('',(#40647));
#16530=EDGE_LOOP('',(#40648));
#16531=EDGE_LOOP('',(#40649));
#16532=EDGE_LOOP('',(#40650));
#16533=EDGE_LOOP('',(#40651));
#16534=EDGE_LOOP('',(#40652));
#16535=EDGE_LOOP('',(#40653));
#16536=EDGE_LOOP('',(#40654));
#16537=EDGE_LOOP('',(#40655));
#16538=EDGE_LOOP('',(#40656));
#16539=EDGE_LOOP('',(#40657));
#16540=EDGE_LOOP('',(#40658));
#16541=EDGE_LOOP('',(#40659));
#16542=EDGE_LOOP('',(#40660));
#16543=EDGE_LOOP('',(#40661));
#16544=EDGE_LOOP('',(#40662));
#16545=EDGE_LOOP('',(#40663));
#16546=EDGE_LOOP('',(#40664));
#16547=EDGE_LOOP('',(#40665));
#16548=EDGE_LOOP('',(#40666));
#16549=EDGE_LOOP('',(#40667));
#16550=EDGE_LOOP('',(#40668));
#16551=EDGE_LOOP('',(#40669));
#16552=EDGE_LOOP('',(#40670));
#16553=EDGE_LOOP('',(#40671));
#16554=EDGE_LOOP('',(#40672));
#16555=EDGE_LOOP('',(#40673));
#16556=EDGE_LOOP('',(#40674));
#16557=EDGE_LOOP('',(#40675));
#16558=EDGE_LOOP('',(#40676));
#16559=EDGE_LOOP('',(#40677));
#16560=EDGE_LOOP('',(#40678));
#16561=EDGE_LOOP('',(#40679));
#16562=EDGE_LOOP('',(#40680));
#16563=EDGE_LOOP('',(#40681));
#16564=EDGE_LOOP('',(#40682));
#16565=EDGE_LOOP('',(#40683));
#16566=EDGE_LOOP('',(#40684));
#16567=EDGE_LOOP('',(#40685));
#16568=EDGE_LOOP('',(#40686));
#16569=EDGE_LOOP('',(#40687));
#16570=EDGE_LOOP('',(#40688));
#16571=EDGE_LOOP('',(#40689));
#16572=EDGE_LOOP('',(#40690));
#16573=EDGE_LOOP('',(#40691));
#16574=EDGE_LOOP('',(#40692));
#16575=EDGE_LOOP('',(#40693));
#16576=EDGE_LOOP('',(#40694));
#16577=EDGE_LOOP('',(#40695));
#16578=EDGE_LOOP('',(#40696));
#16579=EDGE_LOOP('',(#40697));
#16580=EDGE_LOOP('',(#40698));
#16581=EDGE_LOOP('',(#40699));
#16582=EDGE_LOOP('',(#40700));
#16583=EDGE_LOOP('',(#40701));
#16584=EDGE_LOOP('',(#40702));
#16585=EDGE_LOOP('',(#40703));
#16586=EDGE_LOOP('',(#40704));
#16587=EDGE_LOOP('',(#40705));
#16588=EDGE_LOOP('',(#40706));
#16589=EDGE_LOOP('',(#40707));
#16590=EDGE_LOOP('',(#40708));
#16591=EDGE_LOOP('',(#40709));
#16592=EDGE_LOOP('',(#40710));
#16593=EDGE_LOOP('',(#40711));
#16594=EDGE_LOOP('',(#40712));
#16595=EDGE_LOOP('',(#40713));
#16596=EDGE_LOOP('',(#40714));
#16597=EDGE_LOOP('',(#40715));
#16598=EDGE_LOOP('',(#40716));
#16599=EDGE_LOOP('',(#40717));
#16600=EDGE_LOOP('',(#40718));
#16601=EDGE_LOOP('',(#40719));
#16602=EDGE_LOOP('',(#40720));
#16603=EDGE_LOOP('',(#40721));
#16604=EDGE_LOOP('',(#40722));
#16605=EDGE_LOOP('',(#40723));
#16606=EDGE_LOOP('',(#40724));
#16607=EDGE_LOOP('',(#40725));
#16608=EDGE_LOOP('',(#40726));
#16609=EDGE_LOOP('',(#40727));
#16610=EDGE_LOOP('',(#40728));
#16611=EDGE_LOOP('',(#40729));
#16612=EDGE_LOOP('',(#40730));
#16613=EDGE_LOOP('',(#40731));
#16614=EDGE_LOOP('',(#40732));
#16615=EDGE_LOOP('',(#40733));
#16616=EDGE_LOOP('',(#40734));
#16617=EDGE_LOOP('',(#40735));
#16618=EDGE_LOOP('',(#40736));
#16619=EDGE_LOOP('',(#40737));
#16620=EDGE_LOOP('',(#40738));
#16621=EDGE_LOOP('',(#40739));
#16622=EDGE_LOOP('',(#40740));
#16623=EDGE_LOOP('',(#40741));
#16624=EDGE_LOOP('',(#40742));
#16625=EDGE_LOOP('',(#40743));
#16626=EDGE_LOOP('',(#40744));
#16627=EDGE_LOOP('',(#40745));
#16628=EDGE_LOOP('',(#40746));
#16629=EDGE_LOOP('',(#40747));
#16630=EDGE_LOOP('',(#40748));
#16631=EDGE_LOOP('',(#40749));
#16632=EDGE_LOOP('',(#40750));
#16633=EDGE_LOOP('',(#40751));
#16634=EDGE_LOOP('',(#40752));
#16635=EDGE_LOOP('',(#40753));
#16636=EDGE_LOOP('',(#40754));
#16637=EDGE_LOOP('',(#40755));
#16638=EDGE_LOOP('',(#40756));
#16639=EDGE_LOOP('',(#40757));
#16640=EDGE_LOOP('',(#40758));
#16641=EDGE_LOOP('',(#40759));
#16642=EDGE_LOOP('',(#40760));
#16643=EDGE_LOOP('',(#40761));
#16644=EDGE_LOOP('',(#40762));
#16645=EDGE_LOOP('',(#40763));
#16646=EDGE_LOOP('',(#40764));
#16647=EDGE_LOOP('',(#40765));
#16648=EDGE_LOOP('',(#40766));
#16649=EDGE_LOOP('',(#40767));
#16650=EDGE_LOOP('',(#40768));
#16651=EDGE_LOOP('',(#40769));
#16652=EDGE_LOOP('',(#40770));
#16653=EDGE_LOOP('',(#40771));
#16654=EDGE_LOOP('',(#40772));
#16655=EDGE_LOOP('',(#40773));
#16656=EDGE_LOOP('',(#40774));
#16657=EDGE_LOOP('',(#40775));
#16658=EDGE_LOOP('',(#40776));
#16659=EDGE_LOOP('',(#40777));
#16660=EDGE_LOOP('',(#40778));
#16661=EDGE_LOOP('',(#40779));
#16662=EDGE_LOOP('',(#40780));
#16663=EDGE_LOOP('',(#40781));
#16664=EDGE_LOOP('',(#40782));
#16665=EDGE_LOOP('',(#40783));
#16666=EDGE_LOOP('',(#40784));
#16667=EDGE_LOOP('',(#40785));
#16668=EDGE_LOOP('',(#40786));
#16669=EDGE_LOOP('',(#40787));
#16670=EDGE_LOOP('',(#40788));
#16671=EDGE_LOOP('',(#40789));
#16672=EDGE_LOOP('',(#40790));
#16673=EDGE_LOOP('',(#40791));
#16674=EDGE_LOOP('',(#40792));
#16675=EDGE_LOOP('',(#40793));
#16676=EDGE_LOOP('',(#40794));
#16677=EDGE_LOOP('',(#40795));
#16678=EDGE_LOOP('',(#40796));
#16679=EDGE_LOOP('',(#40797));
#16680=EDGE_LOOP('',(#40798));
#16681=EDGE_LOOP('',(#40799));
#16682=EDGE_LOOP('',(#40800));
#16683=EDGE_LOOP('',(#40801));
#16684=EDGE_LOOP('',(#40802));
#16685=EDGE_LOOP('',(#40803));
#16686=EDGE_LOOP('',(#40804));
#16687=EDGE_LOOP('',(#40805));
#16688=EDGE_LOOP('',(#40806));
#16689=EDGE_LOOP('',(#40807));
#16690=EDGE_LOOP('',(#40808));
#16691=EDGE_LOOP('',(#40809));
#16692=EDGE_LOOP('',(#40810));
#16693=EDGE_LOOP('',(#40811));
#16694=EDGE_LOOP('',(#40812));
#16695=EDGE_LOOP('',(#40813));
#16696=EDGE_LOOP('',(#40814));
#16697=EDGE_LOOP('',(#40815));
#16698=EDGE_LOOP('',(#40816));
#16699=EDGE_LOOP('',(#40817));
#16700=EDGE_LOOP('',(#40818));
#16701=EDGE_LOOP('',(#40819));
#16702=EDGE_LOOP('',(#40820));
#16703=EDGE_LOOP('',(#40821));
#16704=EDGE_LOOP('',(#40822));
#16705=EDGE_LOOP('',(#40823));
#16706=EDGE_LOOP('',(#40824));
#16707=EDGE_LOOP('',(#40825));
#16708=EDGE_LOOP('',(#40826));
#16709=EDGE_LOOP('',(#40827));
#16710=EDGE_LOOP('',(#40828));
#16711=EDGE_LOOP('',(#40829));
#16712=EDGE_LOOP('',(#40830));
#16713=EDGE_LOOP('',(#40831));
#16714=EDGE_LOOP('',(#40832));
#16715=EDGE_LOOP('',(#40833));
#16716=EDGE_LOOP('',(#40834));
#16717=EDGE_LOOP('',(#40835));
#16718=EDGE_LOOP('',(#40836));
#16719=EDGE_LOOP('',(#40837));
#16720=EDGE_LOOP('',(#40838));
#16721=EDGE_LOOP('',(#40839));
#16722=EDGE_LOOP('',(#40840));
#16723=EDGE_LOOP('',(#40841));
#16724=EDGE_LOOP('',(#40842));
#16725=EDGE_LOOP('',(#40843));
#16726=EDGE_LOOP('',(#40844));
#16727=EDGE_LOOP('',(#40845));
#16728=EDGE_LOOP('',(#40846));
#16729=EDGE_LOOP('',(#40847));
#16730=EDGE_LOOP('',(#40848));
#16731=EDGE_LOOP('',(#40849));
#16732=EDGE_LOOP('',(#40850));
#16733=EDGE_LOOP('',(#40851));
#16734=EDGE_LOOP('',(#40852));
#16735=EDGE_LOOP('',(#40853));
#16736=EDGE_LOOP('',(#40854));
#16737=EDGE_LOOP('',(#40855));
#16738=EDGE_LOOP('',(#40856));
#16739=EDGE_LOOP('',(#40857));
#16740=EDGE_LOOP('',(#40858));
#16741=EDGE_LOOP('',(#40859));
#16742=EDGE_LOOP('',(#40860));
#16743=EDGE_LOOP('',(#40861));
#16744=EDGE_LOOP('',(#40862));
#16745=EDGE_LOOP('',(#40863));
#16746=EDGE_LOOP('',(#40864));
#16747=EDGE_LOOP('',(#40865));
#16748=EDGE_LOOP('',(#40866));
#16749=EDGE_LOOP('',(#40867));
#16750=EDGE_LOOP('',(#40868));
#16751=EDGE_LOOP('',(#40869));
#16752=EDGE_LOOP('',(#40870));
#16753=EDGE_LOOP('',(#40871));
#16754=EDGE_LOOP('',(#40872));
#16755=EDGE_LOOP('',(#40873));
#16756=EDGE_LOOP('',(#40874));
#16757=EDGE_LOOP('',(#40875));
#16758=EDGE_LOOP('',(#40876));
#16759=EDGE_LOOP('',(#40877));
#16760=EDGE_LOOP('',(#40878));
#16761=EDGE_LOOP('',(#40879));
#16762=EDGE_LOOP('',(#40880));
#16763=EDGE_LOOP('',(#40881));
#16764=EDGE_LOOP('',(#40882));
#16765=EDGE_LOOP('',(#40883));
#16766=EDGE_LOOP('',(#40884));
#16767=EDGE_LOOP('',(#40885));
#16768=EDGE_LOOP('',(#40886));
#16769=EDGE_LOOP('',(#40887));
#16770=EDGE_LOOP('',(#40888));
#16771=EDGE_LOOP('',(#40889));
#16772=EDGE_LOOP('',(#40890));
#16773=EDGE_LOOP('',(#40891));
#16774=EDGE_LOOP('',(#40892));
#16775=EDGE_LOOP('',(#40893));
#16776=EDGE_LOOP('',(#40894));
#16777=EDGE_LOOP('',(#40895));
#16778=EDGE_LOOP('',(#40896));
#16779=EDGE_LOOP('',(#40897));
#16780=EDGE_LOOP('',(#40898));
#16781=EDGE_LOOP('',(#40899));
#16782=EDGE_LOOP('',(#40900));
#16783=EDGE_LOOP('',(#40901));
#16784=EDGE_LOOP('',(#40902));
#16785=EDGE_LOOP('',(#40903));
#16786=EDGE_LOOP('',(#40904));
#16787=EDGE_LOOP('',(#40905));
#16788=EDGE_LOOP('',(#40906));
#16789=EDGE_LOOP('',(#40907));
#16790=EDGE_LOOP('',(#40908));
#16791=EDGE_LOOP('',(#40909));
#16792=EDGE_LOOP('',(#40910));
#16793=EDGE_LOOP('',(#40911));
#16794=EDGE_LOOP('',(#40912));
#16795=EDGE_LOOP('',(#40913));
#16796=EDGE_LOOP('',(#40914));
#16797=EDGE_LOOP('',(#40915));
#16798=EDGE_LOOP('',(#40916));
#16799=EDGE_LOOP('',(#40917));
#16800=EDGE_LOOP('',(#40918));
#16801=EDGE_LOOP('',(#40919));
#16802=EDGE_LOOP('',(#40920));
#16803=EDGE_LOOP('',(#40921));
#16804=EDGE_LOOP('',(#40922));
#16805=EDGE_LOOP('',(#40923));
#16806=EDGE_LOOP('',(#40924));
#16807=EDGE_LOOP('',(#40925));
#16808=EDGE_LOOP('',(#40926));
#16809=EDGE_LOOP('',(#40927));
#16810=EDGE_LOOP('',(#40928));
#16811=EDGE_LOOP('',(#40929));
#16812=EDGE_LOOP('',(#40930));
#16813=EDGE_LOOP('',(#40931));
#16814=EDGE_LOOP('',(#40932));
#16815=EDGE_LOOP('',(#40933));
#16816=EDGE_LOOP('',(#40934));
#16817=EDGE_LOOP('',(#40935));
#16818=EDGE_LOOP('',(#40936));
#16819=EDGE_LOOP('',(#40937));
#16820=EDGE_LOOP('',(#40938));
#16821=EDGE_LOOP('',(#40939));
#16822=EDGE_LOOP('',(#40940));
#16823=EDGE_LOOP('',(#40941));
#16824=EDGE_LOOP('',(#40942));
#16825=EDGE_LOOP('',(#40943));
#16826=EDGE_LOOP('',(#40944));
#16827=EDGE_LOOP('',(#40945));
#16828=EDGE_LOOP('',(#40946));
#16829=EDGE_LOOP('',(#40947));
#16830=EDGE_LOOP('',(#40948));
#16831=EDGE_LOOP('',(#40949));
#16832=EDGE_LOOP('',(#40950));
#16833=EDGE_LOOP('',(#40951));
#16834=EDGE_LOOP('',(#40952));
#16835=EDGE_LOOP('',(#40953));
#16836=EDGE_LOOP('',(#40954));
#16837=EDGE_LOOP('',(#40955));
#16838=EDGE_LOOP('',(#40956));
#16839=EDGE_LOOP('',(#40957));
#16840=EDGE_LOOP('',(#40958));
#16841=EDGE_LOOP('',(#40959));
#16842=EDGE_LOOP('',(#40960));
#16843=EDGE_LOOP('',(#40961));
#16844=EDGE_LOOP('',(#40962));
#16845=EDGE_LOOP('',(#40963));
#16846=EDGE_LOOP('',(#40964));
#16847=EDGE_LOOP('',(#40965));
#16848=EDGE_LOOP('',(#40966));
#16849=EDGE_LOOP('',(#40967));
#16850=EDGE_LOOP('',(#40968));
#16851=EDGE_LOOP('',(#40969));
#16852=EDGE_LOOP('',(#40970));
#16853=EDGE_LOOP('',(#40971));
#16854=EDGE_LOOP('',(#40972));
#16855=EDGE_LOOP('',(#40973));
#16856=EDGE_LOOP('',(#40974));
#16857=EDGE_LOOP('',(#40975));
#16858=EDGE_LOOP('',(#40976));
#16859=EDGE_LOOP('',(#40977));
#16860=EDGE_LOOP('',(#40978));
#16861=EDGE_LOOP('',(#40979));
#16862=EDGE_LOOP('',(#40980));
#16863=EDGE_LOOP('',(#40981));
#16864=EDGE_LOOP('',(#40982));
#16865=EDGE_LOOP('',(#40983));
#16866=EDGE_LOOP('',(#40984));
#16867=EDGE_LOOP('',(#40985));
#16868=EDGE_LOOP('',(#40986));
#16869=EDGE_LOOP('',(#40987));
#16870=EDGE_LOOP('',(#40988));
#16871=EDGE_LOOP('',(#40989));
#16872=EDGE_LOOP('',(#40990));
#16873=EDGE_LOOP('',(#40991));
#16874=EDGE_LOOP('',(#40992));
#16875=EDGE_LOOP('',(#40993));
#16876=EDGE_LOOP('',(#40994));
#16877=EDGE_LOOP('',(#40995));
#16878=EDGE_LOOP('',(#40996));
#16879=EDGE_LOOP('',(#40997));
#16880=EDGE_LOOP('',(#40998));
#16881=EDGE_LOOP('',(#40999));
#16882=EDGE_LOOP('',(#41000));
#16883=EDGE_LOOP('',(#41001));
#16884=EDGE_LOOP('',(#41002));
#16885=EDGE_LOOP('',(#41003));
#16886=EDGE_LOOP('',(#41004));
#16887=EDGE_LOOP('',(#41005));
#16888=EDGE_LOOP('',(#41006));
#16889=EDGE_LOOP('',(#41007));
#16890=EDGE_LOOP('',(#41008));
#16891=EDGE_LOOP('',(#41009));
#16892=EDGE_LOOP('',(#41010));
#16893=EDGE_LOOP('',(#41011));
#16894=EDGE_LOOP('',(#41012));
#16895=EDGE_LOOP('',(#41013));
#16896=EDGE_LOOP('',(#41014));
#16897=EDGE_LOOP('',(#41015));
#16898=EDGE_LOOP('',(#41016));
#16899=EDGE_LOOP('',(#41017));
#16900=EDGE_LOOP('',(#41018));
#16901=EDGE_LOOP('',(#41019));
#16902=EDGE_LOOP('',(#41020));
#16903=EDGE_LOOP('',(#41021));
#16904=EDGE_LOOP('',(#41022));
#16905=EDGE_LOOP('',(#41023));
#16906=EDGE_LOOP('',(#41024));
#16907=EDGE_LOOP('',(#41025));
#16908=EDGE_LOOP('',(#41026));
#16909=EDGE_LOOP('',(#41027));
#16910=EDGE_LOOP('',(#41028));
#16911=EDGE_LOOP('',(#41029));
#16912=EDGE_LOOP('',(#41030));
#16913=EDGE_LOOP('',(#41031));
#16914=EDGE_LOOP('',(#41032));
#16915=EDGE_LOOP('',(#41033));
#16916=EDGE_LOOP('',(#41034));
#16917=EDGE_LOOP('',(#41035));
#16918=EDGE_LOOP('',(#41036));
#16919=EDGE_LOOP('',(#41037));
#16920=EDGE_LOOP('',(#41038));
#16921=EDGE_LOOP('',(#41039));
#16922=EDGE_LOOP('',(#41040));
#16923=EDGE_LOOP('',(#41041));
#16924=EDGE_LOOP('',(#41042));
#16925=EDGE_LOOP('',(#41043));
#16926=EDGE_LOOP('',(#41044));
#16927=EDGE_LOOP('',(#41045));
#16928=EDGE_LOOP('',(#41046));
#16929=EDGE_LOOP('',(#41047));
#16930=EDGE_LOOP('',(#41048));
#16931=EDGE_LOOP('',(#41049));
#16932=EDGE_LOOP('',(#41050));
#16933=EDGE_LOOP('',(#41051));
#16934=EDGE_LOOP('',(#41052));
#16935=EDGE_LOOP('',(#41053));
#16936=EDGE_LOOP('',(#41054));
#16937=EDGE_LOOP('',(#41055));
#16938=EDGE_LOOP('',(#41056));
#16939=EDGE_LOOP('',(#41057));
#16940=EDGE_LOOP('',(#41058));
#16941=EDGE_LOOP('',(#41059));
#16942=EDGE_LOOP('',(#41060));
#16943=EDGE_LOOP('',(#41061));
#16944=EDGE_LOOP('',(#41062));
#16945=EDGE_LOOP('',(#41063));
#16946=EDGE_LOOP('',(#41064));
#16947=EDGE_LOOP('',(#41065));
#16948=EDGE_LOOP('',(#41066));
#16949=EDGE_LOOP('',(#41067));
#16950=EDGE_LOOP('',(#41068));
#16951=EDGE_LOOP('',(#41069));
#16952=EDGE_LOOP('',(#41070));
#16953=EDGE_LOOP('',(#41071));
#16954=EDGE_LOOP('',(#41072));
#16955=EDGE_LOOP('',(#41073));
#16956=EDGE_LOOP('',(#41074));
#16957=EDGE_LOOP('',(#41075));
#16958=EDGE_LOOP('',(#41076));
#16959=EDGE_LOOP('',(#41077));
#16960=EDGE_LOOP('',(#41078));
#16961=EDGE_LOOP('',(#41079));
#16962=EDGE_LOOP('',(#41080));
#16963=EDGE_LOOP('',(#41081));
#16964=EDGE_LOOP('',(#41082));
#16965=EDGE_LOOP('',(#41083));
#16966=EDGE_LOOP('',(#41084));
#16967=EDGE_LOOP('',(#41085));
#16968=EDGE_LOOP('',(#41086));
#16969=EDGE_LOOP('',(#41087));
#16970=EDGE_LOOP('',(#41088));
#16971=EDGE_LOOP('',(#41089));
#16972=EDGE_LOOP('',(#41090));
#16973=EDGE_LOOP('',(#41091));
#16974=EDGE_LOOP('',(#41092));
#16975=EDGE_LOOP('',(#41093));
#16976=EDGE_LOOP('',(#41094));
#16977=EDGE_LOOP('',(#41095));
#16978=EDGE_LOOP('',(#41096));
#16979=EDGE_LOOP('',(#41097));
#16980=EDGE_LOOP('',(#41098));
#16981=EDGE_LOOP('',(#41099));
#16982=EDGE_LOOP('',(#41100));
#16983=EDGE_LOOP('',(#41101));
#16984=EDGE_LOOP('',(#41102));
#16985=EDGE_LOOP('',(#41103));
#16986=EDGE_LOOP('',(#41104));
#16987=EDGE_LOOP('',(#41105));
#16988=EDGE_LOOP('',(#41106));
#16989=EDGE_LOOP('',(#41107));
#16990=EDGE_LOOP('',(#41108));
#16991=EDGE_LOOP('',(#41109));
#16992=EDGE_LOOP('',(#41110));
#16993=EDGE_LOOP('',(#41111));
#16994=EDGE_LOOP('',(#41112));
#16995=EDGE_LOOP('',(#41113));
#16996=EDGE_LOOP('',(#41114));
#16997=EDGE_LOOP('',(#41115));
#16998=EDGE_LOOP('',(#41116));
#16999=EDGE_LOOP('',(#41117));
#17000=EDGE_LOOP('',(#41118));
#17001=EDGE_LOOP('',(#41119));
#17002=EDGE_LOOP('',(#41120));
#17003=EDGE_LOOP('',(#41121));
#17004=EDGE_LOOP('',(#41122));
#17005=EDGE_LOOP('',(#41123));
#17006=EDGE_LOOP('',(#41124));
#17007=EDGE_LOOP('',(#41125));
#17008=EDGE_LOOP('',(#41126));
#17009=EDGE_LOOP('',(#41127));
#17010=EDGE_LOOP('',(#41128));
#17011=EDGE_LOOP('',(#41129));
#17012=EDGE_LOOP('',(#41130));
#17013=EDGE_LOOP('',(#41131));
#17014=EDGE_LOOP('',(#41132));
#17015=EDGE_LOOP('',(#41133));
#17016=EDGE_LOOP('',(#41134));
#17017=EDGE_LOOP('',(#41135));
#17018=EDGE_LOOP('',(#41136));
#17019=EDGE_LOOP('',(#41137));
#17020=EDGE_LOOP('',(#41138));
#17021=EDGE_LOOP('',(#41139));
#17022=EDGE_LOOP('',(#41140));
#17023=EDGE_LOOP('',(#41141));
#17024=EDGE_LOOP('',(#41142));
#17025=EDGE_LOOP('',(#41143));
#17026=EDGE_LOOP('',(#41144));
#17027=EDGE_LOOP('',(#41145));
#17028=EDGE_LOOP('',(#41146));
#17029=EDGE_LOOP('',(#41147));
#17030=EDGE_LOOP('',(#41148));
#17031=EDGE_LOOP('',(#41149));
#17032=EDGE_LOOP('',(#41150));
#17033=EDGE_LOOP('',(#41151));
#17034=EDGE_LOOP('',(#41152));
#17035=EDGE_LOOP('',(#41153));
#17036=EDGE_LOOP('',(#41154));
#17037=EDGE_LOOP('',(#41155));
#17038=EDGE_LOOP('',(#41156));
#17039=EDGE_LOOP('',(#41157));
#17040=EDGE_LOOP('',(#41158));
#17041=EDGE_LOOP('',(#41159));
#17042=EDGE_LOOP('',(#41160));
#17043=EDGE_LOOP('',(#41161));
#17044=EDGE_LOOP('',(#41162));
#17045=EDGE_LOOP('',(#41163));
#17046=EDGE_LOOP('',(#41164));
#17047=EDGE_LOOP('',(#41165));
#17048=EDGE_LOOP('',(#41166));
#17049=EDGE_LOOP('',(#41167));
#17050=EDGE_LOOP('',(#41168));
#17051=EDGE_LOOP('',(#41169));
#17052=EDGE_LOOP('',(#41170));
#17053=EDGE_LOOP('',(#41171));
#17054=EDGE_LOOP('',(#41172));
#17055=EDGE_LOOP('',(#41173));
#17056=EDGE_LOOP('',(#41174));
#17057=EDGE_LOOP('',(#41175));
#17058=EDGE_LOOP('',(#41176));
#17059=EDGE_LOOP('',(#41177));
#17060=EDGE_LOOP('',(#41178));
#17061=EDGE_LOOP('',(#41179));
#17062=EDGE_LOOP('',(#41180));
#17063=EDGE_LOOP('',(#41181));
#17064=EDGE_LOOP('',(#41182));
#17065=EDGE_LOOP('',(#41183));
#17066=EDGE_LOOP('',(#41184));
#17067=EDGE_LOOP('',(#41185));
#17068=EDGE_LOOP('',(#41186));
#17069=EDGE_LOOP('',(#41187));
#17070=EDGE_LOOP('',(#41188));
#17071=EDGE_LOOP('',(#41189));
#17072=EDGE_LOOP('',(#41190));
#17073=EDGE_LOOP('',(#41191));
#17074=EDGE_LOOP('',(#41192));
#17075=EDGE_LOOP('',(#41193));
#17076=EDGE_LOOP('',(#41194));
#17077=EDGE_LOOP('',(#41195));
#17078=EDGE_LOOP('',(#41196));
#17079=EDGE_LOOP('',(#41197));
#17080=EDGE_LOOP('',(#41198));
#17081=EDGE_LOOP('',(#41199));
#17082=EDGE_LOOP('',(#41200));
#17083=EDGE_LOOP('',(#41201));
#17084=EDGE_LOOP('',(#41202));
#17085=EDGE_LOOP('',(#41203));
#17086=EDGE_LOOP('',(#41204));
#17087=EDGE_LOOP('',(#41205));
#17088=EDGE_LOOP('',(#41206));
#17089=EDGE_LOOP('',(#41207));
#17090=EDGE_LOOP('',(#41208));
#17091=EDGE_LOOP('',(#41209));
#17092=EDGE_LOOP('',(#41210));
#17093=EDGE_LOOP('',(#41211));
#17094=EDGE_LOOP('',(#41212));
#17095=EDGE_LOOP('',(#41213));
#17096=EDGE_LOOP('',(#41214));
#17097=EDGE_LOOP('',(#41215));
#17098=EDGE_LOOP('',(#41216));
#17099=EDGE_LOOP('',(#41217));
#17100=EDGE_LOOP('',(#41218));
#17101=EDGE_LOOP('',(#41219));
#17102=EDGE_LOOP('',(#41220));
#17103=EDGE_LOOP('',(#41221));
#17104=EDGE_LOOP('',(#41222));
#17105=EDGE_LOOP('',(#41223));
#17106=EDGE_LOOP('',(#41224));
#17107=EDGE_LOOP('',(#41225));
#17108=EDGE_LOOP('',(#41226));
#17109=EDGE_LOOP('',(#41227));
#17110=EDGE_LOOP('',(#41228));
#17111=EDGE_LOOP('',(#41229));
#17112=EDGE_LOOP('',(#41230));
#17113=EDGE_LOOP('',(#41231));
#17114=EDGE_LOOP('',(#41232));
#17115=EDGE_LOOP('',(#41233));
#17116=EDGE_LOOP('',(#41234));
#17117=EDGE_LOOP('',(#41235));
#17118=EDGE_LOOP('',(#41236));
#17119=EDGE_LOOP('',(#41237));
#17120=EDGE_LOOP('',(#41238));
#17121=EDGE_LOOP('',(#41239));
#17122=EDGE_LOOP('',(#41240));
#17123=EDGE_LOOP('',(#41241));
#17124=EDGE_LOOP('',(#41242));
#17125=EDGE_LOOP('',(#41243));
#17126=EDGE_LOOP('',(#41244));
#17127=EDGE_LOOP('',(#41245));
#17128=EDGE_LOOP('',(#41246));
#17129=EDGE_LOOP('',(#41247));
#17130=EDGE_LOOP('',(#41248));
#17131=EDGE_LOOP('',(#41249));
#17132=EDGE_LOOP('',(#41250));
#17133=EDGE_LOOP('',(#41251));
#17134=EDGE_LOOP('',(#41252));
#17135=EDGE_LOOP('',(#41253));
#17136=EDGE_LOOP('',(#41254));
#17137=EDGE_LOOP('',(#41255));
#17138=EDGE_LOOP('',(#41256));
#17139=EDGE_LOOP('',(#41257));
#17140=EDGE_LOOP('',(#41258));
#17141=EDGE_LOOP('',(#41259));
#17142=EDGE_LOOP('',(#41260));
#17143=EDGE_LOOP('',(#41261));
#17144=EDGE_LOOP('',(#41262));
#17145=EDGE_LOOP('',(#41263));
#17146=EDGE_LOOP('',(#41264));
#17147=EDGE_LOOP('',(#41265));
#17148=EDGE_LOOP('',(#41266));
#17149=EDGE_LOOP('',(#41267));
#17150=EDGE_LOOP('',(#41268));
#17151=EDGE_LOOP('',(#41269));
#17152=EDGE_LOOP('',(#41270));
#17153=EDGE_LOOP('',(#41271));
#17154=EDGE_LOOP('',(#41272));
#17155=EDGE_LOOP('',(#41273));
#17156=EDGE_LOOP('',(#41274));
#17157=EDGE_LOOP('',(#41275));
#17158=EDGE_LOOP('',(#41276));
#17159=EDGE_LOOP('',(#41277));
#17160=EDGE_LOOP('',(#41278));
#17161=EDGE_LOOP('',(#41279));
#17162=EDGE_LOOP('',(#41280));
#17163=EDGE_LOOP('',(#41281));
#17164=EDGE_LOOP('',(#41282));
#17165=EDGE_LOOP('',(#41283));
#17166=EDGE_LOOP('',(#41284));
#17167=EDGE_LOOP('',(#41285));
#17168=EDGE_LOOP('',(#41286));
#17169=EDGE_LOOP('',(#41287));
#17170=EDGE_LOOP('',(#41288));
#17171=EDGE_LOOP('',(#41289));
#17172=EDGE_LOOP('',(#41290));
#17173=EDGE_LOOP('',(#41291));
#17174=EDGE_LOOP('',(#41292));
#17175=EDGE_LOOP('',(#41293));
#17176=EDGE_LOOP('',(#41294));
#17177=EDGE_LOOP('',(#41295));
#17178=EDGE_LOOP('',(#41296));
#17179=EDGE_LOOP('',(#41297));
#17180=EDGE_LOOP('',(#41298));
#17181=EDGE_LOOP('',(#41299));
#17182=EDGE_LOOP('',(#41300));
#17183=EDGE_LOOP('',(#41301));
#17184=EDGE_LOOP('',(#41302));
#17185=EDGE_LOOP('',(#41303));
#17186=EDGE_LOOP('',(#41304));
#17187=EDGE_LOOP('',(#41305));
#17188=EDGE_LOOP('',(#41306));
#17189=EDGE_LOOP('',(#41307));
#17190=EDGE_LOOP('',(#41308));
#17191=EDGE_LOOP('',(#41309));
#17192=EDGE_LOOP('',(#41310));
#17193=EDGE_LOOP('',(#41311));
#17194=EDGE_LOOP('',(#41312));
#17195=EDGE_LOOP('',(#41313));
#17196=EDGE_LOOP('',(#41314));
#17197=EDGE_LOOP('',(#41315));
#17198=EDGE_LOOP('',(#41316));
#17199=EDGE_LOOP('',(#41317));
#17200=EDGE_LOOP('',(#41318));
#17201=EDGE_LOOP('',(#41319));
#17202=EDGE_LOOP('',(#41320));
#17203=EDGE_LOOP('',(#41321));
#17204=EDGE_LOOP('',(#41322));
#17205=EDGE_LOOP('',(#41323));
#17206=EDGE_LOOP('',(#41324));
#17207=EDGE_LOOP('',(#41325));
#17208=EDGE_LOOP('',(#41326));
#17209=EDGE_LOOP('',(#41327));
#17210=EDGE_LOOP('',(#41328));
#17211=EDGE_LOOP('',(#41329));
#17212=EDGE_LOOP('',(#41330));
#17213=EDGE_LOOP('',(#41331));
#17214=EDGE_LOOP('',(#41332));
#17215=EDGE_LOOP('',(#41333));
#17216=EDGE_LOOP('',(#41334));
#17217=EDGE_LOOP('',(#41335));
#17218=EDGE_LOOP('',(#41336));
#17219=EDGE_LOOP('',(#41337));
#17220=EDGE_LOOP('',(#41338));
#17221=EDGE_LOOP('',(#41339));
#17222=EDGE_LOOP('',(#41340));
#17223=EDGE_LOOP('',(#41341));
#17224=EDGE_LOOP('',(#41342));
#17225=EDGE_LOOP('',(#41343));
#17226=EDGE_LOOP('',(#41344));
#17227=EDGE_LOOP('',(#41345));
#17228=EDGE_LOOP('',(#41346));
#17229=EDGE_LOOP('',(#41347));
#17230=EDGE_LOOP('',(#41348));
#17231=EDGE_LOOP('',(#41349));
#17232=EDGE_LOOP('',(#41350));
#17233=EDGE_LOOP('',(#41351));
#17234=EDGE_LOOP('',(#41352));
#17235=EDGE_LOOP('',(#41353));
#17236=EDGE_LOOP('',(#41354));
#17237=EDGE_LOOP('',(#41355));
#17238=EDGE_LOOP('',(#41356));
#17239=EDGE_LOOP('',(#41357));
#17240=EDGE_LOOP('',(#41358));
#17241=EDGE_LOOP('',(#41359));
#17242=EDGE_LOOP('',(#41360));
#17243=EDGE_LOOP('',(#41361));
#17244=EDGE_LOOP('',(#41362));
#17245=EDGE_LOOP('',(#41363));
#17246=EDGE_LOOP('',(#41364));
#17247=EDGE_LOOP('',(#41365));
#17248=EDGE_LOOP('',(#41366));
#17249=EDGE_LOOP('',(#41367));
#17250=EDGE_LOOP('',(#41368));
#17251=EDGE_LOOP('',(#41369));
#17252=EDGE_LOOP('',(#41370));
#17253=EDGE_LOOP('',(#41371));
#17254=EDGE_LOOP('',(#41372));
#17255=EDGE_LOOP('',(#41373));
#17256=EDGE_LOOP('',(#41374));
#17257=EDGE_LOOP('',(#41375));
#17258=EDGE_LOOP('',(#41376));
#17259=EDGE_LOOP('',(#41377));
#17260=EDGE_LOOP('',(#41378));
#17261=EDGE_LOOP('',(#41379));
#17262=EDGE_LOOP('',(#41380));
#17263=EDGE_LOOP('',(#41381));
#17264=EDGE_LOOP('',(#41382));
#17265=EDGE_LOOP('',(#41383));
#17266=EDGE_LOOP('',(#41384));
#17267=EDGE_LOOP('',(#41385));
#17268=EDGE_LOOP('',(#41386));
#17269=EDGE_LOOP('',(#41387));
#17270=EDGE_LOOP('',(#41388));
#17271=EDGE_LOOP('',(#41389));
#17272=EDGE_LOOP('',(#41390));
#17273=EDGE_LOOP('',(#41391));
#17274=EDGE_LOOP('',(#41392));
#17275=EDGE_LOOP('',(#41393));
#17276=EDGE_LOOP('',(#41394));
#17277=EDGE_LOOP('',(#41395));
#17278=EDGE_LOOP('',(#41396));
#17279=EDGE_LOOP('',(#41397));
#17280=EDGE_LOOP('',(#41398));
#17281=EDGE_LOOP('',(#41399));
#17282=EDGE_LOOP('',(#41400));
#17283=EDGE_LOOP('',(#41401));
#17284=EDGE_LOOP('',(#41402));
#17285=EDGE_LOOP('',(#41403));
#17286=EDGE_LOOP('',(#41404));
#17287=EDGE_LOOP('',(#41405));
#17288=EDGE_LOOP('',(#41406));
#17289=EDGE_LOOP('',(#41407));
#17290=EDGE_LOOP('',(#41408));
#17291=EDGE_LOOP('',(#41409));
#17292=EDGE_LOOP('',(#41410));
#17293=EDGE_LOOP('',(#41411));
#17294=EDGE_LOOP('',(#41412));
#17295=EDGE_LOOP('',(#41413));
#17296=EDGE_LOOP('',(#41414));
#17297=EDGE_LOOP('',(#41415));
#17298=EDGE_LOOP('',(#41416));
#17299=EDGE_LOOP('',(#41417));
#17300=EDGE_LOOP('',(#41418));
#17301=EDGE_LOOP('',(#41419));
#17302=EDGE_LOOP('',(#41420));
#17303=EDGE_LOOP('',(#41421));
#17304=EDGE_LOOP('',(#41422));
#17305=EDGE_LOOP('',(#41423));
#17306=EDGE_LOOP('',(#41424));
#17307=EDGE_LOOP('',(#41425));
#17308=EDGE_LOOP('',(#41426));
#17309=EDGE_LOOP('',(#41427));
#17310=EDGE_LOOP('',(#41428));
#17311=EDGE_LOOP('',(#41429));
#17312=EDGE_LOOP('',(#41430));
#17313=EDGE_LOOP('',(#41431));
#17314=EDGE_LOOP('',(#41432));
#17315=EDGE_LOOP('',(#41433));
#17316=EDGE_LOOP('',(#41434));
#17317=EDGE_LOOP('',(#41435));
#17318=EDGE_LOOP('',(#41436));
#17319=EDGE_LOOP('',(#41437));
#17320=EDGE_LOOP('',(#41438));
#17321=EDGE_LOOP('',(#41439));
#17322=EDGE_LOOP('',(#41440));
#17323=EDGE_LOOP('',(#41441));
#17324=EDGE_LOOP('',(#41442));
#17325=EDGE_LOOP('',(#41443));
#17326=EDGE_LOOP('',(#41444));
#17327=EDGE_LOOP('',(#41445));
#17328=EDGE_LOOP('',(#41446));
#17329=EDGE_LOOP('',(#41447));
#17330=EDGE_LOOP('',(#41448));
#17331=EDGE_LOOP('',(#41449));
#17332=EDGE_LOOP('',(#41450));
#17333=EDGE_LOOP('',(#41451));
#17334=EDGE_LOOP('',(#41452));
#17335=EDGE_LOOP('',(#41453));
#17336=EDGE_LOOP('',(#41454));
#17337=EDGE_LOOP('',(#41455));
#17338=EDGE_LOOP('',(#41456));
#17339=EDGE_LOOP('',(#41457));
#17340=EDGE_LOOP('',(#41458));
#17341=EDGE_LOOP('',(#41459));
#17342=EDGE_LOOP('',(#41460));
#17343=EDGE_LOOP('',(#41461));
#17344=EDGE_LOOP('',(#41462));
#17345=EDGE_LOOP('',(#41463));
#17346=EDGE_LOOP('',(#41464));
#17347=EDGE_LOOP('',(#41465));
#17348=EDGE_LOOP('',(#41466,#41467));
#17349=EDGE_LOOP('',(#41468));
#17350=EDGE_LOOP('',(#41469));
#17351=EDGE_LOOP('',(#41470,#41471));
#17352=EDGE_LOOP('',(#41472));
#17353=EDGE_LOOP('',(#41473));
#17354=EDGE_LOOP('',(#41474,#41475));
#17355=EDGE_LOOP('',(#41476));
#17356=EDGE_LOOP('',(#41477));
#17357=EDGE_LOOP('',(#41478,#41479));
#17358=EDGE_LOOP('',(#41480));
#17359=EDGE_LOOP('',(#41481));
#17360=EDGE_LOOP('',(#41482,#41483));
#17361=EDGE_LOOP('',(#41484));
#17362=EDGE_LOOP('',(#41485));
#17363=EDGE_LOOP('',(#41486,#41487));
#17364=EDGE_LOOP('',(#41488));
#17365=EDGE_LOOP('',(#41489));
#17366=EDGE_LOOP('',(#41490,#41491));
#17367=EDGE_LOOP('',(#41492));
#17368=EDGE_LOOP('',(#41493));
#17369=EDGE_LOOP('',(#41494,#41495));
#17370=EDGE_LOOP('',(#41496));
#17371=EDGE_LOOP('',(#41497));
#17372=EDGE_LOOP('',(#41498,#41499));
#17373=EDGE_LOOP('',(#41500));
#17374=EDGE_LOOP('',(#41501));
#17375=EDGE_LOOP('',(#41502,#41503));
#17376=EDGE_LOOP('',(#41504));
#17377=EDGE_LOOP('',(#41505));
#17378=EDGE_LOOP('',(#41506,#41507));
#17379=EDGE_LOOP('',(#41508));
#17380=EDGE_LOOP('',(#41509));
#17381=EDGE_LOOP('',(#41510,#41511));
#17382=EDGE_LOOP('',(#41512));
#17383=EDGE_LOOP('',(#41513));
#17384=EDGE_LOOP('',(#41514,#41515));
#17385=EDGE_LOOP('',(#41516));
#17386=EDGE_LOOP('',(#41517));
#17387=EDGE_LOOP('',(#41518,#41519));
#17388=EDGE_LOOP('',(#41520));
#17389=EDGE_LOOP('',(#41521));
#17390=EDGE_LOOP('',(#41522,#41523));
#17391=EDGE_LOOP('',(#41524));
#17392=EDGE_LOOP('',(#41525));
#17393=EDGE_LOOP('',(#41526,#41527));
#17394=EDGE_LOOP('',(#41528));
#17395=EDGE_LOOP('',(#41529));
#17396=EDGE_LOOP('',(#41530,#41531));
#17397=EDGE_LOOP('',(#41532));
#17398=EDGE_LOOP('',(#41533));
#17399=EDGE_LOOP('',(#41534,#41535));
#17400=EDGE_LOOP('',(#41536));
#17401=EDGE_LOOP('',(#41537));
#17402=EDGE_LOOP('',(#41538,#41539));
#17403=EDGE_LOOP('',(#41540));
#17404=EDGE_LOOP('',(#41541));
#17405=EDGE_LOOP('',(#41542,#41543));
#17406=EDGE_LOOP('',(#41544));
#17407=EDGE_LOOP('',(#41545));
#17408=EDGE_LOOP('',(#41546,#41547));
#17409=EDGE_LOOP('',(#41548));
#17410=EDGE_LOOP('',(#41549));
#17411=EDGE_LOOP('',(#41550,#41551));
#17412=EDGE_LOOP('',(#41552));
#17413=EDGE_LOOP('',(#41553));
#17414=EDGE_LOOP('',(#41554,#41555));
#17415=EDGE_LOOP('',(#41556));
#17416=EDGE_LOOP('',(#41557));
#17417=EDGE_LOOP('',(#41558,#41559));
#17418=EDGE_LOOP('',(#41560));
#17419=EDGE_LOOP('',(#41561));
#17420=EDGE_LOOP('',(#41562,#41563));
#17421=EDGE_LOOP('',(#41564));
#17422=EDGE_LOOP('',(#41565));
#17423=EDGE_LOOP('',(#41566,#41567));
#17424=EDGE_LOOP('',(#41568));
#17425=EDGE_LOOP('',(#41569));
#17426=EDGE_LOOP('',(#41570,#41571));
#17427=EDGE_LOOP('',(#41572));
#17428=EDGE_LOOP('',(#41573));
#17429=EDGE_LOOP('',(#41574,#41575));
#17430=EDGE_LOOP('',(#41576));
#17431=EDGE_LOOP('',(#41577));
#17432=EDGE_LOOP('',(#41578,#41579));
#17433=EDGE_LOOP('',(#41580));
#17434=EDGE_LOOP('',(#41581));
#17435=EDGE_LOOP('',(#41582,#41583));
#17436=EDGE_LOOP('',(#41584));
#17437=EDGE_LOOP('',(#41585));
#17438=EDGE_LOOP('',(#41586,#41587));
#17439=EDGE_LOOP('',(#41588));
#17440=EDGE_LOOP('',(#41589));
#17441=EDGE_LOOP('',(#41590,#41591));
#17442=EDGE_LOOP('',(#41592));
#17443=EDGE_LOOP('',(#41593));
#17444=EDGE_LOOP('',(#41594,#41595));
#17445=EDGE_LOOP('',(#41596));
#17446=EDGE_LOOP('',(#41597));
#17447=EDGE_LOOP('',(#41598,#41599));
#17448=EDGE_LOOP('',(#41600));
#17449=EDGE_LOOP('',(#41601));
#17450=EDGE_LOOP('',(#41602,#41603));
#17451=EDGE_LOOP('',(#41604));
#17452=EDGE_LOOP('',(#41605));
#17453=EDGE_LOOP('',(#41606,#41607));
#17454=EDGE_LOOP('',(#41608));
#17455=EDGE_LOOP('',(#41609));
#17456=EDGE_LOOP('',(#41610,#41611));
#17457=EDGE_LOOP('',(#41612));
#17458=EDGE_LOOP('',(#41613));
#17459=EDGE_LOOP('',(#41614,#41615));
#17460=EDGE_LOOP('',(#41616));
#17461=EDGE_LOOP('',(#41617));
#17462=EDGE_LOOP('',(#41618,#41619));
#17463=EDGE_LOOP('',(#41620));
#17464=EDGE_LOOP('',(#41621));
#17465=EDGE_LOOP('',(#41622,#41623));
#17466=EDGE_LOOP('',(#41624));
#17467=EDGE_LOOP('',(#41625));
#17468=EDGE_LOOP('',(#41626,#41627));
#17469=EDGE_LOOP('',(#41628));
#17470=EDGE_LOOP('',(#41629));
#17471=EDGE_LOOP('',(#41630,#41631));
#17472=EDGE_LOOP('',(#41632));
#17473=EDGE_LOOP('',(#41633));
#17474=EDGE_LOOP('',(#41634,#41635));
#17475=EDGE_LOOP('',(#41636));
#17476=EDGE_LOOP('',(#41637));
#17477=EDGE_LOOP('',(#41638,#41639));
#17478=EDGE_LOOP('',(#41640));
#17479=EDGE_LOOP('',(#41641));
#17480=EDGE_LOOP('',(#41642,#41643));
#17481=EDGE_LOOP('',(#41644));
#17482=EDGE_LOOP('',(#41645));
#17483=EDGE_LOOP('',(#41646,#41647));
#17484=EDGE_LOOP('',(#41648));
#17485=EDGE_LOOP('',(#41649));
#17486=EDGE_LOOP('',(#41650,#41651));
#17487=EDGE_LOOP('',(#41652));
#17488=EDGE_LOOP('',(#41653,#41654));
#17489=EDGE_LOOP('',(#41655,#41656));
#17490=EDGE_LOOP('',(#41657));
#17491=EDGE_LOOP('',(#41658));
#17492=EDGE_LOOP('',(#41659,#41660));
#17493=EDGE_LOOP('',(#41661));
#17494=EDGE_LOOP('',(#41662));
#17495=EDGE_LOOP('',(#41663,#41664));
#17496=EDGE_LOOP('',(#41665));
#17497=EDGE_LOOP('',(#41666));
#17498=EDGE_LOOP('',(#41667,#41668));
#17499=EDGE_LOOP('',(#41669));
#17500=EDGE_LOOP('',(#41670,#41671));
#17501=EDGE_LOOP('',(#41672,#41673));
#17502=EDGE_LOOP('',(#41674));
#17503=EDGE_LOOP('',(#41675));
#17504=EDGE_LOOP('',(#41676,#41677));
#17505=EDGE_LOOP('',(#41678));
#17506=EDGE_LOOP('',(#41679));
#17507=EDGE_LOOP('',(#41680,#41681));
#17508=EDGE_LOOP('',(#41682));
#17509=EDGE_LOOP('',(#41683));
#17510=EDGE_LOOP('',(#41684,#41685));
#17511=EDGE_LOOP('',(#41686));
#17512=EDGE_LOOP('',(#41687,#41688));
#17513=EDGE_LOOP('',(#41689,#41690));
#17514=EDGE_LOOP('',(#41691));
#17515=EDGE_LOOP('',(#41692));
#17516=EDGE_LOOP('',(#41693,#41694));
#17517=EDGE_LOOP('',(#41695));
#17518=EDGE_LOOP('',(#41696));
#17519=EDGE_LOOP('',(#41697,#41698));
#17520=EDGE_LOOP('',(#41699));
#17521=EDGE_LOOP('',(#41700));
#17522=EDGE_LOOP('',(#41701,#41702));
#17523=EDGE_LOOP('',(#41703));
#17524=EDGE_LOOP('',(#41704));
#17525=EDGE_LOOP('',(#41705,#41706));
#17526=EDGE_LOOP('',(#41707));
#17527=EDGE_LOOP('',(#41708));
#17528=EDGE_LOOP('',(#41709,#41710));
#17529=EDGE_LOOP('',(#41711));
#17530=EDGE_LOOP('',(#41712));
#17531=EDGE_LOOP('',(#41713,#41714));
#17532=EDGE_LOOP('',(#41715));
#17533=EDGE_LOOP('',(#41716));
#17534=EDGE_LOOP('',(#41717,#41718));
#17535=EDGE_LOOP('',(#41719));
#17536=EDGE_LOOP('',(#41720));
#17537=EDGE_LOOP('',(#41721,#41722));
#17538=EDGE_LOOP('',(#41723));
#17539=EDGE_LOOP('',(#41724));
#17540=EDGE_LOOP('',(#41725,#41726));
#17541=EDGE_LOOP('',(#41727));
#17542=EDGE_LOOP('',(#41728));
#17543=EDGE_LOOP('',(#41729,#41730));
#17544=EDGE_LOOP('',(#41731));
#17545=EDGE_LOOP('',(#41732));
#17546=EDGE_LOOP('',(#41733,#41734));
#17547=EDGE_LOOP('',(#41735));
#17548=EDGE_LOOP('',(#41736));
#17549=EDGE_LOOP('',(#41737,#41738));
#17550=EDGE_LOOP('',(#41739));
#17551=EDGE_LOOP('',(#41740));
#17552=EDGE_LOOP('',(#41741,#41742));
#17553=EDGE_LOOP('',(#41743));
#17554=EDGE_LOOP('',(#41744));
#17555=EDGE_LOOP('',(#41745,#41746));
#17556=EDGE_LOOP('',(#41747));
#17557=EDGE_LOOP('',(#41748));
#17558=EDGE_LOOP('',(#41749,#41750));
#17559=EDGE_LOOP('',(#41751));
#17560=EDGE_LOOP('',(#41752));
#17561=EDGE_LOOP('',(#41753,#41754));
#17562=EDGE_LOOP('',(#41755));
#17563=EDGE_LOOP('',(#41756));
#17564=EDGE_LOOP('',(#41757,#41758));
#17565=EDGE_LOOP('',(#41759));
#17566=EDGE_LOOP('',(#41760));
#17567=EDGE_LOOP('',(#41761,#41762));
#17568=EDGE_LOOP('',(#41763));
#17569=EDGE_LOOP('',(#41764));
#17570=EDGE_LOOP('',(#41765,#41766));
#17571=EDGE_LOOP('',(#41767));
#17572=EDGE_LOOP('',(#41768));
#17573=EDGE_LOOP('',(#41769,#41770));
#17574=EDGE_LOOP('',(#41771));
#17575=EDGE_LOOP('',(#41772));
#17576=EDGE_LOOP('',(#41773,#41774));
#17577=EDGE_LOOP('',(#41775));
#17578=EDGE_LOOP('',(#41776));
#17579=EDGE_LOOP('',(#41777,#41778));
#17580=EDGE_LOOP('',(#41779));
#17581=EDGE_LOOP('',(#41780));
#17582=EDGE_LOOP('',(#41781,#41782));
#17583=EDGE_LOOP('',(#41783));
#17584=EDGE_LOOP('',(#41784));
#17585=EDGE_LOOP('',(#41785,#41786));
#17586=EDGE_LOOP('',(#41787));
#17587=EDGE_LOOP('',(#41788));
#17588=EDGE_LOOP('',(#41789,#41790));
#17589=EDGE_LOOP('',(#41791));
#17590=EDGE_LOOP('',(#41792));
#17591=EDGE_LOOP('',(#41793,#41794));
#17592=EDGE_LOOP('',(#41795));
#17593=EDGE_LOOP('',(#41796));
#17594=EDGE_LOOP('',(#41797,#41798));
#17595=EDGE_LOOP('',(#41799));
#17596=EDGE_LOOP('',(#41800));
#17597=EDGE_LOOP('',(#41801,#41802));
#17598=EDGE_LOOP('',(#41803));
#17599=EDGE_LOOP('',(#41804));
#17600=EDGE_LOOP('',(#41805,#41806));
#17601=EDGE_LOOP('',(#41807));
#17602=EDGE_LOOP('',(#41808));
#17603=EDGE_LOOP('',(#41809,#41810));
#17604=EDGE_LOOP('',(#41811));
#17605=EDGE_LOOP('',(#41812));
#17606=EDGE_LOOP('',(#41813,#41814));
#17607=EDGE_LOOP('',(#41815));
#17608=EDGE_LOOP('',(#41816));
#17609=EDGE_LOOP('',(#41817,#41818));
#17610=EDGE_LOOP('',(#41819));
#17611=EDGE_LOOP('',(#41820));
#17612=EDGE_LOOP('',(#41821,#41822));
#17613=EDGE_LOOP('',(#41823));
#17614=EDGE_LOOP('',(#41824));
#17615=EDGE_LOOP('',(#41825,#41826));
#17616=EDGE_LOOP('',(#41827));
#17617=EDGE_LOOP('',(#41828));
#17618=EDGE_LOOP('',(#41829,#41830));
#17619=EDGE_LOOP('',(#41831));
#17620=EDGE_LOOP('',(#41832,#41833));
#17621=EDGE_LOOP('',(#41834,#41835));
#17622=EDGE_LOOP('',(#41836));
#17623=EDGE_LOOP('',(#41837));
#17624=EDGE_LOOP('',(#41838,#41839));
#17625=EDGE_LOOP('',(#41840));
#17626=EDGE_LOOP('',(#41841));
#17627=EDGE_LOOP('',(#41842,#41843));
#17628=EDGE_LOOP('',(#41844));
#17629=EDGE_LOOP('',(#41845));
#17630=EDGE_LOOP('',(#41846,#41847));
#17631=EDGE_LOOP('',(#41848));
#17632=EDGE_LOOP('',(#41849));
#17633=EDGE_LOOP('',(#41850,#41851));
#17634=EDGE_LOOP('',(#41852));
#17635=EDGE_LOOP('',(#41853));
#17636=EDGE_LOOP('',(#41854,#41855));
#17637=EDGE_LOOP('',(#41856));
#17638=EDGE_LOOP('',(#41857));
#17639=EDGE_LOOP('',(#41858,#41859));
#17640=EDGE_LOOP('',(#41860));
#17641=EDGE_LOOP('',(#41861));
#17642=EDGE_LOOP('',(#41862,#41863));
#17643=EDGE_LOOP('',(#41864));
#17644=EDGE_LOOP('',(#41865));
#17645=EDGE_LOOP('',(#41866,#41867));
#17646=EDGE_LOOP('',(#41868));
#17647=EDGE_LOOP('',(#41869));
#17648=EDGE_LOOP('',(#41870,#41871));
#17649=EDGE_LOOP('',(#41872));
#17650=EDGE_LOOP('',(#41873));
#17651=EDGE_LOOP('',(#41874,#41875));
#17652=EDGE_LOOP('',(#41876));
#17653=EDGE_LOOP('',(#41877));
#17654=EDGE_LOOP('',(#41878,#41879));
#17655=EDGE_LOOP('',(#41880));
#17656=EDGE_LOOP('',(#41881));
#17657=EDGE_LOOP('',(#41882,#41883));
#17658=EDGE_LOOP('',(#41884));
#17659=EDGE_LOOP('',(#41885));
#17660=EDGE_LOOP('',(#41886,#41887));
#17661=EDGE_LOOP('',(#41888));
#17662=EDGE_LOOP('',(#41889));
#17663=EDGE_LOOP('',(#41890,#41891));
#17664=EDGE_LOOP('',(#41892));
#17665=EDGE_LOOP('',(#41893));
#17666=EDGE_LOOP('',(#41894,#41895));
#17667=EDGE_LOOP('',(#41896));
#17668=EDGE_LOOP('',(#41897));
#17669=EDGE_LOOP('',(#41898,#41899));
#17670=EDGE_LOOP('',(#41900));
#17671=EDGE_LOOP('',(#41901));
#17672=EDGE_LOOP('',(#41902,#41903));
#17673=EDGE_LOOP('',(#41904));
#17674=EDGE_LOOP('',(#41905));
#17675=EDGE_LOOP('',(#41906,#41907));
#17676=EDGE_LOOP('',(#41908));
#17677=EDGE_LOOP('',(#41909));
#17678=EDGE_LOOP('',(#41910,#41911));
#17679=EDGE_LOOP('',(#41912));
#17680=EDGE_LOOP('',(#41913));
#17681=EDGE_LOOP('',(#41914,#41915));
#17682=EDGE_LOOP('',(#41916));
#17683=EDGE_LOOP('',(#41917));
#17684=EDGE_LOOP('',(#41918,#41919));
#17685=EDGE_LOOP('',(#41920));
#17686=EDGE_LOOP('',(#41921));
#17687=EDGE_LOOP('',(#41922,#41923));
#17688=EDGE_LOOP('',(#41924));
#17689=EDGE_LOOP('',(#41925));
#17690=EDGE_LOOP('',(#41926,#41927));
#17691=EDGE_LOOP('',(#41928));
#17692=EDGE_LOOP('',(#41929));
#17693=EDGE_LOOP('',(#41930,#41931));
#17694=EDGE_LOOP('',(#41932));
#17695=EDGE_LOOP('',(#41933));
#17696=EDGE_LOOP('',(#41934,#41935));
#17697=EDGE_LOOP('',(#41936));
#17698=EDGE_LOOP('',(#41937));
#17699=EDGE_LOOP('',(#41938,#41939));
#17700=EDGE_LOOP('',(#41940));
#17701=EDGE_LOOP('',(#41941));
#17702=EDGE_LOOP('',(#41942,#41943));
#19404=CIRCLE('',#48903,85.1127409318642);
#19405=CIRCLE('',#48904,126.822029782344);
#19406=CIRCLE('',#48906,8.51742334960548);
#19407=CIRCLE('',#48907,0.5);
#19408=CIRCLE('',#48908,8.81821463020444);
#19409=CIRCLE('',#48911,0.675444121136126);
#19410=CIRCLE('',#48914,0.498831135992472);
#19411=CIRCLE('',#48917,0.490540748728341);
#19412=CIRCLE('',#48920,0.878303132193281);
#19413=CIRCLE('',#48923,0.675444121136182);
#19414=CIRCLE('',#48926,0.498831135992472);
#19415=CIRCLE('',#48929,0.490540748728341);
#19416=CIRCLE('',#48932,0.878303132193337);
#19417=CIRCLE('',#48935,0.675444121136126);
#19418=CIRCLE('',#48938,0.498831135992472);
#19419=CIRCLE('',#48941,0.490540748728341);
#19420=CIRCLE('',#48944,0.878303132193281);
#19421=CIRCLE('',#48947,0.675444121136126);
#19422=CIRCLE('',#48950,0.498831135992472);
#19423=CIRCLE('',#48953,0.490540748728285);
#19424=CIRCLE('',#48956,0.878303132193226);
#19425=CIRCLE('',#48959,0.675444121136182);
#19426=CIRCLE('',#48962,0.498831135992472);
#19427=CIRCLE('',#48965,0.490540748728341);
#19428=CIRCLE('',#48968,0.878303132193281);
#19429=CIRCLE('',#48971,0.675444121136182);
#19430=CIRCLE('',#48974,0.498831135992472);
#19431=CIRCLE('',#48977,0.490540748728341);
#19432=CIRCLE('',#48980,0.878303132193281);
#19433=CIRCLE('',#48983,0.675444121136182);
#19434=CIRCLE('',#48986,0.498831135992583);
#19435=CIRCLE('',#48989,0.490540748728341);
#19436=CIRCLE('',#48992,0.87830313219317);
#19437=CIRCLE('',#48995,0.675444121136071);
#19438=CIRCLE('',#48998,0.498831135992472);
#19439=CIRCLE('',#49001,0.490540748728341);
#19440=CIRCLE('',#49004,0.87830313219317);
#19441=CIRCLE('',#49007,0.675444121136071);
#19442=CIRCLE('',#49010,0.498831135992361);
#19443=CIRCLE('',#49013,0.490540748728341);
#19444=CIRCLE('',#49016,0.878303132193281);
#19445=CIRCLE('',#49019,0.675444121136182);
#19446=CIRCLE('',#49022,0.498831135992472);
#19447=CIRCLE('',#49025,0.49054074872823);
#19448=CIRCLE('',#49028,0.878303132193337);
#19449=CIRCLE('',#49031,0.675444121136182);
#19450=CIRCLE('',#49034,0.498831135992472);
#19451=CIRCLE('',#49037,0.490540748728341);
#19452=CIRCLE('',#49040,0.878303132193281);
#19453=CIRCLE('',#49043,0.675444121136126);
#19454=CIRCLE('',#49046,0.498831135992472);
#19455=CIRCLE('',#49049,0.490540748728341);
#19456=CIRCLE('',#49052,0.878303132193281);
#19457=CIRCLE('',#49055,0.675444121136182);
#19458=CIRCLE('',#49058,0.498831135992417);
#19459=CIRCLE('',#49061,0.490540748728341);
#19460=CIRCLE('',#49064,0.878303132193281);
#19461=CIRCLE('',#49067,0.675444121136126);
#19462=CIRCLE('',#49070,0.498831135992417);
#19463=CIRCLE('',#49073,0.490540748728341);
#19464=CIRCLE('',#49076,0.878303132193337);
#19465=CIRCLE('',#49079,0.675444121136182);
#19466=CIRCLE('',#49082,0.498831135992417);
#19467=CIRCLE('',#49085,0.490540748728341);
#19468=CIRCLE('',#49088,0.878303132193337);
#19469=CIRCLE('',#49091,0.675444121136126);
#19470=CIRCLE('',#49094,0.498831135992472);
#19471=CIRCLE('',#49097,0.490540748728341);
#19472=CIRCLE('',#49100,0.878303132193281);
#19473=CIRCLE('',#49103,0.675444121136182);
#19474=CIRCLE('',#49106,0.498831135992472);
#19475=CIRCLE('',#49109,0.490540748728341);
#19476=CIRCLE('',#49112,0.878303132193281);
#19477=CIRCLE('',#49115,0.675444121136182);
#19478=CIRCLE('',#49118,0.498831135992472);
#19479=CIRCLE('',#49121,0.490540748728341);
#19480=CIRCLE('',#49124,0.878303132193281);
#19481=CIRCLE('',#49127,0.675444121136126);
#19482=CIRCLE('',#49130,0.498831135992472);
#19483=CIRCLE('',#49133,0.490540748728341);
#19484=CIRCLE('',#49136,0.878303132193337);
#19485=CIRCLE('',#49139,0.675444121136126);
#19486=CIRCLE('',#49142,0.498831135992472);
#19487=CIRCLE('',#49145,0.490540748728341);
#19488=CIRCLE('',#49148,0.878303132193281);
#19489=CIRCLE('',#49151,0.675444121136182);
#19490=CIRCLE('',#49154,0.498831135992472);
#19491=CIRCLE('',#49157,0.490540748728341);
#19492=CIRCLE('',#49160,0.878303132193281);
#19493=CIRCLE('',#49163,0.675444121136126);
#19494=CIRCLE('',#49166,0.498831135992472);
#19495=CIRCLE('',#49169,0.490540748728341);
#19496=CIRCLE('',#49172,0.878303132193281);
#19497=CIRCLE('',#49175,0.675444121136126);
#19498=CIRCLE('',#49178,0.498831135992472);
#19499=CIRCLE('',#49181,0.490540748728396);
#19500=CIRCLE('',#49184,0.878303132193281);
#19501=CIRCLE('',#49187,0.675444121136126);
#19502=CIRCLE('',#49190,0.498831135992417);
#19503=CIRCLE('',#49193,0.490540748728341);
#19504=CIRCLE('',#49196,0.878303132193281);
#19505=CIRCLE('',#49199,0.675444121136126);
#19506=CIRCLE('',#49202,0.498831135992472);
#19507=CIRCLE('',#49205,0.490540748728396);
#19508=CIRCLE('',#49208,0.878303132193281);
#19509=CIRCLE('',#49211,0.675444121136182);
#19510=CIRCLE('',#49214,0.498831135992528);
#19511=CIRCLE('',#49217,0.490540748728341);
#19512=CIRCLE('',#49220,0.878303132193337);
#19513=CIRCLE('',#49223,0.675444121136126);
#19514=CIRCLE('',#49226,0.498831135992472);
#19515=CIRCLE('',#49229,0.490540748728285);
#19516=CIRCLE('',#49232,0.878303132193281);
#19517=CIRCLE('',#49235,0.675444121136126);
#19518=CIRCLE('',#49238,0.498831135992528);
#19519=CIRCLE('',#49241,0.490540748728341);
#19520=CIRCLE('',#49244,0.878303132193337);
#19521=CIRCLE('',#49247,0.675444121136182);
#19522=CIRCLE('',#49250,0.498831135992472);
#19523=CIRCLE('',#49253,0.490540748728285);
#19524=CIRCLE('',#49256,0.878303132193281);
#19525=CIRCLE('',#49259,0.675444121136126);
#19526=CIRCLE('',#49262,0.490540748728341);
#19527=CIRCLE('',#49265,0.498831135992472);
#19528=CIRCLE('',#49267,1.10035806567471);
#19529=CIRCLE('',#49268,1.10035806567471);
#19530=CIRCLE('',#49270,0.500358065674722);
#19531=CIRCLE('',#49271,0.500358065674722);
#19532=CIRCLE('',#49273,1.21403156673711);
#19533=CIRCLE('',#49274,1.21403156673711);
#19534=CIRCLE('',#49276,0.614031566737117);
#19535=CIRCLE('',#49277,0.614031566737117);
#19536=CIRCLE('',#49279,1.32880796357332);
#19537=CIRCLE('',#49280,1.32880796357332);
#19538=CIRCLE('',#49282,0.72880796357333);
#19539=CIRCLE('',#49283,0.72880796357333);
#19540=CIRCLE('',#49285,1.46111700181689);
#19541=CIRCLE('',#49286,1.46111700181689);
#19542=CIRCLE('',#49288,0.861117001816902);
#19543=CIRCLE('',#49289,0.861117001816902);
#19544=CIRCLE('',#49291,1.6204820426246);
#19545=CIRCLE('',#49292,1.6204820426246);
#19546=CIRCLE('',#49294,1.02048204262462);
#19547=CIRCLE('',#49295,1.02048204262462);
#19548=CIRCLE('',#49297,1.70100022308284);
#19549=CIRCLE('',#49298,1.70100022308284);
#19550=CIRCLE('',#49300,1.10100022308285);
#19551=CIRCLE('',#49301,1.10100022308285);
#19552=CIRCLE('',#49303,1.72127463204352);
#19553=CIRCLE('',#49304,1.72127463204352);
#19554=CIRCLE('',#49306,1.12127463204348);
#19555=CIRCLE('',#49307,1.12127463204348);
#19556=CIRCLE('',#49309,1.78199265440493);
#19557=CIRCLE('',#49310,1.78199265440493);
#19558=CIRCLE('',#49312,1.18199265440494);
#19559=CIRCLE('',#49313,1.18199265440494);
#19560=CIRCLE('',#49315,1.66088080992077);
#19561=CIRCLE('',#49316,1.66088080992077);
#19562=CIRCLE('',#49318,1.06088080992078);
#19563=CIRCLE('',#49319,1.06088080992078);
#19564=CIRCLE('',#49321,1.10035806567471);
#19565=CIRCLE('',#49322,1.10035806567471);
#19566=CIRCLE('',#49324,0.500358065674722);
#19567=CIRCLE('',#49325,0.500358065674722);
#19568=CIRCLE('',#49327,1.21403156673716);
#19569=CIRCLE('',#49328,1.21403156673716);
#19570=CIRCLE('',#49330,0.614031566737117);
#19571=CIRCLE('',#49331,0.614031566737117);
#19572=CIRCLE('',#49333,1.32880796357332);
#19573=CIRCLE('',#49334,1.32880796357332);
#19574=CIRCLE('',#49336,0.728807963573275);
#19575=CIRCLE('',#49337,0.728807963573275);
#19576=CIRCLE('',#49339,1.46111700181689);
#19577=CIRCLE('',#49340,1.46111700181689);
#19578=CIRCLE('',#49342,0.861117001816902);
#19579=CIRCLE('',#49343,0.861117001816902);
#19580=CIRCLE('',#49345,1.6204820426246);
#19581=CIRCLE('',#49346,1.6204820426246);
#19582=CIRCLE('',#49348,1.02048204262462);
#19583=CIRCLE('',#49349,1.02048204262462);
#19584=CIRCLE('',#49351,1.70100022308284);
#19585=CIRCLE('',#49352,1.70100022308284);
#19586=CIRCLE('',#49354,1.10100022308285);
#19587=CIRCLE('',#49355,1.10100022308285);
#19588=CIRCLE('',#49357,1.72127463204347);
#19589=CIRCLE('',#49358,1.72127463204347);
#19590=CIRCLE('',#49360,1.12127463204348);
#19591=CIRCLE('',#49361,1.12127463204348);
#19592=CIRCLE('',#49363,1.78199265440493);
#19593=CIRCLE('',#49364,1.78199265440493);
#19594=CIRCLE('',#49366,1.18199265440494);
#19595=CIRCLE('',#49367,1.18199265440494);
#19596=CIRCLE('',#49369,1.66088080992077);
#19597=CIRCLE('',#49370,1.66088080992077);
#19598=CIRCLE('',#49372,1.06088080992078);
#19599=CIRCLE('',#49373,1.06088080992078);
#19600=CIRCLE('',#49375,1.10035806567471);
#19601=CIRCLE('',#49376,1.10035806567471);
#19602=CIRCLE('',#49378,0.500358065674722);
#19603=CIRCLE('',#49379,0.500358065674722);
#19604=CIRCLE('',#49381,1.21403156673716);
#19605=CIRCLE('',#49382,1.21403156673716);
#19606=CIRCLE('',#49384,0.614031566737117);
#19607=CIRCLE('',#49385,0.614031566737117);
#19608=CIRCLE('',#49387,1.32880796357326);
#19609=CIRCLE('',#49388,1.32880796357326);
#19610=CIRCLE('',#49390,0.72880796357333);
#19611=CIRCLE('',#49391,0.72880796357333);
#19612=CIRCLE('',#49393,1.46111700181689);
#19613=CIRCLE('',#49394,1.46111700181689);
#19614=CIRCLE('',#49396,0.861117001816902);
#19615=CIRCLE('',#49397,0.861117001816902);
#19616=CIRCLE('',#49399,1.6204820426246);
#19617=CIRCLE('',#49400,1.6204820426246);
#19618=CIRCLE('',#49402,1.02048204262456);
#19619=CIRCLE('',#49403,1.02048204262456);
#19620=CIRCLE('',#49405,1.70100022308284);
#19621=CIRCLE('',#49406,1.70100022308284);
#19622=CIRCLE('',#49408,1.10100022308285);
#19623=CIRCLE('',#49409,1.10100022308285);
#19624=CIRCLE('',#49411,1.72127463204347);
#19625=CIRCLE('',#49412,1.72127463204347);
#19626=CIRCLE('',#49414,1.12127463204348);
#19627=CIRCLE('',#49415,1.12127463204348);
#19628=CIRCLE('',#49417,1.78199265440493);
#19629=CIRCLE('',#49418,1.78199265440493);
#19630=CIRCLE('',#49420,1.18199265440494);
#19631=CIRCLE('',#49421,1.18199265440494);
#19632=CIRCLE('',#49423,1.66088080992077);
#19633=CIRCLE('',#49424,1.66088080992077);
#19634=CIRCLE('',#49426,1.06088080992078);
#19635=CIRCLE('',#49427,1.06088080992078);
#19636=CIRCLE('',#49429,1.10035806567471);
#19637=CIRCLE('',#49430,1.10035806567471);
#19638=CIRCLE('',#49432,0.500358065674666);
#19639=CIRCLE('',#49433,0.500358065674666);
#19640=CIRCLE('',#49435,1.21403156673711);
#19641=CIRCLE('',#49436,1.21403156673711);
#19642=CIRCLE('',#49438,0.614031566737172);
#19643=CIRCLE('',#49439,0.614031566737172);
#19644=CIRCLE('',#49441,1.32880796357332);
#19645=CIRCLE('',#49442,1.32880796357332);
#19646=CIRCLE('',#49444,0.72880796357333);
#19647=CIRCLE('',#49445,0.72880796357333);
#19648=CIRCLE('',#49447,1.46111700181689);
#19649=CIRCLE('',#49448,1.46111700181689);
#19650=CIRCLE('',#49450,0.861117001816847);
#19651=CIRCLE('',#49451,0.861117001816847);
#19652=CIRCLE('',#49453,1.6204820426246);
#19653=CIRCLE('',#49454,1.6204820426246);
#19654=CIRCLE('',#49456,1.02048204262462);
#19655=CIRCLE('',#49457,1.02048204262462);
#19656=CIRCLE('',#49459,1.70100022308284);
#19657=CIRCLE('',#49460,1.70100022308284);
#19658=CIRCLE('',#49462,1.10100022308285);
#19659=CIRCLE('',#49463,1.10100022308285);
#19660=CIRCLE('',#49465,1.72127463204347);
#19661=CIRCLE('',#49466,1.72127463204347);
#19662=CIRCLE('',#49468,1.12127463204353);
#19663=CIRCLE('',#49469,1.12127463204353);
#19664=CIRCLE('',#49471,1.78199265440498);
#19665=CIRCLE('',#49472,1.78199265440498);
#19666=CIRCLE('',#49474,1.18199265440494);
#19667=CIRCLE('',#49475,1.18199265440494);
#19668=CIRCLE('',#49477,1.66088080992083);
#19669=CIRCLE('',#49478,1.66088080992083);
#19670=CIRCLE('',#49480,1.06088080992078);
#19671=CIRCLE('',#49481,1.06088080992078);
#19672=CIRCLE('',#49483,1.10035806567477);
#19673=CIRCLE('',#49484,1.10035806567477);
#19674=CIRCLE('',#49486,0.500358065674777);
#19675=CIRCLE('',#49487,0.500358065674777);
#19676=CIRCLE('',#49489,1.21403156673711);
#19677=CIRCLE('',#49490,1.21403156673711);
#19678=CIRCLE('',#49492,0.614031566737172);
#19679=CIRCLE('',#49493,0.614031566737172);
#19680=CIRCLE('',#49495,1.32880796357326);
#19681=CIRCLE('',#49496,1.32880796357326);
#19682=CIRCLE('',#49498,0.72880796357333);
#19683=CIRCLE('',#49499,0.72880796357333);
#19684=CIRCLE('',#49501,1.46111700181684);
#19685=CIRCLE('',#49502,1.46111700181684);
#19686=CIRCLE('',#49504,0.861117001816847);
#19687=CIRCLE('',#49505,0.861117001816847);
#19688=CIRCLE('',#49507,1.6204820426246);
#19689=CIRCLE('',#49508,1.6204820426246);
#19690=CIRCLE('',#49510,1.02048204262462);
#19691=CIRCLE('',#49511,1.02048204262462);
#19692=CIRCLE('',#49513,1.70100022308278);
#19693=CIRCLE('',#49514,1.70100022308278);
#19694=CIRCLE('',#49516,1.1010002230829);
#19695=CIRCLE('',#49517,1.1010002230829);
#19696=CIRCLE('',#49519,1.72127463204347);
#19697=CIRCLE('',#49520,1.72127463204347);
#19698=CIRCLE('',#49522,1.12127463204342);
#19699=CIRCLE('',#49523,1.12127463204342);
#19700=CIRCLE('',#49525,1.78199265440487);
#19701=CIRCLE('',#49526,1.78199265440487);
#19702=CIRCLE('',#49528,1.18199265440488);
#19703=CIRCLE('',#49529,1.18199265440488);
#19704=CIRCLE('',#49531,1.66088080992077);
#19705=CIRCLE('',#49532,1.66088080992077);
#19706=CIRCLE('',#49534,1.06088080992078);
#19707=CIRCLE('',#49535,1.06088080992078);
#19708=CIRCLE('',#49537,1.10035806567466);
#19709=CIRCLE('',#49538,1.10035806567466);
#19710=CIRCLE('',#49540,0.500358065674722);
#19711=CIRCLE('',#49541,0.500358065674722);
#19712=CIRCLE('',#49543,1.21403156673716);
#19713=CIRCLE('',#49544,1.21403156673716);
#19714=CIRCLE('',#49546,0.614031566737117);
#19715=CIRCLE('',#49547,0.614031566737117);
#19716=CIRCLE('',#49549,1.32880796357326);
#19717=CIRCLE('',#49550,1.32880796357326);
#19718=CIRCLE('',#49552,0.728807963573275);
#19719=CIRCLE('',#49553,0.728807963573275);
#19720=CIRCLE('',#49555,1.46111700181684);
#19721=CIRCLE('',#49556,1.46111700181684);
#19722=CIRCLE('',#49558,0.861117001816847);
#19723=CIRCLE('',#49559,0.861117001816847);
#19724=CIRCLE('',#49561,1.6204820426246);
#19725=CIRCLE('',#49562,1.6204820426246);
#19726=CIRCLE('',#49564,1.02048204262456);
#19727=CIRCLE('',#49565,1.02048204262456);
#19728=CIRCLE('',#49567,1.70100022308284);
#19729=CIRCLE('',#49568,1.70100022308284);
#19730=CIRCLE('',#49570,1.10100022308279);
#19731=CIRCLE('',#49571,1.10100022308279);
#19732=CIRCLE('',#49573,1.72127463204347);
#19733=CIRCLE('',#49574,1.72127463204347);
#19734=CIRCLE('',#49576,1.12127463204348);
#19735=CIRCLE('',#49577,1.12127463204348);
#19736=CIRCLE('',#49579,1.78199265440493);
#19737=CIRCLE('',#49580,1.78199265440493);
#19738=CIRCLE('',#49582,1.18199265440494);
#19739=CIRCLE('',#49583,1.18199265440494);
#19740=CIRCLE('',#49585,1.66088080992088);
#19741=CIRCLE('',#49586,1.66088080992083);
#19742=CIRCLE('',#49588,1.06088080992084);
#19743=CIRCLE('',#49589,1.06088080992084);
#19744=CIRCLE('',#49591,1.10035806567466);
#19745=CIRCLE('',#49592,1.10035806567466);
#19746=CIRCLE('',#49594,0.500358065674666);
#19747=CIRCLE('',#49595,0.500358065674666);
#19748=CIRCLE('',#49597,1.21403156673716);
#19749=CIRCLE('',#49598,1.21403156673716);
#19750=CIRCLE('',#49600,0.614031566737172);
#19751=CIRCLE('',#49601,0.614031566737172);
#19752=CIRCLE('',#49603,1.32880796357332);
#19753=CIRCLE('',#49604,1.32880796357332);
#19754=CIRCLE('',#49606,0.728807963573275);
#19755=CIRCLE('',#49607,0.728807963573275);
#19756=CIRCLE('',#49609,1.46111700181689);
#19757=CIRCLE('',#49610,1.46111700181689);
#19758=CIRCLE('',#49612,0.861117001816847);
#19759=CIRCLE('',#49613,0.861117001816847);
#19760=CIRCLE('',#49615,1.6204820426246);
#19761=CIRCLE('',#49616,1.6204820426246);
#19762=CIRCLE('',#49618,1.02048204262456);
#19763=CIRCLE('',#49619,1.02048204262456);
#19764=CIRCLE('',#49621,1.70100022308284);
#19765=CIRCLE('',#49622,1.70100022308284);
#19766=CIRCLE('',#49624,1.10100022308285);
#19767=CIRCLE('',#49625,1.10100022308285);
#19768=CIRCLE('',#49627,1.72127463204352);
#19769=CIRCLE('',#49628,1.72127463204352);
#19770=CIRCLE('',#49630,1.12127463204348);
#19771=CIRCLE('',#49631,1.12127463204348);
#19772=CIRCLE('',#49633,1.78199265440493);
#19773=CIRCLE('',#49634,1.78199265440498);
#19774=CIRCLE('',#49636,1.18199265440494);
#19775=CIRCLE('',#49637,1.18199265440494);
#19776=CIRCLE('',#49639,1.66088080992077);
#19777=CIRCLE('',#49640,1.66088080992077);
#19778=CIRCLE('',#49642,1.06088080992073);
#19779=CIRCLE('',#49643,1.06088080992073);
#19780=CIRCLE('',#49645,1.10035806567471);
#19781=CIRCLE('',#49646,1.10035806567471);
#19782=CIRCLE('',#49648,0.500358065674722);
#19783=CIRCLE('',#49649,0.500358065674722);
#19784=CIRCLE('',#49651,1.21403156673716);
#19785=CIRCLE('',#49652,1.21403156673716);
#19786=CIRCLE('',#49654,0.614031566737117);
#19787=CIRCLE('',#49655,0.614031566737117);
#19788=CIRCLE('',#49657,1.32880796357332);
#19789=CIRCLE('',#49658,1.32880796357332);
#19790=CIRCLE('',#49660,0.72880796357333);
#19791=CIRCLE('',#49661,0.72880796357333);
#19792=CIRCLE('',#49663,1.46111700181689);
#19793=CIRCLE('',#49664,1.46111700181689);
#19794=CIRCLE('',#49666,0.861117001816902);
#19795=CIRCLE('',#49667,0.861117001816902);
#19796=CIRCLE('',#49669,1.6204820426246);
#19797=CIRCLE('',#49670,1.6204820426246);
#19798=CIRCLE('',#49672,1.02048204262456);
#19799=CIRCLE('',#49673,1.02048204262456);
#19800=CIRCLE('',#49675,1.70100022308278);
#19801=CIRCLE('',#49676,1.70100022308278);
#19802=CIRCLE('',#49678,1.10100022308285);
#19803=CIRCLE('',#49679,1.10100022308285);
#19804=CIRCLE('',#49681,1.72127463204347);
#19805=CIRCLE('',#49682,1.72127463204347);
#19806=CIRCLE('',#49684,1.12127463204348);
#19807=CIRCLE('',#49685,1.12127463204348);
#19808=CIRCLE('',#49687,1.78199265440493);
#19809=CIRCLE('',#49688,1.78199265440493);
#19810=CIRCLE('',#49690,1.18199265440494);
#19811=CIRCLE('',#49691,1.18199265440494);
#19812=CIRCLE('',#49693,1.66088080992077);
#19813=CIRCLE('',#49694,1.66088080992077);
#19814=CIRCLE('',#49696,1.06088080992073);
#19815=CIRCLE('',#49697,1.06088080992073);
#19816=CIRCLE('',#49699,1.10035806567471);
#19817=CIRCLE('',#49700,1.10035806567471);
#19818=CIRCLE('',#49702,0.500358065674722);
#19819=CIRCLE('',#49703,0.500358065674722);
#19820=CIRCLE('',#49705,1.21403156673711);
#19821=CIRCLE('',#49706,1.21403156673711);
#19822=CIRCLE('',#49708,0.614031566737117);
#19823=CIRCLE('',#49709,0.614031566737117);
#19824=CIRCLE('',#49711,1.32880796357332);
#19825=CIRCLE('',#49712,1.32880796357332);
#19826=CIRCLE('',#49714,0.72880796357333);
#19827=CIRCLE('',#49715,0.72880796357333);
#19828=CIRCLE('',#49717,1.46111700181689);
#19829=CIRCLE('',#49718,1.46111700181689);
#19830=CIRCLE('',#49720,0.861117001816902);
#19831=CIRCLE('',#49721,0.861117001816902);
#19832=CIRCLE('',#49723,1.6204820426246);
#19833=CIRCLE('',#49724,1.6204820426246);
#19834=CIRCLE('',#49726,1.02048204262456);
#19835=CIRCLE('',#49727,1.02048204262456);
#19836=CIRCLE('',#49729,1.70100022308284);
#19837=CIRCLE('',#49730,1.70100022308284);
#19838=CIRCLE('',#49732,1.10100022308285);
#19839=CIRCLE('',#49733,1.10100022308285);
#19840=CIRCLE('',#49735,1.72127463204352);
#19841=CIRCLE('',#49736,1.72127463204352);
#19842=CIRCLE('',#49738,1.12127463204348);
#19843=CIRCLE('',#49739,1.12127463204348);
#19844=CIRCLE('',#49741,1.78199265440487);
#19845=CIRCLE('',#49742,1.78199265440487);
#19846=CIRCLE('',#49744,1.18199265440488);
#19847=CIRCLE('',#49745,1.18199265440488);
#19848=CIRCLE('',#49747,1.66088080992088);
#19849=CIRCLE('',#49748,1.66088080992088);
#19850=CIRCLE('',#49750,1.06088080992073);
#19851=CIRCLE('',#49751,1.06088080992073);
#19852=CIRCLE('',#49753,1.10035806567471);
#19853=CIRCLE('',#49754,1.10035806567471);
#19854=CIRCLE('',#49756,0.500358065674666);
#19855=CIRCLE('',#49757,0.500358065674666);
#19856=CIRCLE('',#49759,1.21403156673716);
#19857=CIRCLE('',#49760,1.21403156673716);
#19858=CIRCLE('',#49762,0.614031566737172);
#19859=CIRCLE('',#49763,0.614031566737172);
#19860=CIRCLE('',#49765,1.32880796357338);
#19861=CIRCLE('',#49766,1.32880796357338);
#19862=CIRCLE('',#49768,0.72880796357333);
#19863=CIRCLE('',#49769,0.72880796357333);
#19864=CIRCLE('',#49771,1.46111700181689);
#19865=CIRCLE('',#49772,1.46111700181689);
#19866=CIRCLE('',#49774,0.861117001816902);
#19867=CIRCLE('',#49775,0.861117001816902);
#19868=CIRCLE('',#49777,1.6204820426246);
#19869=CIRCLE('',#49778,1.6204820426246);
#19870=CIRCLE('',#49780,1.02048204262456);
#19871=CIRCLE('',#49781,1.02048204262456);
#19872=CIRCLE('',#49783,1.70100022308284);
#19873=CIRCLE('',#49784,1.70100022308284);
#19874=CIRCLE('',#49786,1.10100022308285);
#19875=CIRCLE('',#49787,1.10100022308285);
#19876=CIRCLE('',#49789,1.72127463204352);
#19877=CIRCLE('',#49790,1.72127463204352);
#19878=CIRCLE('',#49792,1.12127463204348);
#19879=CIRCLE('',#49793,1.12127463204348);
#19880=CIRCLE('',#49795,1.78199265440498);
#19881=CIRCLE('',#49796,1.78199265440498);
#19882=CIRCLE('',#49798,1.181992654405);
#19883=CIRCLE('',#49799,1.181992654405);
#19884=CIRCLE('',#49801,1.66088080992077);
#19885=CIRCLE('',#49802,1.66088080992077);
#19886=CIRCLE('',#49804,1.06088080992073);
#19887=CIRCLE('',#49805,1.06088080992073);
#19888=CIRCLE('',#49807,1.10035806567471);
#19889=CIRCLE('',#49808,1.10035806567471);
#19890=CIRCLE('',#49810,0.500358065674722);
#19891=CIRCLE('',#49811,0.500358065674722);
#19892=CIRCLE('',#49813,1.21403156673705);
#19893=CIRCLE('',#49814,1.21403156673705);
#19894=CIRCLE('',#49816,0.614031566737117);
#19895=CIRCLE('',#49817,0.614031566737117);
#19896=CIRCLE('',#49819,1.32880796357338);
#19897=CIRCLE('',#49820,1.32880796357338);
#19898=CIRCLE('',#49822,0.72880796357333);
#19899=CIRCLE('',#49823,0.72880796357333);
#19900=CIRCLE('',#49825,1.46111700181689);
#19901=CIRCLE('',#49826,1.46111700181689);
#19902=CIRCLE('',#49828,0.861117001816902);
#19903=CIRCLE('',#49829,0.861117001816902);
#19904=CIRCLE('',#49831,1.6204820426246);
#19905=CIRCLE('',#49832,1.6204820426246);
#19906=CIRCLE('',#49834,1.02048204262462);
#19907=CIRCLE('',#49835,1.02048204262462);
#19908=CIRCLE('',#49837,1.70100022308278);
#19909=CIRCLE('',#49838,1.70100022308278);
#19910=CIRCLE('',#49840,1.10100022308279);
#19911=CIRCLE('',#49841,1.10100022308279);
#19912=CIRCLE('',#49843,1.72127463204352);
#19913=CIRCLE('',#49844,1.72127463204352);
#19914=CIRCLE('',#49846,1.12127463204348);
#19915=CIRCLE('',#49847,1.12127463204348);
#19916=CIRCLE('',#49849,1.78199265440493);
#19917=CIRCLE('',#49850,1.78199265440493);
#19918=CIRCLE('',#49852,1.18199265440494);
#19919=CIRCLE('',#49853,1.18199265440494);
#19920=CIRCLE('',#49855,1.66088080992077);
#19921=CIRCLE('',#49856,1.66088080992077);
#19922=CIRCLE('',#49858,1.06088080992078);
#19923=CIRCLE('',#49859,1.06088080992078);
#19924=CIRCLE('',#49861,1.10035806567471);
#19925=CIRCLE('',#49862,1.10035806567471);
#19926=CIRCLE('',#49864,0.500358065674722);
#19927=CIRCLE('',#49865,0.500358065674722);
#19928=CIRCLE('',#49867,1.21403156673711);
#19929=CIRCLE('',#49868,1.21403156673711);
#19930=CIRCLE('',#49870,0.614031566737117);
#19931=CIRCLE('',#49871,0.614031566737117);
#19932=CIRCLE('',#49873,1.32880796357332);
#19933=CIRCLE('',#49874,1.32880796357332);
#19934=CIRCLE('',#49876,0.72880796357333);
#19935=CIRCLE('',#49877,0.72880796357333);
#19936=CIRCLE('',#49879,1.46111700181689);
#19937=CIRCLE('',#49880,1.46111700181689);
#19938=CIRCLE('',#49882,0.861117001816902);
#19939=CIRCLE('',#49883,0.861117001816902);
#19940=CIRCLE('',#49885,1.62048204262455);
#19941=CIRCLE('',#49886,1.62048204262455);
#19942=CIRCLE('',#49888,1.02048204262462);
#19943=CIRCLE('',#49889,1.02048204262462);
#19944=CIRCLE('',#49891,1.70100022308278);
#19945=CIRCLE('',#49892,1.70100022308278);
#19946=CIRCLE('',#49894,1.10100022308279);
#19947=CIRCLE('',#49895,1.10100022308279);
#19948=CIRCLE('',#49897,1.72127463204347);
#19949=CIRCLE('',#49898,1.72127463204347);
#19950=CIRCLE('',#49900,1.12127463204353);
#19951=CIRCLE('',#49901,1.12127463204353);
#19952=CIRCLE('',#49903,1.78199265440487);
#19953=CIRCLE('',#49904,1.78199265440487);
#19954=CIRCLE('',#49906,1.18199265440494);
#19955=CIRCLE('',#49907,1.18199265440494);
#19956=CIRCLE('',#49909,1.66088080992077);
#19957=CIRCLE('',#49910,1.66088080992077);
#19958=CIRCLE('',#49912,1.06088080992078);
#19959=CIRCLE('',#49913,1.06088080992078);
#19960=CIRCLE('',#49915,1.10035806567471);
#19961=CIRCLE('',#49916,1.10035806567471);
#19962=CIRCLE('',#49918,0.500358065674777);
#19963=CIRCLE('',#49919,0.500358065674777);
#19964=CIRCLE('',#49921,1.21403156673711);
#19965=CIRCLE('',#49922,1.21403156673711);
#19966=CIRCLE('',#49924,0.614031566737117);
#19967=CIRCLE('',#49925,0.614031566737117);
#19968=CIRCLE('',#49927,1.32880796357332);
#19969=CIRCLE('',#49928,1.32880796357332);
#19970=CIRCLE('',#49930,0.728807963573275);
#19971=CIRCLE('',#49931,0.728807963573275);
#19972=CIRCLE('',#49933,1.46111700181695);
#19973=CIRCLE('',#49934,1.46111700181695);
#19974=CIRCLE('',#49936,0.861117001816902);
#19975=CIRCLE('',#49937,0.861117001816902);
#19976=CIRCLE('',#49939,1.6204820426246);
#19977=CIRCLE('',#49940,1.6204820426246);
#19978=CIRCLE('',#49942,1.02048204262462);
#19979=CIRCLE('',#49943,1.02048204262462);
#19980=CIRCLE('',#49945,1.70100022308284);
#19981=CIRCLE('',#49946,1.70100022308284);
#19982=CIRCLE('',#49948,1.10100022308285);
#19983=CIRCLE('',#49949,1.10100022308285);
#19984=CIRCLE('',#49951,1.72127463204347);
#19985=CIRCLE('',#49952,1.72127463204347);
#19986=CIRCLE('',#49954,1.12127463204348);
#19987=CIRCLE('',#49955,1.12127463204348);
#19988=CIRCLE('',#49957,1.78199265440493);
#19989=CIRCLE('',#49958,1.78199265440493);
#19990=CIRCLE('',#49960,1.18199265440488);
#19991=CIRCLE('',#49961,1.18199265440488);
#19992=CIRCLE('',#49963,1.66088080992077);
#19993=CIRCLE('',#49964,1.66088080992077);
#19994=CIRCLE('',#49966,1.06088080992078);
#19995=CIRCLE('',#49967,1.06088080992078);
#19996=CIRCLE('',#49969,1.10035806567471);
#19997=CIRCLE('',#49970,1.10035806567471);
#19998=CIRCLE('',#49972,0.500358065674722);
#19999=CIRCLE('',#49973,0.500358065674722);
#20000=CIRCLE('',#49975,1.21403156673711);
#20001=CIRCLE('',#49976,1.21403156673711);
#20002=CIRCLE('',#49978,0.614031566737117);
#20003=CIRCLE('',#49979,0.614031566737117);
#20004=CIRCLE('',#49981,1.32880796357332);
#20005=CIRCLE('',#49982,1.32880796357332);
#20006=CIRCLE('',#49984,0.72880796357333);
#20007=CIRCLE('',#49985,0.72880796357333);
#20008=CIRCLE('',#49987,1.46111700181689);
#20009=CIRCLE('',#49988,1.46111700181689);
#20010=CIRCLE('',#49990,0.861117001816902);
#20011=CIRCLE('',#49991,0.861117001816902);
#20012=CIRCLE('',#49993,1.62048204262455);
#20013=CIRCLE('',#49994,1.62048204262455);
#20014=CIRCLE('',#49996,1.02048204262456);
#20015=CIRCLE('',#49997,1.02048204262456);
#20016=CIRCLE('',#49999,1.70100022308284);
#20017=CIRCLE('',#50000,1.70100022308284);
#20018=CIRCLE('',#50002,1.10100022308285);
#20019=CIRCLE('',#50003,1.10100022308285);
#20020=CIRCLE('',#50005,1.72127463204347);
#20021=CIRCLE('',#50006,1.72127463204347);
#20022=CIRCLE('',#50008,1.12127463204348);
#20023=CIRCLE('',#50009,1.12127463204348);
#20024=CIRCLE('',#50011,1.78199265440493);
#20025=CIRCLE('',#50012,1.78199265440493);
#20026=CIRCLE('',#50014,1.18199265440494);
#20027=CIRCLE('',#50015,1.18199265440494);
#20028=CIRCLE('',#50017,1.66088080992077);
#20029=CIRCLE('',#50018,1.66088080992077);
#20030=CIRCLE('',#50020,1.06088080992078);
#20031=CIRCLE('',#50021,1.06088080992078);
#20032=CIRCLE('',#50023,1.10035806567471);
#20033=CIRCLE('',#50024,1.10035806567471);
#20034=CIRCLE('',#50026,0.500358065674722);
#20035=CIRCLE('',#50027,0.500358065674722);
#20036=CIRCLE('',#50029,1.21403156673711);
#20037=CIRCLE('',#50030,1.21403156673711);
#20038=CIRCLE('',#50032,0.614031566737117);
#20039=CIRCLE('',#50033,0.614031566737117);
#20040=CIRCLE('',#50035,1.32880796357326);
#20041=CIRCLE('',#50036,1.32880796357326);
#20042=CIRCLE('',#50038,0.728807963573275);
#20043=CIRCLE('',#50039,0.728807963573275);
#20044=CIRCLE('',#50041,1.46111700181689);
#20045=CIRCLE('',#50042,1.46111700181689);
#20046=CIRCLE('',#50044,0.861117001816902);
#20047=CIRCLE('',#50045,0.861117001816902);
#20048=CIRCLE('',#50047,1.6204820426246);
#20049=CIRCLE('',#50048,1.6204820426246);
#20050=CIRCLE('',#50050,1.02048204262456);
#20051=CIRCLE('',#50051,1.02048204262456);
#20052=CIRCLE('',#50053,1.70100022308284);
#20053=CIRCLE('',#50054,1.70100022308284);
#20054=CIRCLE('',#50056,1.10100022308285);
#20055=CIRCLE('',#50057,1.10100022308285);
#20056=CIRCLE('',#50059,1.72127463204352);
#20057=CIRCLE('',#50060,1.72127463204352);
#20058=CIRCLE('',#50062,1.12127463204348);
#20059=CIRCLE('',#50063,1.12127463204348);
#20060=CIRCLE('',#50065,1.78199265440498);
#20061=CIRCLE('',#50066,1.78199265440498);
#20062=CIRCLE('',#50068,1.18199265440494);
#20063=CIRCLE('',#50069,1.18199265440494);
#20064=CIRCLE('',#50071,1.66088080992083);
#20065=CIRCLE('',#50072,1.66088080992083);
#20066=CIRCLE('',#50074,1.06088080992078);
#20067=CIRCLE('',#50075,1.06088080992078);
#20068=CIRCLE('',#50077,1.10035806567471);
#20069=CIRCLE('',#50078,1.10035806567471);
#20070=CIRCLE('',#50080,0.500358065674722);
#20071=CIRCLE('',#50081,0.500358065674722);
#20072=CIRCLE('',#50083,1.21403156673711);
#20073=CIRCLE('',#50084,1.21403156673711);
#20074=CIRCLE('',#50086,0.614031566737117);
#20075=CIRCLE('',#50087,0.614031566737117);
#20076=CIRCLE('',#50089,1.32880796357332);
#20077=CIRCLE('',#50090,1.32880796357332);
#20078=CIRCLE('',#50092,0.72880796357333);
#20079=CIRCLE('',#50093,0.72880796357333);
#20080=CIRCLE('',#50095,1.46111700181689);
#20081=CIRCLE('',#50096,1.46111700181689);
#20082=CIRCLE('',#50098,0.861117001816847);
#20083=CIRCLE('',#50099,0.861117001816847);
#20084=CIRCLE('',#50101,1.6204820426246);
#20085=CIRCLE('',#50102,1.6204820426246);
#20086=CIRCLE('',#50104,1.02048204262462);
#20087=CIRCLE('',#50105,1.02048204262462);
#20088=CIRCLE('',#50107,1.70100022308284);
#20089=CIRCLE('',#50108,1.70100022308284);
#20090=CIRCLE('',#50110,1.10100022308279);
#20091=CIRCLE('',#50111,1.10100022308279);
#20092=CIRCLE('',#50113,1.72127463204347);
#20093=CIRCLE('',#50114,1.72127463204347);
#20094=CIRCLE('',#50116,1.12127463204353);
#20095=CIRCLE('',#50117,1.12127463204353);
#20096=CIRCLE('',#50119,1.78199265440493);
#20097=CIRCLE('',#50120,1.78199265440493);
#20098=CIRCLE('',#50122,1.18199265440494);
#20099=CIRCLE('',#50123,1.18199265440494);
#20100=CIRCLE('',#50125,1.66088080992077);
#20101=CIRCLE('',#50126,1.66088080992077);
#20102=CIRCLE('',#50128,1.06088080992078);
#20103=CIRCLE('',#50129,1.06088080992078);
#20104=CIRCLE('',#50131,1.10035806567471);
#20105=CIRCLE('',#50132,1.10035806567471);
#20106=CIRCLE('',#50134,0.500358065674722);
#20107=CIRCLE('',#50135,0.500358065674722);
#20108=CIRCLE('',#50137,1.21403156673711);
#20109=CIRCLE('',#50138,1.21403156673711);
#20110=CIRCLE('',#50140,0.614031566737117);
#20111=CIRCLE('',#50141,0.614031566737117);
#20112=CIRCLE('',#50143,1.32880796357332);
#20113=CIRCLE('',#50144,1.32880796357332);
#20114=CIRCLE('',#50146,0.72880796357333);
#20115=CIRCLE('',#50147,0.72880796357333);
#20116=CIRCLE('',#50149,1.46111700181689);
#20117=CIRCLE('',#50150,1.46111700181689);
#20118=CIRCLE('',#50152,0.861117001816902);
#20119=CIRCLE('',#50153,0.861117001816902);
#20120=CIRCLE('',#50155,1.6204820426246);
#20121=CIRCLE('',#50156,1.6204820426246);
#20122=CIRCLE('',#50158,1.02048204262462);
#20123=CIRCLE('',#50159,1.02048204262462);
#20124=CIRCLE('',#50161,1.70100022308284);
#20125=CIRCLE('',#50162,1.70100022308284);
#20126=CIRCLE('',#50164,1.10100022308285);
#20127=CIRCLE('',#50165,1.10100022308285);
#20128=CIRCLE('',#50167,1.72127463204347);
#20129=CIRCLE('',#50168,1.72127463204347);
#20130=CIRCLE('',#50170,1.12127463204348);
#20131=CIRCLE('',#50171,1.12127463204348);
#20132=CIRCLE('',#50173,1.78199265440493);
#20133=CIRCLE('',#50174,1.78199265440493);
#20134=CIRCLE('',#50176,1.18199265440494);
#20135=CIRCLE('',#50177,1.18199265440494);
#20136=CIRCLE('',#50179,1.66088080992077);
#20137=CIRCLE('',#50180,1.66088080992077);
#20138=CIRCLE('',#50182,1.06088080992078);
#20139=CIRCLE('',#50183,1.06088080992078);
#20140=CIRCLE('',#50185,1.10035806567471);
#20141=CIRCLE('',#50186,1.10035806567471);
#20142=CIRCLE('',#50188,0.500358065674666);
#20143=CIRCLE('',#50189,0.500358065674666);
#20144=CIRCLE('',#50191,1.21403156673716);
#20145=CIRCLE('',#50192,1.21403156673716);
#20146=CIRCLE('',#50194,0.614031566737117);
#20147=CIRCLE('',#50195,0.614031566737117);
#20148=CIRCLE('',#50197,1.32880796357332);
#20149=CIRCLE('',#50198,1.32880796357332);
#20150=CIRCLE('',#50200,0.72880796357333);
#20151=CIRCLE('',#50201,0.72880796357333);
#20152=CIRCLE('',#50203,1.46111700181689);
#20153=CIRCLE('',#50204,1.46111700181689);
#20154=CIRCLE('',#50206,0.861117001816902);
#20155=CIRCLE('',#50207,0.861117001816902);
#20156=CIRCLE('',#50209,1.6204820426246);
#20157=CIRCLE('',#50210,1.6204820426246);
#20158=CIRCLE('',#50212,1.02048204262462);
#20159=CIRCLE('',#50213,1.02048204262462);
#20160=CIRCLE('',#50215,1.70100022308284);
#20161=CIRCLE('',#50216,1.70100022308284);
#20162=CIRCLE('',#50218,1.10100022308285);
#20163=CIRCLE('',#50219,1.10100022308285);
#20164=CIRCLE('',#50221,1.72127463204352);
#20165=CIRCLE('',#50222,1.72127463204352);
#20166=CIRCLE('',#50224,1.12127463204353);
#20167=CIRCLE('',#50225,1.12127463204353);
#20168=CIRCLE('',#50227,1.78199265440493);
#20169=CIRCLE('',#50228,1.78199265440493);
#20170=CIRCLE('',#50230,1.18199265440494);
#20171=CIRCLE('',#50231,1.18199265440494);
#20172=CIRCLE('',#50233,1.66088080992077);
#20173=CIRCLE('',#50234,1.66088080992077);
#20174=CIRCLE('',#50236,1.06088080992078);
#20175=CIRCLE('',#50237,1.06088080992078);
#20176=CIRCLE('',#50239,1.10035806567471);
#20177=CIRCLE('',#50240,1.10035806567471);
#20178=CIRCLE('',#50242,0.500358065674666);
#20179=CIRCLE('',#50243,0.500358065674666);
#20180=CIRCLE('',#50245,1.21403156673716);
#20181=CIRCLE('',#50246,1.21403156673716);
#20182=CIRCLE('',#50248,0.614031566737172);
#20183=CIRCLE('',#50249,0.614031566737172);
#20184=CIRCLE('',#50251,1.32880796357326);
#20185=CIRCLE('',#50252,1.32880796357326);
#20186=CIRCLE('',#50254,0.728807963573275);
#20187=CIRCLE('',#50255,0.728807963573275);
#20188=CIRCLE('',#50257,1.46111700181689);
#20189=CIRCLE('',#50258,1.46111700181689);
#20190=CIRCLE('',#50260,0.861117001816847);
#20191=CIRCLE('',#50261,0.861117001816847);
#20192=CIRCLE('',#50263,1.62048204262455);
#20193=CIRCLE('',#50264,1.62048204262455);
#20194=CIRCLE('',#50266,1.02048204262462);
#20195=CIRCLE('',#50267,1.02048204262462);
#20196=CIRCLE('',#50269,1.70100022308284);
#20197=CIRCLE('',#50270,1.70100022308284);
#20198=CIRCLE('',#50272,1.10100022308279);
#20199=CIRCLE('',#50273,1.10100022308279);
#20200=CIRCLE('',#50275,1.72127463204352);
#20201=CIRCLE('',#50276,1.72127463204352);
#20202=CIRCLE('',#50278,1.12127463204348);
#20203=CIRCLE('',#50279,1.12127463204348);
#20204=CIRCLE('',#50281,1.78199265440493);
#20205=CIRCLE('',#50282,1.78199265440493);
#20206=CIRCLE('',#50284,1.18199265440494);
#20207=CIRCLE('',#50285,1.18199265440494);
#20208=CIRCLE('',#50287,1.66088080992083);
#20209=CIRCLE('',#50288,1.66088080992083);
#20210=CIRCLE('',#50290,1.06088080992078);
#20211=CIRCLE('',#50291,1.06088080992078);
#20212=CIRCLE('',#50293,1.10035806567471);
#20213=CIRCLE('',#50294,1.10035806567471);
#20214=CIRCLE('',#50296,0.500358065674722);
#20215=CIRCLE('',#50297,0.500358065674722);
#20216=CIRCLE('',#50299,1.21403156673716);
#20217=CIRCLE('',#50300,1.21403156673716);
#20218=CIRCLE('',#50302,0.614031566737172);
#20219=CIRCLE('',#50303,0.614031566737172);
#20220=CIRCLE('',#50305,1.32880796357326);
#20221=CIRCLE('',#50306,1.32880796357326);
#20222=CIRCLE('',#50308,0.72880796357333);
#20223=CIRCLE('',#50309,0.72880796357333);
#20224=CIRCLE('',#50311,1.46111700181689);
#20225=CIRCLE('',#50312,1.46111700181689);
#20226=CIRCLE('',#50314,0.861117001816902);
#20227=CIRCLE('',#50315,0.861117001816902);
#20228=CIRCLE('',#50317,1.6204820426246);
#20229=CIRCLE('',#50318,1.6204820426246);
#20230=CIRCLE('',#50320,1.02048204262456);
#20231=CIRCLE('',#50321,1.02048204262456);
#20232=CIRCLE('',#50323,1.70100022308278);
#20233=CIRCLE('',#50324,1.70100022308278);
#20234=CIRCLE('',#50326,1.10100022308279);
#20235=CIRCLE('',#50327,1.10100022308279);
#20236=CIRCLE('',#50329,1.72127463204347);
#20237=CIRCLE('',#50330,1.72127463204347);
#20238=CIRCLE('',#50332,1.12127463204348);
#20239=CIRCLE('',#50333,1.12127463204348);
#20240=CIRCLE('',#50335,1.78199265440493);
#20241=CIRCLE('',#50336,1.78199265440493);
#20242=CIRCLE('',#50338,1.18199265440494);
#20243=CIRCLE('',#50339,1.18199265440494);
#20244=CIRCLE('',#50341,1.66088080992077);
#20245=CIRCLE('',#50342,1.66088080992077);
#20246=CIRCLE('',#50344,1.06088080992084);
#20247=CIRCLE('',#50345,1.06088080992084);
#20248=CIRCLE('',#50347,1.10035806567471);
#20249=CIRCLE('',#50348,1.10035806567471);
#20250=CIRCLE('',#50350,0.500358065674722);
#20251=CIRCLE('',#50351,0.500358065674722);
#20252=CIRCLE('',#50353,1.21403156673716);
#20253=CIRCLE('',#50354,1.21403156673716);
#20254=CIRCLE('',#50356,0.614031566737117);
#20255=CIRCLE('',#50357,0.614031566737117);
#20256=CIRCLE('',#50359,1.32880796357338);
#20257=CIRCLE('',#50360,1.32880796357338);
#20258=CIRCLE('',#50362,0.728807963573386);
#20259=CIRCLE('',#50363,0.728807963573386);
#20260=CIRCLE('',#50365,1.46111700181695);
#20261=CIRCLE('',#50366,1.46111700181695);
#20262=CIRCLE('',#50368,0.861117001816902);
#20263=CIRCLE('',#50369,0.861117001816902);
#20264=CIRCLE('',#50371,1.6204820426246);
#20265=CIRCLE('',#50372,1.6204820426246);
#20266=CIRCLE('',#50374,1.02048204262456);
#20267=CIRCLE('',#50375,1.02048204262456);
#20268=CIRCLE('',#50377,1.70100022308284);
#20269=CIRCLE('',#50378,1.70100022308284);
#20270=CIRCLE('',#50380,1.10100022308279);
#20271=CIRCLE('',#50381,1.10100022308279);
#20272=CIRCLE('',#50383,1.72127463204352);
#20273=CIRCLE('',#50384,1.72127463204352);
#20274=CIRCLE('',#50386,1.12127463204348);
#20275=CIRCLE('',#50387,1.12127463204348);
#20276=CIRCLE('',#50389,1.78199265440493);
#20277=CIRCLE('',#50390,1.78199265440493);
#20278=CIRCLE('',#50392,1.18199265440494);
#20279=CIRCLE('',#50393,1.18199265440494);
#20280=CIRCLE('',#50395,1.66088080992083);
#20281=CIRCLE('',#50396,1.66088080992083);
#20282=CIRCLE('',#50398,1.06088080992078);
#20283=CIRCLE('',#50399,1.06088080992078);
#20284=CIRCLE('',#50401,1.10035806567466);
#20285=CIRCLE('',#50402,1.10035806567466);
#20286=CIRCLE('',#50404,0.500358065674666);
#20287=CIRCLE('',#50405,0.500358065674666);
#20288=CIRCLE('',#50407,1.21403156673716);
#20289=CIRCLE('',#50408,1.21403156673716);
#20290=CIRCLE('',#50410,0.614031566737172);
#20291=CIRCLE('',#50411,0.614031566737172);
#20292=CIRCLE('',#50413,1.32880796357326);
#20293=CIRCLE('',#50414,1.32880796357326);
#20294=CIRCLE('',#50416,0.728807963573275);
#20295=CIRCLE('',#50417,0.728807963573275);
#20296=CIRCLE('',#50419,1.46111700181689);
#20297=CIRCLE('',#50420,1.46111700181689);
#20298=CIRCLE('',#50422,0.861117001816847);
#20299=CIRCLE('',#50423,0.861117001816847);
#20300=CIRCLE('',#50425,1.6204820426246);
#20301=CIRCLE('',#50426,1.6204820426246);
#20302=CIRCLE('',#50428,1.02048204262456);
#20303=CIRCLE('',#50429,1.02048204262456);
#20304=CIRCLE('',#50431,1.70100022308284);
#20305=CIRCLE('',#50432,1.70100022308284);
#20306=CIRCLE('',#50434,1.10100022308285);
#20307=CIRCLE('',#50435,1.10100022308285);
#20308=CIRCLE('',#50437,1.72127463204352);
#20309=CIRCLE('',#50438,1.72127463204352);
#20310=CIRCLE('',#50440,1.12127463204348);
#20311=CIRCLE('',#50441,1.12127463204348);
#20312=CIRCLE('',#50443,1.78199265440498);
#20313=CIRCLE('',#50444,1.78199265440498);
#20314=CIRCLE('',#50446,1.18199265440494);
#20315=CIRCLE('',#50447,1.18199265440494);
#20316=CIRCLE('',#50449,1.66088080992077);
#20317=CIRCLE('',#50450,1.66088080992077);
#20318=CIRCLE('',#50452,1.06088080992078);
#20319=CIRCLE('',#50453,1.06088080992078);
#20320=CIRCLE('',#50455,1.10035806567471);
#20321=CIRCLE('',#50456,1.10035806567471);
#20322=CIRCLE('',#50458,0.500358065674666);
#20323=CIRCLE('',#50459,0.500358065674666);
#20324=CIRCLE('',#50461,1.21403156673716);
#20325=CIRCLE('',#50462,1.21403156673716);
#20326=CIRCLE('',#50464,0.614031566737117);
#20327=CIRCLE('',#50465,0.614031566737117);
#20328=CIRCLE('',#50467,1.32880796357332);
#20329=CIRCLE('',#50468,1.32880796357332);
#20330=CIRCLE('',#50470,0.72880796357333);
#20331=CIRCLE('',#50471,0.72880796357333);
#20332=CIRCLE('',#50473,1.46111700181689);
#20333=CIRCLE('',#50474,1.46111700181689);
#20334=CIRCLE('',#50476,0.861117001816902);
#20335=CIRCLE('',#50477,0.861117001816902);
#20336=CIRCLE('',#50479,1.62048204262455);
#20337=CIRCLE('',#50480,1.62048204262455);
#20338=CIRCLE('',#50482,1.02048204262456);
#20339=CIRCLE('',#50483,1.02048204262456);
#20340=CIRCLE('',#50485,1.70100022308278);
#20341=CIRCLE('',#50486,1.70100022308278);
#20342=CIRCLE('',#50488,1.10100022308285);
#20343=CIRCLE('',#50489,1.10100022308285);
#20344=CIRCLE('',#50491,1.72127463204347);
#20345=CIRCLE('',#50492,1.72127463204347);
#20346=CIRCLE('',#50494,1.12127463204348);
#20347=CIRCLE('',#50495,1.12127463204348);
#20348=CIRCLE('',#50497,1.78199265440493);
#20349=CIRCLE('',#50498,1.78199265440493);
#20350=CIRCLE('',#50500,1.18199265440488);
#20351=CIRCLE('',#50501,1.18199265440488);
#20352=CIRCLE('',#50503,1.66088080992083);
#20353=CIRCLE('',#50504,1.66088080992083);
#20354=CIRCLE('',#50506,1.06088080992078);
#20355=CIRCLE('',#50507,1.06088080992078);
#20356=CIRCLE('',#50509,1.10035806567471);
#20357=CIRCLE('',#50510,1.10035806567471);
#20358=CIRCLE('',#50512,0.500358065674666);
#20359=CIRCLE('',#50513,0.500358065674666);
#20360=CIRCLE('',#50515,1.21403156673716);
#20361=CIRCLE('',#50516,1.21403156673716);
#20362=CIRCLE('',#50518,0.614031566737117);
#20363=CIRCLE('',#50519,0.614031566737117);
#20364=CIRCLE('',#50521,1.32880796357332);
#20365=CIRCLE('',#50522,1.32880796357332);
#20366=CIRCLE('',#50524,0.72880796357333);
#20367=CIRCLE('',#50525,0.72880796357333);
#20368=CIRCLE('',#50527,1.46111700181689);
#20369=CIRCLE('',#50528,1.46111700181689);
#20370=CIRCLE('',#50530,0.861117001816902);
#20371=CIRCLE('',#50531,0.861117001816902);
#20372=CIRCLE('',#50533,1.6204820426246);
#20373=CIRCLE('',#50534,1.6204820426246);
#20374=CIRCLE('',#50536,1.02048204262462);
#20375=CIRCLE('',#50537,1.02048204262462);
#20376=CIRCLE('',#50539,1.70100022308284);
#20377=CIRCLE('',#50540,1.70100022308284);
#20378=CIRCLE('',#50542,1.10100022308285);
#20379=CIRCLE('',#50543,1.10100022308285);
#20380=CIRCLE('',#50545,1.72127463204352);
#20381=CIRCLE('',#50546,1.72127463204352);
#20382=CIRCLE('',#50548,1.12127463204353);
#20383=CIRCLE('',#50549,1.12127463204353);
#20384=CIRCLE('',#50551,1.78199265440493);
#20385=CIRCLE('',#50552,1.78199265440493);
#20386=CIRCLE('',#50554,1.18199265440488);
#20387=CIRCLE('',#50555,1.18199265440488);
#20388=CIRCLE('',#50557,1.66088080992077);
#20389=CIRCLE('',#50558,1.66088080992077);
#20390=CIRCLE('',#50560,1.06088080992078);
#20391=CIRCLE('',#50561,1.06088080992078);
#20392=CIRCLE('',#50563,1.10035806567477);
#20393=CIRCLE('',#50564,1.10035806567477);
#20394=CIRCLE('',#50566,0.500358065674722);
#20395=CIRCLE('',#50567,0.500358065674722);
#20396=CIRCLE('',#50569,1.21403156673711);
#20397=CIRCLE('',#50570,1.21403156673711);
#20398=CIRCLE('',#50572,0.614031566737061);
#20399=CIRCLE('',#50573,0.614031566737061);
#20400=CIRCLE('',#50575,1.32880796357332);
#20401=CIRCLE('',#50576,1.32880796357332);
#20402=CIRCLE('',#50578,0.728807963573275);
#20403=CIRCLE('',#50579,0.728807963573275);
#20404=CIRCLE('',#50581,1.46111700181684);
#20405=CIRCLE('',#50582,1.46111700181684);
#20406=CIRCLE('',#50584,0.861117001816847);
#20407=CIRCLE('',#50585,0.861117001816847);
#20408=CIRCLE('',#50587,1.6204820426246);
#20409=CIRCLE('',#50588,1.6204820426246);
#20410=CIRCLE('',#50590,1.02048204262456);
#20411=CIRCLE('',#50591,1.02048204262456);
#20412=CIRCLE('',#50593,1.70100022308278);
#20413=CIRCLE('',#50594,1.70100022308278);
#20414=CIRCLE('',#50596,1.10100022308279);
#20415=CIRCLE('',#50597,1.10100022308279);
#20416=CIRCLE('',#50599,1.72127463204352);
#20417=CIRCLE('',#50600,1.72127463204352);
#20418=CIRCLE('',#50602,1.12127463204353);
#20419=CIRCLE('',#50603,1.12127463204353);
#20420=CIRCLE('',#50605,1.78199265440493);
#20421=CIRCLE('',#50606,1.78199265440493);
#20422=CIRCLE('',#50608,1.18199265440494);
#20423=CIRCLE('',#50609,1.18199265440494);
#20424=CIRCLE('',#50611,1.66088080992077);
#20425=CIRCLE('',#50612,1.66088080992077);
#20426=CIRCLE('',#50614,1.06088080992073);
#20427=CIRCLE('',#50615,1.06088080992073);
#20428=CIRCLE('',#50617,1.10035806567471);
#20429=CIRCLE('',#50618,1.10035806567471);
#20430=CIRCLE('',#50620,0.500358065674722);
#20431=CIRCLE('',#50621,0.500358065674722);
#20432=CIRCLE('',#50623,1.21403156673711);
#20433=CIRCLE('',#50624,1.21403156673711);
#20434=CIRCLE('',#50626,0.614031566737117);
#20435=CIRCLE('',#50627,0.614031566737117);
#20436=CIRCLE('',#50629,1.32880796357332);
#20437=CIRCLE('',#50630,1.32880796357332);
#20438=CIRCLE('',#50632,0.728807963573275);
#20439=CIRCLE('',#50633,0.728807963573275);
#20440=CIRCLE('',#50635,1.46111700181684);
#20441=CIRCLE('',#50636,1.46111700181684);
#20442=CIRCLE('',#50638,0.861117001816902);
#20443=CIRCLE('',#50639,0.861117001816902);
#20444=CIRCLE('',#50641,1.6204820426246);
#20445=CIRCLE('',#50642,1.6204820426246);
#20446=CIRCLE('',#50644,1.02048204262462);
#20447=CIRCLE('',#50645,1.02048204262462);
#20448=CIRCLE('',#50647,1.70100022308289);
#20449=CIRCLE('',#50648,1.70100022308289);
#20450=CIRCLE('',#50650,1.10100022308285);
#20451=CIRCLE('',#50651,1.10100022308285);
#20452=CIRCLE('',#50653,1.72127463204347);
#20453=CIRCLE('',#50654,1.72127463204347);
#20454=CIRCLE('',#50656,1.12127463204342);
#20455=CIRCLE('',#50657,1.12127463204342);
#20456=CIRCLE('',#50659,1.78199265440498);
#20457=CIRCLE('',#50660,1.78199265440498);
#20458=CIRCLE('',#50662,1.18199265440494);
#20459=CIRCLE('',#50663,1.18199265440494);
#20460=CIRCLE('',#50665,1.66088080992077);
#20461=CIRCLE('',#50666,1.66088080992077);
#20462=CIRCLE('',#50668,1.06088080992078);
#20463=CIRCLE('',#50669,1.06088080992078);
#20464=CIRCLE('',#50671,1.10035806567471);
#20465=CIRCLE('',#50672,1.10035806567471);
#20466=CIRCLE('',#50674,0.500358065674666);
#20467=CIRCLE('',#50675,0.500358065674666);
#20468=CIRCLE('',#50677,1.21403156673711);
#20469=CIRCLE('',#50678,1.21403156673711);
#20470=CIRCLE('',#50680,0.614031566737117);
#20471=CIRCLE('',#50681,0.614031566737117);
#20472=CIRCLE('',#50683,1.32880796357332);
#20473=CIRCLE('',#50684,1.32880796357332);
#20474=CIRCLE('',#50686,0.72880796357333);
#20475=CIRCLE('',#50687,0.72880796357333);
#20476=CIRCLE('',#50689,1.46111700181684);
#20477=CIRCLE('',#50690,1.46111700181684);
#20478=CIRCLE('',#50692,0.861117001816847);
#20479=CIRCLE('',#50693,0.861117001816847);
#20480=CIRCLE('',#50695,1.6204820426246);
#20481=CIRCLE('',#50696,1.6204820426246);
#20482=CIRCLE('',#50698,1.02048204262456);
#20483=CIRCLE('',#50699,1.02048204262456);
#20484=CIRCLE('',#50701,1.70100022308284);
#20485=CIRCLE('',#50702,1.70100022308284);
#20486=CIRCLE('',#50704,1.10100022308285);
#20487=CIRCLE('',#50705,1.10100022308285);
#20488=CIRCLE('',#50707,1.72127463204347);
#20489=CIRCLE('',#50708,1.72127463204347);
#20490=CIRCLE('',#50710,1.12127463204353);
#20491=CIRCLE('',#50711,1.12127463204353);
#20492=CIRCLE('',#50713,1.78199265440498);
#20493=CIRCLE('',#50714,1.78199265440498);
#20494=CIRCLE('',#50716,1.18199265440494);
#20495=CIRCLE('',#50717,1.18199265440494);
#20496=CIRCLE('',#50719,1.66088080992083);
#20497=CIRCLE('',#50720,1.66088080992083);
#20498=CIRCLE('',#50722,1.06088080992078);
#20499=CIRCLE('',#50723,1.06088080992078);
#20500=CIRCLE('',#50725,1.10035806567477);
#20501=CIRCLE('',#50726,1.10035806567477);
#20502=CIRCLE('',#50728,0.500358065674777);
#20503=CIRCLE('',#50729,0.500358065674777);
#20504=CIRCLE('',#50731,1.21403156673705);
#20505=CIRCLE('',#50732,1.21403156673705);
#20506=CIRCLE('',#50734,0.614031566737117);
#20507=CIRCLE('',#50735,0.614031566737117);
#20508=CIRCLE('',#50737,1.32880796357326);
#20509=CIRCLE('',#50738,1.32880796357326);
#20510=CIRCLE('',#50740,0.728807963573275);
#20511=CIRCLE('',#50741,0.728807963573275);
#20512=CIRCLE('',#50743,1.46111700181684);
#20513=CIRCLE('',#50744,1.46111700181684);
#20514=CIRCLE('',#50746,0.861117001816847);
#20515=CIRCLE('',#50747,0.861117001816847);
#20516=CIRCLE('',#50749,1.6204820426246);
#20517=CIRCLE('',#50750,1.6204820426246);
#20518=CIRCLE('',#50752,1.02048204262462);
#20519=CIRCLE('',#50753,1.02048204262462);
#20520=CIRCLE('',#50755,1.70100022308278);
#20521=CIRCLE('',#50756,1.70100022308278);
#20522=CIRCLE('',#50758,1.10100022308285);
#20523=CIRCLE('',#50759,1.10100022308285);
#20524=CIRCLE('',#50761,1.72127463204347);
#20525=CIRCLE('',#50762,1.72127463204347);
#20526=CIRCLE('',#50764,1.12127463204353);
#20527=CIRCLE('',#50765,1.12127463204353);
#20528=CIRCLE('',#50767,1.78199265440493);
#20529=CIRCLE('',#50768,1.78199265440493);
#20530=CIRCLE('',#50770,1.18199265440494);
#20531=CIRCLE('',#50771,1.18199265440494);
#20532=CIRCLE('',#50773,1.66088080992077);
#20533=CIRCLE('',#50774,1.66088080992077);
#20534=CIRCLE('',#50776,1.06088080992078);
#20535=CIRCLE('',#50777,1.06088080992078);
#20536=CIRCLE('',#50779,1.10035806567471);
#20537=CIRCLE('',#50780,1.10035806567471);
#20538=CIRCLE('',#50782,0.500358065674722);
#20539=CIRCLE('',#50783,0.500358065674722);
#20540=CIRCLE('',#50785,1.21403156673716);
#20541=CIRCLE('',#50786,1.21403156673716);
#20542=CIRCLE('',#50788,0.614031566737117);
#20543=CIRCLE('',#50789,0.614031566737117);
#20544=CIRCLE('',#50791,1.32880796357332);
#20545=CIRCLE('',#50792,1.32880796357332);
#20546=CIRCLE('',#50794,0.72880796357333);
#20547=CIRCLE('',#50795,0.72880796357333);
#20548=CIRCLE('',#50797,1.46111700181689);
#20549=CIRCLE('',#50798,1.46111700181689);
#20550=CIRCLE('',#50800,0.861117001816902);
#20551=CIRCLE('',#50801,0.861117001816902);
#20552=CIRCLE('',#50803,1.6204820426246);
#20553=CIRCLE('',#50804,1.6204820426246);
#20554=CIRCLE('',#50806,1.02048204262462);
#20555=CIRCLE('',#50807,1.02048204262462);
#20556=CIRCLE('',#50809,1.70100022308284);
#20557=CIRCLE('',#50810,1.70100022308284);
#20558=CIRCLE('',#50812,1.10100022308285);
#20559=CIRCLE('',#50813,1.10100022308285);
#20560=CIRCLE('',#50815,1.72127463204352);
#20561=CIRCLE('',#50816,1.72127463204352);
#20562=CIRCLE('',#50818,1.12127463204348);
#20563=CIRCLE('',#50819,1.12127463204348);
#20564=CIRCLE('',#50821,1.78199265440493);
#20565=CIRCLE('',#50822,1.78199265440493);
#20566=CIRCLE('',#50824,1.18199265440488);
#20567=CIRCLE('',#50825,1.18199265440488);
#20568=CIRCLE('',#50827,1.66088080992088);
#20569=CIRCLE('',#50828,1.66088080992088);
#20570=CIRCLE('',#50830,1.06088080992084);
#20571=CIRCLE('',#50831,1.06088080992084);
#20572=CIRCLE('',#50833,1.10035806567471);
#20573=CIRCLE('',#50834,1.10035806567471);
#20574=CIRCLE('',#50836,0.500358065674722);
#20575=CIRCLE('',#50837,0.500358065674722);
#20576=CIRCLE('',#50839,1.21403156673716);
#20577=CIRCLE('',#50840,1.21403156673716);
#20578=CIRCLE('',#50842,0.614031566737117);
#20579=CIRCLE('',#50843,0.614031566737117);
#20580=CIRCLE('',#50845,1.32880796357332);
#20581=CIRCLE('',#50846,1.32880796357332);
#20582=CIRCLE('',#50848,0.72880796357333);
#20583=CIRCLE('',#50849,0.72880796357333);
#20584=CIRCLE('',#50851,1.46111700181689);
#20585=CIRCLE('',#50852,1.46111700181689);
#20586=CIRCLE('',#50854,0.861117001816902);
#20587=CIRCLE('',#50855,0.861117001816902);
#20588=CIRCLE('',#50857,1.6204820426246);
#20589=CIRCLE('',#50858,1.6204820426246);
#20590=CIRCLE('',#50860,1.02048204262462);
#20591=CIRCLE('',#50861,1.02048204262462);
#20592=CIRCLE('',#50863,1.70100022308284);
#20593=CIRCLE('',#50864,1.70100022308284);
#20594=CIRCLE('',#50866,1.10100022308285);
#20595=CIRCLE('',#50867,1.10100022308285);
#20596=CIRCLE('',#50869,1.72127463204352);
#20597=CIRCLE('',#50870,1.72127463204352);
#20598=CIRCLE('',#50872,1.12127463204348);
#20599=CIRCLE('',#50873,1.12127463204348);
#20600=CIRCLE('',#50875,1.78199265440493);
#20601=CIRCLE('',#50876,1.78199265440493);
#20602=CIRCLE('',#50878,1.18199265440494);
#20603=CIRCLE('',#50879,1.18199265440494);
#20604=CIRCLE('',#50881,1.66088080992077);
#20605=CIRCLE('',#50882,1.66088080992077);
#20606=CIRCLE('',#50884,1.06088080992078);
#20607=CIRCLE('',#50885,1.06088080992078);
#20608=CIRCLE('',#50887,0.5);
#20609=CIRCLE('',#50888,127.41606204049);
#20610=CIRCLE('',#50889,126.822029782344);
#20611=CIRCLE('',#50891,127.41606204049);
#20612=CIRCLE('',#50893,11.8670707361131);
#20613=CIRCLE('',#50894,0.5);
#20614=CIRCLE('',#50895,12.3670707361131);
#20615=CIRCLE('',#50896,12.3670707361131);
#20616=CIRCLE('',#50898,11.8670707361131);
#20617=CIRCLE('',#50899,0.5);
#20618=CIRCLE('',#50900,12.3670707361132);
#20619=CIRCLE('',#50903,11.0429795822116);
#20620=CIRCLE('',#50905,16.6476722933764);
#20621=CIRCLE('',#50906,0.5);
#20622=CIRCLE('',#50907,16.1492953136407);
#20623=CIRCLE('',#50909,130.);
#20624=CIRCLE('',#50910,1.);
#20625=CIRCLE('',#50911,129.);
#20626=CIRCLE('',#50913,1.);
#20627=CIRCLE('',#50914,127.91606204049);
#20628=CIRCLE('',#50916,18.5103550292801);
#20629=CIRCLE('',#50918,130.);
#20630=CIRCLE('',#50919,130.);
#20631=CIRCLE('',#50920,1.);
#20632=CIRCLE('',#50921,129.);
#20633=CIRCLE('',#50924,0.878303132193281);
#20634=CIRCLE('',#50933,85.1127409318642);
#22734=VERTEX_POINT('',#106604);
#22735=VERTEX_POINT('',#106605);
#22736=VERTEX_POINT('',#106607);
#22737=VERTEX_POINT('',#106611);
#22738=VERTEX_POINT('',#106616);
#22739=VERTEX_POINT('',#106617);
#22740=VERTEX_POINT('',#106679);
#22741=VERTEX_POINT('',#106680);
#22742=VERTEX_POINT('',#106744);
#22743=VERTEX_POINT('',#106745);
#22744=VERTEX_POINT('',#106809);
#22745=VERTEX_POINT('',#106810);
#22746=VERTEX_POINT('',#106872);
#22747=VERTEX_POINT('',#106873);
#22748=VERTEX_POINT('',#106935);
#22749=VERTEX_POINT('',#106936);
#22750=VERTEX_POINT('',#106998);
#22751=VERTEX_POINT('',#106999);
#22752=VERTEX_POINT('',#107061);
#22753=VERTEX_POINT('',#107062);
#22754=VERTEX_POINT('',#107124);
#22755=VERTEX_POINT('',#107125);
#22756=VERTEX_POINT('',#107187);
#22757=VERTEX_POINT('',#107188);
#22758=VERTEX_POINT('',#107250);
#22759=VERTEX_POINT('',#107251);
#22760=VERTEX_POINT('',#107313);
#22761=VERTEX_POINT('',#107314);
#22762=VERTEX_POINT('',#107378);
#22763=VERTEX_POINT('',#107379);
#22764=VERTEX_POINT('',#107443);
#22765=VERTEX_POINT('',#107444);
#22766=VERTEX_POINT('',#107506);
#22767=VERTEX_POINT('',#107507);
#22768=VERTEX_POINT('',#107571);
#22769=VERTEX_POINT('',#107572);
#22770=VERTEX_POINT('',#107636);
#22771=VERTEX_POINT('',#107637);
#22772=VERTEX_POINT('',#107699);
#22773=VERTEX_POINT('',#107700);
#22774=VERTEX_POINT('',#107764);
#22775=VERTEX_POINT('',#107765);
#22776=VERTEX_POINT('',#107829);
#22777=VERTEX_POINT('',#107830);
#22778=VERTEX_POINT('',#107894);
#22779=VERTEX_POINT('',#107895);
#22780=VERTEX_POINT('',#107950);
#22781=VERTEX_POINT('',#107951);
#22782=VERTEX_POINT('',#108011);
#22783=VERTEX_POINT('',#108012);
#22784=VERTEX_POINT('',#108070);
#22785=VERTEX_POINT('',#108071);
#22786=VERTEX_POINT('',#108129);
#22787=VERTEX_POINT('',#108130);
#22788=VERTEX_POINT('',#108192);
#22789=VERTEX_POINT('',#108193);
#22790=VERTEX_POINT('',#108255);
#22791=VERTEX_POINT('',#108256);
#22792=VERTEX_POINT('',#108318);
#22793=VERTEX_POINT('',#108319);
#22794=VERTEX_POINT('',#108381);
#22795=VERTEX_POINT('',#108382);
#22796=VERTEX_POINT('',#108442);
#22797=VERTEX_POINT('',#108443);
#22798=VERTEX_POINT('',#108503);
#22799=VERTEX_POINT('',#108504);
#22800=VERTEX_POINT('',#108561);
#22801=VERTEX_POINT('',#108562);
#22802=VERTEX_POINT('',#108622);
#22803=VERTEX_POINT('',#108623);
#22804=VERTEX_POINT('',#108687);
#22805=VERTEX_POINT('',#108688);
#22806=VERTEX_POINT('',#108752);
#22807=VERTEX_POINT('',#108753);
#22808=VERTEX_POINT('',#108817);
#22809=VERTEX_POINT('',#108818);
#22810=VERTEX_POINT('',#108882);
#22811=VERTEX_POINT('',#108883);
#22812=VERTEX_POINT('',#108941);
#22813=VERTEX_POINT('',#108942);
#22814=VERTEX_POINT('',#108999);
#22815=VERTEX_POINT('',#109000);
#22816=VERTEX_POINT('',#109060);
#22817=VERTEX_POINT('',#109061);
#22818=VERTEX_POINT('',#109119);
#22819=VERTEX_POINT('',#109120);
#22820=VERTEX_POINT('',#109182);
#22821=VERTEX_POINT('',#109183);
#22822=VERTEX_POINT('',#109245);
#22823=VERTEX_POINT('',#109246);
#22824=VERTEX_POINT('',#109310);
#22825=VERTEX_POINT('',#109311);
#22826=VERTEX_POINT('',#109375);
#22827=VERTEX_POINT('',#109376);
#22828=VERTEX_POINT('',#109438);
#22829=VERTEX_POINT('',#109439);
#22830=VERTEX_POINT('',#109501);
#22831=VERTEX_POINT('',#109502);
#22832=VERTEX_POINT('',#109566);
#22833=VERTEX_POINT('',#109567);
#22834=VERTEX_POINT('',#109631);
#22835=VERTEX_POINT('',#109632);
#22836=VERTEX_POINT('',#109696);
#22837=VERTEX_POINT('',#109697);
#22838=VERTEX_POINT('',#109759);
#22839=VERTEX_POINT('',#109760);
#22840=VERTEX_POINT('',#109819);
#22841=VERTEX_POINT('',#109820);
#22842=VERTEX_POINT('',#109880);
#22843=VERTEX_POINT('',#109881);
#22844=VERTEX_POINT('',#109938);
#22845=VERTEX_POINT('',#109939);
#22846=VERTEX_POINT('',#109998);
#22847=VERTEX_POINT('',#109999);
#22848=VERTEX_POINT('',#110061);
#22849=VERTEX_POINT('',#110062);
#22850=VERTEX_POINT('',#110126);
#22851=VERTEX_POINT('',#110127);
#22852=VERTEX_POINT('',#110189);
#22853=VERTEX_POINT('',#110190);
#22854=VERTEX_POINT('',#110252);
#22855=VERTEX_POINT('',#110253);
#22856=VERTEX_POINT('',#110315);
#22857=VERTEX_POINT('',#110316);
#22858=VERTEX_POINT('',#110374);
#22859=VERTEX_POINT('',#110376);
#22860=VERTEX_POINT('',#110380);
#22861=VERTEX_POINT('',#110421);
#22862=VERTEX_POINT('',#110422);
#22863=VERTEX_POINT('',#110446);
#22864=VERTEX_POINT('',#110470);
#22865=VERTEX_POINT('',#110511);
#22866=VERTEX_POINT('',#110512);
#22867=VERTEX_POINT('',#110535);
#22868=VERTEX_POINT('',#110562);
#22869=VERTEX_POINT('',#110603);
#22870=VERTEX_POINT('',#110604);
#22871=VERTEX_POINT('',#110630);
#22872=VERTEX_POINT('',#110654);
#22873=VERTEX_POINT('',#110695);
#22874=VERTEX_POINT('',#110696);
#22875=VERTEX_POINT('',#110719);
#22876=VERTEX_POINT('',#110743);
#22877=VERTEX_POINT('',#110782);
#22878=VERTEX_POINT('',#110783);
#22879=VERTEX_POINT('',#110809);
#22880=VERTEX_POINT('',#110831);
#22881=VERTEX_POINT('',#110872);
#22882=VERTEX_POINT('',#110873);
#22883=VERTEX_POINT('',#110896);
#22884=VERTEX_POINT('',#110923);
#22885=VERTEX_POINT('',#110964);
#22886=VERTEX_POINT('',#110965);
#22887=VERTEX_POINT('',#110988);
#22888=VERTEX_POINT('',#111015);
#22889=VERTEX_POINT('',#111056);
#22890=VERTEX_POINT('',#111057);
#22891=VERTEX_POINT('',#111083);
#22892=VERTEX_POINT('',#111107);
#22893=VERTEX_POINT('',#111146);
#22894=VERTEX_POINT('',#111147);
#22895=VERTEX_POINT('',#111168);
#22896=VERTEX_POINT('',#111193);
#22897=VERTEX_POINT('',#111234);
#22898=VERTEX_POINT('',#111235);
#22899=VERTEX_POINT('',#111258);
#22900=VERTEX_POINT('',#111285);
#22901=VERTEX_POINT('',#111326);
#22902=VERTEX_POINT('',#111327);
#22903=VERTEX_POINT('',#111350);
#22904=VERTEX_POINT('',#111377);
#22905=VERTEX_POINT('',#111418);
#22906=VERTEX_POINT('',#111419);
#22907=VERTEX_POINT('',#111442);
#22908=VERTEX_POINT('',#111466);
#22909=VERTEX_POINT('',#111505);
#22910=VERTEX_POINT('',#111506);
#22911=VERTEX_POINT('',#111530);
#22912=VERTEX_POINT('',#111554);
#22913=VERTEX_POINT('',#111595);
#22914=VERTEX_POINT('',#111596);
#22915=VERTEX_POINT('',#111622);
#22916=VERTEX_POINT('',#111646);
#22917=VERTEX_POINT('',#111687);
#22918=VERTEX_POINT('',#111688);
#22919=VERTEX_POINT('',#111714);
#22920=VERTEX_POINT('',#111738);
#22921=VERTEX_POINT('',#111779);
#22922=VERTEX_POINT('',#111780);
#22923=VERTEX_POINT('',#111801);
#22924=VERTEX_POINT('',#111884);
#22925=VERTEX_POINT('',#111923);
#22926=VERTEX_POINT('',#111924);
#22927=VERTEX_POINT('',#111948);
#22928=VERTEX_POINT('',#111972);
#22929=VERTEX_POINT('',#112013);
#22930=VERTEX_POINT('',#112014);
#22931=VERTEX_POINT('',#112037);
#22932=VERTEX_POINT('',#112064);
#22933=VERTEX_POINT('',#112103);
#22934=VERTEX_POINT('',#112104);
#22935=VERTEX_POINT('',#112127);
#22936=VERTEX_POINT('',#112152);
#22937=VERTEX_POINT('',#112193);
#22938=VERTEX_POINT('',#112194);
#22939=VERTEX_POINT('',#112217);
#22940=VERTEX_POINT('',#112241);
#22941=VERTEX_POINT('',#112280);
#22942=VERTEX_POINT('',#112281);
#22943=VERTEX_POINT('',#112307);
#22944=VERTEX_POINT('',#112331);
#22945=VERTEX_POINT('',#112372);
#22946=VERTEX_POINT('',#112373);
#22947=VERTEX_POINT('',#112396);
#22948=VERTEX_POINT('',#112423);
#22949=VERTEX_POINT('',#112462);
#22950=VERTEX_POINT('',#112463);
#22951=VERTEX_POINT('',#112487);
#22952=VERTEX_POINT('',#112509);
#22953=VERTEX_POINT('',#112548);
#22954=VERTEX_POINT('',#112549);
#22955=VERTEX_POINT('',#112572);
#22956=VERTEX_POINT('',#112599);
#22957=VERTEX_POINT('',#112638);
#22958=VERTEX_POINT('',#112639);
#22959=VERTEX_POINT('',#112665);
#22960=VERTEX_POINT('',#112689);
#22961=VERTEX_POINT('',#112730);
#22962=VERTEX_POINT('',#112731);
#22963=VERTEX_POINT('',#112754);
#22964=VERTEX_POINT('',#112778);
#22965=VERTEX_POINT('',#112819);
#22966=VERTEX_POINT('',#112820);
#22967=VERTEX_POINT('',#112841);
#22968=VERTEX_POINT('',#112865);
#22969=VERTEX_POINT('',#112867);
#22970=VERTEX_POINT('',#113015);
#22971=VERTEX_POINT('',#113016);
#22972=VERTEX_POINT('',#113039);
#22973=VERTEX_POINT('',#113066);
#22974=VERTEX_POINT('',#113105);
#22975=VERTEX_POINT('',#113106);
#22976=VERTEX_POINT('',#113132);
#22977=VERTEX_POINT('',#113156);
#22978=VERTEX_POINT('',#113197);
#22979=VERTEX_POINT('',#113198);
#22980=VERTEX_POINT('',#113221);
#22981=VERTEX_POINT('',#113245);
#22982=VERTEX_POINT('',#113284);
#22983=VERTEX_POINT('',#113285);
#22984=VERTEX_POINT('',#113306);
#22985=VERTEX_POINT('',#113330);
#22986=VERTEX_POINT('',#113383);
#22987=VERTEX_POINT('',#113422);
#22988=VERTEX_POINT('',#113423);
#22989=VERTEX_POINT('',#113446);
#22990=VERTEX_POINT('',#113471);
#22991=VERTEX_POINT('',#113522);
#22992=VERTEX_POINT('',#113563);
#22993=VERTEX_POINT('',#113564);
#22994=VERTEX_POINT('',#113587);
#22995=VERTEX_POINT('',#113611);
#22996=VERTEX_POINT('',#113652);
#22997=VERTEX_POINT('',#113653);
#22998=VERTEX_POINT('',#113676);
#22999=VERTEX_POINT('',#113700);
#23000=VERTEX_POINT('',#113739);
#23001=VERTEX_POINT('',#113740);
#23002=VERTEX_POINT('',#113763);
#23003=VERTEX_POINT('',#113787);
#23004=VERTEX_POINT('',#113840);
#23005=VERTEX_POINT('',#113879);
#23006=VERTEX_POINT('',#113880);
#23007=VERTEX_POINT('',#113901);
#23008=VERTEX_POINT('',#113928);
#23009=VERTEX_POINT('',#113981);
#23010=VERTEX_POINT('',#114022);
#23011=VERTEX_POINT('',#114023);
#23012=VERTEX_POINT('',#114046);
#23013=VERTEX_POINT('',#114070);
#23014=VERTEX_POINT('',#114123);
#23015=VERTEX_POINT('',#114162);
#23016=VERTEX_POINT('',#114163);
#23017=VERTEX_POINT('',#114186);
#23018=VERTEX_POINT('',#114213);
#23019=VERTEX_POINT('',#114264);
#23020=VERTEX_POINT('',#114305);
#23021=VERTEX_POINT('',#114306);
#23022=VERTEX_POINT('',#114329);
#23023=VERTEX_POINT('',#114353);
#23024=VERTEX_POINT('',#114406);
#23025=VERTEX_POINT('',#114443);
#23026=VERTEX_POINT('',#114444);
#23027=VERTEX_POINT('',#114465);
#23028=VERTEX_POINT('',#114492);
#23029=VERTEX_POINT('',#114547);
#23030=VERTEX_POINT('',#114588);
#23031=VERTEX_POINT('',#114589);
#23032=VERTEX_POINT('',#114612);
#23033=VERTEX_POINT('',#114636);
#23034=VERTEX_POINT('',#114691);
#23035=VERTEX_POINT('',#114730);
#23036=VERTEX_POINT('',#114731);
#23037=VERTEX_POINT('',#114754);
#23038=VERTEX_POINT('',#114778);
#23039=VERTEX_POINT('',#114831);
#23040=VERTEX_POINT('',#114872);
#23041=VERTEX_POINT('',#114873);
#23042=VERTEX_POINT('',#114896);
#23043=VERTEX_POINT('',#114920);
#23044=VERTEX_POINT('',#114975);
#23045=VERTEX_POINT('',#115014);
#23046=VERTEX_POINT('',#115015);
#23047=VERTEX_POINT('',#115036);
#23048=VERTEX_POINT('',#115061);
#23049=VERTEX_POINT('',#115116);
#23050=VERTEX_POINT('',#115157);
#23051=VERTEX_POINT('',#115158);
#23052=VERTEX_POINT('',#115181);
#23053=VERTEX_POINT('',#115208);
#23054=VERTEX_POINT('',#115263);
#23055=VERTEX_POINT('',#115302);
#23056=VERTEX_POINT('',#115303);
#23057=VERTEX_POINT('',#115327);
#23058=VERTEX_POINT('',#115349);
#23059=VERTEX_POINT('',#115404);
#23060=VERTEX_POINT('',#115445);
#23061=VERTEX_POINT('',#115446);
#23062=VERTEX_POINT('',#115472);
#23063=VERTEX_POINT('',#115496);
#23064=VERTEX_POINT('',#115553);
#23065=VERTEX_POINT('',#115592);
#23066=VERTEX_POINT('',#115593);
#23067=VERTEX_POINT('',#115612);
#23068=VERTEX_POINT('',#115641);
#23069=VERTEX_POINT('',#115696);
#23070=VERTEX_POINT('',#115737);
#23071=VERTEX_POINT('',#115738);
#23072=VERTEX_POINT('',#115761);
#23073=VERTEX_POINT('',#115785);
#23074=VERTEX_POINT('',#115840);
#23075=VERTEX_POINT('',#115879);
#23076=VERTEX_POINT('',#115880);
#23077=VERTEX_POINT('',#115901);
#23078=VERTEX_POINT('',#115926);
#23079=VERTEX_POINT('',#115983);
#23080=VERTEX_POINT('',#116024);
#23081=VERTEX_POINT('',#116025);
#23082=VERTEX_POINT('',#116048);
#23083=VERTEX_POINT('',#116072);
#23084=VERTEX_POINT('',#116127);
#23085=VERTEX_POINT('',#116166);
#23086=VERTEX_POINT('',#116167);
#23087=VERTEX_POINT('',#116186);
#23088=VERTEX_POINT('',#116215);
#23089=VERTEX_POINT('',#116270);
#23090=VERTEX_POINT('',#116311);
#23091=VERTEX_POINT('',#116312);
#23092=VERTEX_POINT('',#116335);
#23093=VERTEX_POINT('',#116362);
#23094=VERTEX_POINT('',#116419);
#23095=VERTEX_POINT('',#116458);
#23096=VERTEX_POINT('',#116459);
#23097=VERTEX_POINT('',#116480);
#23098=VERTEX_POINT('',#116507);
#23099=VERTEX_POINT('',#116564);
#23100=VERTEX_POINT('',#116605);
#23101=VERTEX_POINT('',#116606);
#23102=VERTEX_POINT('',#116629);
#23103=VERTEX_POINT('',#116656);
#23104=VERTEX_POINT('',#116713);
#23105=VERTEX_POINT('',#116752);
#23106=VERTEX_POINT('',#116753);
#23107=VERTEX_POINT('',#116772);
#23108=VERTEX_POINT('',#116801);
#23109=VERTEX_POINT('',#116858);
#23110=VERTEX_POINT('',#116897);
#23111=VERTEX_POINT('',#116898);
#23112=VERTEX_POINT('',#116919);
#23113=VERTEX_POINT('',#116948);
#23114=VERTEX_POINT('',#117005);
#23115=VERTEX_POINT('',#117044);
#23116=VERTEX_POINT('',#117045);
#23117=VERTEX_POINT('',#117067);
#23118=VERTEX_POINT('',#117093);
#23119=VERTEX_POINT('',#117150);
#23120=VERTEX_POINT('',#117191);
#23121=VERTEX_POINT('',#117192);
#23122=VERTEX_POINT('',#117215);
#23123=VERTEX_POINT('',#117242);
#23124=VERTEX_POINT('',#117297);
#23125=VERTEX_POINT('',#117338);
#23126=VERTEX_POINT('',#117339);
#23127=VERTEX_POINT('',#117360);
#23128=VERTEX_POINT('',#117387);
#23129=VERTEX_POINT('',#117442);
#23130=VERTEX_POINT('',#117481);
#23131=VERTEX_POINT('',#117482);
#23132=VERTEX_POINT('',#117503);
#23133=VERTEX_POINT('',#117532);
#23134=VERTEX_POINT('',#117589);
#23135=VERTEX_POINT('',#117630);
#23136=VERTEX_POINT('',#117631);
#23137=VERTEX_POINT('',#117657);
#23138=VERTEX_POINT('',#117681);
#23139=VERTEX_POINT('',#117738);
#23140=VERTEX_POINT('',#117779);
#23141=VERTEX_POINT('',#117780);
#23142=VERTEX_POINT('',#117801);
#23143=VERTEX_POINT('',#117830);
#23144=VERTEX_POINT('',#117885);
#23145=VERTEX_POINT('',#117887);
#23146=VERTEX_POINT('',#118033);
#23147=VERTEX_POINT('',#118034);
#23148=VERTEX_POINT('',#118057);
#23149=VERTEX_POINT('',#118084);
#23150=VERTEX_POINT('',#118141);
#23151=VERTEX_POINT('',#118180);
#23152=VERTEX_POINT('',#118181);
#23153=VERTEX_POINT('',#118203);
#23154=VERTEX_POINT('',#118229);
#23155=VERTEX_POINT('',#118286);
#23156=VERTEX_POINT('',#118327);
#23157=VERTEX_POINT('',#118328);
#23158=VERTEX_POINT('',#118349);
#23159=VERTEX_POINT('',#118378);
#23160=VERTEX_POINT('',#118435);
#23161=VERTEX_POINT('',#118476);
#23162=VERTEX_POINT('',#118477);
#23163=VERTEX_POINT('',#118501);
#23164=VERTEX_POINT('',#118527);
#23165=VERTEX_POINT('',#118582);
#23166=VERTEX_POINT('',#118584);
#23167=VERTEX_POINT('',#118730);
#23168=VERTEX_POINT('',#118731);
#23169=VERTEX_POINT('',#118752);
#23170=VERTEX_POINT('',#118781);
#23171=VERTEX_POINT('',#118836);
#23172=VERTEX_POINT('',#118873);
#23173=VERTEX_POINT('',#118874);
#23174=VERTEX_POINT('',#118898);
#23175=VERTEX_POINT('',#118922);
#23176=VERTEX_POINT('',#118979);
#23177=VERTEX_POINT('',#119020);
#23178=VERTEX_POINT('',#119021);
#23179=VERTEX_POINT('',#119047);
#23180=VERTEX_POINT('',#119071);
#23181=VERTEX_POINT('',#119128);
#23182=VERTEX_POINT('',#119169);
#23183=VERTEX_POINT('',#119170);
#23184=VERTEX_POINT('',#119194);
#23185=VERTEX_POINT('',#119220);
#23186=VERTEX_POINT('',#119221);
#23187=VERTEX_POINT('',#119252);
#23188=VERTEX_POINT('',#119254);
#23189=VERTEX_POINT('',#119524);
#23190=VERTEX_POINT('',#119525);
#23191=VERTEX_POINT('',#119548);
#23192=VERTEX_POINT('',#119575);
#23193=VERTEX_POINT('',#119630);
#23194=VERTEX_POINT('',#119669);
#23195=VERTEX_POINT('',#119670);
#23196=VERTEX_POINT('',#119691);
#23197=VERTEX_POINT('',#119720);
#23198=VERTEX_POINT('',#119777);
#23199=VERTEX_POINT('',#119818);
#23200=VERTEX_POINT('',#119819);
#23201=VERTEX_POINT('',#119840);
#23202=VERTEX_POINT('',#119869);
#23203=VERTEX_POINT('',#119926);
#23204=VERTEX_POINT('',#119965);
#23205=VERTEX_POINT('',#119966);
#23206=VERTEX_POINT('',#119987);
#23207=VERTEX_POINT('',#120014);
#23208=VERTEX_POINT('',#120069);
#23209=VERTEX_POINT('',#120110);
#23210=VERTEX_POINT('',#120111);
#23211=VERTEX_POINT('',#120132);
#23212=VERTEX_POINT('',#120161);
#23213=VERTEX_POINT('',#120216);
#23214=VERTEX_POINT('',#120255);
#23215=VERTEX_POINT('',#120256);
#23216=VERTEX_POINT('',#120279);
#23217=VERTEX_POINT('',#120304);
#23218=VERTEX_POINT('',#120361);
#23219=VERTEX_POINT('',#120402);
#23220=VERTEX_POINT('',#120403);
#23221=VERTEX_POINT('',#120429);
#23222=VERTEX_POINT('',#120453);
#23223=VERTEX_POINT('',#120510);
#23224=VERTEX_POINT('',#120549);
#23225=VERTEX_POINT('',#120550);
#23226=VERTEX_POINT('',#120574);
#23227=VERTEX_POINT('',#120600);
#23228=VERTEX_POINT('',#120653);
#23229=VERTEX_POINT('',#120694);
#23230=VERTEX_POINT('',#120695);
#23231=VERTEX_POINT('',#120718);
#23232=VERTEX_POINT('',#120745);
#23233=VERTEX_POINT('',#120800);
#23234=VERTEX_POINT('',#120839);
#23235=VERTEX_POINT('',#120840);
#23236=VERTEX_POINT('',#120863);
#23237=VERTEX_POINT('',#120888);
#23238=VERTEX_POINT('',#120943);
#23239=VERTEX_POINT('',#120984);
#23240=VERTEX_POINT('',#120985);
#23241=VERTEX_POINT('',#121011);
#23242=VERTEX_POINT('',#121035);
#23243=VERTEX_POINT('',#121090);
#23244=VERTEX_POINT('',#121127);
#23245=VERTEX_POINT('',#121128);
#23246=VERTEX_POINT('',#121149);
#23247=VERTEX_POINT('',#121176);
#23248=VERTEX_POINT('',#121227);
#23249=VERTEX_POINT('',#121266);
#23250=VERTEX_POINT('',#121267);
#23251=VERTEX_POINT('',#121286);
#23252=VERTEX_POINT('',#121315);
#23253=VERTEX_POINT('',#121368);
#23254=VERTEX_POINT('',#121407);
#23255=VERTEX_POINT('',#121408);
#23256=VERTEX_POINT('',#121431);
#23257=VERTEX_POINT('',#121456);
#23258=VERTEX_POINT('',#121511);
#23259=VERTEX_POINT('',#121552);
#23260=VERTEX_POINT('',#121553);
#23261=VERTEX_POINT('',#121576);
#23262=VERTEX_POINT('',#121600);
#23263=VERTEX_POINT('',#121655);
#23264=VERTEX_POINT('',#121694);
#23265=VERTEX_POINT('',#121695);
#23266=VERTEX_POINT('',#121718);
#23267=VERTEX_POINT('',#121740);
#23268=VERTEX_POINT('',#121791);
#23269=VERTEX_POINT('',#121830);
#23270=VERTEX_POINT('',#121831);
#23271=VERTEX_POINT('',#121852);
#23272=VERTEX_POINT('',#121879);
#23273=VERTEX_POINT('',#121932);
#23274=VERTEX_POINT('',#121973);
#23275=VERTEX_POINT('',#121974);
#23276=VERTEX_POINT('',#121997);
#23277=VERTEX_POINT('',#122021);
#23278=VERTEX_POINT('',#122074);
#23279=VERTEX_POINT('',#122115);
#23280=VERTEX_POINT('',#122116);
#23281=VERTEX_POINT('',#122139);
#23282=VERTEX_POINT('',#122163);
#23283=VERTEX_POINT('',#122218);
#23284=VERTEX_POINT('',#122257);
#23285=VERTEX_POINT('',#122258);
#23286=VERTEX_POINT('',#122281);
#23287=VERTEX_POINT('',#122303);
#23288=VERTEX_POINT('',#122342);
#23289=VERTEX_POINT('',#122343);
#23290=VERTEX_POINT('',#122364);
#23291=VERTEX_POINT('',#122391);
#23292=VERTEX_POINT('',#122432);
#23293=VERTEX_POINT('',#122433);
#23294=VERTEX_POINT('',#122459);
#23295=VERTEX_POINT('',#122483);
#23296=VERTEX_POINT('',#122534);
#23297=VERTEX_POINT('',#122575);
#23298=VERTEX_POINT('',#122576);
#23299=VERTEX_POINT('',#122599);
#23300=VERTEX_POINT('',#122623);
#23301=VERTEX_POINT('',#122676);
#23302=VERTEX_POINT('',#122717);
#23303=VERTEX_POINT('',#122718);
#23304=VERTEX_POINT('',#122741);
#23305=VERTEX_POINT('',#122765);
#23306=VERTEX_POINT('',#122802);
#23307=VERTEX_POINT('',#122803);
#23308=VERTEX_POINT('',#122824);
#23309=VERTEX_POINT('',#122849);
#23310=VERTEX_POINT('',#122890);
#23311=VERTEX_POINT('',#122891);
#23312=VERTEX_POINT('',#122917);
#23313=VERTEX_POINT('',#122941);
#23314=VERTEX_POINT('',#122982);
#23315=VERTEX_POINT('',#122983);
#23316=VERTEX_POINT('',#123006);
#23317=VERTEX_POINT('',#123030);
#23318=VERTEX_POINT('',#123071);
#23319=VERTEX_POINT('',#123072);
#23320=VERTEX_POINT('',#123095);
#23321=VERTEX_POINT('',#123119);
#23322=VERTEX_POINT('',#123156);
#23323=VERTEX_POINT('',#123157);
#23324=VERTEX_POINT('',#123178);
#23325=VERTEX_POINT('',#123203);
#23326=VERTEX_POINT('',#123244);
#23327=VERTEX_POINT('',#123245);
#23328=VERTEX_POINT('',#123268);
#23329=VERTEX_POINT('',#123292);
#23330=VERTEX_POINT('',#123331);
#23331=VERTEX_POINT('',#123332);
#23332=VERTEX_POINT('',#123353);
#23333=VERTEX_POINT('',#123377);
#23334=VERTEX_POINT('',#123418);
#23335=VERTEX_POINT('',#123419);
#23336=VERTEX_POINT('',#123442);
#23337=VERTEX_POINT('',#123466);
#23338=VERTEX_POINT('',#123503);
#23339=VERTEX_POINT('',#123504);
#23340=VERTEX_POINT('',#123525);
#23341=VERTEX_POINT('',#123550);
#23342=VERTEX_POINT('',#123591);
#23343=VERTEX_POINT('',#123592);
#23344=VERTEX_POINT('',#123618);
#23345=VERTEX_POINT('',#123642);
#23346=VERTEX_POINT('',#123681);
#23347=VERTEX_POINT('',#123682);
#23348=VERTEX_POINT('',#123703);
#23349=VERTEX_POINT('',#123730);
#23350=VERTEX_POINT('',#123771);
#23351=VERTEX_POINT('',#123772);
#23352=VERTEX_POINT('',#123795);
#23353=VERTEX_POINT('',#123822);
#23354=VERTEX_POINT('',#123861);
#23355=VERTEX_POINT('',#123862);
#23356=VERTEX_POINT('',#123885);
#23357=VERTEX_POINT('',#123910);
#23358=VERTEX_POINT('',#123951);
#23359=VERTEX_POINT('',#123952);
#23360=VERTEX_POINT('',#123975);
#23361=VERTEX_POINT('',#123999);
#23362=VERTEX_POINT('',#124038);
#23363=VERTEX_POINT('',#124039);
#23364=VERTEX_POINT('',#124065);
#23365=VERTEX_POINT('',#124087);
#23366=VERTEX_POINT('',#124128);
#23367=VERTEX_POINT('',#124129);
#23368=VERTEX_POINT('',#124152);
#23369=VERTEX_POINT('',#124176);
#23370=VERTEX_POINT('',#124215);
#23371=VERTEX_POINT('',#124216);
#23372=VERTEX_POINT('',#124239);
#23373=VERTEX_POINT('',#124264);
#23374=VERTEX_POINT('',#124305);
#23375=VERTEX_POINT('',#124306);
#23376=VERTEX_POINT('',#124332);
#23377=VERTEX_POINT('',#124356);
#23378=VERTEX_POINT('',#124395);
#23379=VERTEX_POINT('',#124396);
#23380=VERTEX_POINT('',#124422);
#23381=VERTEX_POINT('',#124444);
#23382=VERTEX_POINT('',#124485);
#23383=VERTEX_POINT('',#124486);
#23384=VERTEX_POINT('',#124512);
#23385=VERTEX_POINT('',#124536);
#23386=VERTEX_POINT('',#124575);
#23387=VERTEX_POINT('',#124576);
#23388=VERTEX_POINT('',#124599);
#23389=VERTEX_POINT('',#124626);
#23390=VERTEX_POINT('',#124667);
#23391=VERTEX_POINT('',#124668);
#23392=VERTEX_POINT('',#124692);
#23393=VERTEX_POINT('',#124716);
#23394=VERTEX_POINT('',#124757);
#23395=VERTEX_POINT('',#124758);
#23396=VERTEX_POINT('',#124784);
#23397=VERTEX_POINT('',#124808);
#23398=VERTEX_POINT('',#124847);
#23399=VERTEX_POINT('',#124848);
#23400=VERTEX_POINT('',#124871);
#23401=VERTEX_POINT('',#124898);
#23402=VERTEX_POINT('',#124900);
#23403=VERTEX_POINT('',#124904);
#23404=VERTEX_POINT('',#124906);
#23405=VERTEX_POINT('',#124910);
#23406=VERTEX_POINT('',#124912);
#23407=VERTEX_POINT('',#124916);
#23408=VERTEX_POINT('',#124918);
#23409=VERTEX_POINT('',#124922);
#23410=VERTEX_POINT('',#124924);
#23411=VERTEX_POINT('',#124928);
#23412=VERTEX_POINT('',#124930);
#23413=VERTEX_POINT('',#124934);
#23414=VERTEX_POINT('',#124936);
#23415=VERTEX_POINT('',#124940);
#23416=VERTEX_POINT('',#124942);
#23417=VERTEX_POINT('',#124946);
#23418=VERTEX_POINT('',#124948);
#23419=VERTEX_POINT('',#124952);
#23420=VERTEX_POINT('',#124954);
#23421=VERTEX_POINT('',#124958);
#23422=VERTEX_POINT('',#124960);
#23423=VERTEX_POINT('',#124964);
#23424=VERTEX_POINT('',#124966);
#23425=VERTEX_POINT('',#124970);
#23426=VERTEX_POINT('',#124972);
#23427=VERTEX_POINT('',#124976);
#23428=VERTEX_POINT('',#124978);
#23429=VERTEX_POINT('',#124982);
#23430=VERTEX_POINT('',#124984);
#23431=VERTEX_POINT('',#124988);
#23432=VERTEX_POINT('',#124990);
#23433=VERTEX_POINT('',#124994);
#23434=VERTEX_POINT('',#124996);
#23435=VERTEX_POINT('',#125000);
#23436=VERTEX_POINT('',#125002);
#23437=VERTEX_POINT('',#125006);
#23438=VERTEX_POINT('',#125008);
#23439=VERTEX_POINT('',#125012);
#23440=VERTEX_POINT('',#125014);
#23441=VERTEX_POINT('',#125018);
#23442=VERTEX_POINT('',#125020);
#23443=VERTEX_POINT('',#125024);
#23444=VERTEX_POINT('',#125026);
#23445=VERTEX_POINT('',#125030);
#23446=VERTEX_POINT('',#125032);
#23447=VERTEX_POINT('',#125036);
#23448=VERTEX_POINT('',#125038);
#23449=VERTEX_POINT('',#125042);
#23450=VERTEX_POINT('',#125044);
#23451=VERTEX_POINT('',#125048);
#23452=VERTEX_POINT('',#125050);
#23453=VERTEX_POINT('',#125054);
#23454=VERTEX_POINT('',#125056);
#23455=VERTEX_POINT('',#125060);
#23456=VERTEX_POINT('',#125062);
#23457=VERTEX_POINT('',#125066);
#23458=VERTEX_POINT('',#125068);
#23459=VERTEX_POINT('',#125072);
#23460=VERTEX_POINT('',#125074);
#23461=VERTEX_POINT('',#125078);
#23462=VERTEX_POINT('',#125080);
#23463=VERTEX_POINT('',#125084);
#23464=VERTEX_POINT('',#125086);
#23465=VERTEX_POINT('',#125090);
#23466=VERTEX_POINT('',#125092);
#23467=VERTEX_POINT('',#125096);
#23468=VERTEX_POINT('',#125098);
#23469=VERTEX_POINT('',#125102);
#23470=VERTEX_POINT('',#125104);
#23471=VERTEX_POINT('',#125108);
#23472=VERTEX_POINT('',#125110);
#23473=VERTEX_POINT('',#125114);
#23474=VERTEX_POINT('',#125116);
#23475=VERTEX_POINT('',#125120);
#23476=VERTEX_POINT('',#125122);
#23477=VERTEX_POINT('',#125126);
#23478=VERTEX_POINT('',#125128);
#23479=VERTEX_POINT('',#125132);
#23480=VERTEX_POINT('',#125134);
#23481=VERTEX_POINT('',#125138);
#23482=VERTEX_POINT('',#125140);
#23483=VERTEX_POINT('',#125144);
#23484=VERTEX_POINT('',#125146);
#23485=VERTEX_POINT('',#125150);
#23486=VERTEX_POINT('',#125152);
#23487=VERTEX_POINT('',#125156);
#23488=VERTEX_POINT('',#125158);
#23489=VERTEX_POINT('',#125162);
#23490=VERTEX_POINT('',#125164);
#23491=VERTEX_POINT('',#125168);
#23492=VERTEX_POINT('',#125170);
#23493=VERTEX_POINT('',#125174);
#23494=VERTEX_POINT('',#125176);
#23495=VERTEX_POINT('',#125180);
#23496=VERTEX_POINT('',#125182);
#23497=VERTEX_POINT('',#125186);
#23498=VERTEX_POINT('',#125188);
#23499=VERTEX_POINT('',#125192);
#23500=VERTEX_POINT('',#125194);
#23501=VERTEX_POINT('',#125198);
#23502=VERTEX_POINT('',#125200);
#23503=VERTEX_POINT('',#125204);
#23504=VERTEX_POINT('',#125206);
#23505=VERTEX_POINT('',#125210);
#23506=VERTEX_POINT('',#125212);
#23507=VERTEX_POINT('',#125216);
#23508=VERTEX_POINT('',#125218);
#23509=VERTEX_POINT('',#125222);
#23510=VERTEX_POINT('',#125224);
#23511=VERTEX_POINT('',#125228);
#23512=VERTEX_POINT('',#125230);
#23513=VERTEX_POINT('',#125234);
#23514=VERTEX_POINT('',#125236);
#23515=VERTEX_POINT('',#125240);
#23516=VERTEX_POINT('',#125242);
#23517=VERTEX_POINT('',#125246);
#23518=VERTEX_POINT('',#125248);
#23519=VERTEX_POINT('',#125252);
#23520=VERTEX_POINT('',#125254);
#23521=VERTEX_POINT('',#125258);
#23522=VERTEX_POINT('',#125260);
#23523=VERTEX_POINT('',#125264);
#23524=VERTEX_POINT('',#125266);
#23525=VERTEX_POINT('',#125270);
#23526=VERTEX_POINT('',#125272);
#23527=VERTEX_POINT('',#125276);
#23528=VERTEX_POINT('',#125278);
#23529=VERTEX_POINT('',#125282);
#23530=VERTEX_POINT('',#125284);
#23531=VERTEX_POINT('',#125288);
#23532=VERTEX_POINT('',#125290);
#23533=VERTEX_POINT('',#125294);
#23534=VERTEX_POINT('',#125296);
#23535=VERTEX_POINT('',#125300);
#23536=VERTEX_POINT('',#125302);
#23537=VERTEX_POINT('',#125306);
#23538=VERTEX_POINT('',#125308);
#23539=VERTEX_POINT('',#125312);
#23540=VERTEX_POINT('',#125314);
#23541=VERTEX_POINT('',#125318);
#23542=VERTEX_POINT('',#125320);
#23543=VERTEX_POINT('',#125324);
#23544=VERTEX_POINT('',#125326);
#23545=VERTEX_POINT('',#125330);
#23546=VERTEX_POINT('',#125332);
#23547=VERTEX_POINT('',#125336);
#23548=VERTEX_POINT('',#125338);
#23549=VERTEX_POINT('',#125342);
#23550=VERTEX_POINT('',#125344);
#23551=VERTEX_POINT('',#125348);
#23552=VERTEX_POINT('',#125350);
#23553=VERTEX_POINT('',#125354);
#23554=VERTEX_POINT('',#125356);
#23555=VERTEX_POINT('',#125360);
#23556=VERTEX_POINT('',#125362);
#23557=VERTEX_POINT('',#125366);
#23558=VERTEX_POINT('',#125368);
#23559=VERTEX_POINT('',#125372);
#23560=VERTEX_POINT('',#125374);
#23561=VERTEX_POINT('',#125378);
#23562=VERTEX_POINT('',#125380);
#23563=VERTEX_POINT('',#125384);
#23564=VERTEX_POINT('',#125386);
#23565=VERTEX_POINT('',#125390);
#23566=VERTEX_POINT('',#125392);
#23567=VERTEX_POINT('',#125396);
#23568=VERTEX_POINT('',#125398);
#23569=VERTEX_POINT('',#125402);
#23570=VERTEX_POINT('',#125404);
#23571=VERTEX_POINT('',#125408);
#23572=VERTEX_POINT('',#125410);
#23573=VERTEX_POINT('',#125414);
#23574=VERTEX_POINT('',#125416);
#23575=VERTEX_POINT('',#125420);
#23576=VERTEX_POINT('',#125422);
#23577=VERTEX_POINT('',#125426);
#23578=VERTEX_POINT('',#125428);
#23579=VERTEX_POINT('',#125432);
#23580=VERTEX_POINT('',#125434);
#23581=VERTEX_POINT('',#125438);
#23582=VERTEX_POINT('',#125440);
#23583=VERTEX_POINT('',#125444);
#23584=VERTEX_POINT('',#125446);
#23585=VERTEX_POINT('',#125450);
#23586=VERTEX_POINT('',#125452);
#23587=VERTEX_POINT('',#125456);
#23588=VERTEX_POINT('',#125458);
#23589=VERTEX_POINT('',#125462);
#23590=VERTEX_POINT('',#125464);
#23591=VERTEX_POINT('',#125468);
#23592=VERTEX_POINT('',#125470);
#23593=VERTEX_POINT('',#125474);
#23594=VERTEX_POINT('',#125476);
#23595=VERTEX_POINT('',#125480);
#23596=VERTEX_POINT('',#125482);
#23597=VERTEX_POINT('',#125486);
#23598=VERTEX_POINT('',#125488);
#23599=VERTEX_POINT('',#125492);
#23600=VERTEX_POINT('',#125494);
#23601=VERTEX_POINT('',#125498);
#23602=VERTEX_POINT('',#125500);
#23603=VERTEX_POINT('',#125504);
#23604=VERTEX_POINT('',#125506);
#23605=VERTEX_POINT('',#125510);
#23606=VERTEX_POINT('',#125512);
#23607=VERTEX_POINT('',#125516);
#23608=VERTEX_POINT('',#125518);
#23609=VERTEX_POINT('',#125522);
#23610=VERTEX_POINT('',#125524);
#23611=VERTEX_POINT('',#125528);
#23612=VERTEX_POINT('',#125530);
#23613=VERTEX_POINT('',#125534);
#23614=VERTEX_POINT('',#125536);
#23615=VERTEX_POINT('',#125540);
#23616=VERTEX_POINT('',#125542);
#23617=VERTEX_POINT('',#125546);
#23618=VERTEX_POINT('',#125548);
#23619=VERTEX_POINT('',#125552);
#23620=VERTEX_POINT('',#125554);
#23621=VERTEX_POINT('',#125558);
#23622=VERTEX_POINT('',#125560);
#23623=VERTEX_POINT('',#125564);
#23624=VERTEX_POINT('',#125566);
#23625=VERTEX_POINT('',#125570);
#23626=VERTEX_POINT('',#125572);
#23627=VERTEX_POINT('',#125576);
#23628=VERTEX_POINT('',#125578);
#23629=VERTEX_POINT('',#125582);
#23630=VERTEX_POINT('',#125584);
#23631=VERTEX_POINT('',#125588);
#23632=VERTEX_POINT('',#125590);
#23633=VERTEX_POINT('',#125594);
#23634=VERTEX_POINT('',#125596);
#23635=VERTEX_POINT('',#125600);
#23636=VERTEX_POINT('',#125602);
#23637=VERTEX_POINT('',#125606);
#23638=VERTEX_POINT('',#125608);
#23639=VERTEX_POINT('',#125612);
#23640=VERTEX_POINT('',#125614);
#23641=VERTEX_POINT('',#125618);
#23642=VERTEX_POINT('',#125620);
#23643=VERTEX_POINT('',#125624);
#23644=VERTEX_POINT('',#125626);
#23645=VERTEX_POINT('',#125630);
#23646=VERTEX_POINT('',#125632);
#23647=VERTEX_POINT('',#125636);
#23648=VERTEX_POINT('',#125638);
#23649=VERTEX_POINT('',#125642);
#23650=VERTEX_POINT('',#125644);
#23651=VERTEX_POINT('',#125648);
#23652=VERTEX_POINT('',#125650);
#23653=VERTEX_POINT('',#125654);
#23654=VERTEX_POINT('',#125656);
#23655=VERTEX_POINT('',#125660);
#23656=VERTEX_POINT('',#125662);
#23657=VERTEX_POINT('',#125666);
#23658=VERTEX_POINT('',#125668);
#23659=VERTEX_POINT('',#125672);
#23660=VERTEX_POINT('',#125674);
#23661=VERTEX_POINT('',#125678);
#23662=VERTEX_POINT('',#125680);
#23663=VERTEX_POINT('',#125684);
#23664=VERTEX_POINT('',#125686);
#23665=VERTEX_POINT('',#125690);
#23666=VERTEX_POINT('',#125692);
#23667=VERTEX_POINT('',#125696);
#23668=VERTEX_POINT('',#125698);
#23669=VERTEX_POINT('',#125702);
#23670=VERTEX_POINT('',#125704);
#23671=VERTEX_POINT('',#125708);
#23672=VERTEX_POINT('',#125710);
#23673=VERTEX_POINT('',#125714);
#23674=VERTEX_POINT('',#125716);
#23675=VERTEX_POINT('',#125720);
#23676=VERTEX_POINT('',#125722);
#23677=VERTEX_POINT('',#125726);
#23678=VERTEX_POINT('',#125728);
#23679=VERTEX_POINT('',#125732);
#23680=VERTEX_POINT('',#125734);
#23681=VERTEX_POINT('',#125738);
#23682=VERTEX_POINT('',#125740);
#23683=VERTEX_POINT('',#125744);
#23684=VERTEX_POINT('',#125746);
#23685=VERTEX_POINT('',#125750);
#23686=VERTEX_POINT('',#125752);
#23687=VERTEX_POINT('',#125756);
#23688=VERTEX_POINT('',#125758);
#23689=VERTEX_POINT('',#125762);
#23690=VERTEX_POINT('',#125764);
#23691=VERTEX_POINT('',#125768);
#23692=VERTEX_POINT('',#125770);
#23693=VERTEX_POINT('',#125774);
#23694=VERTEX_POINT('',#125776);
#23695=VERTEX_POINT('',#125780);
#23696=VERTEX_POINT('',#125782);
#23697=VERTEX_POINT('',#125786);
#23698=VERTEX_POINT('',#125788);
#23699=VERTEX_POINT('',#125792);
#23700=VERTEX_POINT('',#125794);
#23701=VERTEX_POINT('',#125798);
#23702=VERTEX_POINT('',#125800);
#23703=VERTEX_POINT('',#125804);
#23704=VERTEX_POINT('',#125806);
#23705=VERTEX_POINT('',#125810);
#23706=VERTEX_POINT('',#125812);
#23707=VERTEX_POINT('',#125816);
#23708=VERTEX_POINT('',#125818);
#23709=VERTEX_POINT('',#125822);
#23710=VERTEX_POINT('',#125824);
#23711=VERTEX_POINT('',#125828);
#23712=VERTEX_POINT('',#125830);
#23713=VERTEX_POINT('',#125834);
#23714=VERTEX_POINT('',#125836);
#23715=VERTEX_POINT('',#125840);
#23716=VERTEX_POINT('',#125842);
#23717=VERTEX_POINT('',#125846);
#23718=VERTEX_POINT('',#125848);
#23719=VERTEX_POINT('',#125852);
#23720=VERTEX_POINT('',#125854);
#23721=VERTEX_POINT('',#125858);
#23722=VERTEX_POINT('',#125860);
#23723=VERTEX_POINT('',#125864);
#23724=VERTEX_POINT('',#125866);
#23725=VERTEX_POINT('',#125870);
#23726=VERTEX_POINT('',#125872);
#23727=VERTEX_POINT('',#125876);
#23728=VERTEX_POINT('',#125878);
#23729=VERTEX_POINT('',#125882);
#23730=VERTEX_POINT('',#125884);
#23731=VERTEX_POINT('',#125888);
#23732=VERTEX_POINT('',#125890);
#23733=VERTEX_POINT('',#125894);
#23734=VERTEX_POINT('',#125896);
#23735=VERTEX_POINT('',#125900);
#23736=VERTEX_POINT('',#125902);
#23737=VERTEX_POINT('',#125906);
#23738=VERTEX_POINT('',#125908);
#23739=VERTEX_POINT('',#125912);
#23740=VERTEX_POINT('',#125914);
#23741=VERTEX_POINT('',#125918);
#23742=VERTEX_POINT('',#125920);
#23743=VERTEX_POINT('',#125924);
#23744=VERTEX_POINT('',#125926);
#23745=VERTEX_POINT('',#125930);
#23746=VERTEX_POINT('',#125932);
#23747=VERTEX_POINT('',#125936);
#23748=VERTEX_POINT('',#125938);
#23749=VERTEX_POINT('',#125942);
#23750=VERTEX_POINT('',#125944);
#23751=VERTEX_POINT('',#125948);
#23752=VERTEX_POINT('',#125950);
#23753=VERTEX_POINT('',#125954);
#23754=VERTEX_POINT('',#125956);
#23755=VERTEX_POINT('',#125960);
#23756=VERTEX_POINT('',#125962);
#23757=VERTEX_POINT('',#125966);
#23758=VERTEX_POINT('',#125968);
#23759=VERTEX_POINT('',#125972);
#23760=VERTEX_POINT('',#125974);
#23761=VERTEX_POINT('',#125978);
#23762=VERTEX_POINT('',#125980);
#23763=VERTEX_POINT('',#125984);
#23764=VERTEX_POINT('',#125986);
#23765=VERTEX_POINT('',#125990);
#23766=VERTEX_POINT('',#125992);
#23767=VERTEX_POINT('',#125996);
#23768=VERTEX_POINT('',#125998);
#23769=VERTEX_POINT('',#126002);
#23770=VERTEX_POINT('',#126004);
#23771=VERTEX_POINT('',#126008);
#23772=VERTEX_POINT('',#126010);
#23773=VERTEX_POINT('',#126014);
#23774=VERTEX_POINT('',#126016);
#23775=VERTEX_POINT('',#126020);
#23776=VERTEX_POINT('',#126022);
#23777=VERTEX_POINT('',#126026);
#23778=VERTEX_POINT('',#126028);
#23779=VERTEX_POINT('',#126032);
#23780=VERTEX_POINT('',#126034);
#23781=VERTEX_POINT('',#126038);
#23782=VERTEX_POINT('',#126040);
#23783=VERTEX_POINT('',#126044);
#23784=VERTEX_POINT('',#126046);
#23785=VERTEX_POINT('',#126050);
#23786=VERTEX_POINT('',#126052);
#23787=VERTEX_POINT('',#126056);
#23788=VERTEX_POINT('',#126058);
#23789=VERTEX_POINT('',#126062);
#23790=VERTEX_POINT('',#126064);
#23791=VERTEX_POINT('',#126068);
#23792=VERTEX_POINT('',#126070);
#23793=VERTEX_POINT('',#126074);
#23794=VERTEX_POINT('',#126076);
#23795=VERTEX_POINT('',#126080);
#23796=VERTEX_POINT('',#126082);
#23797=VERTEX_POINT('',#126086);
#23798=VERTEX_POINT('',#126088);
#23799=VERTEX_POINT('',#126092);
#23800=VERTEX_POINT('',#126094);
#23801=VERTEX_POINT('',#126098);
#23802=VERTEX_POINT('',#126100);
#23803=VERTEX_POINT('',#126104);
#23804=VERTEX_POINT('',#126106);
#23805=VERTEX_POINT('',#126110);
#23806=VERTEX_POINT('',#126112);
#23807=VERTEX_POINT('',#126116);
#23808=VERTEX_POINT('',#126118);
#23809=VERTEX_POINT('',#126122);
#23810=VERTEX_POINT('',#126124);
#23811=VERTEX_POINT('',#126128);
#23812=VERTEX_POINT('',#126130);
#23813=VERTEX_POINT('',#126134);
#23814=VERTEX_POINT('',#126136);
#23815=VERTEX_POINT('',#126140);
#23816=VERTEX_POINT('',#126142);
#23817=VERTEX_POINT('',#126146);
#23818=VERTEX_POINT('',#126148);
#23819=VERTEX_POINT('',#126152);
#23820=VERTEX_POINT('',#126154);
#23821=VERTEX_POINT('',#126158);
#23822=VERTEX_POINT('',#126160);
#23823=VERTEX_POINT('',#126164);
#23824=VERTEX_POINT('',#126166);
#23825=VERTEX_POINT('',#126170);
#23826=VERTEX_POINT('',#126172);
#23827=VERTEX_POINT('',#126176);
#23828=VERTEX_POINT('',#126178);
#23829=VERTEX_POINT('',#126182);
#23830=VERTEX_POINT('',#126184);
#23831=VERTEX_POINT('',#126188);
#23832=VERTEX_POINT('',#126190);
#23833=VERTEX_POINT('',#126194);
#23834=VERTEX_POINT('',#126196);
#23835=VERTEX_POINT('',#126200);
#23836=VERTEX_POINT('',#126202);
#23837=VERTEX_POINT('',#126206);
#23838=VERTEX_POINT('',#126208);
#23839=VERTEX_POINT('',#126212);
#23840=VERTEX_POINT('',#126214);
#23841=VERTEX_POINT('',#126218);
#23842=VERTEX_POINT('',#126220);
#23843=VERTEX_POINT('',#126224);
#23844=VERTEX_POINT('',#126226);
#23845=VERTEX_POINT('',#126230);
#23846=VERTEX_POINT('',#126232);
#23847=VERTEX_POINT('',#126236);
#23848=VERTEX_POINT('',#126238);
#23849=VERTEX_POINT('',#126242);
#23850=VERTEX_POINT('',#126244);
#23851=VERTEX_POINT('',#126248);
#23852=VERTEX_POINT('',#126250);
#23853=VERTEX_POINT('',#126254);
#23854=VERTEX_POINT('',#126256);
#23855=VERTEX_POINT('',#126260);
#23856=VERTEX_POINT('',#126262);
#23857=VERTEX_POINT('',#126266);
#23858=VERTEX_POINT('',#126268);
#23859=VERTEX_POINT('',#126272);
#23860=VERTEX_POINT('',#126274);
#23861=VERTEX_POINT('',#126278);
#23862=VERTEX_POINT('',#126280);
#23863=VERTEX_POINT('',#126284);
#23864=VERTEX_POINT('',#126286);
#23865=VERTEX_POINT('',#126290);
#23866=VERTEX_POINT('',#126292);
#23867=VERTEX_POINT('',#126296);
#23868=VERTEX_POINT('',#126298);
#23869=VERTEX_POINT('',#126302);
#23870=VERTEX_POINT('',#126304);
#23871=VERTEX_POINT('',#126308);
#23872=VERTEX_POINT('',#126310);
#23873=VERTEX_POINT('',#126314);
#23874=VERTEX_POINT('',#126316);
#23875=VERTEX_POINT('',#126320);
#23876=VERTEX_POINT('',#126322);
#23877=VERTEX_POINT('',#126326);
#23878=VERTEX_POINT('',#126328);
#23879=VERTEX_POINT('',#126332);
#23880=VERTEX_POINT('',#126334);
#23881=VERTEX_POINT('',#126338);
#23882=VERTEX_POINT('',#126340);
#23883=VERTEX_POINT('',#126344);
#23884=VERTEX_POINT('',#126346);
#23885=VERTEX_POINT('',#126350);
#23886=VERTEX_POINT('',#126352);
#23887=VERTEX_POINT('',#126356);
#23888=VERTEX_POINT('',#126358);
#23889=VERTEX_POINT('',#126362);
#23890=VERTEX_POINT('',#126364);
#23891=VERTEX_POINT('',#126368);
#23892=VERTEX_POINT('',#126370);
#23893=VERTEX_POINT('',#126374);
#23894=VERTEX_POINT('',#126376);
#23895=VERTEX_POINT('',#126380);
#23896=VERTEX_POINT('',#126382);
#23897=VERTEX_POINT('',#126386);
#23898=VERTEX_POINT('',#126388);
#23899=VERTEX_POINT('',#126392);
#23900=VERTEX_POINT('',#126394);
#23901=VERTEX_POINT('',#126398);
#23902=VERTEX_POINT('',#126400);
#23903=VERTEX_POINT('',#126404);
#23904=VERTEX_POINT('',#126406);
#23905=VERTEX_POINT('',#126410);
#23906=VERTEX_POINT('',#126412);
#23907=VERTEX_POINT('',#126416);
#23908=VERTEX_POINT('',#126418);
#23909=VERTEX_POINT('',#126422);
#23910=VERTEX_POINT('',#126424);
#23911=VERTEX_POINT('',#126428);
#23912=VERTEX_POINT('',#126430);
#23913=VERTEX_POINT('',#126434);
#23914=VERTEX_POINT('',#126436);
#23915=VERTEX_POINT('',#126440);
#23916=VERTEX_POINT('',#126442);
#23917=VERTEX_POINT('',#126446);
#23918=VERTEX_POINT('',#126448);
#23919=VERTEX_POINT('',#126452);
#23920=VERTEX_POINT('',#126454);
#23921=VERTEX_POINT('',#126458);
#23922=VERTEX_POINT('',#126460);
#23923=VERTEX_POINT('',#126464);
#23924=VERTEX_POINT('',#126466);
#23925=VERTEX_POINT('',#126470);
#23926=VERTEX_POINT('',#126472);
#23927=VERTEX_POINT('',#126476);
#23928=VERTEX_POINT('',#126478);
#23929=VERTEX_POINT('',#126482);
#23930=VERTEX_POINT('',#126484);
#23931=VERTEX_POINT('',#126488);
#23932=VERTEX_POINT('',#126490);
#23933=VERTEX_POINT('',#126494);
#23934=VERTEX_POINT('',#126496);
#23935=VERTEX_POINT('',#126500);
#23936=VERTEX_POINT('',#126502);
#23937=VERTEX_POINT('',#126506);
#23938=VERTEX_POINT('',#126508);
#23939=VERTEX_POINT('',#126512);
#23940=VERTEX_POINT('',#126514);
#23941=VERTEX_POINT('',#126518);
#23942=VERTEX_POINT('',#126520);
#23943=VERTEX_POINT('',#126524);
#23944=VERTEX_POINT('',#126526);
#23945=VERTEX_POINT('',#126530);
#23946=VERTEX_POINT('',#126532);
#23947=VERTEX_POINT('',#126536);
#23948=VERTEX_POINT('',#126538);
#23949=VERTEX_POINT('',#126542);
#23950=VERTEX_POINT('',#126544);
#23951=VERTEX_POINT('',#126548);
#23952=VERTEX_POINT('',#126550);
#23953=VERTEX_POINT('',#126554);
#23954=VERTEX_POINT('',#126556);
#23955=VERTEX_POINT('',#126560);
#23956=VERTEX_POINT('',#126562);
#23957=VERTEX_POINT('',#126566);
#23958=VERTEX_POINT('',#126568);
#23959=VERTEX_POINT('',#126572);
#23960=VERTEX_POINT('',#126574);
#23961=VERTEX_POINT('',#126578);
#23962=VERTEX_POINT('',#126580);
#23963=VERTEX_POINT('',#126584);
#23964=VERTEX_POINT('',#126586);
#23965=VERTEX_POINT('',#126590);
#23966=VERTEX_POINT('',#126592);
#23967=VERTEX_POINT('',#126596);
#23968=VERTEX_POINT('',#126598);
#23969=VERTEX_POINT('',#126602);
#23970=VERTEX_POINT('',#126604);
#23971=VERTEX_POINT('',#126608);
#23972=VERTEX_POINT('',#126610);
#23973=VERTEX_POINT('',#126614);
#23974=VERTEX_POINT('',#126616);
#23975=VERTEX_POINT('',#126620);
#23976=VERTEX_POINT('',#126622);
#23977=VERTEX_POINT('',#126626);
#23978=VERTEX_POINT('',#126628);
#23979=VERTEX_POINT('',#126632);
#23980=VERTEX_POINT('',#126634);
#23981=VERTEX_POINT('',#126638);
#23982=VERTEX_POINT('',#126640);
#23983=VERTEX_POINT('',#126644);
#23984=VERTEX_POINT('',#126646);
#23985=VERTEX_POINT('',#126650);
#23986=VERTEX_POINT('',#126652);
#23987=VERTEX_POINT('',#126656);
#23988=VERTEX_POINT('',#126658);
#23989=VERTEX_POINT('',#126662);
#23990=VERTEX_POINT('',#126664);
#23991=VERTEX_POINT('',#126668);
#23992=VERTEX_POINT('',#126670);
#23993=VERTEX_POINT('',#126674);
#23994=VERTEX_POINT('',#126676);
#23995=VERTEX_POINT('',#126680);
#23996=VERTEX_POINT('',#126682);
#23997=VERTEX_POINT('',#126686);
#23998=VERTEX_POINT('',#126688);
#23999=VERTEX_POINT('',#126692);
#24000=VERTEX_POINT('',#126694);
#24001=VERTEX_POINT('',#126698);
#24002=VERTEX_POINT('',#126700);
#24003=VERTEX_POINT('',#126704);
#24004=VERTEX_POINT('',#126706);
#24005=VERTEX_POINT('',#126710);
#24006=VERTEX_POINT('',#126712);
#24007=VERTEX_POINT('',#126716);
#24008=VERTEX_POINT('',#126718);
#24009=VERTEX_POINT('',#126722);
#24010=VERTEX_POINT('',#126724);
#24011=VERTEX_POINT('',#126728);
#24012=VERTEX_POINT('',#126730);
#24013=VERTEX_POINT('',#126734);
#24014=VERTEX_POINT('',#126736);
#24015=VERTEX_POINT('',#126740);
#24016=VERTEX_POINT('',#126742);
#24017=VERTEX_POINT('',#126746);
#24018=VERTEX_POINT('',#126748);
#24019=VERTEX_POINT('',#126752);
#24020=VERTEX_POINT('',#126754);
#24021=VERTEX_POINT('',#126758);
#24022=VERTEX_POINT('',#126760);
#24023=VERTEX_POINT('',#126764);
#24024=VERTEX_POINT('',#126766);
#24025=VERTEX_POINT('',#126770);
#24026=VERTEX_POINT('',#126772);
#24027=VERTEX_POINT('',#126776);
#24028=VERTEX_POINT('',#126778);
#24029=VERTEX_POINT('',#126782);
#24030=VERTEX_POINT('',#126784);
#24031=VERTEX_POINT('',#126788);
#24032=VERTEX_POINT('',#126790);
#24033=VERTEX_POINT('',#126794);
#24034=VERTEX_POINT('',#126796);
#24035=VERTEX_POINT('',#126800);
#24036=VERTEX_POINT('',#126802);
#24037=VERTEX_POINT('',#126806);
#24038=VERTEX_POINT('',#126808);
#24039=VERTEX_POINT('',#126812);
#24040=VERTEX_POINT('',#126814);
#24041=VERTEX_POINT('',#126818);
#24042=VERTEX_POINT('',#126820);
#24043=VERTEX_POINT('',#126824);
#24044=VERTEX_POINT('',#126826);
#24045=VERTEX_POINT('',#126830);
#24046=VERTEX_POINT('',#126832);
#24047=VERTEX_POINT('',#126836);
#24048=VERTEX_POINT('',#126838);
#24049=VERTEX_POINT('',#126842);
#24050=VERTEX_POINT('',#126844);
#24051=VERTEX_POINT('',#126848);
#24052=VERTEX_POINT('',#126850);
#24053=VERTEX_POINT('',#126854);
#24054=VERTEX_POINT('',#126856);
#24055=VERTEX_POINT('',#126860);
#24056=VERTEX_POINT('',#126862);
#24057=VERTEX_POINT('',#126866);
#24058=VERTEX_POINT('',#126868);
#24059=VERTEX_POINT('',#126872);
#24060=VERTEX_POINT('',#126874);
#24061=VERTEX_POINT('',#126878);
#24062=VERTEX_POINT('',#126880);
#24063=VERTEX_POINT('',#126884);
#24064=VERTEX_POINT('',#126886);
#24065=VERTEX_POINT('',#126890);
#24066=VERTEX_POINT('',#126892);
#24067=VERTEX_POINT('',#126896);
#24068=VERTEX_POINT('',#126898);
#24069=VERTEX_POINT('',#126902);
#24070=VERTEX_POINT('',#126904);
#24071=VERTEX_POINT('',#126908);
#24072=VERTEX_POINT('',#126910);
#24073=VERTEX_POINT('',#126914);
#24074=VERTEX_POINT('',#126916);
#24075=VERTEX_POINT('',#126920);
#24076=VERTEX_POINT('',#126922);
#24077=VERTEX_POINT('',#126926);
#24078=VERTEX_POINT('',#126928);
#24079=VERTEX_POINT('',#126932);
#24080=VERTEX_POINT('',#126934);
#24081=VERTEX_POINT('',#126938);
#24082=VERTEX_POINT('',#126940);
#24083=VERTEX_POINT('',#126944);
#24084=VERTEX_POINT('',#126946);
#24085=VERTEX_POINT('',#126950);
#24086=VERTEX_POINT('',#126952);
#24087=VERTEX_POINT('',#126956);
#24088=VERTEX_POINT('',#126958);
#24089=VERTEX_POINT('',#126962);
#24090=VERTEX_POINT('',#126964);
#24091=VERTEX_POINT('',#126968);
#24092=VERTEX_POINT('',#126970);
#24093=VERTEX_POINT('',#126974);
#24094=VERTEX_POINT('',#126976);
#24095=VERTEX_POINT('',#126980);
#24096=VERTEX_POINT('',#126982);
#24097=VERTEX_POINT('',#126986);
#24098=VERTEX_POINT('',#126988);
#24099=VERTEX_POINT('',#126992);
#24100=VERTEX_POINT('',#126994);
#24101=VERTEX_POINT('',#126998);
#24102=VERTEX_POINT('',#127000);
#24103=VERTEX_POINT('',#127004);
#24104=VERTEX_POINT('',#127006);
#24105=VERTEX_POINT('',#127010);
#24106=VERTEX_POINT('',#127012);
#24107=VERTEX_POINT('',#127016);
#24108=VERTEX_POINT('',#127018);
#24109=VERTEX_POINT('',#127022);
#24110=VERTEX_POINT('',#127024);
#24111=VERTEX_POINT('',#127028);
#24112=VERTEX_POINT('',#127030);
#24113=VERTEX_POINT('',#127034);
#24114=VERTEX_POINT('',#127036);
#24115=VERTEX_POINT('',#127040);
#24116=VERTEX_POINT('',#127042);
#24117=VERTEX_POINT('',#127046);
#24118=VERTEX_POINT('',#127048);
#24119=VERTEX_POINT('',#127052);
#24120=VERTEX_POINT('',#127054);
#24121=VERTEX_POINT('',#127058);
#24122=VERTEX_POINT('',#127060);
#24123=VERTEX_POINT('',#127064);
#24124=VERTEX_POINT('',#127066);
#24125=VERTEX_POINT('',#127070);
#24126=VERTEX_POINT('',#127072);
#24127=VERTEX_POINT('',#127076);
#24128=VERTEX_POINT('',#127078);
#24129=VERTEX_POINT('',#127082);
#24130=VERTEX_POINT('',#127084);
#24131=VERTEX_POINT('',#127088);
#24132=VERTEX_POINT('',#127090);
#24133=VERTEX_POINT('',#127094);
#24134=VERTEX_POINT('',#127096);
#24135=VERTEX_POINT('',#127100);
#24136=VERTEX_POINT('',#127102);
#24137=VERTEX_POINT('',#127106);
#24138=VERTEX_POINT('',#127108);
#24139=VERTEX_POINT('',#127112);
#24140=VERTEX_POINT('',#127114);
#24141=VERTEX_POINT('',#127118);
#24142=VERTEX_POINT('',#127120);
#24143=VERTEX_POINT('',#127124);
#24144=VERTEX_POINT('',#127126);
#24145=VERTEX_POINT('',#127130);
#24146=VERTEX_POINT('',#127132);
#24147=VERTEX_POINT('',#127136);
#24148=VERTEX_POINT('',#127138);
#24149=VERTEX_POINT('',#127142);
#24150=VERTEX_POINT('',#127144);
#24151=VERTEX_POINT('',#127148);
#24152=VERTEX_POINT('',#127150);
#24153=VERTEX_POINT('',#127154);
#24154=VERTEX_POINT('',#127156);
#24155=VERTEX_POINT('',#127160);
#24156=VERTEX_POINT('',#127162);
#24157=VERTEX_POINT('',#127166);
#24158=VERTEX_POINT('',#127168);
#24159=VERTEX_POINT('',#127172);
#24160=VERTEX_POINT('',#127174);
#24161=VERTEX_POINT('',#127178);
#24162=VERTEX_POINT('',#127180);
#24163=VERTEX_POINT('',#127184);
#24164=VERTEX_POINT('',#127186);
#24165=VERTEX_POINT('',#127190);
#24166=VERTEX_POINT('',#127192);
#24167=VERTEX_POINT('',#127196);
#24168=VERTEX_POINT('',#127198);
#24169=VERTEX_POINT('',#127202);
#24170=VERTEX_POINT('',#127204);
#24171=VERTEX_POINT('',#127208);
#24172=VERTEX_POINT('',#127210);
#24173=VERTEX_POINT('',#127214);
#24174=VERTEX_POINT('',#127216);
#24175=VERTEX_POINT('',#127220);
#24176=VERTEX_POINT('',#127222);
#24177=VERTEX_POINT('',#127226);
#24178=VERTEX_POINT('',#127228);
#24179=VERTEX_POINT('',#127232);
#24180=VERTEX_POINT('',#127234);
#24181=VERTEX_POINT('',#127238);
#24182=VERTEX_POINT('',#127240);
#24183=VERTEX_POINT('',#127244);
#24184=VERTEX_POINT('',#127246);
#24185=VERTEX_POINT('',#127250);
#24186=VERTEX_POINT('',#127252);
#24187=VERTEX_POINT('',#127256);
#24188=VERTEX_POINT('',#127258);
#24189=VERTEX_POINT('',#127262);
#24190=VERTEX_POINT('',#127264);
#24191=VERTEX_POINT('',#127268);
#24192=VERTEX_POINT('',#127270);
#24193=VERTEX_POINT('',#127274);
#24194=VERTEX_POINT('',#127276);
#24195=VERTEX_POINT('',#127280);
#24196=VERTEX_POINT('',#127282);
#24197=VERTEX_POINT('',#127286);
#24198=VERTEX_POINT('',#127288);
#24199=VERTEX_POINT('',#127292);
#24200=VERTEX_POINT('',#127294);
#24201=VERTEX_POINT('',#127298);
#24202=VERTEX_POINT('',#127300);
#24203=VERTEX_POINT('',#127304);
#24204=VERTEX_POINT('',#127306);
#24205=VERTEX_POINT('',#127310);
#24206=VERTEX_POINT('',#127312);
#24207=VERTEX_POINT('',#127316);
#24208=VERTEX_POINT('',#127318);
#24209=VERTEX_POINT('',#127322);
#24210=VERTEX_POINT('',#127324);
#24211=VERTEX_POINT('',#127328);
#24212=VERTEX_POINT('',#127330);
#24213=VERTEX_POINT('',#127334);
#24214=VERTEX_POINT('',#127336);
#24215=VERTEX_POINT('',#127340);
#24216=VERTEX_POINT('',#127342);
#24217=VERTEX_POINT('',#127346);
#24218=VERTEX_POINT('',#127348);
#24219=VERTEX_POINT('',#127352);
#24220=VERTEX_POINT('',#127354);
#24221=VERTEX_POINT('',#127358);
#24222=VERTEX_POINT('',#127360);
#24223=VERTEX_POINT('',#127364);
#24224=VERTEX_POINT('',#127366);
#24225=VERTEX_POINT('',#127370);
#24226=VERTEX_POINT('',#127372);
#24227=VERTEX_POINT('',#127376);
#24228=VERTEX_POINT('',#127378);
#24229=VERTEX_POINT('',#127382);
#24230=VERTEX_POINT('',#127384);
#24231=VERTEX_POINT('',#127388);
#24232=VERTEX_POINT('',#127390);
#24233=VERTEX_POINT('',#127394);
#24234=VERTEX_POINT('',#127396);
#24235=VERTEX_POINT('',#127400);
#24236=VERTEX_POINT('',#127402);
#24237=VERTEX_POINT('',#127406);
#24238=VERTEX_POINT('',#127408);
#24239=VERTEX_POINT('',#127412);
#24240=VERTEX_POINT('',#127414);
#24241=VERTEX_POINT('',#127418);
#24242=VERTEX_POINT('',#127420);
#24243=VERTEX_POINT('',#127424);
#24244=VERTEX_POINT('',#127426);
#24245=VERTEX_POINT('',#127430);
#24246=VERTEX_POINT('',#127432);
#24247=VERTEX_POINT('',#127436);
#24248=VERTEX_POINT('',#127438);
#24249=VERTEX_POINT('',#127442);
#24250=VERTEX_POINT('',#127444);
#24251=VERTEX_POINT('',#127448);
#24252=VERTEX_POINT('',#127450);
#24253=VERTEX_POINT('',#127454);
#24254=VERTEX_POINT('',#127456);
#24255=VERTEX_POINT('',#127460);
#24256=VERTEX_POINT('',#127462);
#24257=VERTEX_POINT('',#127466);
#24258=VERTEX_POINT('',#127468);
#24259=VERTEX_POINT('',#127472);
#24260=VERTEX_POINT('',#127474);
#24261=VERTEX_POINT('',#127478);
#24262=VERTEX_POINT('',#127480);
#24263=VERTEX_POINT('',#127484);
#24264=VERTEX_POINT('',#127486);
#24265=VERTEX_POINT('',#127490);
#24266=VERTEX_POINT('',#127492);
#24267=VERTEX_POINT('',#127496);
#24268=VERTEX_POINT('',#127498);
#24269=VERTEX_POINT('',#127502);
#24270=VERTEX_POINT('',#127504);
#24271=VERTEX_POINT('',#127508);
#24272=VERTEX_POINT('',#127510);
#24273=VERTEX_POINT('',#127514);
#24274=VERTEX_POINT('',#127516);
#24275=VERTEX_POINT('',#127520);
#24276=VERTEX_POINT('',#127522);
#24277=VERTEX_POINT('',#127526);
#24278=VERTEX_POINT('',#127528);
#24279=VERTEX_POINT('',#127532);
#24280=VERTEX_POINT('',#127534);
#24281=VERTEX_POINT('',#127538);
#24282=VERTEX_POINT('',#127540);
#24283=VERTEX_POINT('',#127544);
#24284=VERTEX_POINT('',#127546);
#24285=VERTEX_POINT('',#127550);
#24286=VERTEX_POINT('',#127552);
#24287=VERTEX_POINT('',#127556);
#24288=VERTEX_POINT('',#127558);
#24289=VERTEX_POINT('',#127562);
#24290=VERTEX_POINT('',#127564);
#24291=VERTEX_POINT('',#127568);
#24292=VERTEX_POINT('',#127570);
#24293=VERTEX_POINT('',#127574);
#24294=VERTEX_POINT('',#127576);
#24295=VERTEX_POINT('',#127580);
#24296=VERTEX_POINT('',#127582);
#24297=VERTEX_POINT('',#127586);
#24298=VERTEX_POINT('',#127588);
#24299=VERTEX_POINT('',#127592);
#24300=VERTEX_POINT('',#127594);
#24301=VERTEX_POINT('',#127598);
#24302=VERTEX_POINT('',#127600);
#24303=VERTEX_POINT('',#127604);
#24304=VERTEX_POINT('',#127606);
#24305=VERTEX_POINT('',#127610);
#24306=VERTEX_POINT('',#127612);
#24307=VERTEX_POINT('',#127616);
#24308=VERTEX_POINT('',#127618);
#24309=VERTEX_POINT('',#127622);
#24310=VERTEX_POINT('',#127624);
#24311=VERTEX_POINT('',#127628);
#24312=VERTEX_POINT('',#127630);
#24313=VERTEX_POINT('',#127634);
#24314=VERTEX_POINT('',#127636);
#24315=VERTEX_POINT('',#127640);
#24316=VERTEX_POINT('',#127642);
#24317=VERTEX_POINT('',#127646);
#24318=VERTEX_POINT('',#127648);
#24319=VERTEX_POINT('',#127652);
#24320=VERTEX_POINT('',#127654);
#24321=VERTEX_POINT('',#127658);
#24322=VERTEX_POINT('',#127660);
#24323=VERTEX_POINT('',#127664);
#24324=VERTEX_POINT('',#127666);
#24325=VERTEX_POINT('',#127670);
#24326=VERTEX_POINT('',#127672);
#24327=VERTEX_POINT('',#127676);
#24328=VERTEX_POINT('',#127678);
#24329=VERTEX_POINT('',#127682);
#24330=VERTEX_POINT('',#127684);
#24331=VERTEX_POINT('',#127688);
#24332=VERTEX_POINT('',#127690);
#24333=VERTEX_POINT('',#127694);
#24334=VERTEX_POINT('',#127696);
#24335=VERTEX_POINT('',#127700);
#24336=VERTEX_POINT('',#127702);
#24337=VERTEX_POINT('',#127706);
#24338=VERTEX_POINT('',#127708);
#24339=VERTEX_POINT('',#127712);
#24340=VERTEX_POINT('',#127714);
#24341=VERTEX_POINT('',#127718);
#24342=VERTEX_POINT('',#127720);
#24343=VERTEX_POINT('',#127724);
#24344=VERTEX_POINT('',#127726);
#24345=VERTEX_POINT('',#127730);
#24346=VERTEX_POINT('',#127732);
#24347=VERTEX_POINT('',#127736);
#24348=VERTEX_POINT('',#127738);
#24349=VERTEX_POINT('',#127742);
#24350=VERTEX_POINT('',#127744);
#24351=VERTEX_POINT('',#127748);
#24352=VERTEX_POINT('',#127750);
#24353=VERTEX_POINT('',#127754);
#24354=VERTEX_POINT('',#127756);
#24355=VERTEX_POINT('',#127760);
#24356=VERTEX_POINT('',#127762);
#24357=VERTEX_POINT('',#127766);
#24358=VERTEX_POINT('',#127768);
#24359=VERTEX_POINT('',#127772);
#24360=VERTEX_POINT('',#127774);
#24361=VERTEX_POINT('',#127778);
#24362=VERTEX_POINT('',#127780);
#24363=VERTEX_POINT('',#127784);
#24364=VERTEX_POINT('',#127786);
#24365=VERTEX_POINT('',#127790);
#24366=VERTEX_POINT('',#127792);
#24367=VERTEX_POINT('',#127796);
#24368=VERTEX_POINT('',#127798);
#24369=VERTEX_POINT('',#127802);
#24370=VERTEX_POINT('',#127804);
#24371=VERTEX_POINT('',#127808);
#24372=VERTEX_POINT('',#127810);
#24373=VERTEX_POINT('',#127814);
#24374=VERTEX_POINT('',#127816);
#24375=VERTEX_POINT('',#127820);
#24376=VERTEX_POINT('',#127822);
#24377=VERTEX_POINT('',#127826);
#24378=VERTEX_POINT('',#127828);
#24379=VERTEX_POINT('',#127832);
#24380=VERTEX_POINT('',#127834);
#24381=VERTEX_POINT('',#127838);
#24382=VERTEX_POINT('',#127840);
#24383=VERTEX_POINT('',#127844);
#24384=VERTEX_POINT('',#127846);
#24385=VERTEX_POINT('',#127850);
#24386=VERTEX_POINT('',#127852);
#24387=VERTEX_POINT('',#127856);
#24388=VERTEX_POINT('',#127858);
#24389=VERTEX_POINT('',#127862);
#24390=VERTEX_POINT('',#127864);
#24391=VERTEX_POINT('',#127868);
#24392=VERTEX_POINT('',#127870);
#24393=VERTEX_POINT('',#127874);
#24394=VERTEX_POINT('',#127876);
#24395=VERTEX_POINT('',#127880);
#24396=VERTEX_POINT('',#127882);
#24397=VERTEX_POINT('',#127886);
#24398=VERTEX_POINT('',#127888);
#24399=VERTEX_POINT('',#127892);
#24400=VERTEX_POINT('',#127894);
#24401=VERTEX_POINT('',#127898);
#24402=VERTEX_POINT('',#127900);
#24403=VERTEX_POINT('',#127904);
#24404=VERTEX_POINT('',#127906);
#24405=VERTEX_POINT('',#127910);
#24406=VERTEX_POINT('',#127912);
#24407=VERTEX_POINT('',#127916);
#24408=VERTEX_POINT('',#127918);
#24409=VERTEX_POINT('',#127922);
#24410=VERTEX_POINT('',#127924);
#24411=VERTEX_POINT('',#127928);
#24412=VERTEX_POINT('',#127930);
#24413=VERTEX_POINT('',#127934);
#24414=VERTEX_POINT('',#127936);
#24415=VERTEX_POINT('',#127940);
#24416=VERTEX_POINT('',#127942);
#24417=VERTEX_POINT('',#127946);
#24418=VERTEX_POINT('',#127948);
#24419=VERTEX_POINT('',#127952);
#24420=VERTEX_POINT('',#127954);
#24421=VERTEX_POINT('',#127958);
#24422=VERTEX_POINT('',#127960);
#24423=VERTEX_POINT('',#127964);
#24424=VERTEX_POINT('',#127966);
#24425=VERTEX_POINT('',#127970);
#24426=VERTEX_POINT('',#127972);
#24427=VERTEX_POINT('',#127976);
#24428=VERTEX_POINT('',#127978);
#24429=VERTEX_POINT('',#127982);
#24430=VERTEX_POINT('',#127984);
#24431=VERTEX_POINT('',#127988);
#24432=VERTEX_POINT('',#127990);
#24433=VERTEX_POINT('',#127994);
#24434=VERTEX_POINT('',#127996);
#24435=VERTEX_POINT('',#128000);
#24436=VERTEX_POINT('',#128002);
#24437=VERTEX_POINT('',#128006);
#24438=VERTEX_POINT('',#128008);
#24439=VERTEX_POINT('',#128012);
#24440=VERTEX_POINT('',#128014);
#24441=VERTEX_POINT('',#128018);
#24442=VERTEX_POINT('',#128020);
#24443=VERTEX_POINT('',#128024);
#24444=VERTEX_POINT('',#128026);
#24445=VERTEX_POINT('',#128030);
#24446=VERTEX_POINT('',#128032);
#24447=VERTEX_POINT('',#128036);
#24448=VERTEX_POINT('',#128038);
#24449=VERTEX_POINT('',#128042);
#24450=VERTEX_POINT('',#128044);
#24451=VERTEX_POINT('',#128048);
#24452=VERTEX_POINT('',#128050);
#24453=VERTEX_POINT('',#128054);
#24454=VERTEX_POINT('',#128056);
#24455=VERTEX_POINT('',#128060);
#24456=VERTEX_POINT('',#128062);
#24457=VERTEX_POINT('',#128066);
#24458=VERTEX_POINT('',#128068);
#24459=VERTEX_POINT('',#128072);
#24460=VERTEX_POINT('',#128074);
#24461=VERTEX_POINT('',#128078);
#24462=VERTEX_POINT('',#128080);
#24463=VERTEX_POINT('',#128084);
#24464=VERTEX_POINT('',#128086);
#24465=VERTEX_POINT('',#128090);
#24466=VERTEX_POINT('',#128092);
#24467=VERTEX_POINT('',#128096);
#24468=VERTEX_POINT('',#128098);
#24469=VERTEX_POINT('',#128102);
#24470=VERTEX_POINT('',#128104);
#24471=VERTEX_POINT('',#128108);
#24472=VERTEX_POINT('',#128110);
#24473=VERTEX_POINT('',#128114);
#24474=VERTEX_POINT('',#128116);
#24475=VERTEX_POINT('',#128120);
#24476=VERTEX_POINT('',#128122);
#24477=VERTEX_POINT('',#128126);
#24478=VERTEX_POINT('',#128128);
#24479=VERTEX_POINT('',#128132);
#24480=VERTEX_POINT('',#128134);
#24481=VERTEX_POINT('',#128138);
#24482=VERTEX_POINT('',#128143);
#24483=VERTEX_POINT('',#128147);
#24484=VERTEX_POINT('',#128149);
#24485=VERTEX_POINT('',#128151);
#24486=VERTEX_POINT('',#128155);
#24487=VERTEX_POINT('',#128157);
#24488=VERTEX_POINT('',#128163);
#24489=VERTEX_POINT('',#128166);
#24490=VERTEX_POINT('',#128168);
#24491=VERTEX_POINT('',#128172);
#24492=VERTEX_POINT('',#128174);
#24493=VERTEX_POINT('',#128178);
#24494=VERTEX_POINT('',#128182);
#24495=VERTEX_POINT('',#128186);
#24496=VERTEX_POINT('',#128187);
#24497=VERTEX_POINT('',#128190);
#24498=VERTEX_POINT('',#128196);
#24499=VERTEX_POINT('',#128197);
#24500=VERTEX_POINT('',#128220);
#24501=VERTEX_POINT('',#128244);
#27754=EDGE_CURVE('',#22734,#22735,#19404,.T.);
#27755=EDGE_CURVE('',#22735,#22736,#2361,.T.);
#27756=EDGE_CURVE('',#22736,#22737,#19405,.T.);
#27757=EDGE_CURVE('',#22734,#22737,#2362,.T.);
#27758=EDGE_CURVE('',#22738,#22739,#2363,.T.);
#27759=EDGE_CURVE('',#22739,#22738,#2364,.T.);
#27760=EDGE_CURVE('',#22740,#22741,#2365,.T.);
#27761=EDGE_CURVE('',#22741,#22740,#2366,.T.);
#27762=EDGE_CURVE('',#22742,#22743,#2367,.T.);
#27763=EDGE_CURVE('',#22743,#22742,#2368,.T.);
#27764=EDGE_CURVE('',#22744,#22745,#2369,.T.);
#27765=EDGE_CURVE('',#22745,#22744,#2370,.T.);
#27766=EDGE_CURVE('',#22746,#22747,#2371,.T.);
#27767=EDGE_CURVE('',#22747,#22746,#2372,.T.);
#27768=EDGE_CURVE('',#22748,#22749,#2373,.T.);
#27769=EDGE_CURVE('',#22749,#22748,#2374,.T.);
#27770=EDGE_CURVE('',#22750,#22751,#2375,.T.);
#27771=EDGE_CURVE('',#22751,#22750,#2376,.T.);
#27772=EDGE_CURVE('',#22752,#22753,#2377,.T.);
#27773=EDGE_CURVE('',#22753,#22752,#2378,.T.);
#27774=EDGE_CURVE('',#22754,#22755,#2379,.T.);
#27775=EDGE_CURVE('',#22755,#22754,#2380,.T.);
#27776=EDGE_CURVE('',#22756,#22757,#2381,.T.);
#27777=EDGE_CURVE('',#22757,#22756,#2382,.T.);
#27778=EDGE_CURVE('',#22758,#22759,#2383,.T.);
#27779=EDGE_CURVE('',#22759,#22758,#2384,.T.);
#27780=EDGE_CURVE('',#22760,#22761,#2385,.T.);
#27781=EDGE_CURVE('',#22761,#22760,#2386,.T.);
#27782=EDGE_CURVE('',#22762,#22763,#2387,.T.);
#27783=EDGE_CURVE('',#22763,#22762,#2388,.T.);
#27784=EDGE_CURVE('',#22764,#22765,#2389,.T.);
#27785=EDGE_CURVE('',#22765,#22764,#2390,.T.);
#27786=EDGE_CURVE('',#22766,#22767,#2391,.T.);
#27787=EDGE_CURVE('',#22767,#22766,#2392,.T.);
#27788=EDGE_CURVE('',#22768,#22769,#2393,.T.);
#27789=EDGE_CURVE('',#22769,#22768,#2394,.T.);
#27790=EDGE_CURVE('',#22770,#22771,#2395,.T.);
#27791=EDGE_CURVE('',#22771,#22770,#2396,.T.);
#27792=EDGE_CURVE('',#22772,#22773,#2397,.T.);
#27793=EDGE_CURVE('',#22773,#22772,#2398,.T.);
#27794=EDGE_CURVE('',#22774,#22775,#2399,.T.);
#27795=EDGE_CURVE('',#22775,#22774,#2400,.T.);
#27796=EDGE_CURVE('',#22776,#22777,#2401,.T.);
#27797=EDGE_CURVE('',#22777,#22776,#2402,.T.);
#27798=EDGE_CURVE('',#22778,#22779,#2403,.T.);
#27799=EDGE_CURVE('',#22779,#22778,#2404,.T.);
#27800=EDGE_CURVE('',#22780,#22781,#2405,.T.);
#27801=EDGE_CURVE('',#22781,#22780,#2406,.T.);
#27802=EDGE_CURVE('',#22782,#22783,#2407,.T.);
#27803=EDGE_CURVE('',#22783,#22782,#2408,.T.);
#27804=EDGE_CURVE('',#22784,#22785,#2409,.T.);
#27805=EDGE_CURVE('',#22785,#22784,#2410,.T.);
#27806=EDGE_CURVE('',#22786,#22787,#2411,.T.);
#27807=EDGE_CURVE('',#22787,#22786,#2412,.T.);
#27808=EDGE_CURVE('',#22788,#22789,#2413,.T.);
#27809=EDGE_CURVE('',#22789,#22788,#2414,.T.);
#27810=EDGE_CURVE('',#22790,#22791,#2415,.T.);
#27811=EDGE_CURVE('',#22791,#22790,#2416,.T.);
#27812=EDGE_CURVE('',#22792,#22793,#2417,.T.);
#27813=EDGE_CURVE('',#22793,#22792,#2418,.T.);
#27814=EDGE_CURVE('',#22794,#22795,#2419,.T.);
#27815=EDGE_CURVE('',#22795,#22794,#2420,.T.);
#27816=EDGE_CURVE('',#22796,#22797,#2421,.T.);
#27817=EDGE_CURVE('',#22797,#22796,#2422,.T.);
#27818=EDGE_CURVE('',#22798,#22799,#2423,.T.);
#27819=EDGE_CURVE('',#22799,#22798,#2424,.T.);
#27820=EDGE_CURVE('',#22800,#22801,#2425,.T.);
#27821=EDGE_CURVE('',#22801,#22800,#2426,.T.);
#27822=EDGE_CURVE('',#22802,#22803,#2427,.T.);
#27823=EDGE_CURVE('',#22803,#22802,#2428,.T.);
#27824=EDGE_CURVE('',#22804,#22805,#2429,.T.);
#27825=EDGE_CURVE('',#22805,#22804,#2430,.T.);
#27826=EDGE_CURVE('',#22806,#22807,#2431,.T.);
#27827=EDGE_CURVE('',#22807,#22806,#2432,.T.);
#27828=EDGE_CURVE('',#22808,#22809,#2433,.T.);
#27829=EDGE_CURVE('',#22809,#22808,#2434,.T.);
#27830=EDGE_CURVE('',#22810,#22811,#2435,.T.);
#27831=EDGE_CURVE('',#22811,#22810,#2436,.T.);
#27832=EDGE_CURVE('',#22812,#22813,#2437,.T.);
#27833=EDGE_CURVE('',#22813,#22812,#2438,.T.);
#27834=EDGE_CURVE('',#22814,#22815,#2439,.T.);
#27835=EDGE_CURVE('',#22815,#22814,#2440,.T.);
#27836=EDGE_CURVE('',#22816,#22817,#2441,.T.);
#27837=EDGE_CURVE('',#22817,#22816,#2442,.T.);
#27838=EDGE_CURVE('',#22818,#22819,#2443,.T.);
#27839=EDGE_CURVE('',#22819,#22818,#2444,.T.);
#27840=EDGE_CURVE('',#22820,#22821,#2445,.T.);
#27841=EDGE_CURVE('',#22821,#22820,#2446,.T.);
#27842=EDGE_CURVE('',#22822,#22823,#2447,.T.);
#27843=EDGE_CURVE('',#22823,#22822,#2448,.T.);
#27844=EDGE_CURVE('',#22824,#22825,#2449,.T.);
#27845=EDGE_CURVE('',#22825,#22824,#2450,.T.);
#27846=EDGE_CURVE('',#22826,#22827,#2451,.T.);
#27847=EDGE_CURVE('',#22827,#22826,#2452,.T.);
#27848=EDGE_CURVE('',#22828,#22829,#2453,.T.);
#27849=EDGE_CURVE('',#22829,#22828,#2454,.T.);
#27850=EDGE_CURVE('',#22830,#22831,#2455,.T.);
#27851=EDGE_CURVE('',#22831,#22830,#2456,.T.);
#27852=EDGE_CURVE('',#22832,#22833,#2457,.T.);
#27853=EDGE_CURVE('',#22833,#22832,#2458,.T.);
#27854=EDGE_CURVE('',#22834,#22835,#2459,.T.);
#27855=EDGE_CURVE('',#22835,#22834,#2460,.T.);
#27856=EDGE_CURVE('',#22836,#22837,#2461,.T.);
#27857=EDGE_CURVE('',#22837,#22836,#2462,.T.);
#27858=EDGE_CURVE('',#22838,#22839,#2463,.T.);
#27859=EDGE_CURVE('',#22839,#22838,#2464,.T.);
#27860=EDGE_CURVE('',#22840,#22841,#2465,.T.);
#27861=EDGE_CURVE('',#22841,#22840,#2466,.T.);
#27862=EDGE_CURVE('',#22842,#22843,#2467,.T.);
#27863=EDGE_CURVE('',#22843,#22842,#2468,.T.);
#27864=EDGE_CURVE('',#22844,#22845,#2469,.T.);
#27865=EDGE_CURVE('',#22845,#22844,#2470,.T.);
#27866=EDGE_CURVE('',#22846,#22847,#2471,.T.);
#27867=EDGE_CURVE('',#22847,#22846,#2472,.T.);
#27868=EDGE_CURVE('',#22848,#22849,#2473,.T.);
#27869=EDGE_CURVE('',#22849,#22848,#2474,.T.);
#27870=EDGE_CURVE('',#22850,#22851,#2475,.T.);
#27871=EDGE_CURVE('',#22851,#22850,#2476,.T.);
#27872=EDGE_CURVE('',#22852,#22853,#2477,.T.);
#27873=EDGE_CURVE('',#22853,#22852,#2478,.T.);
#27874=EDGE_CURVE('',#22854,#22855,#2479,.T.);
#27875=EDGE_CURVE('',#22855,#22854,#2480,.T.);
#27876=EDGE_CURVE('',#22856,#22857,#2481,.T.);
#27877=EDGE_CURVE('',#22857,#22856,#2482,.T.);
#27878=EDGE_CURVE('',#22858,#22858,#19406,.T.);
#27879=EDGE_CURVE('',#22858,#22859,#19407,.T.);
#27880=EDGE_CURVE('',#22859,#22859,#19408,.T.);
#27881=EDGE_CURVE('',#22765,#22860,#5302,.T.);
#27882=EDGE_CURVE('',#22860,#22860,#2483,.T.);
#27883=EDGE_CURVE('',#22861,#22862,#2484,.T.);
#27884=EDGE_CURVE('',#22862,#22863,#5303,.T.);
#27885=EDGE_CURVE('',#22863,#22863,#19409,.T.);
#27886=EDGE_CURVE('',#22862,#22861,#2485,.T.);
#27887=EDGE_CURVE('',#22807,#22864,#5304,.T.);
#27888=EDGE_CURVE('',#22864,#22864,#2486,.T.);
#27889=EDGE_CURVE('',#22865,#22866,#2487,.T.);
#27890=EDGE_CURVE('',#22866,#22867,#5305,.T.);
#27891=EDGE_CURVE('',#22867,#22867,#19410,.T.);
#27892=EDGE_CURVE('',#22866,#22865,#2488,.T.);
#27893=EDGE_CURVE('',#22833,#22868,#5306,.T.);
#27894=EDGE_CURVE('',#22868,#22868,#2489,.T.);
#27895=EDGE_CURVE('',#22869,#22870,#2490,.T.);
#27896=EDGE_CURVE('',#22870,#22871,#5307,.T.);
#27897=EDGE_CURVE('',#22871,#22871,#19411,.T.);
#27898=EDGE_CURVE('',#22870,#22869,#2491,.T.);
#27899=EDGE_CURVE('',#22747,#22872,#5308,.T.);
#27900=EDGE_CURVE('',#22872,#22872,#2492,.T.);
#27901=EDGE_CURVE('',#22873,#22874,#2493,.T.);
#27902=EDGE_CURVE('',#22874,#22875,#5309,.T.);
#27903=EDGE_CURVE('',#22875,#22875,#19412,.T.);
#27904=EDGE_CURVE('',#22874,#22873,#2494,.T.);
#27905=EDGE_CURVE('',#22777,#22876,#5310,.T.);
#27906=EDGE_CURVE('',#22876,#22876,#2495,.T.);
#27907=EDGE_CURVE('',#22877,#22878,#2496,.T.);
#27908=EDGE_CURVE('',#22878,#22879,#5311,.T.);
#27909=EDGE_CURVE('',#22879,#22879,#19413,.T.);
#27910=EDGE_CURVE('',#22878,#22877,#2497,.T.);
#27911=EDGE_CURVE('',#22767,#22880,#5312,.T.);
#27912=EDGE_CURVE('',#22880,#22880,#2498,.T.);
#27913=EDGE_CURVE('',#22881,#22882,#2499,.T.);
#27914=EDGE_CURVE('',#22882,#22883,#5313,.T.);
#27915=EDGE_CURVE('',#22883,#22883,#19414,.T.);
#27916=EDGE_CURVE('',#22882,#22881,#2500,.T.);
#27917=EDGE_CURVE('',#22809,#22884,#5314,.T.);
#27918=EDGE_CURVE('',#22884,#22884,#2501,.T.);
#27919=EDGE_CURVE('',#22885,#22886,#2502,.T.);
#27920=EDGE_CURVE('',#22886,#22887,#5315,.T.);
#27921=EDGE_CURVE('',#22887,#22887,#19415,.T.);
#27922=EDGE_CURVE('',#22886,#22885,#2503,.T.);
#27923=EDGE_CURVE('',#22757,#22888,#5316,.T.);
#27924=EDGE_CURVE('',#22888,#22888,#2504,.T.);
#27925=EDGE_CURVE('',#22889,#22890,#2505,.T.);
#27926=EDGE_CURVE('',#22890,#22891,#5317,.T.);
#27927=EDGE_CURVE('',#22891,#22891,#19416,.T.);
#27928=EDGE_CURVE('',#22890,#22889,#2506,.T.);
#27929=EDGE_CURVE('',#22745,#22892,#5318,.T.);
#27930=EDGE_CURVE('',#22892,#22892,#2507,.T.);
#27931=EDGE_CURVE('',#22893,#22894,#2508,.T.);
#27932=EDGE_CURVE('',#22894,#22895,#5319,.T.);
#27933=EDGE_CURVE('',#22895,#22895,#19417,.T.);
#27934=EDGE_CURVE('',#22894,#22893,#2509,.T.);
#27935=EDGE_CURVE('',#22775,#22896,#5320,.T.);
#27936=EDGE_CURVE('',#22896,#22896,#2510,.T.);
#27937=EDGE_CURVE('',#22897,#22898,#2511,.T.);
#27938=EDGE_CURVE('',#22898,#22899,#5321,.T.);
#27939=EDGE_CURVE('',#22899,#22899,#19418,.T.);
#27940=EDGE_CURVE('',#22898,#22897,#2512,.T.);
#27941=EDGE_CURVE('',#22769,#22900,#5322,.T.);
#27942=EDGE_CURVE('',#22900,#22900,#2513,.T.);
#27943=EDGE_CURVE('',#22901,#22902,#2514,.T.);
#27944=EDGE_CURVE('',#22902,#22903,#5323,.T.);
#27945=EDGE_CURVE('',#22903,#22903,#19419,.T.);
#27946=EDGE_CURVE('',#22902,#22901,#2515,.T.);
#27947=EDGE_CURVE('',#22749,#22904,#5324,.T.);
#27948=EDGE_CURVE('',#22904,#22904,#2516,.T.);
#27949=EDGE_CURVE('',#22905,#22906,#2517,.T.);
#27950=EDGE_CURVE('',#22906,#22907,#5325,.T.);
#27951=EDGE_CURVE('',#22907,#22907,#19420,.T.);
#27952=EDGE_CURVE('',#22906,#22905,#2518,.T.);
#27953=EDGE_CURVE('',#22759,#22908,#5326,.T.);
#27954=EDGE_CURVE('',#22908,#22908,#2519,.T.);
#27955=EDGE_CURVE('',#22909,#22910,#2520,.T.);
#27956=EDGE_CURVE('',#22910,#22911,#5327,.T.);
#27957=EDGE_CURVE('',#22911,#22911,#19421,.T.);
#27958=EDGE_CURVE('',#22910,#22909,#2521,.T.);
#27959=EDGE_CURVE('',#22743,#22912,#5328,.T.);
#27960=EDGE_CURVE('',#22912,#22912,#2522,.T.);
#27961=EDGE_CURVE('',#22913,#22914,#2523,.T.);
#27962=EDGE_CURVE('',#22914,#22915,#5329,.T.);
#27963=EDGE_CURVE('',#22915,#22915,#19422,.T.);
#27964=EDGE_CURVE('',#22914,#22913,#2524,.T.);
#27965=EDGE_CURVE('',#22773,#22916,#5330,.T.);
#27966=EDGE_CURVE('',#22916,#22916,#2525,.T.);
#27967=EDGE_CURVE('',#22917,#22918,#2526,.T.);
#27968=EDGE_CURVE('',#22918,#22919,#5331,.T.);
#27969=EDGE_CURVE('',#22919,#22919,#19423,.T.);
#27970=EDGE_CURVE('',#22918,#22917,#2527,.T.);
#27971=EDGE_CURVE('',#22793,#22920,#5332,.T.);
#27972=EDGE_CURVE('',#22920,#22920,#2528,.T.);
#27973=EDGE_CURVE('',#22921,#22922,#2529,.T.);
#27974=EDGE_CURVE('',#22922,#22923,#5333,.T.);
#27975=EDGE_CURVE('',#22923,#22923,#19424,.T.);
#27976=EDGE_CURVE('',#22922,#22921,#2530,.T.);
#27977=EDGE_CURVE('',#22751,#22924,#5334,.T.);
#27978=EDGE_CURVE('',#22924,#22924,#2531,.T.);
#27979=EDGE_CURVE('',#22925,#22926,#2532,.T.);
#27980=EDGE_CURVE('',#22926,#22927,#5335,.T.);
#27981=EDGE_CURVE('',#22927,#22927,#19425,.T.);
#27982=EDGE_CURVE('',#22926,#22925,#2533,.T.);
#27983=EDGE_CURVE('',#22761,#22928,#5336,.T.);
#27984=EDGE_CURVE('',#22928,#22928,#2534,.T.);
#27985=EDGE_CURVE('',#22929,#22930,#2535,.T.);
#27986=EDGE_CURVE('',#22930,#22931,#5337,.T.);
#27987=EDGE_CURVE('',#22931,#22931,#19426,.T.);
#27988=EDGE_CURVE('',#22930,#22929,#2536,.T.);
#27989=EDGE_CURVE('',#22741,#22932,#5338,.T.);
#27990=EDGE_CURVE('',#22932,#22932,#2537,.T.);
#27991=EDGE_CURVE('',#22933,#22934,#2538,.T.);
#27992=EDGE_CURVE('',#22934,#22935,#5339,.T.);
#27993=EDGE_CURVE('',#22935,#22935,#19427,.T.);
#27994=EDGE_CURVE('',#22934,#22933,#2539,.T.);
#27995=EDGE_CURVE('',#22795,#22936,#5340,.T.);
#27996=EDGE_CURVE('',#22936,#22936,#2540,.T.);
#27997=EDGE_CURVE('',#22937,#22938,#2541,.T.);
#27998=EDGE_CURVE('',#22938,#22939,#5341,.T.);
#27999=EDGE_CURVE('',#22939,#22939,#19428,.T.);
#28000=EDGE_CURVE('',#22938,#22937,#2542,.T.);
#28001=EDGE_CURVE('',#22791,#22940,#5342,.T.);
#28002=EDGE_CURVE('',#22940,#22940,#2543,.T.);
#28003=EDGE_CURVE('',#22941,#22942,#2544,.T.);
#28004=EDGE_CURVE('',#22942,#22943,#5343,.T.);
#28005=EDGE_CURVE('',#22943,#22943,#19429,.T.);
#28006=EDGE_CURVE('',#22942,#22941,#2545,.T.);
#28007=EDGE_CURVE('',#22753,#22944,#5344,.T.);
#28008=EDGE_CURVE('',#22944,#22944,#2546,.T.);
#28009=EDGE_CURVE('',#22945,#22946,#2547,.T.);
#28010=EDGE_CURVE('',#22946,#22947,#5345,.T.);
#28011=EDGE_CURVE('',#22947,#22947,#19430,.T.);
#28012=EDGE_CURVE('',#22946,#22945,#2548,.T.);
#28013=EDGE_CURVE('',#22739,#22948,#5346,.T.);
#28014=EDGE_CURVE('',#22948,#22948,#2549,.T.);
#28015=EDGE_CURVE('',#22949,#22950,#2550,.T.);
#28016=EDGE_CURVE('',#22950,#22951,#5347,.T.);
#28017=EDGE_CURVE('',#22951,#22951,#19431,.T.);
#28018=EDGE_CURVE('',#22950,#22949,#2551,.T.);
#28019=EDGE_CURVE('',#22783,#22952,#5348,.T.);
#28020=EDGE_CURVE('',#22952,#22952,#2552,.T.);
#28021=EDGE_CURVE('',#22953,#22954,#2553,.T.);
#28022=EDGE_CURVE('',#22954,#22955,#5349,.T.);
#28023=EDGE_CURVE('',#22955,#22955,#19432,.T.);
#28024=EDGE_CURVE('',#22954,#22953,#2554,.T.);
#28025=EDGE_CURVE('',#22797,#22956,#5350,.T.);
#28026=EDGE_CURVE('',#22956,#22956,#2555,.T.);
#28027=EDGE_CURVE('',#22957,#22958,#2556,.T.);
#28028=EDGE_CURVE('',#22958,#22959,#5351,.T.);
#28029=EDGE_CURVE('',#22959,#22959,#19433,.T.);
#28030=EDGE_CURVE('',#22958,#22957,#2557,.T.);
#28031=EDGE_CURVE('',#22789,#22960,#5352,.T.);
#28032=EDGE_CURVE('',#22960,#22960,#2558,.T.);
#28033=EDGE_CURVE('',#22961,#22962,#2559,.T.);
#28034=EDGE_CURVE('',#22962,#22963,#5353,.T.);
#28035=EDGE_CURVE('',#22963,#22963,#19434,.T.);
#28036=EDGE_CURVE('',#22962,#22961,#2560,.T.);
#28037=EDGE_CURVE('',#22755,#22964,#5354,.T.);
#28038=EDGE_CURVE('',#22964,#22964,#2561,.T.);
#28039=EDGE_CURVE('',#22965,#22966,#2562,.T.);
#28040=EDGE_CURVE('',#22966,#22967,#5355,.T.);
#28041=EDGE_CURVE('',#22967,#22967,#19435,.T.);
#28042=EDGE_CURVE('',#22966,#22965,#2563,.T.);
#28043=EDGE_CURVE('',#22785,#22968,#5356,.T.);
#28044=EDGE_CURVE('',#22969,#22968,#2564,.T.);
#28045=EDGE_CURVE('',#22968,#22969,#2565,.T.);
#28046=EDGE_CURVE('',#22970,#22971,#2566,.T.);
#28047=EDGE_CURVE('',#22971,#22972,#5357,.T.);
#28048=EDGE_CURVE('',#22972,#22972,#19436,.T.);
#28049=EDGE_CURVE('',#22971,#22970,#2567,.T.);
#28050=EDGE_CURVE('',#22781,#22973,#5358,.T.);
#28051=EDGE_CURVE('',#22973,#22973,#2568,.T.);
#28052=EDGE_CURVE('',#22974,#22975,#2569,.T.);
#28053=EDGE_CURVE('',#22975,#22976,#5359,.T.);
#28054=EDGE_CURVE('',#22976,#22976,#19437,.T.);
#28055=EDGE_CURVE('',#22975,#22974,#2570,.T.);
#28056=EDGE_CURVE('',#22799,#22977,#5360,.T.);
#28057=EDGE_CURVE('',#22977,#22977,#2571,.T.);
#28058=EDGE_CURVE('',#22978,#22979,#2572,.T.);
#28059=EDGE_CURVE('',#22979,#22980,#5361,.T.);
#28060=EDGE_CURVE('',#22980,#22980,#19438,.T.);
#28061=EDGE_CURVE('',#22979,#22978,#2573,.T.);
#28062=EDGE_CURVE('',#22787,#22981,#5362,.T.);
#28063=EDGE_CURVE('',#22981,#22981,#2574,.T.);
#28064=EDGE_CURVE('',#22982,#22983,#2575,.T.);
#28065=EDGE_CURVE('',#22983,#22984,#5363,.T.);
#28066=EDGE_CURVE('',#22984,#22984,#19439,.T.);
#28067=EDGE_CURVE('',#22983,#22982,#2576,.T.);
#28068=EDGE_CURVE('',#22985,#22985,#2577,.T.);
#28069=EDGE_CURVE('',#22985,#22986,#5364,.T.);
#28070=EDGE_CURVE('',#22986,#22986,#2578,.T.);
#28071=EDGE_CURVE('',#22987,#22988,#2579,.T.);
#28072=EDGE_CURVE('',#22988,#22989,#5365,.T.);
#28073=EDGE_CURVE('',#22989,#22989,#19440,.T.);
#28074=EDGE_CURVE('',#22988,#22987,#2580,.T.);
#28075=EDGE_CURVE('',#22990,#22990,#2581,.T.);
#28076=EDGE_CURVE('',#22990,#22991,#5366,.T.);
#28077=EDGE_CURVE('',#22991,#22991,#2582,.T.);
#28078=EDGE_CURVE('',#22992,#22993,#2583,.T.);
#28079=EDGE_CURVE('',#22993,#22994,#5367,.T.);
#28080=EDGE_CURVE('',#22994,#22994,#19441,.T.);
#28081=EDGE_CURVE('',#22993,#22992,#2584,.T.);
#28082=EDGE_CURVE('',#22779,#22995,#5368,.T.);
#28083=EDGE_CURVE('',#22995,#22995,#2585,.T.);
#28084=EDGE_CURVE('',#22996,#22997,#2586,.T.);
#28085=EDGE_CURVE('',#22997,#22998,#5369,.T.);
#28086=EDGE_CURVE('',#22998,#22998,#19442,.T.);
#28087=EDGE_CURVE('',#22997,#22996,#2587,.T.);
#28088=EDGE_CURVE('',#22801,#22999,#5370,.T.);
#28089=EDGE_CURVE('',#22999,#22999,#2588,.T.);
#28090=EDGE_CURVE('',#23000,#23001,#2589,.T.);
#28091=EDGE_CURVE('',#23001,#23002,#5371,.T.);
#28092=EDGE_CURVE('',#23002,#23002,#19443,.T.);
#28093=EDGE_CURVE('',#23001,#23000,#2590,.T.);
#28094=EDGE_CURVE('',#23003,#23003,#2591,.T.);
#28095=EDGE_CURVE('',#23003,#23004,#5372,.T.);
#28096=EDGE_CURVE('',#23004,#23004,#2592,.T.);
#28097=EDGE_CURVE('',#23005,#23006,#2593,.T.);
#28098=EDGE_CURVE('',#23006,#23007,#5373,.T.);
#28099=EDGE_CURVE('',#23007,#23007,#19444,.T.);
#28100=EDGE_CURVE('',#23006,#23005,#2594,.T.);
#28101=EDGE_CURVE('',#23008,#23008,#2595,.T.);
#28102=EDGE_CURVE('',#23008,#23009,#5374,.T.);
#28103=EDGE_CURVE('',#23009,#23009,#2596,.T.);
#28104=EDGE_CURVE('',#23010,#23011,#2597,.T.);
#28105=EDGE_CURVE('',#23011,#23012,#5375,.T.);
#28106=EDGE_CURVE('',#23012,#23012,#19445,.T.);
#28107=EDGE_CURVE('',#23011,#23010,#2598,.T.);
#28108=EDGE_CURVE('',#23013,#23013,#2599,.T.);
#28109=EDGE_CURVE('',#23013,#23014,#5376,.T.);
#28110=EDGE_CURVE('',#23014,#23014,#2600,.T.);
#28111=EDGE_CURVE('',#23015,#23016,#2601,.T.);
#28112=EDGE_CURVE('',#23016,#23017,#5377,.T.);
#28113=EDGE_CURVE('',#23017,#23017,#19446,.T.);
#28114=EDGE_CURVE('',#23016,#23015,#2602,.T.);
#28115=EDGE_CURVE('',#23018,#23018,#2603,.T.);
#28116=EDGE_CURVE('',#23018,#23019,#5378,.T.);
#28117=EDGE_CURVE('',#23019,#23019,#2604,.T.);
#28118=EDGE_CURVE('',#23020,#23021,#2605,.T.);
#28119=EDGE_CURVE('',#23021,#23022,#5379,.T.);
#28120=EDGE_CURVE('',#23022,#23022,#19447,.T.);
#28121=EDGE_CURVE('',#23021,#23020,#2606,.T.);
#28122=EDGE_CURVE('',#23023,#23023,#2607,.T.);
#28123=EDGE_CURVE('',#23023,#23024,#5380,.T.);
#28124=EDGE_CURVE('',#23024,#23024,#2608,.T.);
#28125=EDGE_CURVE('',#23025,#23026,#2609,.T.);
#28126=EDGE_CURVE('',#23026,#23027,#5381,.T.);
#28127=EDGE_CURVE('',#23027,#23027,#19448,.T.);
#28128=EDGE_CURVE('',#23026,#23025,#2610,.T.);
#28129=EDGE_CURVE('',#23028,#23028,#2611,.T.);
#28130=EDGE_CURVE('',#23028,#23029,#5382,.T.);
#28131=EDGE_CURVE('',#23029,#23029,#2612,.T.);
#28132=EDGE_CURVE('',#23030,#23031,#2613,.T.);
#28133=EDGE_CURVE('',#23031,#23032,#5383,.T.);
#28134=EDGE_CURVE('',#23032,#23032,#19449,.T.);
#28135=EDGE_CURVE('',#23031,#23030,#2614,.T.);
#28136=EDGE_CURVE('',#23033,#23033,#2615,.T.);
#28137=EDGE_CURVE('',#23033,#23034,#5384,.T.);
#28138=EDGE_CURVE('',#23034,#23034,#2616,.T.);
#28139=EDGE_CURVE('',#23035,#23036,#2617,.T.);
#28140=EDGE_CURVE('',#23036,#23037,#5385,.T.);
#28141=EDGE_CURVE('',#23037,#23037,#19450,.T.);
#28142=EDGE_CURVE('',#23036,#23035,#2618,.T.);
#28143=EDGE_CURVE('',#23038,#23038,#2619,.T.);
#28144=EDGE_CURVE('',#23038,#23039,#5386,.T.);
#28145=EDGE_CURVE('',#23039,#23039,#2620,.T.);
#28146=EDGE_CURVE('',#23040,#23041,#2621,.T.);
#28147=EDGE_CURVE('',#23041,#23042,#5387,.T.);
#28148=EDGE_CURVE('',#23042,#23042,#19451,.T.);
#28149=EDGE_CURVE('',#23041,#23040,#2622,.T.);
#28150=EDGE_CURVE('',#23043,#23043,#2623,.T.);
#28151=EDGE_CURVE('',#23043,#23044,#5388,.T.);
#28152=EDGE_CURVE('',#23044,#23044,#2624,.T.);
#28153=EDGE_CURVE('',#23045,#23046,#2625,.T.);
#28154=EDGE_CURVE('',#23046,#23047,#5389,.T.);
#28155=EDGE_CURVE('',#23047,#23047,#19452,.T.);
#28156=EDGE_CURVE('',#23046,#23045,#2626,.T.);
#28157=EDGE_CURVE('',#23048,#23048,#2627,.T.);
#28158=EDGE_CURVE('',#23048,#23049,#5390,.T.);
#28159=EDGE_CURVE('',#23049,#23049,#2628,.T.);
#28160=EDGE_CURVE('',#23050,#23051,#2629,.T.);
#28161=EDGE_CURVE('',#23051,#23052,#5391,.T.);
#28162=EDGE_CURVE('',#23052,#23052,#19453,.T.);
#28163=EDGE_CURVE('',#23051,#23050,#2630,.T.);
#28164=EDGE_CURVE('',#23053,#23053,#2631,.T.);
#28165=EDGE_CURVE('',#23053,#23054,#5392,.T.);
#28166=EDGE_CURVE('',#23054,#23054,#2632,.T.);
#28167=EDGE_CURVE('',#23055,#23056,#2633,.T.);
#28168=EDGE_CURVE('',#23056,#23057,#5393,.T.);
#28169=EDGE_CURVE('',#23057,#23057,#19454,.T.);
#28170=EDGE_CURVE('',#23056,#23055,#2634,.T.);
#28171=EDGE_CURVE('',#23058,#23058,#2635,.T.);
#28172=EDGE_CURVE('',#23058,#23059,#5394,.T.);
#28173=EDGE_CURVE('',#23059,#23059,#2636,.T.);
#28174=EDGE_CURVE('',#23060,#23061,#2637,.T.);
#28175=EDGE_CURVE('',#23061,#23062,#5395,.T.);
#28176=EDGE_CURVE('',#23062,#23062,#19455,.T.);
#28177=EDGE_CURVE('',#23061,#23060,#2638,.T.);
#28178=EDGE_CURVE('',#23063,#23063,#2639,.T.);
#28179=EDGE_CURVE('',#23063,#23064,#5396,.T.);
#28180=EDGE_CURVE('',#23064,#23064,#2640,.T.);
#28181=EDGE_CURVE('',#23065,#23066,#2641,.T.);
#28182=EDGE_CURVE('',#23066,#23067,#5397,.T.);
#28183=EDGE_CURVE('',#23067,#23067,#19456,.T.);
#28184=EDGE_CURVE('',#23066,#23065,#2642,.T.);
#28185=EDGE_CURVE('',#23068,#23068,#2643,.T.);
#28186=EDGE_CURVE('',#23068,#23069,#5398,.T.);
#28187=EDGE_CURVE('',#23069,#23069,#2644,.T.);
#28188=EDGE_CURVE('',#23070,#23071,#2645,.T.);
#28189=EDGE_CURVE('',#23071,#23072,#5399,.T.);
#28190=EDGE_CURVE('',#23072,#23072,#19457,.T.);
#28191=EDGE_CURVE('',#23071,#23070,#2646,.T.);
#28192=EDGE_CURVE('',#23073,#23073,#2647,.T.);
#28193=EDGE_CURVE('',#23073,#23074,#5400,.T.);
#28194=EDGE_CURVE('',#23074,#23074,#2648,.T.);
#28195=EDGE_CURVE('',#23075,#23076,#2649,.T.);
#28196=EDGE_CURVE('',#23076,#23077,#5401,.T.);
#28197=EDGE_CURVE('',#23077,#23077,#19458,.T.);
#28198=EDGE_CURVE('',#23076,#23075,#2650,.T.);
#28199=EDGE_CURVE('',#23078,#23078,#2651,.T.);
#28200=EDGE_CURVE('',#23078,#23079,#5402,.T.);
#28201=EDGE_CURVE('',#23079,#23079,#2652,.T.);
#28202=EDGE_CURVE('',#23080,#23081,#2653,.T.);
#28203=EDGE_CURVE('',#23081,#23082,#5403,.T.);
#28204=EDGE_CURVE('',#23082,#23082,#19459,.T.);
#28205=EDGE_CURVE('',#23081,#23080,#2654,.T.);
#28206=EDGE_CURVE('',#23083,#23083,#2655,.T.);
#28207=EDGE_CURVE('',#23083,#23084,#5404,.T.);
#28208=EDGE_CURVE('',#23084,#23084,#2656,.T.);
#28209=EDGE_CURVE('',#23085,#23086,#2657,.T.);
#28210=EDGE_CURVE('',#23086,#23087,#5405,.T.);
#28211=EDGE_CURVE('',#23087,#23087,#19460,.T.);
#28212=EDGE_CURVE('',#23086,#23085,#2658,.T.);
#28213=EDGE_CURVE('',#23088,#23088,#2659,.T.);
#28214=EDGE_CURVE('',#23088,#23089,#5406,.T.);
#28215=EDGE_CURVE('',#23089,#23089,#2660,.T.);
#28216=EDGE_CURVE('',#23090,#23091,#2661,.T.);
#28217=EDGE_CURVE('',#23091,#23092,#5407,.T.);
#28218=EDGE_CURVE('',#23092,#23092,#19461,.T.);
#28219=EDGE_CURVE('',#23091,#23090,#2662,.T.);
#28220=EDGE_CURVE('',#23093,#23093,#2663,.T.);
#28221=EDGE_CURVE('',#23093,#23094,#5408,.T.);
#28222=EDGE_CURVE('',#23094,#23094,#2664,.T.);
#28223=EDGE_CURVE('',#23095,#23096,#2665,.T.);
#28224=EDGE_CURVE('',#23096,#23097,#5409,.T.);
#28225=EDGE_CURVE('',#23097,#23097,#19462,.T.);
#28226=EDGE_CURVE('',#23096,#23095,#2666,.T.);
#28227=EDGE_CURVE('',#23098,#23098,#2667,.T.);
#28228=EDGE_CURVE('',#23098,#23099,#5410,.T.);
#28229=EDGE_CURVE('',#23099,#23099,#2668,.T.);
#28230=EDGE_CURVE('',#23100,#23101,#2669,.T.);
#28231=EDGE_CURVE('',#23101,#23102,#5411,.T.);
#28232=EDGE_CURVE('',#23102,#23102,#19463,.T.);
#28233=EDGE_CURVE('',#23101,#23100,#2670,.T.);
#28234=EDGE_CURVE('',#23103,#23103,#2671,.T.);
#28235=EDGE_CURVE('',#23103,#23104,#5412,.T.);
#28236=EDGE_CURVE('',#23104,#23104,#2672,.T.);
#28237=EDGE_CURVE('',#23105,#23106,#2673,.T.);
#28238=EDGE_CURVE('',#23106,#23107,#5413,.T.);
#28239=EDGE_CURVE('',#23107,#23107,#19464,.T.);
#28240=EDGE_CURVE('',#23106,#23105,#2674,.T.);
#28241=EDGE_CURVE('',#23108,#23108,#2675,.T.);
#28242=EDGE_CURVE('',#23108,#23109,#5414,.T.);
#28243=EDGE_CURVE('',#23109,#23109,#2676,.T.);
#28244=EDGE_CURVE('',#23110,#23111,#2677,.T.);
#28245=EDGE_CURVE('',#23111,#23112,#5415,.T.);
#28246=EDGE_CURVE('',#23112,#23112,#19465,.T.);
#28247=EDGE_CURVE('',#23111,#23110,#2678,.T.);
#28248=EDGE_CURVE('',#23113,#23113,#2679,.T.);
#28249=EDGE_CURVE('',#23113,#23114,#5416,.T.);
#28250=EDGE_CURVE('',#23114,#23114,#2680,.T.);
#28251=EDGE_CURVE('',#23115,#23116,#2681,.T.);
#28252=EDGE_CURVE('',#23116,#23117,#5417,.T.);
#28253=EDGE_CURVE('',#23117,#23117,#19466,.T.);
#28254=EDGE_CURVE('',#23116,#23115,#2682,.T.);
#28255=EDGE_CURVE('',#23118,#23118,#2683,.T.);
#28256=EDGE_CURVE('',#23118,#23119,#5418,.T.);
#28257=EDGE_CURVE('',#23119,#23119,#2684,.T.);
#28258=EDGE_CURVE('',#23120,#23121,#2685,.T.);
#28259=EDGE_CURVE('',#23121,#23122,#5419,.T.);
#28260=EDGE_CURVE('',#23122,#23122,#19467,.T.);
#28261=EDGE_CURVE('',#23121,#23120,#2686,.T.);
#28262=EDGE_CURVE('',#23123,#23123,#2687,.T.);
#28263=EDGE_CURVE('',#23123,#23124,#5420,.T.);
#28264=EDGE_CURVE('',#23124,#23124,#2688,.T.);
#28265=EDGE_CURVE('',#23125,#23126,#2689,.T.);
#28266=EDGE_CURVE('',#23126,#23127,#5421,.T.);
#28267=EDGE_CURVE('',#23127,#23127,#19468,.T.);
#28268=EDGE_CURVE('',#23126,#23125,#2690,.T.);
#28269=EDGE_CURVE('',#23128,#23128,#2691,.T.);
#28270=EDGE_CURVE('',#23128,#23129,#5422,.T.);
#28271=EDGE_CURVE('',#23129,#23129,#2692,.T.);
#28272=EDGE_CURVE('',#23130,#23131,#2693,.T.);
#28273=EDGE_CURVE('',#23131,#23132,#5423,.T.);
#28274=EDGE_CURVE('',#23132,#23132,#19469,.T.);
#28275=EDGE_CURVE('',#23131,#23130,#2694,.T.);
#28276=EDGE_CURVE('',#23133,#23133,#2695,.T.);
#28277=EDGE_CURVE('',#23133,#23134,#5424,.T.);
#28278=EDGE_CURVE('',#23134,#23134,#2696,.T.);
#28279=EDGE_CURVE('',#23135,#23136,#2697,.T.);
#28280=EDGE_CURVE('',#23136,#23137,#5425,.T.);
#28281=EDGE_CURVE('',#23137,#23137,#19470,.T.);
#28282=EDGE_CURVE('',#23136,#23135,#2698,.T.);
#28283=EDGE_CURVE('',#23138,#23138,#2699,.T.);
#28284=EDGE_CURVE('',#23138,#23139,#5426,.T.);
#28285=EDGE_CURVE('',#23139,#23139,#2700,.T.);
#28286=EDGE_CURVE('',#23140,#23141,#2701,.T.);
#28287=EDGE_CURVE('',#23141,#23142,#5427,.T.);
#28288=EDGE_CURVE('',#23142,#23142,#19471,.T.);
#28289=EDGE_CURVE('',#23141,#23140,#2702,.T.);
#28290=EDGE_CURVE('',#23143,#23143,#2703,.T.);
#28291=EDGE_CURVE('',#23143,#23144,#5428,.T.);
#28292=EDGE_CURVE('',#23145,#23144,#2704,.T.);
#28293=EDGE_CURVE('',#23144,#23145,#2705,.T.);
#28294=EDGE_CURVE('',#23146,#23147,#2706,.T.);
#28295=EDGE_CURVE('',#23147,#23148,#5429,.T.);
#28296=EDGE_CURVE('',#23148,#23148,#19472,.T.);
#28297=EDGE_CURVE('',#23147,#23146,#2707,.T.);
#28298=EDGE_CURVE('',#23149,#23149,#2708,.T.);
#28299=EDGE_CURVE('',#23149,#23150,#5430,.T.);
#28300=EDGE_CURVE('',#23150,#23150,#2709,.T.);
#28301=EDGE_CURVE('',#23151,#23152,#2710,.T.);
#28302=EDGE_CURVE('',#23152,#23153,#5431,.T.);
#28303=EDGE_CURVE('',#23153,#23153,#19473,.T.);
#28304=EDGE_CURVE('',#23152,#23151,#2711,.T.);
#28305=EDGE_CURVE('',#23154,#23154,#2712,.T.);
#28306=EDGE_CURVE('',#23154,#23155,#5432,.T.);
#28307=EDGE_CURVE('',#23155,#23155,#2713,.T.);
#28308=EDGE_CURVE('',#23156,#23157,#2714,.T.);
#28309=EDGE_CURVE('',#23157,#23158,#5433,.T.);
#28310=EDGE_CURVE('',#23158,#23158,#19474,.T.);
#28311=EDGE_CURVE('',#23157,#23156,#2715,.T.);
#28312=EDGE_CURVE('',#23159,#23159,#2716,.T.);
#28313=EDGE_CURVE('',#23159,#23160,#5434,.T.);
#28314=EDGE_CURVE('',#23160,#23160,#2717,.T.);
#28315=EDGE_CURVE('',#23161,#23162,#2718,.T.);
#28316=EDGE_CURVE('',#23162,#23163,#5435,.T.);
#28317=EDGE_CURVE('',#23163,#23163,#19475,.T.);
#28318=EDGE_CURVE('',#23162,#23161,#2719,.T.);
#28319=EDGE_CURVE('',#23164,#23164,#2720,.T.);
#28320=EDGE_CURVE('',#23164,#23165,#5436,.T.);
#28321=EDGE_CURVE('',#23166,#23165,#2721,.T.);
#28322=EDGE_CURVE('',#23165,#23166,#2722,.T.);
#28323=EDGE_CURVE('',#23167,#23168,#2723,.T.);
#28324=EDGE_CURVE('',#23168,#23169,#5437,.T.);
#28325=EDGE_CURVE('',#23169,#23169,#19476,.T.);
#28326=EDGE_CURVE('',#23168,#23167,#2724,.T.);
#28327=EDGE_CURVE('',#23170,#23170,#2725,.T.);
#28328=EDGE_CURVE('',#23170,#23171,#5438,.T.);
#28329=EDGE_CURVE('',#23171,#23171,#2726,.T.);
#28330=EDGE_CURVE('',#23172,#23173,#2727,.T.);
#28331=EDGE_CURVE('',#23173,#23174,#5439,.T.);
#28332=EDGE_CURVE('',#23174,#23174,#19477,.T.);
#28333=EDGE_CURVE('',#23173,#23172,#2728,.T.);
#28334=EDGE_CURVE('',#23175,#23175,#2729,.T.);
#28335=EDGE_CURVE('',#23175,#23176,#5440,.T.);
#28336=EDGE_CURVE('',#23176,#23176,#2730,.T.);
#28337=EDGE_CURVE('',#23177,#23178,#2731,.T.);
#28338=EDGE_CURVE('',#23178,#23179,#5441,.T.);
#28339=EDGE_CURVE('',#23179,#23179,#19478,.T.);
#28340=EDGE_CURVE('',#23178,#23177,#2732,.T.);
#28341=EDGE_CURVE('',#23180,#23180,#2733,.T.);
#28342=EDGE_CURVE('',#23180,#23181,#5442,.T.);
#28343=EDGE_CURVE('',#23181,#23181,#2734,.T.);
#28344=EDGE_CURVE('',#23182,#23183,#2735,.T.);
#28345=EDGE_CURVE('',#23183,#23184,#5443,.T.);
#28346=EDGE_CURVE('',#23184,#23184,#19479,.T.);
#28347=EDGE_CURVE('',#23183,#23182,#2736,.T.);
#28348=EDGE_CURVE('',#23185,#23186,#2737,.T.);
#28349=EDGE_CURVE('',#23185,#23187,#5444,.T.);
#28350=EDGE_CURVE('',#23188,#23187,#2738,.T.);
#28351=EDGE_CURVE('',#23187,#23188,#2739,.T.);
#28352=EDGE_CURVE('',#23186,#23185,#2740,.T.);
#28353=EDGE_CURVE('',#23189,#23190,#2741,.T.);
#28354=EDGE_CURVE('',#23190,#23191,#5445,.T.);
#28355=EDGE_CURVE('',#23191,#23191,#19480,.T.);
#28356=EDGE_CURVE('',#23190,#23189,#2742,.T.);
#28357=EDGE_CURVE('',#23192,#23192,#2743,.T.);
#28358=EDGE_CURVE('',#23192,#23193,#5446,.T.);
#28359=EDGE_CURVE('',#23193,#23193,#2744,.T.);
#28360=EDGE_CURVE('',#23194,#23195,#2745,.T.);
#28361=EDGE_CURVE('',#23195,#23196,#5447,.T.);
#28362=EDGE_CURVE('',#23196,#23196,#19481,.T.);
#28363=EDGE_CURVE('',#23195,#23194,#2746,.T.);
#28364=EDGE_CURVE('',#23197,#23197,#2747,.T.);
#28365=EDGE_CURVE('',#23197,#23198,#5448,.T.);
#28366=EDGE_CURVE('',#23198,#23198,#2748,.T.);
#28367=EDGE_CURVE('',#23199,#23200,#2749,.T.);
#28368=EDGE_CURVE('',#23200,#23201,#5449,.T.);
#28369=EDGE_CURVE('',#23201,#23201,#19482,.T.);
#28370=EDGE_CURVE('',#23200,#23199,#2750,.T.);
#28371=EDGE_CURVE('',#23202,#23202,#2751,.T.);
#28372=EDGE_CURVE('',#23202,#23203,#5450,.T.);
#28373=EDGE_CURVE('',#23203,#23203,#2752,.T.);
#28374=EDGE_CURVE('',#23204,#23205,#2753,.T.);
#28375=EDGE_CURVE('',#23205,#23206,#5451,.T.);
#28376=EDGE_CURVE('',#23206,#23206,#19483,.T.);
#28377=EDGE_CURVE('',#23205,#23204,#2754,.T.);
#28378=EDGE_CURVE('',#23207,#23207,#2755,.T.);
#28379=EDGE_CURVE('',#23207,#23208,#5452,.T.);
#28380=EDGE_CURVE('',#23208,#23208,#2756,.T.);
#28381=EDGE_CURVE('',#23209,#23210,#2757,.T.);
#28382=EDGE_CURVE('',#23210,#23211,#5453,.T.);
#28383=EDGE_CURVE('',#23211,#23211,#19484,.T.);
#28384=EDGE_CURVE('',#23210,#23209,#2758,.T.);
#28385=EDGE_CURVE('',#23212,#23212,#2759,.T.);
#28386=EDGE_CURVE('',#23212,#23213,#5454,.T.);
#28387=EDGE_CURVE('',#23213,#23213,#2760,.T.);
#28388=EDGE_CURVE('',#23214,#23215,#2761,.T.);
#28389=EDGE_CURVE('',#23215,#23216,#5455,.T.);
#28390=EDGE_CURVE('',#23216,#23216,#19485,.T.);
#28391=EDGE_CURVE('',#23215,#23214,#2762,.T.);
#28392=EDGE_CURVE('',#23217,#23217,#2763,.T.);
#28393=EDGE_CURVE('',#23217,#23218,#5456,.T.);
#28394=EDGE_CURVE('',#23218,#23218,#2764,.T.);
#28395=EDGE_CURVE('',#23219,#23220,#2765,.T.);
#28396=EDGE_CURVE('',#23220,#23221,#5457,.T.);
#28397=EDGE_CURVE('',#23221,#23221,#19486,.T.);
#28398=EDGE_CURVE('',#23220,#23219,#2766,.T.);
#28399=EDGE_CURVE('',#23222,#23222,#2767,.T.);
#28400=EDGE_CURVE('',#23222,#23223,#5458,.T.);
#28401=EDGE_CURVE('',#23223,#23223,#2768,.T.);
#28402=EDGE_CURVE('',#23224,#23225,#2769,.T.);
#28403=EDGE_CURVE('',#23225,#23226,#5459,.T.);
#28404=EDGE_CURVE('',#23226,#23226,#19487,.T.);
#28405=EDGE_CURVE('',#23225,#23224,#2770,.T.);
#28406=EDGE_CURVE('',#23227,#23227,#2771,.T.);
#28407=EDGE_CURVE('',#23227,#23228,#5460,.T.);
#28408=EDGE_CURVE('',#23228,#23228,#2772,.T.);
#28409=EDGE_CURVE('',#23229,#23230,#2773,.T.);
#28410=EDGE_CURVE('',#23230,#23231,#5461,.T.);
#28411=EDGE_CURVE('',#23231,#23231,#19488,.T.);
#28412=EDGE_CURVE('',#23230,#23229,#2774,.T.);
#28413=EDGE_CURVE('',#23232,#23232,#2775,.T.);
#28414=EDGE_CURVE('',#23232,#23233,#5462,.T.);
#28415=EDGE_CURVE('',#23233,#23233,#2776,.T.);
#28416=EDGE_CURVE('',#23234,#23235,#2777,.T.);
#28417=EDGE_CURVE('',#23235,#23236,#5463,.T.);
#28418=EDGE_CURVE('',#23236,#23236,#19489,.T.);
#28419=EDGE_CURVE('',#23235,#23234,#2778,.T.);
#28420=EDGE_CURVE('',#23237,#23237,#2779,.T.);
#28421=EDGE_CURVE('',#23237,#23238,#5464,.T.);
#28422=EDGE_CURVE('',#23238,#23238,#2780,.T.);
#28423=EDGE_CURVE('',#23239,#23240,#2781,.T.);
#28424=EDGE_CURVE('',#23240,#23241,#5465,.T.);
#28425=EDGE_CURVE('',#23241,#23241,#19490,.T.);
#28426=EDGE_CURVE('',#23240,#23239,#2782,.T.);
#28427=EDGE_CURVE('',#23242,#23242,#2783,.T.);
#28428=EDGE_CURVE('',#23242,#23243,#5466,.T.);
#28429=EDGE_CURVE('',#23243,#23243,#2784,.T.);
#28430=EDGE_CURVE('',#23244,#23245,#2785,.T.);
#28431=EDGE_CURVE('',#23245,#23246,#5467,.T.);
#28432=EDGE_CURVE('',#23246,#23246,#19491,.T.);
#28433=EDGE_CURVE('',#23245,#23244,#2786,.T.);
#28434=EDGE_CURVE('',#23247,#23247,#2787,.T.);
#28435=EDGE_CURVE('',#23247,#23248,#5468,.T.);
#28436=EDGE_CURVE('',#23248,#23248,#2788,.T.);
#28437=EDGE_CURVE('',#23249,#23250,#2789,.T.);
#28438=EDGE_CURVE('',#23250,#23251,#5469,.T.);
#28439=EDGE_CURVE('',#23251,#23251,#19492,.T.);
#28440=EDGE_CURVE('',#23250,#23249,#2790,.T.);
#28441=EDGE_CURVE('',#23252,#23252,#2791,.T.);
#28442=EDGE_CURVE('',#23252,#23253,#5470,.T.);
#28443=EDGE_CURVE('',#23253,#23253,#2792,.T.);
#28444=EDGE_CURVE('',#23254,#23255,#2793,.T.);
#28445=EDGE_CURVE('',#23255,#23256,#5471,.T.);
#28446=EDGE_CURVE('',#23256,#23256,#19493,.T.);
#28447=EDGE_CURVE('',#23255,#23254,#2794,.T.);
#28448=EDGE_CURVE('',#23257,#23257,#2795,.T.);
#28449=EDGE_CURVE('',#23257,#23258,#5472,.T.);
#28450=EDGE_CURVE('',#23258,#23258,#2796,.T.);
#28451=EDGE_CURVE('',#23259,#23260,#2797,.T.);
#28452=EDGE_CURVE('',#23260,#23261,#5473,.T.);
#28453=EDGE_CURVE('',#23261,#23261,#19494,.T.);
#28454=EDGE_CURVE('',#23260,#23259,#2798,.T.);
#28455=EDGE_CURVE('',#23262,#23262,#2799,.T.);
#28456=EDGE_CURVE('',#23262,#23263,#5474,.T.);
#28457=EDGE_CURVE('',#23263,#23263,#2800,.T.);
#28458=EDGE_CURVE('',#23264,#23265,#2801,.T.);
#28459=EDGE_CURVE('',#23265,#23266,#5475,.T.);
#28460=EDGE_CURVE('',#23266,#23266,#19495,.T.);
#28461=EDGE_CURVE('',#23265,#23264,#2802,.T.);
#28462=EDGE_CURVE('',#23267,#23267,#2803,.T.);
#28463=EDGE_CURVE('',#23267,#23268,#5476,.T.);
#28464=EDGE_CURVE('',#23268,#23268,#2804,.T.);
#28465=EDGE_CURVE('',#23269,#23270,#2805,.T.);
#28466=EDGE_CURVE('',#23270,#23271,#5477,.T.);
#28467=EDGE_CURVE('',#23271,#23271,#19496,.T.);
#28468=EDGE_CURVE('',#23270,#23269,#2806,.T.);
#28469=EDGE_CURVE('',#23272,#23272,#2807,.T.);
#28470=EDGE_CURVE('',#23272,#23273,#5478,.T.);
#28471=EDGE_CURVE('',#23273,#23273,#2808,.T.);
#28472=EDGE_CURVE('',#23274,#23275,#2809,.T.);
#28473=EDGE_CURVE('',#23275,#23276,#5479,.T.);
#28474=EDGE_CURVE('',#23276,#23276,#19497,.T.);
#28475=EDGE_CURVE('',#23275,#23274,#2810,.T.);
#28476=EDGE_CURVE('',#23277,#23277,#2811,.T.);
#28477=EDGE_CURVE('',#23277,#23278,#5480,.T.);
#28478=EDGE_CURVE('',#23278,#23278,#2812,.T.);
#28479=EDGE_CURVE('',#23279,#23280,#2813,.T.);
#28480=EDGE_CURVE('',#23280,#23281,#5481,.T.);
#28481=EDGE_CURVE('',#23281,#23281,#19498,.T.);
#28482=EDGE_CURVE('',#23280,#23279,#2814,.T.);
#28483=EDGE_CURVE('',#23282,#23282,#2815,.T.);
#28484=EDGE_CURVE('',#23282,#23283,#5482,.T.);
#28485=EDGE_CURVE('',#23283,#23283,#2816,.T.);
#28486=EDGE_CURVE('',#23284,#23285,#2817,.T.);
#28487=EDGE_CURVE('',#23285,#23286,#5483,.T.);
#28488=EDGE_CURVE('',#23286,#23286,#19499,.T.);
#28489=EDGE_CURVE('',#23285,#23284,#2818,.T.);
#28490=EDGE_CURVE('',#22841,#23287,#5484,.T.);
#28491=EDGE_CURVE('',#23287,#23287,#2819,.T.);
#28492=EDGE_CURVE('',#23288,#23289,#2820,.T.);
#28493=EDGE_CURVE('',#23289,#23290,#5485,.T.);
#28494=EDGE_CURVE('',#23290,#23290,#19500,.T.);
#28495=EDGE_CURVE('',#23289,#23288,#2821,.T.);
#28496=EDGE_CURVE('',#22817,#23291,#5486,.T.);
#28497=EDGE_CURVE('',#23291,#23291,#2822,.T.);
#28498=EDGE_CURVE('',#23292,#23293,#2823,.T.);
#28499=EDGE_CURVE('',#23293,#23294,#5487,.T.);
#28500=EDGE_CURVE('',#23294,#23294,#19501,.T.);
#28501=EDGE_CURVE('',#23293,#23292,#2824,.T.);
#28502=EDGE_CURVE('',#23295,#23295,#2825,.T.);
#28503=EDGE_CURVE('',#23295,#23296,#5488,.T.);
#28504=EDGE_CURVE('',#23296,#23296,#2826,.T.);
#28505=EDGE_CURVE('',#23297,#23298,#2827,.T.);
#28506=EDGE_CURVE('',#23298,#23299,#5489,.T.);
#28507=EDGE_CURVE('',#23299,#23299,#19502,.T.);
#28508=EDGE_CURVE('',#23298,#23297,#2828,.T.);
#28509=EDGE_CURVE('',#23300,#23300,#2829,.T.);
#28510=EDGE_CURVE('',#23300,#23301,#5490,.T.);
#28511=EDGE_CURVE('',#23301,#23301,#2830,.T.);
#28512=EDGE_CURVE('',#23302,#23303,#2831,.T.);
#28513=EDGE_CURVE('',#23303,#23304,#5491,.T.);
#28514=EDGE_CURVE('',#23304,#23304,#19503,.T.);
#28515=EDGE_CURVE('',#23303,#23302,#2832,.T.);
#28516=EDGE_CURVE('',#22857,#23305,#5492,.T.);
#28517=EDGE_CURVE('',#23305,#23305,#2833,.T.);
#28518=EDGE_CURVE('',#23306,#23307,#2834,.T.);
#28519=EDGE_CURVE('',#23307,#23308,#5493,.T.);
#28520=EDGE_CURVE('',#23308,#23308,#19504,.T.);
#28521=EDGE_CURVE('',#23307,#23306,#2835,.T.);
#28522=EDGE_CURVE('',#22843,#23309,#5494,.T.);
#28523=EDGE_CURVE('',#23309,#23309,#2836,.T.);
#28524=EDGE_CURVE('',#23310,#23311,#2837,.T.);
#28525=EDGE_CURVE('',#23311,#23312,#5495,.T.);
#28526=EDGE_CURVE('',#23312,#23312,#19505,.T.);
#28527=EDGE_CURVE('',#23311,#23310,#2838,.T.);
#28528=EDGE_CURVE('',#22815,#23313,#5496,.T.);
#28529=EDGE_CURVE('',#23313,#23313,#2839,.T.);
#28530=EDGE_CURVE('',#23314,#23315,#2840,.T.);
#28531=EDGE_CURVE('',#23315,#23316,#5497,.T.);
#28532=EDGE_CURVE('',#23316,#23316,#19506,.T.);
#28533=EDGE_CURVE('',#23315,#23314,#2841,.T.);
#28534=EDGE_CURVE('',#22811,#23317,#5498,.T.);
#28535=EDGE_CURVE('',#23317,#23317,#2842,.T.);
#28536=EDGE_CURVE('',#23318,#23319,#2843,.T.);
#28537=EDGE_CURVE('',#23319,#23320,#5499,.T.);
#28538=EDGE_CURVE('',#23320,#23320,#19507,.T.);
#28539=EDGE_CURVE('',#23319,#23318,#2844,.T.);
#28540=EDGE_CURVE('',#22855,#23321,#5500,.T.);
#28541=EDGE_CURVE('',#23321,#23321,#2845,.T.);
#28542=EDGE_CURVE('',#23322,#23323,#2846,.T.);
#28543=EDGE_CURVE('',#23323,#23324,#5501,.T.);
#28544=EDGE_CURVE('',#23324,#23324,#19508,.T.);
#28545=EDGE_CURVE('',#23323,#23322,#2847,.T.);
#28546=EDGE_CURVE('',#22839,#23325,#5502,.T.);
#28547=EDGE_CURVE('',#23325,#23325,#2848,.T.);
#28548=EDGE_CURVE('',#23326,#23327,#2849,.T.);
#28549=EDGE_CURVE('',#23327,#23328,#5503,.T.);
#28550=EDGE_CURVE('',#23328,#23328,#19509,.T.);
#28551=EDGE_CURVE('',#23327,#23326,#2850,.T.);
#28552=EDGE_CURVE('',#22845,#23329,#5504,.T.);
#28553=EDGE_CURVE('',#23329,#23329,#2851,.T.);
#28554=EDGE_CURVE('',#23330,#23331,#2852,.T.);
#28555=EDGE_CURVE('',#23331,#23332,#5505,.T.);
#28556=EDGE_CURVE('',#23332,#23332,#19510,.T.);
#28557=EDGE_CURVE('',#23331,#23330,#2853,.T.);
#28558=EDGE_CURVE('',#22813,#23333,#5506,.T.);
#28559=EDGE_CURVE('',#23333,#23333,#2854,.T.);
#28560=EDGE_CURVE('',#23334,#23335,#2855,.T.);
#28561=EDGE_CURVE('',#23335,#23336,#5507,.T.);
#28562=EDGE_CURVE('',#23336,#23336,#19511,.T.);
#28563=EDGE_CURVE('',#23335,#23334,#2856,.T.);
#28564=EDGE_CURVE('',#22819,#23337,#5508,.T.);
#28565=EDGE_CURVE('',#23337,#23337,#2857,.T.);
#28566=EDGE_CURVE('',#23338,#23339,#2858,.T.);
#28567=EDGE_CURVE('',#23339,#23340,#5509,.T.);
#28568=EDGE_CURVE('',#23340,#23340,#19512,.T.);
#28569=EDGE_CURVE('',#23339,#23338,#2859,.T.);
#28570=EDGE_CURVE('',#22853,#23341,#5510,.T.);
#28571=EDGE_CURVE('',#23341,#23341,#2860,.T.);
#28572=EDGE_CURVE('',#23342,#23343,#2861,.T.);
#28573=EDGE_CURVE('',#23343,#23344,#5511,.T.);
#28574=EDGE_CURVE('',#23344,#23344,#19513,.T.);
#28575=EDGE_CURVE('',#23343,#23342,#2862,.T.);
#28576=EDGE_CURVE('',#22837,#23345,#5512,.T.);
#28577=EDGE_CURVE('',#23345,#23345,#2863,.T.);
#28578=EDGE_CURVE('',#23346,#23347,#2864,.T.);
#28579=EDGE_CURVE('',#23347,#23348,#5513,.T.);
#28580=EDGE_CURVE('',#23348,#23348,#19514,.T.);
#28581=EDGE_CURVE('',#23347,#23346,#2865,.T.);
#28582=EDGE_CURVE('',#22847,#23349,#5514,.T.);
#28583=EDGE_CURVE('',#23349,#23349,#2866,.T.);
#28584=EDGE_CURVE('',#23350,#23351,#2867,.T.);
#28585=EDGE_CURVE('',#23351,#23352,#5515,.T.);
#28586=EDGE_CURVE('',#23352,#23352,#19515,.T.);
#28587=EDGE_CURVE('',#23351,#23350,#2868,.T.);
#28588=EDGE_CURVE('',#22827,#23353,#5516,.T.);
#28589=EDGE_CURVE('',#23353,#23353,#2869,.T.);
#28590=EDGE_CURVE('',#23354,#23355,#2870,.T.);
#28591=EDGE_CURVE('',#23355,#23356,#5517,.T.);
#28592=EDGE_CURVE('',#23356,#23356,#19516,.T.);
#28593=EDGE_CURVE('',#23355,#23354,#2871,.T.);
#28594=EDGE_CURVE('',#22821,#23357,#5518,.T.);
#28595=EDGE_CURVE('',#23357,#23357,#2872,.T.);
#28596=EDGE_CURVE('',#23358,#23359,#2873,.T.);
#28597=EDGE_CURVE('',#23359,#23360,#5519,.T.);
#28598=EDGE_CURVE('',#23360,#23360,#19517,.T.);
#28599=EDGE_CURVE('',#23359,#23358,#2874,.T.);
#28600=EDGE_CURVE('',#22851,#23361,#5520,.T.);
#28601=EDGE_CURVE('',#23361,#23361,#2875,.T.);
#28602=EDGE_CURVE('',#23362,#23363,#2876,.T.);
#28603=EDGE_CURVE('',#23363,#23364,#5521,.T.);
#28604=EDGE_CURVE('',#23364,#23364,#19518,.T.);
#28605=EDGE_CURVE('',#23363,#23362,#2877,.T.);
#28606=EDGE_CURVE('',#22835,#23365,#5522,.T.);
#28607=EDGE_CURVE('',#23365,#23365,#2878,.T.);
#28608=EDGE_CURVE('',#23366,#23367,#2879,.T.);
#28609=EDGE_CURVE('',#23367,#23368,#5523,.T.);
#28610=EDGE_CURVE('',#23368,#23368,#19519,.T.);
#28611=EDGE_CURVE('',#23367,#23366,#2880,.T.);
#28612=EDGE_CURVE('',#22803,#23369,#5524,.T.);
#28613=EDGE_CURVE('',#23369,#23369,#2881,.T.);
#28614=EDGE_CURVE('',#23370,#23371,#2882,.T.);
#28615=EDGE_CURVE('',#23371,#23372,#5525,.T.);
#28616=EDGE_CURVE('',#23372,#23372,#19520,.T.);
#28617=EDGE_CURVE('',#23371,#23370,#2883,.T.);
#28618=EDGE_CURVE('',#22829,#23373,#5526,.T.);
#28619=EDGE_CURVE('',#23373,#23373,#2884,.T.);
#28620=EDGE_CURVE('',#23374,#23375,#2885,.T.);
#28621=EDGE_CURVE('',#23375,#23376,#5527,.T.);
#28622=EDGE_CURVE('',#23376,#23376,#19521,.T.);
#28623=EDGE_CURVE('',#23375,#23374,#2886,.T.);
#28624=EDGE_CURVE('',#22823,#23377,#5528,.T.);
#28625=EDGE_CURVE('',#23377,#23377,#2887,.T.);
#28626=EDGE_CURVE('',#23378,#23379,#2888,.T.);
#28627=EDGE_CURVE('',#23379,#23380,#5529,.T.);
#28628=EDGE_CURVE('',#23380,#23380,#19522,.T.);
#28629=EDGE_CURVE('',#23379,#23378,#2889,.T.);
#28630=EDGE_CURVE('',#22849,#23381,#5530,.T.);
#28631=EDGE_CURVE('',#23381,#23381,#2890,.T.);
#28632=EDGE_CURVE('',#23382,#23383,#2891,.T.);
#28633=EDGE_CURVE('',#23383,#23384,#5531,.T.);
#28634=EDGE_CURVE('',#23384,#23384,#19523,.T.);
#28635=EDGE_CURVE('',#23383,#23382,#2892,.T.);
#28636=EDGE_CURVE('',#22763,#23385,#5532,.T.);
#28637=EDGE_CURVE('',#23385,#23385,#2893,.T.);
#28638=EDGE_CURVE('',#23386,#23387,#2894,.T.);
#28639=EDGE_CURVE('',#23387,#23388,#5533,.T.);
#28640=EDGE_CURVE('',#23388,#23388,#19524,.T.);
#28641=EDGE_CURVE('',#23387,#23386,#2895,.T.);
#28642=EDGE_CURVE('',#22805,#23389,#5534,.T.);
#28643=EDGE_CURVE('',#23389,#23389,#2896,.T.);
#28644=EDGE_CURVE('',#23390,#23391,#2897,.T.);
#28645=EDGE_CURVE('',#23391,#23392,#5535,.T.);
#28646=EDGE_CURVE('',#23392,#23392,#19525,.T.);
#28647=EDGE_CURVE('',#23391,#23390,#2898,.T.);
#28648=EDGE_CURVE('',#22825,#23393,#5536,.T.);
#28649=EDGE_CURVE('',#23393,#23393,#2899,.T.);
#28650=EDGE_CURVE('',#23394,#23395,#2900,.T.);
#28651=EDGE_CURVE('',#23395,#23396,#5537,.T.);
#28652=EDGE_CURVE('',#23396,#23396,#19526,.T.);
#28653=EDGE_CURVE('',#23395,#23394,#2901,.T.);
#28654=EDGE_CURVE('',#22831,#23397,#5538,.T.);
#28655=EDGE_CURVE('',#23397,#23397,#2902,.T.);
#28656=EDGE_CURVE('',#23398,#23399,#2903,.T.);
#28657=EDGE_CURVE('',#23399,#23400,#5539,.T.);
#28658=EDGE_CURVE('',#23400,#23400,#19527,.T.);
#28659=EDGE_CURVE('',#23399,#23398,#2904,.T.);
#28660=EDGE_CURVE('',#23401,#23401,#19528,.T.);
#28661=EDGE_CURVE('',#23401,#23402,#5540,.T.);
#28662=EDGE_CURVE('',#23402,#23402,#19529,.T.);
#28663=EDGE_CURVE('',#23403,#23403,#19530,.T.);
#28664=EDGE_CURVE('',#23403,#23404,#5541,.T.);
#28665=EDGE_CURVE('',#23404,#23404,#19531,.T.);
#28666=EDGE_CURVE('',#23405,#23405,#19532,.T.);
#28667=EDGE_CURVE('',#23405,#23406,#5542,.T.);
#28668=EDGE_CURVE('',#23406,#23406,#19533,.T.);
#28669=EDGE_CURVE('',#23407,#23407,#19534,.T.);
#28670=EDGE_CURVE('',#23407,#23408,#5543,.T.);
#28671=EDGE_CURVE('',#23408,#23408,#19535,.T.);
#28672=EDGE_CURVE('',#23409,#23409,#19536,.T.);
#28673=EDGE_CURVE('',#23409,#23410,#5544,.T.);
#28674=EDGE_CURVE('',#23410,#23410,#19537,.T.);
#28675=EDGE_CURVE('',#23411,#23411,#19538,.T.);
#28676=EDGE_CURVE('',#23411,#23412,#5545,.T.);
#28677=EDGE_CURVE('',#23412,#23412,#19539,.T.);
#28678=EDGE_CURVE('',#23413,#23413,#19540,.T.);
#28679=EDGE_CURVE('',#23413,#23414,#5546,.T.);
#28680=EDGE_CURVE('',#23414,#23414,#19541,.T.);
#28681=EDGE_CURVE('',#23415,#23415,#19542,.T.);
#28682=EDGE_CURVE('',#23415,#23416,#5547,.T.);
#28683=EDGE_CURVE('',#23416,#23416,#19543,.T.);
#28684=EDGE_CURVE('',#23417,#23417,#19544,.T.);
#28685=EDGE_CURVE('',#23417,#23418,#5548,.T.);
#28686=EDGE_CURVE('',#23418,#23418,#19545,.T.);
#28687=EDGE_CURVE('',#23419,#23419,#19546,.T.);
#28688=EDGE_CURVE('',#23419,#23420,#5549,.T.);
#28689=EDGE_CURVE('',#23420,#23420,#19547,.T.);
#28690=EDGE_CURVE('',#23421,#23421,#19548,.T.);
#28691=EDGE_CURVE('',#23421,#23422,#5550,.T.);
#28692=EDGE_CURVE('',#23422,#23422,#19549,.T.);
#28693=EDGE_CURVE('',#23423,#23423,#19550,.T.);
#28694=EDGE_CURVE('',#23423,#23424,#5551,.T.);
#28695=EDGE_CURVE('',#23424,#23424,#19551,.T.);
#28696=EDGE_CURVE('',#23425,#23425,#19552,.T.);
#28697=EDGE_CURVE('',#23425,#23426,#5552,.T.);
#28698=EDGE_CURVE('',#23426,#23426,#19553,.T.);
#28699=EDGE_CURVE('',#23427,#23427,#19554,.T.);
#28700=EDGE_CURVE('',#23427,#23428,#5553,.T.);
#28701=EDGE_CURVE('',#23428,#23428,#19555,.T.);
#28702=EDGE_CURVE('',#23429,#23429,#19556,.T.);
#28703=EDGE_CURVE('',#23429,#23430,#5554,.T.);
#28704=EDGE_CURVE('',#23430,#23430,#19557,.T.);
#28705=EDGE_CURVE('',#23431,#23431,#19558,.T.);
#28706=EDGE_CURVE('',#23431,#23432,#5555,.T.);
#28707=EDGE_CURVE('',#23432,#23432,#19559,.T.);
#28708=EDGE_CURVE('',#23433,#23433,#19560,.T.);
#28709=EDGE_CURVE('',#23433,#23434,#5556,.T.);
#28710=EDGE_CURVE('',#23434,#23434,#19561,.T.);
#28711=EDGE_CURVE('',#23435,#23435,#19562,.T.);
#28712=EDGE_CURVE('',#23435,#23436,#5557,.T.);
#28713=EDGE_CURVE('',#23436,#23436,#19563,.T.);
#28714=EDGE_CURVE('',#23437,#23437,#19564,.T.);
#28715=EDGE_CURVE('',#23437,#23438,#5558,.T.);
#28716=EDGE_CURVE('',#23438,#23438,#19565,.T.);
#28717=EDGE_CURVE('',#23439,#23439,#19566,.T.);
#28718=EDGE_CURVE('',#23439,#23440,#5559,.T.);
#28719=EDGE_CURVE('',#23440,#23440,#19567,.T.);
#28720=EDGE_CURVE('',#23441,#23441,#19568,.T.);
#28721=EDGE_CURVE('',#23441,#23442,#5560,.T.);
#28722=EDGE_CURVE('',#23442,#23442,#19569,.T.);
#28723=EDGE_CURVE('',#23443,#23443,#19570,.T.);
#28724=EDGE_CURVE('',#23443,#23444,#5561,.T.);
#28725=EDGE_CURVE('',#23444,#23444,#19571,.T.);
#28726=EDGE_CURVE('',#23445,#23445,#19572,.T.);
#28727=EDGE_CURVE('',#23445,#23446,#5562,.T.);
#28728=EDGE_CURVE('',#23446,#23446,#19573,.T.);
#28729=EDGE_CURVE('',#23447,#23447,#19574,.T.);
#28730=EDGE_CURVE('',#23447,#23448,#5563,.T.);
#28731=EDGE_CURVE('',#23448,#23448,#19575,.T.);
#28732=EDGE_CURVE('',#23449,#23449,#19576,.T.);
#28733=EDGE_CURVE('',#23449,#23450,#5564,.T.);
#28734=EDGE_CURVE('',#23450,#23450,#19577,.T.);
#28735=EDGE_CURVE('',#23451,#23451,#19578,.T.);
#28736=EDGE_CURVE('',#23451,#23452,#5565,.T.);
#28737=EDGE_CURVE('',#23452,#23452,#19579,.T.);
#28738=EDGE_CURVE('',#23453,#23453,#19580,.T.);
#28739=EDGE_CURVE('',#23453,#23454,#5566,.T.);
#28740=EDGE_CURVE('',#23454,#23454,#19581,.T.);
#28741=EDGE_CURVE('',#23455,#23455,#19582,.T.);
#28742=EDGE_CURVE('',#23455,#23456,#5567,.T.);
#28743=EDGE_CURVE('',#23456,#23456,#19583,.T.);
#28744=EDGE_CURVE('',#23457,#23457,#19584,.T.);
#28745=EDGE_CURVE('',#23457,#23458,#5568,.T.);
#28746=EDGE_CURVE('',#23458,#23458,#19585,.T.);
#28747=EDGE_CURVE('',#23459,#23459,#19586,.T.);
#28748=EDGE_CURVE('',#23459,#23460,#5569,.T.);
#28749=EDGE_CURVE('',#23460,#23460,#19587,.T.);
#28750=EDGE_CURVE('',#23461,#23461,#19588,.T.);
#28751=EDGE_CURVE('',#23461,#23462,#5570,.T.);
#28752=EDGE_CURVE('',#23462,#23462,#19589,.T.);
#28753=EDGE_CURVE('',#23463,#23463,#19590,.T.);
#28754=EDGE_CURVE('',#23463,#23464,#5571,.T.);
#28755=EDGE_CURVE('',#23464,#23464,#19591,.T.);
#28756=EDGE_CURVE('',#23465,#23465,#19592,.T.);
#28757=EDGE_CURVE('',#23465,#23466,#5572,.T.);
#28758=EDGE_CURVE('',#23466,#23466,#19593,.T.);
#28759=EDGE_CURVE('',#23467,#23467,#19594,.T.);
#28760=EDGE_CURVE('',#23467,#23468,#5573,.T.);
#28761=EDGE_CURVE('',#23468,#23468,#19595,.T.);
#28762=EDGE_CURVE('',#23469,#23469,#19596,.T.);
#28763=EDGE_CURVE('',#23469,#23470,#5574,.T.);
#28764=EDGE_CURVE('',#23470,#23470,#19597,.T.);
#28765=EDGE_CURVE('',#23471,#23471,#19598,.T.);
#28766=EDGE_CURVE('',#23471,#23472,#5575,.T.);
#28767=EDGE_CURVE('',#23472,#23472,#19599,.T.);
#28768=EDGE_CURVE('',#23473,#23473,#19600,.T.);
#28769=EDGE_CURVE('',#23473,#23474,#5576,.T.);
#28770=EDGE_CURVE('',#23474,#23474,#19601,.T.);
#28771=EDGE_CURVE('',#23475,#23475,#19602,.T.);
#28772=EDGE_CURVE('',#23475,#23476,#5577,.T.);
#28773=EDGE_CURVE('',#23476,#23476,#19603,.T.);
#28774=EDGE_CURVE('',#23477,#23477,#19604,.T.);
#28775=EDGE_CURVE('',#23477,#23478,#5578,.T.);
#28776=EDGE_CURVE('',#23478,#23478,#19605,.T.);
#28777=EDGE_CURVE('',#23479,#23479,#19606,.T.);
#28778=EDGE_CURVE('',#23479,#23480,#5579,.T.);
#28779=EDGE_CURVE('',#23480,#23480,#19607,.T.);
#28780=EDGE_CURVE('',#23481,#23481,#19608,.T.);
#28781=EDGE_CURVE('',#23481,#23482,#5580,.T.);
#28782=EDGE_CURVE('',#23482,#23482,#19609,.T.);
#28783=EDGE_CURVE('',#23483,#23483,#19610,.T.);
#28784=EDGE_CURVE('',#23483,#23484,#5581,.T.);
#28785=EDGE_CURVE('',#23484,#23484,#19611,.T.);
#28786=EDGE_CURVE('',#23485,#23485,#19612,.T.);
#28787=EDGE_CURVE('',#23485,#23486,#5582,.T.);
#28788=EDGE_CURVE('',#23486,#23486,#19613,.T.);
#28789=EDGE_CURVE('',#23487,#23487,#19614,.T.);
#28790=EDGE_CURVE('',#23487,#23488,#5583,.T.);
#28791=EDGE_CURVE('',#23488,#23488,#19615,.T.);
#28792=EDGE_CURVE('',#23489,#23489,#19616,.T.);
#28793=EDGE_CURVE('',#23489,#23490,#5584,.T.);
#28794=EDGE_CURVE('',#23490,#23490,#19617,.T.);
#28795=EDGE_CURVE('',#23491,#23491,#19618,.T.);
#28796=EDGE_CURVE('',#23491,#23492,#5585,.T.);
#28797=EDGE_CURVE('',#23492,#23492,#19619,.T.);
#28798=EDGE_CURVE('',#23493,#23493,#19620,.T.);
#28799=EDGE_CURVE('',#23493,#23494,#5586,.T.);
#28800=EDGE_CURVE('',#23494,#23494,#19621,.T.);
#28801=EDGE_CURVE('',#23495,#23495,#19622,.T.);
#28802=EDGE_CURVE('',#23495,#23496,#5587,.T.);
#28803=EDGE_CURVE('',#23496,#23496,#19623,.T.);
#28804=EDGE_CURVE('',#23497,#23497,#19624,.T.);
#28805=EDGE_CURVE('',#23497,#23498,#5588,.T.);
#28806=EDGE_CURVE('',#23498,#23498,#19625,.T.);
#28807=EDGE_CURVE('',#23499,#23499,#19626,.T.);
#28808=EDGE_CURVE('',#23499,#23500,#5589,.T.);
#28809=EDGE_CURVE('',#23500,#23500,#19627,.T.);
#28810=EDGE_CURVE('',#23501,#23501,#19628,.T.);
#28811=EDGE_CURVE('',#23501,#23502,#5590,.T.);
#28812=EDGE_CURVE('',#23502,#23502,#19629,.T.);
#28813=EDGE_CURVE('',#23503,#23503,#19630,.T.);
#28814=EDGE_CURVE('',#23503,#23504,#5591,.T.);
#28815=EDGE_CURVE('',#23504,#23504,#19631,.T.);
#28816=EDGE_CURVE('',#23505,#23505,#19632,.T.);
#28817=EDGE_CURVE('',#23505,#23506,#5592,.T.);
#28818=EDGE_CURVE('',#23506,#23506,#19633,.T.);
#28819=EDGE_CURVE('',#23507,#23507,#19634,.T.);
#28820=EDGE_CURVE('',#23507,#23508,#5593,.T.);
#28821=EDGE_CURVE('',#23508,#23508,#19635,.T.);
#28822=EDGE_CURVE('',#23509,#23509,#19636,.T.);
#28823=EDGE_CURVE('',#23509,#23510,#5594,.T.);
#28824=EDGE_CURVE('',#23510,#23510,#19637,.T.);
#28825=EDGE_CURVE('',#23511,#23511,#19638,.T.);
#28826=EDGE_CURVE('',#23511,#23512,#5595,.T.);
#28827=EDGE_CURVE('',#23512,#23512,#19639,.T.);
#28828=EDGE_CURVE('',#23513,#23513,#19640,.T.);
#28829=EDGE_CURVE('',#23513,#23514,#5596,.T.);
#28830=EDGE_CURVE('',#23514,#23514,#19641,.T.);
#28831=EDGE_CURVE('',#23515,#23515,#19642,.T.);
#28832=EDGE_CURVE('',#23515,#23516,#5597,.T.);
#28833=EDGE_CURVE('',#23516,#23516,#19643,.T.);
#28834=EDGE_CURVE('',#23517,#23517,#19644,.T.);
#28835=EDGE_CURVE('',#23517,#23518,#5598,.T.);
#28836=EDGE_CURVE('',#23518,#23518,#19645,.T.);
#28837=EDGE_CURVE('',#23519,#23519,#19646,.T.);
#28838=EDGE_CURVE('',#23519,#23520,#5599,.T.);
#28839=EDGE_CURVE('',#23520,#23520,#19647,.T.);
#28840=EDGE_CURVE('',#23521,#23521,#19648,.T.);
#28841=EDGE_CURVE('',#23521,#23522,#5600,.T.);
#28842=EDGE_CURVE('',#23522,#23522,#19649,.T.);
#28843=EDGE_CURVE('',#23523,#23523,#19650,.T.);
#28844=EDGE_CURVE('',#23523,#23524,#5601,.T.);
#28845=EDGE_CURVE('',#23524,#23524,#19651,.T.);
#28846=EDGE_CURVE('',#23525,#23525,#19652,.T.);
#28847=EDGE_CURVE('',#23525,#23526,#5602,.T.);
#28848=EDGE_CURVE('',#23526,#23526,#19653,.T.);
#28849=EDGE_CURVE('',#23527,#23527,#19654,.T.);
#28850=EDGE_CURVE('',#23527,#23528,#5603,.T.);
#28851=EDGE_CURVE('',#23528,#23528,#19655,.T.);
#28852=EDGE_CURVE('',#23529,#23529,#19656,.T.);
#28853=EDGE_CURVE('',#23529,#23530,#5604,.T.);
#28854=EDGE_CURVE('',#23530,#23530,#19657,.T.);
#28855=EDGE_CURVE('',#23531,#23531,#19658,.T.);
#28856=EDGE_CURVE('',#23531,#23532,#5605,.T.);
#28857=EDGE_CURVE('',#23532,#23532,#19659,.T.);
#28858=EDGE_CURVE('',#23533,#23533,#19660,.T.);
#28859=EDGE_CURVE('',#23533,#23534,#5606,.T.);
#28860=EDGE_CURVE('',#23534,#23534,#19661,.T.);
#28861=EDGE_CURVE('',#23535,#23535,#19662,.T.);
#28862=EDGE_CURVE('',#23535,#23536,#5607,.T.);
#28863=EDGE_CURVE('',#23536,#23536,#19663,.T.);
#28864=EDGE_CURVE('',#23537,#23537,#19664,.T.);
#28865=EDGE_CURVE('',#23537,#23538,#5608,.T.);
#28866=EDGE_CURVE('',#23538,#23538,#19665,.T.);
#28867=EDGE_CURVE('',#23539,#23539,#19666,.T.);
#28868=EDGE_CURVE('',#23539,#23540,#5609,.T.);
#28869=EDGE_CURVE('',#23540,#23540,#19667,.T.);
#28870=EDGE_CURVE('',#23541,#23541,#19668,.T.);
#28871=EDGE_CURVE('',#23541,#23542,#5610,.T.);
#28872=EDGE_CURVE('',#23542,#23542,#19669,.T.);
#28873=EDGE_CURVE('',#23543,#23543,#19670,.T.);
#28874=EDGE_CURVE('',#23543,#23544,#5611,.T.);
#28875=EDGE_CURVE('',#23544,#23544,#19671,.T.);
#28876=EDGE_CURVE('',#23545,#23545,#19672,.T.);
#28877=EDGE_CURVE('',#23545,#23546,#5612,.T.);
#28878=EDGE_CURVE('',#23546,#23546,#19673,.T.);
#28879=EDGE_CURVE('',#23547,#23547,#19674,.T.);
#28880=EDGE_CURVE('',#23547,#23548,#5613,.T.);
#28881=EDGE_CURVE('',#23548,#23548,#19675,.T.);
#28882=EDGE_CURVE('',#23549,#23549,#19676,.T.);
#28883=EDGE_CURVE('',#23549,#23550,#5614,.T.);
#28884=EDGE_CURVE('',#23550,#23550,#19677,.T.);
#28885=EDGE_CURVE('',#23551,#23551,#19678,.T.);
#28886=EDGE_CURVE('',#23551,#23552,#5615,.T.);
#28887=EDGE_CURVE('',#23552,#23552,#19679,.T.);
#28888=EDGE_CURVE('',#23553,#23553,#19680,.T.);
#28889=EDGE_CURVE('',#23553,#23554,#5616,.T.);
#28890=EDGE_CURVE('',#23554,#23554,#19681,.T.);
#28891=EDGE_CURVE('',#23555,#23555,#19682,.T.);
#28892=EDGE_CURVE('',#23555,#23556,#5617,.T.);
#28893=EDGE_CURVE('',#23556,#23556,#19683,.T.);
#28894=EDGE_CURVE('',#23557,#23557,#19684,.T.);
#28895=EDGE_CURVE('',#23557,#23558,#5618,.T.);
#28896=EDGE_CURVE('',#23558,#23558,#19685,.T.);
#28897=EDGE_CURVE('',#23559,#23559,#19686,.T.);
#28898=EDGE_CURVE('',#23559,#23560,#5619,.T.);
#28899=EDGE_CURVE('',#23560,#23560,#19687,.T.);
#28900=EDGE_CURVE('',#23561,#23561,#19688,.T.);
#28901=EDGE_CURVE('',#23561,#23562,#5620,.T.);
#28902=EDGE_CURVE('',#23562,#23562,#19689,.T.);
#28903=EDGE_CURVE('',#23563,#23563,#19690,.T.);
#28904=EDGE_CURVE('',#23563,#23564,#5621,.T.);
#28905=EDGE_CURVE('',#23564,#23564,#19691,.T.);
#28906=EDGE_CURVE('',#23565,#23565,#19692,.T.);
#28907=EDGE_CURVE('',#23565,#23566,#5622,.T.);
#28908=EDGE_CURVE('',#23566,#23566,#19693,.T.);
#28909=EDGE_CURVE('',#23567,#23567,#19694,.T.);
#28910=EDGE_CURVE('',#23567,#23568,#5623,.T.);
#28911=EDGE_CURVE('',#23568,#23568,#19695,.T.);
#28912=EDGE_CURVE('',#23569,#23569,#19696,.T.);
#28913=EDGE_CURVE('',#23569,#23570,#5624,.T.);
#28914=EDGE_CURVE('',#23570,#23570,#19697,.T.);
#28915=EDGE_CURVE('',#23571,#23571,#19698,.T.);
#28916=EDGE_CURVE('',#23571,#23572,#5625,.T.);
#28917=EDGE_CURVE('',#23572,#23572,#19699,.T.);
#28918=EDGE_CURVE('',#23573,#23573,#19700,.T.);
#28919=EDGE_CURVE('',#23573,#23574,#5626,.T.);
#28920=EDGE_CURVE('',#23574,#23574,#19701,.T.);
#28921=EDGE_CURVE('',#23575,#23575,#19702,.T.);
#28922=EDGE_CURVE('',#23575,#23576,#5627,.T.);
#28923=EDGE_CURVE('',#23576,#23576,#19703,.T.);
#28924=EDGE_CURVE('',#23577,#23577,#19704,.T.);
#28925=EDGE_CURVE('',#23577,#23578,#5628,.T.);
#28926=EDGE_CURVE('',#23578,#23578,#19705,.T.);
#28927=EDGE_CURVE('',#23579,#23579,#19706,.T.);
#28928=EDGE_CURVE('',#23579,#23580,#5629,.T.);
#28929=EDGE_CURVE('',#23580,#23580,#19707,.T.);
#28930=EDGE_CURVE('',#23581,#23581,#19708,.T.);
#28931=EDGE_CURVE('',#23581,#23582,#5630,.T.);
#28932=EDGE_CURVE('',#23582,#23582,#19709,.T.);
#28933=EDGE_CURVE('',#23583,#23583,#19710,.T.);
#28934=EDGE_CURVE('',#23583,#23584,#5631,.T.);
#28935=EDGE_CURVE('',#23584,#23584,#19711,.T.);
#28936=EDGE_CURVE('',#23585,#23585,#19712,.T.);
#28937=EDGE_CURVE('',#23585,#23586,#5632,.T.);
#28938=EDGE_CURVE('',#23586,#23586,#19713,.T.);
#28939=EDGE_CURVE('',#23587,#23587,#19714,.T.);
#28940=EDGE_CURVE('',#23587,#23588,#5633,.T.);
#28941=EDGE_CURVE('',#23588,#23588,#19715,.T.);
#28942=EDGE_CURVE('',#23589,#23589,#19716,.T.);
#28943=EDGE_CURVE('',#23589,#23590,#5634,.T.);
#28944=EDGE_CURVE('',#23590,#23590,#19717,.T.);
#28945=EDGE_CURVE('',#23591,#23591,#19718,.T.);
#28946=EDGE_CURVE('',#23591,#23592,#5635,.T.);
#28947=EDGE_CURVE('',#23592,#23592,#19719,.T.);
#28948=EDGE_CURVE('',#23593,#23593,#19720,.T.);
#28949=EDGE_CURVE('',#23593,#23594,#5636,.T.);
#28950=EDGE_CURVE('',#23594,#23594,#19721,.T.);
#28951=EDGE_CURVE('',#23595,#23595,#19722,.T.);
#28952=EDGE_CURVE('',#23595,#23596,#5637,.T.);
#28953=EDGE_CURVE('',#23596,#23596,#19723,.T.);
#28954=EDGE_CURVE('',#23597,#23597,#19724,.T.);
#28955=EDGE_CURVE('',#23597,#23598,#5638,.T.);
#28956=EDGE_CURVE('',#23598,#23598,#19725,.T.);
#28957=EDGE_CURVE('',#23599,#23599,#19726,.T.);
#28958=EDGE_CURVE('',#23599,#23600,#5639,.T.);
#28959=EDGE_CURVE('',#23600,#23600,#19727,.T.);
#28960=EDGE_CURVE('',#23601,#23601,#19728,.T.);
#28961=EDGE_CURVE('',#23601,#23602,#5640,.T.);
#28962=EDGE_CURVE('',#23602,#23602,#19729,.T.);
#28963=EDGE_CURVE('',#23603,#23603,#19730,.T.);
#28964=EDGE_CURVE('',#23603,#23604,#5641,.T.);
#28965=EDGE_CURVE('',#23604,#23604,#19731,.T.);
#28966=EDGE_CURVE('',#23605,#23605,#19732,.T.);
#28967=EDGE_CURVE('',#23605,#23606,#5642,.T.);
#28968=EDGE_CURVE('',#23606,#23606,#19733,.T.);
#28969=EDGE_CURVE('',#23607,#23607,#19734,.T.);
#28970=EDGE_CURVE('',#23607,#23608,#5643,.T.);
#28971=EDGE_CURVE('',#23608,#23608,#19735,.T.);
#28972=EDGE_CURVE('',#23609,#23609,#19736,.T.);
#28973=EDGE_CURVE('',#23609,#23610,#5644,.T.);
#28974=EDGE_CURVE('',#23610,#23610,#19737,.T.);
#28975=EDGE_CURVE('',#23611,#23611,#19738,.T.);
#28976=EDGE_CURVE('',#23611,#23612,#5645,.T.);
#28977=EDGE_CURVE('',#23612,#23612,#19739,.T.);
#28978=EDGE_CURVE('',#23613,#23613,#19740,.T.);
#28979=EDGE_CURVE('',#23613,#23614,#5646,.T.);
#28980=EDGE_CURVE('',#23614,#23614,#19741,.T.);
#28981=EDGE_CURVE('',#23615,#23615,#19742,.T.);
#28982=EDGE_CURVE('',#23615,#23616,#5647,.T.);
#28983=EDGE_CURVE('',#23616,#23616,#19743,.T.);
#28984=EDGE_CURVE('',#23617,#23617,#19744,.T.);
#28985=EDGE_CURVE('',#23617,#23618,#5648,.T.);
#28986=EDGE_CURVE('',#23618,#23618,#19745,.T.);
#28987=EDGE_CURVE('',#23619,#23619,#19746,.T.);
#28988=EDGE_CURVE('',#23619,#23620,#5649,.T.);
#28989=EDGE_CURVE('',#23620,#23620,#19747,.T.);
#28990=EDGE_CURVE('',#23621,#23621,#19748,.T.);
#28991=EDGE_CURVE('',#23621,#23622,#5650,.T.);
#28992=EDGE_CURVE('',#23622,#23622,#19749,.T.);
#28993=EDGE_CURVE('',#23623,#23623,#19750,.T.);
#28994=EDGE_CURVE('',#23623,#23624,#5651,.T.);
#28995=EDGE_CURVE('',#23624,#23624,#19751,.T.);
#28996=EDGE_CURVE('',#23625,#23625,#19752,.T.);
#28997=EDGE_CURVE('',#23625,#23626,#5652,.T.);
#28998=EDGE_CURVE('',#23626,#23626,#19753,.T.);
#28999=EDGE_CURVE('',#23627,#23627,#19754,.T.);
#29000=EDGE_CURVE('',#23627,#23628,#5653,.T.);
#29001=EDGE_CURVE('',#23628,#23628,#19755,.T.);
#29002=EDGE_CURVE('',#23629,#23629,#19756,.T.);
#29003=EDGE_CURVE('',#23629,#23630,#5654,.T.);
#29004=EDGE_CURVE('',#23630,#23630,#19757,.T.);
#29005=EDGE_CURVE('',#23631,#23631,#19758,.T.);
#29006=EDGE_CURVE('',#23631,#23632,#5655,.T.);
#29007=EDGE_CURVE('',#23632,#23632,#19759,.T.);
#29008=EDGE_CURVE('',#23633,#23633,#19760,.T.);
#29009=EDGE_CURVE('',#23633,#23634,#5656,.T.);
#29010=EDGE_CURVE('',#23634,#23634,#19761,.T.);
#29011=EDGE_CURVE('',#23635,#23635,#19762,.T.);
#29012=EDGE_CURVE('',#23635,#23636,#5657,.T.);
#29013=EDGE_CURVE('',#23636,#23636,#19763,.T.);
#29014=EDGE_CURVE('',#23637,#23637,#19764,.T.);
#29015=EDGE_CURVE('',#23637,#23638,#5658,.T.);
#29016=EDGE_CURVE('',#23638,#23638,#19765,.T.);
#29017=EDGE_CURVE('',#23639,#23639,#19766,.T.);
#29018=EDGE_CURVE('',#23639,#23640,#5659,.T.);
#29019=EDGE_CURVE('',#23640,#23640,#19767,.T.);
#29020=EDGE_CURVE('',#23641,#23641,#19768,.T.);
#29021=EDGE_CURVE('',#23641,#23642,#5660,.T.);
#29022=EDGE_CURVE('',#23642,#23642,#19769,.T.);
#29023=EDGE_CURVE('',#23643,#23643,#19770,.T.);
#29024=EDGE_CURVE('',#23643,#23644,#5661,.T.);
#29025=EDGE_CURVE('',#23644,#23644,#19771,.T.);
#29026=EDGE_CURVE('',#23645,#23645,#19772,.T.);
#29027=EDGE_CURVE('',#23645,#23646,#5662,.T.);
#29028=EDGE_CURVE('',#23646,#23646,#19773,.T.);
#29029=EDGE_CURVE('',#23647,#23647,#19774,.T.);
#29030=EDGE_CURVE('',#23647,#23648,#5663,.T.);
#29031=EDGE_CURVE('',#23648,#23648,#19775,.T.);
#29032=EDGE_CURVE('',#23649,#23649,#19776,.T.);
#29033=EDGE_CURVE('',#23649,#23650,#5664,.T.);
#29034=EDGE_CURVE('',#23650,#23650,#19777,.T.);
#29035=EDGE_CURVE('',#23651,#23651,#19778,.T.);
#29036=EDGE_CURVE('',#23651,#23652,#5665,.T.);
#29037=EDGE_CURVE('',#23652,#23652,#19779,.T.);
#29038=EDGE_CURVE('',#23653,#23653,#19780,.T.);
#29039=EDGE_CURVE('',#23653,#23654,#5666,.T.);
#29040=EDGE_CURVE('',#23654,#23654,#19781,.T.);
#29041=EDGE_CURVE('',#23655,#23655,#19782,.T.);
#29042=EDGE_CURVE('',#23655,#23656,#5667,.T.);
#29043=EDGE_CURVE('',#23656,#23656,#19783,.T.);
#29044=EDGE_CURVE('',#23657,#23657,#19784,.T.);
#29045=EDGE_CURVE('',#23657,#23658,#5668,.T.);
#29046=EDGE_CURVE('',#23658,#23658,#19785,.T.);
#29047=EDGE_CURVE('',#23659,#23659,#19786,.T.);
#29048=EDGE_CURVE('',#23659,#23660,#5669,.T.);
#29049=EDGE_CURVE('',#23660,#23660,#19787,.T.);
#29050=EDGE_CURVE('',#23661,#23661,#19788,.T.);
#29051=EDGE_CURVE('',#23661,#23662,#5670,.T.);
#29052=EDGE_CURVE('',#23662,#23662,#19789,.T.);
#29053=EDGE_CURVE('',#23663,#23663,#19790,.T.);
#29054=EDGE_CURVE('',#23663,#23664,#5671,.T.);
#29055=EDGE_CURVE('',#23664,#23664,#19791,.T.);
#29056=EDGE_CURVE('',#23665,#23665,#19792,.T.);
#29057=EDGE_CURVE('',#23665,#23666,#5672,.T.);
#29058=EDGE_CURVE('',#23666,#23666,#19793,.T.);
#29059=EDGE_CURVE('',#23667,#23667,#19794,.T.);
#29060=EDGE_CURVE('',#23667,#23668,#5673,.T.);
#29061=EDGE_CURVE('',#23668,#23668,#19795,.T.);
#29062=EDGE_CURVE('',#23669,#23669,#19796,.T.);
#29063=EDGE_CURVE('',#23669,#23670,#5674,.T.);
#29064=EDGE_CURVE('',#23670,#23670,#19797,.T.);
#29065=EDGE_CURVE('',#23671,#23671,#19798,.T.);
#29066=EDGE_CURVE('',#23671,#23672,#5675,.T.);
#29067=EDGE_CURVE('',#23672,#23672,#19799,.T.);
#29068=EDGE_CURVE('',#23673,#23673,#19800,.T.);
#29069=EDGE_CURVE('',#23673,#23674,#5676,.T.);
#29070=EDGE_CURVE('',#23674,#23674,#19801,.T.);
#29071=EDGE_CURVE('',#23675,#23675,#19802,.T.);
#29072=EDGE_CURVE('',#23675,#23676,#5677,.T.);
#29073=EDGE_CURVE('',#23676,#23676,#19803,.T.);
#29074=EDGE_CURVE('',#23677,#23677,#19804,.T.);
#29075=EDGE_CURVE('',#23677,#23678,#5678,.T.);
#29076=EDGE_CURVE('',#23678,#23678,#19805,.T.);
#29077=EDGE_CURVE('',#23679,#23679,#19806,.T.);
#29078=EDGE_CURVE('',#23679,#23680,#5679,.T.);
#29079=EDGE_CURVE('',#23680,#23680,#19807,.T.);
#29080=EDGE_CURVE('',#23681,#23681,#19808,.T.);
#29081=EDGE_CURVE('',#23681,#23682,#5680,.T.);
#29082=EDGE_CURVE('',#23682,#23682,#19809,.T.);
#29083=EDGE_CURVE('',#23683,#23683,#19810,.T.);
#29084=EDGE_CURVE('',#23683,#23684,#5681,.T.);
#29085=EDGE_CURVE('',#23684,#23684,#19811,.T.);
#29086=EDGE_CURVE('',#23685,#23685,#19812,.T.);
#29087=EDGE_CURVE('',#23685,#23686,#5682,.T.);
#29088=EDGE_CURVE('',#23686,#23686,#19813,.T.);
#29089=EDGE_CURVE('',#23687,#23687,#19814,.T.);
#29090=EDGE_CURVE('',#23687,#23688,#5683,.T.);
#29091=EDGE_CURVE('',#23688,#23688,#19815,.T.);
#29092=EDGE_CURVE('',#23689,#23689,#19816,.T.);
#29093=EDGE_CURVE('',#23689,#23690,#5684,.T.);
#29094=EDGE_CURVE('',#23690,#23690,#19817,.T.);
#29095=EDGE_CURVE('',#23691,#23691,#19818,.T.);
#29096=EDGE_CURVE('',#23691,#23692,#5685,.T.);
#29097=EDGE_CURVE('',#23692,#23692,#19819,.T.);
#29098=EDGE_CURVE('',#23693,#23693,#19820,.T.);
#29099=EDGE_CURVE('',#23693,#23694,#5686,.T.);
#29100=EDGE_CURVE('',#23694,#23694,#19821,.T.);
#29101=EDGE_CURVE('',#23695,#23695,#19822,.T.);
#29102=EDGE_CURVE('',#23695,#23696,#5687,.T.);
#29103=EDGE_CURVE('',#23696,#23696,#19823,.T.);
#29104=EDGE_CURVE('',#23697,#23697,#19824,.T.);
#29105=EDGE_CURVE('',#23697,#23698,#5688,.T.);
#29106=EDGE_CURVE('',#23698,#23698,#19825,.T.);
#29107=EDGE_CURVE('',#23699,#23699,#19826,.T.);
#29108=EDGE_CURVE('',#23699,#23700,#5689,.T.);
#29109=EDGE_CURVE('',#23700,#23700,#19827,.T.);
#29110=EDGE_CURVE('',#23701,#23701,#19828,.T.);
#29111=EDGE_CURVE('',#23701,#23702,#5690,.T.);
#29112=EDGE_CURVE('',#23702,#23702,#19829,.T.);
#29113=EDGE_CURVE('',#23703,#23703,#19830,.T.);
#29114=EDGE_CURVE('',#23703,#23704,#5691,.T.);
#29115=EDGE_CURVE('',#23704,#23704,#19831,.T.);
#29116=EDGE_CURVE('',#23705,#23705,#19832,.T.);
#29117=EDGE_CURVE('',#23705,#23706,#5692,.T.);
#29118=EDGE_CURVE('',#23706,#23706,#19833,.T.);
#29119=EDGE_CURVE('',#23707,#23707,#19834,.T.);
#29120=EDGE_CURVE('',#23707,#23708,#5693,.T.);
#29121=EDGE_CURVE('',#23708,#23708,#19835,.T.);
#29122=EDGE_CURVE('',#23709,#23709,#19836,.T.);
#29123=EDGE_CURVE('',#23709,#23710,#5694,.T.);
#29124=EDGE_CURVE('',#23710,#23710,#19837,.T.);
#29125=EDGE_CURVE('',#23711,#23711,#19838,.T.);
#29126=EDGE_CURVE('',#23711,#23712,#5695,.T.);
#29127=EDGE_CURVE('',#23712,#23712,#19839,.T.);
#29128=EDGE_CURVE('',#23713,#23713,#19840,.T.);
#29129=EDGE_CURVE('',#23713,#23714,#5696,.T.);
#29130=EDGE_CURVE('',#23714,#23714,#19841,.T.);
#29131=EDGE_CURVE('',#23715,#23715,#19842,.T.);
#29132=EDGE_CURVE('',#23715,#23716,#5697,.T.);
#29133=EDGE_CURVE('',#23716,#23716,#19843,.T.);
#29134=EDGE_CURVE('',#23717,#23717,#19844,.T.);
#29135=EDGE_CURVE('',#23717,#23718,#5698,.T.);
#29136=EDGE_CURVE('',#23718,#23718,#19845,.T.);
#29137=EDGE_CURVE('',#23719,#23719,#19846,.T.);
#29138=EDGE_CURVE('',#23719,#23720,#5699,.T.);
#29139=EDGE_CURVE('',#23720,#23720,#19847,.T.);
#29140=EDGE_CURVE('',#23721,#23721,#19848,.T.);
#29141=EDGE_CURVE('',#23721,#23722,#5700,.T.);
#29142=EDGE_CURVE('',#23722,#23722,#19849,.T.);
#29143=EDGE_CURVE('',#23723,#23723,#19850,.T.);
#29144=EDGE_CURVE('',#23723,#23724,#5701,.T.);
#29145=EDGE_CURVE('',#23724,#23724,#19851,.T.);
#29146=EDGE_CURVE('',#23725,#23725,#19852,.T.);
#29147=EDGE_CURVE('',#23725,#23726,#5702,.T.);
#29148=EDGE_CURVE('',#23726,#23726,#19853,.T.);
#29149=EDGE_CURVE('',#23727,#23727,#19854,.T.);
#29150=EDGE_CURVE('',#23727,#23728,#5703,.T.);
#29151=EDGE_CURVE('',#23728,#23728,#19855,.T.);
#29152=EDGE_CURVE('',#23729,#23729,#19856,.T.);
#29153=EDGE_CURVE('',#23729,#23730,#5704,.T.);
#29154=EDGE_CURVE('',#23730,#23730,#19857,.T.);
#29155=EDGE_CURVE('',#23731,#23731,#19858,.T.);
#29156=EDGE_CURVE('',#23731,#23732,#5705,.T.);
#29157=EDGE_CURVE('',#23732,#23732,#19859,.T.);
#29158=EDGE_CURVE('',#23733,#23733,#19860,.T.);
#29159=EDGE_CURVE('',#23733,#23734,#5706,.T.);
#29160=EDGE_CURVE('',#23734,#23734,#19861,.T.);
#29161=EDGE_CURVE('',#23735,#23735,#19862,.T.);
#29162=EDGE_CURVE('',#23735,#23736,#5707,.T.);
#29163=EDGE_CURVE('',#23736,#23736,#19863,.T.);
#29164=EDGE_CURVE('',#23737,#23737,#19864,.T.);
#29165=EDGE_CURVE('',#23737,#23738,#5708,.T.);
#29166=EDGE_CURVE('',#23738,#23738,#19865,.T.);
#29167=EDGE_CURVE('',#23739,#23739,#19866,.T.);
#29168=EDGE_CURVE('',#23739,#23740,#5709,.T.);
#29169=EDGE_CURVE('',#23740,#23740,#19867,.T.);
#29170=EDGE_CURVE('',#23741,#23741,#19868,.T.);
#29171=EDGE_CURVE('',#23741,#23742,#5710,.T.);
#29172=EDGE_CURVE('',#23742,#23742,#19869,.T.);
#29173=EDGE_CURVE('',#23743,#23743,#19870,.T.);
#29174=EDGE_CURVE('',#23743,#23744,#5711,.T.);
#29175=EDGE_CURVE('',#23744,#23744,#19871,.T.);
#29176=EDGE_CURVE('',#23745,#23745,#19872,.T.);
#29177=EDGE_CURVE('',#23745,#23746,#5712,.T.);
#29178=EDGE_CURVE('',#23746,#23746,#19873,.T.);
#29179=EDGE_CURVE('',#23747,#23747,#19874,.T.);
#29180=EDGE_CURVE('',#23747,#23748,#5713,.T.);
#29181=EDGE_CURVE('',#23748,#23748,#19875,.T.);
#29182=EDGE_CURVE('',#23749,#23749,#19876,.T.);
#29183=EDGE_CURVE('',#23749,#23750,#5714,.T.);
#29184=EDGE_CURVE('',#23750,#23750,#19877,.T.);
#29185=EDGE_CURVE('',#23751,#23751,#19878,.T.);
#29186=EDGE_CURVE('',#23751,#23752,#5715,.T.);
#29187=EDGE_CURVE('',#23752,#23752,#19879,.T.);
#29188=EDGE_CURVE('',#23753,#23753,#19880,.T.);
#29189=EDGE_CURVE('',#23753,#23754,#5716,.T.);
#29190=EDGE_CURVE('',#23754,#23754,#19881,.T.);
#29191=EDGE_CURVE('',#23755,#23755,#19882,.T.);
#29192=EDGE_CURVE('',#23755,#23756,#5717,.T.);
#29193=EDGE_CURVE('',#23756,#23756,#19883,.T.);
#29194=EDGE_CURVE('',#23757,#23757,#19884,.T.);
#29195=EDGE_CURVE('',#23757,#23758,#5718,.T.);
#29196=EDGE_CURVE('',#23758,#23758,#19885,.T.);
#29197=EDGE_CURVE('',#23759,#23759,#19886,.T.);
#29198=EDGE_CURVE('',#23759,#23760,#5719,.T.);
#29199=EDGE_CURVE('',#23760,#23760,#19887,.T.);
#29200=EDGE_CURVE('',#23761,#23761,#19888,.T.);
#29201=EDGE_CURVE('',#23761,#23762,#5720,.T.);
#29202=EDGE_CURVE('',#23762,#23762,#19889,.T.);
#29203=EDGE_CURVE('',#23763,#23763,#19890,.T.);
#29204=EDGE_CURVE('',#23763,#23764,#5721,.T.);
#29205=EDGE_CURVE('',#23764,#23764,#19891,.T.);
#29206=EDGE_CURVE('',#23765,#23765,#19892,.T.);
#29207=EDGE_CURVE('',#23765,#23766,#5722,.T.);
#29208=EDGE_CURVE('',#23766,#23766,#19893,.T.);
#29209=EDGE_CURVE('',#23767,#23767,#19894,.T.);
#29210=EDGE_CURVE('',#23767,#23768,#5723,.T.);
#29211=EDGE_CURVE('',#23768,#23768,#19895,.T.);
#29212=EDGE_CURVE('',#23769,#23769,#19896,.T.);
#29213=EDGE_CURVE('',#23769,#23770,#5724,.T.);
#29214=EDGE_CURVE('',#23770,#23770,#19897,.T.);
#29215=EDGE_CURVE('',#23771,#23771,#19898,.T.);
#29216=EDGE_CURVE('',#23771,#23772,#5725,.T.);
#29217=EDGE_CURVE('',#23772,#23772,#19899,.T.);
#29218=EDGE_CURVE('',#23773,#23773,#19900,.T.);
#29219=EDGE_CURVE('',#23773,#23774,#5726,.T.);
#29220=EDGE_CURVE('',#23774,#23774,#19901,.T.);
#29221=EDGE_CURVE('',#23775,#23775,#19902,.T.);
#29222=EDGE_CURVE('',#23775,#23776,#5727,.T.);
#29223=EDGE_CURVE('',#23776,#23776,#19903,.T.);
#29224=EDGE_CURVE('',#23777,#23777,#19904,.T.);
#29225=EDGE_CURVE('',#23777,#23778,#5728,.T.);
#29226=EDGE_CURVE('',#23778,#23778,#19905,.T.);
#29227=EDGE_CURVE('',#23779,#23779,#19906,.T.);
#29228=EDGE_CURVE('',#23779,#23780,#5729,.T.);
#29229=EDGE_CURVE('',#23780,#23780,#19907,.T.);
#29230=EDGE_CURVE('',#23781,#23781,#19908,.T.);
#29231=EDGE_CURVE('',#23781,#23782,#5730,.T.);
#29232=EDGE_CURVE('',#23782,#23782,#19909,.T.);
#29233=EDGE_CURVE('',#23783,#23783,#19910,.T.);
#29234=EDGE_CURVE('',#23783,#23784,#5731,.T.);
#29235=EDGE_CURVE('',#23784,#23784,#19911,.T.);
#29236=EDGE_CURVE('',#23785,#23785,#19912,.T.);
#29237=EDGE_CURVE('',#23785,#23786,#5732,.T.);
#29238=EDGE_CURVE('',#23786,#23786,#19913,.T.);
#29239=EDGE_CURVE('',#23787,#23787,#19914,.T.);
#29240=EDGE_CURVE('',#23787,#23788,#5733,.T.);
#29241=EDGE_CURVE('',#23788,#23788,#19915,.T.);
#29242=EDGE_CURVE('',#23789,#23789,#19916,.T.);
#29243=EDGE_CURVE('',#23789,#23790,#5734,.T.);
#29244=EDGE_CURVE('',#23790,#23790,#19917,.T.);
#29245=EDGE_CURVE('',#23791,#23791,#19918,.T.);
#29246=EDGE_CURVE('',#23791,#23792,#5735,.T.);
#29247=EDGE_CURVE('',#23792,#23792,#19919,.T.);
#29248=EDGE_CURVE('',#23793,#23793,#19920,.T.);
#29249=EDGE_CURVE('',#23793,#23794,#5736,.T.);
#29250=EDGE_CURVE('',#23794,#23794,#19921,.T.);
#29251=EDGE_CURVE('',#23795,#23795,#19922,.T.);
#29252=EDGE_CURVE('',#23795,#23796,#5737,.T.);
#29253=EDGE_CURVE('',#23796,#23796,#19923,.T.);
#29254=EDGE_CURVE('',#23797,#23797,#19924,.T.);
#29255=EDGE_CURVE('',#23797,#23798,#5738,.T.);
#29256=EDGE_CURVE('',#23798,#23798,#19925,.T.);
#29257=EDGE_CURVE('',#23799,#23799,#19926,.T.);
#29258=EDGE_CURVE('',#23799,#23800,#5739,.T.);
#29259=EDGE_CURVE('',#23800,#23800,#19927,.T.);
#29260=EDGE_CURVE('',#23801,#23801,#19928,.T.);
#29261=EDGE_CURVE('',#23801,#23802,#5740,.T.);
#29262=EDGE_CURVE('',#23802,#23802,#19929,.T.);
#29263=EDGE_CURVE('',#23803,#23803,#19930,.T.);
#29264=EDGE_CURVE('',#23803,#23804,#5741,.T.);
#29265=EDGE_CURVE('',#23804,#23804,#19931,.T.);
#29266=EDGE_CURVE('',#23805,#23805,#19932,.T.);
#29267=EDGE_CURVE('',#23805,#23806,#5742,.T.);
#29268=EDGE_CURVE('',#23806,#23806,#19933,.T.);
#29269=EDGE_CURVE('',#23807,#23807,#19934,.T.);
#29270=EDGE_CURVE('',#23807,#23808,#5743,.T.);
#29271=EDGE_CURVE('',#23808,#23808,#19935,.T.);
#29272=EDGE_CURVE('',#23809,#23809,#19936,.T.);
#29273=EDGE_CURVE('',#23809,#23810,#5744,.T.);
#29274=EDGE_CURVE('',#23810,#23810,#19937,.T.);
#29275=EDGE_CURVE('',#23811,#23811,#19938,.T.);
#29276=EDGE_CURVE('',#23811,#23812,#5745,.T.);
#29277=EDGE_CURVE('',#23812,#23812,#19939,.T.);
#29278=EDGE_CURVE('',#23813,#23813,#19940,.T.);
#29279=EDGE_CURVE('',#23813,#23814,#5746,.T.);
#29280=EDGE_CURVE('',#23814,#23814,#19941,.T.);
#29281=EDGE_CURVE('',#23815,#23815,#19942,.T.);
#29282=EDGE_CURVE('',#23815,#23816,#5747,.T.);
#29283=EDGE_CURVE('',#23816,#23816,#19943,.T.);
#29284=EDGE_CURVE('',#23817,#23817,#19944,.T.);
#29285=EDGE_CURVE('',#23817,#23818,#5748,.T.);
#29286=EDGE_CURVE('',#23818,#23818,#19945,.T.);
#29287=EDGE_CURVE('',#23819,#23819,#19946,.T.);
#29288=EDGE_CURVE('',#23819,#23820,#5749,.T.);
#29289=EDGE_CURVE('',#23820,#23820,#19947,.T.);
#29290=EDGE_CURVE('',#23821,#23821,#19948,.T.);
#29291=EDGE_CURVE('',#23821,#23822,#5750,.T.);
#29292=EDGE_CURVE('',#23822,#23822,#19949,.T.);
#29293=EDGE_CURVE('',#23823,#23823,#19950,.T.);
#29294=EDGE_CURVE('',#23823,#23824,#5751,.T.);
#29295=EDGE_CURVE('',#23824,#23824,#19951,.T.);
#29296=EDGE_CURVE('',#23825,#23825,#19952,.T.);
#29297=EDGE_CURVE('',#23825,#23826,#5752,.T.);
#29298=EDGE_CURVE('',#23826,#23826,#19953,.T.);
#29299=EDGE_CURVE('',#23827,#23827,#19954,.T.);
#29300=EDGE_CURVE('',#23827,#23828,#5753,.T.);
#29301=EDGE_CURVE('',#23828,#23828,#19955,.T.);
#29302=EDGE_CURVE('',#23829,#23829,#19956,.T.);
#29303=EDGE_CURVE('',#23829,#23830,#5754,.T.);
#29304=EDGE_CURVE('',#23830,#23830,#19957,.T.);
#29305=EDGE_CURVE('',#23831,#23831,#19958,.T.);
#29306=EDGE_CURVE('',#23831,#23832,#5755,.T.);
#29307=EDGE_CURVE('',#23832,#23832,#19959,.T.);
#29308=EDGE_CURVE('',#23833,#23833,#19960,.T.);
#29309=EDGE_CURVE('',#23833,#23834,#5756,.T.);
#29310=EDGE_CURVE('',#23834,#23834,#19961,.T.);
#29311=EDGE_CURVE('',#23835,#23835,#19962,.T.);
#29312=EDGE_CURVE('',#23835,#23836,#5757,.T.);
#29313=EDGE_CURVE('',#23836,#23836,#19963,.T.);
#29314=EDGE_CURVE('',#23837,#23837,#19964,.T.);
#29315=EDGE_CURVE('',#23837,#23838,#5758,.T.);
#29316=EDGE_CURVE('',#23838,#23838,#19965,.T.);
#29317=EDGE_CURVE('',#23839,#23839,#19966,.T.);
#29318=EDGE_CURVE('',#23839,#23840,#5759,.T.);
#29319=EDGE_CURVE('',#23840,#23840,#19967,.T.);
#29320=EDGE_CURVE('',#23841,#23841,#19968,.T.);
#29321=EDGE_CURVE('',#23841,#23842,#5760,.T.);
#29322=EDGE_CURVE('',#23842,#23842,#19969,.T.);
#29323=EDGE_CURVE('',#23843,#23843,#19970,.T.);
#29324=EDGE_CURVE('',#23843,#23844,#5761,.T.);
#29325=EDGE_CURVE('',#23844,#23844,#19971,.T.);
#29326=EDGE_CURVE('',#23845,#23845,#19972,.T.);
#29327=EDGE_CURVE('',#23845,#23846,#5762,.T.);
#29328=EDGE_CURVE('',#23846,#23846,#19973,.T.);
#29329=EDGE_CURVE('',#23847,#23847,#19974,.T.);
#29330=EDGE_CURVE('',#23847,#23848,#5763,.T.);
#29331=EDGE_CURVE('',#23848,#23848,#19975,.T.);
#29332=EDGE_CURVE('',#23849,#23849,#19976,.T.);
#29333=EDGE_CURVE('',#23849,#23850,#5764,.T.);
#29334=EDGE_CURVE('',#23850,#23850,#19977,.T.);
#29335=EDGE_CURVE('',#23851,#23851,#19978,.T.);
#29336=EDGE_CURVE('',#23851,#23852,#5765,.T.);
#29337=EDGE_CURVE('',#23852,#23852,#19979,.T.);
#29338=EDGE_CURVE('',#23853,#23853,#19980,.T.);
#29339=EDGE_CURVE('',#23853,#23854,#5766,.T.);
#29340=EDGE_CURVE('',#23854,#23854,#19981,.T.);
#29341=EDGE_CURVE('',#23855,#23855,#19982,.T.);
#29342=EDGE_CURVE('',#23855,#23856,#5767,.T.);
#29343=EDGE_CURVE('',#23856,#23856,#19983,.T.);
#29344=EDGE_CURVE('',#23857,#23857,#19984,.T.);
#29345=EDGE_CURVE('',#23857,#23858,#5768,.T.);
#29346=EDGE_CURVE('',#23858,#23858,#19985,.T.);
#29347=EDGE_CURVE('',#23859,#23859,#19986,.T.);
#29348=EDGE_CURVE('',#23859,#23860,#5769,.T.);
#29349=EDGE_CURVE('',#23860,#23860,#19987,.T.);
#29350=EDGE_CURVE('',#23861,#23861,#19988,.T.);
#29351=EDGE_CURVE('',#23861,#23862,#5770,.T.);
#29352=EDGE_CURVE('',#23862,#23862,#19989,.T.);
#29353=EDGE_CURVE('',#23863,#23863,#19990,.T.);
#29354=EDGE_CURVE('',#23863,#23864,#5771,.T.);
#29355=EDGE_CURVE('',#23864,#23864,#19991,.T.);
#29356=EDGE_CURVE('',#23865,#23865,#19992,.T.);
#29357=EDGE_CURVE('',#23865,#23866,#5772,.T.);
#29358=EDGE_CURVE('',#23866,#23866,#19993,.T.);
#29359=EDGE_CURVE('',#23867,#23867,#19994,.T.);
#29360=EDGE_CURVE('',#23867,#23868,#5773,.T.);
#29361=EDGE_CURVE('',#23868,#23868,#19995,.T.);
#29362=EDGE_CURVE('',#23869,#23869,#19996,.T.);
#29363=EDGE_CURVE('',#23869,#23870,#5774,.T.);
#29364=EDGE_CURVE('',#23870,#23870,#19997,.T.);
#29365=EDGE_CURVE('',#23871,#23871,#19998,.T.);
#29366=EDGE_CURVE('',#23871,#23872,#5775,.T.);
#29367=EDGE_CURVE('',#23872,#23872,#19999,.T.);
#29368=EDGE_CURVE('',#23873,#23873,#20000,.T.);
#29369=EDGE_CURVE('',#23873,#23874,#5776,.T.);
#29370=EDGE_CURVE('',#23874,#23874,#20001,.T.);
#29371=EDGE_CURVE('',#23875,#23875,#20002,.T.);
#29372=EDGE_CURVE('',#23875,#23876,#5777,.T.);
#29373=EDGE_CURVE('',#23876,#23876,#20003,.T.);
#29374=EDGE_CURVE('',#23877,#23877,#20004,.T.);
#29375=EDGE_CURVE('',#23877,#23878,#5778,.T.);
#29376=EDGE_CURVE('',#23878,#23878,#20005,.T.);
#29377=EDGE_CURVE('',#23879,#23879,#20006,.T.);
#29378=EDGE_CURVE('',#23879,#23880,#5779,.T.);
#29379=EDGE_CURVE('',#23880,#23880,#20007,.T.);
#29380=EDGE_CURVE('',#23881,#23881,#20008,.T.);
#29381=EDGE_CURVE('',#23881,#23882,#5780,.T.);
#29382=EDGE_CURVE('',#23882,#23882,#20009,.T.);
#29383=EDGE_CURVE('',#23883,#23883,#20010,.T.);
#29384=EDGE_CURVE('',#23883,#23884,#5781,.T.);
#29385=EDGE_CURVE('',#23884,#23884,#20011,.T.);
#29386=EDGE_CURVE('',#23885,#23885,#20012,.T.);
#29387=EDGE_CURVE('',#23885,#23886,#5782,.T.);
#29388=EDGE_CURVE('',#23886,#23886,#20013,.T.);
#29389=EDGE_CURVE('',#23887,#23887,#20014,.T.);
#29390=EDGE_CURVE('',#23887,#23888,#5783,.T.);
#29391=EDGE_CURVE('',#23888,#23888,#20015,.T.);
#29392=EDGE_CURVE('',#23889,#23889,#20016,.T.);
#29393=EDGE_CURVE('',#23889,#23890,#5784,.T.);
#29394=EDGE_CURVE('',#23890,#23890,#20017,.T.);
#29395=EDGE_CURVE('',#23891,#23891,#20018,.T.);
#29396=EDGE_CURVE('',#23891,#23892,#5785,.T.);
#29397=EDGE_CURVE('',#23892,#23892,#20019,.T.);
#29398=EDGE_CURVE('',#23893,#23893,#20020,.T.);
#29399=EDGE_CURVE('',#23893,#23894,#5786,.T.);
#29400=EDGE_CURVE('',#23894,#23894,#20021,.T.);
#29401=EDGE_CURVE('',#23895,#23895,#20022,.T.);
#29402=EDGE_CURVE('',#23895,#23896,#5787,.T.);
#29403=EDGE_CURVE('',#23896,#23896,#20023,.T.);
#29404=EDGE_CURVE('',#23897,#23897,#20024,.T.);
#29405=EDGE_CURVE('',#23897,#23898,#5788,.T.);
#29406=EDGE_CURVE('',#23898,#23898,#20025,.T.);
#29407=EDGE_CURVE('',#23899,#23899,#20026,.T.);
#29408=EDGE_CURVE('',#23899,#23900,#5789,.T.);
#29409=EDGE_CURVE('',#23900,#23900,#20027,.T.);
#29410=EDGE_CURVE('',#23901,#23901,#20028,.T.);
#29411=EDGE_CURVE('',#23901,#23902,#5790,.T.);
#29412=EDGE_CURVE('',#23902,#23902,#20029,.T.);
#29413=EDGE_CURVE('',#23903,#23903,#20030,.T.);
#29414=EDGE_CURVE('',#23903,#23904,#5791,.T.);
#29415=EDGE_CURVE('',#23904,#23904,#20031,.T.);
#29416=EDGE_CURVE('',#23905,#23905,#20032,.T.);
#29417=EDGE_CURVE('',#23905,#23906,#5792,.T.);
#29418=EDGE_CURVE('',#23906,#23906,#20033,.T.);
#29419=EDGE_CURVE('',#23907,#23907,#20034,.T.);
#29420=EDGE_CURVE('',#23907,#23908,#5793,.T.);
#29421=EDGE_CURVE('',#23908,#23908,#20035,.T.);
#29422=EDGE_CURVE('',#23909,#23909,#20036,.T.);
#29423=EDGE_CURVE('',#23909,#23910,#5794,.T.);
#29424=EDGE_CURVE('',#23910,#23910,#20037,.T.);
#29425=EDGE_CURVE('',#23911,#23911,#20038,.T.);
#29426=EDGE_CURVE('',#23911,#23912,#5795,.T.);
#29427=EDGE_CURVE('',#23912,#23912,#20039,.T.);
#29428=EDGE_CURVE('',#23913,#23913,#20040,.T.);
#29429=EDGE_CURVE('',#23913,#23914,#5796,.T.);
#29430=EDGE_CURVE('',#23914,#23914,#20041,.T.);
#29431=EDGE_CURVE('',#23915,#23915,#20042,.T.);
#29432=EDGE_CURVE('',#23915,#23916,#5797,.T.);
#29433=EDGE_CURVE('',#23916,#23916,#20043,.T.);
#29434=EDGE_CURVE('',#23917,#23917,#20044,.T.);
#29435=EDGE_CURVE('',#23917,#23918,#5798,.T.);
#29436=EDGE_CURVE('',#23918,#23918,#20045,.T.);
#29437=EDGE_CURVE('',#23919,#23919,#20046,.T.);
#29438=EDGE_CURVE('',#23919,#23920,#5799,.T.);
#29439=EDGE_CURVE('',#23920,#23920,#20047,.T.);
#29440=EDGE_CURVE('',#23921,#23921,#20048,.T.);
#29441=EDGE_CURVE('',#23921,#23922,#5800,.T.);
#29442=EDGE_CURVE('',#23922,#23922,#20049,.T.);
#29443=EDGE_CURVE('',#23923,#23923,#20050,.T.);
#29444=EDGE_CURVE('',#23923,#23924,#5801,.T.);
#29445=EDGE_CURVE('',#23924,#23924,#20051,.T.);
#29446=EDGE_CURVE('',#23925,#23925,#20052,.T.);
#29447=EDGE_CURVE('',#23925,#23926,#5802,.T.);
#29448=EDGE_CURVE('',#23926,#23926,#20053,.T.);
#29449=EDGE_CURVE('',#23927,#23927,#20054,.T.);
#29450=EDGE_CURVE('',#23927,#23928,#5803,.T.);
#29451=EDGE_CURVE('',#23928,#23928,#20055,.T.);
#29452=EDGE_CURVE('',#23929,#23929,#20056,.T.);
#29453=EDGE_CURVE('',#23929,#23930,#5804,.T.);
#29454=EDGE_CURVE('',#23930,#23930,#20057,.T.);
#29455=EDGE_CURVE('',#23931,#23931,#20058,.T.);
#29456=EDGE_CURVE('',#23931,#23932,#5805,.T.);
#29457=EDGE_CURVE('',#23932,#23932,#20059,.T.);
#29458=EDGE_CURVE('',#23933,#23933,#20060,.T.);
#29459=EDGE_CURVE('',#23933,#23934,#5806,.T.);
#29460=EDGE_CURVE('',#23934,#23934,#20061,.T.);
#29461=EDGE_CURVE('',#23935,#23935,#20062,.T.);
#29462=EDGE_CURVE('',#23935,#23936,#5807,.T.);
#29463=EDGE_CURVE('',#23936,#23936,#20063,.T.);
#29464=EDGE_CURVE('',#23937,#23937,#20064,.T.);
#29465=EDGE_CURVE('',#23937,#23938,#5808,.T.);
#29466=EDGE_CURVE('',#23938,#23938,#20065,.T.);
#29467=EDGE_CURVE('',#23939,#23939,#20066,.T.);
#29468=EDGE_CURVE('',#23939,#23940,#5809,.T.);
#29469=EDGE_CURVE('',#23940,#23940,#20067,.T.);
#29470=EDGE_CURVE('',#23941,#23941,#20068,.T.);
#29471=EDGE_CURVE('',#23941,#23942,#5810,.T.);
#29472=EDGE_CURVE('',#23942,#23942,#20069,.T.);
#29473=EDGE_CURVE('',#23943,#23943,#20070,.T.);
#29474=EDGE_CURVE('',#23943,#23944,#5811,.T.);
#29475=EDGE_CURVE('',#23944,#23944,#20071,.T.);
#29476=EDGE_CURVE('',#23945,#23945,#20072,.T.);
#29477=EDGE_CURVE('',#23945,#23946,#5812,.T.);
#29478=EDGE_CURVE('',#23946,#23946,#20073,.T.);
#29479=EDGE_CURVE('',#23947,#23947,#20074,.T.);
#29480=EDGE_CURVE('',#23947,#23948,#5813,.T.);
#29481=EDGE_CURVE('',#23948,#23948,#20075,.T.);
#29482=EDGE_CURVE('',#23949,#23949,#20076,.T.);
#29483=EDGE_CURVE('',#23949,#23950,#5814,.T.);
#29484=EDGE_CURVE('',#23950,#23950,#20077,.T.);
#29485=EDGE_CURVE('',#23951,#23951,#20078,.T.);
#29486=EDGE_CURVE('',#23951,#23952,#5815,.T.);
#29487=EDGE_CURVE('',#23952,#23952,#20079,.T.);
#29488=EDGE_CURVE('',#23953,#23953,#20080,.T.);
#29489=EDGE_CURVE('',#23953,#23954,#5816,.T.);
#29490=EDGE_CURVE('',#23954,#23954,#20081,.T.);
#29491=EDGE_CURVE('',#23955,#23955,#20082,.T.);
#29492=EDGE_CURVE('',#23955,#23956,#5817,.T.);
#29493=EDGE_CURVE('',#23956,#23956,#20083,.T.);
#29494=EDGE_CURVE('',#23957,#23957,#20084,.T.);
#29495=EDGE_CURVE('',#23957,#23958,#5818,.T.);
#29496=EDGE_CURVE('',#23958,#23958,#20085,.T.);
#29497=EDGE_CURVE('',#23959,#23959,#20086,.T.);
#29498=EDGE_CURVE('',#23959,#23960,#5819,.T.);
#29499=EDGE_CURVE('',#23960,#23960,#20087,.T.);
#29500=EDGE_CURVE('',#23961,#23961,#20088,.T.);
#29501=EDGE_CURVE('',#23961,#23962,#5820,.T.);
#29502=EDGE_CURVE('',#23962,#23962,#20089,.T.);
#29503=EDGE_CURVE('',#23963,#23963,#20090,.T.);
#29504=EDGE_CURVE('',#23963,#23964,#5821,.T.);
#29505=EDGE_CURVE('',#23964,#23964,#20091,.T.);
#29506=EDGE_CURVE('',#23965,#23965,#20092,.T.);
#29507=EDGE_CURVE('',#23965,#23966,#5822,.T.);
#29508=EDGE_CURVE('',#23966,#23966,#20093,.T.);
#29509=EDGE_CURVE('',#23967,#23967,#20094,.T.);
#29510=EDGE_CURVE('',#23967,#23968,#5823,.T.);
#29511=EDGE_CURVE('',#23968,#23968,#20095,.T.);
#29512=EDGE_CURVE('',#23969,#23969,#20096,.T.);
#29513=EDGE_CURVE('',#23969,#23970,#5824,.T.);
#29514=EDGE_CURVE('',#23970,#23970,#20097,.T.);
#29515=EDGE_CURVE('',#23971,#23971,#20098,.T.);
#29516=EDGE_CURVE('',#23971,#23972,#5825,.T.);
#29517=EDGE_CURVE('',#23972,#23972,#20099,.T.);
#29518=EDGE_CURVE('',#23973,#23973,#20100,.T.);
#29519=EDGE_CURVE('',#23973,#23974,#5826,.T.);
#29520=EDGE_CURVE('',#23974,#23974,#20101,.T.);
#29521=EDGE_CURVE('',#23975,#23975,#20102,.T.);
#29522=EDGE_CURVE('',#23975,#23976,#5827,.T.);
#29523=EDGE_CURVE('',#23976,#23976,#20103,.T.);
#29524=EDGE_CURVE('',#23977,#23977,#20104,.T.);
#29525=EDGE_CURVE('',#23977,#23978,#5828,.T.);
#29526=EDGE_CURVE('',#23978,#23978,#20105,.T.);
#29527=EDGE_CURVE('',#23979,#23979,#20106,.T.);
#29528=EDGE_CURVE('',#23979,#23980,#5829,.T.);
#29529=EDGE_CURVE('',#23980,#23980,#20107,.T.);
#29530=EDGE_CURVE('',#23981,#23981,#20108,.T.);
#29531=EDGE_CURVE('',#23981,#23982,#5830,.T.);
#29532=EDGE_CURVE('',#23982,#23982,#20109,.T.);
#29533=EDGE_CURVE('',#23983,#23983,#20110,.T.);
#29534=EDGE_CURVE('',#23983,#23984,#5831,.T.);
#29535=EDGE_CURVE('',#23984,#23984,#20111,.T.);
#29536=EDGE_CURVE('',#23985,#23985,#20112,.T.);
#29537=EDGE_CURVE('',#23985,#23986,#5832,.T.);
#29538=EDGE_CURVE('',#23986,#23986,#20113,.T.);
#29539=EDGE_CURVE('',#23987,#23987,#20114,.T.);
#29540=EDGE_CURVE('',#23987,#23988,#5833,.T.);
#29541=EDGE_CURVE('',#23988,#23988,#20115,.T.);
#29542=EDGE_CURVE('',#23989,#23989,#20116,.T.);
#29543=EDGE_CURVE('',#23989,#23990,#5834,.T.);
#29544=EDGE_CURVE('',#23990,#23990,#20117,.T.);
#29545=EDGE_CURVE('',#23991,#23991,#20118,.T.);
#29546=EDGE_CURVE('',#23991,#23992,#5835,.T.);
#29547=EDGE_CURVE('',#23992,#23992,#20119,.T.);
#29548=EDGE_CURVE('',#23993,#23993,#20120,.T.);
#29549=EDGE_CURVE('',#23993,#23994,#5836,.T.);
#29550=EDGE_CURVE('',#23994,#23994,#20121,.T.);
#29551=EDGE_CURVE('',#23995,#23995,#20122,.T.);
#29552=EDGE_CURVE('',#23995,#23996,#5837,.T.);
#29553=EDGE_CURVE('',#23996,#23996,#20123,.T.);
#29554=EDGE_CURVE('',#23997,#23997,#20124,.T.);
#29555=EDGE_CURVE('',#23997,#23998,#5838,.T.);
#29556=EDGE_CURVE('',#23998,#23998,#20125,.T.);
#29557=EDGE_CURVE('',#23999,#23999,#20126,.T.);
#29558=EDGE_CURVE('',#23999,#24000,#5839,.T.);
#29559=EDGE_CURVE('',#24000,#24000,#20127,.T.);
#29560=EDGE_CURVE('',#24001,#24001,#20128,.T.);
#29561=EDGE_CURVE('',#24001,#24002,#5840,.T.);
#29562=EDGE_CURVE('',#24002,#24002,#20129,.T.);
#29563=EDGE_CURVE('',#24003,#24003,#20130,.T.);
#29564=EDGE_CURVE('',#24003,#24004,#5841,.T.);
#29565=EDGE_CURVE('',#24004,#24004,#20131,.T.);
#29566=EDGE_CURVE('',#24005,#24005,#20132,.T.);
#29567=EDGE_CURVE('',#24005,#24006,#5842,.T.);
#29568=EDGE_CURVE('',#24006,#24006,#20133,.T.);
#29569=EDGE_CURVE('',#24007,#24007,#20134,.T.);
#29570=EDGE_CURVE('',#24007,#24008,#5843,.T.);
#29571=EDGE_CURVE('',#24008,#24008,#20135,.T.);
#29572=EDGE_CURVE('',#24009,#24009,#20136,.T.);
#29573=EDGE_CURVE('',#24009,#24010,#5844,.T.);
#29574=EDGE_CURVE('',#24010,#24010,#20137,.T.);
#29575=EDGE_CURVE('',#24011,#24011,#20138,.T.);
#29576=EDGE_CURVE('',#24011,#24012,#5845,.T.);
#29577=EDGE_CURVE('',#24012,#24012,#20139,.T.);
#29578=EDGE_CURVE('',#24013,#24013,#20140,.T.);
#29579=EDGE_CURVE('',#24013,#24014,#5846,.T.);
#29580=EDGE_CURVE('',#24014,#24014,#20141,.T.);
#29581=EDGE_CURVE('',#24015,#24015,#20142,.T.);
#29582=EDGE_CURVE('',#24015,#24016,#5847,.T.);
#29583=EDGE_CURVE('',#24016,#24016,#20143,.T.);
#29584=EDGE_CURVE('',#24017,#24017,#20144,.T.);
#29585=EDGE_CURVE('',#24017,#24018,#5848,.T.);
#29586=EDGE_CURVE('',#24018,#24018,#20145,.T.);
#29587=EDGE_CURVE('',#24019,#24019,#20146,.T.);
#29588=EDGE_CURVE('',#24019,#24020,#5849,.T.);
#29589=EDGE_CURVE('',#24020,#24020,#20147,.T.);
#29590=EDGE_CURVE('',#24021,#24021,#20148,.T.);
#29591=EDGE_CURVE('',#24021,#24022,#5850,.T.);
#29592=EDGE_CURVE('',#24022,#24022,#20149,.T.);
#29593=EDGE_CURVE('',#24023,#24023,#20150,.T.);
#29594=EDGE_CURVE('',#24023,#24024,#5851,.T.);
#29595=EDGE_CURVE('',#24024,#24024,#20151,.T.);
#29596=EDGE_CURVE('',#24025,#24025,#20152,.T.);
#29597=EDGE_CURVE('',#24025,#24026,#5852,.T.);
#29598=EDGE_CURVE('',#24026,#24026,#20153,.T.);
#29599=EDGE_CURVE('',#24027,#24027,#20154,.T.);
#29600=EDGE_CURVE('',#24027,#24028,#5853,.T.);
#29601=EDGE_CURVE('',#24028,#24028,#20155,.T.);
#29602=EDGE_CURVE('',#24029,#24029,#20156,.T.);
#29603=EDGE_CURVE('',#24029,#24030,#5854,.T.);
#29604=EDGE_CURVE('',#24030,#24030,#20157,.T.);
#29605=EDGE_CURVE('',#24031,#24031,#20158,.T.);
#29606=EDGE_CURVE('',#24031,#24032,#5855,.T.);
#29607=EDGE_CURVE('',#24032,#24032,#20159,.T.);
#29608=EDGE_CURVE('',#24033,#24033,#20160,.T.);
#29609=EDGE_CURVE('',#24033,#24034,#5856,.T.);
#29610=EDGE_CURVE('',#24034,#24034,#20161,.T.);
#29611=EDGE_CURVE('',#24035,#24035,#20162,.T.);
#29612=EDGE_CURVE('',#24035,#24036,#5857,.T.);
#29613=EDGE_CURVE('',#24036,#24036,#20163,.T.);
#29614=EDGE_CURVE('',#24037,#24037,#20164,.T.);
#29615=EDGE_CURVE('',#24037,#24038,#5858,.T.);
#29616=EDGE_CURVE('',#24038,#24038,#20165,.T.);
#29617=EDGE_CURVE('',#24039,#24039,#20166,.T.);
#29618=EDGE_CURVE('',#24039,#24040,#5859,.T.);
#29619=EDGE_CURVE('',#24040,#24040,#20167,.T.);
#29620=EDGE_CURVE('',#24041,#24041,#20168,.T.);
#29621=EDGE_CURVE('',#24041,#24042,#5860,.T.);
#29622=EDGE_CURVE('',#24042,#24042,#20169,.T.);
#29623=EDGE_CURVE('',#24043,#24043,#20170,.T.);
#29624=EDGE_CURVE('',#24043,#24044,#5861,.T.);
#29625=EDGE_CURVE('',#24044,#24044,#20171,.T.);
#29626=EDGE_CURVE('',#24045,#24045,#20172,.T.);
#29627=EDGE_CURVE('',#24045,#24046,#5862,.T.);
#29628=EDGE_CURVE('',#24046,#24046,#20173,.T.);
#29629=EDGE_CURVE('',#24047,#24047,#20174,.T.);
#29630=EDGE_CURVE('',#24047,#24048,#5863,.T.);
#29631=EDGE_CURVE('',#24048,#24048,#20175,.T.);
#29632=EDGE_CURVE('',#24049,#24049,#20176,.T.);
#29633=EDGE_CURVE('',#24049,#24050,#5864,.T.);
#29634=EDGE_CURVE('',#24050,#24050,#20177,.T.);
#29635=EDGE_CURVE('',#24051,#24051,#20178,.T.);
#29636=EDGE_CURVE('',#24051,#24052,#5865,.T.);
#29637=EDGE_CURVE('',#24052,#24052,#20179,.T.);
#29638=EDGE_CURVE('',#24053,#24053,#20180,.T.);
#29639=EDGE_CURVE('',#24053,#24054,#5866,.T.);
#29640=EDGE_CURVE('',#24054,#24054,#20181,.T.);
#29641=EDGE_CURVE('',#24055,#24055,#20182,.T.);
#29642=EDGE_CURVE('',#24055,#24056,#5867,.T.);
#29643=EDGE_CURVE('',#24056,#24056,#20183,.T.);
#29644=EDGE_CURVE('',#24057,#24057,#20184,.T.);
#29645=EDGE_CURVE('',#24057,#24058,#5868,.T.);
#29646=EDGE_CURVE('',#24058,#24058,#20185,.T.);
#29647=EDGE_CURVE('',#24059,#24059,#20186,.T.);
#29648=EDGE_CURVE('',#24059,#24060,#5869,.T.);
#29649=EDGE_CURVE('',#24060,#24060,#20187,.T.);
#29650=EDGE_CURVE('',#24061,#24061,#20188,.T.);
#29651=EDGE_CURVE('',#24061,#24062,#5870,.T.);
#29652=EDGE_CURVE('',#24062,#24062,#20189,.T.);
#29653=EDGE_CURVE('',#24063,#24063,#20190,.T.);
#29654=EDGE_CURVE('',#24063,#24064,#5871,.T.);
#29655=EDGE_CURVE('',#24064,#24064,#20191,.T.);
#29656=EDGE_CURVE('',#24065,#24065,#20192,.T.);
#29657=EDGE_CURVE('',#24065,#24066,#5872,.T.);
#29658=EDGE_CURVE('',#24066,#24066,#20193,.T.);
#29659=EDGE_CURVE('',#24067,#24067,#20194,.T.);
#29660=EDGE_CURVE('',#24067,#24068,#5873,.T.);
#29661=EDGE_CURVE('',#24068,#24068,#20195,.T.);
#29662=EDGE_CURVE('',#24069,#24069,#20196,.T.);
#29663=EDGE_CURVE('',#24069,#24070,#5874,.T.);
#29664=EDGE_CURVE('',#24070,#24070,#20197,.T.);
#29665=EDGE_CURVE('',#24071,#24071,#20198,.T.);
#29666=EDGE_CURVE('',#24071,#24072,#5875,.T.);
#29667=EDGE_CURVE('',#24072,#24072,#20199,.T.);
#29668=EDGE_CURVE('',#24073,#24073,#20200,.T.);
#29669=EDGE_CURVE('',#24073,#24074,#5876,.T.);
#29670=EDGE_CURVE('',#24074,#24074,#20201,.T.);
#29671=EDGE_CURVE('',#24075,#24075,#20202,.T.);
#29672=EDGE_CURVE('',#24075,#24076,#5877,.T.);
#29673=EDGE_CURVE('',#24076,#24076,#20203,.T.);
#29674=EDGE_CURVE('',#24077,#24077,#20204,.T.);
#29675=EDGE_CURVE('',#24077,#24078,#5878,.T.);
#29676=EDGE_CURVE('',#24078,#24078,#20205,.T.);
#29677=EDGE_CURVE('',#24079,#24079,#20206,.T.);
#29678=EDGE_CURVE('',#24079,#24080,#5879,.T.);
#29679=EDGE_CURVE('',#24080,#24080,#20207,.T.);
#29680=EDGE_CURVE('',#24081,#24081,#20208,.T.);
#29681=EDGE_CURVE('',#24081,#24082,#5880,.T.);
#29682=EDGE_CURVE('',#24082,#24082,#20209,.T.);
#29683=EDGE_CURVE('',#24083,#24083,#20210,.T.);
#29684=EDGE_CURVE('',#24083,#24084,#5881,.T.);
#29685=EDGE_CURVE('',#24084,#24084,#20211,.T.);
#29686=EDGE_CURVE('',#24085,#24085,#20212,.T.);
#29687=EDGE_CURVE('',#24085,#24086,#5882,.T.);
#29688=EDGE_CURVE('',#24086,#24086,#20213,.T.);
#29689=EDGE_CURVE('',#24087,#24087,#20214,.T.);
#29690=EDGE_CURVE('',#24087,#24088,#5883,.T.);
#29691=EDGE_CURVE('',#24088,#24088,#20215,.T.);
#29692=EDGE_CURVE('',#24089,#24089,#20216,.T.);
#29693=EDGE_CURVE('',#24089,#24090,#5884,.T.);
#29694=EDGE_CURVE('',#24090,#24090,#20217,.T.);
#29695=EDGE_CURVE('',#24091,#24091,#20218,.T.);
#29696=EDGE_CURVE('',#24091,#24092,#5885,.T.);
#29697=EDGE_CURVE('',#24092,#24092,#20219,.T.);
#29698=EDGE_CURVE('',#24093,#24093,#20220,.T.);
#29699=EDGE_CURVE('',#24093,#24094,#5886,.T.);
#29700=EDGE_CURVE('',#24094,#24094,#20221,.T.);
#29701=EDGE_CURVE('',#24095,#24095,#20222,.T.);
#29702=EDGE_CURVE('',#24095,#24096,#5887,.T.);
#29703=EDGE_CURVE('',#24096,#24096,#20223,.T.);
#29704=EDGE_CURVE('',#24097,#24097,#20224,.T.);
#29705=EDGE_CURVE('',#24097,#24098,#5888,.T.);
#29706=EDGE_CURVE('',#24098,#24098,#20225,.T.);
#29707=EDGE_CURVE('',#24099,#24099,#20226,.T.);
#29708=EDGE_CURVE('',#24099,#24100,#5889,.T.);
#29709=EDGE_CURVE('',#24100,#24100,#20227,.T.);
#29710=EDGE_CURVE('',#24101,#24101,#20228,.T.);
#29711=EDGE_CURVE('',#24101,#24102,#5890,.T.);
#29712=EDGE_CURVE('',#24102,#24102,#20229,.T.);
#29713=EDGE_CURVE('',#24103,#24103,#20230,.T.);
#29714=EDGE_CURVE('',#24103,#24104,#5891,.T.);
#29715=EDGE_CURVE('',#24104,#24104,#20231,.T.);
#29716=EDGE_CURVE('',#24105,#24105,#20232,.T.);
#29717=EDGE_CURVE('',#24105,#24106,#5892,.T.);
#29718=EDGE_CURVE('',#24106,#24106,#20233,.T.);
#29719=EDGE_CURVE('',#24107,#24107,#20234,.T.);
#29720=EDGE_CURVE('',#24107,#24108,#5893,.T.);
#29721=EDGE_CURVE('',#24108,#24108,#20235,.T.);
#29722=EDGE_CURVE('',#24109,#24109,#20236,.T.);
#29723=EDGE_CURVE('',#24109,#24110,#5894,.T.);
#29724=EDGE_CURVE('',#24110,#24110,#20237,.T.);
#29725=EDGE_CURVE('',#24111,#24111,#20238,.T.);
#29726=EDGE_CURVE('',#24111,#24112,#5895,.T.);
#29727=EDGE_CURVE('',#24112,#24112,#20239,.T.);
#29728=EDGE_CURVE('',#24113,#24113,#20240,.T.);
#29729=EDGE_CURVE('',#24113,#24114,#5896,.T.);
#29730=EDGE_CURVE('',#24114,#24114,#20241,.T.);
#29731=EDGE_CURVE('',#24115,#24115,#20242,.T.);
#29732=EDGE_CURVE('',#24115,#24116,#5897,.T.);
#29733=EDGE_CURVE('',#24116,#24116,#20243,.T.);
#29734=EDGE_CURVE('',#24117,#24117,#20244,.T.);
#29735=EDGE_CURVE('',#24117,#24118,#5898,.T.);
#29736=EDGE_CURVE('',#24118,#24118,#20245,.T.);
#29737=EDGE_CURVE('',#24119,#24119,#20246,.T.);
#29738=EDGE_CURVE('',#24119,#24120,#5899,.T.);
#29739=EDGE_CURVE('',#24120,#24120,#20247,.T.);
#29740=EDGE_CURVE('',#24121,#24121,#20248,.T.);
#29741=EDGE_CURVE('',#24121,#24122,#5900,.T.);
#29742=EDGE_CURVE('',#24122,#24122,#20249,.T.);
#29743=EDGE_CURVE('',#24123,#24123,#20250,.T.);
#29744=EDGE_CURVE('',#24123,#24124,#5901,.T.);
#29745=EDGE_CURVE('',#24124,#24124,#20251,.T.);
#29746=EDGE_CURVE('',#24125,#24125,#20252,.T.);
#29747=EDGE_CURVE('',#24125,#24126,#5902,.T.);
#29748=EDGE_CURVE('',#24126,#24126,#20253,.T.);
#29749=EDGE_CURVE('',#24127,#24127,#20254,.T.);
#29750=EDGE_CURVE('',#24127,#24128,#5903,.T.);
#29751=EDGE_CURVE('',#24128,#24128,#20255,.T.);
#29752=EDGE_CURVE('',#24129,#24129,#20256,.T.);
#29753=EDGE_CURVE('',#24129,#24130,#5904,.T.);
#29754=EDGE_CURVE('',#24130,#24130,#20257,.T.);
#29755=EDGE_CURVE('',#24131,#24131,#20258,.T.);
#29756=EDGE_CURVE('',#24131,#24132,#5905,.T.);
#29757=EDGE_CURVE('',#24132,#24132,#20259,.T.);
#29758=EDGE_CURVE('',#24133,#24133,#20260,.T.);
#29759=EDGE_CURVE('',#24133,#24134,#5906,.T.);
#29760=EDGE_CURVE('',#24134,#24134,#20261,.T.);
#29761=EDGE_CURVE('',#24135,#24135,#20262,.T.);
#29762=EDGE_CURVE('',#24135,#24136,#5907,.T.);
#29763=EDGE_CURVE('',#24136,#24136,#20263,.T.);
#29764=EDGE_CURVE('',#24137,#24137,#20264,.T.);
#29765=EDGE_CURVE('',#24137,#24138,#5908,.T.);
#29766=EDGE_CURVE('',#24138,#24138,#20265,.T.);
#29767=EDGE_CURVE('',#24139,#24139,#20266,.T.);
#29768=EDGE_CURVE('',#24139,#24140,#5909,.T.);
#29769=EDGE_CURVE('',#24140,#24140,#20267,.T.);
#29770=EDGE_CURVE('',#24141,#24141,#20268,.T.);
#29771=EDGE_CURVE('',#24141,#24142,#5910,.T.);
#29772=EDGE_CURVE('',#24142,#24142,#20269,.T.);
#29773=EDGE_CURVE('',#24143,#24143,#20270,.T.);
#29774=EDGE_CURVE('',#24143,#24144,#5911,.T.);
#29775=EDGE_CURVE('',#24144,#24144,#20271,.T.);
#29776=EDGE_CURVE('',#24145,#24145,#20272,.T.);
#29777=EDGE_CURVE('',#24145,#24146,#5912,.T.);
#29778=EDGE_CURVE('',#24146,#24146,#20273,.T.);
#29779=EDGE_CURVE('',#24147,#24147,#20274,.T.);
#29780=EDGE_CURVE('',#24147,#24148,#5913,.T.);
#29781=EDGE_CURVE('',#24148,#24148,#20275,.T.);
#29782=EDGE_CURVE('',#24149,#24149,#20276,.T.);
#29783=EDGE_CURVE('',#24149,#24150,#5914,.T.);
#29784=EDGE_CURVE('',#24150,#24150,#20277,.T.);
#29785=EDGE_CURVE('',#24151,#24151,#20278,.T.);
#29786=EDGE_CURVE('',#24151,#24152,#5915,.T.);
#29787=EDGE_CURVE('',#24152,#24152,#20279,.T.);
#29788=EDGE_CURVE('',#24153,#24153,#20280,.T.);
#29789=EDGE_CURVE('',#24153,#24154,#5916,.T.);
#29790=EDGE_CURVE('',#24154,#24154,#20281,.T.);
#29791=EDGE_CURVE('',#24155,#24155,#20282,.T.);
#29792=EDGE_CURVE('',#24155,#24156,#5917,.T.);
#29793=EDGE_CURVE('',#24156,#24156,#20283,.T.);
#29794=EDGE_CURVE('',#24157,#24157,#20284,.T.);
#29795=EDGE_CURVE('',#24157,#24158,#5918,.T.);
#29796=EDGE_CURVE('',#24158,#24158,#20285,.T.);
#29797=EDGE_CURVE('',#24159,#24159,#20286,.T.);
#29798=EDGE_CURVE('',#24159,#24160,#5919,.T.);
#29799=EDGE_CURVE('',#24160,#24160,#20287,.T.);
#29800=EDGE_CURVE('',#24161,#24161,#20288,.T.);
#29801=EDGE_CURVE('',#24161,#24162,#5920,.T.);
#29802=EDGE_CURVE('',#24162,#24162,#20289,.T.);
#29803=EDGE_CURVE('',#24163,#24163,#20290,.T.);
#29804=EDGE_CURVE('',#24163,#24164,#5921,.T.);
#29805=EDGE_CURVE('',#24164,#24164,#20291,.T.);
#29806=EDGE_CURVE('',#24165,#24165,#20292,.T.);
#29807=EDGE_CURVE('',#24165,#24166,#5922,.T.);
#29808=EDGE_CURVE('',#24166,#24166,#20293,.T.);
#29809=EDGE_CURVE('',#24167,#24167,#20294,.T.);
#29810=EDGE_CURVE('',#24167,#24168,#5923,.T.);
#29811=EDGE_CURVE('',#24168,#24168,#20295,.T.);
#29812=EDGE_CURVE('',#24169,#24169,#20296,.T.);
#29813=EDGE_CURVE('',#24169,#24170,#5924,.T.);
#29814=EDGE_CURVE('',#24170,#24170,#20297,.T.);
#29815=EDGE_CURVE('',#24171,#24171,#20298,.T.);
#29816=EDGE_CURVE('',#24171,#24172,#5925,.T.);
#29817=EDGE_CURVE('',#24172,#24172,#20299,.T.);
#29818=EDGE_CURVE('',#24173,#24173,#20300,.T.);
#29819=EDGE_CURVE('',#24173,#24174,#5926,.T.);
#29820=EDGE_CURVE('',#24174,#24174,#20301,.T.);
#29821=EDGE_CURVE('',#24175,#24175,#20302,.T.);
#29822=EDGE_CURVE('',#24175,#24176,#5927,.T.);
#29823=EDGE_CURVE('',#24176,#24176,#20303,.T.);
#29824=EDGE_CURVE('',#24177,#24177,#20304,.T.);
#29825=EDGE_CURVE('',#24177,#24178,#5928,.T.);
#29826=EDGE_CURVE('',#24178,#24178,#20305,.T.);
#29827=EDGE_CURVE('',#24179,#24179,#20306,.T.);
#29828=EDGE_CURVE('',#24179,#24180,#5929,.T.);
#29829=EDGE_CURVE('',#24180,#24180,#20307,.T.);
#29830=EDGE_CURVE('',#24181,#24181,#20308,.T.);
#29831=EDGE_CURVE('',#24181,#24182,#5930,.T.);
#29832=EDGE_CURVE('',#24182,#24182,#20309,.T.);
#29833=EDGE_CURVE('',#24183,#24183,#20310,.T.);
#29834=EDGE_CURVE('',#24183,#24184,#5931,.T.);
#29835=EDGE_CURVE('',#24184,#24184,#20311,.T.);
#29836=EDGE_CURVE('',#24185,#24185,#20312,.T.);
#29837=EDGE_CURVE('',#24185,#24186,#5932,.T.);
#29838=EDGE_CURVE('',#24186,#24186,#20313,.T.);
#29839=EDGE_CURVE('',#24187,#24187,#20314,.T.);
#29840=EDGE_CURVE('',#24187,#24188,#5933,.T.);
#29841=EDGE_CURVE('',#24188,#24188,#20315,.T.);
#29842=EDGE_CURVE('',#24189,#24189,#20316,.T.);
#29843=EDGE_CURVE('',#24189,#24190,#5934,.T.);
#29844=EDGE_CURVE('',#24190,#24190,#20317,.T.);
#29845=EDGE_CURVE('',#24191,#24191,#20318,.T.);
#29846=EDGE_CURVE('',#24191,#24192,#5935,.T.);
#29847=EDGE_CURVE('',#24192,#24192,#20319,.T.);
#29848=EDGE_CURVE('',#24193,#24193,#20320,.T.);
#29849=EDGE_CURVE('',#24193,#24194,#5936,.T.);
#29850=EDGE_CURVE('',#24194,#24194,#20321,.T.);
#29851=EDGE_CURVE('',#24195,#24195,#20322,.T.);
#29852=EDGE_CURVE('',#24195,#24196,#5937,.T.);
#29853=EDGE_CURVE('',#24196,#24196,#20323,.T.);
#29854=EDGE_CURVE('',#24197,#24197,#20324,.T.);
#29855=EDGE_CURVE('',#24197,#24198,#5938,.T.);
#29856=EDGE_CURVE('',#24198,#24198,#20325,.T.);
#29857=EDGE_CURVE('',#24199,#24199,#20326,.T.);
#29858=EDGE_CURVE('',#24199,#24200,#5939,.T.);
#29859=EDGE_CURVE('',#24200,#24200,#20327,.T.);
#29860=EDGE_CURVE('',#24201,#24201,#20328,.T.);
#29861=EDGE_CURVE('',#24201,#24202,#5940,.T.);
#29862=EDGE_CURVE('',#24202,#24202,#20329,.T.);
#29863=EDGE_CURVE('',#24203,#24203,#20330,.T.);
#29864=EDGE_CURVE('',#24203,#24204,#5941,.T.);
#29865=EDGE_CURVE('',#24204,#24204,#20331,.T.);
#29866=EDGE_CURVE('',#24205,#24205,#20332,.T.);
#29867=EDGE_CURVE('',#24205,#24206,#5942,.T.);
#29868=EDGE_CURVE('',#24206,#24206,#20333,.T.);
#29869=EDGE_CURVE('',#24207,#24207,#20334,.T.);
#29870=EDGE_CURVE('',#24207,#24208,#5943,.T.);
#29871=EDGE_CURVE('',#24208,#24208,#20335,.T.);
#29872=EDGE_CURVE('',#24209,#24209,#20336,.T.);
#29873=EDGE_CURVE('',#24209,#24210,#5944,.T.);
#29874=EDGE_CURVE('',#24210,#24210,#20337,.T.);
#29875=EDGE_CURVE('',#24211,#24211,#20338,.T.);
#29876=EDGE_CURVE('',#24211,#24212,#5945,.T.);
#29877=EDGE_CURVE('',#24212,#24212,#20339,.T.);
#29878=EDGE_CURVE('',#24213,#24213,#20340,.T.);
#29879=EDGE_CURVE('',#24213,#24214,#5946,.T.);
#29880=EDGE_CURVE('',#24214,#24214,#20341,.T.);
#29881=EDGE_CURVE('',#24215,#24215,#20342,.T.);
#29882=EDGE_CURVE('',#24215,#24216,#5947,.T.);
#29883=EDGE_CURVE('',#24216,#24216,#20343,.T.);
#29884=EDGE_CURVE('',#24217,#24217,#20344,.T.);
#29885=EDGE_CURVE('',#24217,#24218,#5948,.T.);
#29886=EDGE_CURVE('',#24218,#24218,#20345,.T.);
#29887=EDGE_CURVE('',#24219,#24219,#20346,.T.);
#29888=EDGE_CURVE('',#24219,#24220,#5949,.T.);
#29889=EDGE_CURVE('',#24220,#24220,#20347,.T.);
#29890=EDGE_CURVE('',#24221,#24221,#20348,.T.);
#29891=EDGE_CURVE('',#24221,#24222,#5950,.T.);
#29892=EDGE_CURVE('',#24222,#24222,#20349,.T.);
#29893=EDGE_CURVE('',#24223,#24223,#20350,.T.);
#29894=EDGE_CURVE('',#24223,#24224,#5951,.T.);
#29895=EDGE_CURVE('',#24224,#24224,#20351,.T.);
#29896=EDGE_CURVE('',#24225,#24225,#20352,.T.);
#29897=EDGE_CURVE('',#24225,#24226,#5952,.T.);
#29898=EDGE_CURVE('',#24226,#24226,#20353,.T.);
#29899=EDGE_CURVE('',#24227,#24227,#20354,.T.);
#29900=EDGE_CURVE('',#24227,#24228,#5953,.T.);
#29901=EDGE_CURVE('',#24228,#24228,#20355,.T.);
#29902=EDGE_CURVE('',#24229,#24229,#20356,.T.);
#29903=EDGE_CURVE('',#24229,#24230,#5954,.T.);
#29904=EDGE_CURVE('',#24230,#24230,#20357,.T.);
#29905=EDGE_CURVE('',#24231,#24231,#20358,.T.);
#29906=EDGE_CURVE('',#24231,#24232,#5955,.T.);
#29907=EDGE_CURVE('',#24232,#24232,#20359,.T.);
#29908=EDGE_CURVE('',#24233,#24233,#20360,.T.);
#29909=EDGE_CURVE('',#24233,#24234,#5956,.T.);
#29910=EDGE_CURVE('',#24234,#24234,#20361,.T.);
#29911=EDGE_CURVE('',#24235,#24235,#20362,.T.);
#29912=EDGE_CURVE('',#24235,#24236,#5957,.T.);
#29913=EDGE_CURVE('',#24236,#24236,#20363,.T.);
#29914=EDGE_CURVE('',#24237,#24237,#20364,.T.);
#29915=EDGE_CURVE('',#24237,#24238,#5958,.T.);
#29916=EDGE_CURVE('',#24238,#24238,#20365,.T.);
#29917=EDGE_CURVE('',#24239,#24239,#20366,.T.);
#29918=EDGE_CURVE('',#24239,#24240,#5959,.T.);
#29919=EDGE_CURVE('',#24240,#24240,#20367,.T.);
#29920=EDGE_CURVE('',#24241,#24241,#20368,.T.);
#29921=EDGE_CURVE('',#24241,#24242,#5960,.T.);
#29922=EDGE_CURVE('',#24242,#24242,#20369,.T.);
#29923=EDGE_CURVE('',#24243,#24243,#20370,.T.);
#29924=EDGE_CURVE('',#24243,#24244,#5961,.T.);
#29925=EDGE_CURVE('',#24244,#24244,#20371,.T.);
#29926=EDGE_CURVE('',#24245,#24245,#20372,.T.);
#29927=EDGE_CURVE('',#24245,#24246,#5962,.T.);
#29928=EDGE_CURVE('',#24246,#24246,#20373,.T.);
#29929=EDGE_CURVE('',#24247,#24247,#20374,.T.);
#29930=EDGE_CURVE('',#24247,#24248,#5963,.T.);
#29931=EDGE_CURVE('',#24248,#24248,#20375,.T.);
#29932=EDGE_CURVE('',#24249,#24249,#20376,.T.);
#29933=EDGE_CURVE('',#24249,#24250,#5964,.T.);
#29934=EDGE_CURVE('',#24250,#24250,#20377,.T.);
#29935=EDGE_CURVE('',#24251,#24251,#20378,.T.);
#29936=EDGE_CURVE('',#24251,#24252,#5965,.T.);
#29937=EDGE_CURVE('',#24252,#24252,#20379,.T.);
#29938=EDGE_CURVE('',#24253,#24253,#20380,.T.);
#29939=EDGE_CURVE('',#24253,#24254,#5966,.T.);
#29940=EDGE_CURVE('',#24254,#24254,#20381,.T.);
#29941=EDGE_CURVE('',#24255,#24255,#20382,.T.);
#29942=EDGE_CURVE('',#24255,#24256,#5967,.T.);
#29943=EDGE_CURVE('',#24256,#24256,#20383,.T.);
#29944=EDGE_CURVE('',#24257,#24257,#20384,.T.);
#29945=EDGE_CURVE('',#24257,#24258,#5968,.T.);
#29946=EDGE_CURVE('',#24258,#24258,#20385,.T.);
#29947=EDGE_CURVE('',#24259,#24259,#20386,.T.);
#29948=EDGE_CURVE('',#24259,#24260,#5969,.T.);
#29949=EDGE_CURVE('',#24260,#24260,#20387,.T.);
#29950=EDGE_CURVE('',#24261,#24261,#20388,.T.);
#29951=EDGE_CURVE('',#24261,#24262,#5970,.T.);
#29952=EDGE_CURVE('',#24262,#24262,#20389,.T.);
#29953=EDGE_CURVE('',#24263,#24263,#20390,.T.);
#29954=EDGE_CURVE('',#24263,#24264,#5971,.T.);
#29955=EDGE_CURVE('',#24264,#24264,#20391,.T.);
#29956=EDGE_CURVE('',#24265,#24265,#20392,.T.);
#29957=EDGE_CURVE('',#24265,#24266,#5972,.T.);
#29958=EDGE_CURVE('',#24266,#24266,#20393,.T.);
#29959=EDGE_CURVE('',#24267,#24267,#20394,.T.);
#29960=EDGE_CURVE('',#24267,#24268,#5973,.T.);
#29961=EDGE_CURVE('',#24268,#24268,#20395,.T.);
#29962=EDGE_CURVE('',#24269,#24269,#20396,.T.);
#29963=EDGE_CURVE('',#24269,#24270,#5974,.T.);
#29964=EDGE_CURVE('',#24270,#24270,#20397,.T.);
#29965=EDGE_CURVE('',#24271,#24271,#20398,.T.);
#29966=EDGE_CURVE('',#24271,#24272,#5975,.T.);
#29967=EDGE_CURVE('',#24272,#24272,#20399,.T.);
#29968=EDGE_CURVE('',#24273,#24273,#20400,.T.);
#29969=EDGE_CURVE('',#24273,#24274,#5976,.T.);
#29970=EDGE_CURVE('',#24274,#24274,#20401,.T.);
#29971=EDGE_CURVE('',#24275,#24275,#20402,.T.);
#29972=EDGE_CURVE('',#24275,#24276,#5977,.T.);
#29973=EDGE_CURVE('',#24276,#24276,#20403,.T.);
#29974=EDGE_CURVE('',#24277,#24277,#20404,.T.);
#29975=EDGE_CURVE('',#24277,#24278,#5978,.T.);
#29976=EDGE_CURVE('',#24278,#24278,#20405,.T.);
#29977=EDGE_CURVE('',#24279,#24279,#20406,.T.);
#29978=EDGE_CURVE('',#24279,#24280,#5979,.T.);
#29979=EDGE_CURVE('',#24280,#24280,#20407,.T.);
#29980=EDGE_CURVE('',#24281,#24281,#20408,.T.);
#29981=EDGE_CURVE('',#24281,#24282,#5980,.T.);
#29982=EDGE_CURVE('',#24282,#24282,#20409,.T.);
#29983=EDGE_CURVE('',#24283,#24283,#20410,.T.);
#29984=EDGE_CURVE('',#24283,#24284,#5981,.T.);
#29985=EDGE_CURVE('',#24284,#24284,#20411,.T.);
#29986=EDGE_CURVE('',#24285,#24285,#20412,.T.);
#29987=EDGE_CURVE('',#24285,#24286,#5982,.T.);
#29988=EDGE_CURVE('',#24286,#24286,#20413,.T.);
#29989=EDGE_CURVE('',#24287,#24287,#20414,.T.);
#29990=EDGE_CURVE('',#24287,#24288,#5983,.T.);
#29991=EDGE_CURVE('',#24288,#24288,#20415,.T.);
#29992=EDGE_CURVE('',#24289,#24289,#20416,.T.);
#29993=EDGE_CURVE('',#24289,#24290,#5984,.T.);
#29994=EDGE_CURVE('',#24290,#24290,#20417,.T.);
#29995=EDGE_CURVE('',#24291,#24291,#20418,.T.);
#29996=EDGE_CURVE('',#24291,#24292,#5985,.T.);
#29997=EDGE_CURVE('',#24292,#24292,#20419,.T.);
#29998=EDGE_CURVE('',#24293,#24293,#20420,.T.);
#29999=EDGE_CURVE('',#24293,#24294,#5986,.T.);
#30000=EDGE_CURVE('',#24294,#24294,#20421,.T.);
#30001=EDGE_CURVE('',#24295,#24295,#20422,.T.);
#30002=EDGE_CURVE('',#24295,#24296,#5987,.T.);
#30003=EDGE_CURVE('',#24296,#24296,#20423,.T.);
#30004=EDGE_CURVE('',#24297,#24297,#20424,.T.);
#30005=EDGE_CURVE('',#24297,#24298,#5988,.T.);
#30006=EDGE_CURVE('',#24298,#24298,#20425,.T.);
#30007=EDGE_CURVE('',#24299,#24299,#20426,.T.);
#30008=EDGE_CURVE('',#24299,#24300,#5989,.T.);
#30009=EDGE_CURVE('',#24300,#24300,#20427,.T.);
#30010=EDGE_CURVE('',#24301,#24301,#20428,.T.);
#30011=EDGE_CURVE('',#24301,#24302,#5990,.T.);
#30012=EDGE_CURVE('',#24302,#24302,#20429,.T.);
#30013=EDGE_CURVE('',#24303,#24303,#20430,.T.);
#30014=EDGE_CURVE('',#24303,#24304,#5991,.T.);
#30015=EDGE_CURVE('',#24304,#24304,#20431,.T.);
#30016=EDGE_CURVE('',#24305,#24305,#20432,.T.);
#30017=EDGE_CURVE('',#24305,#24306,#5992,.T.);
#30018=EDGE_CURVE('',#24306,#24306,#20433,.T.);
#30019=EDGE_CURVE('',#24307,#24307,#20434,.T.);
#30020=EDGE_CURVE('',#24307,#24308,#5993,.T.);
#30021=EDGE_CURVE('',#24308,#24308,#20435,.T.);
#30022=EDGE_CURVE('',#24309,#24309,#20436,.T.);
#30023=EDGE_CURVE('',#24309,#24310,#5994,.T.);
#30024=EDGE_CURVE('',#24310,#24310,#20437,.T.);
#30025=EDGE_CURVE('',#24311,#24311,#20438,.T.);
#30026=EDGE_CURVE('',#24311,#24312,#5995,.T.);
#30027=EDGE_CURVE('',#24312,#24312,#20439,.T.);
#30028=EDGE_CURVE('',#24313,#24313,#20440,.T.);
#30029=EDGE_CURVE('',#24313,#24314,#5996,.T.);
#30030=EDGE_CURVE('',#24314,#24314,#20441,.T.);
#30031=EDGE_CURVE('',#24315,#24315,#20442,.T.);
#30032=EDGE_CURVE('',#24315,#24316,#5997,.T.);
#30033=EDGE_CURVE('',#24316,#24316,#20443,.T.);
#30034=EDGE_CURVE('',#24317,#24317,#20444,.T.);
#30035=EDGE_CURVE('',#24317,#24318,#5998,.T.);
#30036=EDGE_CURVE('',#24318,#24318,#20445,.T.);
#30037=EDGE_CURVE('',#24319,#24319,#20446,.T.);
#30038=EDGE_CURVE('',#24319,#24320,#5999,.T.);
#30039=EDGE_CURVE('',#24320,#24320,#20447,.T.);
#30040=EDGE_CURVE('',#24321,#24321,#20448,.T.);
#30041=EDGE_CURVE('',#24321,#24322,#6000,.T.);
#30042=EDGE_CURVE('',#24322,#24322,#20449,.T.);
#30043=EDGE_CURVE('',#24323,#24323,#20450,.T.);
#30044=EDGE_CURVE('',#24323,#24324,#6001,.T.);
#30045=EDGE_CURVE('',#24324,#24324,#20451,.T.);
#30046=EDGE_CURVE('',#24325,#24325,#20452,.T.);
#30047=EDGE_CURVE('',#24325,#24326,#6002,.T.);
#30048=EDGE_CURVE('',#24326,#24326,#20453,.T.);
#30049=EDGE_CURVE('',#24327,#24327,#20454,.T.);
#30050=EDGE_CURVE('',#24327,#24328,#6003,.T.);
#30051=EDGE_CURVE('',#24328,#24328,#20455,.T.);
#30052=EDGE_CURVE('',#24329,#24329,#20456,.T.);
#30053=EDGE_CURVE('',#24329,#24330,#6004,.T.);
#30054=EDGE_CURVE('',#24330,#24330,#20457,.T.);
#30055=EDGE_CURVE('',#24331,#24331,#20458,.T.);
#30056=EDGE_CURVE('',#24331,#24332,#6005,.T.);
#30057=EDGE_CURVE('',#24332,#24332,#20459,.T.);
#30058=EDGE_CURVE('',#24333,#24333,#20460,.T.);
#30059=EDGE_CURVE('',#24333,#24334,#6006,.T.);
#30060=EDGE_CURVE('',#24334,#24334,#20461,.T.);
#30061=EDGE_CURVE('',#24335,#24335,#20462,.T.);
#30062=EDGE_CURVE('',#24335,#24336,#6007,.T.);
#30063=EDGE_CURVE('',#24336,#24336,#20463,.T.);
#30064=EDGE_CURVE('',#24337,#24337,#20464,.T.);
#30065=EDGE_CURVE('',#24337,#24338,#6008,.T.);
#30066=EDGE_CURVE('',#24338,#24338,#20465,.T.);
#30067=EDGE_CURVE('',#24339,#24339,#20466,.T.);
#30068=EDGE_CURVE('',#24339,#24340,#6009,.T.);
#30069=EDGE_CURVE('',#24340,#24340,#20467,.T.);
#30070=EDGE_CURVE('',#24341,#24341,#20468,.T.);
#30071=EDGE_CURVE('',#24341,#24342,#6010,.T.);
#30072=EDGE_CURVE('',#24342,#24342,#20469,.T.);
#30073=EDGE_CURVE('',#24343,#24343,#20470,.T.);
#30074=EDGE_CURVE('',#24343,#24344,#6011,.T.);
#30075=EDGE_CURVE('',#24344,#24344,#20471,.T.);
#30076=EDGE_CURVE('',#24345,#24345,#20472,.T.);
#30077=EDGE_CURVE('',#24345,#24346,#6012,.T.);
#30078=EDGE_CURVE('',#24346,#24346,#20473,.T.);
#30079=EDGE_CURVE('',#24347,#24347,#20474,.T.);
#30080=EDGE_CURVE('',#24347,#24348,#6013,.T.);
#30081=EDGE_CURVE('',#24348,#24348,#20475,.T.);
#30082=EDGE_CURVE('',#24349,#24349,#20476,.T.);
#30083=EDGE_CURVE('',#24349,#24350,#6014,.T.);
#30084=EDGE_CURVE('',#24350,#24350,#20477,.T.);
#30085=EDGE_CURVE('',#24351,#24351,#20478,.T.);
#30086=EDGE_CURVE('',#24351,#24352,#6015,.T.);
#30087=EDGE_CURVE('',#24352,#24352,#20479,.T.);
#30088=EDGE_CURVE('',#24353,#24353,#20480,.T.);
#30089=EDGE_CURVE('',#24353,#24354,#6016,.T.);
#30090=EDGE_CURVE('',#24354,#24354,#20481,.T.);
#30091=EDGE_CURVE('',#24355,#24355,#20482,.T.);
#30092=EDGE_CURVE('',#24355,#24356,#6017,.T.);
#30093=EDGE_CURVE('',#24356,#24356,#20483,.T.);
#30094=EDGE_CURVE('',#24357,#24357,#20484,.T.);
#30095=EDGE_CURVE('',#24357,#24358,#6018,.T.);
#30096=EDGE_CURVE('',#24358,#24358,#20485,.T.);
#30097=EDGE_CURVE('',#24359,#24359,#20486,.T.);
#30098=EDGE_CURVE('',#24359,#24360,#6019,.T.);
#30099=EDGE_CURVE('',#24360,#24360,#20487,.T.);
#30100=EDGE_CURVE('',#24361,#24361,#20488,.T.);
#30101=EDGE_CURVE('',#24361,#24362,#6020,.T.);
#30102=EDGE_CURVE('',#24362,#24362,#20489,.T.);
#30103=EDGE_CURVE('',#24363,#24363,#20490,.T.);
#30104=EDGE_CURVE('',#24363,#24364,#6021,.T.);
#30105=EDGE_CURVE('',#24364,#24364,#20491,.T.);
#30106=EDGE_CURVE('',#24365,#24365,#20492,.T.);
#30107=EDGE_CURVE('',#24365,#24366,#6022,.T.);
#30108=EDGE_CURVE('',#24366,#24366,#20493,.T.);
#30109=EDGE_CURVE('',#24367,#24367,#20494,.T.);
#30110=EDGE_CURVE('',#24367,#24368,#6023,.T.);
#30111=EDGE_CURVE('',#24368,#24368,#20495,.T.);
#30112=EDGE_CURVE('',#24369,#24369,#20496,.T.);
#30113=EDGE_CURVE('',#24369,#24370,#6024,.T.);
#30114=EDGE_CURVE('',#24370,#24370,#20497,.T.);
#30115=EDGE_CURVE('',#24371,#24371,#20498,.T.);
#30116=EDGE_CURVE('',#24371,#24372,#6025,.T.);
#30117=EDGE_CURVE('',#24372,#24372,#20499,.T.);
#30118=EDGE_CURVE('',#24373,#24373,#20500,.T.);
#30119=EDGE_CURVE('',#24373,#24374,#6026,.T.);
#30120=EDGE_CURVE('',#24374,#24374,#20501,.T.);
#30121=EDGE_CURVE('',#24375,#24375,#20502,.T.);
#30122=EDGE_CURVE('',#24375,#24376,#6027,.T.);
#30123=EDGE_CURVE('',#24376,#24376,#20503,.T.);
#30124=EDGE_CURVE('',#24377,#24377,#20504,.T.);
#30125=EDGE_CURVE('',#24377,#24378,#6028,.T.);
#30126=EDGE_CURVE('',#24378,#24378,#20505,.T.);
#30127=EDGE_CURVE('',#24379,#24379,#20506,.T.);
#30128=EDGE_CURVE('',#24379,#24380,#6029,.T.);
#30129=EDGE_CURVE('',#24380,#24380,#20507,.T.);
#30130=EDGE_CURVE('',#24381,#24381,#20508,.T.);
#30131=EDGE_CURVE('',#24381,#24382,#6030,.T.);
#30132=EDGE_CURVE('',#24382,#24382,#20509,.T.);
#30133=EDGE_CURVE('',#24383,#24383,#20510,.T.);
#30134=EDGE_CURVE('',#24383,#24384,#6031,.T.);
#30135=EDGE_CURVE('',#24384,#24384,#20511,.T.);
#30136=EDGE_CURVE('',#24385,#24385,#20512,.T.);
#30137=EDGE_CURVE('',#24385,#24386,#6032,.T.);
#30138=EDGE_CURVE('',#24386,#24386,#20513,.T.);
#30139=EDGE_CURVE('',#24387,#24387,#20514,.T.);
#30140=EDGE_CURVE('',#24387,#24388,#6033,.T.);
#30141=EDGE_CURVE('',#24388,#24388,#20515,.T.);
#30142=EDGE_CURVE('',#24389,#24389,#20516,.T.);
#30143=EDGE_CURVE('',#24389,#24390,#6034,.T.);
#30144=EDGE_CURVE('',#24390,#24390,#20517,.T.);
#30145=EDGE_CURVE('',#24391,#24391,#20518,.T.);
#30146=EDGE_CURVE('',#24391,#24392,#6035,.T.);
#30147=EDGE_CURVE('',#24392,#24392,#20519,.T.);
#30148=EDGE_CURVE('',#24393,#24393,#20520,.T.);
#30149=EDGE_CURVE('',#24393,#24394,#6036,.T.);
#30150=EDGE_CURVE('',#24394,#24394,#20521,.T.);
#30151=EDGE_CURVE('',#24395,#24395,#20522,.T.);
#30152=EDGE_CURVE('',#24395,#24396,#6037,.T.);
#30153=EDGE_CURVE('',#24396,#24396,#20523,.T.);
#30154=EDGE_CURVE('',#24397,#24397,#20524,.T.);
#30155=EDGE_CURVE('',#24397,#24398,#6038,.T.);
#30156=EDGE_CURVE('',#24398,#24398,#20525,.T.);
#30157=EDGE_CURVE('',#24399,#24399,#20526,.T.);
#30158=EDGE_CURVE('',#24399,#24400,#6039,.T.);
#30159=EDGE_CURVE('',#24400,#24400,#20527,.T.);
#30160=EDGE_CURVE('',#24401,#24401,#20528,.T.);
#30161=EDGE_CURVE('',#24401,#24402,#6040,.T.);
#30162=EDGE_CURVE('',#24402,#24402,#20529,.T.);
#30163=EDGE_CURVE('',#24403,#24403,#20530,.T.);
#30164=EDGE_CURVE('',#24403,#24404,#6041,.T.);
#30165=EDGE_CURVE('',#24404,#24404,#20531,.T.);
#30166=EDGE_CURVE('',#24405,#24405,#20532,.T.);
#30167=EDGE_CURVE('',#24405,#24406,#6042,.T.);
#30168=EDGE_CURVE('',#24406,#24406,#20533,.T.);
#30169=EDGE_CURVE('',#24407,#24407,#20534,.T.);
#30170=EDGE_CURVE('',#24407,#24408,#6043,.T.);
#30171=EDGE_CURVE('',#24408,#24408,#20535,.T.);
#30172=EDGE_CURVE('',#24409,#24409,#20536,.T.);
#30173=EDGE_CURVE('',#24409,#24410,#6044,.T.);
#30174=EDGE_CURVE('',#24410,#24410,#20537,.T.);
#30175=EDGE_CURVE('',#24411,#24411,#20538,.T.);
#30176=EDGE_CURVE('',#24411,#24412,#6045,.T.);
#30177=EDGE_CURVE('',#24412,#24412,#20539,.T.);
#30178=EDGE_CURVE('',#24413,#24413,#20540,.T.);
#30179=EDGE_CURVE('',#24413,#24414,#6046,.T.);
#30180=EDGE_CURVE('',#24414,#24414,#20541,.T.);
#30181=EDGE_CURVE('',#24415,#24415,#20542,.T.);
#30182=EDGE_CURVE('',#24415,#24416,#6047,.T.);
#30183=EDGE_CURVE('',#24416,#24416,#20543,.T.);
#30184=EDGE_CURVE('',#24417,#24417,#20544,.T.);
#30185=EDGE_CURVE('',#24417,#24418,#6048,.T.);
#30186=EDGE_CURVE('',#24418,#24418,#20545,.T.);
#30187=EDGE_CURVE('',#24419,#24419,#20546,.T.);
#30188=EDGE_CURVE('',#24419,#24420,#6049,.T.);
#30189=EDGE_CURVE('',#24420,#24420,#20547,.T.);
#30190=EDGE_CURVE('',#24421,#24421,#20548,.T.);
#30191=EDGE_CURVE('',#24421,#24422,#6050,.T.);
#30192=EDGE_CURVE('',#24422,#24422,#20549,.T.);
#30193=EDGE_CURVE('',#24423,#24423,#20550,.T.);
#30194=EDGE_CURVE('',#24423,#24424,#6051,.T.);
#30195=EDGE_CURVE('',#24424,#24424,#20551,.T.);
#30196=EDGE_CURVE('',#24425,#24425,#20552,.T.);
#30197=EDGE_CURVE('',#24425,#24426,#6052,.T.);
#30198=EDGE_CURVE('',#24426,#24426,#20553,.T.);
#30199=EDGE_CURVE('',#24427,#24427,#20554,.T.);
#30200=EDGE_CURVE('',#24427,#24428,#6053,.T.);
#30201=EDGE_CURVE('',#24428,#24428,#20555,.T.);
#30202=EDGE_CURVE('',#24429,#24429,#20556,.T.);
#30203=EDGE_CURVE('',#24429,#24430,#6054,.T.);
#30204=EDGE_CURVE('',#24430,#24430,#20557,.T.);
#30205=EDGE_CURVE('',#24431,#24431,#20558,.T.);
#30206=EDGE_CURVE('',#24431,#24432,#6055,.T.);
#30207=EDGE_CURVE('',#24432,#24432,#20559,.T.);
#30208=EDGE_CURVE('',#24433,#24433,#20560,.T.);
#30209=EDGE_CURVE('',#24433,#24434,#6056,.T.);
#30210=EDGE_CURVE('',#24434,#24434,#20561,.T.);
#30211=EDGE_CURVE('',#24435,#24435,#20562,.T.);
#30212=EDGE_CURVE('',#24435,#24436,#6057,.T.);
#30213=EDGE_CURVE('',#24436,#24436,#20563,.T.);
#30214=EDGE_CURVE('',#24437,#24437,#20564,.T.);
#30215=EDGE_CURVE('',#24437,#24438,#6058,.T.);
#30216=EDGE_CURVE('',#24438,#24438,#20565,.T.);
#30217=EDGE_CURVE('',#24439,#24439,#20566,.T.);
#30218=EDGE_CURVE('',#24439,#24440,#6059,.T.);
#30219=EDGE_CURVE('',#24440,#24440,#20567,.T.);
#30220=EDGE_CURVE('',#24441,#24441,#20568,.T.);
#30221=EDGE_CURVE('',#24441,#24442,#6060,.T.);
#30222=EDGE_CURVE('',#24442,#24442,#20569,.T.);
#30223=EDGE_CURVE('',#24443,#24443,#20570,.T.);
#30224=EDGE_CURVE('',#24443,#24444,#6061,.T.);
#30225=EDGE_CURVE('',#24444,#24444,#20571,.T.);
#30226=EDGE_CURVE('',#24445,#24445,#20572,.T.);
#30227=EDGE_CURVE('',#24445,#24446,#6062,.T.);
#30228=EDGE_CURVE('',#24446,#24446,#20573,.T.);
#30229=EDGE_CURVE('',#24447,#24447,#20574,.T.);
#30230=EDGE_CURVE('',#24447,#24448,#6063,.T.);
#30231=EDGE_CURVE('',#24448,#24448,#20575,.T.);
#30232=EDGE_CURVE('',#24449,#24449,#20576,.T.);
#30233=EDGE_CURVE('',#24449,#24450,#6064,.T.);
#30234=EDGE_CURVE('',#24450,#24450,#20577,.T.);
#30235=EDGE_CURVE('',#24451,#24451,#20578,.T.);
#30236=EDGE_CURVE('',#24451,#24452,#6065,.T.);
#30237=EDGE_CURVE('',#24452,#24452,#20579,.T.);
#30238=EDGE_CURVE('',#24453,#24453,#20580,.T.);
#30239=EDGE_CURVE('',#24453,#24454,#6066,.T.);
#30240=EDGE_CURVE('',#24454,#24454,#20581,.T.);
#30241=EDGE_CURVE('',#24455,#24455,#20582,.T.);
#30242=EDGE_CURVE('',#24455,#24456,#6067,.T.);
#30243=EDGE_CURVE('',#24456,#24456,#20583,.T.);
#30244=EDGE_CURVE('',#24457,#24457,#20584,.T.);
#30245=EDGE_CURVE('',#24457,#24458,#6068,.T.);
#30246=EDGE_CURVE('',#24458,#24458,#20585,.T.);
#30247=EDGE_CURVE('',#24459,#24459,#20586,.T.);
#30248=EDGE_CURVE('',#24459,#24460,#6069,.T.);
#30249=EDGE_CURVE('',#24460,#24460,#20587,.T.);
#30250=EDGE_CURVE('',#24461,#24461,#20588,.T.);
#30251=EDGE_CURVE('',#24461,#24462,#6070,.T.);
#30252=EDGE_CURVE('',#24462,#24462,#20589,.T.);
#30253=EDGE_CURVE('',#24463,#24463,#20590,.T.);
#30254=EDGE_CURVE('',#24463,#24464,#6071,.T.);
#30255=EDGE_CURVE('',#24464,#24464,#20591,.T.);
#30256=EDGE_CURVE('',#24465,#24465,#20592,.T.);
#30257=EDGE_CURVE('',#24465,#24466,#6072,.T.);
#30258=EDGE_CURVE('',#24466,#24466,#20593,.T.);
#30259=EDGE_CURVE('',#24467,#24467,#20594,.T.);
#30260=EDGE_CURVE('',#24467,#24468,#6073,.T.);
#30261=EDGE_CURVE('',#24468,#24468,#20595,.T.);
#30262=EDGE_CURVE('',#24469,#24469,#20596,.T.);
#30263=EDGE_CURVE('',#24469,#24470,#6074,.T.);
#30264=EDGE_CURVE('',#24470,#24470,#20597,.T.);
#30265=EDGE_CURVE('',#24471,#24471,#20598,.T.);
#30266=EDGE_CURVE('',#24471,#24472,#6075,.T.);
#30267=EDGE_CURVE('',#24472,#24472,#20599,.T.);
#30268=EDGE_CURVE('',#24473,#24473,#20600,.T.);
#30269=EDGE_CURVE('',#24473,#24474,#6076,.T.);
#30270=EDGE_CURVE('',#24474,#24474,#20601,.T.);
#30271=EDGE_CURVE('',#24475,#24475,#20602,.T.);
#30272=EDGE_CURVE('',#24475,#24476,#6077,.T.);
#30273=EDGE_CURVE('',#24476,#24476,#20603,.T.);
#30274=EDGE_CURVE('',#24477,#24477,#20604,.T.);
#30275=EDGE_CURVE('',#24477,#24478,#6078,.T.);
#30276=EDGE_CURVE('',#24478,#24478,#20605,.T.);
#30277=EDGE_CURVE('',#24479,#24479,#20606,.T.);
#30278=EDGE_CURVE('',#24479,#24480,#6079,.T.);
#30279=EDGE_CURVE('',#24480,#24480,#20607,.T.);
#30280=EDGE_CURVE('',#22736,#24481,#20608,.T.);
#30281=EDGE_CURVE('',#24481,#24481,#20609,.T.);
#30282=EDGE_CURVE('',#22737,#22736,#20610,.T.);
#30283=EDGE_CURVE('',#24481,#24482,#6080,.T.);
#30284=EDGE_CURVE('',#24482,#24482,#20611,.T.);
#30285=EDGE_CURVE('',#24483,#24483,#20612,.T.);
#30286=EDGE_CURVE('',#24483,#24484,#20613,.T.);
#30287=EDGE_CURVE('',#24485,#24484,#20614,.T.);
#30288=EDGE_CURVE('',#24484,#24485,#20615,.T.);
#30289=EDGE_CURVE('',#24486,#24486,#20616,.T.);
#30290=EDGE_CURVE('',#24486,#24487,#20617,.T.);
#30291=EDGE_CURVE('',#24487,#24487,#20618,.T.);
#30292=EDGE_CURVE('',#24487,#24485,#6081,.T.);
#30293=EDGE_CURVE('',#24488,#24488,#20619,.T.);
#30294=EDGE_CURVE('',#24489,#24489,#20620,.T.);
#30295=EDGE_CURVE('',#24489,#24490,#20621,.T.);
#30296=EDGE_CURVE('',#24490,#24490,#20622,.T.);
#30297=EDGE_CURVE('',#24491,#24491,#20623,.T.);
#30298=EDGE_CURVE('',#24491,#24492,#20624,.T.);
#30299=EDGE_CURVE('',#24492,#24492,#20625,.T.);
#30300=EDGE_CURVE('',#24482,#24493,#20626,.T.);
#30301=EDGE_CURVE('',#24493,#24493,#20627,.T.);
#30302=EDGE_CURVE('',#24494,#24494,#20628,.T.);
#30303=EDGE_CURVE('',#24494,#24489,#6082,.T.);
#30304=EDGE_CURVE('',#24495,#24496,#20629,.T.);
#30305=EDGE_CURVE('',#24496,#24495,#20630,.T.);
#30306=EDGE_CURVE('',#24496,#24497,#20631,.T.);
#30307=EDGE_CURVE('',#24497,#24497,#20632,.T.);
#30308=EDGE_CURVE('',#24495,#24491,#6083,.T.);
#30309=EDGE_CURVE('',#24498,#24499,#2905,.T.);
#30310=EDGE_CURVE('',#24499,#24500,#6084,.T.);
#30311=EDGE_CURVE('',#24500,#24500,#20633,.T.);
#30312=EDGE_CURVE('',#24499,#24498,#2906,.T.);
#30313=EDGE_CURVE('',#22771,#24501,#6085,.T.);
#30314=EDGE_CURVE('',#24501,#24501,#2907,.T.);
#30315=EDGE_CURVE('',#22735,#22734,#20634,.T.);
#36820=ORIENTED_EDGE('',*,*,#27754,.T.);
#36821=ORIENTED_EDGE('',*,*,#27755,.T.);
#36822=ORIENTED_EDGE('',*,*,#27756,.T.);
#36823=ORIENTED_EDGE('',*,*,#27757,.F.);
#36824=ORIENTED_EDGE('',*,*,#27758,.T.);
#36825=ORIENTED_EDGE('',*,*,#27759,.T.);
#36826=ORIENTED_EDGE('',*,*,#27760,.T.);
#36827=ORIENTED_EDGE('',*,*,#27761,.T.);
#36828=ORIENTED_EDGE('',*,*,#27762,.T.);
#36829=ORIENTED_EDGE('',*,*,#27763,.T.);
#36830=ORIENTED_EDGE('',*,*,#27764,.T.);
#36831=ORIENTED_EDGE('',*,*,#27765,.T.);
#36832=ORIENTED_EDGE('',*,*,#27766,.T.);
#36833=ORIENTED_EDGE('',*,*,#27767,.T.);
#36834=ORIENTED_EDGE('',*,*,#27768,.T.);
#36835=ORIENTED_EDGE('',*,*,#27769,.T.);
#36836=ORIENTED_EDGE('',*,*,#27770,.T.);
#36837=ORIENTED_EDGE('',*,*,#27771,.T.);
#36838=ORIENTED_EDGE('',*,*,#27772,.T.);
#36839=ORIENTED_EDGE('',*,*,#27773,.T.);
#36840=ORIENTED_EDGE('',*,*,#27774,.T.);
#36841=ORIENTED_EDGE('',*,*,#27775,.T.);
#36842=ORIENTED_EDGE('',*,*,#27776,.T.);
#36843=ORIENTED_EDGE('',*,*,#27777,.T.);
#36844=ORIENTED_EDGE('',*,*,#27778,.T.);
#36845=ORIENTED_EDGE('',*,*,#27779,.T.);
#36846=ORIENTED_EDGE('',*,*,#27780,.T.);
#36847=ORIENTED_EDGE('',*,*,#27781,.T.);
#36848=ORIENTED_EDGE('',*,*,#27782,.T.);
#36849=ORIENTED_EDGE('',*,*,#27783,.T.);
#36850=ORIENTED_EDGE('',*,*,#27784,.T.);
#36851=ORIENTED_EDGE('',*,*,#27785,.T.);
#36852=ORIENTED_EDGE('',*,*,#27786,.T.);
#36853=ORIENTED_EDGE('',*,*,#27787,.T.);
#36854=ORIENTED_EDGE('',*,*,#27788,.T.);
#36855=ORIENTED_EDGE('',*,*,#27789,.T.);
#36856=ORIENTED_EDGE('',*,*,#27790,.T.);
#36857=ORIENTED_EDGE('',*,*,#27791,.T.);
#36858=ORIENTED_EDGE('',*,*,#27792,.T.);
#36859=ORIENTED_EDGE('',*,*,#27793,.T.);
#36860=ORIENTED_EDGE('',*,*,#27794,.T.);
#36861=ORIENTED_EDGE('',*,*,#27795,.T.);
#36862=ORIENTED_EDGE('',*,*,#27796,.T.);
#36863=ORIENTED_EDGE('',*,*,#27797,.T.);
#36864=ORIENTED_EDGE('',*,*,#27798,.T.);
#36865=ORIENTED_EDGE('',*,*,#27799,.T.);
#36866=ORIENTED_EDGE('',*,*,#27800,.T.);
#36867=ORIENTED_EDGE('',*,*,#27801,.T.);
#36868=ORIENTED_EDGE('',*,*,#27802,.T.);
#36869=ORIENTED_EDGE('',*,*,#27803,.T.);
#36870=ORIENTED_EDGE('',*,*,#27804,.T.);
#36871=ORIENTED_EDGE('',*,*,#27805,.T.);
#36872=ORIENTED_EDGE('',*,*,#27806,.T.);
#36873=ORIENTED_EDGE('',*,*,#27807,.T.);
#36874=ORIENTED_EDGE('',*,*,#27808,.T.);
#36875=ORIENTED_EDGE('',*,*,#27809,.T.);
#36876=ORIENTED_EDGE('',*,*,#27810,.T.);
#36877=ORIENTED_EDGE('',*,*,#27811,.T.);
#36878=ORIENTED_EDGE('',*,*,#27812,.T.);
#36879=ORIENTED_EDGE('',*,*,#27813,.T.);
#36880=ORIENTED_EDGE('',*,*,#27814,.T.);
#36881=ORIENTED_EDGE('',*,*,#27815,.T.);
#36882=ORIENTED_EDGE('',*,*,#27816,.T.);
#36883=ORIENTED_EDGE('',*,*,#27817,.T.);
#36884=ORIENTED_EDGE('',*,*,#27818,.T.);
#36885=ORIENTED_EDGE('',*,*,#27819,.T.);
#36886=ORIENTED_EDGE('',*,*,#27820,.T.);
#36887=ORIENTED_EDGE('',*,*,#27821,.T.);
#36888=ORIENTED_EDGE('',*,*,#27822,.T.);
#36889=ORIENTED_EDGE('',*,*,#27823,.T.);
#36890=ORIENTED_EDGE('',*,*,#27824,.T.);
#36891=ORIENTED_EDGE('',*,*,#27825,.T.);
#36892=ORIENTED_EDGE('',*,*,#27826,.T.);
#36893=ORIENTED_EDGE('',*,*,#27827,.T.);
#36894=ORIENTED_EDGE('',*,*,#27828,.T.);
#36895=ORIENTED_EDGE('',*,*,#27829,.T.);
#36896=ORIENTED_EDGE('',*,*,#27830,.T.);
#36897=ORIENTED_EDGE('',*,*,#27831,.T.);
#36898=ORIENTED_EDGE('',*,*,#27832,.T.);
#36899=ORIENTED_EDGE('',*,*,#27833,.T.);
#36900=ORIENTED_EDGE('',*,*,#27834,.T.);
#36901=ORIENTED_EDGE('',*,*,#27835,.T.);
#36902=ORIENTED_EDGE('',*,*,#27836,.T.);
#36903=ORIENTED_EDGE('',*,*,#27837,.T.);
#36904=ORIENTED_EDGE('',*,*,#27838,.T.);
#36905=ORIENTED_EDGE('',*,*,#27839,.T.);
#36906=ORIENTED_EDGE('',*,*,#27840,.T.);
#36907=ORIENTED_EDGE('',*,*,#27841,.T.);
#36908=ORIENTED_EDGE('',*,*,#27842,.T.);
#36909=ORIENTED_EDGE('',*,*,#27843,.T.);
#36910=ORIENTED_EDGE('',*,*,#27844,.T.);
#36911=ORIENTED_EDGE('',*,*,#27845,.T.);
#36912=ORIENTED_EDGE('',*,*,#27846,.T.);
#36913=ORIENTED_EDGE('',*,*,#27847,.T.);
#36914=ORIENTED_EDGE('',*,*,#27848,.T.);
#36915=ORIENTED_EDGE('',*,*,#27849,.T.);
#36916=ORIENTED_EDGE('',*,*,#27850,.T.);
#36917=ORIENTED_EDGE('',*,*,#27851,.T.);
#36918=ORIENTED_EDGE('',*,*,#27852,.T.);
#36919=ORIENTED_EDGE('',*,*,#27853,.T.);
#36920=ORIENTED_EDGE('',*,*,#27854,.T.);
#36921=ORIENTED_EDGE('',*,*,#27855,.T.);
#36922=ORIENTED_EDGE('',*,*,#27856,.T.);
#36923=ORIENTED_EDGE('',*,*,#27857,.T.);
#36924=ORIENTED_EDGE('',*,*,#27858,.T.);
#36925=ORIENTED_EDGE('',*,*,#27859,.T.);
#36926=ORIENTED_EDGE('',*,*,#27860,.T.);
#36927=ORIENTED_EDGE('',*,*,#27861,.T.);
#36928=ORIENTED_EDGE('',*,*,#27862,.T.);
#36929=ORIENTED_EDGE('',*,*,#27863,.T.);
#36930=ORIENTED_EDGE('',*,*,#27864,.T.);
#36931=ORIENTED_EDGE('',*,*,#27865,.T.);
#36932=ORIENTED_EDGE('',*,*,#27866,.T.);
#36933=ORIENTED_EDGE('',*,*,#27867,.T.);
#36934=ORIENTED_EDGE('',*,*,#27868,.T.);
#36935=ORIENTED_EDGE('',*,*,#27869,.T.);
#36936=ORIENTED_EDGE('',*,*,#27870,.T.);
#36937=ORIENTED_EDGE('',*,*,#27871,.T.);
#36938=ORIENTED_EDGE('',*,*,#27872,.T.);
#36939=ORIENTED_EDGE('',*,*,#27873,.T.);
#36940=ORIENTED_EDGE('',*,*,#27874,.T.);
#36941=ORIENTED_EDGE('',*,*,#27875,.T.);
#36942=ORIENTED_EDGE('',*,*,#27876,.T.);
#36943=ORIENTED_EDGE('',*,*,#27877,.T.);
#36944=ORIENTED_EDGE('',*,*,#27878,.F.);
#36945=ORIENTED_EDGE('',*,*,#27879,.T.);
#36946=ORIENTED_EDGE('',*,*,#27880,.F.);
#36947=ORIENTED_EDGE('',*,*,#27879,.F.);
#36948=ORIENTED_EDGE('',*,*,#27784,.F.);
#36949=ORIENTED_EDGE('',*,*,#27785,.F.);
#36950=ORIENTED_EDGE('',*,*,#27881,.T.);
#36951=ORIENTED_EDGE('',*,*,#27882,.F.);
#36952=ORIENTED_EDGE('',*,*,#27881,.F.);
#36953=ORIENTED_EDGE('',*,*,#27883,.T.);
#36954=ORIENTED_EDGE('',*,*,#27884,.T.);
#36955=ORIENTED_EDGE('',*,*,#27885,.F.);
#36956=ORIENTED_EDGE('',*,*,#27884,.F.);
#36957=ORIENTED_EDGE('',*,*,#27886,.T.);
#36958=ORIENTED_EDGE('',*,*,#27826,.F.);
#36959=ORIENTED_EDGE('',*,*,#27827,.F.);
#36960=ORIENTED_EDGE('',*,*,#27887,.T.);
#36961=ORIENTED_EDGE('',*,*,#27888,.F.);
#36962=ORIENTED_EDGE('',*,*,#27887,.F.);
#36963=ORIENTED_EDGE('',*,*,#27889,.T.);
#36964=ORIENTED_EDGE('',*,*,#27890,.T.);
#36965=ORIENTED_EDGE('',*,*,#27891,.F.);
#36966=ORIENTED_EDGE('',*,*,#27890,.F.);
#36967=ORIENTED_EDGE('',*,*,#27892,.T.);
#36968=ORIENTED_EDGE('',*,*,#27852,.F.);
#36969=ORIENTED_EDGE('',*,*,#27853,.F.);
#36970=ORIENTED_EDGE('',*,*,#27893,.T.);
#36971=ORIENTED_EDGE('',*,*,#27894,.F.);
#36972=ORIENTED_EDGE('',*,*,#27893,.F.);
#36973=ORIENTED_EDGE('',*,*,#27895,.T.);
#36974=ORIENTED_EDGE('',*,*,#27896,.T.);
#36975=ORIENTED_EDGE('',*,*,#27897,.F.);
#36976=ORIENTED_EDGE('',*,*,#27896,.F.);
#36977=ORIENTED_EDGE('',*,*,#27898,.T.);
#36978=ORIENTED_EDGE('',*,*,#27766,.F.);
#36979=ORIENTED_EDGE('',*,*,#27767,.F.);
#36980=ORIENTED_EDGE('',*,*,#27899,.T.);
#36981=ORIENTED_EDGE('',*,*,#27900,.F.);
#36982=ORIENTED_EDGE('',*,*,#27899,.F.);
#36983=ORIENTED_EDGE('',*,*,#27901,.T.);
#36984=ORIENTED_EDGE('',*,*,#27902,.T.);
#36985=ORIENTED_EDGE('',*,*,#27903,.F.);
#36986=ORIENTED_EDGE('',*,*,#27902,.F.);
#36987=ORIENTED_EDGE('',*,*,#27904,.T.);
#36988=ORIENTED_EDGE('',*,*,#27796,.F.);
#36989=ORIENTED_EDGE('',*,*,#27797,.F.);
#36990=ORIENTED_EDGE('',*,*,#27905,.T.);
#36991=ORIENTED_EDGE('',*,*,#27906,.F.);
#36992=ORIENTED_EDGE('',*,*,#27905,.F.);
#36993=ORIENTED_EDGE('',*,*,#27907,.T.);
#36994=ORIENTED_EDGE('',*,*,#27908,.T.);
#36995=ORIENTED_EDGE('',*,*,#27909,.F.);
#36996=ORIENTED_EDGE('',*,*,#27908,.F.);
#36997=ORIENTED_EDGE('',*,*,#27910,.T.);
#36998=ORIENTED_EDGE('',*,*,#27786,.F.);
#36999=ORIENTED_EDGE('',*,*,#27787,.F.);
#37000=ORIENTED_EDGE('',*,*,#27911,.T.);
#37001=ORIENTED_EDGE('',*,*,#27912,.F.);
#37002=ORIENTED_EDGE('',*,*,#27911,.F.);
#37003=ORIENTED_EDGE('',*,*,#27913,.T.);
#37004=ORIENTED_EDGE('',*,*,#27914,.T.);
#37005=ORIENTED_EDGE('',*,*,#27915,.F.);
#37006=ORIENTED_EDGE('',*,*,#27914,.F.);
#37007=ORIENTED_EDGE('',*,*,#27916,.T.);
#37008=ORIENTED_EDGE('',*,*,#27828,.F.);
#37009=ORIENTED_EDGE('',*,*,#27829,.F.);
#37010=ORIENTED_EDGE('',*,*,#27917,.T.);
#37011=ORIENTED_EDGE('',*,*,#27918,.F.);
#37012=ORIENTED_EDGE('',*,*,#27917,.F.);
#37013=ORIENTED_EDGE('',*,*,#27919,.T.);
#37014=ORIENTED_EDGE('',*,*,#27920,.T.);
#37015=ORIENTED_EDGE('',*,*,#27921,.F.);
#37016=ORIENTED_EDGE('',*,*,#27920,.F.);
#37017=ORIENTED_EDGE('',*,*,#27922,.T.);
#37018=ORIENTED_EDGE('',*,*,#27776,.F.);
#37019=ORIENTED_EDGE('',*,*,#27777,.F.);
#37020=ORIENTED_EDGE('',*,*,#27923,.T.);
#37021=ORIENTED_EDGE('',*,*,#27924,.F.);
#37022=ORIENTED_EDGE('',*,*,#27923,.F.);
#37023=ORIENTED_EDGE('',*,*,#27925,.T.);
#37024=ORIENTED_EDGE('',*,*,#27926,.T.);
#37025=ORIENTED_EDGE('',*,*,#27927,.F.);
#37026=ORIENTED_EDGE('',*,*,#27926,.F.);
#37027=ORIENTED_EDGE('',*,*,#27928,.T.);
#37028=ORIENTED_EDGE('',*,*,#27764,.F.);
#37029=ORIENTED_EDGE('',*,*,#27765,.F.);
#37030=ORIENTED_EDGE('',*,*,#27929,.T.);
#37031=ORIENTED_EDGE('',*,*,#27930,.F.);
#37032=ORIENTED_EDGE('',*,*,#27929,.F.);
#37033=ORIENTED_EDGE('',*,*,#27931,.T.);
#37034=ORIENTED_EDGE('',*,*,#27932,.T.);
#37035=ORIENTED_EDGE('',*,*,#27933,.F.);
#37036=ORIENTED_EDGE('',*,*,#27932,.F.);
#37037=ORIENTED_EDGE('',*,*,#27934,.T.);
#37038=ORIENTED_EDGE('',*,*,#27794,.F.);
#37039=ORIENTED_EDGE('',*,*,#27795,.F.);
#37040=ORIENTED_EDGE('',*,*,#27935,.T.);
#37041=ORIENTED_EDGE('',*,*,#27936,.F.);
#37042=ORIENTED_EDGE('',*,*,#27935,.F.);
#37043=ORIENTED_EDGE('',*,*,#27937,.T.);
#37044=ORIENTED_EDGE('',*,*,#27938,.T.);
#37045=ORIENTED_EDGE('',*,*,#27939,.F.);
#37046=ORIENTED_EDGE('',*,*,#27938,.F.);
#37047=ORIENTED_EDGE('',*,*,#27940,.T.);
#37048=ORIENTED_EDGE('',*,*,#27788,.F.);
#37049=ORIENTED_EDGE('',*,*,#27789,.F.);
#37050=ORIENTED_EDGE('',*,*,#27941,.T.);
#37051=ORIENTED_EDGE('',*,*,#27942,.F.);
#37052=ORIENTED_EDGE('',*,*,#27941,.F.);
#37053=ORIENTED_EDGE('',*,*,#27943,.T.);
#37054=ORIENTED_EDGE('',*,*,#27944,.T.);
#37055=ORIENTED_EDGE('',*,*,#27945,.F.);
#37056=ORIENTED_EDGE('',*,*,#27944,.F.);
#37057=ORIENTED_EDGE('',*,*,#27946,.T.);
#37058=ORIENTED_EDGE('',*,*,#27768,.F.);
#37059=ORIENTED_EDGE('',*,*,#27769,.F.);
#37060=ORIENTED_EDGE('',*,*,#27947,.T.);
#37061=ORIENTED_EDGE('',*,*,#27948,.F.);
#37062=ORIENTED_EDGE('',*,*,#27947,.F.);
#37063=ORIENTED_EDGE('',*,*,#27949,.T.);
#37064=ORIENTED_EDGE('',*,*,#27950,.T.);
#37065=ORIENTED_EDGE('',*,*,#27951,.F.);
#37066=ORIENTED_EDGE('',*,*,#27950,.F.);
#37067=ORIENTED_EDGE('',*,*,#27952,.T.);
#37068=ORIENTED_EDGE('',*,*,#27778,.F.);
#37069=ORIENTED_EDGE('',*,*,#27779,.F.);
#37070=ORIENTED_EDGE('',*,*,#27953,.T.);
#37071=ORIENTED_EDGE('',*,*,#27954,.F.);
#37072=ORIENTED_EDGE('',*,*,#27953,.F.);
#37073=ORIENTED_EDGE('',*,*,#27955,.T.);
#37074=ORIENTED_EDGE('',*,*,#27956,.T.);
#37075=ORIENTED_EDGE('',*,*,#27957,.F.);
#37076=ORIENTED_EDGE('',*,*,#27956,.F.);
#37077=ORIENTED_EDGE('',*,*,#27958,.T.);
#37078=ORIENTED_EDGE('',*,*,#27762,.F.);
#37079=ORIENTED_EDGE('',*,*,#27763,.F.);
#37080=ORIENTED_EDGE('',*,*,#27959,.T.);
#37081=ORIENTED_EDGE('',*,*,#27960,.F.);
#37082=ORIENTED_EDGE('',*,*,#27959,.F.);
#37083=ORIENTED_EDGE('',*,*,#27961,.T.);
#37084=ORIENTED_EDGE('',*,*,#27962,.T.);
#37085=ORIENTED_EDGE('',*,*,#27963,.F.);
#37086=ORIENTED_EDGE('',*,*,#27962,.F.);
#37087=ORIENTED_EDGE('',*,*,#27964,.T.);
#37088=ORIENTED_EDGE('',*,*,#27792,.F.);
#37089=ORIENTED_EDGE('',*,*,#27793,.F.);
#37090=ORIENTED_EDGE('',*,*,#27965,.T.);
#37091=ORIENTED_EDGE('',*,*,#27966,.F.);
#37092=ORIENTED_EDGE('',*,*,#27965,.F.);
#37093=ORIENTED_EDGE('',*,*,#27967,.T.);
#37094=ORIENTED_EDGE('',*,*,#27968,.T.);
#37095=ORIENTED_EDGE('',*,*,#27969,.F.);
#37096=ORIENTED_EDGE('',*,*,#27968,.F.);
#37097=ORIENTED_EDGE('',*,*,#27970,.T.);
#37098=ORIENTED_EDGE('',*,*,#27812,.F.);
#37099=ORIENTED_EDGE('',*,*,#27813,.F.);
#37100=ORIENTED_EDGE('',*,*,#27971,.T.);
#37101=ORIENTED_EDGE('',*,*,#27972,.F.);
#37102=ORIENTED_EDGE('',*,*,#27971,.F.);
#37103=ORIENTED_EDGE('',*,*,#27973,.T.);
#37104=ORIENTED_EDGE('',*,*,#27974,.T.);
#37105=ORIENTED_EDGE('',*,*,#27975,.F.);
#37106=ORIENTED_EDGE('',*,*,#27974,.F.);
#37107=ORIENTED_EDGE('',*,*,#27976,.T.);
#37108=ORIENTED_EDGE('',*,*,#27770,.F.);
#37109=ORIENTED_EDGE('',*,*,#27771,.F.);
#37110=ORIENTED_EDGE('',*,*,#27977,.T.);
#37111=ORIENTED_EDGE('',*,*,#27978,.F.);
#37112=ORIENTED_EDGE('',*,*,#27977,.F.);
#37113=ORIENTED_EDGE('',*,*,#27979,.T.);
#37114=ORIENTED_EDGE('',*,*,#27980,.T.);
#37115=ORIENTED_EDGE('',*,*,#27981,.F.);
#37116=ORIENTED_EDGE('',*,*,#27980,.F.);
#37117=ORIENTED_EDGE('',*,*,#27982,.T.);
#37118=ORIENTED_EDGE('',*,*,#27780,.F.);
#37119=ORIENTED_EDGE('',*,*,#27781,.F.);
#37120=ORIENTED_EDGE('',*,*,#27983,.T.);
#37121=ORIENTED_EDGE('',*,*,#27984,.F.);
#37122=ORIENTED_EDGE('',*,*,#27983,.F.);
#37123=ORIENTED_EDGE('',*,*,#27985,.T.);
#37124=ORIENTED_EDGE('',*,*,#27986,.T.);
#37125=ORIENTED_EDGE('',*,*,#27987,.F.);
#37126=ORIENTED_EDGE('',*,*,#27986,.F.);
#37127=ORIENTED_EDGE('',*,*,#27988,.T.);
#37128=ORIENTED_EDGE('',*,*,#27760,.F.);
#37129=ORIENTED_EDGE('',*,*,#27761,.F.);
#37130=ORIENTED_EDGE('',*,*,#27989,.T.);
#37131=ORIENTED_EDGE('',*,*,#27990,.F.);
#37132=ORIENTED_EDGE('',*,*,#27989,.F.);
#37133=ORIENTED_EDGE('',*,*,#27991,.T.);
#37134=ORIENTED_EDGE('',*,*,#27992,.T.);
#37135=ORIENTED_EDGE('',*,*,#27993,.F.);
#37136=ORIENTED_EDGE('',*,*,#27992,.F.);
#37137=ORIENTED_EDGE('',*,*,#27994,.T.);
#37138=ORIENTED_EDGE('',*,*,#27814,.F.);
#37139=ORIENTED_EDGE('',*,*,#27815,.F.);
#37140=ORIENTED_EDGE('',*,*,#27995,.T.);
#37141=ORIENTED_EDGE('',*,*,#27996,.F.);
#37142=ORIENTED_EDGE('',*,*,#27995,.F.);
#37143=ORIENTED_EDGE('',*,*,#27997,.T.);
#37144=ORIENTED_EDGE('',*,*,#27998,.T.);
#37145=ORIENTED_EDGE('',*,*,#27999,.F.);
#37146=ORIENTED_EDGE('',*,*,#27998,.F.);
#37147=ORIENTED_EDGE('',*,*,#28000,.T.);
#37148=ORIENTED_EDGE('',*,*,#27810,.F.);
#37149=ORIENTED_EDGE('',*,*,#27811,.F.);
#37150=ORIENTED_EDGE('',*,*,#28001,.T.);
#37151=ORIENTED_EDGE('',*,*,#28002,.F.);
#37152=ORIENTED_EDGE('',*,*,#28001,.F.);
#37153=ORIENTED_EDGE('',*,*,#28003,.T.);
#37154=ORIENTED_EDGE('',*,*,#28004,.T.);
#37155=ORIENTED_EDGE('',*,*,#28005,.F.);
#37156=ORIENTED_EDGE('',*,*,#28004,.F.);
#37157=ORIENTED_EDGE('',*,*,#28006,.T.);
#37158=ORIENTED_EDGE('',*,*,#27772,.F.);
#37159=ORIENTED_EDGE('',*,*,#27773,.F.);
#37160=ORIENTED_EDGE('',*,*,#28007,.T.);
#37161=ORIENTED_EDGE('',*,*,#28008,.F.);
#37162=ORIENTED_EDGE('',*,*,#28007,.F.);
#37163=ORIENTED_EDGE('',*,*,#28009,.T.);
#37164=ORIENTED_EDGE('',*,*,#28010,.T.);
#37165=ORIENTED_EDGE('',*,*,#28011,.F.);
#37166=ORIENTED_EDGE('',*,*,#28010,.F.);
#37167=ORIENTED_EDGE('',*,*,#28012,.T.);
#37168=ORIENTED_EDGE('',*,*,#27758,.F.);
#37169=ORIENTED_EDGE('',*,*,#27759,.F.);
#37170=ORIENTED_EDGE('',*,*,#28013,.T.);
#37171=ORIENTED_EDGE('',*,*,#28014,.F.);
#37172=ORIENTED_EDGE('',*,*,#28013,.F.);
#37173=ORIENTED_EDGE('',*,*,#28015,.T.);
#37174=ORIENTED_EDGE('',*,*,#28016,.T.);
#37175=ORIENTED_EDGE('',*,*,#28017,.F.);
#37176=ORIENTED_EDGE('',*,*,#28016,.F.);
#37177=ORIENTED_EDGE('',*,*,#28018,.T.);
#37178=ORIENTED_EDGE('',*,*,#27802,.F.);
#37179=ORIENTED_EDGE('',*,*,#27803,.F.);
#37180=ORIENTED_EDGE('',*,*,#28019,.T.);
#37181=ORIENTED_EDGE('',*,*,#28020,.F.);
#37182=ORIENTED_EDGE('',*,*,#28019,.F.);
#37183=ORIENTED_EDGE('',*,*,#28021,.T.);
#37184=ORIENTED_EDGE('',*,*,#28022,.T.);
#37185=ORIENTED_EDGE('',*,*,#28023,.F.);
#37186=ORIENTED_EDGE('',*,*,#28022,.F.);
#37187=ORIENTED_EDGE('',*,*,#28024,.T.);
#37188=ORIENTED_EDGE('',*,*,#27816,.F.);
#37189=ORIENTED_EDGE('',*,*,#27817,.F.);
#37190=ORIENTED_EDGE('',*,*,#28025,.T.);
#37191=ORIENTED_EDGE('',*,*,#28026,.F.);
#37192=ORIENTED_EDGE('',*,*,#28025,.F.);
#37193=ORIENTED_EDGE('',*,*,#28027,.T.);
#37194=ORIENTED_EDGE('',*,*,#28028,.T.);
#37195=ORIENTED_EDGE('',*,*,#28029,.F.);
#37196=ORIENTED_EDGE('',*,*,#28028,.F.);
#37197=ORIENTED_EDGE('',*,*,#28030,.T.);
#37198=ORIENTED_EDGE('',*,*,#27808,.F.);
#37199=ORIENTED_EDGE('',*,*,#27809,.F.);
#37200=ORIENTED_EDGE('',*,*,#28031,.T.);
#37201=ORIENTED_EDGE('',*,*,#28032,.F.);
#37202=ORIENTED_EDGE('',*,*,#28031,.F.);
#37203=ORIENTED_EDGE('',*,*,#28033,.T.);
#37204=ORIENTED_EDGE('',*,*,#28034,.T.);
#37205=ORIENTED_EDGE('',*,*,#28035,.F.);
#37206=ORIENTED_EDGE('',*,*,#28034,.F.);
#37207=ORIENTED_EDGE('',*,*,#28036,.T.);
#37208=ORIENTED_EDGE('',*,*,#27774,.F.);
#37209=ORIENTED_EDGE('',*,*,#27775,.F.);
#37210=ORIENTED_EDGE('',*,*,#28037,.T.);
#37211=ORIENTED_EDGE('',*,*,#28038,.F.);
#37212=ORIENTED_EDGE('',*,*,#28037,.F.);
#37213=ORIENTED_EDGE('',*,*,#28039,.T.);
#37214=ORIENTED_EDGE('',*,*,#28040,.T.);
#37215=ORIENTED_EDGE('',*,*,#28041,.F.);
#37216=ORIENTED_EDGE('',*,*,#28040,.F.);
#37217=ORIENTED_EDGE('',*,*,#28042,.T.);
#37218=ORIENTED_EDGE('',*,*,#27804,.F.);
#37219=ORIENTED_EDGE('',*,*,#27805,.F.);
#37220=ORIENTED_EDGE('',*,*,#28043,.T.);
#37221=ORIENTED_EDGE('',*,*,#28044,.F.);
#37222=ORIENTED_EDGE('',*,*,#28045,.F.);
#37223=ORIENTED_EDGE('',*,*,#28043,.F.);
#37224=ORIENTED_EDGE('',*,*,#28046,.T.);
#37225=ORIENTED_EDGE('',*,*,#28047,.T.);
#37226=ORIENTED_EDGE('',*,*,#28048,.F.);
#37227=ORIENTED_EDGE('',*,*,#28047,.F.);
#37228=ORIENTED_EDGE('',*,*,#28049,.T.);
#37229=ORIENTED_EDGE('',*,*,#27800,.F.);
#37230=ORIENTED_EDGE('',*,*,#27801,.F.);
#37231=ORIENTED_EDGE('',*,*,#28050,.T.);
#37232=ORIENTED_EDGE('',*,*,#28051,.F.);
#37233=ORIENTED_EDGE('',*,*,#28050,.F.);
#37234=ORIENTED_EDGE('',*,*,#28052,.T.);
#37235=ORIENTED_EDGE('',*,*,#28053,.T.);
#37236=ORIENTED_EDGE('',*,*,#28054,.F.);
#37237=ORIENTED_EDGE('',*,*,#28053,.F.);
#37238=ORIENTED_EDGE('',*,*,#28055,.T.);
#37239=ORIENTED_EDGE('',*,*,#27818,.F.);
#37240=ORIENTED_EDGE('',*,*,#27819,.F.);
#37241=ORIENTED_EDGE('',*,*,#28056,.T.);
#37242=ORIENTED_EDGE('',*,*,#28057,.F.);
#37243=ORIENTED_EDGE('',*,*,#28056,.F.);
#37244=ORIENTED_EDGE('',*,*,#28058,.T.);
#37245=ORIENTED_EDGE('',*,*,#28059,.T.);
#37246=ORIENTED_EDGE('',*,*,#28060,.F.);
#37247=ORIENTED_EDGE('',*,*,#28059,.F.);
#37248=ORIENTED_EDGE('',*,*,#28061,.T.);
#37249=ORIENTED_EDGE('',*,*,#27806,.F.);
#37250=ORIENTED_EDGE('',*,*,#27807,.F.);
#37251=ORIENTED_EDGE('',*,*,#28062,.T.);
#37252=ORIENTED_EDGE('',*,*,#28063,.F.);
#37253=ORIENTED_EDGE('',*,*,#28062,.F.);
#37254=ORIENTED_EDGE('',*,*,#28064,.T.);
#37255=ORIENTED_EDGE('',*,*,#28065,.T.);
#37256=ORIENTED_EDGE('',*,*,#28066,.F.);
#37257=ORIENTED_EDGE('',*,*,#28065,.F.);
#37258=ORIENTED_EDGE('',*,*,#28067,.T.);
#37259=ORIENTED_EDGE('',*,*,#28068,.F.);
#37260=ORIENTED_EDGE('',*,*,#28069,.T.);
#37261=ORIENTED_EDGE('',*,*,#28070,.F.);
#37262=ORIENTED_EDGE('',*,*,#28069,.F.);
#37263=ORIENTED_EDGE('',*,*,#28071,.T.);
#37264=ORIENTED_EDGE('',*,*,#28072,.T.);
#37265=ORIENTED_EDGE('',*,*,#28073,.F.);
#37266=ORIENTED_EDGE('',*,*,#28072,.F.);
#37267=ORIENTED_EDGE('',*,*,#28074,.T.);
#37268=ORIENTED_EDGE('',*,*,#28075,.F.);
#37269=ORIENTED_EDGE('',*,*,#28076,.T.);
#37270=ORIENTED_EDGE('',*,*,#28077,.F.);
#37271=ORIENTED_EDGE('',*,*,#28076,.F.);
#37272=ORIENTED_EDGE('',*,*,#28078,.T.);
#37273=ORIENTED_EDGE('',*,*,#28079,.T.);
#37274=ORIENTED_EDGE('',*,*,#28080,.F.);
#37275=ORIENTED_EDGE('',*,*,#28079,.F.);
#37276=ORIENTED_EDGE('',*,*,#28081,.T.);
#37277=ORIENTED_EDGE('',*,*,#27798,.F.);
#37278=ORIENTED_EDGE('',*,*,#27799,.F.);
#37279=ORIENTED_EDGE('',*,*,#28082,.T.);
#37280=ORIENTED_EDGE('',*,*,#28083,.F.);
#37281=ORIENTED_EDGE('',*,*,#28082,.F.);
#37282=ORIENTED_EDGE('',*,*,#28084,.T.);
#37283=ORIENTED_EDGE('',*,*,#28085,.T.);
#37284=ORIENTED_EDGE('',*,*,#28086,.F.);
#37285=ORIENTED_EDGE('',*,*,#28085,.F.);
#37286=ORIENTED_EDGE('',*,*,#28087,.T.);
#37287=ORIENTED_EDGE('',*,*,#27820,.F.);
#37288=ORIENTED_EDGE('',*,*,#27821,.F.);
#37289=ORIENTED_EDGE('',*,*,#28088,.T.);
#37290=ORIENTED_EDGE('',*,*,#28089,.F.);
#37291=ORIENTED_EDGE('',*,*,#28088,.F.);
#37292=ORIENTED_EDGE('',*,*,#28090,.T.);
#37293=ORIENTED_EDGE('',*,*,#28091,.T.);
#37294=ORIENTED_EDGE('',*,*,#28092,.F.);
#37295=ORIENTED_EDGE('',*,*,#28091,.F.);
#37296=ORIENTED_EDGE('',*,*,#28093,.T.);
#37297=ORIENTED_EDGE('',*,*,#28094,.F.);
#37298=ORIENTED_EDGE('',*,*,#28095,.T.);
#37299=ORIENTED_EDGE('',*,*,#28096,.F.);
#37300=ORIENTED_EDGE('',*,*,#28095,.F.);
#37301=ORIENTED_EDGE('',*,*,#28097,.T.);
#37302=ORIENTED_EDGE('',*,*,#28098,.T.);
#37303=ORIENTED_EDGE('',*,*,#28099,.F.);
#37304=ORIENTED_EDGE('',*,*,#28098,.F.);
#37305=ORIENTED_EDGE('',*,*,#28100,.T.);
#37306=ORIENTED_EDGE('',*,*,#28101,.F.);
#37307=ORIENTED_EDGE('',*,*,#28102,.T.);
#37308=ORIENTED_EDGE('',*,*,#28103,.F.);
#37309=ORIENTED_EDGE('',*,*,#28102,.F.);
#37310=ORIENTED_EDGE('',*,*,#28104,.T.);
#37311=ORIENTED_EDGE('',*,*,#28105,.T.);
#37312=ORIENTED_EDGE('',*,*,#28106,.F.);
#37313=ORIENTED_EDGE('',*,*,#28105,.F.);
#37314=ORIENTED_EDGE('',*,*,#28107,.T.);
#37315=ORIENTED_EDGE('',*,*,#28108,.F.);
#37316=ORIENTED_EDGE('',*,*,#28109,.T.);
#37317=ORIENTED_EDGE('',*,*,#28110,.F.);
#37318=ORIENTED_EDGE('',*,*,#28109,.F.);
#37319=ORIENTED_EDGE('',*,*,#28111,.T.);
#37320=ORIENTED_EDGE('',*,*,#28112,.T.);
#37321=ORIENTED_EDGE('',*,*,#28113,.F.);
#37322=ORIENTED_EDGE('',*,*,#28112,.F.);
#37323=ORIENTED_EDGE('',*,*,#28114,.T.);
#37324=ORIENTED_EDGE('',*,*,#28115,.F.);
#37325=ORIENTED_EDGE('',*,*,#28116,.T.);
#37326=ORIENTED_EDGE('',*,*,#28117,.F.);
#37327=ORIENTED_EDGE('',*,*,#28116,.F.);
#37328=ORIENTED_EDGE('',*,*,#28118,.T.);
#37329=ORIENTED_EDGE('',*,*,#28119,.T.);
#37330=ORIENTED_EDGE('',*,*,#28120,.F.);
#37331=ORIENTED_EDGE('',*,*,#28119,.F.);
#37332=ORIENTED_EDGE('',*,*,#28121,.T.);
#37333=ORIENTED_EDGE('',*,*,#28122,.F.);
#37334=ORIENTED_EDGE('',*,*,#28123,.T.);
#37335=ORIENTED_EDGE('',*,*,#28124,.F.);
#37336=ORIENTED_EDGE('',*,*,#28123,.F.);
#37337=ORIENTED_EDGE('',*,*,#28125,.T.);
#37338=ORIENTED_EDGE('',*,*,#28126,.T.);
#37339=ORIENTED_EDGE('',*,*,#28127,.F.);
#37340=ORIENTED_EDGE('',*,*,#28126,.F.);
#37341=ORIENTED_EDGE('',*,*,#28128,.T.);
#37342=ORIENTED_EDGE('',*,*,#28129,.F.);
#37343=ORIENTED_EDGE('',*,*,#28130,.T.);
#37344=ORIENTED_EDGE('',*,*,#28131,.F.);
#37345=ORIENTED_EDGE('',*,*,#28130,.F.);
#37346=ORIENTED_EDGE('',*,*,#28132,.T.);
#37347=ORIENTED_EDGE('',*,*,#28133,.T.);
#37348=ORIENTED_EDGE('',*,*,#28134,.F.);
#37349=ORIENTED_EDGE('',*,*,#28133,.F.);
#37350=ORIENTED_EDGE('',*,*,#28135,.T.);
#37351=ORIENTED_EDGE('',*,*,#28136,.F.);
#37352=ORIENTED_EDGE('',*,*,#28137,.T.);
#37353=ORIENTED_EDGE('',*,*,#28138,.F.);
#37354=ORIENTED_EDGE('',*,*,#28137,.F.);
#37355=ORIENTED_EDGE('',*,*,#28139,.T.);
#37356=ORIENTED_EDGE('',*,*,#28140,.T.);
#37357=ORIENTED_EDGE('',*,*,#28141,.F.);
#37358=ORIENTED_EDGE('',*,*,#28140,.F.);
#37359=ORIENTED_EDGE('',*,*,#28142,.T.);
#37360=ORIENTED_EDGE('',*,*,#28143,.F.);
#37361=ORIENTED_EDGE('',*,*,#28144,.T.);
#37362=ORIENTED_EDGE('',*,*,#28145,.F.);
#37363=ORIENTED_EDGE('',*,*,#28144,.F.);
#37364=ORIENTED_EDGE('',*,*,#28146,.T.);
#37365=ORIENTED_EDGE('',*,*,#28147,.T.);
#37366=ORIENTED_EDGE('',*,*,#28148,.F.);
#37367=ORIENTED_EDGE('',*,*,#28147,.F.);
#37368=ORIENTED_EDGE('',*,*,#28149,.T.);
#37369=ORIENTED_EDGE('',*,*,#28150,.F.);
#37370=ORIENTED_EDGE('',*,*,#28151,.T.);
#37371=ORIENTED_EDGE('',*,*,#28152,.F.);
#37372=ORIENTED_EDGE('',*,*,#28151,.F.);
#37373=ORIENTED_EDGE('',*,*,#28153,.T.);
#37374=ORIENTED_EDGE('',*,*,#28154,.T.);
#37375=ORIENTED_EDGE('',*,*,#28155,.F.);
#37376=ORIENTED_EDGE('',*,*,#28154,.F.);
#37377=ORIENTED_EDGE('',*,*,#28156,.T.);
#37378=ORIENTED_EDGE('',*,*,#28157,.F.);
#37379=ORIENTED_EDGE('',*,*,#28158,.T.);
#37380=ORIENTED_EDGE('',*,*,#28159,.F.);
#37381=ORIENTED_EDGE('',*,*,#28158,.F.);
#37382=ORIENTED_EDGE('',*,*,#28160,.T.);
#37383=ORIENTED_EDGE('',*,*,#28161,.T.);
#37384=ORIENTED_EDGE('',*,*,#28162,.F.);
#37385=ORIENTED_EDGE('',*,*,#28161,.F.);
#37386=ORIENTED_EDGE('',*,*,#28163,.T.);
#37387=ORIENTED_EDGE('',*,*,#28164,.F.);
#37388=ORIENTED_EDGE('',*,*,#28165,.T.);
#37389=ORIENTED_EDGE('',*,*,#28166,.F.);
#37390=ORIENTED_EDGE('',*,*,#28165,.F.);
#37391=ORIENTED_EDGE('',*,*,#28167,.T.);
#37392=ORIENTED_EDGE('',*,*,#28168,.T.);
#37393=ORIENTED_EDGE('',*,*,#28169,.F.);
#37394=ORIENTED_EDGE('',*,*,#28168,.F.);
#37395=ORIENTED_EDGE('',*,*,#28170,.T.);
#37396=ORIENTED_EDGE('',*,*,#28171,.F.);
#37397=ORIENTED_EDGE('',*,*,#28172,.T.);
#37398=ORIENTED_EDGE('',*,*,#28173,.F.);
#37399=ORIENTED_EDGE('',*,*,#28172,.F.);
#37400=ORIENTED_EDGE('',*,*,#28174,.T.);
#37401=ORIENTED_EDGE('',*,*,#28175,.T.);
#37402=ORIENTED_EDGE('',*,*,#28176,.F.);
#37403=ORIENTED_EDGE('',*,*,#28175,.F.);
#37404=ORIENTED_EDGE('',*,*,#28177,.T.);
#37405=ORIENTED_EDGE('',*,*,#28178,.F.);
#37406=ORIENTED_EDGE('',*,*,#28179,.T.);
#37407=ORIENTED_EDGE('',*,*,#28180,.F.);
#37408=ORIENTED_EDGE('',*,*,#28179,.F.);
#37409=ORIENTED_EDGE('',*,*,#28181,.T.);
#37410=ORIENTED_EDGE('',*,*,#28182,.T.);
#37411=ORIENTED_EDGE('',*,*,#28183,.F.);
#37412=ORIENTED_EDGE('',*,*,#28182,.F.);
#37413=ORIENTED_EDGE('',*,*,#28184,.T.);
#37414=ORIENTED_EDGE('',*,*,#28185,.F.);
#37415=ORIENTED_EDGE('',*,*,#28186,.T.);
#37416=ORIENTED_EDGE('',*,*,#28187,.F.);
#37417=ORIENTED_EDGE('',*,*,#28186,.F.);
#37418=ORIENTED_EDGE('',*,*,#28188,.T.);
#37419=ORIENTED_EDGE('',*,*,#28189,.T.);
#37420=ORIENTED_EDGE('',*,*,#28190,.F.);
#37421=ORIENTED_EDGE('',*,*,#28189,.F.);
#37422=ORIENTED_EDGE('',*,*,#28191,.T.);
#37423=ORIENTED_EDGE('',*,*,#28192,.F.);
#37424=ORIENTED_EDGE('',*,*,#28193,.T.);
#37425=ORIENTED_EDGE('',*,*,#28194,.F.);
#37426=ORIENTED_EDGE('',*,*,#28193,.F.);
#37427=ORIENTED_EDGE('',*,*,#28195,.T.);
#37428=ORIENTED_EDGE('',*,*,#28196,.T.);
#37429=ORIENTED_EDGE('',*,*,#28197,.F.);
#37430=ORIENTED_EDGE('',*,*,#28196,.F.);
#37431=ORIENTED_EDGE('',*,*,#28198,.T.);
#37432=ORIENTED_EDGE('',*,*,#28199,.F.);
#37433=ORIENTED_EDGE('',*,*,#28200,.T.);
#37434=ORIENTED_EDGE('',*,*,#28201,.F.);
#37435=ORIENTED_EDGE('',*,*,#28200,.F.);
#37436=ORIENTED_EDGE('',*,*,#28202,.T.);
#37437=ORIENTED_EDGE('',*,*,#28203,.T.);
#37438=ORIENTED_EDGE('',*,*,#28204,.F.);
#37439=ORIENTED_EDGE('',*,*,#28203,.F.);
#37440=ORIENTED_EDGE('',*,*,#28205,.T.);
#37441=ORIENTED_EDGE('',*,*,#28206,.F.);
#37442=ORIENTED_EDGE('',*,*,#28207,.T.);
#37443=ORIENTED_EDGE('',*,*,#28208,.F.);
#37444=ORIENTED_EDGE('',*,*,#28207,.F.);
#37445=ORIENTED_EDGE('',*,*,#28209,.T.);
#37446=ORIENTED_EDGE('',*,*,#28210,.T.);
#37447=ORIENTED_EDGE('',*,*,#28211,.F.);
#37448=ORIENTED_EDGE('',*,*,#28210,.F.);
#37449=ORIENTED_EDGE('',*,*,#28212,.T.);
#37450=ORIENTED_EDGE('',*,*,#28213,.F.);
#37451=ORIENTED_EDGE('',*,*,#28214,.T.);
#37452=ORIENTED_EDGE('',*,*,#28215,.F.);
#37453=ORIENTED_EDGE('',*,*,#28214,.F.);
#37454=ORIENTED_EDGE('',*,*,#28216,.T.);
#37455=ORIENTED_EDGE('',*,*,#28217,.T.);
#37456=ORIENTED_EDGE('',*,*,#28218,.F.);
#37457=ORIENTED_EDGE('',*,*,#28217,.F.);
#37458=ORIENTED_EDGE('',*,*,#28219,.T.);
#37459=ORIENTED_EDGE('',*,*,#28220,.F.);
#37460=ORIENTED_EDGE('',*,*,#28221,.T.);
#37461=ORIENTED_EDGE('',*,*,#28222,.F.);
#37462=ORIENTED_EDGE('',*,*,#28221,.F.);
#37463=ORIENTED_EDGE('',*,*,#28223,.T.);
#37464=ORIENTED_EDGE('',*,*,#28224,.T.);
#37465=ORIENTED_EDGE('',*,*,#28225,.F.);
#37466=ORIENTED_EDGE('',*,*,#28224,.F.);
#37467=ORIENTED_EDGE('',*,*,#28226,.T.);
#37468=ORIENTED_EDGE('',*,*,#28227,.F.);
#37469=ORIENTED_EDGE('',*,*,#28228,.T.);
#37470=ORIENTED_EDGE('',*,*,#28229,.F.);
#37471=ORIENTED_EDGE('',*,*,#28228,.F.);
#37472=ORIENTED_EDGE('',*,*,#28230,.T.);
#37473=ORIENTED_EDGE('',*,*,#28231,.T.);
#37474=ORIENTED_EDGE('',*,*,#28232,.F.);
#37475=ORIENTED_EDGE('',*,*,#28231,.F.);
#37476=ORIENTED_EDGE('',*,*,#28233,.T.);
#37477=ORIENTED_EDGE('',*,*,#28234,.F.);
#37478=ORIENTED_EDGE('',*,*,#28235,.T.);
#37479=ORIENTED_EDGE('',*,*,#28236,.F.);
#37480=ORIENTED_EDGE('',*,*,#28235,.F.);
#37481=ORIENTED_EDGE('',*,*,#28237,.T.);
#37482=ORIENTED_EDGE('',*,*,#28238,.T.);
#37483=ORIENTED_EDGE('',*,*,#28239,.F.);
#37484=ORIENTED_EDGE('',*,*,#28238,.F.);
#37485=ORIENTED_EDGE('',*,*,#28240,.T.);
#37486=ORIENTED_EDGE('',*,*,#28241,.F.);
#37487=ORIENTED_EDGE('',*,*,#28242,.T.);
#37488=ORIENTED_EDGE('',*,*,#28243,.F.);
#37489=ORIENTED_EDGE('',*,*,#28242,.F.);
#37490=ORIENTED_EDGE('',*,*,#28244,.T.);
#37491=ORIENTED_EDGE('',*,*,#28245,.T.);
#37492=ORIENTED_EDGE('',*,*,#28246,.F.);
#37493=ORIENTED_EDGE('',*,*,#28245,.F.);
#37494=ORIENTED_EDGE('',*,*,#28247,.T.);
#37495=ORIENTED_EDGE('',*,*,#28248,.F.);
#37496=ORIENTED_EDGE('',*,*,#28249,.T.);
#37497=ORIENTED_EDGE('',*,*,#28250,.F.);
#37498=ORIENTED_EDGE('',*,*,#28249,.F.);
#37499=ORIENTED_EDGE('',*,*,#28251,.T.);
#37500=ORIENTED_EDGE('',*,*,#28252,.T.);
#37501=ORIENTED_EDGE('',*,*,#28253,.F.);
#37502=ORIENTED_EDGE('',*,*,#28252,.F.);
#37503=ORIENTED_EDGE('',*,*,#28254,.T.);
#37504=ORIENTED_EDGE('',*,*,#28255,.F.);
#37505=ORIENTED_EDGE('',*,*,#28256,.T.);
#37506=ORIENTED_EDGE('',*,*,#28257,.F.);
#37507=ORIENTED_EDGE('',*,*,#28256,.F.);
#37508=ORIENTED_EDGE('',*,*,#28258,.T.);
#37509=ORIENTED_EDGE('',*,*,#28259,.T.);
#37510=ORIENTED_EDGE('',*,*,#28260,.F.);
#37511=ORIENTED_EDGE('',*,*,#28259,.F.);
#37512=ORIENTED_EDGE('',*,*,#28261,.T.);
#37513=ORIENTED_EDGE('',*,*,#28262,.F.);
#37514=ORIENTED_EDGE('',*,*,#28263,.T.);
#37515=ORIENTED_EDGE('',*,*,#28264,.F.);
#37516=ORIENTED_EDGE('',*,*,#28263,.F.);
#37517=ORIENTED_EDGE('',*,*,#28265,.T.);
#37518=ORIENTED_EDGE('',*,*,#28266,.T.);
#37519=ORIENTED_EDGE('',*,*,#28267,.F.);
#37520=ORIENTED_EDGE('',*,*,#28266,.F.);
#37521=ORIENTED_EDGE('',*,*,#28268,.T.);
#37522=ORIENTED_EDGE('',*,*,#28269,.F.);
#37523=ORIENTED_EDGE('',*,*,#28270,.T.);
#37524=ORIENTED_EDGE('',*,*,#28271,.F.);
#37525=ORIENTED_EDGE('',*,*,#28270,.F.);
#37526=ORIENTED_EDGE('',*,*,#28272,.T.);
#37527=ORIENTED_EDGE('',*,*,#28273,.T.);
#37528=ORIENTED_EDGE('',*,*,#28274,.F.);
#37529=ORIENTED_EDGE('',*,*,#28273,.F.);
#37530=ORIENTED_EDGE('',*,*,#28275,.T.);
#37531=ORIENTED_EDGE('',*,*,#28276,.F.);
#37532=ORIENTED_EDGE('',*,*,#28277,.T.);
#37533=ORIENTED_EDGE('',*,*,#28278,.F.);
#37534=ORIENTED_EDGE('',*,*,#28277,.F.);
#37535=ORIENTED_EDGE('',*,*,#28279,.T.);
#37536=ORIENTED_EDGE('',*,*,#28280,.T.);
#37537=ORIENTED_EDGE('',*,*,#28281,.F.);
#37538=ORIENTED_EDGE('',*,*,#28280,.F.);
#37539=ORIENTED_EDGE('',*,*,#28282,.T.);
#37540=ORIENTED_EDGE('',*,*,#28283,.F.);
#37541=ORIENTED_EDGE('',*,*,#28284,.T.);
#37542=ORIENTED_EDGE('',*,*,#28285,.F.);
#37543=ORIENTED_EDGE('',*,*,#28284,.F.);
#37544=ORIENTED_EDGE('',*,*,#28286,.T.);
#37545=ORIENTED_EDGE('',*,*,#28287,.T.);
#37546=ORIENTED_EDGE('',*,*,#28288,.F.);
#37547=ORIENTED_EDGE('',*,*,#28287,.F.);
#37548=ORIENTED_EDGE('',*,*,#28289,.T.);
#37549=ORIENTED_EDGE('',*,*,#28290,.F.);
#37550=ORIENTED_EDGE('',*,*,#28291,.T.);
#37551=ORIENTED_EDGE('',*,*,#28292,.F.);
#37552=ORIENTED_EDGE('',*,*,#28293,.F.);
#37553=ORIENTED_EDGE('',*,*,#28291,.F.);
#37554=ORIENTED_EDGE('',*,*,#28294,.T.);
#37555=ORIENTED_EDGE('',*,*,#28295,.T.);
#37556=ORIENTED_EDGE('',*,*,#28296,.F.);
#37557=ORIENTED_EDGE('',*,*,#28295,.F.);
#37558=ORIENTED_EDGE('',*,*,#28297,.T.);
#37559=ORIENTED_EDGE('',*,*,#28298,.F.);
#37560=ORIENTED_EDGE('',*,*,#28299,.T.);
#37561=ORIENTED_EDGE('',*,*,#28300,.F.);
#37562=ORIENTED_EDGE('',*,*,#28299,.F.);
#37563=ORIENTED_EDGE('',*,*,#28301,.T.);
#37564=ORIENTED_EDGE('',*,*,#28302,.T.);
#37565=ORIENTED_EDGE('',*,*,#28303,.F.);
#37566=ORIENTED_EDGE('',*,*,#28302,.F.);
#37567=ORIENTED_EDGE('',*,*,#28304,.T.);
#37568=ORIENTED_EDGE('',*,*,#28305,.F.);
#37569=ORIENTED_EDGE('',*,*,#28306,.T.);
#37570=ORIENTED_EDGE('',*,*,#28307,.F.);
#37571=ORIENTED_EDGE('',*,*,#28306,.F.);
#37572=ORIENTED_EDGE('',*,*,#28308,.T.);
#37573=ORIENTED_EDGE('',*,*,#28309,.T.);
#37574=ORIENTED_EDGE('',*,*,#28310,.F.);
#37575=ORIENTED_EDGE('',*,*,#28309,.F.);
#37576=ORIENTED_EDGE('',*,*,#28311,.T.);
#37577=ORIENTED_EDGE('',*,*,#28312,.F.);
#37578=ORIENTED_EDGE('',*,*,#28313,.T.);
#37579=ORIENTED_EDGE('',*,*,#28314,.F.);
#37580=ORIENTED_EDGE('',*,*,#28313,.F.);
#37581=ORIENTED_EDGE('',*,*,#28315,.T.);
#37582=ORIENTED_EDGE('',*,*,#28316,.T.);
#37583=ORIENTED_EDGE('',*,*,#28317,.F.);
#37584=ORIENTED_EDGE('',*,*,#28316,.F.);
#37585=ORIENTED_EDGE('',*,*,#28318,.T.);
#37586=ORIENTED_EDGE('',*,*,#28319,.F.);
#37587=ORIENTED_EDGE('',*,*,#28320,.T.);
#37588=ORIENTED_EDGE('',*,*,#28321,.F.);
#37589=ORIENTED_EDGE('',*,*,#28322,.F.);
#37590=ORIENTED_EDGE('',*,*,#28320,.F.);
#37591=ORIENTED_EDGE('',*,*,#28323,.T.);
#37592=ORIENTED_EDGE('',*,*,#28324,.T.);
#37593=ORIENTED_EDGE('',*,*,#28325,.F.);
#37594=ORIENTED_EDGE('',*,*,#28324,.F.);
#37595=ORIENTED_EDGE('',*,*,#28326,.T.);
#37596=ORIENTED_EDGE('',*,*,#28327,.F.);
#37597=ORIENTED_EDGE('',*,*,#28328,.T.);
#37598=ORIENTED_EDGE('',*,*,#28329,.F.);
#37599=ORIENTED_EDGE('',*,*,#28328,.F.);
#37600=ORIENTED_EDGE('',*,*,#28330,.T.);
#37601=ORIENTED_EDGE('',*,*,#28331,.T.);
#37602=ORIENTED_EDGE('',*,*,#28332,.F.);
#37603=ORIENTED_EDGE('',*,*,#28331,.F.);
#37604=ORIENTED_EDGE('',*,*,#28333,.T.);
#37605=ORIENTED_EDGE('',*,*,#28334,.F.);
#37606=ORIENTED_EDGE('',*,*,#28335,.T.);
#37607=ORIENTED_EDGE('',*,*,#28336,.F.);
#37608=ORIENTED_EDGE('',*,*,#28335,.F.);
#37609=ORIENTED_EDGE('',*,*,#28337,.T.);
#37610=ORIENTED_EDGE('',*,*,#28338,.T.);
#37611=ORIENTED_EDGE('',*,*,#28339,.F.);
#37612=ORIENTED_EDGE('',*,*,#28338,.F.);
#37613=ORIENTED_EDGE('',*,*,#28340,.T.);
#37614=ORIENTED_EDGE('',*,*,#28341,.F.);
#37615=ORIENTED_EDGE('',*,*,#28342,.T.);
#37616=ORIENTED_EDGE('',*,*,#28343,.F.);
#37617=ORIENTED_EDGE('',*,*,#28342,.F.);
#37618=ORIENTED_EDGE('',*,*,#28344,.T.);
#37619=ORIENTED_EDGE('',*,*,#28345,.T.);
#37620=ORIENTED_EDGE('',*,*,#28346,.F.);
#37621=ORIENTED_EDGE('',*,*,#28345,.F.);
#37622=ORIENTED_EDGE('',*,*,#28347,.T.);
#37623=ORIENTED_EDGE('',*,*,#28348,.F.);
#37624=ORIENTED_EDGE('',*,*,#28349,.T.);
#37625=ORIENTED_EDGE('',*,*,#28350,.F.);
#37626=ORIENTED_EDGE('',*,*,#28351,.F.);
#37627=ORIENTED_EDGE('',*,*,#28349,.F.);
#37628=ORIENTED_EDGE('',*,*,#28352,.F.);
#37629=ORIENTED_EDGE('',*,*,#28353,.T.);
#37630=ORIENTED_EDGE('',*,*,#28354,.T.);
#37631=ORIENTED_EDGE('',*,*,#28355,.F.);
#37632=ORIENTED_EDGE('',*,*,#28354,.F.);
#37633=ORIENTED_EDGE('',*,*,#28356,.T.);
#37634=ORIENTED_EDGE('',*,*,#28357,.F.);
#37635=ORIENTED_EDGE('',*,*,#28358,.T.);
#37636=ORIENTED_EDGE('',*,*,#28359,.F.);
#37637=ORIENTED_EDGE('',*,*,#28358,.F.);
#37638=ORIENTED_EDGE('',*,*,#28360,.T.);
#37639=ORIENTED_EDGE('',*,*,#28361,.T.);
#37640=ORIENTED_EDGE('',*,*,#28362,.F.);
#37641=ORIENTED_EDGE('',*,*,#28361,.F.);
#37642=ORIENTED_EDGE('',*,*,#28363,.T.);
#37643=ORIENTED_EDGE('',*,*,#28364,.F.);
#37644=ORIENTED_EDGE('',*,*,#28365,.T.);
#37645=ORIENTED_EDGE('',*,*,#28366,.F.);
#37646=ORIENTED_EDGE('',*,*,#28365,.F.);
#37647=ORIENTED_EDGE('',*,*,#28367,.T.);
#37648=ORIENTED_EDGE('',*,*,#28368,.T.);
#37649=ORIENTED_EDGE('',*,*,#28369,.F.);
#37650=ORIENTED_EDGE('',*,*,#28368,.F.);
#37651=ORIENTED_EDGE('',*,*,#28370,.T.);
#37652=ORIENTED_EDGE('',*,*,#28371,.F.);
#37653=ORIENTED_EDGE('',*,*,#28372,.T.);
#37654=ORIENTED_EDGE('',*,*,#28373,.F.);
#37655=ORIENTED_EDGE('',*,*,#28372,.F.);
#37656=ORIENTED_EDGE('',*,*,#28374,.T.);
#37657=ORIENTED_EDGE('',*,*,#28375,.T.);
#37658=ORIENTED_EDGE('',*,*,#28376,.F.);
#37659=ORIENTED_EDGE('',*,*,#28375,.F.);
#37660=ORIENTED_EDGE('',*,*,#28377,.T.);
#37661=ORIENTED_EDGE('',*,*,#28378,.F.);
#37662=ORIENTED_EDGE('',*,*,#28379,.T.);
#37663=ORIENTED_EDGE('',*,*,#28380,.F.);
#37664=ORIENTED_EDGE('',*,*,#28379,.F.);
#37665=ORIENTED_EDGE('',*,*,#28381,.T.);
#37666=ORIENTED_EDGE('',*,*,#28382,.T.);
#37667=ORIENTED_EDGE('',*,*,#28383,.F.);
#37668=ORIENTED_EDGE('',*,*,#28382,.F.);
#37669=ORIENTED_EDGE('',*,*,#28384,.T.);
#37670=ORIENTED_EDGE('',*,*,#28385,.F.);
#37671=ORIENTED_EDGE('',*,*,#28386,.T.);
#37672=ORIENTED_EDGE('',*,*,#28387,.F.);
#37673=ORIENTED_EDGE('',*,*,#28386,.F.);
#37674=ORIENTED_EDGE('',*,*,#28388,.T.);
#37675=ORIENTED_EDGE('',*,*,#28389,.T.);
#37676=ORIENTED_EDGE('',*,*,#28390,.F.);
#37677=ORIENTED_EDGE('',*,*,#28389,.F.);
#37678=ORIENTED_EDGE('',*,*,#28391,.T.);
#37679=ORIENTED_EDGE('',*,*,#28392,.F.);
#37680=ORIENTED_EDGE('',*,*,#28393,.T.);
#37681=ORIENTED_EDGE('',*,*,#28394,.F.);
#37682=ORIENTED_EDGE('',*,*,#28393,.F.);
#37683=ORIENTED_EDGE('',*,*,#28395,.T.);
#37684=ORIENTED_EDGE('',*,*,#28396,.T.);
#37685=ORIENTED_EDGE('',*,*,#28397,.F.);
#37686=ORIENTED_EDGE('',*,*,#28396,.F.);
#37687=ORIENTED_EDGE('',*,*,#28398,.T.);
#37688=ORIENTED_EDGE('',*,*,#28399,.F.);
#37689=ORIENTED_EDGE('',*,*,#28400,.T.);
#37690=ORIENTED_EDGE('',*,*,#28401,.F.);
#37691=ORIENTED_EDGE('',*,*,#28400,.F.);
#37692=ORIENTED_EDGE('',*,*,#28402,.T.);
#37693=ORIENTED_EDGE('',*,*,#28403,.T.);
#37694=ORIENTED_EDGE('',*,*,#28404,.F.);
#37695=ORIENTED_EDGE('',*,*,#28403,.F.);
#37696=ORIENTED_EDGE('',*,*,#28405,.T.);
#37697=ORIENTED_EDGE('',*,*,#28406,.F.);
#37698=ORIENTED_EDGE('',*,*,#28407,.T.);
#37699=ORIENTED_EDGE('',*,*,#28408,.F.);
#37700=ORIENTED_EDGE('',*,*,#28407,.F.);
#37701=ORIENTED_EDGE('',*,*,#28409,.T.);
#37702=ORIENTED_EDGE('',*,*,#28410,.T.);
#37703=ORIENTED_EDGE('',*,*,#28411,.F.);
#37704=ORIENTED_EDGE('',*,*,#28410,.F.);
#37705=ORIENTED_EDGE('',*,*,#28412,.T.);
#37706=ORIENTED_EDGE('',*,*,#28413,.F.);
#37707=ORIENTED_EDGE('',*,*,#28414,.T.);
#37708=ORIENTED_EDGE('',*,*,#28415,.F.);
#37709=ORIENTED_EDGE('',*,*,#28414,.F.);
#37710=ORIENTED_EDGE('',*,*,#28416,.T.);
#37711=ORIENTED_EDGE('',*,*,#28417,.T.);
#37712=ORIENTED_EDGE('',*,*,#28418,.F.);
#37713=ORIENTED_EDGE('',*,*,#28417,.F.);
#37714=ORIENTED_EDGE('',*,*,#28419,.T.);
#37715=ORIENTED_EDGE('',*,*,#28420,.F.);
#37716=ORIENTED_EDGE('',*,*,#28421,.T.);
#37717=ORIENTED_EDGE('',*,*,#28422,.F.);
#37718=ORIENTED_EDGE('',*,*,#28421,.F.);
#37719=ORIENTED_EDGE('',*,*,#28423,.T.);
#37720=ORIENTED_EDGE('',*,*,#28424,.T.);
#37721=ORIENTED_EDGE('',*,*,#28425,.F.);
#37722=ORIENTED_EDGE('',*,*,#28424,.F.);
#37723=ORIENTED_EDGE('',*,*,#28426,.T.);
#37724=ORIENTED_EDGE('',*,*,#28427,.F.);
#37725=ORIENTED_EDGE('',*,*,#28428,.T.);
#37726=ORIENTED_EDGE('',*,*,#28429,.F.);
#37727=ORIENTED_EDGE('',*,*,#28428,.F.);
#37728=ORIENTED_EDGE('',*,*,#28430,.T.);
#37729=ORIENTED_EDGE('',*,*,#28431,.T.);
#37730=ORIENTED_EDGE('',*,*,#28432,.F.);
#37731=ORIENTED_EDGE('',*,*,#28431,.F.);
#37732=ORIENTED_EDGE('',*,*,#28433,.T.);
#37733=ORIENTED_EDGE('',*,*,#28434,.F.);
#37734=ORIENTED_EDGE('',*,*,#28435,.T.);
#37735=ORIENTED_EDGE('',*,*,#28436,.F.);
#37736=ORIENTED_EDGE('',*,*,#28435,.F.);
#37737=ORIENTED_EDGE('',*,*,#28437,.T.);
#37738=ORIENTED_EDGE('',*,*,#28438,.T.);
#37739=ORIENTED_EDGE('',*,*,#28439,.F.);
#37740=ORIENTED_EDGE('',*,*,#28438,.F.);
#37741=ORIENTED_EDGE('',*,*,#28440,.T.);
#37742=ORIENTED_EDGE('',*,*,#28441,.F.);
#37743=ORIENTED_EDGE('',*,*,#28442,.T.);
#37744=ORIENTED_EDGE('',*,*,#28443,.F.);
#37745=ORIENTED_EDGE('',*,*,#28442,.F.);
#37746=ORIENTED_EDGE('',*,*,#28444,.T.);
#37747=ORIENTED_EDGE('',*,*,#28445,.T.);
#37748=ORIENTED_EDGE('',*,*,#28446,.F.);
#37749=ORIENTED_EDGE('',*,*,#28445,.F.);
#37750=ORIENTED_EDGE('',*,*,#28447,.T.);
#37751=ORIENTED_EDGE('',*,*,#28448,.F.);
#37752=ORIENTED_EDGE('',*,*,#28449,.T.);
#37753=ORIENTED_EDGE('',*,*,#28450,.F.);
#37754=ORIENTED_EDGE('',*,*,#28449,.F.);
#37755=ORIENTED_EDGE('',*,*,#28451,.T.);
#37756=ORIENTED_EDGE('',*,*,#28452,.T.);
#37757=ORIENTED_EDGE('',*,*,#28453,.F.);
#37758=ORIENTED_EDGE('',*,*,#28452,.F.);
#37759=ORIENTED_EDGE('',*,*,#28454,.T.);
#37760=ORIENTED_EDGE('',*,*,#28455,.F.);
#37761=ORIENTED_EDGE('',*,*,#28456,.T.);
#37762=ORIENTED_EDGE('',*,*,#28457,.F.);
#37763=ORIENTED_EDGE('',*,*,#28456,.F.);
#37764=ORIENTED_EDGE('',*,*,#28458,.T.);
#37765=ORIENTED_EDGE('',*,*,#28459,.T.);
#37766=ORIENTED_EDGE('',*,*,#28460,.F.);
#37767=ORIENTED_EDGE('',*,*,#28459,.F.);
#37768=ORIENTED_EDGE('',*,*,#28461,.T.);
#37769=ORIENTED_EDGE('',*,*,#28462,.F.);
#37770=ORIENTED_EDGE('',*,*,#28463,.T.);
#37771=ORIENTED_EDGE('',*,*,#28464,.F.);
#37772=ORIENTED_EDGE('',*,*,#28463,.F.);
#37773=ORIENTED_EDGE('',*,*,#28465,.T.);
#37774=ORIENTED_EDGE('',*,*,#28466,.T.);
#37775=ORIENTED_EDGE('',*,*,#28467,.F.);
#37776=ORIENTED_EDGE('',*,*,#28466,.F.);
#37777=ORIENTED_EDGE('',*,*,#28468,.T.);
#37778=ORIENTED_EDGE('',*,*,#28469,.F.);
#37779=ORIENTED_EDGE('',*,*,#28470,.T.);
#37780=ORIENTED_EDGE('',*,*,#28471,.F.);
#37781=ORIENTED_EDGE('',*,*,#28470,.F.);
#37782=ORIENTED_EDGE('',*,*,#28472,.T.);
#37783=ORIENTED_EDGE('',*,*,#28473,.T.);
#37784=ORIENTED_EDGE('',*,*,#28474,.F.);
#37785=ORIENTED_EDGE('',*,*,#28473,.F.);
#37786=ORIENTED_EDGE('',*,*,#28475,.T.);
#37787=ORIENTED_EDGE('',*,*,#28476,.F.);
#37788=ORIENTED_EDGE('',*,*,#28477,.T.);
#37789=ORIENTED_EDGE('',*,*,#28478,.F.);
#37790=ORIENTED_EDGE('',*,*,#28477,.F.);
#37791=ORIENTED_EDGE('',*,*,#28479,.T.);
#37792=ORIENTED_EDGE('',*,*,#28480,.T.);
#37793=ORIENTED_EDGE('',*,*,#28481,.F.);
#37794=ORIENTED_EDGE('',*,*,#28480,.F.);
#37795=ORIENTED_EDGE('',*,*,#28482,.T.);
#37796=ORIENTED_EDGE('',*,*,#28483,.F.);
#37797=ORIENTED_EDGE('',*,*,#28484,.T.);
#37798=ORIENTED_EDGE('',*,*,#28485,.F.);
#37799=ORIENTED_EDGE('',*,*,#28484,.F.);
#37800=ORIENTED_EDGE('',*,*,#28486,.T.);
#37801=ORIENTED_EDGE('',*,*,#28487,.T.);
#37802=ORIENTED_EDGE('',*,*,#28488,.F.);
#37803=ORIENTED_EDGE('',*,*,#28487,.F.);
#37804=ORIENTED_EDGE('',*,*,#28489,.T.);
#37805=ORIENTED_EDGE('',*,*,#27860,.F.);
#37806=ORIENTED_EDGE('',*,*,#27861,.F.);
#37807=ORIENTED_EDGE('',*,*,#28490,.T.);
#37808=ORIENTED_EDGE('',*,*,#28491,.F.);
#37809=ORIENTED_EDGE('',*,*,#28490,.F.);
#37810=ORIENTED_EDGE('',*,*,#28492,.T.);
#37811=ORIENTED_EDGE('',*,*,#28493,.T.);
#37812=ORIENTED_EDGE('',*,*,#28494,.F.);
#37813=ORIENTED_EDGE('',*,*,#28493,.F.);
#37814=ORIENTED_EDGE('',*,*,#28495,.T.);
#37815=ORIENTED_EDGE('',*,*,#27836,.F.);
#37816=ORIENTED_EDGE('',*,*,#27837,.F.);
#37817=ORIENTED_EDGE('',*,*,#28496,.T.);
#37818=ORIENTED_EDGE('',*,*,#28497,.F.);
#37819=ORIENTED_EDGE('',*,*,#28496,.F.);
#37820=ORIENTED_EDGE('',*,*,#28498,.T.);
#37821=ORIENTED_EDGE('',*,*,#28499,.T.);
#37822=ORIENTED_EDGE('',*,*,#28500,.F.);
#37823=ORIENTED_EDGE('',*,*,#28499,.F.);
#37824=ORIENTED_EDGE('',*,*,#28501,.T.);
#37825=ORIENTED_EDGE('',*,*,#28502,.F.);
#37826=ORIENTED_EDGE('',*,*,#28503,.T.);
#37827=ORIENTED_EDGE('',*,*,#28504,.F.);
#37828=ORIENTED_EDGE('',*,*,#28503,.F.);
#37829=ORIENTED_EDGE('',*,*,#28505,.T.);
#37830=ORIENTED_EDGE('',*,*,#28506,.T.);
#37831=ORIENTED_EDGE('',*,*,#28507,.F.);
#37832=ORIENTED_EDGE('',*,*,#28506,.F.);
#37833=ORIENTED_EDGE('',*,*,#28508,.T.);
#37834=ORIENTED_EDGE('',*,*,#28509,.F.);
#37835=ORIENTED_EDGE('',*,*,#28510,.T.);
#37836=ORIENTED_EDGE('',*,*,#28511,.F.);
#37837=ORIENTED_EDGE('',*,*,#28510,.F.);
#37838=ORIENTED_EDGE('',*,*,#28512,.T.);
#37839=ORIENTED_EDGE('',*,*,#28513,.T.);
#37840=ORIENTED_EDGE('',*,*,#28514,.F.);
#37841=ORIENTED_EDGE('',*,*,#28513,.F.);
#37842=ORIENTED_EDGE('',*,*,#28515,.T.);
#37843=ORIENTED_EDGE('',*,*,#27876,.F.);
#37844=ORIENTED_EDGE('',*,*,#27877,.F.);
#37845=ORIENTED_EDGE('',*,*,#28516,.T.);
#37846=ORIENTED_EDGE('',*,*,#28517,.F.);
#37847=ORIENTED_EDGE('',*,*,#28516,.F.);
#37848=ORIENTED_EDGE('',*,*,#28518,.T.);
#37849=ORIENTED_EDGE('',*,*,#28519,.T.);
#37850=ORIENTED_EDGE('',*,*,#28520,.F.);
#37851=ORIENTED_EDGE('',*,*,#28519,.F.);
#37852=ORIENTED_EDGE('',*,*,#28521,.T.);
#37853=ORIENTED_EDGE('',*,*,#27862,.F.);
#37854=ORIENTED_EDGE('',*,*,#27863,.F.);
#37855=ORIENTED_EDGE('',*,*,#28522,.T.);
#37856=ORIENTED_EDGE('',*,*,#28523,.F.);
#37857=ORIENTED_EDGE('',*,*,#28522,.F.);
#37858=ORIENTED_EDGE('',*,*,#28524,.T.);
#37859=ORIENTED_EDGE('',*,*,#28525,.T.);
#37860=ORIENTED_EDGE('',*,*,#28526,.F.);
#37861=ORIENTED_EDGE('',*,*,#28525,.F.);
#37862=ORIENTED_EDGE('',*,*,#28527,.T.);
#37863=ORIENTED_EDGE('',*,*,#27834,.F.);
#37864=ORIENTED_EDGE('',*,*,#27835,.F.);
#37865=ORIENTED_EDGE('',*,*,#28528,.T.);
#37866=ORIENTED_EDGE('',*,*,#28529,.F.);
#37867=ORIENTED_EDGE('',*,*,#28528,.F.);
#37868=ORIENTED_EDGE('',*,*,#28530,.T.);
#37869=ORIENTED_EDGE('',*,*,#28531,.T.);
#37870=ORIENTED_EDGE('',*,*,#28532,.F.);
#37871=ORIENTED_EDGE('',*,*,#28531,.F.);
#37872=ORIENTED_EDGE('',*,*,#28533,.T.);
#37873=ORIENTED_EDGE('',*,*,#27830,.F.);
#37874=ORIENTED_EDGE('',*,*,#27831,.F.);
#37875=ORIENTED_EDGE('',*,*,#28534,.T.);
#37876=ORIENTED_EDGE('',*,*,#28535,.F.);
#37877=ORIENTED_EDGE('',*,*,#28534,.F.);
#37878=ORIENTED_EDGE('',*,*,#28536,.T.);
#37879=ORIENTED_EDGE('',*,*,#28537,.T.);
#37880=ORIENTED_EDGE('',*,*,#28538,.F.);
#37881=ORIENTED_EDGE('',*,*,#28537,.F.);
#37882=ORIENTED_EDGE('',*,*,#28539,.T.);
#37883=ORIENTED_EDGE('',*,*,#27874,.F.);
#37884=ORIENTED_EDGE('',*,*,#27875,.F.);
#37885=ORIENTED_EDGE('',*,*,#28540,.T.);
#37886=ORIENTED_EDGE('',*,*,#28541,.F.);
#37887=ORIENTED_EDGE('',*,*,#28540,.F.);
#37888=ORIENTED_EDGE('',*,*,#28542,.T.);
#37889=ORIENTED_EDGE('',*,*,#28543,.T.);
#37890=ORIENTED_EDGE('',*,*,#28544,.F.);
#37891=ORIENTED_EDGE('',*,*,#28543,.F.);
#37892=ORIENTED_EDGE('',*,*,#28545,.T.);
#37893=ORIENTED_EDGE('',*,*,#27858,.F.);
#37894=ORIENTED_EDGE('',*,*,#27859,.F.);
#37895=ORIENTED_EDGE('',*,*,#28546,.T.);
#37896=ORIENTED_EDGE('',*,*,#28547,.F.);
#37897=ORIENTED_EDGE('',*,*,#28546,.F.);
#37898=ORIENTED_EDGE('',*,*,#28548,.T.);
#37899=ORIENTED_EDGE('',*,*,#28549,.T.);
#37900=ORIENTED_EDGE('',*,*,#28550,.F.);
#37901=ORIENTED_EDGE('',*,*,#28549,.F.);
#37902=ORIENTED_EDGE('',*,*,#28551,.T.);
#37903=ORIENTED_EDGE('',*,*,#27864,.F.);
#37904=ORIENTED_EDGE('',*,*,#27865,.F.);
#37905=ORIENTED_EDGE('',*,*,#28552,.T.);
#37906=ORIENTED_EDGE('',*,*,#28553,.F.);
#37907=ORIENTED_EDGE('',*,*,#28552,.F.);
#37908=ORIENTED_EDGE('',*,*,#28554,.T.);
#37909=ORIENTED_EDGE('',*,*,#28555,.T.);
#37910=ORIENTED_EDGE('',*,*,#28556,.F.);
#37911=ORIENTED_EDGE('',*,*,#28555,.F.);
#37912=ORIENTED_EDGE('',*,*,#28557,.T.);
#37913=ORIENTED_EDGE('',*,*,#27832,.F.);
#37914=ORIENTED_EDGE('',*,*,#27833,.F.);
#37915=ORIENTED_EDGE('',*,*,#28558,.T.);
#37916=ORIENTED_EDGE('',*,*,#28559,.F.);
#37917=ORIENTED_EDGE('',*,*,#28558,.F.);
#37918=ORIENTED_EDGE('',*,*,#28560,.T.);
#37919=ORIENTED_EDGE('',*,*,#28561,.T.);
#37920=ORIENTED_EDGE('',*,*,#28562,.F.);
#37921=ORIENTED_EDGE('',*,*,#28561,.F.);
#37922=ORIENTED_EDGE('',*,*,#28563,.T.);
#37923=ORIENTED_EDGE('',*,*,#27838,.F.);
#37924=ORIENTED_EDGE('',*,*,#27839,.F.);
#37925=ORIENTED_EDGE('',*,*,#28564,.T.);
#37926=ORIENTED_EDGE('',*,*,#28565,.F.);
#37927=ORIENTED_EDGE('',*,*,#28564,.F.);
#37928=ORIENTED_EDGE('',*,*,#28566,.T.);
#37929=ORIENTED_EDGE('',*,*,#28567,.T.);
#37930=ORIENTED_EDGE('',*,*,#28568,.F.);
#37931=ORIENTED_EDGE('',*,*,#28567,.F.);
#37932=ORIENTED_EDGE('',*,*,#28569,.T.);
#37933=ORIENTED_EDGE('',*,*,#27872,.F.);
#37934=ORIENTED_EDGE('',*,*,#27873,.F.);
#37935=ORIENTED_EDGE('',*,*,#28570,.T.);
#37936=ORIENTED_EDGE('',*,*,#28571,.F.);
#37937=ORIENTED_EDGE('',*,*,#28570,.F.);
#37938=ORIENTED_EDGE('',*,*,#28572,.T.);
#37939=ORIENTED_EDGE('',*,*,#28573,.T.);
#37940=ORIENTED_EDGE('',*,*,#28574,.F.);
#37941=ORIENTED_EDGE('',*,*,#28573,.F.);
#37942=ORIENTED_EDGE('',*,*,#28575,.T.);
#37943=ORIENTED_EDGE('',*,*,#27856,.F.);
#37944=ORIENTED_EDGE('',*,*,#27857,.F.);
#37945=ORIENTED_EDGE('',*,*,#28576,.T.);
#37946=ORIENTED_EDGE('',*,*,#28577,.F.);
#37947=ORIENTED_EDGE('',*,*,#28576,.F.);
#37948=ORIENTED_EDGE('',*,*,#28578,.T.);
#37949=ORIENTED_EDGE('',*,*,#28579,.T.);
#37950=ORIENTED_EDGE('',*,*,#28580,.F.);
#37951=ORIENTED_EDGE('',*,*,#28579,.F.);
#37952=ORIENTED_EDGE('',*,*,#28581,.T.);
#37953=ORIENTED_EDGE('',*,*,#27866,.F.);
#37954=ORIENTED_EDGE('',*,*,#27867,.F.);
#37955=ORIENTED_EDGE('',*,*,#28582,.T.);
#37956=ORIENTED_EDGE('',*,*,#28583,.F.);
#37957=ORIENTED_EDGE('',*,*,#28582,.F.);
#37958=ORIENTED_EDGE('',*,*,#28584,.T.);
#37959=ORIENTED_EDGE('',*,*,#28585,.T.);
#37960=ORIENTED_EDGE('',*,*,#28586,.F.);
#37961=ORIENTED_EDGE('',*,*,#28585,.F.);
#37962=ORIENTED_EDGE('',*,*,#28587,.T.);
#37963=ORIENTED_EDGE('',*,*,#27846,.F.);
#37964=ORIENTED_EDGE('',*,*,#27847,.F.);
#37965=ORIENTED_EDGE('',*,*,#28588,.T.);
#37966=ORIENTED_EDGE('',*,*,#28589,.F.);
#37967=ORIENTED_EDGE('',*,*,#28588,.F.);
#37968=ORIENTED_EDGE('',*,*,#28590,.T.);
#37969=ORIENTED_EDGE('',*,*,#28591,.T.);
#37970=ORIENTED_EDGE('',*,*,#28592,.F.);
#37971=ORIENTED_EDGE('',*,*,#28591,.F.);
#37972=ORIENTED_EDGE('',*,*,#28593,.T.);
#37973=ORIENTED_EDGE('',*,*,#27840,.F.);
#37974=ORIENTED_EDGE('',*,*,#27841,.F.);
#37975=ORIENTED_EDGE('',*,*,#28594,.T.);
#37976=ORIENTED_EDGE('',*,*,#28595,.F.);
#37977=ORIENTED_EDGE('',*,*,#28594,.F.);
#37978=ORIENTED_EDGE('',*,*,#28596,.T.);
#37979=ORIENTED_EDGE('',*,*,#28597,.T.);
#37980=ORIENTED_EDGE('',*,*,#28598,.F.);
#37981=ORIENTED_EDGE('',*,*,#28597,.F.);
#37982=ORIENTED_EDGE('',*,*,#28599,.T.);
#37983=ORIENTED_EDGE('',*,*,#27870,.F.);
#37984=ORIENTED_EDGE('',*,*,#27871,.F.);
#37985=ORIENTED_EDGE('',*,*,#28600,.T.);
#37986=ORIENTED_EDGE('',*,*,#28601,.F.);
#37987=ORIENTED_EDGE('',*,*,#28600,.F.);
#37988=ORIENTED_EDGE('',*,*,#28602,.T.);
#37989=ORIENTED_EDGE('',*,*,#28603,.T.);
#37990=ORIENTED_EDGE('',*,*,#28604,.F.);
#37991=ORIENTED_EDGE('',*,*,#28603,.F.);
#37992=ORIENTED_EDGE('',*,*,#28605,.T.);
#37993=ORIENTED_EDGE('',*,*,#27854,.F.);
#37994=ORIENTED_EDGE('',*,*,#27855,.F.);
#37995=ORIENTED_EDGE('',*,*,#28606,.T.);
#37996=ORIENTED_EDGE('',*,*,#28607,.F.);
#37997=ORIENTED_EDGE('',*,*,#28606,.F.);
#37998=ORIENTED_EDGE('',*,*,#28608,.T.);
#37999=ORIENTED_EDGE('',*,*,#28609,.T.);
#38000=ORIENTED_EDGE('',*,*,#28610,.F.);
#38001=ORIENTED_EDGE('',*,*,#28609,.F.);
#38002=ORIENTED_EDGE('',*,*,#28611,.T.);
#38003=ORIENTED_EDGE('',*,*,#27822,.F.);
#38004=ORIENTED_EDGE('',*,*,#27823,.F.);
#38005=ORIENTED_EDGE('',*,*,#28612,.T.);
#38006=ORIENTED_EDGE('',*,*,#28613,.F.);
#38007=ORIENTED_EDGE('',*,*,#28612,.F.);
#38008=ORIENTED_EDGE('',*,*,#28614,.T.);
#38009=ORIENTED_EDGE('',*,*,#28615,.T.);
#38010=ORIENTED_EDGE('',*,*,#28616,.F.);
#38011=ORIENTED_EDGE('',*,*,#28615,.F.);
#38012=ORIENTED_EDGE('',*,*,#28617,.T.);
#38013=ORIENTED_EDGE('',*,*,#27848,.F.);
#38014=ORIENTED_EDGE('',*,*,#27849,.F.);
#38015=ORIENTED_EDGE('',*,*,#28618,.T.);
#38016=ORIENTED_EDGE('',*,*,#28619,.F.);
#38017=ORIENTED_EDGE('',*,*,#28618,.F.);
#38018=ORIENTED_EDGE('',*,*,#28620,.T.);
#38019=ORIENTED_EDGE('',*,*,#28621,.T.);
#38020=ORIENTED_EDGE('',*,*,#28622,.F.);
#38021=ORIENTED_EDGE('',*,*,#28621,.F.);
#38022=ORIENTED_EDGE('',*,*,#28623,.T.);
#38023=ORIENTED_EDGE('',*,*,#27842,.F.);
#38024=ORIENTED_EDGE('',*,*,#27843,.F.);
#38025=ORIENTED_EDGE('',*,*,#28624,.T.);
#38026=ORIENTED_EDGE('',*,*,#28625,.F.);
#38027=ORIENTED_EDGE('',*,*,#28624,.F.);
#38028=ORIENTED_EDGE('',*,*,#28626,.T.);
#38029=ORIENTED_EDGE('',*,*,#28627,.T.);
#38030=ORIENTED_EDGE('',*,*,#28628,.F.);
#38031=ORIENTED_EDGE('',*,*,#28627,.F.);
#38032=ORIENTED_EDGE('',*,*,#28629,.T.);
#38033=ORIENTED_EDGE('',*,*,#27868,.F.);
#38034=ORIENTED_EDGE('',*,*,#27869,.F.);
#38035=ORIENTED_EDGE('',*,*,#28630,.T.);
#38036=ORIENTED_EDGE('',*,*,#28631,.F.);
#38037=ORIENTED_EDGE('',*,*,#28630,.F.);
#38038=ORIENTED_EDGE('',*,*,#28632,.T.);
#38039=ORIENTED_EDGE('',*,*,#28633,.T.);
#38040=ORIENTED_EDGE('',*,*,#28634,.F.);
#38041=ORIENTED_EDGE('',*,*,#28633,.F.);
#38042=ORIENTED_EDGE('',*,*,#28635,.T.);
#38043=ORIENTED_EDGE('',*,*,#27782,.F.);
#38044=ORIENTED_EDGE('',*,*,#27783,.F.);
#38045=ORIENTED_EDGE('',*,*,#28636,.T.);
#38046=ORIENTED_EDGE('',*,*,#28637,.F.);
#38047=ORIENTED_EDGE('',*,*,#28636,.F.);
#38048=ORIENTED_EDGE('',*,*,#28638,.T.);
#38049=ORIENTED_EDGE('',*,*,#28639,.T.);
#38050=ORIENTED_EDGE('',*,*,#28640,.F.);
#38051=ORIENTED_EDGE('',*,*,#28639,.F.);
#38052=ORIENTED_EDGE('',*,*,#28641,.T.);
#38053=ORIENTED_EDGE('',*,*,#27824,.F.);
#38054=ORIENTED_EDGE('',*,*,#27825,.F.);
#38055=ORIENTED_EDGE('',*,*,#28642,.T.);
#38056=ORIENTED_EDGE('',*,*,#28643,.F.);
#38057=ORIENTED_EDGE('',*,*,#28642,.F.);
#38058=ORIENTED_EDGE('',*,*,#28644,.T.);
#38059=ORIENTED_EDGE('',*,*,#28645,.T.);
#38060=ORIENTED_EDGE('',*,*,#28646,.F.);
#38061=ORIENTED_EDGE('',*,*,#28645,.F.);
#38062=ORIENTED_EDGE('',*,*,#28647,.T.);
#38063=ORIENTED_EDGE('',*,*,#27844,.F.);
#38064=ORIENTED_EDGE('',*,*,#27845,.F.);
#38065=ORIENTED_EDGE('',*,*,#28648,.T.);
#38066=ORIENTED_EDGE('',*,*,#28649,.F.);
#38067=ORIENTED_EDGE('',*,*,#28648,.F.);
#38068=ORIENTED_EDGE('',*,*,#28650,.T.);
#38069=ORIENTED_EDGE('',*,*,#28651,.T.);
#38070=ORIENTED_EDGE('',*,*,#28652,.F.);
#38071=ORIENTED_EDGE('',*,*,#28651,.F.);
#38072=ORIENTED_EDGE('',*,*,#28653,.T.);
#38073=ORIENTED_EDGE('',*,*,#27850,.F.);
#38074=ORIENTED_EDGE('',*,*,#27851,.F.);
#38075=ORIENTED_EDGE('',*,*,#28654,.T.);
#38076=ORIENTED_EDGE('',*,*,#28655,.F.);
#38077=ORIENTED_EDGE('',*,*,#28654,.F.);
#38078=ORIENTED_EDGE('',*,*,#28656,.T.);
#38079=ORIENTED_EDGE('',*,*,#28657,.T.);
#38080=ORIENTED_EDGE('',*,*,#28658,.F.);
#38081=ORIENTED_EDGE('',*,*,#28657,.F.);
#38082=ORIENTED_EDGE('',*,*,#28659,.T.);
#38083=ORIENTED_EDGE('',*,*,#28660,.F.);
#38084=ORIENTED_EDGE('',*,*,#28661,.T.);
#38085=ORIENTED_EDGE('',*,*,#28662,.F.);
#38086=ORIENTED_EDGE('',*,*,#28661,.F.);
#38087=ORIENTED_EDGE('',*,*,#28663,.T.);
#38088=ORIENTED_EDGE('',*,*,#28664,.T.);
#38089=ORIENTED_EDGE('',*,*,#28665,.F.);
#38090=ORIENTED_EDGE('',*,*,#28664,.F.);
#38091=ORIENTED_EDGE('',*,*,#28666,.F.);
#38092=ORIENTED_EDGE('',*,*,#28667,.T.);
#38093=ORIENTED_EDGE('',*,*,#28668,.F.);
#38094=ORIENTED_EDGE('',*,*,#28667,.F.);
#38095=ORIENTED_EDGE('',*,*,#28669,.T.);
#38096=ORIENTED_EDGE('',*,*,#28670,.T.);
#38097=ORIENTED_EDGE('',*,*,#28671,.F.);
#38098=ORIENTED_EDGE('',*,*,#28670,.F.);
#38099=ORIENTED_EDGE('',*,*,#28672,.F.);
#38100=ORIENTED_EDGE('',*,*,#28673,.T.);
#38101=ORIENTED_EDGE('',*,*,#28674,.F.);
#38102=ORIENTED_EDGE('',*,*,#28673,.F.);
#38103=ORIENTED_EDGE('',*,*,#28675,.T.);
#38104=ORIENTED_EDGE('',*,*,#28676,.T.);
#38105=ORIENTED_EDGE('',*,*,#28677,.F.);
#38106=ORIENTED_EDGE('',*,*,#28676,.F.);
#38107=ORIENTED_EDGE('',*,*,#28678,.F.);
#38108=ORIENTED_EDGE('',*,*,#28679,.T.);
#38109=ORIENTED_EDGE('',*,*,#28680,.F.);
#38110=ORIENTED_EDGE('',*,*,#28679,.F.);
#38111=ORIENTED_EDGE('',*,*,#28681,.T.);
#38112=ORIENTED_EDGE('',*,*,#28682,.T.);
#38113=ORIENTED_EDGE('',*,*,#28683,.F.);
#38114=ORIENTED_EDGE('',*,*,#28682,.F.);
#38115=ORIENTED_EDGE('',*,*,#28684,.F.);
#38116=ORIENTED_EDGE('',*,*,#28685,.T.);
#38117=ORIENTED_EDGE('',*,*,#28686,.F.);
#38118=ORIENTED_EDGE('',*,*,#28685,.F.);
#38119=ORIENTED_EDGE('',*,*,#28687,.T.);
#38120=ORIENTED_EDGE('',*,*,#28688,.T.);
#38121=ORIENTED_EDGE('',*,*,#28689,.F.);
#38122=ORIENTED_EDGE('',*,*,#28688,.F.);
#38123=ORIENTED_EDGE('',*,*,#28690,.F.);
#38124=ORIENTED_EDGE('',*,*,#28691,.T.);
#38125=ORIENTED_EDGE('',*,*,#28692,.F.);
#38126=ORIENTED_EDGE('',*,*,#28691,.F.);
#38127=ORIENTED_EDGE('',*,*,#28693,.T.);
#38128=ORIENTED_EDGE('',*,*,#28694,.T.);
#38129=ORIENTED_EDGE('',*,*,#28695,.F.);
#38130=ORIENTED_EDGE('',*,*,#28694,.F.);
#38131=ORIENTED_EDGE('',*,*,#28696,.F.);
#38132=ORIENTED_EDGE('',*,*,#28697,.T.);
#38133=ORIENTED_EDGE('',*,*,#28698,.F.);
#38134=ORIENTED_EDGE('',*,*,#28697,.F.);
#38135=ORIENTED_EDGE('',*,*,#28699,.T.);
#38136=ORIENTED_EDGE('',*,*,#28700,.T.);
#38137=ORIENTED_EDGE('',*,*,#28701,.F.);
#38138=ORIENTED_EDGE('',*,*,#28700,.F.);
#38139=ORIENTED_EDGE('',*,*,#28702,.F.);
#38140=ORIENTED_EDGE('',*,*,#28703,.T.);
#38141=ORIENTED_EDGE('',*,*,#28704,.F.);
#38142=ORIENTED_EDGE('',*,*,#28703,.F.);
#38143=ORIENTED_EDGE('',*,*,#28705,.T.);
#38144=ORIENTED_EDGE('',*,*,#28706,.T.);
#38145=ORIENTED_EDGE('',*,*,#28707,.F.);
#38146=ORIENTED_EDGE('',*,*,#28706,.F.);
#38147=ORIENTED_EDGE('',*,*,#28708,.F.);
#38148=ORIENTED_EDGE('',*,*,#28709,.T.);
#38149=ORIENTED_EDGE('',*,*,#28710,.F.);
#38150=ORIENTED_EDGE('',*,*,#28709,.F.);
#38151=ORIENTED_EDGE('',*,*,#28711,.T.);
#38152=ORIENTED_EDGE('',*,*,#28712,.T.);
#38153=ORIENTED_EDGE('',*,*,#28713,.F.);
#38154=ORIENTED_EDGE('',*,*,#28712,.F.);
#38155=ORIENTED_EDGE('',*,*,#28714,.F.);
#38156=ORIENTED_EDGE('',*,*,#28715,.T.);
#38157=ORIENTED_EDGE('',*,*,#28716,.F.);
#38158=ORIENTED_EDGE('',*,*,#28715,.F.);
#38159=ORIENTED_EDGE('',*,*,#28717,.T.);
#38160=ORIENTED_EDGE('',*,*,#28718,.T.);
#38161=ORIENTED_EDGE('',*,*,#28719,.F.);
#38162=ORIENTED_EDGE('',*,*,#28718,.F.);
#38163=ORIENTED_EDGE('',*,*,#28720,.F.);
#38164=ORIENTED_EDGE('',*,*,#28721,.T.);
#38165=ORIENTED_EDGE('',*,*,#28722,.F.);
#38166=ORIENTED_EDGE('',*,*,#28721,.F.);
#38167=ORIENTED_EDGE('',*,*,#28723,.T.);
#38168=ORIENTED_EDGE('',*,*,#28724,.T.);
#38169=ORIENTED_EDGE('',*,*,#28725,.F.);
#38170=ORIENTED_EDGE('',*,*,#28724,.F.);
#38171=ORIENTED_EDGE('',*,*,#28726,.F.);
#38172=ORIENTED_EDGE('',*,*,#28727,.T.);
#38173=ORIENTED_EDGE('',*,*,#28728,.F.);
#38174=ORIENTED_EDGE('',*,*,#28727,.F.);
#38175=ORIENTED_EDGE('',*,*,#28729,.T.);
#38176=ORIENTED_EDGE('',*,*,#28730,.T.);
#38177=ORIENTED_EDGE('',*,*,#28731,.F.);
#38178=ORIENTED_EDGE('',*,*,#28730,.F.);
#38179=ORIENTED_EDGE('',*,*,#28732,.F.);
#38180=ORIENTED_EDGE('',*,*,#28733,.T.);
#38181=ORIENTED_EDGE('',*,*,#28734,.F.);
#38182=ORIENTED_EDGE('',*,*,#28733,.F.);
#38183=ORIENTED_EDGE('',*,*,#28735,.T.);
#38184=ORIENTED_EDGE('',*,*,#28736,.T.);
#38185=ORIENTED_EDGE('',*,*,#28737,.F.);
#38186=ORIENTED_EDGE('',*,*,#28736,.F.);
#38187=ORIENTED_EDGE('',*,*,#28738,.F.);
#38188=ORIENTED_EDGE('',*,*,#28739,.T.);
#38189=ORIENTED_EDGE('',*,*,#28740,.F.);
#38190=ORIENTED_EDGE('',*,*,#28739,.F.);
#38191=ORIENTED_EDGE('',*,*,#28741,.T.);
#38192=ORIENTED_EDGE('',*,*,#28742,.T.);
#38193=ORIENTED_EDGE('',*,*,#28743,.F.);
#38194=ORIENTED_EDGE('',*,*,#28742,.F.);
#38195=ORIENTED_EDGE('',*,*,#28744,.F.);
#38196=ORIENTED_EDGE('',*,*,#28745,.T.);
#38197=ORIENTED_EDGE('',*,*,#28746,.F.);
#38198=ORIENTED_EDGE('',*,*,#28745,.F.);
#38199=ORIENTED_EDGE('',*,*,#28747,.T.);
#38200=ORIENTED_EDGE('',*,*,#28748,.T.);
#38201=ORIENTED_EDGE('',*,*,#28749,.F.);
#38202=ORIENTED_EDGE('',*,*,#28748,.F.);
#38203=ORIENTED_EDGE('',*,*,#28750,.F.);
#38204=ORIENTED_EDGE('',*,*,#28751,.T.);
#38205=ORIENTED_EDGE('',*,*,#28752,.F.);
#38206=ORIENTED_EDGE('',*,*,#28751,.F.);
#38207=ORIENTED_EDGE('',*,*,#28753,.T.);
#38208=ORIENTED_EDGE('',*,*,#28754,.T.);
#38209=ORIENTED_EDGE('',*,*,#28755,.F.);
#38210=ORIENTED_EDGE('',*,*,#28754,.F.);
#38211=ORIENTED_EDGE('',*,*,#28756,.F.);
#38212=ORIENTED_EDGE('',*,*,#28757,.T.);
#38213=ORIENTED_EDGE('',*,*,#28758,.F.);
#38214=ORIENTED_EDGE('',*,*,#28757,.F.);
#38215=ORIENTED_EDGE('',*,*,#28759,.T.);
#38216=ORIENTED_EDGE('',*,*,#28760,.T.);
#38217=ORIENTED_EDGE('',*,*,#28761,.F.);
#38218=ORIENTED_EDGE('',*,*,#28760,.F.);
#38219=ORIENTED_EDGE('',*,*,#28762,.F.);
#38220=ORIENTED_EDGE('',*,*,#28763,.T.);
#38221=ORIENTED_EDGE('',*,*,#28764,.F.);
#38222=ORIENTED_EDGE('',*,*,#28763,.F.);
#38223=ORIENTED_EDGE('',*,*,#28765,.T.);
#38224=ORIENTED_EDGE('',*,*,#28766,.T.);
#38225=ORIENTED_EDGE('',*,*,#28767,.F.);
#38226=ORIENTED_EDGE('',*,*,#28766,.F.);
#38227=ORIENTED_EDGE('',*,*,#28768,.F.);
#38228=ORIENTED_EDGE('',*,*,#28769,.T.);
#38229=ORIENTED_EDGE('',*,*,#28770,.F.);
#38230=ORIENTED_EDGE('',*,*,#28769,.F.);
#38231=ORIENTED_EDGE('',*,*,#28771,.T.);
#38232=ORIENTED_EDGE('',*,*,#28772,.T.);
#38233=ORIENTED_EDGE('',*,*,#28773,.F.);
#38234=ORIENTED_EDGE('',*,*,#28772,.F.);
#38235=ORIENTED_EDGE('',*,*,#28774,.F.);
#38236=ORIENTED_EDGE('',*,*,#28775,.T.);
#38237=ORIENTED_EDGE('',*,*,#28776,.F.);
#38238=ORIENTED_EDGE('',*,*,#28775,.F.);
#38239=ORIENTED_EDGE('',*,*,#28777,.T.);
#38240=ORIENTED_EDGE('',*,*,#28778,.T.);
#38241=ORIENTED_EDGE('',*,*,#28779,.F.);
#38242=ORIENTED_EDGE('',*,*,#28778,.F.);
#38243=ORIENTED_EDGE('',*,*,#28780,.F.);
#38244=ORIENTED_EDGE('',*,*,#28781,.T.);
#38245=ORIENTED_EDGE('',*,*,#28782,.F.);
#38246=ORIENTED_EDGE('',*,*,#28781,.F.);
#38247=ORIENTED_EDGE('',*,*,#28783,.T.);
#38248=ORIENTED_EDGE('',*,*,#28784,.T.);
#38249=ORIENTED_EDGE('',*,*,#28785,.F.);
#38250=ORIENTED_EDGE('',*,*,#28784,.F.);
#38251=ORIENTED_EDGE('',*,*,#28786,.F.);
#38252=ORIENTED_EDGE('',*,*,#28787,.T.);
#38253=ORIENTED_EDGE('',*,*,#28788,.F.);
#38254=ORIENTED_EDGE('',*,*,#28787,.F.);
#38255=ORIENTED_EDGE('',*,*,#28789,.T.);
#38256=ORIENTED_EDGE('',*,*,#28790,.T.);
#38257=ORIENTED_EDGE('',*,*,#28791,.F.);
#38258=ORIENTED_EDGE('',*,*,#28790,.F.);
#38259=ORIENTED_EDGE('',*,*,#28792,.F.);
#38260=ORIENTED_EDGE('',*,*,#28793,.T.);
#38261=ORIENTED_EDGE('',*,*,#28794,.F.);
#38262=ORIENTED_EDGE('',*,*,#28793,.F.);
#38263=ORIENTED_EDGE('',*,*,#28795,.T.);
#38264=ORIENTED_EDGE('',*,*,#28796,.T.);
#38265=ORIENTED_EDGE('',*,*,#28797,.F.);
#38266=ORIENTED_EDGE('',*,*,#28796,.F.);
#38267=ORIENTED_EDGE('',*,*,#28798,.F.);
#38268=ORIENTED_EDGE('',*,*,#28799,.T.);
#38269=ORIENTED_EDGE('',*,*,#28800,.F.);
#38270=ORIENTED_EDGE('',*,*,#28799,.F.);
#38271=ORIENTED_EDGE('',*,*,#28801,.T.);
#38272=ORIENTED_EDGE('',*,*,#28802,.T.);
#38273=ORIENTED_EDGE('',*,*,#28803,.F.);
#38274=ORIENTED_EDGE('',*,*,#28802,.F.);
#38275=ORIENTED_EDGE('',*,*,#28804,.F.);
#38276=ORIENTED_EDGE('',*,*,#28805,.T.);
#38277=ORIENTED_EDGE('',*,*,#28806,.F.);
#38278=ORIENTED_EDGE('',*,*,#28805,.F.);
#38279=ORIENTED_EDGE('',*,*,#28807,.T.);
#38280=ORIENTED_EDGE('',*,*,#28808,.T.);
#38281=ORIENTED_EDGE('',*,*,#28809,.F.);
#38282=ORIENTED_EDGE('',*,*,#28808,.F.);
#38283=ORIENTED_EDGE('',*,*,#28810,.F.);
#38284=ORIENTED_EDGE('',*,*,#28811,.T.);
#38285=ORIENTED_EDGE('',*,*,#28812,.F.);
#38286=ORIENTED_EDGE('',*,*,#28811,.F.);
#38287=ORIENTED_EDGE('',*,*,#28813,.T.);
#38288=ORIENTED_EDGE('',*,*,#28814,.T.);
#38289=ORIENTED_EDGE('',*,*,#28815,.F.);
#38290=ORIENTED_EDGE('',*,*,#28814,.F.);
#38291=ORIENTED_EDGE('',*,*,#28816,.F.);
#38292=ORIENTED_EDGE('',*,*,#28817,.T.);
#38293=ORIENTED_EDGE('',*,*,#28818,.F.);
#38294=ORIENTED_EDGE('',*,*,#28817,.F.);
#38295=ORIENTED_EDGE('',*,*,#28819,.T.);
#38296=ORIENTED_EDGE('',*,*,#28820,.T.);
#38297=ORIENTED_EDGE('',*,*,#28821,.F.);
#38298=ORIENTED_EDGE('',*,*,#28820,.F.);
#38299=ORIENTED_EDGE('',*,*,#28822,.F.);
#38300=ORIENTED_EDGE('',*,*,#28823,.T.);
#38301=ORIENTED_EDGE('',*,*,#28824,.F.);
#38302=ORIENTED_EDGE('',*,*,#28823,.F.);
#38303=ORIENTED_EDGE('',*,*,#28825,.T.);
#38304=ORIENTED_EDGE('',*,*,#28826,.T.);
#38305=ORIENTED_EDGE('',*,*,#28827,.F.);
#38306=ORIENTED_EDGE('',*,*,#28826,.F.);
#38307=ORIENTED_EDGE('',*,*,#28828,.F.);
#38308=ORIENTED_EDGE('',*,*,#28829,.T.);
#38309=ORIENTED_EDGE('',*,*,#28830,.F.);
#38310=ORIENTED_EDGE('',*,*,#28829,.F.);
#38311=ORIENTED_EDGE('',*,*,#28831,.T.);
#38312=ORIENTED_EDGE('',*,*,#28832,.T.);
#38313=ORIENTED_EDGE('',*,*,#28833,.F.);
#38314=ORIENTED_EDGE('',*,*,#28832,.F.);
#38315=ORIENTED_EDGE('',*,*,#28834,.F.);
#38316=ORIENTED_EDGE('',*,*,#28835,.T.);
#38317=ORIENTED_EDGE('',*,*,#28836,.F.);
#38318=ORIENTED_EDGE('',*,*,#28835,.F.);
#38319=ORIENTED_EDGE('',*,*,#28837,.T.);
#38320=ORIENTED_EDGE('',*,*,#28838,.T.);
#38321=ORIENTED_EDGE('',*,*,#28839,.F.);
#38322=ORIENTED_EDGE('',*,*,#28838,.F.);
#38323=ORIENTED_EDGE('',*,*,#28840,.F.);
#38324=ORIENTED_EDGE('',*,*,#28841,.T.);
#38325=ORIENTED_EDGE('',*,*,#28842,.F.);
#38326=ORIENTED_EDGE('',*,*,#28841,.F.);
#38327=ORIENTED_EDGE('',*,*,#28843,.T.);
#38328=ORIENTED_EDGE('',*,*,#28844,.T.);
#38329=ORIENTED_EDGE('',*,*,#28845,.F.);
#38330=ORIENTED_EDGE('',*,*,#28844,.F.);
#38331=ORIENTED_EDGE('',*,*,#28846,.F.);
#38332=ORIENTED_EDGE('',*,*,#28847,.T.);
#38333=ORIENTED_EDGE('',*,*,#28848,.F.);
#38334=ORIENTED_EDGE('',*,*,#28847,.F.);
#38335=ORIENTED_EDGE('',*,*,#28849,.T.);
#38336=ORIENTED_EDGE('',*,*,#28850,.T.);
#38337=ORIENTED_EDGE('',*,*,#28851,.F.);
#38338=ORIENTED_EDGE('',*,*,#28850,.F.);
#38339=ORIENTED_EDGE('',*,*,#28852,.F.);
#38340=ORIENTED_EDGE('',*,*,#28853,.T.);
#38341=ORIENTED_EDGE('',*,*,#28854,.F.);
#38342=ORIENTED_EDGE('',*,*,#28853,.F.);
#38343=ORIENTED_EDGE('',*,*,#28855,.T.);
#38344=ORIENTED_EDGE('',*,*,#28856,.T.);
#38345=ORIENTED_EDGE('',*,*,#28857,.F.);
#38346=ORIENTED_EDGE('',*,*,#28856,.F.);
#38347=ORIENTED_EDGE('',*,*,#28858,.F.);
#38348=ORIENTED_EDGE('',*,*,#28859,.T.);
#38349=ORIENTED_EDGE('',*,*,#28860,.F.);
#38350=ORIENTED_EDGE('',*,*,#28859,.F.);
#38351=ORIENTED_EDGE('',*,*,#28861,.T.);
#38352=ORIENTED_EDGE('',*,*,#28862,.T.);
#38353=ORIENTED_EDGE('',*,*,#28863,.F.);
#38354=ORIENTED_EDGE('',*,*,#28862,.F.);
#38355=ORIENTED_EDGE('',*,*,#28864,.F.);
#38356=ORIENTED_EDGE('',*,*,#28865,.T.);
#38357=ORIENTED_EDGE('',*,*,#28866,.F.);
#38358=ORIENTED_EDGE('',*,*,#28865,.F.);
#38359=ORIENTED_EDGE('',*,*,#28867,.T.);
#38360=ORIENTED_EDGE('',*,*,#28868,.T.);
#38361=ORIENTED_EDGE('',*,*,#28869,.F.);
#38362=ORIENTED_EDGE('',*,*,#28868,.F.);
#38363=ORIENTED_EDGE('',*,*,#28870,.F.);
#38364=ORIENTED_EDGE('',*,*,#28871,.T.);
#38365=ORIENTED_EDGE('',*,*,#28872,.F.);
#38366=ORIENTED_EDGE('',*,*,#28871,.F.);
#38367=ORIENTED_EDGE('',*,*,#28873,.T.);
#38368=ORIENTED_EDGE('',*,*,#28874,.T.);
#38369=ORIENTED_EDGE('',*,*,#28875,.F.);
#38370=ORIENTED_EDGE('',*,*,#28874,.F.);
#38371=ORIENTED_EDGE('',*,*,#28876,.F.);
#38372=ORIENTED_EDGE('',*,*,#28877,.T.);
#38373=ORIENTED_EDGE('',*,*,#28878,.F.);
#38374=ORIENTED_EDGE('',*,*,#28877,.F.);
#38375=ORIENTED_EDGE('',*,*,#28879,.T.);
#38376=ORIENTED_EDGE('',*,*,#28880,.T.);
#38377=ORIENTED_EDGE('',*,*,#28881,.F.);
#38378=ORIENTED_EDGE('',*,*,#28880,.F.);
#38379=ORIENTED_EDGE('',*,*,#28882,.F.);
#38380=ORIENTED_EDGE('',*,*,#28883,.T.);
#38381=ORIENTED_EDGE('',*,*,#28884,.F.);
#38382=ORIENTED_EDGE('',*,*,#28883,.F.);
#38383=ORIENTED_EDGE('',*,*,#28885,.T.);
#38384=ORIENTED_EDGE('',*,*,#28886,.T.);
#38385=ORIENTED_EDGE('',*,*,#28887,.F.);
#38386=ORIENTED_EDGE('',*,*,#28886,.F.);
#38387=ORIENTED_EDGE('',*,*,#28888,.F.);
#38388=ORIENTED_EDGE('',*,*,#28889,.T.);
#38389=ORIENTED_EDGE('',*,*,#28890,.F.);
#38390=ORIENTED_EDGE('',*,*,#28889,.F.);
#38391=ORIENTED_EDGE('',*,*,#28891,.T.);
#38392=ORIENTED_EDGE('',*,*,#28892,.T.);
#38393=ORIENTED_EDGE('',*,*,#28893,.F.);
#38394=ORIENTED_EDGE('',*,*,#28892,.F.);
#38395=ORIENTED_EDGE('',*,*,#28894,.F.);
#38396=ORIENTED_EDGE('',*,*,#28895,.T.);
#38397=ORIENTED_EDGE('',*,*,#28896,.F.);
#38398=ORIENTED_EDGE('',*,*,#28895,.F.);
#38399=ORIENTED_EDGE('',*,*,#28897,.T.);
#38400=ORIENTED_EDGE('',*,*,#28898,.T.);
#38401=ORIENTED_EDGE('',*,*,#28899,.F.);
#38402=ORIENTED_EDGE('',*,*,#28898,.F.);
#38403=ORIENTED_EDGE('',*,*,#28900,.F.);
#38404=ORIENTED_EDGE('',*,*,#28901,.T.);
#38405=ORIENTED_EDGE('',*,*,#28902,.F.);
#38406=ORIENTED_EDGE('',*,*,#28901,.F.);
#38407=ORIENTED_EDGE('',*,*,#28903,.T.);
#38408=ORIENTED_EDGE('',*,*,#28904,.T.);
#38409=ORIENTED_EDGE('',*,*,#28905,.F.);
#38410=ORIENTED_EDGE('',*,*,#28904,.F.);
#38411=ORIENTED_EDGE('',*,*,#28906,.F.);
#38412=ORIENTED_EDGE('',*,*,#28907,.T.);
#38413=ORIENTED_EDGE('',*,*,#28908,.F.);
#38414=ORIENTED_EDGE('',*,*,#28907,.F.);
#38415=ORIENTED_EDGE('',*,*,#28909,.T.);
#38416=ORIENTED_EDGE('',*,*,#28910,.T.);
#38417=ORIENTED_EDGE('',*,*,#28911,.F.);
#38418=ORIENTED_EDGE('',*,*,#28910,.F.);
#38419=ORIENTED_EDGE('',*,*,#28912,.F.);
#38420=ORIENTED_EDGE('',*,*,#28913,.T.);
#38421=ORIENTED_EDGE('',*,*,#28914,.F.);
#38422=ORIENTED_EDGE('',*,*,#28913,.F.);
#38423=ORIENTED_EDGE('',*,*,#28915,.T.);
#38424=ORIENTED_EDGE('',*,*,#28916,.T.);
#38425=ORIENTED_EDGE('',*,*,#28917,.F.);
#38426=ORIENTED_EDGE('',*,*,#28916,.F.);
#38427=ORIENTED_EDGE('',*,*,#28918,.F.);
#38428=ORIENTED_EDGE('',*,*,#28919,.T.);
#38429=ORIENTED_EDGE('',*,*,#28920,.F.);
#38430=ORIENTED_EDGE('',*,*,#28919,.F.);
#38431=ORIENTED_EDGE('',*,*,#28921,.T.);
#38432=ORIENTED_EDGE('',*,*,#28922,.T.);
#38433=ORIENTED_EDGE('',*,*,#28923,.F.);
#38434=ORIENTED_EDGE('',*,*,#28922,.F.);
#38435=ORIENTED_EDGE('',*,*,#28924,.F.);
#38436=ORIENTED_EDGE('',*,*,#28925,.T.);
#38437=ORIENTED_EDGE('',*,*,#28926,.F.);
#38438=ORIENTED_EDGE('',*,*,#28925,.F.);
#38439=ORIENTED_EDGE('',*,*,#28927,.T.);
#38440=ORIENTED_EDGE('',*,*,#28928,.T.);
#38441=ORIENTED_EDGE('',*,*,#28929,.F.);
#38442=ORIENTED_EDGE('',*,*,#28928,.F.);
#38443=ORIENTED_EDGE('',*,*,#28930,.F.);
#38444=ORIENTED_EDGE('',*,*,#28931,.T.);
#38445=ORIENTED_EDGE('',*,*,#28932,.F.);
#38446=ORIENTED_EDGE('',*,*,#28931,.F.);
#38447=ORIENTED_EDGE('',*,*,#28933,.T.);
#38448=ORIENTED_EDGE('',*,*,#28934,.T.);
#38449=ORIENTED_EDGE('',*,*,#28935,.F.);
#38450=ORIENTED_EDGE('',*,*,#28934,.F.);
#38451=ORIENTED_EDGE('',*,*,#28936,.F.);
#38452=ORIENTED_EDGE('',*,*,#28937,.T.);
#38453=ORIENTED_EDGE('',*,*,#28938,.F.);
#38454=ORIENTED_EDGE('',*,*,#28937,.F.);
#38455=ORIENTED_EDGE('',*,*,#28939,.T.);
#38456=ORIENTED_EDGE('',*,*,#28940,.T.);
#38457=ORIENTED_EDGE('',*,*,#28941,.F.);
#38458=ORIENTED_EDGE('',*,*,#28940,.F.);
#38459=ORIENTED_EDGE('',*,*,#28942,.F.);
#38460=ORIENTED_EDGE('',*,*,#28943,.T.);
#38461=ORIENTED_EDGE('',*,*,#28944,.F.);
#38462=ORIENTED_EDGE('',*,*,#28943,.F.);
#38463=ORIENTED_EDGE('',*,*,#28945,.T.);
#38464=ORIENTED_EDGE('',*,*,#28946,.T.);
#38465=ORIENTED_EDGE('',*,*,#28947,.F.);
#38466=ORIENTED_EDGE('',*,*,#28946,.F.);
#38467=ORIENTED_EDGE('',*,*,#28948,.F.);
#38468=ORIENTED_EDGE('',*,*,#28949,.T.);
#38469=ORIENTED_EDGE('',*,*,#28950,.F.);
#38470=ORIENTED_EDGE('',*,*,#28949,.F.);
#38471=ORIENTED_EDGE('',*,*,#28951,.T.);
#38472=ORIENTED_EDGE('',*,*,#28952,.T.);
#38473=ORIENTED_EDGE('',*,*,#28953,.F.);
#38474=ORIENTED_EDGE('',*,*,#28952,.F.);
#38475=ORIENTED_EDGE('',*,*,#28954,.F.);
#38476=ORIENTED_EDGE('',*,*,#28955,.T.);
#38477=ORIENTED_EDGE('',*,*,#28956,.F.);
#38478=ORIENTED_EDGE('',*,*,#28955,.F.);
#38479=ORIENTED_EDGE('',*,*,#28957,.T.);
#38480=ORIENTED_EDGE('',*,*,#28958,.T.);
#38481=ORIENTED_EDGE('',*,*,#28959,.F.);
#38482=ORIENTED_EDGE('',*,*,#28958,.F.);
#38483=ORIENTED_EDGE('',*,*,#28960,.F.);
#38484=ORIENTED_EDGE('',*,*,#28961,.T.);
#38485=ORIENTED_EDGE('',*,*,#28962,.F.);
#38486=ORIENTED_EDGE('',*,*,#28961,.F.);
#38487=ORIENTED_EDGE('',*,*,#28963,.T.);
#38488=ORIENTED_EDGE('',*,*,#28964,.T.);
#38489=ORIENTED_EDGE('',*,*,#28965,.F.);
#38490=ORIENTED_EDGE('',*,*,#28964,.F.);
#38491=ORIENTED_EDGE('',*,*,#28966,.F.);
#38492=ORIENTED_EDGE('',*,*,#28967,.T.);
#38493=ORIENTED_EDGE('',*,*,#28968,.F.);
#38494=ORIENTED_EDGE('',*,*,#28967,.F.);
#38495=ORIENTED_EDGE('',*,*,#28969,.T.);
#38496=ORIENTED_EDGE('',*,*,#28970,.T.);
#38497=ORIENTED_EDGE('',*,*,#28971,.F.);
#38498=ORIENTED_EDGE('',*,*,#28970,.F.);
#38499=ORIENTED_EDGE('',*,*,#28972,.F.);
#38500=ORIENTED_EDGE('',*,*,#28973,.T.);
#38501=ORIENTED_EDGE('',*,*,#28974,.F.);
#38502=ORIENTED_EDGE('',*,*,#28973,.F.);
#38503=ORIENTED_EDGE('',*,*,#28975,.T.);
#38504=ORIENTED_EDGE('',*,*,#28976,.T.);
#38505=ORIENTED_EDGE('',*,*,#28977,.F.);
#38506=ORIENTED_EDGE('',*,*,#28976,.F.);
#38507=ORIENTED_EDGE('',*,*,#28978,.F.);
#38508=ORIENTED_EDGE('',*,*,#28979,.T.);
#38509=ORIENTED_EDGE('',*,*,#28980,.F.);
#38510=ORIENTED_EDGE('',*,*,#28979,.F.);
#38511=ORIENTED_EDGE('',*,*,#28981,.T.);
#38512=ORIENTED_EDGE('',*,*,#28982,.T.);
#38513=ORIENTED_EDGE('',*,*,#28983,.F.);
#38514=ORIENTED_EDGE('',*,*,#28982,.F.);
#38515=ORIENTED_EDGE('',*,*,#28984,.F.);
#38516=ORIENTED_EDGE('',*,*,#28985,.T.);
#38517=ORIENTED_EDGE('',*,*,#28986,.F.);
#38518=ORIENTED_EDGE('',*,*,#28985,.F.);
#38519=ORIENTED_EDGE('',*,*,#28987,.T.);
#38520=ORIENTED_EDGE('',*,*,#28988,.T.);
#38521=ORIENTED_EDGE('',*,*,#28989,.F.);
#38522=ORIENTED_EDGE('',*,*,#28988,.F.);
#38523=ORIENTED_EDGE('',*,*,#28990,.F.);
#38524=ORIENTED_EDGE('',*,*,#28991,.T.);
#38525=ORIENTED_EDGE('',*,*,#28992,.F.);
#38526=ORIENTED_EDGE('',*,*,#28991,.F.);
#38527=ORIENTED_EDGE('',*,*,#28993,.T.);
#38528=ORIENTED_EDGE('',*,*,#28994,.T.);
#38529=ORIENTED_EDGE('',*,*,#28995,.F.);
#38530=ORIENTED_EDGE('',*,*,#28994,.F.);
#38531=ORIENTED_EDGE('',*,*,#28996,.F.);
#38532=ORIENTED_EDGE('',*,*,#28997,.T.);
#38533=ORIENTED_EDGE('',*,*,#28998,.F.);
#38534=ORIENTED_EDGE('',*,*,#28997,.F.);
#38535=ORIENTED_EDGE('',*,*,#28999,.T.);
#38536=ORIENTED_EDGE('',*,*,#29000,.T.);
#38537=ORIENTED_EDGE('',*,*,#29001,.F.);
#38538=ORIENTED_EDGE('',*,*,#29000,.F.);
#38539=ORIENTED_EDGE('',*,*,#29002,.F.);
#38540=ORIENTED_EDGE('',*,*,#29003,.T.);
#38541=ORIENTED_EDGE('',*,*,#29004,.F.);
#38542=ORIENTED_EDGE('',*,*,#29003,.F.);
#38543=ORIENTED_EDGE('',*,*,#29005,.T.);
#38544=ORIENTED_EDGE('',*,*,#29006,.T.);
#38545=ORIENTED_EDGE('',*,*,#29007,.F.);
#38546=ORIENTED_EDGE('',*,*,#29006,.F.);
#38547=ORIENTED_EDGE('',*,*,#29008,.F.);
#38548=ORIENTED_EDGE('',*,*,#29009,.T.);
#38549=ORIENTED_EDGE('',*,*,#29010,.F.);
#38550=ORIENTED_EDGE('',*,*,#29009,.F.);
#38551=ORIENTED_EDGE('',*,*,#29011,.T.);
#38552=ORIENTED_EDGE('',*,*,#29012,.T.);
#38553=ORIENTED_EDGE('',*,*,#29013,.F.);
#38554=ORIENTED_EDGE('',*,*,#29012,.F.);
#38555=ORIENTED_EDGE('',*,*,#29014,.F.);
#38556=ORIENTED_EDGE('',*,*,#29015,.T.);
#38557=ORIENTED_EDGE('',*,*,#29016,.F.);
#38558=ORIENTED_EDGE('',*,*,#29015,.F.);
#38559=ORIENTED_EDGE('',*,*,#29017,.T.);
#38560=ORIENTED_EDGE('',*,*,#29018,.T.);
#38561=ORIENTED_EDGE('',*,*,#29019,.F.);
#38562=ORIENTED_EDGE('',*,*,#29018,.F.);
#38563=ORIENTED_EDGE('',*,*,#29020,.F.);
#38564=ORIENTED_EDGE('',*,*,#29021,.T.);
#38565=ORIENTED_EDGE('',*,*,#29022,.F.);
#38566=ORIENTED_EDGE('',*,*,#29021,.F.);
#38567=ORIENTED_EDGE('',*,*,#29023,.T.);
#38568=ORIENTED_EDGE('',*,*,#29024,.T.);
#38569=ORIENTED_EDGE('',*,*,#29025,.F.);
#38570=ORIENTED_EDGE('',*,*,#29024,.F.);
#38571=ORIENTED_EDGE('',*,*,#29026,.F.);
#38572=ORIENTED_EDGE('',*,*,#29027,.T.);
#38573=ORIENTED_EDGE('',*,*,#29028,.F.);
#38574=ORIENTED_EDGE('',*,*,#29027,.F.);
#38575=ORIENTED_EDGE('',*,*,#29029,.T.);
#38576=ORIENTED_EDGE('',*,*,#29030,.T.);
#38577=ORIENTED_EDGE('',*,*,#29031,.F.);
#38578=ORIENTED_EDGE('',*,*,#29030,.F.);
#38579=ORIENTED_EDGE('',*,*,#29032,.F.);
#38580=ORIENTED_EDGE('',*,*,#29033,.T.);
#38581=ORIENTED_EDGE('',*,*,#29034,.F.);
#38582=ORIENTED_EDGE('',*,*,#29033,.F.);
#38583=ORIENTED_EDGE('',*,*,#29035,.T.);
#38584=ORIENTED_EDGE('',*,*,#29036,.T.);
#38585=ORIENTED_EDGE('',*,*,#29037,.F.);
#38586=ORIENTED_EDGE('',*,*,#29036,.F.);
#38587=ORIENTED_EDGE('',*,*,#29038,.F.);
#38588=ORIENTED_EDGE('',*,*,#29039,.T.);
#38589=ORIENTED_EDGE('',*,*,#29040,.F.);
#38590=ORIENTED_EDGE('',*,*,#29039,.F.);
#38591=ORIENTED_EDGE('',*,*,#29041,.T.);
#38592=ORIENTED_EDGE('',*,*,#29042,.T.);
#38593=ORIENTED_EDGE('',*,*,#29043,.F.);
#38594=ORIENTED_EDGE('',*,*,#29042,.F.);
#38595=ORIENTED_EDGE('',*,*,#29044,.F.);
#38596=ORIENTED_EDGE('',*,*,#29045,.T.);
#38597=ORIENTED_EDGE('',*,*,#29046,.F.);
#38598=ORIENTED_EDGE('',*,*,#29045,.F.);
#38599=ORIENTED_EDGE('',*,*,#29047,.T.);
#38600=ORIENTED_EDGE('',*,*,#29048,.T.);
#38601=ORIENTED_EDGE('',*,*,#29049,.F.);
#38602=ORIENTED_EDGE('',*,*,#29048,.F.);
#38603=ORIENTED_EDGE('',*,*,#29050,.F.);
#38604=ORIENTED_EDGE('',*,*,#29051,.T.);
#38605=ORIENTED_EDGE('',*,*,#29052,.F.);
#38606=ORIENTED_EDGE('',*,*,#29051,.F.);
#38607=ORIENTED_EDGE('',*,*,#29053,.T.);
#38608=ORIENTED_EDGE('',*,*,#29054,.T.);
#38609=ORIENTED_EDGE('',*,*,#29055,.F.);
#38610=ORIENTED_EDGE('',*,*,#29054,.F.);
#38611=ORIENTED_EDGE('',*,*,#29056,.F.);
#38612=ORIENTED_EDGE('',*,*,#29057,.T.);
#38613=ORIENTED_EDGE('',*,*,#29058,.F.);
#38614=ORIENTED_EDGE('',*,*,#29057,.F.);
#38615=ORIENTED_EDGE('',*,*,#29059,.T.);
#38616=ORIENTED_EDGE('',*,*,#29060,.T.);
#38617=ORIENTED_EDGE('',*,*,#29061,.F.);
#38618=ORIENTED_EDGE('',*,*,#29060,.F.);
#38619=ORIENTED_EDGE('',*,*,#29062,.F.);
#38620=ORIENTED_EDGE('',*,*,#29063,.T.);
#38621=ORIENTED_EDGE('',*,*,#29064,.F.);
#38622=ORIENTED_EDGE('',*,*,#29063,.F.);
#38623=ORIENTED_EDGE('',*,*,#29065,.T.);
#38624=ORIENTED_EDGE('',*,*,#29066,.T.);
#38625=ORIENTED_EDGE('',*,*,#29067,.F.);
#38626=ORIENTED_EDGE('',*,*,#29066,.F.);
#38627=ORIENTED_EDGE('',*,*,#29068,.F.);
#38628=ORIENTED_EDGE('',*,*,#29069,.T.);
#38629=ORIENTED_EDGE('',*,*,#29070,.F.);
#38630=ORIENTED_EDGE('',*,*,#29069,.F.);
#38631=ORIENTED_EDGE('',*,*,#29071,.T.);
#38632=ORIENTED_EDGE('',*,*,#29072,.T.);
#38633=ORIENTED_EDGE('',*,*,#29073,.F.);
#38634=ORIENTED_EDGE('',*,*,#29072,.F.);
#38635=ORIENTED_EDGE('',*,*,#29074,.F.);
#38636=ORIENTED_EDGE('',*,*,#29075,.T.);
#38637=ORIENTED_EDGE('',*,*,#29076,.F.);
#38638=ORIENTED_EDGE('',*,*,#29075,.F.);
#38639=ORIENTED_EDGE('',*,*,#29077,.T.);
#38640=ORIENTED_EDGE('',*,*,#29078,.T.);
#38641=ORIENTED_EDGE('',*,*,#29079,.F.);
#38642=ORIENTED_EDGE('',*,*,#29078,.F.);
#38643=ORIENTED_EDGE('',*,*,#29080,.F.);
#38644=ORIENTED_EDGE('',*,*,#29081,.T.);
#38645=ORIENTED_EDGE('',*,*,#29082,.F.);
#38646=ORIENTED_EDGE('',*,*,#29081,.F.);
#38647=ORIENTED_EDGE('',*,*,#29083,.T.);
#38648=ORIENTED_EDGE('',*,*,#29084,.T.);
#38649=ORIENTED_EDGE('',*,*,#29085,.F.);
#38650=ORIENTED_EDGE('',*,*,#29084,.F.);
#38651=ORIENTED_EDGE('',*,*,#29086,.F.);
#38652=ORIENTED_EDGE('',*,*,#29087,.T.);
#38653=ORIENTED_EDGE('',*,*,#29088,.F.);
#38654=ORIENTED_EDGE('',*,*,#29087,.F.);
#38655=ORIENTED_EDGE('',*,*,#29089,.T.);
#38656=ORIENTED_EDGE('',*,*,#29090,.T.);
#38657=ORIENTED_EDGE('',*,*,#29091,.F.);
#38658=ORIENTED_EDGE('',*,*,#29090,.F.);
#38659=ORIENTED_EDGE('',*,*,#29092,.F.);
#38660=ORIENTED_EDGE('',*,*,#29093,.T.);
#38661=ORIENTED_EDGE('',*,*,#29094,.F.);
#38662=ORIENTED_EDGE('',*,*,#29093,.F.);
#38663=ORIENTED_EDGE('',*,*,#29095,.T.);
#38664=ORIENTED_EDGE('',*,*,#29096,.T.);
#38665=ORIENTED_EDGE('',*,*,#29097,.F.);
#38666=ORIENTED_EDGE('',*,*,#29096,.F.);
#38667=ORIENTED_EDGE('',*,*,#29098,.F.);
#38668=ORIENTED_EDGE('',*,*,#29099,.T.);
#38669=ORIENTED_EDGE('',*,*,#29100,.F.);
#38670=ORIENTED_EDGE('',*,*,#29099,.F.);
#38671=ORIENTED_EDGE('',*,*,#29101,.T.);
#38672=ORIENTED_EDGE('',*,*,#29102,.T.);
#38673=ORIENTED_EDGE('',*,*,#29103,.F.);
#38674=ORIENTED_EDGE('',*,*,#29102,.F.);
#38675=ORIENTED_EDGE('',*,*,#29104,.F.);
#38676=ORIENTED_EDGE('',*,*,#29105,.T.);
#38677=ORIENTED_EDGE('',*,*,#29106,.F.);
#38678=ORIENTED_EDGE('',*,*,#29105,.F.);
#38679=ORIENTED_EDGE('',*,*,#29107,.T.);
#38680=ORIENTED_EDGE('',*,*,#29108,.T.);
#38681=ORIENTED_EDGE('',*,*,#29109,.F.);
#38682=ORIENTED_EDGE('',*,*,#29108,.F.);
#38683=ORIENTED_EDGE('',*,*,#29110,.F.);
#38684=ORIENTED_EDGE('',*,*,#29111,.T.);
#38685=ORIENTED_EDGE('',*,*,#29112,.F.);
#38686=ORIENTED_EDGE('',*,*,#29111,.F.);
#38687=ORIENTED_EDGE('',*,*,#29113,.T.);
#38688=ORIENTED_EDGE('',*,*,#29114,.T.);
#38689=ORIENTED_EDGE('',*,*,#29115,.F.);
#38690=ORIENTED_EDGE('',*,*,#29114,.F.);
#38691=ORIENTED_EDGE('',*,*,#29116,.F.);
#38692=ORIENTED_EDGE('',*,*,#29117,.T.);
#38693=ORIENTED_EDGE('',*,*,#29118,.F.);
#38694=ORIENTED_EDGE('',*,*,#29117,.F.);
#38695=ORIENTED_EDGE('',*,*,#29119,.T.);
#38696=ORIENTED_EDGE('',*,*,#29120,.T.);
#38697=ORIENTED_EDGE('',*,*,#29121,.F.);
#38698=ORIENTED_EDGE('',*,*,#29120,.F.);
#38699=ORIENTED_EDGE('',*,*,#29122,.F.);
#38700=ORIENTED_EDGE('',*,*,#29123,.T.);
#38701=ORIENTED_EDGE('',*,*,#29124,.F.);
#38702=ORIENTED_EDGE('',*,*,#29123,.F.);
#38703=ORIENTED_EDGE('',*,*,#29125,.T.);
#38704=ORIENTED_EDGE('',*,*,#29126,.T.);
#38705=ORIENTED_EDGE('',*,*,#29127,.F.);
#38706=ORIENTED_EDGE('',*,*,#29126,.F.);
#38707=ORIENTED_EDGE('',*,*,#29128,.F.);
#38708=ORIENTED_EDGE('',*,*,#29129,.T.);
#38709=ORIENTED_EDGE('',*,*,#29130,.F.);
#38710=ORIENTED_EDGE('',*,*,#29129,.F.);
#38711=ORIENTED_EDGE('',*,*,#29131,.T.);
#38712=ORIENTED_EDGE('',*,*,#29132,.T.);
#38713=ORIENTED_EDGE('',*,*,#29133,.F.);
#38714=ORIENTED_EDGE('',*,*,#29132,.F.);
#38715=ORIENTED_EDGE('',*,*,#29134,.F.);
#38716=ORIENTED_EDGE('',*,*,#29135,.T.);
#38717=ORIENTED_EDGE('',*,*,#29136,.F.);
#38718=ORIENTED_EDGE('',*,*,#29135,.F.);
#38719=ORIENTED_EDGE('',*,*,#29137,.T.);
#38720=ORIENTED_EDGE('',*,*,#29138,.T.);
#38721=ORIENTED_EDGE('',*,*,#29139,.F.);
#38722=ORIENTED_EDGE('',*,*,#29138,.F.);
#38723=ORIENTED_EDGE('',*,*,#29140,.F.);
#38724=ORIENTED_EDGE('',*,*,#29141,.T.);
#38725=ORIENTED_EDGE('',*,*,#29142,.F.);
#38726=ORIENTED_EDGE('',*,*,#29141,.F.);
#38727=ORIENTED_EDGE('',*,*,#29143,.T.);
#38728=ORIENTED_EDGE('',*,*,#29144,.T.);
#38729=ORIENTED_EDGE('',*,*,#29145,.F.);
#38730=ORIENTED_EDGE('',*,*,#29144,.F.);
#38731=ORIENTED_EDGE('',*,*,#29146,.F.);
#38732=ORIENTED_EDGE('',*,*,#29147,.T.);
#38733=ORIENTED_EDGE('',*,*,#29148,.F.);
#38734=ORIENTED_EDGE('',*,*,#29147,.F.);
#38735=ORIENTED_EDGE('',*,*,#29149,.T.);
#38736=ORIENTED_EDGE('',*,*,#29150,.T.);
#38737=ORIENTED_EDGE('',*,*,#29151,.F.);
#38738=ORIENTED_EDGE('',*,*,#29150,.F.);
#38739=ORIENTED_EDGE('',*,*,#29152,.F.);
#38740=ORIENTED_EDGE('',*,*,#29153,.T.);
#38741=ORIENTED_EDGE('',*,*,#29154,.F.);
#38742=ORIENTED_EDGE('',*,*,#29153,.F.);
#38743=ORIENTED_EDGE('',*,*,#29155,.T.);
#38744=ORIENTED_EDGE('',*,*,#29156,.T.);
#38745=ORIENTED_EDGE('',*,*,#29157,.F.);
#38746=ORIENTED_EDGE('',*,*,#29156,.F.);
#38747=ORIENTED_EDGE('',*,*,#29158,.F.);
#38748=ORIENTED_EDGE('',*,*,#29159,.T.);
#38749=ORIENTED_EDGE('',*,*,#29160,.F.);
#38750=ORIENTED_EDGE('',*,*,#29159,.F.);
#38751=ORIENTED_EDGE('',*,*,#29161,.T.);
#38752=ORIENTED_EDGE('',*,*,#29162,.T.);
#38753=ORIENTED_EDGE('',*,*,#29163,.F.);
#38754=ORIENTED_EDGE('',*,*,#29162,.F.);
#38755=ORIENTED_EDGE('',*,*,#29164,.F.);
#38756=ORIENTED_EDGE('',*,*,#29165,.T.);
#38757=ORIENTED_EDGE('',*,*,#29166,.F.);
#38758=ORIENTED_EDGE('',*,*,#29165,.F.);
#38759=ORIENTED_EDGE('',*,*,#29167,.T.);
#38760=ORIENTED_EDGE('',*,*,#29168,.T.);
#38761=ORIENTED_EDGE('',*,*,#29169,.F.);
#38762=ORIENTED_EDGE('',*,*,#29168,.F.);
#38763=ORIENTED_EDGE('',*,*,#29170,.F.);
#38764=ORIENTED_EDGE('',*,*,#29171,.T.);
#38765=ORIENTED_EDGE('',*,*,#29172,.F.);
#38766=ORIENTED_EDGE('',*,*,#29171,.F.);
#38767=ORIENTED_EDGE('',*,*,#29173,.T.);
#38768=ORIENTED_EDGE('',*,*,#29174,.T.);
#38769=ORIENTED_EDGE('',*,*,#29175,.F.);
#38770=ORIENTED_EDGE('',*,*,#29174,.F.);
#38771=ORIENTED_EDGE('',*,*,#29176,.F.);
#38772=ORIENTED_EDGE('',*,*,#29177,.T.);
#38773=ORIENTED_EDGE('',*,*,#29178,.F.);
#38774=ORIENTED_EDGE('',*,*,#29177,.F.);
#38775=ORIENTED_EDGE('',*,*,#29179,.T.);
#38776=ORIENTED_EDGE('',*,*,#29180,.T.);
#38777=ORIENTED_EDGE('',*,*,#29181,.F.);
#38778=ORIENTED_EDGE('',*,*,#29180,.F.);
#38779=ORIENTED_EDGE('',*,*,#29182,.F.);
#38780=ORIENTED_EDGE('',*,*,#29183,.T.);
#38781=ORIENTED_EDGE('',*,*,#29184,.F.);
#38782=ORIENTED_EDGE('',*,*,#29183,.F.);
#38783=ORIENTED_EDGE('',*,*,#29185,.T.);
#38784=ORIENTED_EDGE('',*,*,#29186,.T.);
#38785=ORIENTED_EDGE('',*,*,#29187,.F.);
#38786=ORIENTED_EDGE('',*,*,#29186,.F.);
#38787=ORIENTED_EDGE('',*,*,#29188,.F.);
#38788=ORIENTED_EDGE('',*,*,#29189,.T.);
#38789=ORIENTED_EDGE('',*,*,#29190,.F.);
#38790=ORIENTED_EDGE('',*,*,#29189,.F.);
#38791=ORIENTED_EDGE('',*,*,#29191,.T.);
#38792=ORIENTED_EDGE('',*,*,#29192,.T.);
#38793=ORIENTED_EDGE('',*,*,#29193,.F.);
#38794=ORIENTED_EDGE('',*,*,#29192,.F.);
#38795=ORIENTED_EDGE('',*,*,#29194,.F.);
#38796=ORIENTED_EDGE('',*,*,#29195,.T.);
#38797=ORIENTED_EDGE('',*,*,#29196,.F.);
#38798=ORIENTED_EDGE('',*,*,#29195,.F.);
#38799=ORIENTED_EDGE('',*,*,#29197,.T.);
#38800=ORIENTED_EDGE('',*,*,#29198,.T.);
#38801=ORIENTED_EDGE('',*,*,#29199,.F.);
#38802=ORIENTED_EDGE('',*,*,#29198,.F.);
#38803=ORIENTED_EDGE('',*,*,#29200,.F.);
#38804=ORIENTED_EDGE('',*,*,#29201,.T.);
#38805=ORIENTED_EDGE('',*,*,#29202,.F.);
#38806=ORIENTED_EDGE('',*,*,#29201,.F.);
#38807=ORIENTED_EDGE('',*,*,#29203,.T.);
#38808=ORIENTED_EDGE('',*,*,#29204,.T.);
#38809=ORIENTED_EDGE('',*,*,#29205,.F.);
#38810=ORIENTED_EDGE('',*,*,#29204,.F.);
#38811=ORIENTED_EDGE('',*,*,#29206,.F.);
#38812=ORIENTED_EDGE('',*,*,#29207,.T.);
#38813=ORIENTED_EDGE('',*,*,#29208,.F.);
#38814=ORIENTED_EDGE('',*,*,#29207,.F.);
#38815=ORIENTED_EDGE('',*,*,#29209,.T.);
#38816=ORIENTED_EDGE('',*,*,#29210,.T.);
#38817=ORIENTED_EDGE('',*,*,#29211,.F.);
#38818=ORIENTED_EDGE('',*,*,#29210,.F.);
#38819=ORIENTED_EDGE('',*,*,#29212,.F.);
#38820=ORIENTED_EDGE('',*,*,#29213,.T.);
#38821=ORIENTED_EDGE('',*,*,#29214,.F.);
#38822=ORIENTED_EDGE('',*,*,#29213,.F.);
#38823=ORIENTED_EDGE('',*,*,#29215,.T.);
#38824=ORIENTED_EDGE('',*,*,#29216,.T.);
#38825=ORIENTED_EDGE('',*,*,#29217,.F.);
#38826=ORIENTED_EDGE('',*,*,#29216,.F.);
#38827=ORIENTED_EDGE('',*,*,#29218,.F.);
#38828=ORIENTED_EDGE('',*,*,#29219,.T.);
#38829=ORIENTED_EDGE('',*,*,#29220,.F.);
#38830=ORIENTED_EDGE('',*,*,#29219,.F.);
#38831=ORIENTED_EDGE('',*,*,#29221,.T.);
#38832=ORIENTED_EDGE('',*,*,#29222,.T.);
#38833=ORIENTED_EDGE('',*,*,#29223,.F.);
#38834=ORIENTED_EDGE('',*,*,#29222,.F.);
#38835=ORIENTED_EDGE('',*,*,#29224,.F.);
#38836=ORIENTED_EDGE('',*,*,#29225,.T.);
#38837=ORIENTED_EDGE('',*,*,#29226,.F.);
#38838=ORIENTED_EDGE('',*,*,#29225,.F.);
#38839=ORIENTED_EDGE('',*,*,#29227,.T.);
#38840=ORIENTED_EDGE('',*,*,#29228,.T.);
#38841=ORIENTED_EDGE('',*,*,#29229,.F.);
#38842=ORIENTED_EDGE('',*,*,#29228,.F.);
#38843=ORIENTED_EDGE('',*,*,#29230,.F.);
#38844=ORIENTED_EDGE('',*,*,#29231,.T.);
#38845=ORIENTED_EDGE('',*,*,#29232,.F.);
#38846=ORIENTED_EDGE('',*,*,#29231,.F.);
#38847=ORIENTED_EDGE('',*,*,#29233,.T.);
#38848=ORIENTED_EDGE('',*,*,#29234,.T.);
#38849=ORIENTED_EDGE('',*,*,#29235,.F.);
#38850=ORIENTED_EDGE('',*,*,#29234,.F.);
#38851=ORIENTED_EDGE('',*,*,#29236,.F.);
#38852=ORIENTED_EDGE('',*,*,#29237,.T.);
#38853=ORIENTED_EDGE('',*,*,#29238,.F.);
#38854=ORIENTED_EDGE('',*,*,#29237,.F.);
#38855=ORIENTED_EDGE('',*,*,#29239,.T.);
#38856=ORIENTED_EDGE('',*,*,#29240,.T.);
#38857=ORIENTED_EDGE('',*,*,#29241,.F.);
#38858=ORIENTED_EDGE('',*,*,#29240,.F.);
#38859=ORIENTED_EDGE('',*,*,#29242,.F.);
#38860=ORIENTED_EDGE('',*,*,#29243,.T.);
#38861=ORIENTED_EDGE('',*,*,#29244,.F.);
#38862=ORIENTED_EDGE('',*,*,#29243,.F.);
#38863=ORIENTED_EDGE('',*,*,#29245,.T.);
#38864=ORIENTED_EDGE('',*,*,#29246,.T.);
#38865=ORIENTED_EDGE('',*,*,#29247,.F.);
#38866=ORIENTED_EDGE('',*,*,#29246,.F.);
#38867=ORIENTED_EDGE('',*,*,#29248,.F.);
#38868=ORIENTED_EDGE('',*,*,#29249,.T.);
#38869=ORIENTED_EDGE('',*,*,#29250,.F.);
#38870=ORIENTED_EDGE('',*,*,#29249,.F.);
#38871=ORIENTED_EDGE('',*,*,#29251,.T.);
#38872=ORIENTED_EDGE('',*,*,#29252,.T.);
#38873=ORIENTED_EDGE('',*,*,#29253,.F.);
#38874=ORIENTED_EDGE('',*,*,#29252,.F.);
#38875=ORIENTED_EDGE('',*,*,#29254,.F.);
#38876=ORIENTED_EDGE('',*,*,#29255,.T.);
#38877=ORIENTED_EDGE('',*,*,#29256,.F.);
#38878=ORIENTED_EDGE('',*,*,#29255,.F.);
#38879=ORIENTED_EDGE('',*,*,#29257,.T.);
#38880=ORIENTED_EDGE('',*,*,#29258,.T.);
#38881=ORIENTED_EDGE('',*,*,#29259,.F.);
#38882=ORIENTED_EDGE('',*,*,#29258,.F.);
#38883=ORIENTED_EDGE('',*,*,#29260,.F.);
#38884=ORIENTED_EDGE('',*,*,#29261,.T.);
#38885=ORIENTED_EDGE('',*,*,#29262,.F.);
#38886=ORIENTED_EDGE('',*,*,#29261,.F.);
#38887=ORIENTED_EDGE('',*,*,#29263,.T.);
#38888=ORIENTED_EDGE('',*,*,#29264,.T.);
#38889=ORIENTED_EDGE('',*,*,#29265,.F.);
#38890=ORIENTED_EDGE('',*,*,#29264,.F.);
#38891=ORIENTED_EDGE('',*,*,#29266,.F.);
#38892=ORIENTED_EDGE('',*,*,#29267,.T.);
#38893=ORIENTED_EDGE('',*,*,#29268,.F.);
#38894=ORIENTED_EDGE('',*,*,#29267,.F.);
#38895=ORIENTED_EDGE('',*,*,#29269,.T.);
#38896=ORIENTED_EDGE('',*,*,#29270,.T.);
#38897=ORIENTED_EDGE('',*,*,#29271,.F.);
#38898=ORIENTED_EDGE('',*,*,#29270,.F.);
#38899=ORIENTED_EDGE('',*,*,#29272,.F.);
#38900=ORIENTED_EDGE('',*,*,#29273,.T.);
#38901=ORIENTED_EDGE('',*,*,#29274,.F.);
#38902=ORIENTED_EDGE('',*,*,#29273,.F.);
#38903=ORIENTED_EDGE('',*,*,#29275,.T.);
#38904=ORIENTED_EDGE('',*,*,#29276,.T.);
#38905=ORIENTED_EDGE('',*,*,#29277,.F.);
#38906=ORIENTED_EDGE('',*,*,#29276,.F.);
#38907=ORIENTED_EDGE('',*,*,#29278,.F.);
#38908=ORIENTED_EDGE('',*,*,#29279,.T.);
#38909=ORIENTED_EDGE('',*,*,#29280,.F.);
#38910=ORIENTED_EDGE('',*,*,#29279,.F.);
#38911=ORIENTED_EDGE('',*,*,#29281,.T.);
#38912=ORIENTED_EDGE('',*,*,#29282,.T.);
#38913=ORIENTED_EDGE('',*,*,#29283,.F.);
#38914=ORIENTED_EDGE('',*,*,#29282,.F.);
#38915=ORIENTED_EDGE('',*,*,#29284,.F.);
#38916=ORIENTED_EDGE('',*,*,#29285,.T.);
#38917=ORIENTED_EDGE('',*,*,#29286,.F.);
#38918=ORIENTED_EDGE('',*,*,#29285,.F.);
#38919=ORIENTED_EDGE('',*,*,#29287,.T.);
#38920=ORIENTED_EDGE('',*,*,#29288,.T.);
#38921=ORIENTED_EDGE('',*,*,#29289,.F.);
#38922=ORIENTED_EDGE('',*,*,#29288,.F.);
#38923=ORIENTED_EDGE('',*,*,#29290,.F.);
#38924=ORIENTED_EDGE('',*,*,#29291,.T.);
#38925=ORIENTED_EDGE('',*,*,#29292,.F.);
#38926=ORIENTED_EDGE('',*,*,#29291,.F.);
#38927=ORIENTED_EDGE('',*,*,#29293,.T.);
#38928=ORIENTED_EDGE('',*,*,#29294,.T.);
#38929=ORIENTED_EDGE('',*,*,#29295,.F.);
#38930=ORIENTED_EDGE('',*,*,#29294,.F.);
#38931=ORIENTED_EDGE('',*,*,#29296,.F.);
#38932=ORIENTED_EDGE('',*,*,#29297,.T.);
#38933=ORIENTED_EDGE('',*,*,#29298,.F.);
#38934=ORIENTED_EDGE('',*,*,#29297,.F.);
#38935=ORIENTED_EDGE('',*,*,#29299,.T.);
#38936=ORIENTED_EDGE('',*,*,#29300,.T.);
#38937=ORIENTED_EDGE('',*,*,#29301,.F.);
#38938=ORIENTED_EDGE('',*,*,#29300,.F.);
#38939=ORIENTED_EDGE('',*,*,#29302,.F.);
#38940=ORIENTED_EDGE('',*,*,#29303,.T.);
#38941=ORIENTED_EDGE('',*,*,#29304,.F.);
#38942=ORIENTED_EDGE('',*,*,#29303,.F.);
#38943=ORIENTED_EDGE('',*,*,#29305,.T.);
#38944=ORIENTED_EDGE('',*,*,#29306,.T.);
#38945=ORIENTED_EDGE('',*,*,#29307,.F.);
#38946=ORIENTED_EDGE('',*,*,#29306,.F.);
#38947=ORIENTED_EDGE('',*,*,#29308,.F.);
#38948=ORIENTED_EDGE('',*,*,#29309,.T.);
#38949=ORIENTED_EDGE('',*,*,#29310,.F.);
#38950=ORIENTED_EDGE('',*,*,#29309,.F.);
#38951=ORIENTED_EDGE('',*,*,#29311,.T.);
#38952=ORIENTED_EDGE('',*,*,#29312,.T.);
#38953=ORIENTED_EDGE('',*,*,#29313,.F.);
#38954=ORIENTED_EDGE('',*,*,#29312,.F.);
#38955=ORIENTED_EDGE('',*,*,#29314,.F.);
#38956=ORIENTED_EDGE('',*,*,#29315,.T.);
#38957=ORIENTED_EDGE('',*,*,#29316,.F.);
#38958=ORIENTED_EDGE('',*,*,#29315,.F.);
#38959=ORIENTED_EDGE('',*,*,#29317,.T.);
#38960=ORIENTED_EDGE('',*,*,#29318,.T.);
#38961=ORIENTED_EDGE('',*,*,#29319,.F.);
#38962=ORIENTED_EDGE('',*,*,#29318,.F.);
#38963=ORIENTED_EDGE('',*,*,#29320,.F.);
#38964=ORIENTED_EDGE('',*,*,#29321,.T.);
#38965=ORIENTED_EDGE('',*,*,#29322,.F.);
#38966=ORIENTED_EDGE('',*,*,#29321,.F.);
#38967=ORIENTED_EDGE('',*,*,#29323,.T.);
#38968=ORIENTED_EDGE('',*,*,#29324,.T.);
#38969=ORIENTED_EDGE('',*,*,#29325,.F.);
#38970=ORIENTED_EDGE('',*,*,#29324,.F.);
#38971=ORIENTED_EDGE('',*,*,#29326,.F.);
#38972=ORIENTED_EDGE('',*,*,#29327,.T.);
#38973=ORIENTED_EDGE('',*,*,#29328,.F.);
#38974=ORIENTED_EDGE('',*,*,#29327,.F.);
#38975=ORIENTED_EDGE('',*,*,#29329,.T.);
#38976=ORIENTED_EDGE('',*,*,#29330,.T.);
#38977=ORIENTED_EDGE('',*,*,#29331,.F.);
#38978=ORIENTED_EDGE('',*,*,#29330,.F.);
#38979=ORIENTED_EDGE('',*,*,#29332,.F.);
#38980=ORIENTED_EDGE('',*,*,#29333,.T.);
#38981=ORIENTED_EDGE('',*,*,#29334,.F.);
#38982=ORIENTED_EDGE('',*,*,#29333,.F.);
#38983=ORIENTED_EDGE('',*,*,#29335,.T.);
#38984=ORIENTED_EDGE('',*,*,#29336,.T.);
#38985=ORIENTED_EDGE('',*,*,#29337,.F.);
#38986=ORIENTED_EDGE('',*,*,#29336,.F.);
#38987=ORIENTED_EDGE('',*,*,#29338,.F.);
#38988=ORIENTED_EDGE('',*,*,#29339,.T.);
#38989=ORIENTED_EDGE('',*,*,#29340,.F.);
#38990=ORIENTED_EDGE('',*,*,#29339,.F.);
#38991=ORIENTED_EDGE('',*,*,#29341,.T.);
#38992=ORIENTED_EDGE('',*,*,#29342,.T.);
#38993=ORIENTED_EDGE('',*,*,#29343,.F.);
#38994=ORIENTED_EDGE('',*,*,#29342,.F.);
#38995=ORIENTED_EDGE('',*,*,#29344,.F.);
#38996=ORIENTED_EDGE('',*,*,#29345,.T.);
#38997=ORIENTED_EDGE('',*,*,#29346,.F.);
#38998=ORIENTED_EDGE('',*,*,#29345,.F.);
#38999=ORIENTED_EDGE('',*,*,#29347,.T.);
#39000=ORIENTED_EDGE('',*,*,#29348,.T.);
#39001=ORIENTED_EDGE('',*,*,#29349,.F.);
#39002=ORIENTED_EDGE('',*,*,#29348,.F.);
#39003=ORIENTED_EDGE('',*,*,#29350,.F.);
#39004=ORIENTED_EDGE('',*,*,#29351,.T.);
#39005=ORIENTED_EDGE('',*,*,#29352,.F.);
#39006=ORIENTED_EDGE('',*,*,#29351,.F.);
#39007=ORIENTED_EDGE('',*,*,#29353,.T.);
#39008=ORIENTED_EDGE('',*,*,#29354,.T.);
#39009=ORIENTED_EDGE('',*,*,#29355,.F.);
#39010=ORIENTED_EDGE('',*,*,#29354,.F.);
#39011=ORIENTED_EDGE('',*,*,#29356,.F.);
#39012=ORIENTED_EDGE('',*,*,#29357,.T.);
#39013=ORIENTED_EDGE('',*,*,#29358,.F.);
#39014=ORIENTED_EDGE('',*,*,#29357,.F.);
#39015=ORIENTED_EDGE('',*,*,#29359,.T.);
#39016=ORIENTED_EDGE('',*,*,#29360,.T.);
#39017=ORIENTED_EDGE('',*,*,#29361,.F.);
#39018=ORIENTED_EDGE('',*,*,#29360,.F.);
#39019=ORIENTED_EDGE('',*,*,#29362,.F.);
#39020=ORIENTED_EDGE('',*,*,#29363,.T.);
#39021=ORIENTED_EDGE('',*,*,#29364,.F.);
#39022=ORIENTED_EDGE('',*,*,#29363,.F.);
#39023=ORIENTED_EDGE('',*,*,#29365,.T.);
#39024=ORIENTED_EDGE('',*,*,#29366,.T.);
#39025=ORIENTED_EDGE('',*,*,#29367,.F.);
#39026=ORIENTED_EDGE('',*,*,#29366,.F.);
#39027=ORIENTED_EDGE('',*,*,#29368,.F.);
#39028=ORIENTED_EDGE('',*,*,#29369,.T.);
#39029=ORIENTED_EDGE('',*,*,#29370,.F.);
#39030=ORIENTED_EDGE('',*,*,#29369,.F.);
#39031=ORIENTED_EDGE('',*,*,#29371,.T.);
#39032=ORIENTED_EDGE('',*,*,#29372,.T.);
#39033=ORIENTED_EDGE('',*,*,#29373,.F.);
#39034=ORIENTED_EDGE('',*,*,#29372,.F.);
#39035=ORIENTED_EDGE('',*,*,#29374,.F.);
#39036=ORIENTED_EDGE('',*,*,#29375,.T.);
#39037=ORIENTED_EDGE('',*,*,#29376,.F.);
#39038=ORIENTED_EDGE('',*,*,#29375,.F.);
#39039=ORIENTED_EDGE('',*,*,#29377,.T.);
#39040=ORIENTED_EDGE('',*,*,#29378,.T.);
#39041=ORIENTED_EDGE('',*,*,#29379,.F.);
#39042=ORIENTED_EDGE('',*,*,#29378,.F.);
#39043=ORIENTED_EDGE('',*,*,#29380,.F.);
#39044=ORIENTED_EDGE('',*,*,#29381,.T.);
#39045=ORIENTED_EDGE('',*,*,#29382,.F.);
#39046=ORIENTED_EDGE('',*,*,#29381,.F.);
#39047=ORIENTED_EDGE('',*,*,#29383,.T.);
#39048=ORIENTED_EDGE('',*,*,#29384,.T.);
#39049=ORIENTED_EDGE('',*,*,#29385,.F.);
#39050=ORIENTED_EDGE('',*,*,#29384,.F.);
#39051=ORIENTED_EDGE('',*,*,#29386,.F.);
#39052=ORIENTED_EDGE('',*,*,#29387,.T.);
#39053=ORIENTED_EDGE('',*,*,#29388,.F.);
#39054=ORIENTED_EDGE('',*,*,#29387,.F.);
#39055=ORIENTED_EDGE('',*,*,#29389,.T.);
#39056=ORIENTED_EDGE('',*,*,#29390,.T.);
#39057=ORIENTED_EDGE('',*,*,#29391,.F.);
#39058=ORIENTED_EDGE('',*,*,#29390,.F.);
#39059=ORIENTED_EDGE('',*,*,#29392,.F.);
#39060=ORIENTED_EDGE('',*,*,#29393,.T.);
#39061=ORIENTED_EDGE('',*,*,#29394,.F.);
#39062=ORIENTED_EDGE('',*,*,#29393,.F.);
#39063=ORIENTED_EDGE('',*,*,#29395,.T.);
#39064=ORIENTED_EDGE('',*,*,#29396,.T.);
#39065=ORIENTED_EDGE('',*,*,#29397,.F.);
#39066=ORIENTED_EDGE('',*,*,#29396,.F.);
#39067=ORIENTED_EDGE('',*,*,#29398,.F.);
#39068=ORIENTED_EDGE('',*,*,#29399,.T.);
#39069=ORIENTED_EDGE('',*,*,#29400,.F.);
#39070=ORIENTED_EDGE('',*,*,#29399,.F.);
#39071=ORIENTED_EDGE('',*,*,#29401,.T.);
#39072=ORIENTED_EDGE('',*,*,#29402,.T.);
#39073=ORIENTED_EDGE('',*,*,#29403,.F.);
#39074=ORIENTED_EDGE('',*,*,#29402,.F.);
#39075=ORIENTED_EDGE('',*,*,#29404,.F.);
#39076=ORIENTED_EDGE('',*,*,#29405,.T.);
#39077=ORIENTED_EDGE('',*,*,#29406,.F.);
#39078=ORIENTED_EDGE('',*,*,#29405,.F.);
#39079=ORIENTED_EDGE('',*,*,#29407,.T.);
#39080=ORIENTED_EDGE('',*,*,#29408,.T.);
#39081=ORIENTED_EDGE('',*,*,#29409,.F.);
#39082=ORIENTED_EDGE('',*,*,#29408,.F.);
#39083=ORIENTED_EDGE('',*,*,#29410,.F.);
#39084=ORIENTED_EDGE('',*,*,#29411,.T.);
#39085=ORIENTED_EDGE('',*,*,#29412,.F.);
#39086=ORIENTED_EDGE('',*,*,#29411,.F.);
#39087=ORIENTED_EDGE('',*,*,#29413,.T.);
#39088=ORIENTED_EDGE('',*,*,#29414,.T.);
#39089=ORIENTED_EDGE('',*,*,#29415,.F.);
#39090=ORIENTED_EDGE('',*,*,#29414,.F.);
#39091=ORIENTED_EDGE('',*,*,#29416,.F.);
#39092=ORIENTED_EDGE('',*,*,#29417,.T.);
#39093=ORIENTED_EDGE('',*,*,#29418,.F.);
#39094=ORIENTED_EDGE('',*,*,#29417,.F.);
#39095=ORIENTED_EDGE('',*,*,#29419,.T.);
#39096=ORIENTED_EDGE('',*,*,#29420,.T.);
#39097=ORIENTED_EDGE('',*,*,#29421,.F.);
#39098=ORIENTED_EDGE('',*,*,#29420,.F.);
#39099=ORIENTED_EDGE('',*,*,#29422,.F.);
#39100=ORIENTED_EDGE('',*,*,#29423,.T.);
#39101=ORIENTED_EDGE('',*,*,#29424,.F.);
#39102=ORIENTED_EDGE('',*,*,#29423,.F.);
#39103=ORIENTED_EDGE('',*,*,#29425,.T.);
#39104=ORIENTED_EDGE('',*,*,#29426,.T.);
#39105=ORIENTED_EDGE('',*,*,#29427,.F.);
#39106=ORIENTED_EDGE('',*,*,#29426,.F.);
#39107=ORIENTED_EDGE('',*,*,#29428,.F.);
#39108=ORIENTED_EDGE('',*,*,#29429,.T.);
#39109=ORIENTED_EDGE('',*,*,#29430,.F.);
#39110=ORIENTED_EDGE('',*,*,#29429,.F.);
#39111=ORIENTED_EDGE('',*,*,#29431,.T.);
#39112=ORIENTED_EDGE('',*,*,#29432,.T.);
#39113=ORIENTED_EDGE('',*,*,#29433,.F.);
#39114=ORIENTED_EDGE('',*,*,#29432,.F.);
#39115=ORIENTED_EDGE('',*,*,#29434,.F.);
#39116=ORIENTED_EDGE('',*,*,#29435,.T.);
#39117=ORIENTED_EDGE('',*,*,#29436,.F.);
#39118=ORIENTED_EDGE('',*,*,#29435,.F.);
#39119=ORIENTED_EDGE('',*,*,#29437,.T.);
#39120=ORIENTED_EDGE('',*,*,#29438,.T.);
#39121=ORIENTED_EDGE('',*,*,#29439,.F.);
#39122=ORIENTED_EDGE('',*,*,#29438,.F.);
#39123=ORIENTED_EDGE('',*,*,#29440,.F.);
#39124=ORIENTED_EDGE('',*,*,#29441,.T.);
#39125=ORIENTED_EDGE('',*,*,#29442,.F.);
#39126=ORIENTED_EDGE('',*,*,#29441,.F.);
#39127=ORIENTED_EDGE('',*,*,#29443,.T.);
#39128=ORIENTED_EDGE('',*,*,#29444,.T.);
#39129=ORIENTED_EDGE('',*,*,#29445,.F.);
#39130=ORIENTED_EDGE('',*,*,#29444,.F.);
#39131=ORIENTED_EDGE('',*,*,#29446,.F.);
#39132=ORIENTED_EDGE('',*,*,#29447,.T.);
#39133=ORIENTED_EDGE('',*,*,#29448,.F.);
#39134=ORIENTED_EDGE('',*,*,#29447,.F.);
#39135=ORIENTED_EDGE('',*,*,#29449,.T.);
#39136=ORIENTED_EDGE('',*,*,#29450,.T.);
#39137=ORIENTED_EDGE('',*,*,#29451,.F.);
#39138=ORIENTED_EDGE('',*,*,#29450,.F.);
#39139=ORIENTED_EDGE('',*,*,#29452,.F.);
#39140=ORIENTED_EDGE('',*,*,#29453,.T.);
#39141=ORIENTED_EDGE('',*,*,#29454,.F.);
#39142=ORIENTED_EDGE('',*,*,#29453,.F.);
#39143=ORIENTED_EDGE('',*,*,#29455,.T.);
#39144=ORIENTED_EDGE('',*,*,#29456,.T.);
#39145=ORIENTED_EDGE('',*,*,#29457,.F.);
#39146=ORIENTED_EDGE('',*,*,#29456,.F.);
#39147=ORIENTED_EDGE('',*,*,#29458,.F.);
#39148=ORIENTED_EDGE('',*,*,#29459,.T.);
#39149=ORIENTED_EDGE('',*,*,#29460,.F.);
#39150=ORIENTED_EDGE('',*,*,#29459,.F.);
#39151=ORIENTED_EDGE('',*,*,#29461,.T.);
#39152=ORIENTED_EDGE('',*,*,#29462,.T.);
#39153=ORIENTED_EDGE('',*,*,#29463,.F.);
#39154=ORIENTED_EDGE('',*,*,#29462,.F.);
#39155=ORIENTED_EDGE('',*,*,#29464,.F.);
#39156=ORIENTED_EDGE('',*,*,#29465,.T.);
#39157=ORIENTED_EDGE('',*,*,#29466,.F.);
#39158=ORIENTED_EDGE('',*,*,#29465,.F.);
#39159=ORIENTED_EDGE('',*,*,#29467,.T.);
#39160=ORIENTED_EDGE('',*,*,#29468,.T.);
#39161=ORIENTED_EDGE('',*,*,#29469,.F.);
#39162=ORIENTED_EDGE('',*,*,#29468,.F.);
#39163=ORIENTED_EDGE('',*,*,#29470,.F.);
#39164=ORIENTED_EDGE('',*,*,#29471,.T.);
#39165=ORIENTED_EDGE('',*,*,#29472,.F.);
#39166=ORIENTED_EDGE('',*,*,#29471,.F.);
#39167=ORIENTED_EDGE('',*,*,#29473,.T.);
#39168=ORIENTED_EDGE('',*,*,#29474,.T.);
#39169=ORIENTED_EDGE('',*,*,#29475,.F.);
#39170=ORIENTED_EDGE('',*,*,#29474,.F.);
#39171=ORIENTED_EDGE('',*,*,#29476,.F.);
#39172=ORIENTED_EDGE('',*,*,#29477,.T.);
#39173=ORIENTED_EDGE('',*,*,#29478,.F.);
#39174=ORIENTED_EDGE('',*,*,#29477,.F.);
#39175=ORIENTED_EDGE('',*,*,#29479,.T.);
#39176=ORIENTED_EDGE('',*,*,#29480,.T.);
#39177=ORIENTED_EDGE('',*,*,#29481,.F.);
#39178=ORIENTED_EDGE('',*,*,#29480,.F.);
#39179=ORIENTED_EDGE('',*,*,#29482,.F.);
#39180=ORIENTED_EDGE('',*,*,#29483,.T.);
#39181=ORIENTED_EDGE('',*,*,#29484,.F.);
#39182=ORIENTED_EDGE('',*,*,#29483,.F.);
#39183=ORIENTED_EDGE('',*,*,#29485,.T.);
#39184=ORIENTED_EDGE('',*,*,#29486,.T.);
#39185=ORIENTED_EDGE('',*,*,#29487,.F.);
#39186=ORIENTED_EDGE('',*,*,#29486,.F.);
#39187=ORIENTED_EDGE('',*,*,#29488,.F.);
#39188=ORIENTED_EDGE('',*,*,#29489,.T.);
#39189=ORIENTED_EDGE('',*,*,#29490,.F.);
#39190=ORIENTED_EDGE('',*,*,#29489,.F.);
#39191=ORIENTED_EDGE('',*,*,#29491,.T.);
#39192=ORIENTED_EDGE('',*,*,#29492,.T.);
#39193=ORIENTED_EDGE('',*,*,#29493,.F.);
#39194=ORIENTED_EDGE('',*,*,#29492,.F.);
#39195=ORIENTED_EDGE('',*,*,#29494,.F.);
#39196=ORIENTED_EDGE('',*,*,#29495,.T.);
#39197=ORIENTED_EDGE('',*,*,#29496,.F.);
#39198=ORIENTED_EDGE('',*,*,#29495,.F.);
#39199=ORIENTED_EDGE('',*,*,#29497,.T.);
#39200=ORIENTED_EDGE('',*,*,#29498,.T.);
#39201=ORIENTED_EDGE('',*,*,#29499,.F.);
#39202=ORIENTED_EDGE('',*,*,#29498,.F.);
#39203=ORIENTED_EDGE('',*,*,#29500,.F.);
#39204=ORIENTED_EDGE('',*,*,#29501,.T.);
#39205=ORIENTED_EDGE('',*,*,#29502,.F.);
#39206=ORIENTED_EDGE('',*,*,#29501,.F.);
#39207=ORIENTED_EDGE('',*,*,#29503,.T.);
#39208=ORIENTED_EDGE('',*,*,#29504,.T.);
#39209=ORIENTED_EDGE('',*,*,#29505,.F.);
#39210=ORIENTED_EDGE('',*,*,#29504,.F.);
#39211=ORIENTED_EDGE('',*,*,#29506,.F.);
#39212=ORIENTED_EDGE('',*,*,#29507,.T.);
#39213=ORIENTED_EDGE('',*,*,#29508,.F.);
#39214=ORIENTED_EDGE('',*,*,#29507,.F.);
#39215=ORIENTED_EDGE('',*,*,#29509,.T.);
#39216=ORIENTED_EDGE('',*,*,#29510,.T.);
#39217=ORIENTED_EDGE('',*,*,#29511,.F.);
#39218=ORIENTED_EDGE('',*,*,#29510,.F.);
#39219=ORIENTED_EDGE('',*,*,#29512,.F.);
#39220=ORIENTED_EDGE('',*,*,#29513,.T.);
#39221=ORIENTED_EDGE('',*,*,#29514,.F.);
#39222=ORIENTED_EDGE('',*,*,#29513,.F.);
#39223=ORIENTED_EDGE('',*,*,#29515,.T.);
#39224=ORIENTED_EDGE('',*,*,#29516,.T.);
#39225=ORIENTED_EDGE('',*,*,#29517,.F.);
#39226=ORIENTED_EDGE('',*,*,#29516,.F.);
#39227=ORIENTED_EDGE('',*,*,#29518,.F.);
#39228=ORIENTED_EDGE('',*,*,#29519,.T.);
#39229=ORIENTED_EDGE('',*,*,#29520,.F.);
#39230=ORIENTED_EDGE('',*,*,#29519,.F.);
#39231=ORIENTED_EDGE('',*,*,#29521,.T.);
#39232=ORIENTED_EDGE('',*,*,#29522,.T.);
#39233=ORIENTED_EDGE('',*,*,#29523,.F.);
#39234=ORIENTED_EDGE('',*,*,#29522,.F.);
#39235=ORIENTED_EDGE('',*,*,#29524,.F.);
#39236=ORIENTED_EDGE('',*,*,#29525,.T.);
#39237=ORIENTED_EDGE('',*,*,#29526,.F.);
#39238=ORIENTED_EDGE('',*,*,#29525,.F.);
#39239=ORIENTED_EDGE('',*,*,#29527,.T.);
#39240=ORIENTED_EDGE('',*,*,#29528,.T.);
#39241=ORIENTED_EDGE('',*,*,#29529,.F.);
#39242=ORIENTED_EDGE('',*,*,#29528,.F.);
#39243=ORIENTED_EDGE('',*,*,#29530,.F.);
#39244=ORIENTED_EDGE('',*,*,#29531,.T.);
#39245=ORIENTED_EDGE('',*,*,#29532,.F.);
#39246=ORIENTED_EDGE('',*,*,#29531,.F.);
#39247=ORIENTED_EDGE('',*,*,#29533,.T.);
#39248=ORIENTED_EDGE('',*,*,#29534,.T.);
#39249=ORIENTED_EDGE('',*,*,#29535,.F.);
#39250=ORIENTED_EDGE('',*,*,#29534,.F.);
#39251=ORIENTED_EDGE('',*,*,#29536,.F.);
#39252=ORIENTED_EDGE('',*,*,#29537,.T.);
#39253=ORIENTED_EDGE('',*,*,#29538,.F.);
#39254=ORIENTED_EDGE('',*,*,#29537,.F.);
#39255=ORIENTED_EDGE('',*,*,#29539,.T.);
#39256=ORIENTED_EDGE('',*,*,#29540,.T.);
#39257=ORIENTED_EDGE('',*,*,#29541,.F.);
#39258=ORIENTED_EDGE('',*,*,#29540,.F.);
#39259=ORIENTED_EDGE('',*,*,#29542,.F.);
#39260=ORIENTED_EDGE('',*,*,#29543,.T.);
#39261=ORIENTED_EDGE('',*,*,#29544,.F.);
#39262=ORIENTED_EDGE('',*,*,#29543,.F.);
#39263=ORIENTED_EDGE('',*,*,#29545,.T.);
#39264=ORIENTED_EDGE('',*,*,#29546,.T.);
#39265=ORIENTED_EDGE('',*,*,#29547,.F.);
#39266=ORIENTED_EDGE('',*,*,#29546,.F.);
#39267=ORIENTED_EDGE('',*,*,#29548,.F.);
#39268=ORIENTED_EDGE('',*,*,#29549,.T.);
#39269=ORIENTED_EDGE('',*,*,#29550,.F.);
#39270=ORIENTED_EDGE('',*,*,#29549,.F.);
#39271=ORIENTED_EDGE('',*,*,#29551,.T.);
#39272=ORIENTED_EDGE('',*,*,#29552,.T.);
#39273=ORIENTED_EDGE('',*,*,#29553,.F.);
#39274=ORIENTED_EDGE('',*,*,#29552,.F.);
#39275=ORIENTED_EDGE('',*,*,#29554,.F.);
#39276=ORIENTED_EDGE('',*,*,#29555,.T.);
#39277=ORIENTED_EDGE('',*,*,#29556,.F.);
#39278=ORIENTED_EDGE('',*,*,#29555,.F.);
#39279=ORIENTED_EDGE('',*,*,#29557,.T.);
#39280=ORIENTED_EDGE('',*,*,#29558,.T.);
#39281=ORIENTED_EDGE('',*,*,#29559,.F.);
#39282=ORIENTED_EDGE('',*,*,#29558,.F.);
#39283=ORIENTED_EDGE('',*,*,#29560,.F.);
#39284=ORIENTED_EDGE('',*,*,#29561,.T.);
#39285=ORIENTED_EDGE('',*,*,#29562,.F.);
#39286=ORIENTED_EDGE('',*,*,#29561,.F.);
#39287=ORIENTED_EDGE('',*,*,#29563,.T.);
#39288=ORIENTED_EDGE('',*,*,#29564,.T.);
#39289=ORIENTED_EDGE('',*,*,#29565,.F.);
#39290=ORIENTED_EDGE('',*,*,#29564,.F.);
#39291=ORIENTED_EDGE('',*,*,#29566,.F.);
#39292=ORIENTED_EDGE('',*,*,#29567,.T.);
#39293=ORIENTED_EDGE('',*,*,#29568,.F.);
#39294=ORIENTED_EDGE('',*,*,#29567,.F.);
#39295=ORIENTED_EDGE('',*,*,#29569,.T.);
#39296=ORIENTED_EDGE('',*,*,#29570,.T.);
#39297=ORIENTED_EDGE('',*,*,#29571,.F.);
#39298=ORIENTED_EDGE('',*,*,#29570,.F.);
#39299=ORIENTED_EDGE('',*,*,#29572,.F.);
#39300=ORIENTED_EDGE('',*,*,#29573,.T.);
#39301=ORIENTED_EDGE('',*,*,#29574,.F.);
#39302=ORIENTED_EDGE('',*,*,#29573,.F.);
#39303=ORIENTED_EDGE('',*,*,#29575,.T.);
#39304=ORIENTED_EDGE('',*,*,#29576,.T.);
#39305=ORIENTED_EDGE('',*,*,#29577,.F.);
#39306=ORIENTED_EDGE('',*,*,#29576,.F.);
#39307=ORIENTED_EDGE('',*,*,#29578,.F.);
#39308=ORIENTED_EDGE('',*,*,#29579,.T.);
#39309=ORIENTED_EDGE('',*,*,#29580,.F.);
#39310=ORIENTED_EDGE('',*,*,#29579,.F.);
#39311=ORIENTED_EDGE('',*,*,#29581,.T.);
#39312=ORIENTED_EDGE('',*,*,#29582,.T.);
#39313=ORIENTED_EDGE('',*,*,#29583,.F.);
#39314=ORIENTED_EDGE('',*,*,#29582,.F.);
#39315=ORIENTED_EDGE('',*,*,#29584,.F.);
#39316=ORIENTED_EDGE('',*,*,#29585,.T.);
#39317=ORIENTED_EDGE('',*,*,#29586,.F.);
#39318=ORIENTED_EDGE('',*,*,#29585,.F.);
#39319=ORIENTED_EDGE('',*,*,#29587,.T.);
#39320=ORIENTED_EDGE('',*,*,#29588,.T.);
#39321=ORIENTED_EDGE('',*,*,#29589,.F.);
#39322=ORIENTED_EDGE('',*,*,#29588,.F.);
#39323=ORIENTED_EDGE('',*,*,#29590,.F.);
#39324=ORIENTED_EDGE('',*,*,#29591,.T.);
#39325=ORIENTED_EDGE('',*,*,#29592,.F.);
#39326=ORIENTED_EDGE('',*,*,#29591,.F.);
#39327=ORIENTED_EDGE('',*,*,#29593,.T.);
#39328=ORIENTED_EDGE('',*,*,#29594,.T.);
#39329=ORIENTED_EDGE('',*,*,#29595,.F.);
#39330=ORIENTED_EDGE('',*,*,#29594,.F.);
#39331=ORIENTED_EDGE('',*,*,#29596,.F.);
#39332=ORIENTED_EDGE('',*,*,#29597,.T.);
#39333=ORIENTED_EDGE('',*,*,#29598,.F.);
#39334=ORIENTED_EDGE('',*,*,#29597,.F.);
#39335=ORIENTED_EDGE('',*,*,#29599,.T.);
#39336=ORIENTED_EDGE('',*,*,#29600,.T.);
#39337=ORIENTED_EDGE('',*,*,#29601,.F.);
#39338=ORIENTED_EDGE('',*,*,#29600,.F.);
#39339=ORIENTED_EDGE('',*,*,#29602,.F.);
#39340=ORIENTED_EDGE('',*,*,#29603,.T.);
#39341=ORIENTED_EDGE('',*,*,#29604,.F.);
#39342=ORIENTED_EDGE('',*,*,#29603,.F.);
#39343=ORIENTED_EDGE('',*,*,#29605,.T.);
#39344=ORIENTED_EDGE('',*,*,#29606,.T.);
#39345=ORIENTED_EDGE('',*,*,#29607,.F.);
#39346=ORIENTED_EDGE('',*,*,#29606,.F.);
#39347=ORIENTED_EDGE('',*,*,#29608,.F.);
#39348=ORIENTED_EDGE('',*,*,#29609,.T.);
#39349=ORIENTED_EDGE('',*,*,#29610,.F.);
#39350=ORIENTED_EDGE('',*,*,#29609,.F.);
#39351=ORIENTED_EDGE('',*,*,#29611,.T.);
#39352=ORIENTED_EDGE('',*,*,#29612,.T.);
#39353=ORIENTED_EDGE('',*,*,#29613,.F.);
#39354=ORIENTED_EDGE('',*,*,#29612,.F.);
#39355=ORIENTED_EDGE('',*,*,#29614,.F.);
#39356=ORIENTED_EDGE('',*,*,#29615,.T.);
#39357=ORIENTED_EDGE('',*,*,#29616,.F.);
#39358=ORIENTED_EDGE('',*,*,#29615,.F.);
#39359=ORIENTED_EDGE('',*,*,#29617,.T.);
#39360=ORIENTED_EDGE('',*,*,#29618,.T.);
#39361=ORIENTED_EDGE('',*,*,#29619,.F.);
#39362=ORIENTED_EDGE('',*,*,#29618,.F.);
#39363=ORIENTED_EDGE('',*,*,#29620,.F.);
#39364=ORIENTED_EDGE('',*,*,#29621,.T.);
#39365=ORIENTED_EDGE('',*,*,#29622,.F.);
#39366=ORIENTED_EDGE('',*,*,#29621,.F.);
#39367=ORIENTED_EDGE('',*,*,#29623,.T.);
#39368=ORIENTED_EDGE('',*,*,#29624,.T.);
#39369=ORIENTED_EDGE('',*,*,#29625,.F.);
#39370=ORIENTED_EDGE('',*,*,#29624,.F.);
#39371=ORIENTED_EDGE('',*,*,#29626,.F.);
#39372=ORIENTED_EDGE('',*,*,#29627,.T.);
#39373=ORIENTED_EDGE('',*,*,#29628,.F.);
#39374=ORIENTED_EDGE('',*,*,#29627,.F.);
#39375=ORIENTED_EDGE('',*,*,#29629,.T.);
#39376=ORIENTED_EDGE('',*,*,#29630,.T.);
#39377=ORIENTED_EDGE('',*,*,#29631,.F.);
#39378=ORIENTED_EDGE('',*,*,#29630,.F.);
#39379=ORIENTED_EDGE('',*,*,#29632,.F.);
#39380=ORIENTED_EDGE('',*,*,#29633,.T.);
#39381=ORIENTED_EDGE('',*,*,#29634,.F.);
#39382=ORIENTED_EDGE('',*,*,#29633,.F.);
#39383=ORIENTED_EDGE('',*,*,#29635,.T.);
#39384=ORIENTED_EDGE('',*,*,#29636,.T.);
#39385=ORIENTED_EDGE('',*,*,#29637,.F.);
#39386=ORIENTED_EDGE('',*,*,#29636,.F.);
#39387=ORIENTED_EDGE('',*,*,#29638,.F.);
#39388=ORIENTED_EDGE('',*,*,#29639,.T.);
#39389=ORIENTED_EDGE('',*,*,#29640,.F.);
#39390=ORIENTED_EDGE('',*,*,#29639,.F.);
#39391=ORIENTED_EDGE('',*,*,#29641,.T.);
#39392=ORIENTED_EDGE('',*,*,#29642,.T.);
#39393=ORIENTED_EDGE('',*,*,#29643,.F.);
#39394=ORIENTED_EDGE('',*,*,#29642,.F.);
#39395=ORIENTED_EDGE('',*,*,#29644,.F.);
#39396=ORIENTED_EDGE('',*,*,#29645,.T.);
#39397=ORIENTED_EDGE('',*,*,#29646,.F.);
#39398=ORIENTED_EDGE('',*,*,#29645,.F.);
#39399=ORIENTED_EDGE('',*,*,#29647,.T.);
#39400=ORIENTED_EDGE('',*,*,#29648,.T.);
#39401=ORIENTED_EDGE('',*,*,#29649,.F.);
#39402=ORIENTED_EDGE('',*,*,#29648,.F.);
#39403=ORIENTED_EDGE('',*,*,#29650,.F.);
#39404=ORIENTED_EDGE('',*,*,#29651,.T.);
#39405=ORIENTED_EDGE('',*,*,#29652,.F.);
#39406=ORIENTED_EDGE('',*,*,#29651,.F.);
#39407=ORIENTED_EDGE('',*,*,#29653,.T.);
#39408=ORIENTED_EDGE('',*,*,#29654,.T.);
#39409=ORIENTED_EDGE('',*,*,#29655,.F.);
#39410=ORIENTED_EDGE('',*,*,#29654,.F.);
#39411=ORIENTED_EDGE('',*,*,#29656,.F.);
#39412=ORIENTED_EDGE('',*,*,#29657,.T.);
#39413=ORIENTED_EDGE('',*,*,#29658,.F.);
#39414=ORIENTED_EDGE('',*,*,#29657,.F.);
#39415=ORIENTED_EDGE('',*,*,#29659,.T.);
#39416=ORIENTED_EDGE('',*,*,#29660,.T.);
#39417=ORIENTED_EDGE('',*,*,#29661,.F.);
#39418=ORIENTED_EDGE('',*,*,#29660,.F.);
#39419=ORIENTED_EDGE('',*,*,#29662,.F.);
#39420=ORIENTED_EDGE('',*,*,#29663,.T.);
#39421=ORIENTED_EDGE('',*,*,#29664,.F.);
#39422=ORIENTED_EDGE('',*,*,#29663,.F.);
#39423=ORIENTED_EDGE('',*,*,#29665,.T.);
#39424=ORIENTED_EDGE('',*,*,#29666,.T.);
#39425=ORIENTED_EDGE('',*,*,#29667,.F.);
#39426=ORIENTED_EDGE('',*,*,#29666,.F.);
#39427=ORIENTED_EDGE('',*,*,#29668,.F.);
#39428=ORIENTED_EDGE('',*,*,#29669,.T.);
#39429=ORIENTED_EDGE('',*,*,#29670,.F.);
#39430=ORIENTED_EDGE('',*,*,#29669,.F.);
#39431=ORIENTED_EDGE('',*,*,#29671,.T.);
#39432=ORIENTED_EDGE('',*,*,#29672,.T.);
#39433=ORIENTED_EDGE('',*,*,#29673,.F.);
#39434=ORIENTED_EDGE('',*,*,#29672,.F.);
#39435=ORIENTED_EDGE('',*,*,#29674,.F.);
#39436=ORIENTED_EDGE('',*,*,#29675,.T.);
#39437=ORIENTED_EDGE('',*,*,#29676,.F.);
#39438=ORIENTED_EDGE('',*,*,#29675,.F.);
#39439=ORIENTED_EDGE('',*,*,#29677,.T.);
#39440=ORIENTED_EDGE('',*,*,#29678,.T.);
#39441=ORIENTED_EDGE('',*,*,#29679,.F.);
#39442=ORIENTED_EDGE('',*,*,#29678,.F.);
#39443=ORIENTED_EDGE('',*,*,#29680,.F.);
#39444=ORIENTED_EDGE('',*,*,#29681,.T.);
#39445=ORIENTED_EDGE('',*,*,#29682,.F.);
#39446=ORIENTED_EDGE('',*,*,#29681,.F.);
#39447=ORIENTED_EDGE('',*,*,#29683,.T.);
#39448=ORIENTED_EDGE('',*,*,#29684,.T.);
#39449=ORIENTED_EDGE('',*,*,#29685,.F.);
#39450=ORIENTED_EDGE('',*,*,#29684,.F.);
#39451=ORIENTED_EDGE('',*,*,#29686,.F.);
#39452=ORIENTED_EDGE('',*,*,#29687,.T.);
#39453=ORIENTED_EDGE('',*,*,#29688,.F.);
#39454=ORIENTED_EDGE('',*,*,#29687,.F.);
#39455=ORIENTED_EDGE('',*,*,#29689,.T.);
#39456=ORIENTED_EDGE('',*,*,#29690,.T.);
#39457=ORIENTED_EDGE('',*,*,#29691,.F.);
#39458=ORIENTED_EDGE('',*,*,#29690,.F.);
#39459=ORIENTED_EDGE('',*,*,#29692,.F.);
#39460=ORIENTED_EDGE('',*,*,#29693,.T.);
#39461=ORIENTED_EDGE('',*,*,#29694,.F.);
#39462=ORIENTED_EDGE('',*,*,#29693,.F.);
#39463=ORIENTED_EDGE('',*,*,#29695,.T.);
#39464=ORIENTED_EDGE('',*,*,#29696,.T.);
#39465=ORIENTED_EDGE('',*,*,#29697,.F.);
#39466=ORIENTED_EDGE('',*,*,#29696,.F.);
#39467=ORIENTED_EDGE('',*,*,#29698,.F.);
#39468=ORIENTED_EDGE('',*,*,#29699,.T.);
#39469=ORIENTED_EDGE('',*,*,#29700,.F.);
#39470=ORIENTED_EDGE('',*,*,#29699,.F.);
#39471=ORIENTED_EDGE('',*,*,#29701,.T.);
#39472=ORIENTED_EDGE('',*,*,#29702,.T.);
#39473=ORIENTED_EDGE('',*,*,#29703,.F.);
#39474=ORIENTED_EDGE('',*,*,#29702,.F.);
#39475=ORIENTED_EDGE('',*,*,#29704,.F.);
#39476=ORIENTED_EDGE('',*,*,#29705,.T.);
#39477=ORIENTED_EDGE('',*,*,#29706,.F.);
#39478=ORIENTED_EDGE('',*,*,#29705,.F.);
#39479=ORIENTED_EDGE('',*,*,#29707,.T.);
#39480=ORIENTED_EDGE('',*,*,#29708,.T.);
#39481=ORIENTED_EDGE('',*,*,#29709,.F.);
#39482=ORIENTED_EDGE('',*,*,#29708,.F.);
#39483=ORIENTED_EDGE('',*,*,#29710,.F.);
#39484=ORIENTED_EDGE('',*,*,#29711,.T.);
#39485=ORIENTED_EDGE('',*,*,#29712,.F.);
#39486=ORIENTED_EDGE('',*,*,#29711,.F.);
#39487=ORIENTED_EDGE('',*,*,#29713,.T.);
#39488=ORIENTED_EDGE('',*,*,#29714,.T.);
#39489=ORIENTED_EDGE('',*,*,#29715,.F.);
#39490=ORIENTED_EDGE('',*,*,#29714,.F.);
#39491=ORIENTED_EDGE('',*,*,#29716,.F.);
#39492=ORIENTED_EDGE('',*,*,#29717,.T.);
#39493=ORIENTED_EDGE('',*,*,#29718,.F.);
#39494=ORIENTED_EDGE('',*,*,#29717,.F.);
#39495=ORIENTED_EDGE('',*,*,#29719,.T.);
#39496=ORIENTED_EDGE('',*,*,#29720,.T.);
#39497=ORIENTED_EDGE('',*,*,#29721,.F.);
#39498=ORIENTED_EDGE('',*,*,#29720,.F.);
#39499=ORIENTED_EDGE('',*,*,#29722,.F.);
#39500=ORIENTED_EDGE('',*,*,#29723,.T.);
#39501=ORIENTED_EDGE('',*,*,#29724,.F.);
#39502=ORIENTED_EDGE('',*,*,#29723,.F.);
#39503=ORIENTED_EDGE('',*,*,#29725,.T.);
#39504=ORIENTED_EDGE('',*,*,#29726,.T.);
#39505=ORIENTED_EDGE('',*,*,#29727,.F.);
#39506=ORIENTED_EDGE('',*,*,#29726,.F.);
#39507=ORIENTED_EDGE('',*,*,#29728,.F.);
#39508=ORIENTED_EDGE('',*,*,#29729,.T.);
#39509=ORIENTED_EDGE('',*,*,#29730,.F.);
#39510=ORIENTED_EDGE('',*,*,#29729,.F.);
#39511=ORIENTED_EDGE('',*,*,#29731,.T.);
#39512=ORIENTED_EDGE('',*,*,#29732,.T.);
#39513=ORIENTED_EDGE('',*,*,#29733,.F.);
#39514=ORIENTED_EDGE('',*,*,#29732,.F.);
#39515=ORIENTED_EDGE('',*,*,#29734,.F.);
#39516=ORIENTED_EDGE('',*,*,#29735,.T.);
#39517=ORIENTED_EDGE('',*,*,#29736,.F.);
#39518=ORIENTED_EDGE('',*,*,#29735,.F.);
#39519=ORIENTED_EDGE('',*,*,#29737,.T.);
#39520=ORIENTED_EDGE('',*,*,#29738,.T.);
#39521=ORIENTED_EDGE('',*,*,#29739,.F.);
#39522=ORIENTED_EDGE('',*,*,#29738,.F.);
#39523=ORIENTED_EDGE('',*,*,#29740,.F.);
#39524=ORIENTED_EDGE('',*,*,#29741,.T.);
#39525=ORIENTED_EDGE('',*,*,#29742,.F.);
#39526=ORIENTED_EDGE('',*,*,#29741,.F.);
#39527=ORIENTED_EDGE('',*,*,#29743,.T.);
#39528=ORIENTED_EDGE('',*,*,#29744,.T.);
#39529=ORIENTED_EDGE('',*,*,#29745,.F.);
#39530=ORIENTED_EDGE('',*,*,#29744,.F.);
#39531=ORIENTED_EDGE('',*,*,#29746,.F.);
#39532=ORIENTED_EDGE('',*,*,#29747,.T.);
#39533=ORIENTED_EDGE('',*,*,#29748,.F.);
#39534=ORIENTED_EDGE('',*,*,#29747,.F.);
#39535=ORIENTED_EDGE('',*,*,#29749,.T.);
#39536=ORIENTED_EDGE('',*,*,#29750,.T.);
#39537=ORIENTED_EDGE('',*,*,#29751,.F.);
#39538=ORIENTED_EDGE('',*,*,#29750,.F.);
#39539=ORIENTED_EDGE('',*,*,#29752,.F.);
#39540=ORIENTED_EDGE('',*,*,#29753,.T.);
#39541=ORIENTED_EDGE('',*,*,#29754,.F.);
#39542=ORIENTED_EDGE('',*,*,#29753,.F.);
#39543=ORIENTED_EDGE('',*,*,#29755,.T.);
#39544=ORIENTED_EDGE('',*,*,#29756,.T.);
#39545=ORIENTED_EDGE('',*,*,#29757,.F.);
#39546=ORIENTED_EDGE('',*,*,#29756,.F.);
#39547=ORIENTED_EDGE('',*,*,#29758,.F.);
#39548=ORIENTED_EDGE('',*,*,#29759,.T.);
#39549=ORIENTED_EDGE('',*,*,#29760,.F.);
#39550=ORIENTED_EDGE('',*,*,#29759,.F.);
#39551=ORIENTED_EDGE('',*,*,#29761,.T.);
#39552=ORIENTED_EDGE('',*,*,#29762,.T.);
#39553=ORIENTED_EDGE('',*,*,#29763,.F.);
#39554=ORIENTED_EDGE('',*,*,#29762,.F.);
#39555=ORIENTED_EDGE('',*,*,#29764,.F.);
#39556=ORIENTED_EDGE('',*,*,#29765,.T.);
#39557=ORIENTED_EDGE('',*,*,#29766,.F.);
#39558=ORIENTED_EDGE('',*,*,#29765,.F.);
#39559=ORIENTED_EDGE('',*,*,#29767,.T.);
#39560=ORIENTED_EDGE('',*,*,#29768,.T.);
#39561=ORIENTED_EDGE('',*,*,#29769,.F.);
#39562=ORIENTED_EDGE('',*,*,#29768,.F.);
#39563=ORIENTED_EDGE('',*,*,#29770,.F.);
#39564=ORIENTED_EDGE('',*,*,#29771,.T.);
#39565=ORIENTED_EDGE('',*,*,#29772,.F.);
#39566=ORIENTED_EDGE('',*,*,#29771,.F.);
#39567=ORIENTED_EDGE('',*,*,#29773,.T.);
#39568=ORIENTED_EDGE('',*,*,#29774,.T.);
#39569=ORIENTED_EDGE('',*,*,#29775,.F.);
#39570=ORIENTED_EDGE('',*,*,#29774,.F.);
#39571=ORIENTED_EDGE('',*,*,#29776,.F.);
#39572=ORIENTED_EDGE('',*,*,#29777,.T.);
#39573=ORIENTED_EDGE('',*,*,#29778,.F.);
#39574=ORIENTED_EDGE('',*,*,#29777,.F.);
#39575=ORIENTED_EDGE('',*,*,#29779,.T.);
#39576=ORIENTED_EDGE('',*,*,#29780,.T.);
#39577=ORIENTED_EDGE('',*,*,#29781,.F.);
#39578=ORIENTED_EDGE('',*,*,#29780,.F.);
#39579=ORIENTED_EDGE('',*,*,#29782,.F.);
#39580=ORIENTED_EDGE('',*,*,#29783,.T.);
#39581=ORIENTED_EDGE('',*,*,#29784,.F.);
#39582=ORIENTED_EDGE('',*,*,#29783,.F.);
#39583=ORIENTED_EDGE('',*,*,#29785,.T.);
#39584=ORIENTED_EDGE('',*,*,#29786,.T.);
#39585=ORIENTED_EDGE('',*,*,#29787,.F.);
#39586=ORIENTED_EDGE('',*,*,#29786,.F.);
#39587=ORIENTED_EDGE('',*,*,#29788,.F.);
#39588=ORIENTED_EDGE('',*,*,#29789,.T.);
#39589=ORIENTED_EDGE('',*,*,#29790,.F.);
#39590=ORIENTED_EDGE('',*,*,#29789,.F.);
#39591=ORIENTED_EDGE('',*,*,#29791,.T.);
#39592=ORIENTED_EDGE('',*,*,#29792,.T.);
#39593=ORIENTED_EDGE('',*,*,#29793,.F.);
#39594=ORIENTED_EDGE('',*,*,#29792,.F.);
#39595=ORIENTED_EDGE('',*,*,#29794,.F.);
#39596=ORIENTED_EDGE('',*,*,#29795,.T.);
#39597=ORIENTED_EDGE('',*,*,#29796,.F.);
#39598=ORIENTED_EDGE('',*,*,#29795,.F.);
#39599=ORIENTED_EDGE('',*,*,#29797,.T.);
#39600=ORIENTED_EDGE('',*,*,#29798,.T.);
#39601=ORIENTED_EDGE('',*,*,#29799,.F.);
#39602=ORIENTED_EDGE('',*,*,#29798,.F.);
#39603=ORIENTED_EDGE('',*,*,#29800,.F.);
#39604=ORIENTED_EDGE('',*,*,#29801,.T.);
#39605=ORIENTED_EDGE('',*,*,#29802,.F.);
#39606=ORIENTED_EDGE('',*,*,#29801,.F.);
#39607=ORIENTED_EDGE('',*,*,#29803,.T.);
#39608=ORIENTED_EDGE('',*,*,#29804,.T.);
#39609=ORIENTED_EDGE('',*,*,#29805,.F.);
#39610=ORIENTED_EDGE('',*,*,#29804,.F.);
#39611=ORIENTED_EDGE('',*,*,#29806,.F.);
#39612=ORIENTED_EDGE('',*,*,#29807,.T.);
#39613=ORIENTED_EDGE('',*,*,#29808,.F.);
#39614=ORIENTED_EDGE('',*,*,#29807,.F.);
#39615=ORIENTED_EDGE('',*,*,#29809,.T.);
#39616=ORIENTED_EDGE('',*,*,#29810,.T.);
#39617=ORIENTED_EDGE('',*,*,#29811,.F.);
#39618=ORIENTED_EDGE('',*,*,#29810,.F.);
#39619=ORIENTED_EDGE('',*,*,#29812,.F.);
#39620=ORIENTED_EDGE('',*,*,#29813,.T.);
#39621=ORIENTED_EDGE('',*,*,#29814,.F.);
#39622=ORIENTED_EDGE('',*,*,#29813,.F.);
#39623=ORIENTED_EDGE('',*,*,#29815,.T.);
#39624=ORIENTED_EDGE('',*,*,#29816,.T.);
#39625=ORIENTED_EDGE('',*,*,#29817,.F.);
#39626=ORIENTED_EDGE('',*,*,#29816,.F.);
#39627=ORIENTED_EDGE('',*,*,#29818,.F.);
#39628=ORIENTED_EDGE('',*,*,#29819,.T.);
#39629=ORIENTED_EDGE('',*,*,#29820,.F.);
#39630=ORIENTED_EDGE('',*,*,#29819,.F.);
#39631=ORIENTED_EDGE('',*,*,#29821,.T.);
#39632=ORIENTED_EDGE('',*,*,#29822,.T.);
#39633=ORIENTED_EDGE('',*,*,#29823,.F.);
#39634=ORIENTED_EDGE('',*,*,#29822,.F.);
#39635=ORIENTED_EDGE('',*,*,#29824,.F.);
#39636=ORIENTED_EDGE('',*,*,#29825,.T.);
#39637=ORIENTED_EDGE('',*,*,#29826,.F.);
#39638=ORIENTED_EDGE('',*,*,#29825,.F.);
#39639=ORIENTED_EDGE('',*,*,#29827,.T.);
#39640=ORIENTED_EDGE('',*,*,#29828,.T.);
#39641=ORIENTED_EDGE('',*,*,#29829,.F.);
#39642=ORIENTED_EDGE('',*,*,#29828,.F.);
#39643=ORIENTED_EDGE('',*,*,#29830,.F.);
#39644=ORIENTED_EDGE('',*,*,#29831,.T.);
#39645=ORIENTED_EDGE('',*,*,#29832,.F.);
#39646=ORIENTED_EDGE('',*,*,#29831,.F.);
#39647=ORIENTED_EDGE('',*,*,#29833,.T.);
#39648=ORIENTED_EDGE('',*,*,#29834,.T.);
#39649=ORIENTED_EDGE('',*,*,#29835,.F.);
#39650=ORIENTED_EDGE('',*,*,#29834,.F.);
#39651=ORIENTED_EDGE('',*,*,#29836,.F.);
#39652=ORIENTED_EDGE('',*,*,#29837,.T.);
#39653=ORIENTED_EDGE('',*,*,#29838,.F.);
#39654=ORIENTED_EDGE('',*,*,#29837,.F.);
#39655=ORIENTED_EDGE('',*,*,#29839,.T.);
#39656=ORIENTED_EDGE('',*,*,#29840,.T.);
#39657=ORIENTED_EDGE('',*,*,#29841,.F.);
#39658=ORIENTED_EDGE('',*,*,#29840,.F.);
#39659=ORIENTED_EDGE('',*,*,#29842,.F.);
#39660=ORIENTED_EDGE('',*,*,#29843,.T.);
#39661=ORIENTED_EDGE('',*,*,#29844,.F.);
#39662=ORIENTED_EDGE('',*,*,#29843,.F.);
#39663=ORIENTED_EDGE('',*,*,#29845,.T.);
#39664=ORIENTED_EDGE('',*,*,#29846,.T.);
#39665=ORIENTED_EDGE('',*,*,#29847,.F.);
#39666=ORIENTED_EDGE('',*,*,#29846,.F.);
#39667=ORIENTED_EDGE('',*,*,#29848,.F.);
#39668=ORIENTED_EDGE('',*,*,#29849,.T.);
#39669=ORIENTED_EDGE('',*,*,#29850,.F.);
#39670=ORIENTED_EDGE('',*,*,#29849,.F.);
#39671=ORIENTED_EDGE('',*,*,#29851,.T.);
#39672=ORIENTED_EDGE('',*,*,#29852,.T.);
#39673=ORIENTED_EDGE('',*,*,#29853,.F.);
#39674=ORIENTED_EDGE('',*,*,#29852,.F.);
#39675=ORIENTED_EDGE('',*,*,#29854,.F.);
#39676=ORIENTED_EDGE('',*,*,#29855,.T.);
#39677=ORIENTED_EDGE('',*,*,#29856,.F.);
#39678=ORIENTED_EDGE('',*,*,#29855,.F.);
#39679=ORIENTED_EDGE('',*,*,#29857,.T.);
#39680=ORIENTED_EDGE('',*,*,#29858,.T.);
#39681=ORIENTED_EDGE('',*,*,#29859,.F.);
#39682=ORIENTED_EDGE('',*,*,#29858,.F.);
#39683=ORIENTED_EDGE('',*,*,#29860,.F.);
#39684=ORIENTED_EDGE('',*,*,#29861,.T.);
#39685=ORIENTED_EDGE('',*,*,#29862,.F.);
#39686=ORIENTED_EDGE('',*,*,#29861,.F.);
#39687=ORIENTED_EDGE('',*,*,#29863,.T.);
#39688=ORIENTED_EDGE('',*,*,#29864,.T.);
#39689=ORIENTED_EDGE('',*,*,#29865,.F.);
#39690=ORIENTED_EDGE('',*,*,#29864,.F.);
#39691=ORIENTED_EDGE('',*,*,#29866,.F.);
#39692=ORIENTED_EDGE('',*,*,#29867,.T.);
#39693=ORIENTED_EDGE('',*,*,#29868,.F.);
#39694=ORIENTED_EDGE('',*,*,#29867,.F.);
#39695=ORIENTED_EDGE('',*,*,#29869,.T.);
#39696=ORIENTED_EDGE('',*,*,#29870,.T.);
#39697=ORIENTED_EDGE('',*,*,#29871,.F.);
#39698=ORIENTED_EDGE('',*,*,#29870,.F.);
#39699=ORIENTED_EDGE('',*,*,#29872,.F.);
#39700=ORIENTED_EDGE('',*,*,#29873,.T.);
#39701=ORIENTED_EDGE('',*,*,#29874,.F.);
#39702=ORIENTED_EDGE('',*,*,#29873,.F.);
#39703=ORIENTED_EDGE('',*,*,#29875,.T.);
#39704=ORIENTED_EDGE('',*,*,#29876,.T.);
#39705=ORIENTED_EDGE('',*,*,#29877,.F.);
#39706=ORIENTED_EDGE('',*,*,#29876,.F.);
#39707=ORIENTED_EDGE('',*,*,#29878,.F.);
#39708=ORIENTED_EDGE('',*,*,#29879,.T.);
#39709=ORIENTED_EDGE('',*,*,#29880,.F.);
#39710=ORIENTED_EDGE('',*,*,#29879,.F.);
#39711=ORIENTED_EDGE('',*,*,#29881,.T.);
#39712=ORIENTED_EDGE('',*,*,#29882,.T.);
#39713=ORIENTED_EDGE('',*,*,#29883,.F.);
#39714=ORIENTED_EDGE('',*,*,#29882,.F.);
#39715=ORIENTED_EDGE('',*,*,#29884,.F.);
#39716=ORIENTED_EDGE('',*,*,#29885,.T.);
#39717=ORIENTED_EDGE('',*,*,#29886,.F.);
#39718=ORIENTED_EDGE('',*,*,#29885,.F.);
#39719=ORIENTED_EDGE('',*,*,#29887,.T.);
#39720=ORIENTED_EDGE('',*,*,#29888,.T.);
#39721=ORIENTED_EDGE('',*,*,#29889,.F.);
#39722=ORIENTED_EDGE('',*,*,#29888,.F.);
#39723=ORIENTED_EDGE('',*,*,#29890,.F.);
#39724=ORIENTED_EDGE('',*,*,#29891,.T.);
#39725=ORIENTED_EDGE('',*,*,#29892,.F.);
#39726=ORIENTED_EDGE('',*,*,#29891,.F.);
#39727=ORIENTED_EDGE('',*,*,#29893,.T.);
#39728=ORIENTED_EDGE('',*,*,#29894,.T.);
#39729=ORIENTED_EDGE('',*,*,#29895,.F.);
#39730=ORIENTED_EDGE('',*,*,#29894,.F.);
#39731=ORIENTED_EDGE('',*,*,#29896,.F.);
#39732=ORIENTED_EDGE('',*,*,#29897,.T.);
#39733=ORIENTED_EDGE('',*,*,#29898,.F.);
#39734=ORIENTED_EDGE('',*,*,#29897,.F.);
#39735=ORIENTED_EDGE('',*,*,#29899,.T.);
#39736=ORIENTED_EDGE('',*,*,#29900,.T.);
#39737=ORIENTED_EDGE('',*,*,#29901,.F.);
#39738=ORIENTED_EDGE('',*,*,#29900,.F.);
#39739=ORIENTED_EDGE('',*,*,#29902,.F.);
#39740=ORIENTED_EDGE('',*,*,#29903,.T.);
#39741=ORIENTED_EDGE('',*,*,#29904,.F.);
#39742=ORIENTED_EDGE('',*,*,#29903,.F.);
#39743=ORIENTED_EDGE('',*,*,#29905,.T.);
#39744=ORIENTED_EDGE('',*,*,#29906,.T.);
#39745=ORIENTED_EDGE('',*,*,#29907,.F.);
#39746=ORIENTED_EDGE('',*,*,#29906,.F.);
#39747=ORIENTED_EDGE('',*,*,#29908,.F.);
#39748=ORIENTED_EDGE('',*,*,#29909,.T.);
#39749=ORIENTED_EDGE('',*,*,#29910,.F.);
#39750=ORIENTED_EDGE('',*,*,#29909,.F.);
#39751=ORIENTED_EDGE('',*,*,#29911,.T.);
#39752=ORIENTED_EDGE('',*,*,#29912,.T.);
#39753=ORIENTED_EDGE('',*,*,#29913,.F.);
#39754=ORIENTED_EDGE('',*,*,#29912,.F.);
#39755=ORIENTED_EDGE('',*,*,#29914,.F.);
#39756=ORIENTED_EDGE('',*,*,#29915,.T.);
#39757=ORIENTED_EDGE('',*,*,#29916,.F.);
#39758=ORIENTED_EDGE('',*,*,#29915,.F.);
#39759=ORIENTED_EDGE('',*,*,#29917,.T.);
#39760=ORIENTED_EDGE('',*,*,#29918,.T.);
#39761=ORIENTED_EDGE('',*,*,#29919,.F.);
#39762=ORIENTED_EDGE('',*,*,#29918,.F.);
#39763=ORIENTED_EDGE('',*,*,#29920,.F.);
#39764=ORIENTED_EDGE('',*,*,#29921,.T.);
#39765=ORIENTED_EDGE('',*,*,#29922,.F.);
#39766=ORIENTED_EDGE('',*,*,#29921,.F.);
#39767=ORIENTED_EDGE('',*,*,#29923,.T.);
#39768=ORIENTED_EDGE('',*,*,#29924,.T.);
#39769=ORIENTED_EDGE('',*,*,#29925,.F.);
#39770=ORIENTED_EDGE('',*,*,#29924,.F.);
#39771=ORIENTED_EDGE('',*,*,#29926,.F.);
#39772=ORIENTED_EDGE('',*,*,#29927,.T.);
#39773=ORIENTED_EDGE('',*,*,#29928,.F.);
#39774=ORIENTED_EDGE('',*,*,#29927,.F.);
#39775=ORIENTED_EDGE('',*,*,#29929,.T.);
#39776=ORIENTED_EDGE('',*,*,#29930,.T.);
#39777=ORIENTED_EDGE('',*,*,#29931,.F.);
#39778=ORIENTED_EDGE('',*,*,#29930,.F.);
#39779=ORIENTED_EDGE('',*,*,#29932,.F.);
#39780=ORIENTED_EDGE('',*,*,#29933,.T.);
#39781=ORIENTED_EDGE('',*,*,#29934,.F.);
#39782=ORIENTED_EDGE('',*,*,#29933,.F.);
#39783=ORIENTED_EDGE('',*,*,#29935,.T.);
#39784=ORIENTED_EDGE('',*,*,#29936,.T.);
#39785=ORIENTED_EDGE('',*,*,#29937,.F.);
#39786=ORIENTED_EDGE('',*,*,#29936,.F.);
#39787=ORIENTED_EDGE('',*,*,#29938,.F.);
#39788=ORIENTED_EDGE('',*,*,#29939,.T.);
#39789=ORIENTED_EDGE('',*,*,#29940,.F.);
#39790=ORIENTED_EDGE('',*,*,#29939,.F.);
#39791=ORIENTED_EDGE('',*,*,#29941,.T.);
#39792=ORIENTED_EDGE('',*,*,#29942,.T.);
#39793=ORIENTED_EDGE('',*,*,#29943,.F.);
#39794=ORIENTED_EDGE('',*,*,#29942,.F.);
#39795=ORIENTED_EDGE('',*,*,#29944,.F.);
#39796=ORIENTED_EDGE('',*,*,#29945,.T.);
#39797=ORIENTED_EDGE('',*,*,#29946,.F.);
#39798=ORIENTED_EDGE('',*,*,#29945,.F.);
#39799=ORIENTED_EDGE('',*,*,#29947,.T.);
#39800=ORIENTED_EDGE('',*,*,#29948,.T.);
#39801=ORIENTED_EDGE('',*,*,#29949,.F.);
#39802=ORIENTED_EDGE('',*,*,#29948,.F.);
#39803=ORIENTED_EDGE('',*,*,#29950,.F.);
#39804=ORIENTED_EDGE('',*,*,#29951,.T.);
#39805=ORIENTED_EDGE('',*,*,#29952,.F.);
#39806=ORIENTED_EDGE('',*,*,#29951,.F.);
#39807=ORIENTED_EDGE('',*,*,#29953,.T.);
#39808=ORIENTED_EDGE('',*,*,#29954,.T.);
#39809=ORIENTED_EDGE('',*,*,#29955,.F.);
#39810=ORIENTED_EDGE('',*,*,#29954,.F.);
#39811=ORIENTED_EDGE('',*,*,#29956,.F.);
#39812=ORIENTED_EDGE('',*,*,#29957,.T.);
#39813=ORIENTED_EDGE('',*,*,#29958,.F.);
#39814=ORIENTED_EDGE('',*,*,#29957,.F.);
#39815=ORIENTED_EDGE('',*,*,#29959,.T.);
#39816=ORIENTED_EDGE('',*,*,#29960,.T.);
#39817=ORIENTED_EDGE('',*,*,#29961,.F.);
#39818=ORIENTED_EDGE('',*,*,#29960,.F.);
#39819=ORIENTED_EDGE('',*,*,#29962,.F.);
#39820=ORIENTED_EDGE('',*,*,#29963,.T.);
#39821=ORIENTED_EDGE('',*,*,#29964,.F.);
#39822=ORIENTED_EDGE('',*,*,#29963,.F.);
#39823=ORIENTED_EDGE('',*,*,#29965,.T.);
#39824=ORIENTED_EDGE('',*,*,#29966,.T.);
#39825=ORIENTED_EDGE('',*,*,#29967,.F.);
#39826=ORIENTED_EDGE('',*,*,#29966,.F.);
#39827=ORIENTED_EDGE('',*,*,#29968,.F.);
#39828=ORIENTED_EDGE('',*,*,#29969,.T.);
#39829=ORIENTED_EDGE('',*,*,#29970,.F.);
#39830=ORIENTED_EDGE('',*,*,#29969,.F.);
#39831=ORIENTED_EDGE('',*,*,#29971,.T.);
#39832=ORIENTED_EDGE('',*,*,#29972,.T.);
#39833=ORIENTED_EDGE('',*,*,#29973,.F.);
#39834=ORIENTED_EDGE('',*,*,#29972,.F.);
#39835=ORIENTED_EDGE('',*,*,#29974,.F.);
#39836=ORIENTED_EDGE('',*,*,#29975,.T.);
#39837=ORIENTED_EDGE('',*,*,#29976,.F.);
#39838=ORIENTED_EDGE('',*,*,#29975,.F.);
#39839=ORIENTED_EDGE('',*,*,#29977,.T.);
#39840=ORIENTED_EDGE('',*,*,#29978,.T.);
#39841=ORIENTED_EDGE('',*,*,#29979,.F.);
#39842=ORIENTED_EDGE('',*,*,#29978,.F.);
#39843=ORIENTED_EDGE('',*,*,#29980,.F.);
#39844=ORIENTED_EDGE('',*,*,#29981,.T.);
#39845=ORIENTED_EDGE('',*,*,#29982,.F.);
#39846=ORIENTED_EDGE('',*,*,#29981,.F.);
#39847=ORIENTED_EDGE('',*,*,#29983,.T.);
#39848=ORIENTED_EDGE('',*,*,#29984,.T.);
#39849=ORIENTED_EDGE('',*,*,#29985,.F.);
#39850=ORIENTED_EDGE('',*,*,#29984,.F.);
#39851=ORIENTED_EDGE('',*,*,#29986,.F.);
#39852=ORIENTED_EDGE('',*,*,#29987,.T.);
#39853=ORIENTED_EDGE('',*,*,#29988,.F.);
#39854=ORIENTED_EDGE('',*,*,#29987,.F.);
#39855=ORIENTED_EDGE('',*,*,#29989,.T.);
#39856=ORIENTED_EDGE('',*,*,#29990,.T.);
#39857=ORIENTED_EDGE('',*,*,#29991,.F.);
#39858=ORIENTED_EDGE('',*,*,#29990,.F.);
#39859=ORIENTED_EDGE('',*,*,#29992,.F.);
#39860=ORIENTED_EDGE('',*,*,#29993,.T.);
#39861=ORIENTED_EDGE('',*,*,#29994,.F.);
#39862=ORIENTED_EDGE('',*,*,#29993,.F.);
#39863=ORIENTED_EDGE('',*,*,#29995,.T.);
#39864=ORIENTED_EDGE('',*,*,#29996,.T.);
#39865=ORIENTED_EDGE('',*,*,#29997,.F.);
#39866=ORIENTED_EDGE('',*,*,#29996,.F.);
#39867=ORIENTED_EDGE('',*,*,#29998,.F.);
#39868=ORIENTED_EDGE('',*,*,#29999,.T.);
#39869=ORIENTED_EDGE('',*,*,#30000,.F.);
#39870=ORIENTED_EDGE('',*,*,#29999,.F.);
#39871=ORIENTED_EDGE('',*,*,#30001,.T.);
#39872=ORIENTED_EDGE('',*,*,#30002,.T.);
#39873=ORIENTED_EDGE('',*,*,#30003,.F.);
#39874=ORIENTED_EDGE('',*,*,#30002,.F.);
#39875=ORIENTED_EDGE('',*,*,#30004,.F.);
#39876=ORIENTED_EDGE('',*,*,#30005,.T.);
#39877=ORIENTED_EDGE('',*,*,#30006,.F.);
#39878=ORIENTED_EDGE('',*,*,#30005,.F.);
#39879=ORIENTED_EDGE('',*,*,#30007,.T.);
#39880=ORIENTED_EDGE('',*,*,#30008,.T.);
#39881=ORIENTED_EDGE('',*,*,#30009,.F.);
#39882=ORIENTED_EDGE('',*,*,#30008,.F.);
#39883=ORIENTED_EDGE('',*,*,#30010,.F.);
#39884=ORIENTED_EDGE('',*,*,#30011,.T.);
#39885=ORIENTED_EDGE('',*,*,#30012,.F.);
#39886=ORIENTED_EDGE('',*,*,#30011,.F.);
#39887=ORIENTED_EDGE('',*,*,#30013,.T.);
#39888=ORIENTED_EDGE('',*,*,#30014,.T.);
#39889=ORIENTED_EDGE('',*,*,#30015,.F.);
#39890=ORIENTED_EDGE('',*,*,#30014,.F.);
#39891=ORIENTED_EDGE('',*,*,#30016,.F.);
#39892=ORIENTED_EDGE('',*,*,#30017,.T.);
#39893=ORIENTED_EDGE('',*,*,#30018,.F.);
#39894=ORIENTED_EDGE('',*,*,#30017,.F.);
#39895=ORIENTED_EDGE('',*,*,#30019,.T.);
#39896=ORIENTED_EDGE('',*,*,#30020,.T.);
#39897=ORIENTED_EDGE('',*,*,#30021,.F.);
#39898=ORIENTED_EDGE('',*,*,#30020,.F.);
#39899=ORIENTED_EDGE('',*,*,#30022,.F.);
#39900=ORIENTED_EDGE('',*,*,#30023,.T.);
#39901=ORIENTED_EDGE('',*,*,#30024,.F.);
#39902=ORIENTED_EDGE('',*,*,#30023,.F.);
#39903=ORIENTED_EDGE('',*,*,#30025,.T.);
#39904=ORIENTED_EDGE('',*,*,#30026,.T.);
#39905=ORIENTED_EDGE('',*,*,#30027,.F.);
#39906=ORIENTED_EDGE('',*,*,#30026,.F.);
#39907=ORIENTED_EDGE('',*,*,#30028,.F.);
#39908=ORIENTED_EDGE('',*,*,#30029,.T.);
#39909=ORIENTED_EDGE('',*,*,#30030,.F.);
#39910=ORIENTED_EDGE('',*,*,#30029,.F.);
#39911=ORIENTED_EDGE('',*,*,#30031,.T.);
#39912=ORIENTED_EDGE('',*,*,#30032,.T.);
#39913=ORIENTED_EDGE('',*,*,#30033,.F.);
#39914=ORIENTED_EDGE('',*,*,#30032,.F.);
#39915=ORIENTED_EDGE('',*,*,#30034,.F.);
#39916=ORIENTED_EDGE('',*,*,#30035,.T.);
#39917=ORIENTED_EDGE('',*,*,#30036,.F.);
#39918=ORIENTED_EDGE('',*,*,#30035,.F.);
#39919=ORIENTED_EDGE('',*,*,#30037,.T.);
#39920=ORIENTED_EDGE('',*,*,#30038,.T.);
#39921=ORIENTED_EDGE('',*,*,#30039,.F.);
#39922=ORIENTED_EDGE('',*,*,#30038,.F.);
#39923=ORIENTED_EDGE('',*,*,#30040,.F.);
#39924=ORIENTED_EDGE('',*,*,#30041,.T.);
#39925=ORIENTED_EDGE('',*,*,#30042,.F.);
#39926=ORIENTED_EDGE('',*,*,#30041,.F.);
#39927=ORIENTED_EDGE('',*,*,#30043,.T.);
#39928=ORIENTED_EDGE('',*,*,#30044,.T.);
#39929=ORIENTED_EDGE('',*,*,#30045,.F.);
#39930=ORIENTED_EDGE('',*,*,#30044,.F.);
#39931=ORIENTED_EDGE('',*,*,#30046,.F.);
#39932=ORIENTED_EDGE('',*,*,#30047,.T.);
#39933=ORIENTED_EDGE('',*,*,#30048,.F.);
#39934=ORIENTED_EDGE('',*,*,#30047,.F.);
#39935=ORIENTED_EDGE('',*,*,#30049,.T.);
#39936=ORIENTED_EDGE('',*,*,#30050,.T.);
#39937=ORIENTED_EDGE('',*,*,#30051,.F.);
#39938=ORIENTED_EDGE('',*,*,#30050,.F.);
#39939=ORIENTED_EDGE('',*,*,#30052,.F.);
#39940=ORIENTED_EDGE('',*,*,#30053,.T.);
#39941=ORIENTED_EDGE('',*,*,#30054,.F.);
#39942=ORIENTED_EDGE('',*,*,#30053,.F.);
#39943=ORIENTED_EDGE('',*,*,#30055,.T.);
#39944=ORIENTED_EDGE('',*,*,#30056,.T.);
#39945=ORIENTED_EDGE('',*,*,#30057,.F.);
#39946=ORIENTED_EDGE('',*,*,#30056,.F.);
#39947=ORIENTED_EDGE('',*,*,#30058,.F.);
#39948=ORIENTED_EDGE('',*,*,#30059,.T.);
#39949=ORIENTED_EDGE('',*,*,#30060,.F.);
#39950=ORIENTED_EDGE('',*,*,#30059,.F.);
#39951=ORIENTED_EDGE('',*,*,#30061,.T.);
#39952=ORIENTED_EDGE('',*,*,#30062,.T.);
#39953=ORIENTED_EDGE('',*,*,#30063,.F.);
#39954=ORIENTED_EDGE('',*,*,#30062,.F.);
#39955=ORIENTED_EDGE('',*,*,#30064,.F.);
#39956=ORIENTED_EDGE('',*,*,#30065,.T.);
#39957=ORIENTED_EDGE('',*,*,#30066,.F.);
#39958=ORIENTED_EDGE('',*,*,#30065,.F.);
#39959=ORIENTED_EDGE('',*,*,#30067,.T.);
#39960=ORIENTED_EDGE('',*,*,#30068,.T.);
#39961=ORIENTED_EDGE('',*,*,#30069,.F.);
#39962=ORIENTED_EDGE('',*,*,#30068,.F.);
#39963=ORIENTED_EDGE('',*,*,#30070,.F.);
#39964=ORIENTED_EDGE('',*,*,#30071,.T.);
#39965=ORIENTED_EDGE('',*,*,#30072,.F.);
#39966=ORIENTED_EDGE('',*,*,#30071,.F.);
#39967=ORIENTED_EDGE('',*,*,#30073,.T.);
#39968=ORIENTED_EDGE('',*,*,#30074,.T.);
#39969=ORIENTED_EDGE('',*,*,#30075,.F.);
#39970=ORIENTED_EDGE('',*,*,#30074,.F.);
#39971=ORIENTED_EDGE('',*,*,#30076,.F.);
#39972=ORIENTED_EDGE('',*,*,#30077,.T.);
#39973=ORIENTED_EDGE('',*,*,#30078,.F.);
#39974=ORIENTED_EDGE('',*,*,#30077,.F.);
#39975=ORIENTED_EDGE('',*,*,#30079,.T.);
#39976=ORIENTED_EDGE('',*,*,#30080,.T.);
#39977=ORIENTED_EDGE('',*,*,#30081,.F.);
#39978=ORIENTED_EDGE('',*,*,#30080,.F.);
#39979=ORIENTED_EDGE('',*,*,#30082,.F.);
#39980=ORIENTED_EDGE('',*,*,#30083,.T.);
#39981=ORIENTED_EDGE('',*,*,#30084,.F.);
#39982=ORIENTED_EDGE('',*,*,#30083,.F.);
#39983=ORIENTED_EDGE('',*,*,#30085,.T.);
#39984=ORIENTED_EDGE('',*,*,#30086,.T.);
#39985=ORIENTED_EDGE('',*,*,#30087,.F.);
#39986=ORIENTED_EDGE('',*,*,#30086,.F.);
#39987=ORIENTED_EDGE('',*,*,#30088,.F.);
#39988=ORIENTED_EDGE('',*,*,#30089,.T.);
#39989=ORIENTED_EDGE('',*,*,#30090,.F.);
#39990=ORIENTED_EDGE('',*,*,#30089,.F.);
#39991=ORIENTED_EDGE('',*,*,#30091,.T.);
#39992=ORIENTED_EDGE('',*,*,#30092,.T.);
#39993=ORIENTED_EDGE('',*,*,#30093,.F.);
#39994=ORIENTED_EDGE('',*,*,#30092,.F.);
#39995=ORIENTED_EDGE('',*,*,#30094,.F.);
#39996=ORIENTED_EDGE('',*,*,#30095,.T.);
#39997=ORIENTED_EDGE('',*,*,#30096,.F.);
#39998=ORIENTED_EDGE('',*,*,#30095,.F.);
#39999=ORIENTED_EDGE('',*,*,#30097,.T.);
#40000=ORIENTED_EDGE('',*,*,#30098,.T.);
#40001=ORIENTED_EDGE('',*,*,#30099,.F.);
#40002=ORIENTED_EDGE('',*,*,#30098,.F.);
#40003=ORIENTED_EDGE('',*,*,#30100,.F.);
#40004=ORIENTED_EDGE('',*,*,#30101,.T.);
#40005=ORIENTED_EDGE('',*,*,#30102,.F.);
#40006=ORIENTED_EDGE('',*,*,#30101,.F.);
#40007=ORIENTED_EDGE('',*,*,#30103,.T.);
#40008=ORIENTED_EDGE('',*,*,#30104,.T.);
#40009=ORIENTED_EDGE('',*,*,#30105,.F.);
#40010=ORIENTED_EDGE('',*,*,#30104,.F.);
#40011=ORIENTED_EDGE('',*,*,#30106,.F.);
#40012=ORIENTED_EDGE('',*,*,#30107,.T.);
#40013=ORIENTED_EDGE('',*,*,#30108,.F.);
#40014=ORIENTED_EDGE('',*,*,#30107,.F.);
#40015=ORIENTED_EDGE('',*,*,#30109,.T.);
#40016=ORIENTED_EDGE('',*,*,#30110,.T.);
#40017=ORIENTED_EDGE('',*,*,#30111,.F.);
#40018=ORIENTED_EDGE('',*,*,#30110,.F.);
#40019=ORIENTED_EDGE('',*,*,#30112,.F.);
#40020=ORIENTED_EDGE('',*,*,#30113,.T.);
#40021=ORIENTED_EDGE('',*,*,#30114,.F.);
#40022=ORIENTED_EDGE('',*,*,#30113,.F.);
#40023=ORIENTED_EDGE('',*,*,#30115,.T.);
#40024=ORIENTED_EDGE('',*,*,#30116,.T.);
#40025=ORIENTED_EDGE('',*,*,#30117,.F.);
#40026=ORIENTED_EDGE('',*,*,#30116,.F.);
#40027=ORIENTED_EDGE('',*,*,#30118,.F.);
#40028=ORIENTED_EDGE('',*,*,#30119,.T.);
#40029=ORIENTED_EDGE('',*,*,#30120,.F.);
#40030=ORIENTED_EDGE('',*,*,#30119,.F.);
#40031=ORIENTED_EDGE('',*,*,#30121,.T.);
#40032=ORIENTED_EDGE('',*,*,#30122,.T.);
#40033=ORIENTED_EDGE('',*,*,#30123,.F.);
#40034=ORIENTED_EDGE('',*,*,#30122,.F.);
#40035=ORIENTED_EDGE('',*,*,#30124,.F.);
#40036=ORIENTED_EDGE('',*,*,#30125,.T.);
#40037=ORIENTED_EDGE('',*,*,#30126,.F.);
#40038=ORIENTED_EDGE('',*,*,#30125,.F.);
#40039=ORIENTED_EDGE('',*,*,#30127,.T.);
#40040=ORIENTED_EDGE('',*,*,#30128,.T.);
#40041=ORIENTED_EDGE('',*,*,#30129,.F.);
#40042=ORIENTED_EDGE('',*,*,#30128,.F.);
#40043=ORIENTED_EDGE('',*,*,#30130,.F.);
#40044=ORIENTED_EDGE('',*,*,#30131,.T.);
#40045=ORIENTED_EDGE('',*,*,#30132,.F.);
#40046=ORIENTED_EDGE('',*,*,#30131,.F.);
#40047=ORIENTED_EDGE('',*,*,#30133,.T.);
#40048=ORIENTED_EDGE('',*,*,#30134,.T.);
#40049=ORIENTED_EDGE('',*,*,#30135,.F.);
#40050=ORIENTED_EDGE('',*,*,#30134,.F.);
#40051=ORIENTED_EDGE('',*,*,#30136,.F.);
#40052=ORIENTED_EDGE('',*,*,#30137,.T.);
#40053=ORIENTED_EDGE('',*,*,#30138,.F.);
#40054=ORIENTED_EDGE('',*,*,#30137,.F.);
#40055=ORIENTED_EDGE('',*,*,#30139,.T.);
#40056=ORIENTED_EDGE('',*,*,#30140,.T.);
#40057=ORIENTED_EDGE('',*,*,#30141,.F.);
#40058=ORIENTED_EDGE('',*,*,#30140,.F.);
#40059=ORIENTED_EDGE('',*,*,#30142,.F.);
#40060=ORIENTED_EDGE('',*,*,#30143,.T.);
#40061=ORIENTED_EDGE('',*,*,#30144,.F.);
#40062=ORIENTED_EDGE('',*,*,#30143,.F.);
#40063=ORIENTED_EDGE('',*,*,#30145,.T.);
#40064=ORIENTED_EDGE('',*,*,#30146,.T.);
#40065=ORIENTED_EDGE('',*,*,#30147,.F.);
#40066=ORIENTED_EDGE('',*,*,#30146,.F.);
#40067=ORIENTED_EDGE('',*,*,#30148,.F.);
#40068=ORIENTED_EDGE('',*,*,#30149,.T.);
#40069=ORIENTED_EDGE('',*,*,#30150,.F.);
#40070=ORIENTED_EDGE('',*,*,#30149,.F.);
#40071=ORIENTED_EDGE('',*,*,#30151,.T.);
#40072=ORIENTED_EDGE('',*,*,#30152,.T.);
#40073=ORIENTED_EDGE('',*,*,#30153,.F.);
#40074=ORIENTED_EDGE('',*,*,#30152,.F.);
#40075=ORIENTED_EDGE('',*,*,#30154,.F.);
#40076=ORIENTED_EDGE('',*,*,#30155,.T.);
#40077=ORIENTED_EDGE('',*,*,#30156,.F.);
#40078=ORIENTED_EDGE('',*,*,#30155,.F.);
#40079=ORIENTED_EDGE('',*,*,#30157,.T.);
#40080=ORIENTED_EDGE('',*,*,#30158,.T.);
#40081=ORIENTED_EDGE('',*,*,#30159,.F.);
#40082=ORIENTED_EDGE('',*,*,#30158,.F.);
#40083=ORIENTED_EDGE('',*,*,#30160,.F.);
#40084=ORIENTED_EDGE('',*,*,#30161,.T.);
#40085=ORIENTED_EDGE('',*,*,#30162,.F.);
#40086=ORIENTED_EDGE('',*,*,#30161,.F.);
#40087=ORIENTED_EDGE('',*,*,#30163,.T.);
#40088=ORIENTED_EDGE('',*,*,#30164,.T.);
#40089=ORIENTED_EDGE('',*,*,#30165,.F.);
#40090=ORIENTED_EDGE('',*,*,#30164,.F.);
#40091=ORIENTED_EDGE('',*,*,#30166,.F.);
#40092=ORIENTED_EDGE('',*,*,#30167,.T.);
#40093=ORIENTED_EDGE('',*,*,#30168,.F.);
#40094=ORIENTED_EDGE('',*,*,#30167,.F.);
#40095=ORIENTED_EDGE('',*,*,#30169,.T.);
#40096=ORIENTED_EDGE('',*,*,#30170,.T.);
#40097=ORIENTED_EDGE('',*,*,#30171,.F.);
#40098=ORIENTED_EDGE('',*,*,#30170,.F.);
#40099=ORIENTED_EDGE('',*,*,#30172,.F.);
#40100=ORIENTED_EDGE('',*,*,#30173,.T.);
#40101=ORIENTED_EDGE('',*,*,#30174,.F.);
#40102=ORIENTED_EDGE('',*,*,#30173,.F.);
#40103=ORIENTED_EDGE('',*,*,#30175,.T.);
#40104=ORIENTED_EDGE('',*,*,#30176,.T.);
#40105=ORIENTED_EDGE('',*,*,#30177,.F.);
#40106=ORIENTED_EDGE('',*,*,#30176,.F.);
#40107=ORIENTED_EDGE('',*,*,#30178,.F.);
#40108=ORIENTED_EDGE('',*,*,#30179,.T.);
#40109=ORIENTED_EDGE('',*,*,#30180,.F.);
#40110=ORIENTED_EDGE('',*,*,#30179,.F.);
#40111=ORIENTED_EDGE('',*,*,#30181,.T.);
#40112=ORIENTED_EDGE('',*,*,#30182,.T.);
#40113=ORIENTED_EDGE('',*,*,#30183,.F.);
#40114=ORIENTED_EDGE('',*,*,#30182,.F.);
#40115=ORIENTED_EDGE('',*,*,#30184,.F.);
#40116=ORIENTED_EDGE('',*,*,#30185,.T.);
#40117=ORIENTED_EDGE('',*,*,#30186,.F.);
#40118=ORIENTED_EDGE('',*,*,#30185,.F.);
#40119=ORIENTED_EDGE('',*,*,#30187,.T.);
#40120=ORIENTED_EDGE('',*,*,#30188,.T.);
#40121=ORIENTED_EDGE('',*,*,#30189,.F.);
#40122=ORIENTED_EDGE('',*,*,#30188,.F.);
#40123=ORIENTED_EDGE('',*,*,#30190,.F.);
#40124=ORIENTED_EDGE('',*,*,#30191,.T.);
#40125=ORIENTED_EDGE('',*,*,#30192,.F.);
#40126=ORIENTED_EDGE('',*,*,#30191,.F.);
#40127=ORIENTED_EDGE('',*,*,#30193,.T.);
#40128=ORIENTED_EDGE('',*,*,#30194,.T.);
#40129=ORIENTED_EDGE('',*,*,#30195,.F.);
#40130=ORIENTED_EDGE('',*,*,#30194,.F.);
#40131=ORIENTED_EDGE('',*,*,#30196,.F.);
#40132=ORIENTED_EDGE('',*,*,#30197,.T.);
#40133=ORIENTED_EDGE('',*,*,#30198,.F.);
#40134=ORIENTED_EDGE('',*,*,#30197,.F.);
#40135=ORIENTED_EDGE('',*,*,#30199,.T.);
#40136=ORIENTED_EDGE('',*,*,#30200,.T.);
#40137=ORIENTED_EDGE('',*,*,#30201,.F.);
#40138=ORIENTED_EDGE('',*,*,#30200,.F.);
#40139=ORIENTED_EDGE('',*,*,#30202,.F.);
#40140=ORIENTED_EDGE('',*,*,#30203,.T.);
#40141=ORIENTED_EDGE('',*,*,#30204,.F.);
#40142=ORIENTED_EDGE('',*,*,#30203,.F.);
#40143=ORIENTED_EDGE('',*,*,#30205,.T.);
#40144=ORIENTED_EDGE('',*,*,#30206,.T.);
#40145=ORIENTED_EDGE('',*,*,#30207,.F.);
#40146=ORIENTED_EDGE('',*,*,#30206,.F.);
#40147=ORIENTED_EDGE('',*,*,#30208,.F.);
#40148=ORIENTED_EDGE('',*,*,#30209,.T.);
#40149=ORIENTED_EDGE('',*,*,#30210,.F.);
#40150=ORIENTED_EDGE('',*,*,#30209,.F.);
#40151=ORIENTED_EDGE('',*,*,#30211,.T.);
#40152=ORIENTED_EDGE('',*,*,#30212,.T.);
#40153=ORIENTED_EDGE('',*,*,#30213,.F.);
#40154=ORIENTED_EDGE('',*,*,#30212,.F.);
#40155=ORIENTED_EDGE('',*,*,#30214,.F.);
#40156=ORIENTED_EDGE('',*,*,#30215,.T.);
#40157=ORIENTED_EDGE('',*,*,#30216,.F.);
#40158=ORIENTED_EDGE('',*,*,#30215,.F.);
#40159=ORIENTED_EDGE('',*,*,#30217,.T.);
#40160=ORIENTED_EDGE('',*,*,#30218,.T.);
#40161=ORIENTED_EDGE('',*,*,#30219,.F.);
#40162=ORIENTED_EDGE('',*,*,#30218,.F.);
#40163=ORIENTED_EDGE('',*,*,#30220,.F.);
#40164=ORIENTED_EDGE('',*,*,#30221,.T.);
#40165=ORIENTED_EDGE('',*,*,#30222,.F.);
#40166=ORIENTED_EDGE('',*,*,#30221,.F.);
#40167=ORIENTED_EDGE('',*,*,#30223,.T.);
#40168=ORIENTED_EDGE('',*,*,#30224,.T.);
#40169=ORIENTED_EDGE('',*,*,#30225,.F.);
#40170=ORIENTED_EDGE('',*,*,#30224,.F.);
#40171=ORIENTED_EDGE('',*,*,#30226,.F.);
#40172=ORIENTED_EDGE('',*,*,#30227,.T.);
#40173=ORIENTED_EDGE('',*,*,#30228,.F.);
#40174=ORIENTED_EDGE('',*,*,#30227,.F.);
#40175=ORIENTED_EDGE('',*,*,#30229,.T.);
#40176=ORIENTED_EDGE('',*,*,#30230,.T.);
#40177=ORIENTED_EDGE('',*,*,#30231,.F.);
#40178=ORIENTED_EDGE('',*,*,#30230,.F.);
#40179=ORIENTED_EDGE('',*,*,#30232,.F.);
#40180=ORIENTED_EDGE('',*,*,#30233,.T.);
#40181=ORIENTED_EDGE('',*,*,#30234,.F.);
#40182=ORIENTED_EDGE('',*,*,#30233,.F.);
#40183=ORIENTED_EDGE('',*,*,#30235,.T.);
#40184=ORIENTED_EDGE('',*,*,#30236,.T.);
#40185=ORIENTED_EDGE('',*,*,#30237,.F.);
#40186=ORIENTED_EDGE('',*,*,#30236,.F.);
#40187=ORIENTED_EDGE('',*,*,#30238,.F.);
#40188=ORIENTED_EDGE('',*,*,#30239,.T.);
#40189=ORIENTED_EDGE('',*,*,#30240,.F.);
#40190=ORIENTED_EDGE('',*,*,#30239,.F.);
#40191=ORIENTED_EDGE('',*,*,#30241,.T.);
#40192=ORIENTED_EDGE('',*,*,#30242,.T.);
#40193=ORIENTED_EDGE('',*,*,#30243,.F.);
#40194=ORIENTED_EDGE('',*,*,#30242,.F.);
#40195=ORIENTED_EDGE('',*,*,#30244,.F.);
#40196=ORIENTED_EDGE('',*,*,#30245,.T.);
#40197=ORIENTED_EDGE('',*,*,#30246,.F.);
#40198=ORIENTED_EDGE('',*,*,#30245,.F.);
#40199=ORIENTED_EDGE('',*,*,#30247,.T.);
#40200=ORIENTED_EDGE('',*,*,#30248,.T.);
#40201=ORIENTED_EDGE('',*,*,#30249,.F.);
#40202=ORIENTED_EDGE('',*,*,#30248,.F.);
#40203=ORIENTED_EDGE('',*,*,#30250,.F.);
#40204=ORIENTED_EDGE('',*,*,#30251,.T.);
#40205=ORIENTED_EDGE('',*,*,#30252,.F.);
#40206=ORIENTED_EDGE('',*,*,#30251,.F.);
#40207=ORIENTED_EDGE('',*,*,#30253,.T.);
#40208=ORIENTED_EDGE('',*,*,#30254,.T.);
#40209=ORIENTED_EDGE('',*,*,#30255,.F.);
#40210=ORIENTED_EDGE('',*,*,#30254,.F.);
#40211=ORIENTED_EDGE('',*,*,#30256,.F.);
#40212=ORIENTED_EDGE('',*,*,#30257,.T.);
#40213=ORIENTED_EDGE('',*,*,#30258,.F.);
#40214=ORIENTED_EDGE('',*,*,#30257,.F.);
#40215=ORIENTED_EDGE('',*,*,#30259,.T.);
#40216=ORIENTED_EDGE('',*,*,#30260,.T.);
#40217=ORIENTED_EDGE('',*,*,#30261,.F.);
#40218=ORIENTED_EDGE('',*,*,#30260,.F.);
#40219=ORIENTED_EDGE('',*,*,#30262,.F.);
#40220=ORIENTED_EDGE('',*,*,#30263,.T.);
#40221=ORIENTED_EDGE('',*,*,#30264,.F.);
#40222=ORIENTED_EDGE('',*,*,#30263,.F.);
#40223=ORIENTED_EDGE('',*,*,#30265,.T.);
#40224=ORIENTED_EDGE('',*,*,#30266,.T.);
#40225=ORIENTED_EDGE('',*,*,#30267,.F.);
#40226=ORIENTED_EDGE('',*,*,#30266,.F.);
#40227=ORIENTED_EDGE('',*,*,#30268,.F.);
#40228=ORIENTED_EDGE('',*,*,#30269,.T.);
#40229=ORIENTED_EDGE('',*,*,#30270,.F.);
#40230=ORIENTED_EDGE('',*,*,#30269,.F.);
#40231=ORIENTED_EDGE('',*,*,#30271,.T.);
#40232=ORIENTED_EDGE('',*,*,#30272,.T.);
#40233=ORIENTED_EDGE('',*,*,#30273,.F.);
#40234=ORIENTED_EDGE('',*,*,#30272,.F.);
#40235=ORIENTED_EDGE('',*,*,#30274,.F.);
#40236=ORIENTED_EDGE('',*,*,#30275,.T.);
#40237=ORIENTED_EDGE('',*,*,#30276,.F.);
#40238=ORIENTED_EDGE('',*,*,#30275,.F.);
#40239=ORIENTED_EDGE('',*,*,#30277,.T.);
#40240=ORIENTED_EDGE('',*,*,#30278,.T.);
#40241=ORIENTED_EDGE('',*,*,#30279,.F.);
#40242=ORIENTED_EDGE('',*,*,#30278,.F.);
#40243=ORIENTED_EDGE('',*,*,#27756,.F.);
#40244=ORIENTED_EDGE('',*,*,#30280,.T.);
#40245=ORIENTED_EDGE('',*,*,#30281,.F.);
#40246=ORIENTED_EDGE('',*,*,#30280,.F.);
#40247=ORIENTED_EDGE('',*,*,#30282,.F.);
#40248=ORIENTED_EDGE('',*,*,#30281,.T.);
#40249=ORIENTED_EDGE('',*,*,#30283,.T.);
#40250=ORIENTED_EDGE('',*,*,#30284,.T.);
#40251=ORIENTED_EDGE('',*,*,#30283,.F.);
#40252=ORIENTED_EDGE('',*,*,#30285,.F.);
#40253=ORIENTED_EDGE('',*,*,#30286,.T.);
#40254=ORIENTED_EDGE('',*,*,#30287,.F.);
#40255=ORIENTED_EDGE('',*,*,#30288,.F.);
#40256=ORIENTED_EDGE('',*,*,#30286,.F.);
#40257=ORIENTED_EDGE('',*,*,#30289,.F.);
#40258=ORIENTED_EDGE('',*,*,#30290,.T.);
#40259=ORIENTED_EDGE('',*,*,#30291,.F.);
#40260=ORIENTED_EDGE('',*,*,#30290,.F.);
#40261=ORIENTED_EDGE('',*,*,#30291,.T.);
#40262=ORIENTED_EDGE('',*,*,#30292,.T.);
#40263=ORIENTED_EDGE('',*,*,#30287,.T.);
#40264=ORIENTED_EDGE('',*,*,#30288,.T.);
#40265=ORIENTED_EDGE('',*,*,#30292,.F.);
#40266=ORIENTED_EDGE('',*,*,#30293,.F.);
#40267=ORIENTED_EDGE('',*,*,#27878,.T.);
#40268=ORIENTED_EDGE('',*,*,#30294,.F.);
#40269=ORIENTED_EDGE('',*,*,#30295,.T.);
#40270=ORIENTED_EDGE('',*,*,#30296,.F.);
#40271=ORIENTED_EDGE('',*,*,#30295,.F.);
#40272=ORIENTED_EDGE('',*,*,#30297,.F.);
#40273=ORIENTED_EDGE('',*,*,#30298,.T.);
#40274=ORIENTED_EDGE('',*,*,#30299,.F.);
#40275=ORIENTED_EDGE('',*,*,#30298,.F.);
#40276=ORIENTED_EDGE('',*,*,#30284,.F.);
#40277=ORIENTED_EDGE('',*,*,#30300,.T.);
#40278=ORIENTED_EDGE('',*,*,#30301,.F.);
#40279=ORIENTED_EDGE('',*,*,#30300,.F.);
#40280=ORIENTED_EDGE('',*,*,#30302,.T.);
#40281=ORIENTED_EDGE('',*,*,#30303,.T.);
#40282=ORIENTED_EDGE('',*,*,#30294,.T.);
#40283=ORIENTED_EDGE('',*,*,#30303,.F.);
#40284=ORIENTED_EDGE('',*,*,#30304,.F.);
#40285=ORIENTED_EDGE('',*,*,#30305,.F.);
#40286=ORIENTED_EDGE('',*,*,#30306,.T.);
#40287=ORIENTED_EDGE('',*,*,#30307,.F.);
#40288=ORIENTED_EDGE('',*,*,#30306,.F.);
#40289=ORIENTED_EDGE('',*,*,#30304,.T.);
#40290=ORIENTED_EDGE('',*,*,#30305,.T.);
#40291=ORIENTED_EDGE('',*,*,#30308,.T.);
#40292=ORIENTED_EDGE('',*,*,#30297,.T.);
#40293=ORIENTED_EDGE('',*,*,#30308,.F.);
#40294=ORIENTED_EDGE('',*,*,#30309,.T.);
#40295=ORIENTED_EDGE('',*,*,#30310,.T.);
#40296=ORIENTED_EDGE('',*,*,#30311,.F.);
#40297=ORIENTED_EDGE('',*,*,#30310,.F.);
#40298=ORIENTED_EDGE('',*,*,#30312,.T.);
#40299=ORIENTED_EDGE('',*,*,#27790,.F.);
#40300=ORIENTED_EDGE('',*,*,#27791,.F.);
#40301=ORIENTED_EDGE('',*,*,#30313,.T.);
#40302=ORIENTED_EDGE('',*,*,#30314,.F.);
#40303=ORIENTED_EDGE('',*,*,#30313,.F.);
#40304=ORIENTED_EDGE('',*,*,#30314,.T.);
#40305=ORIENTED_EDGE('',*,*,#30309,.F.);
#40306=ORIENTED_EDGE('',*,*,#30312,.F.);
#40307=ORIENTED_EDGE('',*,*,#30311,.T.);
#40308=ORIENTED_EDGE('',*,*,#30299,.T.);
#40309=ORIENTED_EDGE('',*,*,#30301,.T.);
#40310=ORIENTED_EDGE('',*,*,#30307,.T.);
#40311=ORIENTED_EDGE('',*,*,#30302,.F.);
#40312=ORIENTED_EDGE('',*,*,#30296,.T.);
#40313=ORIENTED_EDGE('',*,*,#30293,.T.);
#40314=ORIENTED_EDGE('',*,*,#30289,.T.);
#40315=ORIENTED_EDGE('',*,*,#30285,.T.);
#40316=ORIENTED_EDGE('',*,*,#27880,.T.);
#40317=ORIENTED_EDGE('',*,*,#27754,.F.);
#40318=ORIENTED_EDGE('',*,*,#30315,.F.);
#40319=ORIENTED_EDGE('',*,*,#29350,.T.);
#40320=ORIENTED_EDGE('',*,*,#29290,.T.);
#40321=ORIENTED_EDGE('',*,*,#29230,.T.);
#40322=ORIENTED_EDGE('',*,*,#29170,.T.);
#40323=ORIENTED_EDGE('',*,*,#29110,.T.);
#40324=ORIENTED_EDGE('',*,*,#29050,.T.);
#40325=ORIENTED_EDGE('',*,*,#28990,.T.);
#40326=ORIENTED_EDGE('',*,*,#28930,.T.);
#40327=ORIENTED_EDGE('',*,*,#29464,.T.);
#40328=ORIENTED_EDGE('',*,*,#29404,.T.);
#40329=ORIENTED_EDGE('',*,*,#29344,.T.);
#40330=ORIENTED_EDGE('',*,*,#29284,.T.);
#40331=ORIENTED_EDGE('',*,*,#29356,.T.);
#40332=ORIENTED_EDGE('',*,*,#29296,.T.);
#40333=ORIENTED_EDGE('',*,*,#29236,.T.);
#40334=ORIENTED_EDGE('',*,*,#29176,.T.);
#40335=ORIENTED_EDGE('',*,*,#29116,.T.);
#40336=ORIENTED_EDGE('',*,*,#29056,.T.);
#40337=ORIENTED_EDGE('',*,*,#29410,.T.);
#40338=ORIENTED_EDGE('',*,*,#28876,.T.);
#40339=ORIENTED_EDGE('',*,*,#28936,.T.);
#40340=ORIENTED_EDGE('',*,*,#28996,.T.);
#40341=ORIENTED_EDGE('',*,*,#29512,.T.);
#40342=ORIENTED_EDGE('',*,*,#29572,.T.);
#40343=ORIENTED_EDGE('',*,*,#29038,.T.);
#40344=ORIENTED_EDGE('',*,*,#29098,.T.);
#40345=ORIENTED_EDGE('',*,*,#29212,.T.);
#40346=ORIENTED_EDGE('',*,*,#29152,.T.);
#40347=ORIENTED_EDGE('',*,*,#29092,.T.);
#40348=ORIENTED_EDGE('',*,*,#29272,.T.);
#40349=ORIENTED_EDGE('',*,*,#29332,.T.);
#40350=ORIENTED_EDGE('',*,*,#29392,.T.);
#40351=ORIENTED_EDGE('',*,*,#29452,.T.);
#40352=ORIENTED_EDGE('',*,*,#29224,.T.);
#40353=ORIENTED_EDGE('',*,*,#29164,.T.);
#40354=ORIENTED_EDGE('',*,*,#29104,.T.);
#40355=ORIENTED_EDGE('',*,*,#29044,.T.);
#40356=ORIENTED_EDGE('',*,*,#28984,.T.);
#40357=ORIENTED_EDGE('',*,*,#29518,.T.);
#40358=ORIENTED_EDGE('',*,*,#29458,.T.);
#40359=ORIENTED_EDGE('',*,*,#29398,.T.);
#40360=ORIENTED_EDGE('',*,*,#29338,.T.);
#40361=ORIENTED_EDGE('',*,*,#29278,.T.);
#40362=ORIENTED_EDGE('',*,*,#29218,.T.);
#40363=ORIENTED_EDGE('',*,*,#29158,.T.);
#40364=ORIENTED_EDGE('',*,*,#28780,.T.);
#40365=ORIENTED_EDGE('',*,*,#28720,.T.);
#40366=ORIENTED_EDGE('',*,*,#28660,.T.);
#40367=ORIENTED_EDGE('',*,*,#28840,.T.);
#40368=ORIENTED_EDGE('',*,*,#28900,.T.);
#40369=ORIENTED_EDGE('',*,*,#28960,.T.);
#40370=ORIENTED_EDGE('',*,*,#29020,.T.);
#40371=ORIENTED_EDGE('',*,*,#29194,.T.);
#40372=ORIENTED_EDGE('',*,*,#29134,.T.);
#40373=ORIENTED_EDGE('',*,*,#29074,.T.);
#40374=ORIENTED_EDGE('',*,*,#29014,.T.);
#40375=ORIENTED_EDGE('',*,*,#28954,.T.);
#40376=ORIENTED_EDGE('',*,*,#29086,.T.);
#40377=ORIENTED_EDGE('',*,*,#29026,.T.);
#40378=ORIENTED_EDGE('',*,*,#28966,.T.);
#40379=ORIENTED_EDGE('',*,*,#28906,.T.);
#40380=ORIENTED_EDGE('',*,*,#28846,.T.);
#40381=ORIENTED_EDGE('',*,*,#28786,.T.);
#40382=ORIENTED_EDGE('',*,*,#28726,.T.);
#40383=ORIENTED_EDGE('',*,*,#29080,.T.);
#40384=ORIENTED_EDGE('',*,*,#29140,.T.);
#40385=ORIENTED_EDGE('',*,*,#30226,.T.);
#40386=ORIENTED_EDGE('',*,*,#28666,.T.);
#40387=ORIENTED_EDGE('',*,*,#28768,.T.);
#40388=ORIENTED_EDGE('',*,*,#29302,.T.);
#40389=ORIENTED_EDGE('',*,*,#29242,.T.);
#40390=ORIENTED_EDGE('',*,*,#29182,.T.);
#40391=ORIENTED_EDGE('',*,*,#29122,.T.);
#40392=ORIENTED_EDGE('',*,*,#29062,.T.);
#40393=ORIENTED_EDGE('',*,*,#29002,.T.);
#40394=ORIENTED_EDGE('',*,*,#28942,.T.);
#40395=ORIENTED_EDGE('',*,*,#28882,.T.);
#40396=ORIENTED_EDGE('',*,*,#28822,.T.);
#40397=ORIENTED_EDGE('',*,*,#28894,.T.);
#40398=ORIENTED_EDGE('',*,*,#28834,.T.);
#40399=ORIENTED_EDGE('',*,*,#28774,.T.);
#40400=ORIENTED_EDGE('',*,*,#28714,.T.);
#40401=ORIENTED_EDGE('',*,*,#29248,.T.);
#40402=ORIENTED_EDGE('',*,*,#29188,.T.);
#40403=ORIENTED_EDGE('',*,*,#29128,.T.);
#40404=ORIENTED_EDGE('',*,*,#29068,.T.);
#40405=ORIENTED_EDGE('',*,*,#29008,.T.);
#40406=ORIENTED_EDGE('',*,*,#28948,.T.);
#40407=ORIENTED_EDGE('',*,*,#28888,.T.);
#40408=ORIENTED_EDGE('',*,*,#28828,.T.);
#40409=ORIENTED_EDGE('',*,*,#29950,.T.);
#40410=ORIENTED_EDGE('',*,*,#29890,.T.);
#40411=ORIENTED_EDGE('',*,*,#29830,.T.);
#40412=ORIENTED_EDGE('',*,*,#29770,.T.);
#40413=ORIENTED_EDGE('',*,*,#29710,.T.);
#40414=ORIENTED_EDGE('',*,*,#29650,.T.);
#40415=ORIENTED_EDGE('',*,*,#29590,.T.);
#40416=ORIENTED_EDGE('',*,*,#29944,.T.);
#40417=ORIENTED_EDGE('',*,*,#30004,.T.);
#40418=ORIENTED_EDGE('',*,*,#29470,.T.);
#40419=ORIENTED_EDGE('',*,*,#29530,.T.);
#40420=ORIENTED_EDGE('',*,*,#29896,.T.);
#40421=ORIENTED_EDGE('',*,*,#29836,.T.);
#40422=ORIENTED_EDGE('',*,*,#29776,.T.);
#40423=ORIENTED_EDGE('',*,*,#29716,.T.);
#40424=ORIENTED_EDGE('',*,*,#29656,.T.);
#40425=ORIENTED_EDGE('',*,*,#29596,.T.);
#40426=ORIENTED_EDGE('',*,*,#29536,.T.);
#40427=ORIENTED_EDGE('',*,*,#29476,.T.);
#40428=ORIENTED_EDGE('',*,*,#29416,.T.);
#40429=ORIENTED_EDGE('',*,*,#29758,.T.);
#40430=ORIENTED_EDGE('',*,*,#29698,.T.);
#40431=ORIENTED_EDGE('',*,*,#29638,.T.);
#40432=ORIENTED_EDGE('',*,*,#29578,.T.);
#40433=ORIENTED_EDGE('',*,*,#30112,.T.);
#40434=ORIENTED_EDGE('',*,*,#30052,.T.);
#40435=ORIENTED_EDGE('',*,*,#29992,.T.);
#40436=ORIENTED_EDGE('',*,*,#29932,.T.);
#40437=ORIENTED_EDGE('',*,*,#29872,.T.);
#40438=ORIENTED_EDGE('',*,*,#29812,.T.);
#40439=ORIENTED_EDGE('',*,*,#29752,.T.);
#40440=ORIENTED_EDGE('',*,*,#29692,.T.);
#40441=ORIENTED_EDGE('',*,*,#29644,.T.);
#40442=ORIENTED_EDGE('',*,*,#29584,.T.);
#40443=ORIENTED_EDGE('',*,*,#29524,.T.);
#40444=ORIENTED_EDGE('',*,*,#29704,.T.);
#40445=ORIENTED_EDGE('',*,*,#29764,.T.);
#40446=ORIENTED_EDGE('',*,*,#29824,.T.);
#40447=ORIENTED_EDGE('',*,*,#29884,.T.);
#40448=ORIENTED_EDGE('',*,*,#30058,.T.);
#40449=ORIENTED_EDGE('',*,*,#29998,.T.);
#40450=ORIENTED_EDGE('',*,*,#29938,.T.);
#40451=ORIENTED_EDGE('',*,*,#29878,.T.);
#40452=ORIENTED_EDGE('',*,*,#29818,.T.);
#40453=ORIENTED_EDGE('',*,*,#29680,.T.);
#40454=ORIENTED_EDGE('',*,*,#29620,.T.);
#40455=ORIENTED_EDGE('',*,*,#29560,.T.);
#40456=ORIENTED_EDGE('',*,*,#29500,.T.);
#40457=ORIENTED_EDGE('',*,*,#29440,.T.);
#40458=ORIENTED_EDGE('',*,*,#29380,.T.);
#40459=ORIENTED_EDGE('',*,*,#29320,.T.);
#40460=ORIENTED_EDGE('',*,*,#29260,.T.);
#40461=ORIENTED_EDGE('',*,*,#29200,.T.);
#40462=ORIENTED_EDGE('',*,*,#29734,.T.);
#40463=ORIENTED_EDGE('',*,*,#29674,.T.);
#40464=ORIENTED_EDGE('',*,*,#29614,.T.);
#40465=ORIENTED_EDGE('',*,*,#29626,.T.);
#40466=ORIENTED_EDGE('',*,*,#29566,.T.);
#40467=ORIENTED_EDGE('',*,*,#29506,.T.);
#40468=ORIENTED_EDGE('',*,*,#29446,.T.);
#40469=ORIENTED_EDGE('',*,*,#29386,.T.);
#40470=ORIENTED_EDGE('',*,*,#29326,.T.);
#40471=ORIENTED_EDGE('',*,*,#29266,.T.);
#40472=ORIENTED_EDGE('',*,*,#29206,.T.);
#40473=ORIENTED_EDGE('',*,*,#29146,.T.);
#40474=ORIENTED_EDGE('',*,*,#29842,.T.);
#40475=ORIENTED_EDGE('',*,*,#29308,.T.);
#40476=ORIENTED_EDGE('',*,*,#29368,.T.);
#40477=ORIENTED_EDGE('',*,*,#29428,.T.);
#40478=ORIENTED_EDGE('',*,*,#29782,.T.);
#40479=ORIENTED_EDGE('',*,*,#29722,.T.);
#40480=ORIENTED_EDGE('',*,*,#29662,.T.);
#40481=ORIENTED_EDGE('',*,*,#29602,.T.);
#40482=ORIENTED_EDGE('',*,*,#29542,.T.);
#40483=ORIENTED_EDGE('',*,*,#29482,.T.);
#40484=ORIENTED_EDGE('',*,*,#29422,.T.);
#40485=ORIENTED_EDGE('',*,*,#29362,.T.);
#40486=ORIENTED_EDGE('',*,*,#29554,.T.);
#40487=ORIENTED_EDGE('',*,*,#29494,.T.);
#40488=ORIENTED_EDGE('',*,*,#29434,.T.);
#40489=ORIENTED_EDGE('',*,*,#29374,.T.);
#40490=ORIENTED_EDGE('',*,*,#29314,.T.);
#40491=ORIENTED_EDGE('',*,*,#29254,.T.);
#40492=ORIENTED_EDGE('',*,*,#29788,.T.);
#40493=ORIENTED_EDGE('',*,*,#29728,.T.);
#40494=ORIENTED_EDGE('',*,*,#29668,.T.);
#40495=ORIENTED_EDGE('',*,*,#29608,.T.);
#40496=ORIENTED_EDGE('',*,*,#29548,.T.);
#40497=ORIENTED_EDGE('',*,*,#29488,.T.);
#40498=ORIENTED_EDGE('',*,*,#30166,.T.);
#40499=ORIENTED_EDGE('',*,*,#28690,.T.);
#40500=ORIENTED_EDGE('',*,*,#30250,.T.);
#40501=ORIENTED_EDGE('',*,*,#30190,.T.);
#40502=ORIENTED_EDGE('',*,*,#30130,.T.);
#40503=ORIENTED_EDGE('',*,*,#30070,.T.);
#40504=ORIENTED_EDGE('',*,*,#30010,.T.);
#40505=ORIENTED_EDGE('',*,*,#28924,.T.);
#40506=ORIENTED_EDGE('',*,*,#28864,.T.);
#40507=ORIENTED_EDGE('',*,*,#28804,.T.);
#40508=ORIENTED_EDGE('',*,*,#28744,.T.);
#40509=ORIENTED_EDGE('',*,*,#28684,.T.);
#40510=ORIENTED_EDGE('',*,*,#30244,.T.);
#40511=ORIENTED_EDGE('',*,*,#28816,.T.);
#40512=ORIENTED_EDGE('',*,*,#28756,.T.);
#40513=ORIENTED_EDGE('',*,*,#28696,.T.);
#40514=ORIENTED_EDGE('',*,*,#30256,.T.);
#40515=ORIENTED_EDGE('',*,*,#30196,.T.);
#40516=ORIENTED_EDGE('',*,*,#30136,.T.);
#40517=ORIENTED_EDGE('',*,*,#30076,.T.);
#40518=ORIENTED_EDGE('',*,*,#30016,.T.);
#40519=ORIENTED_EDGE('',*,*,#28750,.T.);
#40520=ORIENTED_EDGE('',*,*,#28810,.T.);
#40521=ORIENTED_EDGE('',*,*,#28870,.T.);
#40522=ORIENTED_EDGE('',*,*,#29956,.T.);
#40523=ORIENTED_EDGE('',*,*,#29032,.T.);
#40524=ORIENTED_EDGE('',*,*,#28972,.T.);
#40525=ORIENTED_EDGE('',*,*,#28912,.T.);
#40526=ORIENTED_EDGE('',*,*,#28852,.T.);
#40527=ORIENTED_EDGE('',*,*,#28792,.T.);
#40528=ORIENTED_EDGE('',*,*,#28732,.T.);
#40529=ORIENTED_EDGE('',*,*,#28672,.T.);
#40530=ORIENTED_EDGE('',*,*,#30232,.T.);
#40531=ORIENTED_EDGE('',*,*,#30172,.T.);
#40532=ORIENTED_EDGE('',*,*,#28978,.T.);
#40533=ORIENTED_EDGE('',*,*,#30064,.T.);
#40534=ORIENTED_EDGE('',*,*,#30124,.T.);
#40535=ORIENTED_EDGE('',*,*,#30184,.T.);
#40536=ORIENTED_EDGE('',*,*,#28918,.T.);
#40537=ORIENTED_EDGE('',*,*,#28858,.T.);
#40538=ORIENTED_EDGE('',*,*,#28798,.T.);
#40539=ORIENTED_EDGE('',*,*,#28738,.T.);
#40540=ORIENTED_EDGE('',*,*,#28678,.T.);
#40541=ORIENTED_EDGE('',*,*,#30238,.T.);
#40542=ORIENTED_EDGE('',*,*,#30178,.T.);
#40543=ORIENTED_EDGE('',*,*,#30118,.T.);
#40544=ORIENTED_EDGE('',*,*,#29980,.T.);
#40545=ORIENTED_EDGE('',*,*,#29920,.T.);
#40546=ORIENTED_EDGE('',*,*,#29860,.T.);
#40547=ORIENTED_EDGE('',*,*,#29800,.T.);
#40548=ORIENTED_EDGE('',*,*,#29740,.T.);
#40549=ORIENTED_EDGE('',*,*,#30274,.T.);
#40550=ORIENTED_EDGE('',*,*,#30214,.T.);
#40551=ORIENTED_EDGE('',*,*,#30154,.T.);
#40552=ORIENTED_EDGE('',*,*,#30094,.T.);
#40553=ORIENTED_EDGE('',*,*,#30034,.T.);
#40554=ORIENTED_EDGE('',*,*,#29974,.T.);
#40555=ORIENTED_EDGE('',*,*,#29914,.T.);
#40556=ORIENTED_EDGE('',*,*,#30106,.T.);
#40557=ORIENTED_EDGE('',*,*,#30046,.T.);
#40558=ORIENTED_EDGE('',*,*,#29986,.T.);
#40559=ORIENTED_EDGE('',*,*,#29926,.T.);
#40560=ORIENTED_EDGE('',*,*,#29866,.T.);
#40561=ORIENTED_EDGE('',*,*,#29806,.T.);
#40562=ORIENTED_EDGE('',*,*,#29746,.T.);
#40563=ORIENTED_EDGE('',*,*,#29686,.T.);
#40564=ORIENTED_EDGE('',*,*,#30220,.T.);
#40565=ORIENTED_EDGE('',*,*,#30160,.T.);
#40566=ORIENTED_EDGE('',*,*,#30100,.T.);
#40567=ORIENTED_EDGE('',*,*,#30040,.T.);
#40568=ORIENTED_EDGE('',*,*,#28762,.T.);
#40569=ORIENTED_EDGE('',*,*,#28702,.T.);
#40570=ORIENTED_EDGE('',*,*,#30262,.T.);
#40571=ORIENTED_EDGE('',*,*,#30202,.T.);
#40572=ORIENTED_EDGE('',*,*,#30142,.T.);
#40573=ORIENTED_EDGE('',*,*,#30082,.T.);
#40574=ORIENTED_EDGE('',*,*,#30022,.T.);
#40575=ORIENTED_EDGE('',*,*,#29962,.T.);
#40576=ORIENTED_EDGE('',*,*,#29902,.T.);
#40577=ORIENTED_EDGE('',*,*,#30268,.T.);
#40578=ORIENTED_EDGE('',*,*,#28708,.T.);
#40579=ORIENTED_EDGE('',*,*,#29794,.T.);
#40580=ORIENTED_EDGE('',*,*,#29854,.T.);
#40581=ORIENTED_EDGE('',*,*,#29848,.T.);
#40582=ORIENTED_EDGE('',*,*,#29908,.T.);
#40583=ORIENTED_EDGE('',*,*,#29968,.T.);
#40584=ORIENTED_EDGE('',*,*,#30028,.T.);
#40585=ORIENTED_EDGE('',*,*,#30088,.T.);
#40586=ORIENTED_EDGE('',*,*,#30148,.T.);
#40587=ORIENTED_EDGE('',*,*,#30208,.T.);
#40588=ORIENTED_EDGE('',*,*,#29632,.T.);
#40589=ORIENTED_EDGE('',*,*,#27755,.F.);
#40590=ORIENTED_EDGE('',*,*,#30315,.T.);
#40591=ORIENTED_EDGE('',*,*,#27757,.T.);
#40592=ORIENTED_EDGE('',*,*,#30282,.T.);
#40593=ORIENTED_EDGE('',*,*,#28371,.T.);
#40594=ORIENTED_EDGE('',*,*,#28334,.T.);
#40595=ORIENTED_EDGE('',*,*,#28298,.T.);
#40596=ORIENTED_EDGE('',*,*,#28262,.T.);
#40597=ORIENTED_EDGE('',*,*,#28241,.T.);
#40598=ORIENTED_EDGE('',*,*,#28206,.T.);
#40599=ORIENTED_EDGE('',*,*,#28234,.T.);
#40600=ORIENTED_EDGE('',*,*,#28269,.T.);
#40601=ORIENTED_EDGE('',*,*,#28305,.T.);
#40602=ORIENTED_EDGE('',*,*,#28341,.T.);
#40603=ORIENTED_EDGE('',*,*,#28319,.T.);
#40604=ORIENTED_EDGE('',*,*,#28357,.T.);
#40605=ORIENTED_EDGE('',*,*,#28392,.T.);
#40606=ORIENTED_EDGE('',*,*,#28427,.T.);
#40607=ORIENTED_EDGE('',*,*,#28455,.T.);
#40608=ORIENTED_EDGE('',*,*,#28327,.T.);
#40609=ORIENTED_EDGE('',*,*,#28364,.T.);
#40610=ORIENTED_EDGE('',*,*,#28399,.T.);
#40611=ORIENTED_EDGE('',*,*,#28290,.T.);
#40612=ORIENTED_EDGE('',*,*,#28227,.T.);
#40613=ORIENTED_EDGE('',*,*,#28192,.T.);
#40614=ORIENTED_EDGE('',*,*,#28157,.T.);
#40615=ORIENTED_EDGE('',*,*,#28122,.T.);
#40616=ORIENTED_EDGE('',*,*,#28068,.T.);
#40617=ORIENTED_EDGE('',*,*,#28094,.T.);
#40618=ORIENTED_EDGE('',*,*,#28129,.T.);
#40619=ORIENTED_EDGE('',*,*,#28164,.T.);
#40620=ORIENTED_EDGE('',*,*,#28199,.T.);
#40621=ORIENTED_EDGE('',*,*,#28283,.T.);
#40622=ORIENTED_EDGE('',*,*,#28248,.T.);
#40623=ORIENTED_EDGE('',*,*,#28213,.T.);
#40624=ORIENTED_EDGE('',*,*,#28178,.T.);
#40625=ORIENTED_EDGE('',*,*,#28312,.T.);
#40626=ORIENTED_EDGE('',*,*,#28276,.T.);
#40627=ORIENTED_EDGE('',*,*,#28255,.T.);
#40628=ORIENTED_EDGE('',*,*,#28220,.T.);
#40629=ORIENTED_EDGE('',*,*,#28185,.T.);
#40630=ORIENTED_EDGE('',*,*,#28150,.T.);
#40631=ORIENTED_EDGE('',*,*,#28509,.T.);
#40632=ORIENTED_EDGE('',*,*,#28476,.T.);
#40633=ORIENTED_EDGE('',*,*,#28441,.T.);
#40634=ORIENTED_EDGE('',*,*,#28406,.T.);
#40635=ORIENTED_EDGE('',*,*,#28420,.T.);
#40636=ORIENTED_EDGE('',*,*,#28385,.T.);
#40637=ORIENTED_EDGE('',*,*,#28352,.T.);
#40638=ORIENTED_EDGE('',*,*,#28348,.T.);
#40639=ORIENTED_EDGE('',*,*,#28483,.T.);
#40640=ORIENTED_EDGE('',*,*,#28448,.T.);
#40641=ORIENTED_EDGE('',*,*,#28413,.T.);
#40642=ORIENTED_EDGE('',*,*,#28378,.T.);
#40643=ORIENTED_EDGE('',*,*,#28462,.T.);
#40644=ORIENTED_EDGE('',*,*,#28502,.T.);
#40645=ORIENTED_EDGE('',*,*,#28469,.T.);
#40646=ORIENTED_EDGE('',*,*,#28434,.T.);
#40647=ORIENTED_EDGE('',*,*,#28143,.T.);
#40648=ORIENTED_EDGE('',*,*,#28108,.T.);
#40649=ORIENTED_EDGE('',*,*,#28075,.T.);
#40650=ORIENTED_EDGE('',*,*,#28101,.T.);
#40651=ORIENTED_EDGE('',*,*,#28136,.T.);
#40652=ORIENTED_EDGE('',*,*,#28171,.T.);
#40653=ORIENTED_EDGE('',*,*,#28115,.T.);
#40654=ORIENTED_EDGE('',*,*,#30279,.T.);
#40655=ORIENTED_EDGE('',*,*,#30276,.T.);
#40656=ORIENTED_EDGE('',*,*,#30277,.F.);
#40657=ORIENTED_EDGE('',*,*,#30273,.T.);
#40658=ORIENTED_EDGE('',*,*,#30270,.T.);
#40659=ORIENTED_EDGE('',*,*,#30271,.F.);
#40660=ORIENTED_EDGE('',*,*,#30267,.T.);
#40661=ORIENTED_EDGE('',*,*,#30264,.T.);
#40662=ORIENTED_EDGE('',*,*,#30265,.F.);
#40663=ORIENTED_EDGE('',*,*,#30261,.T.);
#40664=ORIENTED_EDGE('',*,*,#30258,.T.);
#40665=ORIENTED_EDGE('',*,*,#30259,.F.);
#40666=ORIENTED_EDGE('',*,*,#30255,.T.);
#40667=ORIENTED_EDGE('',*,*,#30252,.T.);
#40668=ORIENTED_EDGE('',*,*,#30253,.F.);
#40669=ORIENTED_EDGE('',*,*,#30249,.T.);
#40670=ORIENTED_EDGE('',*,*,#30246,.T.);
#40671=ORIENTED_EDGE('',*,*,#30247,.F.);
#40672=ORIENTED_EDGE('',*,*,#30243,.T.);
#40673=ORIENTED_EDGE('',*,*,#30240,.T.);
#40674=ORIENTED_EDGE('',*,*,#30241,.F.);
#40675=ORIENTED_EDGE('',*,*,#30237,.T.);
#40676=ORIENTED_EDGE('',*,*,#30234,.T.);
#40677=ORIENTED_EDGE('',*,*,#30235,.F.);
#40678=ORIENTED_EDGE('',*,*,#30231,.T.);
#40679=ORIENTED_EDGE('',*,*,#30228,.T.);
#40680=ORIENTED_EDGE('',*,*,#30229,.F.);
#40681=ORIENTED_EDGE('',*,*,#30225,.T.);
#40682=ORIENTED_EDGE('',*,*,#30222,.T.);
#40683=ORIENTED_EDGE('',*,*,#30223,.F.);
#40684=ORIENTED_EDGE('',*,*,#30219,.T.);
#40685=ORIENTED_EDGE('',*,*,#30216,.T.);
#40686=ORIENTED_EDGE('',*,*,#30217,.F.);
#40687=ORIENTED_EDGE('',*,*,#30213,.T.);
#40688=ORIENTED_EDGE('',*,*,#30210,.T.);
#40689=ORIENTED_EDGE('',*,*,#30211,.F.);
#40690=ORIENTED_EDGE('',*,*,#30207,.T.);
#40691=ORIENTED_EDGE('',*,*,#30204,.T.);
#40692=ORIENTED_EDGE('',*,*,#30205,.F.);
#40693=ORIENTED_EDGE('',*,*,#30201,.T.);
#40694=ORIENTED_EDGE('',*,*,#30198,.T.);
#40695=ORIENTED_EDGE('',*,*,#30199,.F.);
#40696=ORIENTED_EDGE('',*,*,#30195,.T.);
#40697=ORIENTED_EDGE('',*,*,#30192,.T.);
#40698=ORIENTED_EDGE('',*,*,#30193,.F.);
#40699=ORIENTED_EDGE('',*,*,#30189,.T.);
#40700=ORIENTED_EDGE('',*,*,#30186,.T.);
#40701=ORIENTED_EDGE('',*,*,#30187,.F.);
#40702=ORIENTED_EDGE('',*,*,#30183,.T.);
#40703=ORIENTED_EDGE('',*,*,#30180,.T.);
#40704=ORIENTED_EDGE('',*,*,#30181,.F.);
#40705=ORIENTED_EDGE('',*,*,#30177,.T.);
#40706=ORIENTED_EDGE('',*,*,#30174,.T.);
#40707=ORIENTED_EDGE('',*,*,#30175,.F.);
#40708=ORIENTED_EDGE('',*,*,#30171,.T.);
#40709=ORIENTED_EDGE('',*,*,#30168,.T.);
#40710=ORIENTED_EDGE('',*,*,#30169,.F.);
#40711=ORIENTED_EDGE('',*,*,#30165,.T.);
#40712=ORIENTED_EDGE('',*,*,#30162,.T.);
#40713=ORIENTED_EDGE('',*,*,#30163,.F.);
#40714=ORIENTED_EDGE('',*,*,#30159,.T.);
#40715=ORIENTED_EDGE('',*,*,#30156,.T.);
#40716=ORIENTED_EDGE('',*,*,#30157,.F.);
#40717=ORIENTED_EDGE('',*,*,#30153,.T.);
#40718=ORIENTED_EDGE('',*,*,#30150,.T.);
#40719=ORIENTED_EDGE('',*,*,#30151,.F.);
#40720=ORIENTED_EDGE('',*,*,#30147,.T.);
#40721=ORIENTED_EDGE('',*,*,#30144,.T.);
#40722=ORIENTED_EDGE('',*,*,#30145,.F.);
#40723=ORIENTED_EDGE('',*,*,#30141,.T.);
#40724=ORIENTED_EDGE('',*,*,#30138,.T.);
#40725=ORIENTED_EDGE('',*,*,#30139,.F.);
#40726=ORIENTED_EDGE('',*,*,#30135,.T.);
#40727=ORIENTED_EDGE('',*,*,#30132,.T.);
#40728=ORIENTED_EDGE('',*,*,#30133,.F.);
#40729=ORIENTED_EDGE('',*,*,#30129,.T.);
#40730=ORIENTED_EDGE('',*,*,#30126,.T.);
#40731=ORIENTED_EDGE('',*,*,#30127,.F.);
#40732=ORIENTED_EDGE('',*,*,#30123,.T.);
#40733=ORIENTED_EDGE('',*,*,#30120,.T.);
#40734=ORIENTED_EDGE('',*,*,#30121,.F.);
#40735=ORIENTED_EDGE('',*,*,#30117,.T.);
#40736=ORIENTED_EDGE('',*,*,#30114,.T.);
#40737=ORIENTED_EDGE('',*,*,#30115,.F.);
#40738=ORIENTED_EDGE('',*,*,#30111,.T.);
#40739=ORIENTED_EDGE('',*,*,#30108,.T.);
#40740=ORIENTED_EDGE('',*,*,#30109,.F.);
#40741=ORIENTED_EDGE('',*,*,#30105,.T.);
#40742=ORIENTED_EDGE('',*,*,#30102,.T.);
#40743=ORIENTED_EDGE('',*,*,#30103,.F.);
#40744=ORIENTED_EDGE('',*,*,#30099,.T.);
#40745=ORIENTED_EDGE('',*,*,#30096,.T.);
#40746=ORIENTED_EDGE('',*,*,#30097,.F.);
#40747=ORIENTED_EDGE('',*,*,#30093,.T.);
#40748=ORIENTED_EDGE('',*,*,#30090,.T.);
#40749=ORIENTED_EDGE('',*,*,#30091,.F.);
#40750=ORIENTED_EDGE('',*,*,#30087,.T.);
#40751=ORIENTED_EDGE('',*,*,#30084,.T.);
#40752=ORIENTED_EDGE('',*,*,#30085,.F.);
#40753=ORIENTED_EDGE('',*,*,#30081,.T.);
#40754=ORIENTED_EDGE('',*,*,#30078,.T.);
#40755=ORIENTED_EDGE('',*,*,#30079,.F.);
#40756=ORIENTED_EDGE('',*,*,#30075,.T.);
#40757=ORIENTED_EDGE('',*,*,#30072,.T.);
#40758=ORIENTED_EDGE('',*,*,#30073,.F.);
#40759=ORIENTED_EDGE('',*,*,#30069,.T.);
#40760=ORIENTED_EDGE('',*,*,#30066,.T.);
#40761=ORIENTED_EDGE('',*,*,#30067,.F.);
#40762=ORIENTED_EDGE('',*,*,#30063,.T.);
#40763=ORIENTED_EDGE('',*,*,#30060,.T.);
#40764=ORIENTED_EDGE('',*,*,#30061,.F.);
#40765=ORIENTED_EDGE('',*,*,#30057,.T.);
#40766=ORIENTED_EDGE('',*,*,#30054,.T.);
#40767=ORIENTED_EDGE('',*,*,#30055,.F.);
#40768=ORIENTED_EDGE('',*,*,#30051,.T.);
#40769=ORIENTED_EDGE('',*,*,#30048,.T.);
#40770=ORIENTED_EDGE('',*,*,#30049,.F.);
#40771=ORIENTED_EDGE('',*,*,#30045,.T.);
#40772=ORIENTED_EDGE('',*,*,#30042,.T.);
#40773=ORIENTED_EDGE('',*,*,#30043,.F.);
#40774=ORIENTED_EDGE('',*,*,#30039,.T.);
#40775=ORIENTED_EDGE('',*,*,#30036,.T.);
#40776=ORIENTED_EDGE('',*,*,#30037,.F.);
#40777=ORIENTED_EDGE('',*,*,#30033,.T.);
#40778=ORIENTED_EDGE('',*,*,#30030,.T.);
#40779=ORIENTED_EDGE('',*,*,#30031,.F.);
#40780=ORIENTED_EDGE('',*,*,#30027,.T.);
#40781=ORIENTED_EDGE('',*,*,#30024,.T.);
#40782=ORIENTED_EDGE('',*,*,#30025,.F.);
#40783=ORIENTED_EDGE('',*,*,#30021,.T.);
#40784=ORIENTED_EDGE('',*,*,#30018,.T.);
#40785=ORIENTED_EDGE('',*,*,#30019,.F.);
#40786=ORIENTED_EDGE('',*,*,#30015,.T.);
#40787=ORIENTED_EDGE('',*,*,#30012,.T.);
#40788=ORIENTED_EDGE('',*,*,#30013,.F.);
#40789=ORIENTED_EDGE('',*,*,#30009,.T.);
#40790=ORIENTED_EDGE('',*,*,#30006,.T.);
#40791=ORIENTED_EDGE('',*,*,#30007,.F.);
#40792=ORIENTED_EDGE('',*,*,#30003,.T.);
#40793=ORIENTED_EDGE('',*,*,#30000,.T.);
#40794=ORIENTED_EDGE('',*,*,#30001,.F.);
#40795=ORIENTED_EDGE('',*,*,#29997,.T.);
#40796=ORIENTED_EDGE('',*,*,#29994,.T.);
#40797=ORIENTED_EDGE('',*,*,#29995,.F.);
#40798=ORIENTED_EDGE('',*,*,#29991,.T.);
#40799=ORIENTED_EDGE('',*,*,#29988,.T.);
#40800=ORIENTED_EDGE('',*,*,#29989,.F.);
#40801=ORIENTED_EDGE('',*,*,#29985,.T.);
#40802=ORIENTED_EDGE('',*,*,#29982,.T.);
#40803=ORIENTED_EDGE('',*,*,#29983,.F.);
#40804=ORIENTED_EDGE('',*,*,#29979,.T.);
#40805=ORIENTED_EDGE('',*,*,#29976,.T.);
#40806=ORIENTED_EDGE('',*,*,#29977,.F.);
#40807=ORIENTED_EDGE('',*,*,#29973,.T.);
#40808=ORIENTED_EDGE('',*,*,#29970,.T.);
#40809=ORIENTED_EDGE('',*,*,#29971,.F.);
#40810=ORIENTED_EDGE('',*,*,#29967,.T.);
#40811=ORIENTED_EDGE('',*,*,#29964,.T.);
#40812=ORIENTED_EDGE('',*,*,#29965,.F.);
#40813=ORIENTED_EDGE('',*,*,#29961,.T.);
#40814=ORIENTED_EDGE('',*,*,#29958,.T.);
#40815=ORIENTED_EDGE('',*,*,#29959,.F.);
#40816=ORIENTED_EDGE('',*,*,#29955,.T.);
#40817=ORIENTED_EDGE('',*,*,#29952,.T.);
#40818=ORIENTED_EDGE('',*,*,#29953,.F.);
#40819=ORIENTED_EDGE('',*,*,#29949,.T.);
#40820=ORIENTED_EDGE('',*,*,#29946,.T.);
#40821=ORIENTED_EDGE('',*,*,#29947,.F.);
#40822=ORIENTED_EDGE('',*,*,#29943,.T.);
#40823=ORIENTED_EDGE('',*,*,#29940,.T.);
#40824=ORIENTED_EDGE('',*,*,#29941,.F.);
#40825=ORIENTED_EDGE('',*,*,#29937,.T.);
#40826=ORIENTED_EDGE('',*,*,#29934,.T.);
#40827=ORIENTED_EDGE('',*,*,#29935,.F.);
#40828=ORIENTED_EDGE('',*,*,#29931,.T.);
#40829=ORIENTED_EDGE('',*,*,#29928,.T.);
#40830=ORIENTED_EDGE('',*,*,#29929,.F.);
#40831=ORIENTED_EDGE('',*,*,#29925,.T.);
#40832=ORIENTED_EDGE('',*,*,#29922,.T.);
#40833=ORIENTED_EDGE('',*,*,#29923,.F.);
#40834=ORIENTED_EDGE('',*,*,#29919,.T.);
#40835=ORIENTED_EDGE('',*,*,#29916,.T.);
#40836=ORIENTED_EDGE('',*,*,#29917,.F.);
#40837=ORIENTED_EDGE('',*,*,#29913,.T.);
#40838=ORIENTED_EDGE('',*,*,#29910,.T.);
#40839=ORIENTED_EDGE('',*,*,#29911,.F.);
#40840=ORIENTED_EDGE('',*,*,#29907,.T.);
#40841=ORIENTED_EDGE('',*,*,#29904,.T.);
#40842=ORIENTED_EDGE('',*,*,#29905,.F.);
#40843=ORIENTED_EDGE('',*,*,#29901,.T.);
#40844=ORIENTED_EDGE('',*,*,#29898,.T.);
#40845=ORIENTED_EDGE('',*,*,#29899,.F.);
#40846=ORIENTED_EDGE('',*,*,#29895,.T.);
#40847=ORIENTED_EDGE('',*,*,#29892,.T.);
#40848=ORIENTED_EDGE('',*,*,#29893,.F.);
#40849=ORIENTED_EDGE('',*,*,#29889,.T.);
#40850=ORIENTED_EDGE('',*,*,#29886,.T.);
#40851=ORIENTED_EDGE('',*,*,#29887,.F.);
#40852=ORIENTED_EDGE('',*,*,#29883,.T.);
#40853=ORIENTED_EDGE('',*,*,#29880,.T.);
#40854=ORIENTED_EDGE('',*,*,#29881,.F.);
#40855=ORIENTED_EDGE('',*,*,#29877,.T.);
#40856=ORIENTED_EDGE('',*,*,#29874,.T.);
#40857=ORIENTED_EDGE('',*,*,#29875,.F.);
#40858=ORIENTED_EDGE('',*,*,#29871,.T.);
#40859=ORIENTED_EDGE('',*,*,#29868,.T.);
#40860=ORIENTED_EDGE('',*,*,#29869,.F.);
#40861=ORIENTED_EDGE('',*,*,#29865,.T.);
#40862=ORIENTED_EDGE('',*,*,#29862,.T.);
#40863=ORIENTED_EDGE('',*,*,#29863,.F.);
#40864=ORIENTED_EDGE('',*,*,#29859,.T.);
#40865=ORIENTED_EDGE('',*,*,#29856,.T.);
#40866=ORIENTED_EDGE('',*,*,#29857,.F.);
#40867=ORIENTED_EDGE('',*,*,#29853,.T.);
#40868=ORIENTED_EDGE('',*,*,#29850,.T.);
#40869=ORIENTED_EDGE('',*,*,#29851,.F.);
#40870=ORIENTED_EDGE('',*,*,#29847,.T.);
#40871=ORIENTED_EDGE('',*,*,#29844,.T.);
#40872=ORIENTED_EDGE('',*,*,#29845,.F.);
#40873=ORIENTED_EDGE('',*,*,#29841,.T.);
#40874=ORIENTED_EDGE('',*,*,#29838,.T.);
#40875=ORIENTED_EDGE('',*,*,#29839,.F.);
#40876=ORIENTED_EDGE('',*,*,#29835,.T.);
#40877=ORIENTED_EDGE('',*,*,#29832,.T.);
#40878=ORIENTED_EDGE('',*,*,#29833,.F.);
#40879=ORIENTED_EDGE('',*,*,#29829,.T.);
#40880=ORIENTED_EDGE('',*,*,#29826,.T.);
#40881=ORIENTED_EDGE('',*,*,#29827,.F.);
#40882=ORIENTED_EDGE('',*,*,#29823,.T.);
#40883=ORIENTED_EDGE('',*,*,#29820,.T.);
#40884=ORIENTED_EDGE('',*,*,#29821,.F.);
#40885=ORIENTED_EDGE('',*,*,#29817,.T.);
#40886=ORIENTED_EDGE('',*,*,#29814,.T.);
#40887=ORIENTED_EDGE('',*,*,#29815,.F.);
#40888=ORIENTED_EDGE('',*,*,#29811,.T.);
#40889=ORIENTED_EDGE('',*,*,#29808,.T.);
#40890=ORIENTED_EDGE('',*,*,#29809,.F.);
#40891=ORIENTED_EDGE('',*,*,#29805,.T.);
#40892=ORIENTED_EDGE('',*,*,#29802,.T.);
#40893=ORIENTED_EDGE('',*,*,#29803,.F.);
#40894=ORIENTED_EDGE('',*,*,#29799,.T.);
#40895=ORIENTED_EDGE('',*,*,#29796,.T.);
#40896=ORIENTED_EDGE('',*,*,#29797,.F.);
#40897=ORIENTED_EDGE('',*,*,#29793,.T.);
#40898=ORIENTED_EDGE('',*,*,#29790,.T.);
#40899=ORIENTED_EDGE('',*,*,#29791,.F.);
#40900=ORIENTED_EDGE('',*,*,#29787,.T.);
#40901=ORIENTED_EDGE('',*,*,#29784,.T.);
#40902=ORIENTED_EDGE('',*,*,#29785,.F.);
#40903=ORIENTED_EDGE('',*,*,#29781,.T.);
#40904=ORIENTED_EDGE('',*,*,#29778,.T.);
#40905=ORIENTED_EDGE('',*,*,#29779,.F.);
#40906=ORIENTED_EDGE('',*,*,#29775,.T.);
#40907=ORIENTED_EDGE('',*,*,#29772,.T.);
#40908=ORIENTED_EDGE('',*,*,#29773,.F.);
#40909=ORIENTED_EDGE('',*,*,#29769,.T.);
#40910=ORIENTED_EDGE('',*,*,#29766,.T.);
#40911=ORIENTED_EDGE('',*,*,#29767,.F.);
#40912=ORIENTED_EDGE('',*,*,#29763,.T.);
#40913=ORIENTED_EDGE('',*,*,#29760,.T.);
#40914=ORIENTED_EDGE('',*,*,#29761,.F.);
#40915=ORIENTED_EDGE('',*,*,#29757,.T.);
#40916=ORIENTED_EDGE('',*,*,#29754,.T.);
#40917=ORIENTED_EDGE('',*,*,#29755,.F.);
#40918=ORIENTED_EDGE('',*,*,#29751,.T.);
#40919=ORIENTED_EDGE('',*,*,#29748,.T.);
#40920=ORIENTED_EDGE('',*,*,#29749,.F.);
#40921=ORIENTED_EDGE('',*,*,#29745,.T.);
#40922=ORIENTED_EDGE('',*,*,#29742,.T.);
#40923=ORIENTED_EDGE('',*,*,#29743,.F.);
#40924=ORIENTED_EDGE('',*,*,#29739,.T.);
#40925=ORIENTED_EDGE('',*,*,#29736,.T.);
#40926=ORIENTED_EDGE('',*,*,#29737,.F.);
#40927=ORIENTED_EDGE('',*,*,#29733,.T.);
#40928=ORIENTED_EDGE('',*,*,#29730,.T.);
#40929=ORIENTED_EDGE('',*,*,#29731,.F.);
#40930=ORIENTED_EDGE('',*,*,#29727,.T.);
#40931=ORIENTED_EDGE('',*,*,#29724,.T.);
#40932=ORIENTED_EDGE('',*,*,#29725,.F.);
#40933=ORIENTED_EDGE('',*,*,#29721,.T.);
#40934=ORIENTED_EDGE('',*,*,#29718,.T.);
#40935=ORIENTED_EDGE('',*,*,#29719,.F.);
#40936=ORIENTED_EDGE('',*,*,#29715,.T.);
#40937=ORIENTED_EDGE('',*,*,#29712,.T.);
#40938=ORIENTED_EDGE('',*,*,#29713,.F.);
#40939=ORIENTED_EDGE('',*,*,#29709,.T.);
#40940=ORIENTED_EDGE('',*,*,#29706,.T.);
#40941=ORIENTED_EDGE('',*,*,#29707,.F.);
#40942=ORIENTED_EDGE('',*,*,#29703,.T.);
#40943=ORIENTED_EDGE('',*,*,#29700,.T.);
#40944=ORIENTED_EDGE('',*,*,#29701,.F.);
#40945=ORIENTED_EDGE('',*,*,#29697,.T.);
#40946=ORIENTED_EDGE('',*,*,#29694,.T.);
#40947=ORIENTED_EDGE('',*,*,#29695,.F.);
#40948=ORIENTED_EDGE('',*,*,#29691,.T.);
#40949=ORIENTED_EDGE('',*,*,#29688,.T.);
#40950=ORIENTED_EDGE('',*,*,#29689,.F.);
#40951=ORIENTED_EDGE('',*,*,#29685,.T.);
#40952=ORIENTED_EDGE('',*,*,#29682,.T.);
#40953=ORIENTED_EDGE('',*,*,#29683,.F.);
#40954=ORIENTED_EDGE('',*,*,#29679,.T.);
#40955=ORIENTED_EDGE('',*,*,#29676,.T.);
#40956=ORIENTED_EDGE('',*,*,#29677,.F.);
#40957=ORIENTED_EDGE('',*,*,#29673,.T.);
#40958=ORIENTED_EDGE('',*,*,#29670,.T.);
#40959=ORIENTED_EDGE('',*,*,#29671,.F.);
#40960=ORIENTED_EDGE('',*,*,#29667,.T.);
#40961=ORIENTED_EDGE('',*,*,#29664,.T.);
#40962=ORIENTED_EDGE('',*,*,#29665,.F.);
#40963=ORIENTED_EDGE('',*,*,#29661,.T.);
#40964=ORIENTED_EDGE('',*,*,#29658,.T.);
#40965=ORIENTED_EDGE('',*,*,#29659,.F.);
#40966=ORIENTED_EDGE('',*,*,#29655,.T.);
#40967=ORIENTED_EDGE('',*,*,#29652,.T.);
#40968=ORIENTED_EDGE('',*,*,#29653,.F.);
#40969=ORIENTED_EDGE('',*,*,#29649,.T.);
#40970=ORIENTED_EDGE('',*,*,#29646,.T.);
#40971=ORIENTED_EDGE('',*,*,#29647,.F.);
#40972=ORIENTED_EDGE('',*,*,#29643,.T.);
#40973=ORIENTED_EDGE('',*,*,#29640,.T.);
#40974=ORIENTED_EDGE('',*,*,#29641,.F.);
#40975=ORIENTED_EDGE('',*,*,#29637,.T.);
#40976=ORIENTED_EDGE('',*,*,#29634,.T.);
#40977=ORIENTED_EDGE('',*,*,#29635,.F.);
#40978=ORIENTED_EDGE('',*,*,#29631,.T.);
#40979=ORIENTED_EDGE('',*,*,#29628,.T.);
#40980=ORIENTED_EDGE('',*,*,#29629,.F.);
#40981=ORIENTED_EDGE('',*,*,#29625,.T.);
#40982=ORIENTED_EDGE('',*,*,#29622,.T.);
#40983=ORIENTED_EDGE('',*,*,#29623,.F.);
#40984=ORIENTED_EDGE('',*,*,#29619,.T.);
#40985=ORIENTED_EDGE('',*,*,#29616,.T.);
#40986=ORIENTED_EDGE('',*,*,#29617,.F.);
#40987=ORIENTED_EDGE('',*,*,#29613,.T.);
#40988=ORIENTED_EDGE('',*,*,#29610,.T.);
#40989=ORIENTED_EDGE('',*,*,#29611,.F.);
#40990=ORIENTED_EDGE('',*,*,#29607,.T.);
#40991=ORIENTED_EDGE('',*,*,#29604,.T.);
#40992=ORIENTED_EDGE('',*,*,#29605,.F.);
#40993=ORIENTED_EDGE('',*,*,#29601,.T.);
#40994=ORIENTED_EDGE('',*,*,#29598,.T.);
#40995=ORIENTED_EDGE('',*,*,#29599,.F.);
#40996=ORIENTED_EDGE('',*,*,#29595,.T.);
#40997=ORIENTED_EDGE('',*,*,#29592,.T.);
#40998=ORIENTED_EDGE('',*,*,#29593,.F.);
#40999=ORIENTED_EDGE('',*,*,#29589,.T.);
#41000=ORIENTED_EDGE('',*,*,#29586,.T.);
#41001=ORIENTED_EDGE('',*,*,#29587,.F.);
#41002=ORIENTED_EDGE('',*,*,#29583,.T.);
#41003=ORIENTED_EDGE('',*,*,#29580,.T.);
#41004=ORIENTED_EDGE('',*,*,#29581,.F.);
#41005=ORIENTED_EDGE('',*,*,#29577,.T.);
#41006=ORIENTED_EDGE('',*,*,#29574,.T.);
#41007=ORIENTED_EDGE('',*,*,#29575,.F.);
#41008=ORIENTED_EDGE('',*,*,#29571,.T.);
#41009=ORIENTED_EDGE('',*,*,#29568,.T.);
#41010=ORIENTED_EDGE('',*,*,#29569,.F.);
#41011=ORIENTED_EDGE('',*,*,#29565,.T.);
#41012=ORIENTED_EDGE('',*,*,#29562,.T.);
#41013=ORIENTED_EDGE('',*,*,#29563,.F.);
#41014=ORIENTED_EDGE('',*,*,#29559,.T.);
#41015=ORIENTED_EDGE('',*,*,#29556,.T.);
#41016=ORIENTED_EDGE('',*,*,#29557,.F.);
#41017=ORIENTED_EDGE('',*,*,#29553,.T.);
#41018=ORIENTED_EDGE('',*,*,#29550,.T.);
#41019=ORIENTED_EDGE('',*,*,#29551,.F.);
#41020=ORIENTED_EDGE('',*,*,#29547,.T.);
#41021=ORIENTED_EDGE('',*,*,#29544,.T.);
#41022=ORIENTED_EDGE('',*,*,#29545,.F.);
#41023=ORIENTED_EDGE('',*,*,#29541,.T.);
#41024=ORIENTED_EDGE('',*,*,#29538,.T.);
#41025=ORIENTED_EDGE('',*,*,#29539,.F.);
#41026=ORIENTED_EDGE('',*,*,#29535,.T.);
#41027=ORIENTED_EDGE('',*,*,#29532,.T.);
#41028=ORIENTED_EDGE('',*,*,#29533,.F.);
#41029=ORIENTED_EDGE('',*,*,#29529,.T.);
#41030=ORIENTED_EDGE('',*,*,#29526,.T.);
#41031=ORIENTED_EDGE('',*,*,#29527,.F.);
#41032=ORIENTED_EDGE('',*,*,#29523,.T.);
#41033=ORIENTED_EDGE('',*,*,#29520,.T.);
#41034=ORIENTED_EDGE('',*,*,#29521,.F.);
#41035=ORIENTED_EDGE('',*,*,#29517,.T.);
#41036=ORIENTED_EDGE('',*,*,#29514,.T.);
#41037=ORIENTED_EDGE('',*,*,#29515,.F.);
#41038=ORIENTED_EDGE('',*,*,#29511,.T.);
#41039=ORIENTED_EDGE('',*,*,#29508,.T.);
#41040=ORIENTED_EDGE('',*,*,#29509,.F.);
#41041=ORIENTED_EDGE('',*,*,#29505,.T.);
#41042=ORIENTED_EDGE('',*,*,#29502,.T.);
#41043=ORIENTED_EDGE('',*,*,#29503,.F.);
#41044=ORIENTED_EDGE('',*,*,#29499,.T.);
#41045=ORIENTED_EDGE('',*,*,#29496,.T.);
#41046=ORIENTED_EDGE('',*,*,#29497,.F.);
#41047=ORIENTED_EDGE('',*,*,#29493,.T.);
#41048=ORIENTED_EDGE('',*,*,#29490,.T.);
#41049=ORIENTED_EDGE('',*,*,#29491,.F.);
#41050=ORIENTED_EDGE('',*,*,#29487,.T.);
#41051=ORIENTED_EDGE('',*,*,#29484,.T.);
#41052=ORIENTED_EDGE('',*,*,#29485,.F.);
#41053=ORIENTED_EDGE('',*,*,#29481,.T.);
#41054=ORIENTED_EDGE('',*,*,#29478,.T.);
#41055=ORIENTED_EDGE('',*,*,#29479,.F.);
#41056=ORIENTED_EDGE('',*,*,#29475,.T.);
#41057=ORIENTED_EDGE('',*,*,#29472,.T.);
#41058=ORIENTED_EDGE('',*,*,#29473,.F.);
#41059=ORIENTED_EDGE('',*,*,#29469,.T.);
#41060=ORIENTED_EDGE('',*,*,#29466,.T.);
#41061=ORIENTED_EDGE('',*,*,#29467,.F.);
#41062=ORIENTED_EDGE('',*,*,#29463,.T.);
#41063=ORIENTED_EDGE('',*,*,#29460,.T.);
#41064=ORIENTED_EDGE('',*,*,#29461,.F.);
#41065=ORIENTED_EDGE('',*,*,#29457,.T.);
#41066=ORIENTED_EDGE('',*,*,#29454,.T.);
#41067=ORIENTED_EDGE('',*,*,#29455,.F.);
#41068=ORIENTED_EDGE('',*,*,#29451,.T.);
#41069=ORIENTED_EDGE('',*,*,#29448,.T.);
#41070=ORIENTED_EDGE('',*,*,#29449,.F.);
#41071=ORIENTED_EDGE('',*,*,#29445,.T.);
#41072=ORIENTED_EDGE('',*,*,#29442,.T.);
#41073=ORIENTED_EDGE('',*,*,#29443,.F.);
#41074=ORIENTED_EDGE('',*,*,#29439,.T.);
#41075=ORIENTED_EDGE('',*,*,#29436,.T.);
#41076=ORIENTED_EDGE('',*,*,#29437,.F.);
#41077=ORIENTED_EDGE('',*,*,#29433,.T.);
#41078=ORIENTED_EDGE('',*,*,#29430,.T.);
#41079=ORIENTED_EDGE('',*,*,#29431,.F.);
#41080=ORIENTED_EDGE('',*,*,#29427,.T.);
#41081=ORIENTED_EDGE('',*,*,#29424,.T.);
#41082=ORIENTED_EDGE('',*,*,#29425,.F.);
#41083=ORIENTED_EDGE('',*,*,#29421,.T.);
#41084=ORIENTED_EDGE('',*,*,#29418,.T.);
#41085=ORIENTED_EDGE('',*,*,#29419,.F.);
#41086=ORIENTED_EDGE('',*,*,#29415,.T.);
#41087=ORIENTED_EDGE('',*,*,#29412,.T.);
#41088=ORIENTED_EDGE('',*,*,#29413,.F.);
#41089=ORIENTED_EDGE('',*,*,#29409,.T.);
#41090=ORIENTED_EDGE('',*,*,#29406,.T.);
#41091=ORIENTED_EDGE('',*,*,#29407,.F.);
#41092=ORIENTED_EDGE('',*,*,#29403,.T.);
#41093=ORIENTED_EDGE('',*,*,#29400,.T.);
#41094=ORIENTED_EDGE('',*,*,#29401,.F.);
#41095=ORIENTED_EDGE('',*,*,#29397,.T.);
#41096=ORIENTED_EDGE('',*,*,#29394,.T.);
#41097=ORIENTED_EDGE('',*,*,#29395,.F.);
#41098=ORIENTED_EDGE('',*,*,#29391,.T.);
#41099=ORIENTED_EDGE('',*,*,#29388,.T.);
#41100=ORIENTED_EDGE('',*,*,#29389,.F.);
#41101=ORIENTED_EDGE('',*,*,#29385,.T.);
#41102=ORIENTED_EDGE('',*,*,#29382,.T.);
#41103=ORIENTED_EDGE('',*,*,#29383,.F.);
#41104=ORIENTED_EDGE('',*,*,#29379,.T.);
#41105=ORIENTED_EDGE('',*,*,#29376,.T.);
#41106=ORIENTED_EDGE('',*,*,#29377,.F.);
#41107=ORIENTED_EDGE('',*,*,#29373,.T.);
#41108=ORIENTED_EDGE('',*,*,#29370,.T.);
#41109=ORIENTED_EDGE('',*,*,#29371,.F.);
#41110=ORIENTED_EDGE('',*,*,#29367,.T.);
#41111=ORIENTED_EDGE('',*,*,#29364,.T.);
#41112=ORIENTED_EDGE('',*,*,#29365,.F.);
#41113=ORIENTED_EDGE('',*,*,#29361,.T.);
#41114=ORIENTED_EDGE('',*,*,#29358,.T.);
#41115=ORIENTED_EDGE('',*,*,#29359,.F.);
#41116=ORIENTED_EDGE('',*,*,#29355,.T.);
#41117=ORIENTED_EDGE('',*,*,#29352,.T.);
#41118=ORIENTED_EDGE('',*,*,#29353,.F.);
#41119=ORIENTED_EDGE('',*,*,#29349,.T.);
#41120=ORIENTED_EDGE('',*,*,#29346,.T.);
#41121=ORIENTED_EDGE('',*,*,#29347,.F.);
#41122=ORIENTED_EDGE('',*,*,#29343,.T.);
#41123=ORIENTED_EDGE('',*,*,#29340,.T.);
#41124=ORIENTED_EDGE('',*,*,#29341,.F.);
#41125=ORIENTED_EDGE('',*,*,#29337,.T.);
#41126=ORIENTED_EDGE('',*,*,#29334,.T.);
#41127=ORIENTED_EDGE('',*,*,#29335,.F.);
#41128=ORIENTED_EDGE('',*,*,#29331,.T.);
#41129=ORIENTED_EDGE('',*,*,#29328,.T.);
#41130=ORIENTED_EDGE('',*,*,#29329,.F.);
#41131=ORIENTED_EDGE('',*,*,#29325,.T.);
#41132=ORIENTED_EDGE('',*,*,#29322,.T.);
#41133=ORIENTED_EDGE('',*,*,#29323,.F.);
#41134=ORIENTED_EDGE('',*,*,#29319,.T.);
#41135=ORIENTED_EDGE('',*,*,#29316,.T.);
#41136=ORIENTED_EDGE('',*,*,#29317,.F.);
#41137=ORIENTED_EDGE('',*,*,#29313,.T.);
#41138=ORIENTED_EDGE('',*,*,#29310,.T.);
#41139=ORIENTED_EDGE('',*,*,#29311,.F.);
#41140=ORIENTED_EDGE('',*,*,#29307,.T.);
#41141=ORIENTED_EDGE('',*,*,#29304,.T.);
#41142=ORIENTED_EDGE('',*,*,#29305,.F.);
#41143=ORIENTED_EDGE('',*,*,#29301,.T.);
#41144=ORIENTED_EDGE('',*,*,#29298,.T.);
#41145=ORIENTED_EDGE('',*,*,#29299,.F.);
#41146=ORIENTED_EDGE('',*,*,#29295,.T.);
#41147=ORIENTED_EDGE('',*,*,#29292,.T.);
#41148=ORIENTED_EDGE('',*,*,#29293,.F.);
#41149=ORIENTED_EDGE('',*,*,#29289,.T.);
#41150=ORIENTED_EDGE('',*,*,#29286,.T.);
#41151=ORIENTED_EDGE('',*,*,#29287,.F.);
#41152=ORIENTED_EDGE('',*,*,#29283,.T.);
#41153=ORIENTED_EDGE('',*,*,#29280,.T.);
#41154=ORIENTED_EDGE('',*,*,#29281,.F.);
#41155=ORIENTED_EDGE('',*,*,#29277,.T.);
#41156=ORIENTED_EDGE('',*,*,#29274,.T.);
#41157=ORIENTED_EDGE('',*,*,#29275,.F.);
#41158=ORIENTED_EDGE('',*,*,#29271,.T.);
#41159=ORIENTED_EDGE('',*,*,#29268,.T.);
#41160=ORIENTED_EDGE('',*,*,#29269,.F.);
#41161=ORIENTED_EDGE('',*,*,#29265,.T.);
#41162=ORIENTED_EDGE('',*,*,#29262,.T.);
#41163=ORIENTED_EDGE('',*,*,#29263,.F.);
#41164=ORIENTED_EDGE('',*,*,#29259,.T.);
#41165=ORIENTED_EDGE('',*,*,#29256,.T.);
#41166=ORIENTED_EDGE('',*,*,#29257,.F.);
#41167=ORIENTED_EDGE('',*,*,#29253,.T.);
#41168=ORIENTED_EDGE('',*,*,#29250,.T.);
#41169=ORIENTED_EDGE('',*,*,#29251,.F.);
#41170=ORIENTED_EDGE('',*,*,#29247,.T.);
#41171=ORIENTED_EDGE('',*,*,#29244,.T.);
#41172=ORIENTED_EDGE('',*,*,#29245,.F.);
#41173=ORIENTED_EDGE('',*,*,#29241,.T.);
#41174=ORIENTED_EDGE('',*,*,#29238,.T.);
#41175=ORIENTED_EDGE('',*,*,#29239,.F.);
#41176=ORIENTED_EDGE('',*,*,#29235,.T.);
#41177=ORIENTED_EDGE('',*,*,#29232,.T.);
#41178=ORIENTED_EDGE('',*,*,#29233,.F.);
#41179=ORIENTED_EDGE('',*,*,#29229,.T.);
#41180=ORIENTED_EDGE('',*,*,#29226,.T.);
#41181=ORIENTED_EDGE('',*,*,#29227,.F.);
#41182=ORIENTED_EDGE('',*,*,#29223,.T.);
#41183=ORIENTED_EDGE('',*,*,#29220,.T.);
#41184=ORIENTED_EDGE('',*,*,#29221,.F.);
#41185=ORIENTED_EDGE('',*,*,#29217,.T.);
#41186=ORIENTED_EDGE('',*,*,#29214,.T.);
#41187=ORIENTED_EDGE('',*,*,#29215,.F.);
#41188=ORIENTED_EDGE('',*,*,#29211,.T.);
#41189=ORIENTED_EDGE('',*,*,#29208,.T.);
#41190=ORIENTED_EDGE('',*,*,#29209,.F.);
#41191=ORIENTED_EDGE('',*,*,#29205,.T.);
#41192=ORIENTED_EDGE('',*,*,#29202,.T.);
#41193=ORIENTED_EDGE('',*,*,#29203,.F.);
#41194=ORIENTED_EDGE('',*,*,#29199,.T.);
#41195=ORIENTED_EDGE('',*,*,#29196,.T.);
#41196=ORIENTED_EDGE('',*,*,#29197,.F.);
#41197=ORIENTED_EDGE('',*,*,#29193,.T.);
#41198=ORIENTED_EDGE('',*,*,#29190,.T.);
#41199=ORIENTED_EDGE('',*,*,#29191,.F.);
#41200=ORIENTED_EDGE('',*,*,#29187,.T.);
#41201=ORIENTED_EDGE('',*,*,#29184,.T.);
#41202=ORIENTED_EDGE('',*,*,#29185,.F.);
#41203=ORIENTED_EDGE('',*,*,#29181,.T.);
#41204=ORIENTED_EDGE('',*,*,#29178,.T.);
#41205=ORIENTED_EDGE('',*,*,#29179,.F.);
#41206=ORIENTED_EDGE('',*,*,#29175,.T.);
#41207=ORIENTED_EDGE('',*,*,#29172,.T.);
#41208=ORIENTED_EDGE('',*,*,#29173,.F.);
#41209=ORIENTED_EDGE('',*,*,#29169,.T.);
#41210=ORIENTED_EDGE('',*,*,#29166,.T.);
#41211=ORIENTED_EDGE('',*,*,#29167,.F.);
#41212=ORIENTED_EDGE('',*,*,#29163,.T.);
#41213=ORIENTED_EDGE('',*,*,#29160,.T.);
#41214=ORIENTED_EDGE('',*,*,#29161,.F.);
#41215=ORIENTED_EDGE('',*,*,#29157,.T.);
#41216=ORIENTED_EDGE('',*,*,#29154,.T.);
#41217=ORIENTED_EDGE('',*,*,#29155,.F.);
#41218=ORIENTED_EDGE('',*,*,#29151,.T.);
#41219=ORIENTED_EDGE('',*,*,#29148,.T.);
#41220=ORIENTED_EDGE('',*,*,#29149,.F.);
#41221=ORIENTED_EDGE('',*,*,#29145,.T.);
#41222=ORIENTED_EDGE('',*,*,#29142,.T.);
#41223=ORIENTED_EDGE('',*,*,#29143,.F.);
#41224=ORIENTED_EDGE('',*,*,#29139,.T.);
#41225=ORIENTED_EDGE('',*,*,#29136,.T.);
#41226=ORIENTED_EDGE('',*,*,#29137,.F.);
#41227=ORIENTED_EDGE('',*,*,#29133,.T.);
#41228=ORIENTED_EDGE('',*,*,#29130,.T.);
#41229=ORIENTED_EDGE('',*,*,#29131,.F.);
#41230=ORIENTED_EDGE('',*,*,#29127,.T.);
#41231=ORIENTED_EDGE('',*,*,#29124,.T.);
#41232=ORIENTED_EDGE('',*,*,#29125,.F.);
#41233=ORIENTED_EDGE('',*,*,#29121,.T.);
#41234=ORIENTED_EDGE('',*,*,#29118,.T.);
#41235=ORIENTED_EDGE('',*,*,#29119,.F.);
#41236=ORIENTED_EDGE('',*,*,#29115,.T.);
#41237=ORIENTED_EDGE('',*,*,#29112,.T.);
#41238=ORIENTED_EDGE('',*,*,#29113,.F.);
#41239=ORIENTED_EDGE('',*,*,#29109,.T.);
#41240=ORIENTED_EDGE('',*,*,#29106,.T.);
#41241=ORIENTED_EDGE('',*,*,#29107,.F.);
#41242=ORIENTED_EDGE('',*,*,#29103,.T.);
#41243=ORIENTED_EDGE('',*,*,#29100,.T.);
#41244=ORIENTED_EDGE('',*,*,#29101,.F.);
#41245=ORIENTED_EDGE('',*,*,#29097,.T.);
#41246=ORIENTED_EDGE('',*,*,#29094,.T.);
#41247=ORIENTED_EDGE('',*,*,#29095,.F.);
#41248=ORIENTED_EDGE('',*,*,#29091,.T.);
#41249=ORIENTED_EDGE('',*,*,#29088,.T.);
#41250=ORIENTED_EDGE('',*,*,#29089,.F.);
#41251=ORIENTED_EDGE('',*,*,#29085,.T.);
#41252=ORIENTED_EDGE('',*,*,#29082,.T.);
#41253=ORIENTED_EDGE('',*,*,#29083,.F.);
#41254=ORIENTED_EDGE('',*,*,#29079,.T.);
#41255=ORIENTED_EDGE('',*,*,#29076,.T.);
#41256=ORIENTED_EDGE('',*,*,#29077,.F.);
#41257=ORIENTED_EDGE('',*,*,#29073,.T.);
#41258=ORIENTED_EDGE('',*,*,#29070,.T.);
#41259=ORIENTED_EDGE('',*,*,#29071,.F.);
#41260=ORIENTED_EDGE('',*,*,#29067,.T.);
#41261=ORIENTED_EDGE('',*,*,#29064,.T.);
#41262=ORIENTED_EDGE('',*,*,#29065,.F.);
#41263=ORIENTED_EDGE('',*,*,#29061,.T.);
#41264=ORIENTED_EDGE('',*,*,#29058,.T.);
#41265=ORIENTED_EDGE('',*,*,#29059,.F.);
#41266=ORIENTED_EDGE('',*,*,#29055,.T.);
#41267=ORIENTED_EDGE('',*,*,#29052,.T.);
#41268=ORIENTED_EDGE('',*,*,#29053,.F.);
#41269=ORIENTED_EDGE('',*,*,#29049,.T.);
#41270=ORIENTED_EDGE('',*,*,#29046,.T.);
#41271=ORIENTED_EDGE('',*,*,#29047,.F.);
#41272=ORIENTED_EDGE('',*,*,#29043,.T.);
#41273=ORIENTED_EDGE('',*,*,#29040,.T.);
#41274=ORIENTED_EDGE('',*,*,#29041,.F.);
#41275=ORIENTED_EDGE('',*,*,#29037,.T.);
#41276=ORIENTED_EDGE('',*,*,#29034,.T.);
#41277=ORIENTED_EDGE('',*,*,#29035,.F.);
#41278=ORIENTED_EDGE('',*,*,#29031,.T.);
#41279=ORIENTED_EDGE('',*,*,#29028,.T.);
#41280=ORIENTED_EDGE('',*,*,#29029,.F.);
#41281=ORIENTED_EDGE('',*,*,#29025,.T.);
#41282=ORIENTED_EDGE('',*,*,#29022,.T.);
#41283=ORIENTED_EDGE('',*,*,#29023,.F.);
#41284=ORIENTED_EDGE('',*,*,#29019,.T.);
#41285=ORIENTED_EDGE('',*,*,#29016,.T.);
#41286=ORIENTED_EDGE('',*,*,#29017,.F.);
#41287=ORIENTED_EDGE('',*,*,#29013,.T.);
#41288=ORIENTED_EDGE('',*,*,#29010,.T.);
#41289=ORIENTED_EDGE('',*,*,#29011,.F.);
#41290=ORIENTED_EDGE('',*,*,#29007,.T.);
#41291=ORIENTED_EDGE('',*,*,#29004,.T.);
#41292=ORIENTED_EDGE('',*,*,#29005,.F.);
#41293=ORIENTED_EDGE('',*,*,#29001,.T.);
#41294=ORIENTED_EDGE('',*,*,#28998,.T.);
#41295=ORIENTED_EDGE('',*,*,#28999,.F.);
#41296=ORIENTED_EDGE('',*,*,#28995,.T.);
#41297=ORIENTED_EDGE('',*,*,#28992,.T.);
#41298=ORIENTED_EDGE('',*,*,#28993,.F.);
#41299=ORIENTED_EDGE('',*,*,#28989,.T.);
#41300=ORIENTED_EDGE('',*,*,#28986,.T.);
#41301=ORIENTED_EDGE('',*,*,#28987,.F.);
#41302=ORIENTED_EDGE('',*,*,#28983,.T.);
#41303=ORIENTED_EDGE('',*,*,#28980,.T.);
#41304=ORIENTED_EDGE('',*,*,#28981,.F.);
#41305=ORIENTED_EDGE('',*,*,#28977,.T.);
#41306=ORIENTED_EDGE('',*,*,#28974,.T.);
#41307=ORIENTED_EDGE('',*,*,#28975,.F.);
#41308=ORIENTED_EDGE('',*,*,#28971,.T.);
#41309=ORIENTED_EDGE('',*,*,#28968,.T.);
#41310=ORIENTED_EDGE('',*,*,#28969,.F.);
#41311=ORIENTED_EDGE('',*,*,#28965,.T.);
#41312=ORIENTED_EDGE('',*,*,#28962,.T.);
#41313=ORIENTED_EDGE('',*,*,#28963,.F.);
#41314=ORIENTED_EDGE('',*,*,#28959,.T.);
#41315=ORIENTED_EDGE('',*,*,#28956,.T.);
#41316=ORIENTED_EDGE('',*,*,#28957,.F.);
#41317=ORIENTED_EDGE('',*,*,#28953,.T.);
#41318=ORIENTED_EDGE('',*,*,#28950,.T.);
#41319=ORIENTED_EDGE('',*,*,#28951,.F.);
#41320=ORIENTED_EDGE('',*,*,#28947,.T.);
#41321=ORIENTED_EDGE('',*,*,#28944,.T.);
#41322=ORIENTED_EDGE('',*,*,#28945,.F.);
#41323=ORIENTED_EDGE('',*,*,#28941,.T.);
#41324=ORIENTED_EDGE('',*,*,#28938,.T.);
#41325=ORIENTED_EDGE('',*,*,#28939,.F.);
#41326=ORIENTED_EDGE('',*,*,#28935,.T.);
#41327=ORIENTED_EDGE('',*,*,#28932,.T.);
#41328=ORIENTED_EDGE('',*,*,#28933,.F.);
#41329=ORIENTED_EDGE('',*,*,#28929,.T.);
#41330=ORIENTED_EDGE('',*,*,#28926,.T.);
#41331=ORIENTED_EDGE('',*,*,#28927,.F.);
#41332=ORIENTED_EDGE('',*,*,#28923,.T.);
#41333=ORIENTED_EDGE('',*,*,#28920,.T.);
#41334=ORIENTED_EDGE('',*,*,#28921,.F.);
#41335=ORIENTED_EDGE('',*,*,#28917,.T.);
#41336=ORIENTED_EDGE('',*,*,#28914,.T.);
#41337=ORIENTED_EDGE('',*,*,#28915,.F.);
#41338=ORIENTED_EDGE('',*,*,#28911,.T.);
#41339=ORIENTED_EDGE('',*,*,#28908,.T.);
#41340=ORIENTED_EDGE('',*,*,#28909,.F.);
#41341=ORIENTED_EDGE('',*,*,#28905,.T.);
#41342=ORIENTED_EDGE('',*,*,#28902,.T.);
#41343=ORIENTED_EDGE('',*,*,#28903,.F.);
#41344=ORIENTED_EDGE('',*,*,#28899,.T.);
#41345=ORIENTED_EDGE('',*,*,#28896,.T.);
#41346=ORIENTED_EDGE('',*,*,#28897,.F.);
#41347=ORIENTED_EDGE('',*,*,#28893,.T.);
#41348=ORIENTED_EDGE('',*,*,#28890,.T.);
#41349=ORIENTED_EDGE('',*,*,#28891,.F.);
#41350=ORIENTED_EDGE('',*,*,#28887,.T.);
#41351=ORIENTED_EDGE('',*,*,#28884,.T.);
#41352=ORIENTED_EDGE('',*,*,#28885,.F.);
#41353=ORIENTED_EDGE('',*,*,#28881,.T.);
#41354=ORIENTED_EDGE('',*,*,#28878,.T.);
#41355=ORIENTED_EDGE('',*,*,#28879,.F.);
#41356=ORIENTED_EDGE('',*,*,#28875,.T.);
#41357=ORIENTED_EDGE('',*,*,#28872,.T.);
#41358=ORIENTED_EDGE('',*,*,#28873,.F.);
#41359=ORIENTED_EDGE('',*,*,#28869,.T.);
#41360=ORIENTED_EDGE('',*,*,#28866,.T.);
#41361=ORIENTED_EDGE('',*,*,#28867,.F.);
#41362=ORIENTED_EDGE('',*,*,#28863,.T.);
#41363=ORIENTED_EDGE('',*,*,#28860,.T.);
#41364=ORIENTED_EDGE('',*,*,#28861,.F.);
#41365=ORIENTED_EDGE('',*,*,#28857,.T.);
#41366=ORIENTED_EDGE('',*,*,#28854,.T.);
#41367=ORIENTED_EDGE('',*,*,#28855,.F.);
#41368=ORIENTED_EDGE('',*,*,#28851,.T.);
#41369=ORIENTED_EDGE('',*,*,#28848,.T.);
#41370=ORIENTED_EDGE('',*,*,#28849,.F.);
#41371=ORIENTED_EDGE('',*,*,#28845,.T.);
#41372=ORIENTED_EDGE('',*,*,#28842,.T.);
#41373=ORIENTED_EDGE('',*,*,#28843,.F.);
#41374=ORIENTED_EDGE('',*,*,#28839,.T.);
#41375=ORIENTED_EDGE('',*,*,#28836,.T.);
#41376=ORIENTED_EDGE('',*,*,#28837,.F.);
#41377=ORIENTED_EDGE('',*,*,#28833,.T.);
#41378=ORIENTED_EDGE('',*,*,#28830,.T.);
#41379=ORIENTED_EDGE('',*,*,#28831,.F.);
#41380=ORIENTED_EDGE('',*,*,#28827,.T.);
#41381=ORIENTED_EDGE('',*,*,#28824,.T.);
#41382=ORIENTED_EDGE('',*,*,#28825,.F.);
#41383=ORIENTED_EDGE('',*,*,#28821,.T.);
#41384=ORIENTED_EDGE('',*,*,#28818,.T.);
#41385=ORIENTED_EDGE('',*,*,#28819,.F.);
#41386=ORIENTED_EDGE('',*,*,#28815,.T.);
#41387=ORIENTED_EDGE('',*,*,#28812,.T.);
#41388=ORIENTED_EDGE('',*,*,#28813,.F.);
#41389=ORIENTED_EDGE('',*,*,#28809,.T.);
#41390=ORIENTED_EDGE('',*,*,#28806,.T.);
#41391=ORIENTED_EDGE('',*,*,#28807,.F.);
#41392=ORIENTED_EDGE('',*,*,#28803,.T.);
#41393=ORIENTED_EDGE('',*,*,#28800,.T.);
#41394=ORIENTED_EDGE('',*,*,#28801,.F.);
#41395=ORIENTED_EDGE('',*,*,#28797,.T.);
#41396=ORIENTED_EDGE('',*,*,#28794,.T.);
#41397=ORIENTED_EDGE('',*,*,#28795,.F.);
#41398=ORIENTED_EDGE('',*,*,#28791,.T.);
#41399=ORIENTED_EDGE('',*,*,#28788,.T.);
#41400=ORIENTED_EDGE('',*,*,#28789,.F.);
#41401=ORIENTED_EDGE('',*,*,#28785,.T.);
#41402=ORIENTED_EDGE('',*,*,#28782,.T.);
#41403=ORIENTED_EDGE('',*,*,#28783,.F.);
#41404=ORIENTED_EDGE('',*,*,#28779,.T.);
#41405=ORIENTED_EDGE('',*,*,#28776,.T.);
#41406=ORIENTED_EDGE('',*,*,#28777,.F.);
#41407=ORIENTED_EDGE('',*,*,#28773,.T.);
#41408=ORIENTED_EDGE('',*,*,#28770,.T.);
#41409=ORIENTED_EDGE('',*,*,#28771,.F.);
#41410=ORIENTED_EDGE('',*,*,#28767,.T.);
#41411=ORIENTED_EDGE('',*,*,#28764,.T.);
#41412=ORIENTED_EDGE('',*,*,#28765,.F.);
#41413=ORIENTED_EDGE('',*,*,#28761,.T.);
#41414=ORIENTED_EDGE('',*,*,#28758,.T.);
#41415=ORIENTED_EDGE('',*,*,#28759,.F.);
#41416=ORIENTED_EDGE('',*,*,#28755,.T.);
#41417=ORIENTED_EDGE('',*,*,#28752,.T.);
#41418=ORIENTED_EDGE('',*,*,#28753,.F.);
#41419=ORIENTED_EDGE('',*,*,#28749,.T.);
#41420=ORIENTED_EDGE('',*,*,#28746,.T.);
#41421=ORIENTED_EDGE('',*,*,#28747,.F.);
#41422=ORIENTED_EDGE('',*,*,#28743,.T.);
#41423=ORIENTED_EDGE('',*,*,#28740,.T.);
#41424=ORIENTED_EDGE('',*,*,#28741,.F.);
#41425=ORIENTED_EDGE('',*,*,#28737,.T.);
#41426=ORIENTED_EDGE('',*,*,#28734,.T.);
#41427=ORIENTED_EDGE('',*,*,#28735,.F.);
#41428=ORIENTED_EDGE('',*,*,#28731,.T.);
#41429=ORIENTED_EDGE('',*,*,#28728,.T.);
#41430=ORIENTED_EDGE('',*,*,#28729,.F.);
#41431=ORIENTED_EDGE('',*,*,#28725,.T.);
#41432=ORIENTED_EDGE('',*,*,#28722,.T.);
#41433=ORIENTED_EDGE('',*,*,#28723,.F.);
#41434=ORIENTED_EDGE('',*,*,#28719,.T.);
#41435=ORIENTED_EDGE('',*,*,#28716,.T.);
#41436=ORIENTED_EDGE('',*,*,#28717,.F.);
#41437=ORIENTED_EDGE('',*,*,#28713,.T.);
#41438=ORIENTED_EDGE('',*,*,#28710,.T.);
#41439=ORIENTED_EDGE('',*,*,#28711,.F.);
#41440=ORIENTED_EDGE('',*,*,#28707,.T.);
#41441=ORIENTED_EDGE('',*,*,#28704,.T.);
#41442=ORIENTED_EDGE('',*,*,#28705,.F.);
#41443=ORIENTED_EDGE('',*,*,#28701,.T.);
#41444=ORIENTED_EDGE('',*,*,#28698,.T.);
#41445=ORIENTED_EDGE('',*,*,#28699,.F.);
#41446=ORIENTED_EDGE('',*,*,#28695,.T.);
#41447=ORIENTED_EDGE('',*,*,#28692,.T.);
#41448=ORIENTED_EDGE('',*,*,#28693,.F.);
#41449=ORIENTED_EDGE('',*,*,#28689,.T.);
#41450=ORIENTED_EDGE('',*,*,#28686,.T.);
#41451=ORIENTED_EDGE('',*,*,#28687,.F.);
#41452=ORIENTED_EDGE('',*,*,#28683,.T.);
#41453=ORIENTED_EDGE('',*,*,#28680,.T.);
#41454=ORIENTED_EDGE('',*,*,#28681,.F.);
#41455=ORIENTED_EDGE('',*,*,#28677,.T.);
#41456=ORIENTED_EDGE('',*,*,#28674,.T.);
#41457=ORIENTED_EDGE('',*,*,#28675,.F.);
#41458=ORIENTED_EDGE('',*,*,#28671,.T.);
#41459=ORIENTED_EDGE('',*,*,#28668,.T.);
#41460=ORIENTED_EDGE('',*,*,#28669,.F.);
#41461=ORIENTED_EDGE('',*,*,#28665,.T.);
#41462=ORIENTED_EDGE('',*,*,#28662,.T.);
#41463=ORIENTED_EDGE('',*,*,#28663,.F.);
#41464=ORIENTED_EDGE('',*,*,#28658,.T.);
#41465=ORIENTED_EDGE('',*,*,#28655,.T.);
#41466=ORIENTED_EDGE('',*,*,#28656,.F.);
#41467=ORIENTED_EDGE('',*,*,#28659,.F.);
#41468=ORIENTED_EDGE('',*,*,#28652,.T.);
#41469=ORIENTED_EDGE('',*,*,#28649,.T.);
#41470=ORIENTED_EDGE('',*,*,#28650,.F.);
#41471=ORIENTED_EDGE('',*,*,#28653,.F.);
#41472=ORIENTED_EDGE('',*,*,#28646,.T.);
#41473=ORIENTED_EDGE('',*,*,#28643,.T.);
#41474=ORIENTED_EDGE('',*,*,#28644,.F.);
#41475=ORIENTED_EDGE('',*,*,#28647,.F.);
#41476=ORIENTED_EDGE('',*,*,#28640,.T.);
#41477=ORIENTED_EDGE('',*,*,#28637,.T.);
#41478=ORIENTED_EDGE('',*,*,#28638,.F.);
#41479=ORIENTED_EDGE('',*,*,#28641,.F.);
#41480=ORIENTED_EDGE('',*,*,#28634,.T.);
#41481=ORIENTED_EDGE('',*,*,#28631,.T.);
#41482=ORIENTED_EDGE('',*,*,#28632,.F.);
#41483=ORIENTED_EDGE('',*,*,#28635,.F.);
#41484=ORIENTED_EDGE('',*,*,#28628,.T.);
#41485=ORIENTED_EDGE('',*,*,#28625,.T.);
#41486=ORIENTED_EDGE('',*,*,#28626,.F.);
#41487=ORIENTED_EDGE('',*,*,#28629,.F.);
#41488=ORIENTED_EDGE('',*,*,#28622,.T.);
#41489=ORIENTED_EDGE('',*,*,#28619,.T.);
#41490=ORIENTED_EDGE('',*,*,#28620,.F.);
#41491=ORIENTED_EDGE('',*,*,#28623,.F.);
#41492=ORIENTED_EDGE('',*,*,#28616,.T.);
#41493=ORIENTED_EDGE('',*,*,#28613,.T.);
#41494=ORIENTED_EDGE('',*,*,#28614,.F.);
#41495=ORIENTED_EDGE('',*,*,#28617,.F.);
#41496=ORIENTED_EDGE('',*,*,#28610,.T.);
#41497=ORIENTED_EDGE('',*,*,#28607,.T.);
#41498=ORIENTED_EDGE('',*,*,#28608,.F.);
#41499=ORIENTED_EDGE('',*,*,#28611,.F.);
#41500=ORIENTED_EDGE('',*,*,#28604,.T.);
#41501=ORIENTED_EDGE('',*,*,#28601,.T.);
#41502=ORIENTED_EDGE('',*,*,#28602,.F.);
#41503=ORIENTED_EDGE('',*,*,#28605,.F.);
#41504=ORIENTED_EDGE('',*,*,#28598,.T.);
#41505=ORIENTED_EDGE('',*,*,#28595,.T.);
#41506=ORIENTED_EDGE('',*,*,#28596,.F.);
#41507=ORIENTED_EDGE('',*,*,#28599,.F.);
#41508=ORIENTED_EDGE('',*,*,#28592,.T.);
#41509=ORIENTED_EDGE('',*,*,#28589,.T.);
#41510=ORIENTED_EDGE('',*,*,#28590,.F.);
#41511=ORIENTED_EDGE('',*,*,#28593,.F.);
#41512=ORIENTED_EDGE('',*,*,#28586,.T.);
#41513=ORIENTED_EDGE('',*,*,#28583,.T.);
#41514=ORIENTED_EDGE('',*,*,#28584,.F.);
#41515=ORIENTED_EDGE('',*,*,#28587,.F.);
#41516=ORIENTED_EDGE('',*,*,#28580,.T.);
#41517=ORIENTED_EDGE('',*,*,#28577,.T.);
#41518=ORIENTED_EDGE('',*,*,#28578,.F.);
#41519=ORIENTED_EDGE('',*,*,#28581,.F.);
#41520=ORIENTED_EDGE('',*,*,#28574,.T.);
#41521=ORIENTED_EDGE('',*,*,#28571,.T.);
#41522=ORIENTED_EDGE('',*,*,#28572,.F.);
#41523=ORIENTED_EDGE('',*,*,#28575,.F.);
#41524=ORIENTED_EDGE('',*,*,#28568,.T.);
#41525=ORIENTED_EDGE('',*,*,#28565,.T.);
#41526=ORIENTED_EDGE('',*,*,#28566,.F.);
#41527=ORIENTED_EDGE('',*,*,#28569,.F.);
#41528=ORIENTED_EDGE('',*,*,#28562,.T.);
#41529=ORIENTED_EDGE('',*,*,#28559,.T.);
#41530=ORIENTED_EDGE('',*,*,#28560,.F.);
#41531=ORIENTED_EDGE('',*,*,#28563,.F.);
#41532=ORIENTED_EDGE('',*,*,#28556,.T.);
#41533=ORIENTED_EDGE('',*,*,#28553,.T.);
#41534=ORIENTED_EDGE('',*,*,#28554,.F.);
#41535=ORIENTED_EDGE('',*,*,#28557,.F.);
#41536=ORIENTED_EDGE('',*,*,#28550,.T.);
#41537=ORIENTED_EDGE('',*,*,#28547,.T.);
#41538=ORIENTED_EDGE('',*,*,#28548,.F.);
#41539=ORIENTED_EDGE('',*,*,#28551,.F.);
#41540=ORIENTED_EDGE('',*,*,#28544,.T.);
#41541=ORIENTED_EDGE('',*,*,#28541,.T.);
#41542=ORIENTED_EDGE('',*,*,#28542,.F.);
#41543=ORIENTED_EDGE('',*,*,#28545,.F.);
#41544=ORIENTED_EDGE('',*,*,#28538,.T.);
#41545=ORIENTED_EDGE('',*,*,#28535,.T.);
#41546=ORIENTED_EDGE('',*,*,#28536,.F.);
#41547=ORIENTED_EDGE('',*,*,#28539,.F.);
#41548=ORIENTED_EDGE('',*,*,#28532,.T.);
#41549=ORIENTED_EDGE('',*,*,#28529,.T.);
#41550=ORIENTED_EDGE('',*,*,#28530,.F.);
#41551=ORIENTED_EDGE('',*,*,#28533,.F.);
#41552=ORIENTED_EDGE('',*,*,#28526,.T.);
#41553=ORIENTED_EDGE('',*,*,#28523,.T.);
#41554=ORIENTED_EDGE('',*,*,#28524,.F.);
#41555=ORIENTED_EDGE('',*,*,#28527,.F.);
#41556=ORIENTED_EDGE('',*,*,#28520,.T.);
#41557=ORIENTED_EDGE('',*,*,#28517,.T.);
#41558=ORIENTED_EDGE('',*,*,#28518,.F.);
#41559=ORIENTED_EDGE('',*,*,#28521,.F.);
#41560=ORIENTED_EDGE('',*,*,#28514,.T.);
#41561=ORIENTED_EDGE('',*,*,#28511,.T.);
#41562=ORIENTED_EDGE('',*,*,#28512,.F.);
#41563=ORIENTED_EDGE('',*,*,#28515,.F.);
#41564=ORIENTED_EDGE('',*,*,#28507,.T.);
#41565=ORIENTED_EDGE('',*,*,#28504,.T.);
#41566=ORIENTED_EDGE('',*,*,#28505,.F.);
#41567=ORIENTED_EDGE('',*,*,#28508,.F.);
#41568=ORIENTED_EDGE('',*,*,#28500,.T.);
#41569=ORIENTED_EDGE('',*,*,#28497,.T.);
#41570=ORIENTED_EDGE('',*,*,#28498,.F.);
#41571=ORIENTED_EDGE('',*,*,#28501,.F.);
#41572=ORIENTED_EDGE('',*,*,#28494,.T.);
#41573=ORIENTED_EDGE('',*,*,#28491,.T.);
#41574=ORIENTED_EDGE('',*,*,#28492,.F.);
#41575=ORIENTED_EDGE('',*,*,#28495,.F.);
#41576=ORIENTED_EDGE('',*,*,#28488,.T.);
#41577=ORIENTED_EDGE('',*,*,#28485,.T.);
#41578=ORIENTED_EDGE('',*,*,#28486,.F.);
#41579=ORIENTED_EDGE('',*,*,#28489,.F.);
#41580=ORIENTED_EDGE('',*,*,#28481,.T.);
#41581=ORIENTED_EDGE('',*,*,#28478,.T.);
#41582=ORIENTED_EDGE('',*,*,#28479,.F.);
#41583=ORIENTED_EDGE('',*,*,#28482,.F.);
#41584=ORIENTED_EDGE('',*,*,#28474,.T.);
#41585=ORIENTED_EDGE('',*,*,#28471,.T.);
#41586=ORIENTED_EDGE('',*,*,#28472,.F.);
#41587=ORIENTED_EDGE('',*,*,#28475,.F.);
#41588=ORIENTED_EDGE('',*,*,#28467,.T.);
#41589=ORIENTED_EDGE('',*,*,#28464,.T.);
#41590=ORIENTED_EDGE('',*,*,#28465,.F.);
#41591=ORIENTED_EDGE('',*,*,#28468,.F.);
#41592=ORIENTED_EDGE('',*,*,#28460,.T.);
#41593=ORIENTED_EDGE('',*,*,#28457,.T.);
#41594=ORIENTED_EDGE('',*,*,#28458,.F.);
#41595=ORIENTED_EDGE('',*,*,#28461,.F.);
#41596=ORIENTED_EDGE('',*,*,#28453,.T.);
#41597=ORIENTED_EDGE('',*,*,#28450,.T.);
#41598=ORIENTED_EDGE('',*,*,#28451,.F.);
#41599=ORIENTED_EDGE('',*,*,#28454,.F.);
#41600=ORIENTED_EDGE('',*,*,#28446,.T.);
#41601=ORIENTED_EDGE('',*,*,#28443,.T.);
#41602=ORIENTED_EDGE('',*,*,#28444,.F.);
#41603=ORIENTED_EDGE('',*,*,#28447,.F.);
#41604=ORIENTED_EDGE('',*,*,#28439,.T.);
#41605=ORIENTED_EDGE('',*,*,#28436,.T.);
#41606=ORIENTED_EDGE('',*,*,#28437,.F.);
#41607=ORIENTED_EDGE('',*,*,#28440,.F.);
#41608=ORIENTED_EDGE('',*,*,#28432,.T.);
#41609=ORIENTED_EDGE('',*,*,#28429,.T.);
#41610=ORIENTED_EDGE('',*,*,#28430,.F.);
#41611=ORIENTED_EDGE('',*,*,#28433,.F.);
#41612=ORIENTED_EDGE('',*,*,#28425,.T.);
#41613=ORIENTED_EDGE('',*,*,#28422,.T.);
#41614=ORIENTED_EDGE('',*,*,#28423,.F.);
#41615=ORIENTED_EDGE('',*,*,#28426,.F.);
#41616=ORIENTED_EDGE('',*,*,#28418,.T.);
#41617=ORIENTED_EDGE('',*,*,#28415,.T.);
#41618=ORIENTED_EDGE('',*,*,#28416,.F.);
#41619=ORIENTED_EDGE('',*,*,#28419,.F.);
#41620=ORIENTED_EDGE('',*,*,#28411,.T.);
#41621=ORIENTED_EDGE('',*,*,#28408,.T.);
#41622=ORIENTED_EDGE('',*,*,#28409,.F.);
#41623=ORIENTED_EDGE('',*,*,#28412,.F.);
#41624=ORIENTED_EDGE('',*,*,#28404,.T.);
#41625=ORIENTED_EDGE('',*,*,#28401,.T.);
#41626=ORIENTED_EDGE('',*,*,#28402,.F.);
#41627=ORIENTED_EDGE('',*,*,#28405,.F.);
#41628=ORIENTED_EDGE('',*,*,#28397,.T.);
#41629=ORIENTED_EDGE('',*,*,#28394,.T.);
#41630=ORIENTED_EDGE('',*,*,#28395,.F.);
#41631=ORIENTED_EDGE('',*,*,#28398,.F.);
#41632=ORIENTED_EDGE('',*,*,#28390,.T.);
#41633=ORIENTED_EDGE('',*,*,#28387,.T.);
#41634=ORIENTED_EDGE('',*,*,#28388,.F.);
#41635=ORIENTED_EDGE('',*,*,#28391,.F.);
#41636=ORIENTED_EDGE('',*,*,#28383,.T.);
#41637=ORIENTED_EDGE('',*,*,#28380,.T.);
#41638=ORIENTED_EDGE('',*,*,#28381,.F.);
#41639=ORIENTED_EDGE('',*,*,#28384,.F.);
#41640=ORIENTED_EDGE('',*,*,#28376,.T.);
#41641=ORIENTED_EDGE('',*,*,#28373,.T.);
#41642=ORIENTED_EDGE('',*,*,#28374,.F.);
#41643=ORIENTED_EDGE('',*,*,#28377,.F.);
#41644=ORIENTED_EDGE('',*,*,#28369,.T.);
#41645=ORIENTED_EDGE('',*,*,#28366,.T.);
#41646=ORIENTED_EDGE('',*,*,#28367,.F.);
#41647=ORIENTED_EDGE('',*,*,#28370,.F.);
#41648=ORIENTED_EDGE('',*,*,#28362,.T.);
#41649=ORIENTED_EDGE('',*,*,#28359,.T.);
#41650=ORIENTED_EDGE('',*,*,#28360,.F.);
#41651=ORIENTED_EDGE('',*,*,#28363,.F.);
#41652=ORIENTED_EDGE('',*,*,#28355,.T.);
#41653=ORIENTED_EDGE('',*,*,#28350,.T.);
#41654=ORIENTED_EDGE('',*,*,#28351,.T.);
#41655=ORIENTED_EDGE('',*,*,#28353,.F.);
#41656=ORIENTED_EDGE('',*,*,#28356,.F.);
#41657=ORIENTED_EDGE('',*,*,#28346,.T.);
#41658=ORIENTED_EDGE('',*,*,#28343,.T.);
#41659=ORIENTED_EDGE('',*,*,#28344,.F.);
#41660=ORIENTED_EDGE('',*,*,#28347,.F.);
#41661=ORIENTED_EDGE('',*,*,#28339,.T.);
#41662=ORIENTED_EDGE('',*,*,#28336,.T.);
#41663=ORIENTED_EDGE('',*,*,#28337,.F.);
#41664=ORIENTED_EDGE('',*,*,#28340,.F.);
#41665=ORIENTED_EDGE('',*,*,#28332,.T.);
#41666=ORIENTED_EDGE('',*,*,#28329,.T.);
#41667=ORIENTED_EDGE('',*,*,#28330,.F.);
#41668=ORIENTED_EDGE('',*,*,#28333,.F.);
#41669=ORIENTED_EDGE('',*,*,#28325,.T.);
#41670=ORIENTED_EDGE('',*,*,#28321,.T.);
#41671=ORIENTED_EDGE('',*,*,#28322,.T.);
#41672=ORIENTED_EDGE('',*,*,#28323,.F.);
#41673=ORIENTED_EDGE('',*,*,#28326,.F.);
#41674=ORIENTED_EDGE('',*,*,#28317,.T.);
#41675=ORIENTED_EDGE('',*,*,#28314,.T.);
#41676=ORIENTED_EDGE('',*,*,#28315,.F.);
#41677=ORIENTED_EDGE('',*,*,#28318,.F.);
#41678=ORIENTED_EDGE('',*,*,#28310,.T.);
#41679=ORIENTED_EDGE('',*,*,#28307,.T.);
#41680=ORIENTED_EDGE('',*,*,#28308,.F.);
#41681=ORIENTED_EDGE('',*,*,#28311,.F.);
#41682=ORIENTED_EDGE('',*,*,#28303,.T.);
#41683=ORIENTED_EDGE('',*,*,#28300,.T.);
#41684=ORIENTED_EDGE('',*,*,#28301,.F.);
#41685=ORIENTED_EDGE('',*,*,#28304,.F.);
#41686=ORIENTED_EDGE('',*,*,#28296,.T.);
#41687=ORIENTED_EDGE('',*,*,#28292,.T.);
#41688=ORIENTED_EDGE('',*,*,#28293,.T.);
#41689=ORIENTED_EDGE('',*,*,#28294,.F.);
#41690=ORIENTED_EDGE('',*,*,#28297,.F.);
#41691=ORIENTED_EDGE('',*,*,#28288,.T.);
#41692=ORIENTED_EDGE('',*,*,#28285,.T.);
#41693=ORIENTED_EDGE('',*,*,#28286,.F.);
#41694=ORIENTED_EDGE('',*,*,#28289,.F.);
#41695=ORIENTED_EDGE('',*,*,#28281,.T.);
#41696=ORIENTED_EDGE('',*,*,#28278,.T.);
#41697=ORIENTED_EDGE('',*,*,#28279,.F.);
#41698=ORIENTED_EDGE('',*,*,#28282,.F.);
#41699=ORIENTED_EDGE('',*,*,#28274,.T.);
#41700=ORIENTED_EDGE('',*,*,#28271,.T.);
#41701=ORIENTED_EDGE('',*,*,#28272,.F.);
#41702=ORIENTED_EDGE('',*,*,#28275,.F.);
#41703=ORIENTED_EDGE('',*,*,#28267,.T.);
#41704=ORIENTED_EDGE('',*,*,#28264,.T.);
#41705=ORIENTED_EDGE('',*,*,#28265,.F.);
#41706=ORIENTED_EDGE('',*,*,#28268,.F.);
#41707=ORIENTED_EDGE('',*,*,#28260,.T.);
#41708=ORIENTED_EDGE('',*,*,#28257,.T.);
#41709=ORIENTED_EDGE('',*,*,#28258,.F.);
#41710=ORIENTED_EDGE('',*,*,#28261,.F.);
#41711=ORIENTED_EDGE('',*,*,#28253,.T.);
#41712=ORIENTED_EDGE('',*,*,#28250,.T.);
#41713=ORIENTED_EDGE('',*,*,#28251,.F.);
#41714=ORIENTED_EDGE('',*,*,#28254,.F.);
#41715=ORIENTED_EDGE('',*,*,#28246,.T.);
#41716=ORIENTED_EDGE('',*,*,#28243,.T.);
#41717=ORIENTED_EDGE('',*,*,#28244,.F.);
#41718=ORIENTED_EDGE('',*,*,#28247,.F.);
#41719=ORIENTED_EDGE('',*,*,#28239,.T.);
#41720=ORIENTED_EDGE('',*,*,#28236,.T.);
#41721=ORIENTED_EDGE('',*,*,#28237,.F.);
#41722=ORIENTED_EDGE('',*,*,#28240,.F.);
#41723=ORIENTED_EDGE('',*,*,#28232,.T.);
#41724=ORIENTED_EDGE('',*,*,#28229,.T.);
#41725=ORIENTED_EDGE('',*,*,#28230,.F.);
#41726=ORIENTED_EDGE('',*,*,#28233,.F.);
#41727=ORIENTED_EDGE('',*,*,#28225,.T.);
#41728=ORIENTED_EDGE('',*,*,#28222,.T.);
#41729=ORIENTED_EDGE('',*,*,#28223,.F.);
#41730=ORIENTED_EDGE('',*,*,#28226,.F.);
#41731=ORIENTED_EDGE('',*,*,#28218,.T.);
#41732=ORIENTED_EDGE('',*,*,#28215,.T.);
#41733=ORIENTED_EDGE('',*,*,#28216,.F.);
#41734=ORIENTED_EDGE('',*,*,#28219,.F.);
#41735=ORIENTED_EDGE('',*,*,#28211,.T.);
#41736=ORIENTED_EDGE('',*,*,#28208,.T.);
#41737=ORIENTED_EDGE('',*,*,#28209,.F.);
#41738=ORIENTED_EDGE('',*,*,#28212,.F.);
#41739=ORIENTED_EDGE('',*,*,#28204,.T.);
#41740=ORIENTED_EDGE('',*,*,#28201,.T.);
#41741=ORIENTED_EDGE('',*,*,#28202,.F.);
#41742=ORIENTED_EDGE('',*,*,#28205,.F.);
#41743=ORIENTED_EDGE('',*,*,#28197,.T.);
#41744=ORIENTED_EDGE('',*,*,#28194,.T.);
#41745=ORIENTED_EDGE('',*,*,#28195,.F.);
#41746=ORIENTED_EDGE('',*,*,#28198,.F.);
#41747=ORIENTED_EDGE('',*,*,#28190,.T.);
#41748=ORIENTED_EDGE('',*,*,#28187,.T.);
#41749=ORIENTED_EDGE('',*,*,#28188,.F.);
#41750=ORIENTED_EDGE('',*,*,#28191,.F.);
#41751=ORIENTED_EDGE('',*,*,#28183,.T.);
#41752=ORIENTED_EDGE('',*,*,#28180,.T.);
#41753=ORIENTED_EDGE('',*,*,#28181,.F.);
#41754=ORIENTED_EDGE('',*,*,#28184,.F.);
#41755=ORIENTED_EDGE('',*,*,#28176,.T.);
#41756=ORIENTED_EDGE('',*,*,#28173,.T.);
#41757=ORIENTED_EDGE('',*,*,#28174,.F.);
#41758=ORIENTED_EDGE('',*,*,#28177,.F.);
#41759=ORIENTED_EDGE('',*,*,#28169,.T.);
#41760=ORIENTED_EDGE('',*,*,#28166,.T.);
#41761=ORIENTED_EDGE('',*,*,#28167,.F.);
#41762=ORIENTED_EDGE('',*,*,#28170,.F.);
#41763=ORIENTED_EDGE('',*,*,#28162,.T.);
#41764=ORIENTED_EDGE('',*,*,#28159,.T.);
#41765=ORIENTED_EDGE('',*,*,#28160,.F.);
#41766=ORIENTED_EDGE('',*,*,#28163,.F.);
#41767=ORIENTED_EDGE('',*,*,#28155,.T.);
#41768=ORIENTED_EDGE('',*,*,#28152,.T.);
#41769=ORIENTED_EDGE('',*,*,#28153,.F.);
#41770=ORIENTED_EDGE('',*,*,#28156,.F.);
#41771=ORIENTED_EDGE('',*,*,#28148,.T.);
#41772=ORIENTED_EDGE('',*,*,#28145,.T.);
#41773=ORIENTED_EDGE('',*,*,#28146,.F.);
#41774=ORIENTED_EDGE('',*,*,#28149,.F.);
#41775=ORIENTED_EDGE('',*,*,#28141,.T.);
#41776=ORIENTED_EDGE('',*,*,#28138,.T.);
#41777=ORIENTED_EDGE('',*,*,#28139,.F.);
#41778=ORIENTED_EDGE('',*,*,#28142,.F.);
#41779=ORIENTED_EDGE('',*,*,#28134,.T.);
#41780=ORIENTED_EDGE('',*,*,#28131,.T.);
#41781=ORIENTED_EDGE('',*,*,#28132,.F.);
#41782=ORIENTED_EDGE('',*,*,#28135,.F.);
#41783=ORIENTED_EDGE('',*,*,#28127,.T.);
#41784=ORIENTED_EDGE('',*,*,#28124,.T.);
#41785=ORIENTED_EDGE('',*,*,#28125,.F.);
#41786=ORIENTED_EDGE('',*,*,#28128,.F.);
#41787=ORIENTED_EDGE('',*,*,#28120,.T.);
#41788=ORIENTED_EDGE('',*,*,#28117,.T.);
#41789=ORIENTED_EDGE('',*,*,#28118,.F.);
#41790=ORIENTED_EDGE('',*,*,#28121,.F.);
#41791=ORIENTED_EDGE('',*,*,#28113,.T.);
#41792=ORIENTED_EDGE('',*,*,#28110,.T.);
#41793=ORIENTED_EDGE('',*,*,#28111,.F.);
#41794=ORIENTED_EDGE('',*,*,#28114,.F.);
#41795=ORIENTED_EDGE('',*,*,#28106,.T.);
#41796=ORIENTED_EDGE('',*,*,#28103,.T.);
#41797=ORIENTED_EDGE('',*,*,#28104,.F.);
#41798=ORIENTED_EDGE('',*,*,#28107,.F.);
#41799=ORIENTED_EDGE('',*,*,#28099,.T.);
#41800=ORIENTED_EDGE('',*,*,#28096,.T.);
#41801=ORIENTED_EDGE('',*,*,#28097,.F.);
#41802=ORIENTED_EDGE('',*,*,#28100,.F.);
#41803=ORIENTED_EDGE('',*,*,#28092,.T.);
#41804=ORIENTED_EDGE('',*,*,#28089,.T.);
#41805=ORIENTED_EDGE('',*,*,#28090,.F.);
#41806=ORIENTED_EDGE('',*,*,#28093,.F.);
#41807=ORIENTED_EDGE('',*,*,#28086,.T.);
#41808=ORIENTED_EDGE('',*,*,#28083,.T.);
#41809=ORIENTED_EDGE('',*,*,#28084,.F.);
#41810=ORIENTED_EDGE('',*,*,#28087,.F.);
#41811=ORIENTED_EDGE('',*,*,#28080,.T.);
#41812=ORIENTED_EDGE('',*,*,#28077,.T.);
#41813=ORIENTED_EDGE('',*,*,#28078,.F.);
#41814=ORIENTED_EDGE('',*,*,#28081,.F.);
#41815=ORIENTED_EDGE('',*,*,#28073,.T.);
#41816=ORIENTED_EDGE('',*,*,#28070,.T.);
#41817=ORIENTED_EDGE('',*,*,#28071,.F.);
#41818=ORIENTED_EDGE('',*,*,#28074,.F.);
#41819=ORIENTED_EDGE('',*,*,#28066,.T.);
#41820=ORIENTED_EDGE('',*,*,#28063,.T.);
#41821=ORIENTED_EDGE('',*,*,#28064,.F.);
#41822=ORIENTED_EDGE('',*,*,#28067,.F.);
#41823=ORIENTED_EDGE('',*,*,#28060,.T.);
#41824=ORIENTED_EDGE('',*,*,#28057,.T.);
#41825=ORIENTED_EDGE('',*,*,#28058,.F.);
#41826=ORIENTED_EDGE('',*,*,#28061,.F.);
#41827=ORIENTED_EDGE('',*,*,#28054,.T.);
#41828=ORIENTED_EDGE('',*,*,#28051,.T.);
#41829=ORIENTED_EDGE('',*,*,#28052,.F.);
#41830=ORIENTED_EDGE('',*,*,#28055,.F.);
#41831=ORIENTED_EDGE('',*,*,#28048,.T.);
#41832=ORIENTED_EDGE('',*,*,#28044,.T.);
#41833=ORIENTED_EDGE('',*,*,#28045,.T.);
#41834=ORIENTED_EDGE('',*,*,#28046,.F.);
#41835=ORIENTED_EDGE('',*,*,#28049,.F.);
#41836=ORIENTED_EDGE('',*,*,#28041,.T.);
#41837=ORIENTED_EDGE('',*,*,#28038,.T.);
#41838=ORIENTED_EDGE('',*,*,#28039,.F.);
#41839=ORIENTED_EDGE('',*,*,#28042,.F.);
#41840=ORIENTED_EDGE('',*,*,#28035,.T.);
#41841=ORIENTED_EDGE('',*,*,#28032,.T.);
#41842=ORIENTED_EDGE('',*,*,#28033,.F.);
#41843=ORIENTED_EDGE('',*,*,#28036,.F.);
#41844=ORIENTED_EDGE('',*,*,#28029,.T.);
#41845=ORIENTED_EDGE('',*,*,#28026,.T.);
#41846=ORIENTED_EDGE('',*,*,#28027,.F.);
#41847=ORIENTED_EDGE('',*,*,#28030,.F.);
#41848=ORIENTED_EDGE('',*,*,#28023,.T.);
#41849=ORIENTED_EDGE('',*,*,#28020,.T.);
#41850=ORIENTED_EDGE('',*,*,#28021,.F.);
#41851=ORIENTED_EDGE('',*,*,#28024,.F.);
#41852=ORIENTED_EDGE('',*,*,#28017,.T.);
#41853=ORIENTED_EDGE('',*,*,#28014,.T.);
#41854=ORIENTED_EDGE('',*,*,#28015,.F.);
#41855=ORIENTED_EDGE('',*,*,#28018,.F.);
#41856=ORIENTED_EDGE('',*,*,#28011,.T.);
#41857=ORIENTED_EDGE('',*,*,#28008,.T.);
#41858=ORIENTED_EDGE('',*,*,#28009,.F.);
#41859=ORIENTED_EDGE('',*,*,#28012,.F.);
#41860=ORIENTED_EDGE('',*,*,#28005,.T.);
#41861=ORIENTED_EDGE('',*,*,#28002,.T.);
#41862=ORIENTED_EDGE('',*,*,#28003,.F.);
#41863=ORIENTED_EDGE('',*,*,#28006,.F.);
#41864=ORIENTED_EDGE('',*,*,#27999,.T.);
#41865=ORIENTED_EDGE('',*,*,#27996,.T.);
#41866=ORIENTED_EDGE('',*,*,#27997,.F.);
#41867=ORIENTED_EDGE('',*,*,#28000,.F.);
#41868=ORIENTED_EDGE('',*,*,#27993,.T.);
#41869=ORIENTED_EDGE('',*,*,#27990,.T.);
#41870=ORIENTED_EDGE('',*,*,#27991,.F.);
#41871=ORIENTED_EDGE('',*,*,#27994,.F.);
#41872=ORIENTED_EDGE('',*,*,#27987,.T.);
#41873=ORIENTED_EDGE('',*,*,#27984,.T.);
#41874=ORIENTED_EDGE('',*,*,#27985,.F.);
#41875=ORIENTED_EDGE('',*,*,#27988,.F.);
#41876=ORIENTED_EDGE('',*,*,#27981,.T.);
#41877=ORIENTED_EDGE('',*,*,#27978,.T.);
#41878=ORIENTED_EDGE('',*,*,#27979,.F.);
#41879=ORIENTED_EDGE('',*,*,#27982,.F.);
#41880=ORIENTED_EDGE('',*,*,#27975,.T.);
#41881=ORIENTED_EDGE('',*,*,#27972,.T.);
#41882=ORIENTED_EDGE('',*,*,#27973,.F.);
#41883=ORIENTED_EDGE('',*,*,#27976,.F.);
#41884=ORIENTED_EDGE('',*,*,#27969,.T.);
#41885=ORIENTED_EDGE('',*,*,#27966,.T.);
#41886=ORIENTED_EDGE('',*,*,#27967,.F.);
#41887=ORIENTED_EDGE('',*,*,#27970,.F.);
#41888=ORIENTED_EDGE('',*,*,#27963,.T.);
#41889=ORIENTED_EDGE('',*,*,#27960,.T.);
#41890=ORIENTED_EDGE('',*,*,#27961,.F.);
#41891=ORIENTED_EDGE('',*,*,#27964,.F.);
#41892=ORIENTED_EDGE('',*,*,#27957,.T.);
#41893=ORIENTED_EDGE('',*,*,#27954,.T.);
#41894=ORIENTED_EDGE('',*,*,#27955,.F.);
#41895=ORIENTED_EDGE('',*,*,#27958,.F.);
#41896=ORIENTED_EDGE('',*,*,#27951,.T.);
#41897=ORIENTED_EDGE('',*,*,#27948,.T.);
#41898=ORIENTED_EDGE('',*,*,#27949,.F.);
#41899=ORIENTED_EDGE('',*,*,#27952,.F.);
#41900=ORIENTED_EDGE('',*,*,#27945,.T.);
#41901=ORIENTED_EDGE('',*,*,#27942,.T.);
#41902=ORIENTED_EDGE('',*,*,#27943,.F.);
#41903=ORIENTED_EDGE('',*,*,#27946,.F.);
#41904=ORIENTED_EDGE('',*,*,#27939,.T.);
#41905=ORIENTED_EDGE('',*,*,#27936,.T.);
#41906=ORIENTED_EDGE('',*,*,#27937,.F.);
#41907=ORIENTED_EDGE('',*,*,#27940,.F.);
#41908=ORIENTED_EDGE('',*,*,#27933,.T.);
#41909=ORIENTED_EDGE('',*,*,#27930,.T.);
#41910=ORIENTED_EDGE('',*,*,#27931,.F.);
#41911=ORIENTED_EDGE('',*,*,#27934,.F.);
#41912=ORIENTED_EDGE('',*,*,#27927,.T.);
#41913=ORIENTED_EDGE('',*,*,#27924,.T.);
#41914=ORIENTED_EDGE('',*,*,#27925,.F.);
#41915=ORIENTED_EDGE('',*,*,#27928,.F.);
#41916=ORIENTED_EDGE('',*,*,#27921,.T.);
#41917=ORIENTED_EDGE('',*,*,#27918,.T.);
#41918=ORIENTED_EDGE('',*,*,#27919,.F.);
#41919=ORIENTED_EDGE('',*,*,#27922,.F.);
#41920=ORIENTED_EDGE('',*,*,#27915,.T.);
#41921=ORIENTED_EDGE('',*,*,#27912,.T.);
#41922=ORIENTED_EDGE('',*,*,#27913,.F.);
#41923=ORIENTED_EDGE('',*,*,#27916,.F.);
#41924=ORIENTED_EDGE('',*,*,#27909,.T.);
#41925=ORIENTED_EDGE('',*,*,#27906,.T.);
#41926=ORIENTED_EDGE('',*,*,#27907,.F.);
#41927=ORIENTED_EDGE('',*,*,#27910,.F.);
#41928=ORIENTED_EDGE('',*,*,#27903,.T.);
#41929=ORIENTED_EDGE('',*,*,#27900,.T.);
#41930=ORIENTED_EDGE('',*,*,#27901,.F.);
#41931=ORIENTED_EDGE('',*,*,#27904,.F.);
#41932=ORIENTED_EDGE('',*,*,#27897,.T.);
#41933=ORIENTED_EDGE('',*,*,#27894,.T.);
#41934=ORIENTED_EDGE('',*,*,#27895,.F.);
#41935=ORIENTED_EDGE('',*,*,#27898,.F.);
#41936=ORIENTED_EDGE('',*,*,#27891,.T.);
#41937=ORIENTED_EDGE('',*,*,#27888,.T.);
#41938=ORIENTED_EDGE('',*,*,#27889,.F.);
#41939=ORIENTED_EDGE('',*,*,#27892,.F.);
#41940=ORIENTED_EDGE('',*,*,#27885,.T.);
#41941=ORIENTED_EDGE('',*,*,#27882,.T.);
#41942=ORIENTED_EDGE('',*,*,#27883,.F.);
#41943=ORIENTED_EDGE('',*,*,#27886,.F.);
#42039=TOROIDAL_SURFACE('',#48905,8.81821463020445,0.5);
#42040=TOROIDAL_SURFACE('',#50886,126.91606204049,0.5);
#42041=TOROIDAL_SURFACE('',#50892,11.8670707361131,0.5);
#42042=TOROIDAL_SURFACE('',#50897,11.8670707361131,0.5);
#42043=TOROIDAL_SURFACE('',#50904,16.1492953136408,0.5);
#42044=TOROIDAL_SURFACE('',#50908,129.,1.);
#42045=TOROIDAL_SURFACE('',#50912,128.41606204049,1.);
#42046=TOROIDAL_SURFACE('',#50917,129.,1.);
#43867=ADVANCED_FACE('',(#11287,#732,#733,#734,#735,#736,#737,#738,#739,
#740,#741,#742,#743,#744,#745,#746,#747,#748,#749,#750,#751,#752,#753,#754,
#755,#756,#757,#758,#759,#760,#761,#762,#763,#764,#765,#766,#767,#768,#769,
#770,#771,#772,#773,#774,#775,#776,#777,#778,#779,#780,#781,#782,#783,#784,
#785,#786,#787,#788,#789,#790,#791),#1686,.F.);
#43868=ADVANCED_FACE('',(#11288),#42039,.F.);
#43869=ADVANCED_FACE('',(#11289),#8684,.T.);
#43870=ADVANCED_FACE('',(#11290),#8685,.F.);
#43871=ADVANCED_FACE('',(#11291),#8686,.T.);
#43872=ADVANCED_FACE('',(#11292),#8687,.F.);
#43873=ADVANCED_FACE('',(#11293),#8688,.T.);
#43874=ADVANCED_FACE('',(#11294),#8689,.F.);
#43875=ADVANCED_FACE('',(#11295),#8690,.T.);
#43876=ADVANCED_FACE('',(#11296),#8691,.F.);
#43877=ADVANCED_FACE('',(#11297),#8692,.T.);
#43878=ADVANCED_FACE('',(#11298),#8693,.F.);
#43879=ADVANCED_FACE('',(#11299),#8694,.T.);
#43880=ADVANCED_FACE('',(#11300),#8695,.F.);
#43881=ADVANCED_FACE('',(#11301),#8696,.T.);
#43882=ADVANCED_FACE('',(#11302),#8697,.F.);
#43883=ADVANCED_FACE('',(#11303),#8698,.T.);
#43884=ADVANCED_FACE('',(#11304),#8699,.F.);
#43885=ADVANCED_FACE('',(#11305),#8700,.T.);
#43886=ADVANCED_FACE('',(#11306),#8701,.F.);
#43887=ADVANCED_FACE('',(#11307),#8702,.T.);
#43888=ADVANCED_FACE('',(#11308),#8703,.F.);
#43889=ADVANCED_FACE('',(#11309),#8704,.T.);
#43890=ADVANCED_FACE('',(#11310),#8705,.F.);
#43891=ADVANCED_FACE('',(#11311),#8706,.T.);
#43892=ADVANCED_FACE('',(#11312),#8707,.F.);
#43893=ADVANCED_FACE('',(#11313),#8708,.T.);
#43894=ADVANCED_FACE('',(#11314),#8709,.F.);
#43895=ADVANCED_FACE('',(#11315),#8710,.T.);
#43896=ADVANCED_FACE('',(#11316),#8711,.F.);
#43897=ADVANCED_FACE('',(#11317),#8712,.T.);
#43898=ADVANCED_FACE('',(#11318),#8713,.F.);
#43899=ADVANCED_FACE('',(#11319),#8714,.T.);
#43900=ADVANCED_FACE('',(#11320),#8715,.F.);
#43901=ADVANCED_FACE('',(#11321),#8716,.T.);
#43902=ADVANCED_FACE('',(#11322),#8717,.F.);
#43903=ADVANCED_FACE('',(#11323),#8718,.T.);
#43904=ADVANCED_FACE('',(#11324),#8719,.F.);
#43905=ADVANCED_FACE('',(#11325),#8720,.T.);
#43906=ADVANCED_FACE('',(#11326),#8721,.F.);
#43907=ADVANCED_FACE('',(#11327),#8722,.T.);
#43908=ADVANCED_FACE('',(#11328),#8723,.F.);
#43909=ADVANCED_FACE('',(#11329),#8724,.T.);
#43910=ADVANCED_FACE('',(#11330),#8725,.F.);
#43911=ADVANCED_FACE('',(#11331),#8726,.T.);
#43912=ADVANCED_FACE('',(#11332),#8727,.F.);
#43913=ADVANCED_FACE('',(#11333),#8728,.T.);
#43914=ADVANCED_FACE('',(#11334),#8729,.F.);
#43915=ADVANCED_FACE('',(#11335),#8730,.T.);
#43916=ADVANCED_FACE('',(#11336),#8731,.F.);
#43917=ADVANCED_FACE('',(#11337),#8732,.T.);
#43918=ADVANCED_FACE('',(#11338),#8733,.F.);
#43919=ADVANCED_FACE('',(#11339),#8734,.T.);
#43920=ADVANCED_FACE('',(#11340),#8735,.F.);
#43921=ADVANCED_FACE('',(#11341),#8736,.T.);
#43922=ADVANCED_FACE('',(#11342),#8737,.F.);
#43923=ADVANCED_FACE('',(#11343),#8738,.T.);
#43924=ADVANCED_FACE('',(#11344),#8739,.F.);
#43925=ADVANCED_FACE('',(#11345),#8740,.T.);
#43926=ADVANCED_FACE('',(#11346),#8741,.F.);
#43927=ADVANCED_FACE('',(#11347),#8742,.T.);
#43928=ADVANCED_FACE('',(#11348),#8743,.F.);
#43929=ADVANCED_FACE('',(#11349),#8744,.T.);
#43930=ADVANCED_FACE('',(#11350),#8745,.F.);
#43931=ADVANCED_FACE('',(#11351),#8746,.T.);
#43932=ADVANCED_FACE('',(#11352),#8747,.F.);
#43933=ADVANCED_FACE('',(#11353),#8748,.T.);
#43934=ADVANCED_FACE('',(#11354),#8749,.F.);
#43935=ADVANCED_FACE('',(#11355),#8750,.T.);
#43936=ADVANCED_FACE('',(#11356),#8751,.F.);
#43937=ADVANCED_FACE('',(#11357),#8752,.T.);
#43938=ADVANCED_FACE('',(#11358),#8753,.F.);
#43939=ADVANCED_FACE('',(#11359),#8754,.T.);
#43940=ADVANCED_FACE('',(#11360),#8755,.F.);
#43941=ADVANCED_FACE('',(#11361),#8756,.T.);
#43942=ADVANCED_FACE('',(#11362),#8757,.F.);
#43943=ADVANCED_FACE('',(#11363),#8758,.T.);
#43944=ADVANCED_FACE('',(#11364),#8759,.F.);
#43945=ADVANCED_FACE('',(#11365),#8760,.T.);
#43946=ADVANCED_FACE('',(#11366),#8761,.F.);
#43947=ADVANCED_FACE('',(#11367),#8762,.T.);
#43948=ADVANCED_FACE('',(#11368),#8763,.F.);
#43949=ADVANCED_FACE('',(#11369),#8764,.T.);
#43950=ADVANCED_FACE('',(#11370),#8765,.F.);
#43951=ADVANCED_FACE('',(#11371),#8766,.T.);
#43952=ADVANCED_FACE('',(#11372),#8767,.F.);
#43953=ADVANCED_FACE('',(#11373),#8768,.T.);
#43954=ADVANCED_FACE('',(#11374),#8769,.F.);
#43955=ADVANCED_FACE('',(#11375),#8770,.T.);
#43956=ADVANCED_FACE('',(#11376),#8771,.F.);
#43957=ADVANCED_FACE('',(#11377),#8772,.T.);
#43958=ADVANCED_FACE('',(#11378),#8773,.F.);
#43959=ADVANCED_FACE('',(#11379),#8774,.T.);
#43960=ADVANCED_FACE('',(#11380),#8775,.F.);
#43961=ADVANCED_FACE('',(#11381),#8776,.T.);
#43962=ADVANCED_FACE('',(#11382),#8777,.F.);
#43963=ADVANCED_FACE('',(#11383),#8778,.T.);
#43964=ADVANCED_FACE('',(#11384),#8779,.F.);
#43965=ADVANCED_FACE('',(#11385),#8780,.T.);
#43966=ADVANCED_FACE('',(#11386),#8781,.F.);
#43967=ADVANCED_FACE('',(#11387),#8782,.T.);
#43968=ADVANCED_FACE('',(#11388),#8783,.F.);
#43969=ADVANCED_FACE('',(#11389),#8784,.T.);
#43970=ADVANCED_FACE('',(#11390),#8785,.F.);
#43971=ADVANCED_FACE('',(#11391),#8786,.T.);
#43972=ADVANCED_FACE('',(#11392),#8787,.F.);
#43973=ADVANCED_FACE('',(#11393),#8788,.T.);
#43974=ADVANCED_FACE('',(#11394),#8789,.F.);
#43975=ADVANCED_FACE('',(#11395),#8790,.T.);
#43976=ADVANCED_FACE('',(#11396),#8791,.F.);
#43977=ADVANCED_FACE('',(#11397),#8792,.T.);
#43978=ADVANCED_FACE('',(#11398),#8793,.F.);
#43979=ADVANCED_FACE('',(#11399),#8794,.T.);
#43980=ADVANCED_FACE('',(#11400),#8795,.F.);
#43981=ADVANCED_FACE('',(#11401),#8796,.T.);
#43982=ADVANCED_FACE('',(#11402),#8797,.F.);
#43983=ADVANCED_FACE('',(#11403),#8798,.T.);
#43984=ADVANCED_FACE('',(#11404),#8799,.F.);
#43985=ADVANCED_FACE('',(#11405),#8800,.T.);
#43986=ADVANCED_FACE('',(#11406),#8801,.F.);
#43987=ADVANCED_FACE('',(#11407),#8802,.T.);
#43988=ADVANCED_FACE('',(#11408),#8803,.F.);
#43989=ADVANCED_FACE('',(#11409),#8804,.T.);
#43990=ADVANCED_FACE('',(#11410),#8805,.F.);
#43991=ADVANCED_FACE('',(#11411),#8806,.T.);
#43992=ADVANCED_FACE('',(#11412),#8807,.F.);
#43993=ADVANCED_FACE('',(#11413),#8808,.T.);
#43994=ADVANCED_FACE('',(#11414),#8809,.F.);
#43995=ADVANCED_FACE('',(#11415),#8810,.T.);
#43996=ADVANCED_FACE('',(#11416),#8811,.F.);
#43997=ADVANCED_FACE('',(#11417),#8812,.T.);
#43998=ADVANCED_FACE('',(#11418),#8813,.F.);
#43999=ADVANCED_FACE('',(#11419),#8814,.T.);
#44000=ADVANCED_FACE('',(#11420),#8815,.F.);
#44001=ADVANCED_FACE('',(#11421),#8816,.T.);
#44002=ADVANCED_FACE('',(#11422),#8817,.F.);
#44003=ADVANCED_FACE('',(#11423),#8818,.T.);
#44004=ADVANCED_FACE('',(#11424),#8819,.F.);
#44005=ADVANCED_FACE('',(#11425),#8820,.T.);
#44006=ADVANCED_FACE('',(#11426),#8821,.F.);
#44007=ADVANCED_FACE('',(#11427),#8822,.T.);
#44008=ADVANCED_FACE('',(#11428),#8823,.F.);
#44009=ADVANCED_FACE('',(#11429),#8824,.T.);
#44010=ADVANCED_FACE('',(#11430),#8825,.F.);
#44011=ADVANCED_FACE('',(#11431),#8826,.T.);
#44012=ADVANCED_FACE('',(#11432),#8827,.F.);
#44013=ADVANCED_FACE('',(#11433),#8828,.T.);
#44014=ADVANCED_FACE('',(#11434),#8829,.F.);
#44015=ADVANCED_FACE('',(#11435),#8830,.T.);
#44016=ADVANCED_FACE('',(#11436),#8831,.F.);
#44017=ADVANCED_FACE('',(#11437),#8832,.T.);
#44018=ADVANCED_FACE('',(#11438),#8833,.F.);
#44019=ADVANCED_FACE('',(#11439),#8834,.T.);
#44020=ADVANCED_FACE('',(#11440),#8835,.F.);
#44021=ADVANCED_FACE('',(#11441),#8836,.T.);
#44022=ADVANCED_FACE('',(#11442),#8837,.F.);
#44023=ADVANCED_FACE('',(#11443),#8838,.T.);
#44024=ADVANCED_FACE('',(#11444),#8839,.F.);
#44025=ADVANCED_FACE('',(#11445),#8840,.T.);
#44026=ADVANCED_FACE('',(#11446),#8841,.F.);
#44027=ADVANCED_FACE('',(#11447),#8842,.T.);
#44028=ADVANCED_FACE('',(#11448),#8843,.F.);
#44029=ADVANCED_FACE('',(#11449),#8844,.T.);
#44030=ADVANCED_FACE('',(#11450),#8845,.F.);
#44031=ADVANCED_FACE('',(#11451),#8846,.T.);
#44032=ADVANCED_FACE('',(#11452),#8847,.F.);
#44033=ADVANCED_FACE('',(#11453),#8848,.T.);
#44034=ADVANCED_FACE('',(#11454),#8849,.F.);
#44035=ADVANCED_FACE('',(#11455),#8850,.T.);
#44036=ADVANCED_FACE('',(#11456),#8851,.F.);
#44037=ADVANCED_FACE('',(#11457),#8852,.T.);
#44038=ADVANCED_FACE('',(#11458),#8853,.F.);
#44039=ADVANCED_FACE('',(#11459),#8854,.T.);
#44040=ADVANCED_FACE('',(#11460),#8855,.F.);
#44041=ADVANCED_FACE('',(#11461),#8856,.T.);
#44042=ADVANCED_FACE('',(#11462),#8857,.F.);
#44043=ADVANCED_FACE('',(#11463),#8858,.T.);
#44044=ADVANCED_FACE('',(#11464),#8859,.F.);
#44045=ADVANCED_FACE('',(#11465),#8860,.T.);
#44046=ADVANCED_FACE('',(#11466),#8861,.F.);
#44047=ADVANCED_FACE('',(#11467),#8862,.T.);
#44048=ADVANCED_FACE('',(#11468),#8863,.F.);
#44049=ADVANCED_FACE('',(#11469),#8864,.T.);
#44050=ADVANCED_FACE('',(#11470),#8865,.F.);
#44051=ADVANCED_FACE('',(#11471),#8866,.T.);
#44052=ADVANCED_FACE('',(#11472),#8867,.F.);
#44053=ADVANCED_FACE('',(#11473),#8868,.T.);
#44054=ADVANCED_FACE('',(#11474),#8869,.F.);
#44055=ADVANCED_FACE('',(#11475),#8870,.T.);
#44056=ADVANCED_FACE('',(#11476),#8871,.F.);
#44057=ADVANCED_FACE('',(#11477),#8872,.T.);
#44058=ADVANCED_FACE('',(#11478),#8873,.F.);
#44059=ADVANCED_FACE('',(#11479),#8874,.T.);
#44060=ADVANCED_FACE('',(#11480),#8875,.F.);
#44061=ADVANCED_FACE('',(#11481),#8876,.T.);
#44062=ADVANCED_FACE('',(#11482),#8877,.F.);
#44063=ADVANCED_FACE('',(#11483),#8878,.T.);
#44064=ADVANCED_FACE('',(#11484),#8879,.F.);
#44065=ADVANCED_FACE('',(#11485),#8880,.T.);
#44066=ADVANCED_FACE('',(#11486),#8881,.F.);
#44067=ADVANCED_FACE('',(#11487),#8882,.T.);
#44068=ADVANCED_FACE('',(#11488),#8883,.F.);
#44069=ADVANCED_FACE('',(#11489),#8884,.T.);
#44070=ADVANCED_FACE('',(#11490),#8885,.F.);
#44071=ADVANCED_FACE('',(#11491),#8886,.T.);
#44072=ADVANCED_FACE('',(#11492),#8887,.F.);
#44073=ADVANCED_FACE('',(#11493),#8888,.T.);
#44074=ADVANCED_FACE('',(#11494),#8889,.F.);
#44075=ADVANCED_FACE('',(#11495),#8890,.T.);
#44076=ADVANCED_FACE('',(#11496),#8891,.F.);
#44077=ADVANCED_FACE('',(#11497),#8892,.T.);
#44078=ADVANCED_FACE('',(#11498),#8893,.F.);
#44079=ADVANCED_FACE('',(#11499),#8894,.T.);
#44080=ADVANCED_FACE('',(#11500),#8895,.F.);
#44081=ADVANCED_FACE('',(#11501),#8896,.T.);
#44082=ADVANCED_FACE('',(#11502),#8897,.F.);
#44083=ADVANCED_FACE('',(#11503),#8898,.T.);
#44084=ADVANCED_FACE('',(#11504),#8899,.F.);
#44085=ADVANCED_FACE('',(#11505),#8900,.T.);
#44086=ADVANCED_FACE('',(#11506),#8901,.F.);
#44087=ADVANCED_FACE('',(#11507),#8902,.T.);
#44088=ADVANCED_FACE('',(#11508),#8903,.F.);
#44089=ADVANCED_FACE('',(#11509),#8904,.T.);
#44090=ADVANCED_FACE('',(#11510),#8905,.F.);
#44091=ADVANCED_FACE('',(#11511),#8906,.T.);
#44092=ADVANCED_FACE('',(#11512),#8907,.F.);
#44093=ADVANCED_FACE('',(#11513),#8908,.T.);
#44094=ADVANCED_FACE('',(#11514),#8909,.F.);
#44095=ADVANCED_FACE('',(#11515),#8910,.T.);
#44096=ADVANCED_FACE('',(#11516),#8911,.F.);
#44097=ADVANCED_FACE('',(#11517),#8912,.T.);
#44098=ADVANCED_FACE('',(#11518),#8913,.F.);
#44099=ADVANCED_FACE('',(#11519),#8914,.T.);
#44100=ADVANCED_FACE('',(#11520),#8915,.F.);
#44101=ADVANCED_FACE('',(#11521),#8916,.T.);
#44102=ADVANCED_FACE('',(#11522),#8917,.F.);
#44103=ADVANCED_FACE('',(#11523),#8918,.T.);
#44104=ADVANCED_FACE('',(#11524),#8919,.F.);
#44105=ADVANCED_FACE('',(#11525),#8920,.T.);
#44106=ADVANCED_FACE('',(#11526),#8921,.F.);
#44107=ADVANCED_FACE('',(#11527),#8922,.T.);
#44108=ADVANCED_FACE('',(#11528),#8923,.F.);
#44109=ADVANCED_FACE('',(#11529),#8924,.T.);
#44110=ADVANCED_FACE('',(#11530),#8925,.F.);
#44111=ADVANCED_FACE('',(#11531),#8926,.T.);
#44112=ADVANCED_FACE('',(#11532),#8927,.F.);
#44113=ADVANCED_FACE('',(#11533),#8928,.T.);
#44114=ADVANCED_FACE('',(#11534),#8929,.F.);
#44115=ADVANCED_FACE('',(#11535),#8930,.T.);
#44116=ADVANCED_FACE('',(#11536),#8931,.F.);
#44117=ADVANCED_FACE('',(#11537),#8932,.T.);
#44118=ADVANCED_FACE('',(#11538),#8933,.F.);
#44119=ADVANCED_FACE('',(#11539),#8934,.T.);
#44120=ADVANCED_FACE('',(#11540),#8935,.F.);
#44121=ADVANCED_FACE('',(#11541),#8936,.T.);
#44122=ADVANCED_FACE('',(#11542),#8937,.F.);
#44123=ADVANCED_FACE('',(#11543),#8938,.T.);
#44124=ADVANCED_FACE('',(#11544),#8939,.F.);
#44125=ADVANCED_FACE('',(#11545),#8940,.T.);
#44126=ADVANCED_FACE('',(#11546),#8941,.F.);
#44127=ADVANCED_FACE('',(#11547),#8942,.T.);
#44128=ADVANCED_FACE('',(#11548),#8943,.F.);
#44129=ADVANCED_FACE('',(#11549),#8944,.T.);
#44130=ADVANCED_FACE('',(#11550),#8945,.F.);
#44131=ADVANCED_FACE('',(#11551),#8946,.T.);
#44132=ADVANCED_FACE('',(#11552),#8947,.F.);
#44133=ADVANCED_FACE('',(#11553),#8948,.T.);
#44134=ADVANCED_FACE('',(#11554),#8949,.F.);
#44135=ADVANCED_FACE('',(#11555),#8950,.T.);
#44136=ADVANCED_FACE('',(#11556),#8951,.F.);
#44137=ADVANCED_FACE('',(#11557),#8952,.T.);
#44138=ADVANCED_FACE('',(#11558),#8953,.F.);
#44139=ADVANCED_FACE('',(#11559),#8954,.T.);
#44140=ADVANCED_FACE('',(#11560),#8955,.F.);
#44141=ADVANCED_FACE('',(#11561),#8956,.T.);
#44142=ADVANCED_FACE('',(#11562),#8957,.F.);
#44143=ADVANCED_FACE('',(#11563),#8958,.T.);
#44144=ADVANCED_FACE('',(#11564),#8959,.F.);
#44145=ADVANCED_FACE('',(#11565),#8960,.T.);
#44146=ADVANCED_FACE('',(#11566),#8961,.F.);
#44147=ADVANCED_FACE('',(#11567),#8962,.T.);
#44148=ADVANCED_FACE('',(#11568),#8963,.F.);
#44149=ADVANCED_FACE('',(#11569),#8964,.T.);
#44150=ADVANCED_FACE('',(#11570),#8965,.F.);
#44151=ADVANCED_FACE('',(#11571),#8966,.T.);
#44152=ADVANCED_FACE('',(#11572),#8967,.F.);
#44153=ADVANCED_FACE('',(#11573),#8968,.T.);
#44154=ADVANCED_FACE('',(#11574),#8969,.F.);
#44155=ADVANCED_FACE('',(#11575),#8970,.T.);
#44156=ADVANCED_FACE('',(#11576),#8971,.F.);
#44157=ADVANCED_FACE('',(#11577),#8972,.T.);
#44158=ADVANCED_FACE('',(#11578),#8973,.F.);
#44159=ADVANCED_FACE('',(#11579),#8974,.T.);
#44160=ADVANCED_FACE('',(#11580),#8975,.F.);
#44161=ADVANCED_FACE('',(#11581),#8976,.T.);
#44162=ADVANCED_FACE('',(#11582),#8977,.F.);
#44163=ADVANCED_FACE('',(#11583),#8978,.T.);
#44164=ADVANCED_FACE('',(#11584),#8979,.F.);
#44165=ADVANCED_FACE('',(#11585),#8980,.T.);
#44166=ADVANCED_FACE('',(#11586),#8981,.F.);
#44167=ADVANCED_FACE('',(#11587),#8982,.T.);
#44168=ADVANCED_FACE('',(#11588),#8983,.F.);
#44169=ADVANCED_FACE('',(#11589),#8984,.T.);
#44170=ADVANCED_FACE('',(#11590),#8985,.F.);
#44171=ADVANCED_FACE('',(#11591),#8986,.T.);
#44172=ADVANCED_FACE('',(#11592),#8987,.F.);
#44173=ADVANCED_FACE('',(#11593),#8988,.T.);
#44174=ADVANCED_FACE('',(#11594),#8989,.F.);
#44175=ADVANCED_FACE('',(#11595),#8990,.T.);
#44176=ADVANCED_FACE('',(#11596),#8991,.F.);
#44177=ADVANCED_FACE('',(#11597),#8992,.T.);
#44178=ADVANCED_FACE('',(#11598),#8993,.F.);
#44179=ADVANCED_FACE('',(#11599),#8994,.T.);
#44180=ADVANCED_FACE('',(#11600),#8995,.F.);
#44181=ADVANCED_FACE('',(#11601),#8996,.T.);
#44182=ADVANCED_FACE('',(#11602),#8997,.F.);
#44183=ADVANCED_FACE('',(#11603),#8998,.T.);
#44184=ADVANCED_FACE('',(#11604),#8999,.F.);
#44185=ADVANCED_FACE('',(#11605),#9000,.T.);
#44186=ADVANCED_FACE('',(#11606),#9001,.F.);
#44187=ADVANCED_FACE('',(#11607),#9002,.T.);
#44188=ADVANCED_FACE('',(#11608),#9003,.F.);
#44189=ADVANCED_FACE('',(#11609),#9004,.T.);
#44190=ADVANCED_FACE('',(#11610),#9005,.F.);
#44191=ADVANCED_FACE('',(#11611),#9006,.T.);
#44192=ADVANCED_FACE('',(#11612),#9007,.F.);
#44193=ADVANCED_FACE('',(#11613),#9008,.T.);
#44194=ADVANCED_FACE('',(#11614),#9009,.F.);
#44195=ADVANCED_FACE('',(#11615),#9010,.T.);
#44196=ADVANCED_FACE('',(#11616),#9011,.F.);
#44197=ADVANCED_FACE('',(#11617),#9012,.T.);
#44198=ADVANCED_FACE('',(#11618),#9013,.F.);
#44199=ADVANCED_FACE('',(#11619),#9014,.T.);
#44200=ADVANCED_FACE('',(#11620),#9015,.F.);
#44201=ADVANCED_FACE('',(#11621),#9016,.T.);
#44202=ADVANCED_FACE('',(#11622),#9017,.F.);
#44203=ADVANCED_FACE('',(#11623),#9018,.T.);
#44204=ADVANCED_FACE('',(#11624),#9019,.F.);
#44205=ADVANCED_FACE('',(#11625),#9020,.T.);
#44206=ADVANCED_FACE('',(#11626),#9021,.F.);
#44207=ADVANCED_FACE('',(#11627),#9022,.T.);
#44208=ADVANCED_FACE('',(#11628),#9023,.F.);
#44209=ADVANCED_FACE('',(#11629),#9024,.T.);
#44210=ADVANCED_FACE('',(#11630),#9025,.F.);
#44211=ADVANCED_FACE('',(#11631),#9026,.T.);
#44212=ADVANCED_FACE('',(#11632),#9027,.F.);
#44213=ADVANCED_FACE('',(#11633),#9028,.T.);
#44214=ADVANCED_FACE('',(#11634),#9029,.F.);
#44215=ADVANCED_FACE('',(#11635),#9030,.T.);
#44216=ADVANCED_FACE('',(#11636),#9031,.F.);
#44217=ADVANCED_FACE('',(#11637),#9032,.T.);
#44218=ADVANCED_FACE('',(#11638),#9033,.F.);
#44219=ADVANCED_FACE('',(#11639),#9034,.T.);
#44220=ADVANCED_FACE('',(#11640),#9035,.F.);
#44221=ADVANCED_FACE('',(#11641),#9036,.T.);
#44222=ADVANCED_FACE('',(#11642),#9037,.F.);
#44223=ADVANCED_FACE('',(#11643),#9038,.T.);
#44224=ADVANCED_FACE('',(#11644),#9039,.F.);
#44225=ADVANCED_FACE('',(#11645),#9040,.T.);
#44226=ADVANCED_FACE('',(#11646),#9041,.F.);
#44227=ADVANCED_FACE('',(#11647),#9042,.T.);
#44228=ADVANCED_FACE('',(#11648),#9043,.F.);
#44229=ADVANCED_FACE('',(#11649),#9044,.T.);
#44230=ADVANCED_FACE('',(#11650),#9045,.F.);
#44231=ADVANCED_FACE('',(#11651),#9046,.T.);
#44232=ADVANCED_FACE('',(#11652),#9047,.F.);
#44233=ADVANCED_FACE('',(#11653),#9048,.T.);
#44234=ADVANCED_FACE('',(#11654),#9049,.F.);
#44235=ADVANCED_FACE('',(#11655),#9050,.T.);
#44236=ADVANCED_FACE('',(#11656),#9051,.F.);
#44237=ADVANCED_FACE('',(#11657),#9052,.T.);
#44238=ADVANCED_FACE('',(#11658),#9053,.F.);
#44239=ADVANCED_FACE('',(#11659),#9054,.T.);
#44240=ADVANCED_FACE('',(#11660),#9055,.F.);
#44241=ADVANCED_FACE('',(#11661),#9056,.T.);
#44242=ADVANCED_FACE('',(#11662),#9057,.F.);
#44243=ADVANCED_FACE('',(#11663),#9058,.T.);
#44244=ADVANCED_FACE('',(#11664),#9059,.F.);
#44245=ADVANCED_FACE('',(#11665),#9060,.T.);
#44246=ADVANCED_FACE('',(#11666),#9061,.F.);
#44247=ADVANCED_FACE('',(#11667),#9062,.T.);
#44248=ADVANCED_FACE('',(#11668),#9063,.F.);
#44249=ADVANCED_FACE('',(#11669),#9064,.T.);
#44250=ADVANCED_FACE('',(#11670),#9065,.F.);
#44251=ADVANCED_FACE('',(#11671),#9066,.T.);
#44252=ADVANCED_FACE('',(#11672),#9067,.F.);
#44253=ADVANCED_FACE('',(#11673),#9068,.T.);
#44254=ADVANCED_FACE('',(#11674),#9069,.F.);
#44255=ADVANCED_FACE('',(#11675),#9070,.T.);
#44256=ADVANCED_FACE('',(#11676),#9071,.F.);
#44257=ADVANCED_FACE('',(#11677),#9072,.T.);
#44258=ADVANCED_FACE('',(#11678),#9073,.F.);
#44259=ADVANCED_FACE('',(#11679),#9074,.T.);
#44260=ADVANCED_FACE('',(#11680),#9075,.F.);
#44261=ADVANCED_FACE('',(#11681),#9076,.T.);
#44262=ADVANCED_FACE('',(#11682),#9077,.F.);
#44263=ADVANCED_FACE('',(#11683),#9078,.T.);
#44264=ADVANCED_FACE('',(#11684),#9079,.F.);
#44265=ADVANCED_FACE('',(#11685),#9080,.T.);
#44266=ADVANCED_FACE('',(#11686),#9081,.F.);
#44267=ADVANCED_FACE('',(#11687),#9082,.T.);
#44268=ADVANCED_FACE('',(#11688),#9083,.F.);
#44269=ADVANCED_FACE('',(#11689),#9084,.T.);
#44270=ADVANCED_FACE('',(#11690),#9085,.F.);
#44271=ADVANCED_FACE('',(#11691),#9086,.T.);
#44272=ADVANCED_FACE('',(#11692),#9087,.F.);
#44273=ADVANCED_FACE('',(#11693),#9088,.T.);
#44274=ADVANCED_FACE('',(#11694),#9089,.F.);
#44275=ADVANCED_FACE('',(#11695),#9090,.T.);
#44276=ADVANCED_FACE('',(#11696),#9091,.F.);
#44277=ADVANCED_FACE('',(#11697),#9092,.T.);
#44278=ADVANCED_FACE('',(#11698),#9093,.F.);
#44279=ADVANCED_FACE('',(#11699),#9094,.T.);
#44280=ADVANCED_FACE('',(#11700),#9095,.F.);
#44281=ADVANCED_FACE('',(#11701),#9096,.T.);
#44282=ADVANCED_FACE('',(#11702),#9097,.F.);
#44283=ADVANCED_FACE('',(#11703),#9098,.T.);
#44284=ADVANCED_FACE('',(#11704),#9099,.F.);
#44285=ADVANCED_FACE('',(#11705),#9100,.T.);
#44286=ADVANCED_FACE('',(#11706),#9101,.F.);
#44287=ADVANCED_FACE('',(#11707),#9102,.T.);
#44288=ADVANCED_FACE('',(#11708),#9103,.F.);
#44289=ADVANCED_FACE('',(#11709),#9104,.T.);
#44290=ADVANCED_FACE('',(#11710),#9105,.F.);
#44291=ADVANCED_FACE('',(#11711),#9106,.T.);
#44292=ADVANCED_FACE('',(#11712),#9107,.F.);
#44293=ADVANCED_FACE('',(#11713),#9108,.T.);
#44294=ADVANCED_FACE('',(#11714),#9109,.F.);
#44295=ADVANCED_FACE('',(#11715),#9110,.T.);
#44296=ADVANCED_FACE('',(#11716),#9111,.F.);
#44297=ADVANCED_FACE('',(#11717),#9112,.T.);
#44298=ADVANCED_FACE('',(#11718),#9113,.F.);
#44299=ADVANCED_FACE('',(#11719),#9114,.T.);
#44300=ADVANCED_FACE('',(#11720),#9115,.F.);
#44301=ADVANCED_FACE('',(#11721),#9116,.T.);
#44302=ADVANCED_FACE('',(#11722),#9117,.F.);
#44303=ADVANCED_FACE('',(#11723),#9118,.T.);
#44304=ADVANCED_FACE('',(#11724),#9119,.F.);
#44305=ADVANCED_FACE('',(#11725),#9120,.T.);
#44306=ADVANCED_FACE('',(#11726),#9121,.F.);
#44307=ADVANCED_FACE('',(#11727),#9122,.T.);
#44308=ADVANCED_FACE('',(#11728),#9123,.F.);
#44309=ADVANCED_FACE('',(#11729),#9124,.T.);
#44310=ADVANCED_FACE('',(#11730),#9125,.F.);
#44311=ADVANCED_FACE('',(#11731),#9126,.T.);
#44312=ADVANCED_FACE('',(#11732),#9127,.F.);
#44313=ADVANCED_FACE('',(#11733),#9128,.T.);
#44314=ADVANCED_FACE('',(#11734),#9129,.F.);
#44315=ADVANCED_FACE('',(#11735),#9130,.T.);
#44316=ADVANCED_FACE('',(#11736),#9131,.F.);
#44317=ADVANCED_FACE('',(#11737),#9132,.T.);
#44318=ADVANCED_FACE('',(#11738),#9133,.F.);
#44319=ADVANCED_FACE('',(#11739),#9134,.T.);
#44320=ADVANCED_FACE('',(#11740),#9135,.F.);
#44321=ADVANCED_FACE('',(#11741),#9136,.T.);
#44322=ADVANCED_FACE('',(#11742),#9137,.F.);
#44323=ADVANCED_FACE('',(#11743),#9138,.T.);
#44324=ADVANCED_FACE('',(#11744),#9139,.F.);
#44325=ADVANCED_FACE('',(#11745),#9140,.T.);
#44326=ADVANCED_FACE('',(#11746),#9141,.F.);
#44327=ADVANCED_FACE('',(#11747),#9142,.T.);
#44328=ADVANCED_FACE('',(#11748),#9143,.F.);
#44329=ADVANCED_FACE('',(#11749),#9144,.T.);
#44330=ADVANCED_FACE('',(#11750),#9145,.F.);
#44331=ADVANCED_FACE('',(#11751),#9146,.T.);
#44332=ADVANCED_FACE('',(#11752),#9147,.F.);
#44333=ADVANCED_FACE('',(#11753),#9148,.T.);
#44334=ADVANCED_FACE('',(#11754),#9149,.F.);
#44335=ADVANCED_FACE('',(#11755),#9150,.T.);
#44336=ADVANCED_FACE('',(#11756),#9151,.F.);
#44337=ADVANCED_FACE('',(#11757),#9152,.T.);
#44338=ADVANCED_FACE('',(#11758),#9153,.F.);
#44339=ADVANCED_FACE('',(#11759),#9154,.T.);
#44340=ADVANCED_FACE('',(#11760),#9155,.F.);
#44341=ADVANCED_FACE('',(#11761),#9156,.T.);
#44342=ADVANCED_FACE('',(#11762),#9157,.F.);
#44343=ADVANCED_FACE('',(#11763),#9158,.T.);
#44344=ADVANCED_FACE('',(#11764),#9159,.F.);
#44345=ADVANCED_FACE('',(#11765),#9160,.T.);
#44346=ADVANCED_FACE('',(#11766),#9161,.F.);
#44347=ADVANCED_FACE('',(#11767),#9162,.T.);
#44348=ADVANCED_FACE('',(#11768),#9163,.F.);
#44349=ADVANCED_FACE('',(#11769),#9164,.T.);
#44350=ADVANCED_FACE('',(#11770),#9165,.F.);
#44351=ADVANCED_FACE('',(#11771),#9166,.T.);
#44352=ADVANCED_FACE('',(#11772),#9167,.F.);
#44353=ADVANCED_FACE('',(#11773),#9168,.T.);
#44354=ADVANCED_FACE('',(#11774),#9169,.F.);
#44355=ADVANCED_FACE('',(#11775),#9170,.T.);
#44356=ADVANCED_FACE('',(#11776),#9171,.F.);
#44357=ADVANCED_FACE('',(#11777),#9172,.T.);
#44358=ADVANCED_FACE('',(#11778),#9173,.F.);
#44359=ADVANCED_FACE('',(#11779),#9174,.T.);
#44360=ADVANCED_FACE('',(#11780),#9175,.F.);
#44361=ADVANCED_FACE('',(#11781),#9176,.T.);
#44362=ADVANCED_FACE('',(#11782),#9177,.F.);
#44363=ADVANCED_FACE('',(#11783),#9178,.T.);
#44364=ADVANCED_FACE('',(#11784),#9179,.F.);
#44365=ADVANCED_FACE('',(#11785),#9180,.T.);
#44366=ADVANCED_FACE('',(#11786),#9181,.F.);
#44367=ADVANCED_FACE('',(#11787),#9182,.T.);
#44368=ADVANCED_FACE('',(#11788),#9183,.F.);
#44369=ADVANCED_FACE('',(#11789),#9184,.T.);
#44370=ADVANCED_FACE('',(#11790),#9185,.F.);
#44371=ADVANCED_FACE('',(#11791),#9186,.T.);
#44372=ADVANCED_FACE('',(#11792),#9187,.F.);
#44373=ADVANCED_FACE('',(#11793),#9188,.T.);
#44374=ADVANCED_FACE('',(#11794),#9189,.F.);
#44375=ADVANCED_FACE('',(#11795),#9190,.T.);
#44376=ADVANCED_FACE('',(#11796),#9191,.F.);
#44377=ADVANCED_FACE('',(#11797),#9192,.T.);
#44378=ADVANCED_FACE('',(#11798),#9193,.F.);
#44379=ADVANCED_FACE('',(#11799),#9194,.T.);
#44380=ADVANCED_FACE('',(#11800),#9195,.F.);
#44381=ADVANCED_FACE('',(#11801),#9196,.T.);
#44382=ADVANCED_FACE('',(#11802),#9197,.F.);
#44383=ADVANCED_FACE('',(#11803),#9198,.T.);
#44384=ADVANCED_FACE('',(#11804),#9199,.F.);
#44385=ADVANCED_FACE('',(#11805),#9200,.T.);
#44386=ADVANCED_FACE('',(#11806),#9201,.F.);
#44387=ADVANCED_FACE('',(#11807),#9202,.T.);
#44388=ADVANCED_FACE('',(#11808),#9203,.F.);
#44389=ADVANCED_FACE('',(#11809),#9204,.T.);
#44390=ADVANCED_FACE('',(#11810),#9205,.F.);
#44391=ADVANCED_FACE('',(#11811),#9206,.T.);
#44392=ADVANCED_FACE('',(#11812),#9207,.F.);
#44393=ADVANCED_FACE('',(#11813),#9208,.T.);
#44394=ADVANCED_FACE('',(#11814),#9209,.F.);
#44395=ADVANCED_FACE('',(#11815),#9210,.T.);
#44396=ADVANCED_FACE('',(#11816),#9211,.F.);
#44397=ADVANCED_FACE('',(#11817),#9212,.T.);
#44398=ADVANCED_FACE('',(#11818),#9213,.F.);
#44399=ADVANCED_FACE('',(#11819),#9214,.T.);
#44400=ADVANCED_FACE('',(#11820),#9215,.F.);
#44401=ADVANCED_FACE('',(#11821),#9216,.T.);
#44402=ADVANCED_FACE('',(#11822),#9217,.F.);
#44403=ADVANCED_FACE('',(#11823),#9218,.T.);
#44404=ADVANCED_FACE('',(#11824),#9219,.F.);
#44405=ADVANCED_FACE('',(#11825),#9220,.T.);
#44406=ADVANCED_FACE('',(#11826),#9221,.F.);
#44407=ADVANCED_FACE('',(#11827),#9222,.T.);
#44408=ADVANCED_FACE('',(#11828),#9223,.F.);
#44409=ADVANCED_FACE('',(#11829),#9224,.T.);
#44410=ADVANCED_FACE('',(#11830),#9225,.F.);
#44411=ADVANCED_FACE('',(#11831),#9226,.T.);
#44412=ADVANCED_FACE('',(#11832),#9227,.F.);
#44413=ADVANCED_FACE('',(#11833),#9228,.T.);
#44414=ADVANCED_FACE('',(#11834),#9229,.F.);
#44415=ADVANCED_FACE('',(#11835),#9230,.T.);
#44416=ADVANCED_FACE('',(#11836),#9231,.F.);
#44417=ADVANCED_FACE('',(#11837),#9232,.T.);
#44418=ADVANCED_FACE('',(#11838),#9233,.F.);
#44419=ADVANCED_FACE('',(#11839),#9234,.T.);
#44420=ADVANCED_FACE('',(#11840),#9235,.F.);
#44421=ADVANCED_FACE('',(#11841),#9236,.T.);
#44422=ADVANCED_FACE('',(#11842),#9237,.F.);
#44423=ADVANCED_FACE('',(#11843),#9238,.T.);
#44424=ADVANCED_FACE('',(#11844),#9239,.F.);
#44425=ADVANCED_FACE('',(#11845),#9240,.T.);
#44426=ADVANCED_FACE('',(#11846),#9241,.F.);
#44427=ADVANCED_FACE('',(#11847),#9242,.T.);
#44428=ADVANCED_FACE('',(#11848),#9243,.F.);
#44429=ADVANCED_FACE('',(#11849),#9244,.T.);
#44430=ADVANCED_FACE('',(#11850),#9245,.F.);
#44431=ADVANCED_FACE('',(#11851),#9246,.T.);
#44432=ADVANCED_FACE('',(#11852),#9247,.F.);
#44433=ADVANCED_FACE('',(#11853),#9248,.T.);
#44434=ADVANCED_FACE('',(#11854),#9249,.F.);
#44435=ADVANCED_FACE('',(#11855),#9250,.T.);
#44436=ADVANCED_FACE('',(#11856),#9251,.F.);
#44437=ADVANCED_FACE('',(#11857),#9252,.T.);
#44438=ADVANCED_FACE('',(#11858),#9253,.F.);
#44439=ADVANCED_FACE('',(#11859),#9254,.T.);
#44440=ADVANCED_FACE('',(#11860),#9255,.F.);
#44441=ADVANCED_FACE('',(#11861),#9256,.T.);
#44442=ADVANCED_FACE('',(#11862),#9257,.F.);
#44443=ADVANCED_FACE('',(#11863),#9258,.T.);
#44444=ADVANCED_FACE('',(#11864),#9259,.F.);
#44445=ADVANCED_FACE('',(#11865),#9260,.T.);
#44446=ADVANCED_FACE('',(#11866),#9261,.F.);
#44447=ADVANCED_FACE('',(#11867),#9262,.T.);
#44448=ADVANCED_FACE('',(#11868),#9263,.F.);
#44449=ADVANCED_FACE('',(#11869),#9264,.T.);
#44450=ADVANCED_FACE('',(#11870),#9265,.F.);
#44451=ADVANCED_FACE('',(#11871),#9266,.T.);
#44452=ADVANCED_FACE('',(#11872),#9267,.F.);
#44453=ADVANCED_FACE('',(#11873),#9268,.T.);
#44454=ADVANCED_FACE('',(#11874),#9269,.F.);
#44455=ADVANCED_FACE('',(#11875),#9270,.T.);
#44456=ADVANCED_FACE('',(#11876),#9271,.F.);
#44457=ADVANCED_FACE('',(#11877),#9272,.T.);
#44458=ADVANCED_FACE('',(#11878),#9273,.F.);
#44459=ADVANCED_FACE('',(#11879),#9274,.T.);
#44460=ADVANCED_FACE('',(#11880),#9275,.F.);
#44461=ADVANCED_FACE('',(#11881),#9276,.T.);
#44462=ADVANCED_FACE('',(#11882),#9277,.F.);
#44463=ADVANCED_FACE('',(#11883),#9278,.T.);
#44464=ADVANCED_FACE('',(#11884),#9279,.F.);
#44465=ADVANCED_FACE('',(#11885),#9280,.T.);
#44466=ADVANCED_FACE('',(#11886),#9281,.F.);
#44467=ADVANCED_FACE('',(#11887),#9282,.T.);
#44468=ADVANCED_FACE('',(#11888),#9283,.F.);
#44469=ADVANCED_FACE('',(#11889),#9284,.T.);
#44470=ADVANCED_FACE('',(#11890),#9285,.F.);
#44471=ADVANCED_FACE('',(#11891),#9286,.T.);
#44472=ADVANCED_FACE('',(#11892),#9287,.F.);
#44473=ADVANCED_FACE('',(#11893),#9288,.T.);
#44474=ADVANCED_FACE('',(#11894),#9289,.F.);
#44475=ADVANCED_FACE('',(#11895),#9290,.T.);
#44476=ADVANCED_FACE('',(#11896),#9291,.F.);
#44477=ADVANCED_FACE('',(#11897),#9292,.T.);
#44478=ADVANCED_FACE('',(#11898),#9293,.F.);
#44479=ADVANCED_FACE('',(#11899),#9294,.T.);
#44480=ADVANCED_FACE('',(#11900),#9295,.F.);
#44481=ADVANCED_FACE('',(#11901),#9296,.T.);
#44482=ADVANCED_FACE('',(#11902),#9297,.F.);
#44483=ADVANCED_FACE('',(#11903),#9298,.T.);
#44484=ADVANCED_FACE('',(#11904),#9299,.F.);
#44485=ADVANCED_FACE('',(#11905),#9300,.T.);
#44486=ADVANCED_FACE('',(#11906),#9301,.F.);
#44487=ADVANCED_FACE('',(#11907),#9302,.T.);
#44488=ADVANCED_FACE('',(#11908),#9303,.F.);
#44489=ADVANCED_FACE('',(#11909),#9304,.T.);
#44490=ADVANCED_FACE('',(#11910),#9305,.F.);
#44491=ADVANCED_FACE('',(#11911),#9306,.T.);
#44492=ADVANCED_FACE('',(#11912),#9307,.F.);
#44493=ADVANCED_FACE('',(#11913),#9308,.T.);
#44494=ADVANCED_FACE('',(#11914),#9309,.F.);
#44495=ADVANCED_FACE('',(#11915),#9310,.T.);
#44496=ADVANCED_FACE('',(#11916),#9311,.F.);
#44497=ADVANCED_FACE('',(#11917),#9312,.T.);
#44498=ADVANCED_FACE('',(#11918),#9313,.F.);
#44499=ADVANCED_FACE('',(#11919),#9314,.T.);
#44500=ADVANCED_FACE('',(#11920),#9315,.F.);
#44501=ADVANCED_FACE('',(#11921),#9316,.T.);
#44502=ADVANCED_FACE('',(#11922),#9317,.F.);
#44503=ADVANCED_FACE('',(#11923),#9318,.T.);
#44504=ADVANCED_FACE('',(#11924),#9319,.F.);
#44505=ADVANCED_FACE('',(#11925),#9320,.T.);
#44506=ADVANCED_FACE('',(#11926),#9321,.F.);
#44507=ADVANCED_FACE('',(#11927),#9322,.T.);
#44508=ADVANCED_FACE('',(#11928),#9323,.F.);
#44509=ADVANCED_FACE('',(#11929),#9324,.T.);
#44510=ADVANCED_FACE('',(#11930),#9325,.F.);
#44511=ADVANCED_FACE('',(#11931),#9326,.T.);
#44512=ADVANCED_FACE('',(#11932),#9327,.F.);
#44513=ADVANCED_FACE('',(#11933),#9328,.T.);
#44514=ADVANCED_FACE('',(#11934),#9329,.F.);
#44515=ADVANCED_FACE('',(#11935),#9330,.T.);
#44516=ADVANCED_FACE('',(#11936),#9331,.F.);
#44517=ADVANCED_FACE('',(#11937),#9332,.T.);
#44518=ADVANCED_FACE('',(#11938),#9333,.F.);
#44519=ADVANCED_FACE('',(#11939),#9334,.T.);
#44520=ADVANCED_FACE('',(#11940),#9335,.F.);
#44521=ADVANCED_FACE('',(#11941),#9336,.T.);
#44522=ADVANCED_FACE('',(#11942),#9337,.F.);
#44523=ADVANCED_FACE('',(#11943),#9338,.T.);
#44524=ADVANCED_FACE('',(#11944),#9339,.F.);
#44525=ADVANCED_FACE('',(#11945),#9340,.T.);
#44526=ADVANCED_FACE('',(#11946),#9341,.F.);
#44527=ADVANCED_FACE('',(#11947),#9342,.T.);
#44528=ADVANCED_FACE('',(#11948),#9343,.F.);
#44529=ADVANCED_FACE('',(#11949),#9344,.T.);
#44530=ADVANCED_FACE('',(#11950),#9345,.F.);
#44531=ADVANCED_FACE('',(#11951),#9346,.T.);
#44532=ADVANCED_FACE('',(#11952),#9347,.F.);
#44533=ADVANCED_FACE('',(#11953),#9348,.T.);
#44534=ADVANCED_FACE('',(#11954),#9349,.F.);
#44535=ADVANCED_FACE('',(#11955),#9350,.T.);
#44536=ADVANCED_FACE('',(#11956),#9351,.F.);
#44537=ADVANCED_FACE('',(#11957),#9352,.T.);
#44538=ADVANCED_FACE('',(#11958),#9353,.F.);
#44539=ADVANCED_FACE('',(#11959),#9354,.T.);
#44540=ADVANCED_FACE('',(#11960),#9355,.F.);
#44541=ADVANCED_FACE('',(#11961),#9356,.T.);
#44542=ADVANCED_FACE('',(#11962),#9357,.F.);
#44543=ADVANCED_FACE('',(#11963),#9358,.T.);
#44544=ADVANCED_FACE('',(#11964),#9359,.F.);
#44545=ADVANCED_FACE('',(#11965),#9360,.T.);
#44546=ADVANCED_FACE('',(#11966),#9361,.F.);
#44547=ADVANCED_FACE('',(#11967),#9362,.T.);
#44548=ADVANCED_FACE('',(#11968),#9363,.F.);
#44549=ADVANCED_FACE('',(#11969),#9364,.T.);
#44550=ADVANCED_FACE('',(#11970),#9365,.F.);
#44551=ADVANCED_FACE('',(#11971),#9366,.T.);
#44552=ADVANCED_FACE('',(#11972),#9367,.F.);
#44553=ADVANCED_FACE('',(#11973),#9368,.T.);
#44554=ADVANCED_FACE('',(#11974),#9369,.F.);
#44555=ADVANCED_FACE('',(#11975),#9370,.T.);
#44556=ADVANCED_FACE('',(#11976),#9371,.F.);
#44557=ADVANCED_FACE('',(#11977),#9372,.T.);
#44558=ADVANCED_FACE('',(#11978),#9373,.F.);
#44559=ADVANCED_FACE('',(#11979),#9374,.T.);
#44560=ADVANCED_FACE('',(#11980),#9375,.F.);
#44561=ADVANCED_FACE('',(#11981),#9376,.T.);
#44562=ADVANCED_FACE('',(#11982),#9377,.F.);
#44563=ADVANCED_FACE('',(#11983),#9378,.T.);
#44564=ADVANCED_FACE('',(#11984),#9379,.F.);
#44565=ADVANCED_FACE('',(#11985),#9380,.T.);
#44566=ADVANCED_FACE('',(#11986),#9381,.F.);
#44567=ADVANCED_FACE('',(#11987),#9382,.T.);
#44568=ADVANCED_FACE('',(#11988),#9383,.F.);
#44569=ADVANCED_FACE('',(#11989),#9384,.T.);
#44570=ADVANCED_FACE('',(#11990),#9385,.F.);
#44571=ADVANCED_FACE('',(#11991),#9386,.T.);
#44572=ADVANCED_FACE('',(#11992),#9387,.F.);
#44573=ADVANCED_FACE('',(#11993),#9388,.T.);
#44574=ADVANCED_FACE('',(#11994),#9389,.F.);
#44575=ADVANCED_FACE('',(#11995),#9390,.T.);
#44576=ADVANCED_FACE('',(#11996),#9391,.F.);
#44577=ADVANCED_FACE('',(#11997),#9392,.T.);
#44578=ADVANCED_FACE('',(#11998),#9393,.F.);
#44579=ADVANCED_FACE('',(#11999),#9394,.T.);
#44580=ADVANCED_FACE('',(#12000),#9395,.F.);
#44581=ADVANCED_FACE('',(#12001),#9396,.T.);
#44582=ADVANCED_FACE('',(#12002),#9397,.F.);
#44583=ADVANCED_FACE('',(#12003),#9398,.T.);
#44584=ADVANCED_FACE('',(#12004),#9399,.F.);
#44585=ADVANCED_FACE('',(#12005),#9400,.T.);
#44586=ADVANCED_FACE('',(#12006),#9401,.F.);
#44587=ADVANCED_FACE('',(#12007),#9402,.T.);
#44588=ADVANCED_FACE('',(#12008),#9403,.F.);
#44589=ADVANCED_FACE('',(#12009),#9404,.T.);
#44590=ADVANCED_FACE('',(#12010),#9405,.F.);
#44591=ADVANCED_FACE('',(#12011),#9406,.T.);
#44592=ADVANCED_FACE('',(#12012),#9407,.F.);
#44593=ADVANCED_FACE('',(#12013),#9408,.T.);
#44594=ADVANCED_FACE('',(#12014),#9409,.F.);
#44595=ADVANCED_FACE('',(#12015),#9410,.T.);
#44596=ADVANCED_FACE('',(#12016),#9411,.F.);
#44597=ADVANCED_FACE('',(#12017),#9412,.T.);
#44598=ADVANCED_FACE('',(#12018),#9413,.F.);
#44599=ADVANCED_FACE('',(#12019),#9414,.T.);
#44600=ADVANCED_FACE('',(#12020),#9415,.F.);
#44601=ADVANCED_FACE('',(#12021),#9416,.T.);
#44602=ADVANCED_FACE('',(#12022),#9417,.F.);
#44603=ADVANCED_FACE('',(#12023),#9418,.T.);
#44604=ADVANCED_FACE('',(#12024),#9419,.F.);
#44605=ADVANCED_FACE('',(#12025),#9420,.T.);
#44606=ADVANCED_FACE('',(#12026),#9421,.F.);
#44607=ADVANCED_FACE('',(#12027),#9422,.T.);
#44608=ADVANCED_FACE('',(#12028),#9423,.F.);
#44609=ADVANCED_FACE('',(#12029),#9424,.T.);
#44610=ADVANCED_FACE('',(#12030),#9425,.F.);
#44611=ADVANCED_FACE('',(#12031),#9426,.T.);
#44612=ADVANCED_FACE('',(#12032),#9427,.F.);
#44613=ADVANCED_FACE('',(#12033),#9428,.T.);
#44614=ADVANCED_FACE('',(#12034),#9429,.F.);
#44615=ADVANCED_FACE('',(#12035),#9430,.T.);
#44616=ADVANCED_FACE('',(#12036),#9431,.F.);
#44617=ADVANCED_FACE('',(#12037),#9432,.T.);
#44618=ADVANCED_FACE('',(#12038),#9433,.F.);
#44619=ADVANCED_FACE('',(#12039),#9434,.T.);
#44620=ADVANCED_FACE('',(#12040),#9435,.F.);
#44621=ADVANCED_FACE('',(#12041),#9436,.T.);
#44622=ADVANCED_FACE('',(#12042),#9437,.F.);
#44623=ADVANCED_FACE('',(#12043),#9438,.T.);
#44624=ADVANCED_FACE('',(#12044),#9439,.F.);
#44625=ADVANCED_FACE('',(#12045),#9440,.T.);
#44626=ADVANCED_FACE('',(#12046),#9441,.F.);
#44627=ADVANCED_FACE('',(#12047),#9442,.T.);
#44628=ADVANCED_FACE('',(#12048),#9443,.F.);
#44629=ADVANCED_FACE('',(#12049),#9444,.T.);
#44630=ADVANCED_FACE('',(#12050),#9445,.F.);
#44631=ADVANCED_FACE('',(#12051),#9446,.T.);
#44632=ADVANCED_FACE('',(#12052),#9447,.F.);
#44633=ADVANCED_FACE('',(#12053),#9448,.T.);
#44634=ADVANCED_FACE('',(#12054),#9449,.F.);
#44635=ADVANCED_FACE('',(#12055),#9450,.T.);
#44636=ADVANCED_FACE('',(#12056),#9451,.F.);
#44637=ADVANCED_FACE('',(#12057),#9452,.T.);
#44638=ADVANCED_FACE('',(#12058),#9453,.F.);
#44639=ADVANCED_FACE('',(#12059),#9454,.T.);
#44640=ADVANCED_FACE('',(#12060),#9455,.F.);
#44641=ADVANCED_FACE('',(#12061),#9456,.T.);
#44642=ADVANCED_FACE('',(#12062),#9457,.F.);
#44643=ADVANCED_FACE('',(#12063),#9458,.T.);
#44644=ADVANCED_FACE('',(#12064),#9459,.F.);
#44645=ADVANCED_FACE('',(#12065),#9460,.T.);
#44646=ADVANCED_FACE('',(#12066),#9461,.F.);
#44647=ADVANCED_FACE('',(#12067),#42040,.T.);
#44648=ADVANCED_FACE('',(#12068),#9462,.T.);
#44649=ADVANCED_FACE('',(#12069),#42041,.T.);
#44650=ADVANCED_FACE('',(#12070),#42042,.T.);
#44651=ADVANCED_FACE('',(#12071),#9463,.T.);
#44652=ADVANCED_FACE('',(#12072,#792),#70,.T.);
#44653=ADVANCED_FACE('',(#12073),#42043,.T.);
#44654=ADVANCED_FACE('',(#12074),#42044,.T.);
#44655=ADVANCED_FACE('',(#12075),#42045,.T.);
#44656=ADVANCED_FACE('',(#12076),#82,.T.);
#44657=ADVANCED_FACE('',(#12077),#42046,.T.);
#44658=ADVANCED_FACE('',(#12078),#9464,.T.);
#44659=ADVANCED_FACE('',(#12079),#9465,.F.);
#44660=ADVANCED_FACE('',(#12080),#9466,.T.);
#44661=ADVANCED_FACE('',(#12081,#793),#1687,.T.);
#44662=ADVANCED_FACE('',(#12082),#3646,.F.);
#44663=ADVANCED_FACE('',(#12083,#794),#3647,.F.);
#44664=ADVANCED_FACE('',(#12084,#795),#3648,.F.);
#44665=ADVANCED_FACE('',(#12085,#796),#3649,.F.);
#44666=ADVANCED_FACE('',(#12086),#3650,.T.);
#44667=ADVANCED_FACE('',(#12087,#797),#3651,.T.);
#44668=ADVANCED_FACE('',(#12088,#798,#799,#800,#801,#802,#803,#804,#805,
#806,#807,#808,#809,#810,#811,#812,#813,#814,#815,#816,#817,#818,#819,#820,
#821,#822,#823,#824,#825,#826,#827,#828,#829,#830,#831,#832,#833,#834,#835,
#836,#837,#838,#839,#840,#841,#842,#843,#844,#845,#846,#847,#848,#849,#850,
#851,#852,#853,#854,#855,#856,#857,#858,#859,#860,#861,#862,#863,#864,#865,
#866,#867,#868,#869,#870,#871,#872,#873,#874,#875,#876,#877,#878,#879,#880,
#881,#882,#883,#884,#885,#886,#887,#888,#889,#890,#891,#892,#893,#894,#895,
#896,#897,#898,#899,#900,#901,#902,#903,#904,#905,#906,#907,#908,#909,#910,
#911,#912,#913,#914,#915,#916,#917,#918,#919,#920,#921,#922,#923,#924,#925,
#926,#927,#928,#929,#930,#931,#932,#933,#934,#935,#936,#937,#938,#939,#940,
#941,#942,#943,#944,#945,#946,#947,#948,#949,#950,#951,#952,#953,#954,#955,
#956,#957,#958,#959,#960,#961,#962,#963,#964,#965,#966,#967,#968,#969,#970,
#971,#972,#973,#974,#975,#976,#977,#978,#979,#980,#981,#982,#983,#984,#985,
#986,#987,#988,#989,#990,#991,#992,#993,#994,#995,#996,#997,#998,#999,#1000,
#1001,#1002,#1003,#1004,#1005,#1006,#1007,#1008,#1009,#1010,#1011,#1012,
#1013,#1014,#1015,#1016,#1017,#1018,#1019,#1020,#1021,#1022,#1023,#1024,
#1025,#1026,#1027,#1028,#1029,#1030,#1031,#1032,#1033,#1034,#1035,#1036,
#1037,#1038,#1039,#1040,#1041,#1042,#1043,#1044,#1045,#1046,#1047,#1048,
#1049,#1050,#1051,#1052,#1053,#1054,#1055,#1056,#1057,#1058,#1059,#1060,
#1061,#1062,#1063,#1064,#1065,#1066,#1067),#3652,.F.);
#44669=ADVANCED_FACE('',(#12089,#1068,#1069,#1070,#1071,#1072,#1073,#1074,
#1075,#1076,#1077,#1078,#1079,#1080,#1081,#1082,#1083,#1084,#1085,#1086,
#1087,#1088,#1089,#1090,#1091,#1092,#1093,#1094,#1095,#1096,#1097,#1098,
#1099,#1100,#1101,#1102,#1103,#1104,#1105,#1106,#1107,#1108,#1109,#1110,
#1111,#1112,#1113,#1114,#1115,#1116,#1117,#1118,#1119,#1120,#1121,#1122,
#1123,#1124,#1125,#1126,#1127),#1688,.F.);
#44670=ADVANCED_FACE('',(#12090),#3653,.F.);
#44671=ADVANCED_FACE('',(#12091,#1128),#3654,.T.);
#44672=ADVANCED_FACE('',(#12092),#3655,.F.);
#44673=ADVANCED_FACE('',(#12093,#1129),#3656,.T.);
#44674=ADVANCED_FACE('',(#12094),#3657,.F.);
#44675=ADVANCED_FACE('',(#12095,#1130),#3658,.T.);
#44676=ADVANCED_FACE('',(#12096),#3659,.F.);
#44677=ADVANCED_FACE('',(#12097,#1131),#3660,.T.);
#44678=ADVANCED_FACE('',(#12098),#3661,.F.);
#44679=ADVANCED_FACE('',(#12099,#1132),#3662,.T.);
#44680=ADVANCED_FACE('',(#12100),#3663,.F.);
#44681=ADVANCED_FACE('',(#12101,#1133),#3664,.T.);
#44682=ADVANCED_FACE('',(#12102),#3665,.F.);
#44683=ADVANCED_FACE('',(#12103,#1134),#3666,.T.);
#44684=ADVANCED_FACE('',(#12104),#3667,.F.);
#44685=ADVANCED_FACE('',(#12105,#1135),#3668,.T.);
#44686=ADVANCED_FACE('',(#12106),#3669,.F.);
#44687=ADVANCED_FACE('',(#12107,#1136),#3670,.T.);
#44688=ADVANCED_FACE('',(#12108),#3671,.F.);
#44689=ADVANCED_FACE('',(#12109,#1137),#3672,.T.);
#44690=ADVANCED_FACE('',(#12110),#3673,.F.);
#44691=ADVANCED_FACE('',(#12111,#1138),#3674,.T.);
#44692=ADVANCED_FACE('',(#12112),#3675,.F.);
#44693=ADVANCED_FACE('',(#12113,#1139),#3676,.T.);
#44694=ADVANCED_FACE('',(#12114),#3677,.F.);
#44695=ADVANCED_FACE('',(#12115,#1140),#3678,.T.);
#44696=ADVANCED_FACE('',(#12116),#3679,.F.);
#44697=ADVANCED_FACE('',(#12117,#1141),#3680,.T.);
#44698=ADVANCED_FACE('',(#12118),#3681,.F.);
#44699=ADVANCED_FACE('',(#12119,#1142),#3682,.T.);
#44700=ADVANCED_FACE('',(#12120),#3683,.F.);
#44701=ADVANCED_FACE('',(#12121,#1143),#3684,.T.);
#44702=ADVANCED_FACE('',(#12122),#3685,.F.);
#44703=ADVANCED_FACE('',(#12123,#1144),#3686,.T.);
#44704=ADVANCED_FACE('',(#12124),#3687,.F.);
#44705=ADVANCED_FACE('',(#12125,#1145),#3688,.T.);
#44706=ADVANCED_FACE('',(#12126),#3689,.F.);
#44707=ADVANCED_FACE('',(#12127,#1146),#3690,.T.);
#44708=ADVANCED_FACE('',(#12128),#3691,.F.);
#44709=ADVANCED_FACE('',(#12129,#1147),#3692,.T.);
#44710=ADVANCED_FACE('',(#12130),#3693,.F.);
#44711=ADVANCED_FACE('',(#12131,#1148),#3694,.T.);
#44712=ADVANCED_FACE('',(#12132),#3695,.F.);
#44713=ADVANCED_FACE('',(#12133,#1149),#3696,.T.);
#44714=ADVANCED_FACE('',(#12134),#3697,.F.);
#44715=ADVANCED_FACE('',(#12135,#1150),#3698,.T.);
#44716=ADVANCED_FACE('',(#12136),#3699,.F.);
#44717=ADVANCED_FACE('',(#12137,#1151),#3700,.T.);
#44718=ADVANCED_FACE('',(#12138),#3701,.F.);
#44719=ADVANCED_FACE('',(#12139,#1152),#3702,.T.);
#44720=ADVANCED_FACE('',(#12140),#3703,.F.);
#44721=ADVANCED_FACE('',(#12141,#1153),#3704,.T.);
#44722=ADVANCED_FACE('',(#12142),#3705,.F.);
#44723=ADVANCED_FACE('',(#12143,#1154),#3706,.T.);
#44724=ADVANCED_FACE('',(#12144),#3707,.F.);
#44725=ADVANCED_FACE('',(#12145,#1155),#3708,.T.);
#44726=ADVANCED_FACE('',(#12146),#3709,.F.);
#44727=ADVANCED_FACE('',(#12147,#1156),#3710,.T.);
#44728=ADVANCED_FACE('',(#12148),#3711,.F.);
#44729=ADVANCED_FACE('',(#12149,#1157),#3712,.T.);
#44730=ADVANCED_FACE('',(#12150),#3713,.F.);
#44731=ADVANCED_FACE('',(#12151,#1158),#3714,.T.);
#44732=ADVANCED_FACE('',(#12152),#3715,.F.);
#44733=ADVANCED_FACE('',(#12153,#1159),#3716,.T.);
#44734=ADVANCED_FACE('',(#12154),#3717,.F.);
#44735=ADVANCED_FACE('',(#12155,#1160),#3718,.T.);
#44736=ADVANCED_FACE('',(#12156),#3719,.F.);
#44737=ADVANCED_FACE('',(#12157,#1161),#3720,.T.);
#44738=ADVANCED_FACE('',(#12158),#3721,.F.);
#44739=ADVANCED_FACE('',(#12159,#1162),#3722,.T.);
#44740=ADVANCED_FACE('',(#12160),#3723,.F.);
#44741=ADVANCED_FACE('',(#12161,#1163),#3724,.T.);
#44742=ADVANCED_FACE('',(#12162),#3725,.F.);
#44743=ADVANCED_FACE('',(#12163,#1164),#3726,.T.);
#44744=ADVANCED_FACE('',(#12164),#3727,.F.);
#44745=ADVANCED_FACE('',(#12165,#1165),#3728,.T.);
#44746=ADVANCED_FACE('',(#12166),#3729,.F.);
#44747=ADVANCED_FACE('',(#12167,#1166),#3730,.T.);
#44748=ADVANCED_FACE('',(#12168),#3731,.F.);
#44749=ADVANCED_FACE('',(#12169,#1167),#3732,.T.);
#44750=ADVANCED_FACE('',(#12170),#3733,.F.);
#44751=ADVANCED_FACE('',(#12171,#1168),#3734,.T.);
#44752=ADVANCED_FACE('',(#12172),#3735,.F.);
#44753=ADVANCED_FACE('',(#12173,#1169),#3736,.T.);
#44754=ADVANCED_FACE('',(#12174),#3737,.F.);
#44755=ADVANCED_FACE('',(#12175,#1170),#3738,.T.);
#44756=ADVANCED_FACE('',(#12176),#3739,.F.);
#44757=ADVANCED_FACE('',(#12177,#1171),#3740,.T.);
#44758=ADVANCED_FACE('',(#12178),#3741,.F.);
#44759=ADVANCED_FACE('',(#12179,#1172),#3742,.T.);
#44760=ADVANCED_FACE('',(#12180),#3743,.F.);
#44761=ADVANCED_FACE('',(#12181,#1173),#3744,.T.);
#44762=ADVANCED_FACE('',(#12182),#3745,.F.);
#44763=ADVANCED_FACE('',(#12183,#1174),#3746,.T.);
#44764=ADVANCED_FACE('',(#12184),#3747,.F.);
#44765=ADVANCED_FACE('',(#12185,#1175),#3748,.T.);
#44766=ADVANCED_FACE('',(#12186),#3749,.F.);
#44767=ADVANCED_FACE('',(#12187,#1176),#3750,.T.);
#44768=ADVANCED_FACE('',(#12188),#3751,.F.);
#44769=ADVANCED_FACE('',(#12189,#1177),#3752,.T.);
#44770=ADVANCED_FACE('',(#12190),#3753,.F.);
#44771=ADVANCED_FACE('',(#12191,#1178),#3754,.T.);
#44772=ADVANCED_FACE('',(#12192),#3755,.F.);
#44773=ADVANCED_FACE('',(#12193,#1179),#3756,.T.);
#44774=ADVANCED_FACE('',(#12194),#3757,.F.);
#44775=ADVANCED_FACE('',(#12195,#1180),#3758,.T.);
#44776=ADVANCED_FACE('',(#12196),#3759,.F.);
#44777=ADVANCED_FACE('',(#12197,#1181),#3760,.T.);
#44778=ADVANCED_FACE('',(#12198),#3761,.F.);
#44779=ADVANCED_FACE('',(#12199,#1182),#3762,.T.);
#44780=ADVANCED_FACE('',(#12200),#3763,.F.);
#44781=ADVANCED_FACE('',(#12201,#1183),#3764,.T.);
#44782=ADVANCED_FACE('',(#12202),#3765,.F.);
#44783=ADVANCED_FACE('',(#12203,#1184),#3766,.T.);
#44784=ADVANCED_FACE('',(#12204),#3767,.F.);
#44785=ADVANCED_FACE('',(#12205,#1185),#3768,.T.);
#44786=ADVANCED_FACE('',(#12206),#3769,.F.);
#44787=ADVANCED_FACE('',(#12207,#1186),#3770,.T.);
#44788=ADVANCED_FACE('',(#12208),#3771,.F.);
#44789=ADVANCED_FACE('',(#12209,#1187),#3772,.T.);
#44790=ADVANCED_FACE('',(#12210),#3773,.F.);
#44791=ADVANCED_FACE('',(#12211,#1188),#3774,.T.);
#44792=ADVANCED_FACE('',(#12212),#3775,.F.);
#44793=ADVANCED_FACE('',(#12213,#1189),#3776,.T.);
#44794=ADVANCED_FACE('',(#12214),#3777,.F.);
#44795=ADVANCED_FACE('',(#12215,#1190),#3778,.T.);
#44796=ADVANCED_FACE('',(#12216),#3779,.F.);
#44797=ADVANCED_FACE('',(#12217,#1191),#3780,.T.);
#44798=ADVANCED_FACE('',(#12218),#3781,.F.);
#44799=ADVANCED_FACE('',(#12219,#1192),#3782,.T.);
#44800=ADVANCED_FACE('',(#12220),#3783,.F.);
#44801=ADVANCED_FACE('',(#12221,#1193),#3784,.T.);
#44802=ADVANCED_FACE('',(#12222),#3785,.F.);
#44803=ADVANCED_FACE('',(#12223,#1194),#3786,.T.);
#44804=ADVANCED_FACE('',(#12224),#3787,.F.);
#44805=ADVANCED_FACE('',(#12225,#1195),#3788,.T.);
#44806=ADVANCED_FACE('',(#12226),#3789,.F.);
#44807=ADVANCED_FACE('',(#12227,#1196),#3790,.T.);
#44808=ADVANCED_FACE('',(#12228),#3791,.F.);
#44809=ADVANCED_FACE('',(#12229,#1197),#3792,.T.);
#44810=ADVANCED_FACE('',(#12230),#3793,.F.);
#44811=ADVANCED_FACE('',(#12231,#1198),#3794,.T.);
#44812=ADVANCED_FACE('',(#12232),#3795,.F.);
#44813=ADVANCED_FACE('',(#12233,#1199),#3796,.T.);
#44814=ADVANCED_FACE('',(#12234),#3797,.F.);
#44815=ADVANCED_FACE('',(#12235,#1200),#3798,.T.);
#44816=ADVANCED_FACE('',(#12236),#3799,.F.);
#44817=ADVANCED_FACE('',(#12237,#1201),#3800,.T.);
#44818=ADVANCED_FACE('',(#12238),#3801,.F.);
#44819=ADVANCED_FACE('',(#12239,#1202),#3802,.T.);
#44820=ADVANCED_FACE('',(#12240),#3803,.F.);
#44821=ADVANCED_FACE('',(#12241,#1203),#3804,.T.);
#44822=ADVANCED_FACE('',(#12242),#3805,.F.);
#44823=ADVANCED_FACE('',(#12243,#1204),#3806,.T.);
#44824=ADVANCED_FACE('',(#12244),#3807,.F.);
#44825=ADVANCED_FACE('',(#12245,#1205),#3808,.T.);
#44826=ADVANCED_FACE('',(#12246),#3809,.F.);
#44827=ADVANCED_FACE('',(#12247,#1206),#3810,.T.);
#44828=ADVANCED_FACE('',(#12248),#3811,.F.);
#44829=ADVANCED_FACE('',(#12249,#1207),#3812,.T.);
#44830=ADVANCED_FACE('',(#12250),#3813,.F.);
#44831=ADVANCED_FACE('',(#12251,#1208),#3814,.T.);
#44832=ADVANCED_FACE('',(#12252),#3815,.F.);
#44833=ADVANCED_FACE('',(#12253,#1209),#3816,.T.);
#44834=ADVANCED_FACE('',(#12254),#3817,.F.);
#44835=ADVANCED_FACE('',(#12255,#1210),#3818,.T.);
#44836=ADVANCED_FACE('',(#12256),#3819,.F.);
#44837=ADVANCED_FACE('',(#12257,#1211),#3820,.T.);
#44838=ADVANCED_FACE('',(#12258),#3821,.F.);
#44839=ADVANCED_FACE('',(#12259,#1212),#3822,.T.);
#44840=ADVANCED_FACE('',(#12260),#3823,.F.);
#44841=ADVANCED_FACE('',(#12261,#1213),#3824,.T.);
#44842=ADVANCED_FACE('',(#12262),#3825,.F.);
#44843=ADVANCED_FACE('',(#12263,#1214),#3826,.T.);
#44844=ADVANCED_FACE('',(#12264),#3827,.F.);
#44845=ADVANCED_FACE('',(#12265,#1215),#3828,.T.);
#44846=ADVANCED_FACE('',(#12266),#3829,.F.);
#44847=ADVANCED_FACE('',(#12267,#1216),#3830,.T.);
#44848=ADVANCED_FACE('',(#12268),#3831,.F.);
#44849=ADVANCED_FACE('',(#12269,#1217),#3832,.T.);
#44850=ADVANCED_FACE('',(#12270),#3833,.F.);
#44851=ADVANCED_FACE('',(#12271,#1218),#3834,.T.);
#44852=ADVANCED_FACE('',(#12272),#3835,.F.);
#44853=ADVANCED_FACE('',(#12273,#1219),#3836,.T.);
#44854=ADVANCED_FACE('',(#12274),#3837,.F.);
#44855=ADVANCED_FACE('',(#12275,#1220),#3838,.T.);
#44856=ADVANCED_FACE('',(#12276),#3839,.F.);
#44857=ADVANCED_FACE('',(#12277,#1221),#3840,.T.);
#44858=ADVANCED_FACE('',(#12278),#3841,.F.);
#44859=ADVANCED_FACE('',(#12279,#1222),#3842,.T.);
#44860=ADVANCED_FACE('',(#12280),#3843,.F.);
#44861=ADVANCED_FACE('',(#12281,#1223),#3844,.T.);
#44862=ADVANCED_FACE('',(#12282),#3845,.F.);
#44863=ADVANCED_FACE('',(#12283,#1224),#3846,.T.);
#44864=ADVANCED_FACE('',(#12284),#3847,.F.);
#44865=ADVANCED_FACE('',(#12285,#1225),#3848,.T.);
#44866=ADVANCED_FACE('',(#12286),#3849,.F.);
#44867=ADVANCED_FACE('',(#12287,#1226),#3850,.T.);
#44868=ADVANCED_FACE('',(#12288),#3851,.F.);
#44869=ADVANCED_FACE('',(#12289,#1227),#3852,.T.);
#44870=ADVANCED_FACE('',(#12290),#3853,.F.);
#44871=ADVANCED_FACE('',(#12291,#1228),#3854,.T.);
#44872=ADVANCED_FACE('',(#12292),#3855,.F.);
#44873=ADVANCED_FACE('',(#12293,#1229),#3856,.T.);
#44874=ADVANCED_FACE('',(#12294),#3857,.F.);
#44875=ADVANCED_FACE('',(#12295,#1230),#3858,.T.);
#44876=ADVANCED_FACE('',(#12296),#3859,.F.);
#44877=ADVANCED_FACE('',(#12297,#1231),#3860,.T.);
#44878=ADVANCED_FACE('',(#12298),#3861,.F.);
#44879=ADVANCED_FACE('',(#12299,#1232),#3862,.T.);
#44880=ADVANCED_FACE('',(#12300),#3863,.F.);
#44881=ADVANCED_FACE('',(#12301,#1233),#3864,.T.);
#44882=ADVANCED_FACE('',(#12302),#3865,.F.);
#44883=ADVANCED_FACE('',(#12303,#1234),#3866,.T.);
#44884=ADVANCED_FACE('',(#12304),#3867,.F.);
#44885=ADVANCED_FACE('',(#12305,#1235),#3868,.T.);
#44886=ADVANCED_FACE('',(#12306),#3869,.F.);
#44887=ADVANCED_FACE('',(#12307,#1236),#3870,.T.);
#44888=ADVANCED_FACE('',(#12308),#3871,.F.);
#44889=ADVANCED_FACE('',(#12309,#1237),#3872,.T.);
#44890=ADVANCED_FACE('',(#12310),#3873,.F.);
#44891=ADVANCED_FACE('',(#12311,#1238),#3874,.T.);
#44892=ADVANCED_FACE('',(#12312),#3875,.F.);
#44893=ADVANCED_FACE('',(#12313,#1239),#3876,.T.);
#44894=ADVANCED_FACE('',(#12314),#3877,.F.);
#44895=ADVANCED_FACE('',(#12315,#1240),#3878,.T.);
#44896=ADVANCED_FACE('',(#12316),#3879,.F.);
#44897=ADVANCED_FACE('',(#12317,#1241),#3880,.T.);
#44898=ADVANCED_FACE('',(#12318),#3881,.F.);
#44899=ADVANCED_FACE('',(#12319,#1242),#3882,.T.);
#44900=ADVANCED_FACE('',(#12320),#3883,.F.);
#44901=ADVANCED_FACE('',(#12321,#1243),#3884,.T.);
#44902=ADVANCED_FACE('',(#12322),#3885,.F.);
#44903=ADVANCED_FACE('',(#12323,#1244),#3886,.T.);
#44904=ADVANCED_FACE('',(#12324),#3887,.F.);
#44905=ADVANCED_FACE('',(#12325,#1245),#3888,.T.);
#44906=ADVANCED_FACE('',(#12326),#3889,.F.);
#44907=ADVANCED_FACE('',(#12327,#1246),#3890,.T.);
#44908=ADVANCED_FACE('',(#12328),#3891,.F.);
#44909=ADVANCED_FACE('',(#12329,#1247),#3892,.T.);
#44910=ADVANCED_FACE('',(#12330),#3893,.F.);
#44911=ADVANCED_FACE('',(#12331,#1248),#3894,.T.);
#44912=ADVANCED_FACE('',(#12332),#3895,.F.);
#44913=ADVANCED_FACE('',(#12333,#1249),#3896,.T.);
#44914=ADVANCED_FACE('',(#12334),#3897,.F.);
#44915=ADVANCED_FACE('',(#12335,#1250),#3898,.T.);
#44916=ADVANCED_FACE('',(#12336),#3899,.F.);
#44917=ADVANCED_FACE('',(#12337,#1251),#3900,.T.);
#44918=ADVANCED_FACE('',(#12338),#3901,.F.);
#44919=ADVANCED_FACE('',(#12339,#1252),#3902,.T.);
#44920=ADVANCED_FACE('',(#12340),#3903,.F.);
#44921=ADVANCED_FACE('',(#12341,#1253),#3904,.T.);
#44922=ADVANCED_FACE('',(#12342),#3905,.F.);
#44923=ADVANCED_FACE('',(#12343,#1254),#3906,.T.);
#44924=ADVANCED_FACE('',(#12344),#3907,.F.);
#44925=ADVANCED_FACE('',(#12345,#1255),#3908,.T.);
#44926=ADVANCED_FACE('',(#12346),#3909,.F.);
#44927=ADVANCED_FACE('',(#12347,#1256),#3910,.T.);
#44928=ADVANCED_FACE('',(#12348),#3911,.F.);
#44929=ADVANCED_FACE('',(#12349,#1257),#3912,.T.);
#44930=ADVANCED_FACE('',(#12350),#3913,.F.);
#44931=ADVANCED_FACE('',(#12351,#1258),#3914,.T.);
#44932=ADVANCED_FACE('',(#12352),#3915,.F.);
#44933=ADVANCED_FACE('',(#12353,#1259),#3916,.T.);
#44934=ADVANCED_FACE('',(#12354),#3917,.F.);
#44935=ADVANCED_FACE('',(#12355,#1260),#3918,.T.);
#44936=ADVANCED_FACE('',(#12356),#3919,.F.);
#44937=ADVANCED_FACE('',(#12357,#1261),#3920,.T.);
#44938=ADVANCED_FACE('',(#12358),#3921,.F.);
#44939=ADVANCED_FACE('',(#12359,#1262),#3922,.T.);
#44940=ADVANCED_FACE('',(#12360),#3923,.F.);
#44941=ADVANCED_FACE('',(#12361,#1263),#3924,.T.);
#44942=ADVANCED_FACE('',(#12362),#3925,.F.);
#44943=ADVANCED_FACE('',(#12363,#1264),#3926,.T.);
#44944=ADVANCED_FACE('',(#12364),#3927,.F.);
#44945=ADVANCED_FACE('',(#12365,#1265),#3928,.T.);
#44946=ADVANCED_FACE('',(#12366),#3929,.F.);
#44947=ADVANCED_FACE('',(#12367,#1266),#3930,.T.);
#44948=ADVANCED_FACE('',(#12368),#3931,.F.);
#44949=ADVANCED_FACE('',(#12369,#1267),#3932,.T.);
#44950=ADVANCED_FACE('',(#12370),#3933,.F.);
#44951=ADVANCED_FACE('',(#12371,#1268),#3934,.T.);
#44952=ADVANCED_FACE('',(#12372),#3935,.F.);
#44953=ADVANCED_FACE('',(#12373,#1269),#3936,.T.);
#44954=ADVANCED_FACE('',(#12374),#3937,.F.);
#44955=ADVANCED_FACE('',(#12375,#1270),#3938,.T.);
#44956=ADVANCED_FACE('',(#12376),#3939,.F.);
#44957=ADVANCED_FACE('',(#12377,#1271),#3940,.T.);
#44958=ADVANCED_FACE('',(#12378),#3941,.F.);
#44959=ADVANCED_FACE('',(#12379,#1272),#3942,.T.);
#44960=ADVANCED_FACE('',(#12380),#3943,.F.);
#44961=ADVANCED_FACE('',(#12381,#1273),#3944,.T.);
#44962=ADVANCED_FACE('',(#12382),#3945,.F.);
#44963=ADVANCED_FACE('',(#12383,#1274),#3946,.T.);
#44964=ADVANCED_FACE('',(#12384),#3947,.F.);
#44965=ADVANCED_FACE('',(#12385,#1275),#3948,.T.);
#44966=ADVANCED_FACE('',(#12386),#3949,.F.);
#44967=ADVANCED_FACE('',(#12387,#1276),#3950,.T.);
#44968=ADVANCED_FACE('',(#12388),#3951,.F.);
#44969=ADVANCED_FACE('',(#12389,#1277),#3952,.T.);
#44970=ADVANCED_FACE('',(#12390),#3953,.F.);
#44971=ADVANCED_FACE('',(#12391,#1278),#3954,.T.);
#44972=ADVANCED_FACE('',(#12392),#3955,.F.);
#44973=ADVANCED_FACE('',(#12393,#1279),#3956,.T.);
#44974=ADVANCED_FACE('',(#12394),#3957,.F.);
#44975=ADVANCED_FACE('',(#12395,#1280),#3958,.T.);
#44976=ADVANCED_FACE('',(#12396),#3959,.F.);
#44977=ADVANCED_FACE('',(#12397,#1281),#3960,.T.);
#44978=ADVANCED_FACE('',(#12398),#3961,.F.);
#44979=ADVANCED_FACE('',(#12399,#1282),#3962,.T.);
#44980=ADVANCED_FACE('',(#12400),#3963,.F.);
#44981=ADVANCED_FACE('',(#12401,#1283),#3964,.T.);
#44982=ADVANCED_FACE('',(#12402),#3965,.F.);
#44983=ADVANCED_FACE('',(#12403,#1284),#3966,.T.);
#44984=ADVANCED_FACE('',(#12404),#3967,.F.);
#44985=ADVANCED_FACE('',(#12405,#1285),#3968,.T.);
#44986=ADVANCED_FACE('',(#12406),#3969,.F.);
#44987=ADVANCED_FACE('',(#12407,#1286),#3970,.T.);
#44988=ADVANCED_FACE('',(#12408),#3971,.F.);
#44989=ADVANCED_FACE('',(#12409,#1287),#3972,.T.);
#44990=ADVANCED_FACE('',(#12410),#3973,.F.);
#44991=ADVANCED_FACE('',(#12411,#1288),#3974,.T.);
#44992=ADVANCED_FACE('',(#12412),#3975,.F.);
#44993=ADVANCED_FACE('',(#12413,#1289),#3976,.T.);
#44994=ADVANCED_FACE('',(#12414),#3977,.F.);
#44995=ADVANCED_FACE('',(#12415,#1290),#3978,.T.);
#44996=ADVANCED_FACE('',(#12416),#3979,.F.);
#44997=ADVANCED_FACE('',(#12417,#1291),#3980,.T.);
#44998=ADVANCED_FACE('',(#12418),#3981,.F.);
#44999=ADVANCED_FACE('',(#12419,#1292),#3982,.T.);
#45000=ADVANCED_FACE('',(#12420),#3983,.F.);
#45001=ADVANCED_FACE('',(#12421,#1293),#3984,.T.);
#45002=ADVANCED_FACE('',(#12422),#3985,.F.);
#45003=ADVANCED_FACE('',(#12423,#1294),#3986,.T.);
#45004=ADVANCED_FACE('',(#12424),#3987,.F.);
#45005=ADVANCED_FACE('',(#12425,#1295),#3988,.T.);
#45006=ADVANCED_FACE('',(#12426),#3989,.F.);
#45007=ADVANCED_FACE('',(#12427,#1296),#3990,.T.);
#45008=ADVANCED_FACE('',(#12428),#3991,.F.);
#45009=ADVANCED_FACE('',(#12429,#1297),#3992,.T.);
#45010=ADVANCED_FACE('',(#12430),#3993,.F.);
#45011=ADVANCED_FACE('',(#12431,#1298),#3994,.T.);
#45012=ADVANCED_FACE('',(#12432),#3995,.F.);
#45013=ADVANCED_FACE('',(#12433,#1299),#3996,.T.);
#45014=ADVANCED_FACE('',(#12434),#3997,.F.);
#45015=ADVANCED_FACE('',(#12435,#1300),#3998,.T.);
#45016=ADVANCED_FACE('',(#12436),#3999,.F.);
#45017=ADVANCED_FACE('',(#12437,#1301),#4000,.T.);
#45018=ADVANCED_FACE('',(#12438),#4001,.F.);
#45019=ADVANCED_FACE('',(#12439,#1302),#4002,.T.);
#45020=ADVANCED_FACE('',(#12440),#4003,.F.);
#45021=ADVANCED_FACE('',(#12441,#1303),#4004,.T.);
#45022=ADVANCED_FACE('',(#12442),#4005,.F.);
#45023=ADVANCED_FACE('',(#12443,#1304),#4006,.T.);
#45024=ADVANCED_FACE('',(#12444),#4007,.F.);
#45025=ADVANCED_FACE('',(#12445,#1305),#4008,.T.);
#45026=ADVANCED_FACE('',(#12446),#4009,.F.);
#45027=ADVANCED_FACE('',(#12447,#1306),#4010,.T.);
#45028=ADVANCED_FACE('',(#12448),#4011,.F.);
#45029=ADVANCED_FACE('',(#12449,#1307),#4012,.T.);
#45030=ADVANCED_FACE('',(#12450),#4013,.F.);
#45031=ADVANCED_FACE('',(#12451,#1308),#4014,.T.);
#45032=ADVANCED_FACE('',(#12452),#4015,.F.);
#45033=ADVANCED_FACE('',(#12453,#1309),#4016,.T.);
#45034=ADVANCED_FACE('',(#12454),#4017,.F.);
#45035=ADVANCED_FACE('',(#12455,#1310),#4018,.T.);
#45036=ADVANCED_FACE('',(#12456),#4019,.F.);
#45037=ADVANCED_FACE('',(#12457,#1311),#4020,.T.);
#45038=ADVANCED_FACE('',(#12458),#4021,.F.);
#45039=ADVANCED_FACE('',(#12459,#1312),#4022,.T.);
#45040=ADVANCED_FACE('',(#12460),#4023,.F.);
#45041=ADVANCED_FACE('',(#12461,#1313),#4024,.T.);
#45042=ADVANCED_FACE('',(#12462),#4025,.F.);
#45043=ADVANCED_FACE('',(#12463,#1314),#4026,.T.);
#45044=ADVANCED_FACE('',(#12464),#4027,.F.);
#45045=ADVANCED_FACE('',(#12465,#1315),#4028,.T.);
#45046=ADVANCED_FACE('',(#12466),#4029,.F.);
#45047=ADVANCED_FACE('',(#12467,#1316),#4030,.T.);
#45048=ADVANCED_FACE('',(#12468),#4031,.F.);
#45049=ADVANCED_FACE('',(#12469,#1317),#4032,.T.);
#45050=ADVANCED_FACE('',(#12470),#4033,.F.);
#45051=ADVANCED_FACE('',(#12471,#1318),#4034,.T.);
#45052=ADVANCED_FACE('',(#12472),#4035,.F.);
#45053=ADVANCED_FACE('',(#12473,#1319),#4036,.T.);
#45054=ADVANCED_FACE('',(#12474),#4037,.F.);
#45055=ADVANCED_FACE('',(#12475,#1320),#4038,.T.);
#45056=ADVANCED_FACE('',(#12476),#4039,.F.);
#45057=ADVANCED_FACE('',(#12477,#1321),#4040,.T.);
#45058=ADVANCED_FACE('',(#12478),#4041,.F.);
#45059=ADVANCED_FACE('',(#12479,#1322),#4042,.T.);
#45060=ADVANCED_FACE('',(#12480),#4043,.F.);
#45061=ADVANCED_FACE('',(#12481,#1323),#4044,.T.);
#45062=ADVANCED_FACE('',(#12482),#4045,.F.);
#45063=ADVANCED_FACE('',(#12483,#1324),#4046,.T.);
#45064=ADVANCED_FACE('',(#12484),#4047,.F.);
#45065=ADVANCED_FACE('',(#12485,#1325),#4048,.T.);
#45066=ADVANCED_FACE('',(#12486),#4049,.F.);
#45067=ADVANCED_FACE('',(#12487,#1326),#4050,.T.);
#45068=ADVANCED_FACE('',(#12488),#4051,.F.);
#45069=ADVANCED_FACE('',(#12489,#1327),#4052,.T.);
#45070=ADVANCED_FACE('',(#12490),#4053,.F.);
#45071=ADVANCED_FACE('',(#12491,#1328),#4054,.T.);
#45072=ADVANCED_FACE('',(#12492),#4055,.F.);
#45073=ADVANCED_FACE('',(#12493,#1329),#4056,.T.);
#45074=ADVANCED_FACE('',(#12494),#4057,.F.);
#45075=ADVANCED_FACE('',(#12495,#1330),#4058,.T.);
#45076=ADVANCED_FACE('',(#12496),#4059,.F.);
#45077=ADVANCED_FACE('',(#12497,#1331),#4060,.T.);
#45078=ADVANCED_FACE('',(#12498),#4061,.F.);
#45079=ADVANCED_FACE('',(#12499,#1332),#4062,.T.);
#45080=ADVANCED_FACE('',(#12500),#4063,.F.);
#45081=ADVANCED_FACE('',(#12501,#1333),#4064,.T.);
#45082=ADVANCED_FACE('',(#12502),#4065,.F.);
#45083=ADVANCED_FACE('',(#12503,#1334),#4066,.T.);
#45084=ADVANCED_FACE('',(#12504),#4067,.F.);
#45085=ADVANCED_FACE('',(#12505,#1335),#4068,.T.);
#45086=ADVANCED_FACE('',(#12506),#4069,.F.);
#45087=ADVANCED_FACE('',(#12507,#1336),#4070,.T.);
#45088=ADVANCED_FACE('',(#12508),#4071,.F.);
#45089=ADVANCED_FACE('',(#12509,#1337),#4072,.T.);
#45090=ADVANCED_FACE('',(#12510),#4073,.F.);
#45091=ADVANCED_FACE('',(#12511,#1338),#4074,.T.);
#45092=ADVANCED_FACE('',(#12512),#4075,.F.);
#45093=ADVANCED_FACE('',(#12513,#1339),#4076,.T.);
#45094=ADVANCED_FACE('',(#12514),#4077,.F.);
#45095=ADVANCED_FACE('',(#12515,#1340),#4078,.T.);
#45096=ADVANCED_FACE('',(#12516),#4079,.F.);
#45097=ADVANCED_FACE('',(#12517,#1341),#4080,.T.);
#45098=ADVANCED_FACE('',(#12518),#4081,.F.);
#45099=ADVANCED_FACE('',(#12519,#1342),#4082,.T.);
#45100=ADVANCED_FACE('',(#12520),#4083,.F.);
#45101=ADVANCED_FACE('',(#12521,#1343),#4084,.T.);
#45102=ADVANCED_FACE('',(#12522),#4085,.F.);
#45103=ADVANCED_FACE('',(#12523,#1344),#4086,.T.);
#45104=ADVANCED_FACE('',(#12524),#4087,.F.);
#45105=ADVANCED_FACE('',(#12525,#1345),#4088,.T.);
#45106=ADVANCED_FACE('',(#12526),#4089,.F.);
#45107=ADVANCED_FACE('',(#12527,#1346),#4090,.T.);
#45108=ADVANCED_FACE('',(#12528),#4091,.F.);
#45109=ADVANCED_FACE('',(#12529,#1347),#4092,.T.);
#45110=ADVANCED_FACE('',(#12530),#4093,.F.);
#45111=ADVANCED_FACE('',(#12531,#1348),#4094,.T.);
#45112=ADVANCED_FACE('',(#12532),#4095,.F.);
#45113=ADVANCED_FACE('',(#12533,#1349),#4096,.T.);
#45114=ADVANCED_FACE('',(#12534),#4097,.F.);
#45115=ADVANCED_FACE('',(#12535,#1350),#4098,.T.);
#45116=ADVANCED_FACE('',(#12536),#4099,.F.);
#45117=ADVANCED_FACE('',(#12537,#1351),#4100,.T.);
#45118=ADVANCED_FACE('',(#12538),#4101,.F.);
#45119=ADVANCED_FACE('',(#12539,#1352),#4102,.T.);
#45120=ADVANCED_FACE('',(#12540),#4103,.F.);
#45121=ADVANCED_FACE('',(#12541,#1353),#4104,.T.);
#45122=ADVANCED_FACE('',(#12542),#4105,.F.);
#45123=ADVANCED_FACE('',(#12543,#1354),#4106,.T.);
#45124=ADVANCED_FACE('',(#12544),#4107,.F.);
#45125=ADVANCED_FACE('',(#12545,#1355),#4108,.T.);
#45126=ADVANCED_FACE('',(#12546),#4109,.F.);
#45127=ADVANCED_FACE('',(#12547,#1356),#4110,.T.);
#45128=ADVANCED_FACE('',(#12548),#4111,.F.);
#45129=ADVANCED_FACE('',(#12549,#1357),#4112,.T.);
#45130=ADVANCED_FACE('',(#12550),#4113,.F.);
#45131=ADVANCED_FACE('',(#12551,#1358),#4114,.T.);
#45132=ADVANCED_FACE('',(#12552),#4115,.F.);
#45133=ADVANCED_FACE('',(#12553,#1359),#4116,.T.);
#45134=ADVANCED_FACE('',(#12554),#4117,.F.);
#45135=ADVANCED_FACE('',(#12555,#1360),#4118,.T.);
#45136=ADVANCED_FACE('',(#12556),#4119,.F.);
#45137=ADVANCED_FACE('',(#12557,#1361),#4120,.T.);
#45138=ADVANCED_FACE('',(#12558),#4121,.F.);
#45139=ADVANCED_FACE('',(#12559,#1362),#4122,.T.);
#45140=ADVANCED_FACE('',(#12560),#4123,.F.);
#45141=ADVANCED_FACE('',(#12561,#1363),#4124,.T.);
#45142=ADVANCED_FACE('',(#12562),#4125,.F.);
#45143=ADVANCED_FACE('',(#12563,#1364),#4126,.T.);
#45144=ADVANCED_FACE('',(#12564),#4127,.F.);
#45145=ADVANCED_FACE('',(#12565,#1365),#4128,.T.);
#45146=ADVANCED_FACE('',(#12566),#4129,.F.);
#45147=ADVANCED_FACE('',(#12567,#1366),#4130,.T.);
#45148=ADVANCED_FACE('',(#12568),#4131,.F.);
#45149=ADVANCED_FACE('',(#12569,#1367),#4132,.T.);
#45150=ADVANCED_FACE('',(#12570),#4133,.F.);
#45151=ADVANCED_FACE('',(#12571,#1368),#4134,.T.);
#45152=ADVANCED_FACE('',(#12572),#4135,.F.);
#45153=ADVANCED_FACE('',(#12573,#1369),#4136,.T.);
#45154=ADVANCED_FACE('',(#12574),#4137,.F.);
#45155=ADVANCED_FACE('',(#12575,#1370),#4138,.T.);
#45156=ADVANCED_FACE('',(#12576),#4139,.F.);
#45157=ADVANCED_FACE('',(#12577,#1371),#4140,.T.);
#45158=ADVANCED_FACE('',(#12578),#4141,.F.);
#45159=ADVANCED_FACE('',(#12579,#1372),#4142,.T.);
#45160=ADVANCED_FACE('',(#12580),#4143,.F.);
#45161=ADVANCED_FACE('',(#12581,#1373),#4144,.T.);
#45162=ADVANCED_FACE('',(#12582),#4145,.F.);
#45163=ADVANCED_FACE('',(#12583,#1374),#4146,.T.);
#45164=ADVANCED_FACE('',(#12584),#4147,.F.);
#45165=ADVANCED_FACE('',(#12585,#1375),#4148,.T.);
#45166=ADVANCED_FACE('',(#12586),#4149,.F.);
#45167=ADVANCED_FACE('',(#12587,#1376),#4150,.T.);
#45168=ADVANCED_FACE('',(#12588),#4151,.F.);
#45169=ADVANCED_FACE('',(#12589,#1377),#4152,.T.);
#45170=ADVANCED_FACE('',(#12590),#4153,.F.);
#45171=ADVANCED_FACE('',(#12591,#1378),#4154,.T.);
#45172=ADVANCED_FACE('',(#12592),#4155,.F.);
#45173=ADVANCED_FACE('',(#12593,#1379),#4156,.T.);
#45174=ADVANCED_FACE('',(#12594),#4157,.F.);
#45175=ADVANCED_FACE('',(#12595,#1380),#4158,.T.);
#45176=ADVANCED_FACE('',(#12596),#4159,.F.);
#45177=ADVANCED_FACE('',(#12597,#1381),#4160,.T.);
#45178=ADVANCED_FACE('',(#12598),#4161,.F.);
#45179=ADVANCED_FACE('',(#12599,#1382),#4162,.T.);
#45180=ADVANCED_FACE('',(#12600),#4163,.F.);
#45181=ADVANCED_FACE('',(#12601,#1383),#4164,.T.);
#45182=ADVANCED_FACE('',(#12602),#4165,.F.);
#45183=ADVANCED_FACE('',(#12603,#1384),#4166,.T.);
#45184=ADVANCED_FACE('',(#12604),#4167,.F.);
#45185=ADVANCED_FACE('',(#12605,#1385),#4168,.T.);
#45186=ADVANCED_FACE('',(#12606),#4169,.F.);
#45187=ADVANCED_FACE('',(#12607,#1386),#4170,.T.);
#45188=ADVANCED_FACE('',(#12608),#4171,.F.);
#45189=ADVANCED_FACE('',(#12609,#1387),#4172,.T.);
#45190=ADVANCED_FACE('',(#12610),#4173,.F.);
#45191=ADVANCED_FACE('',(#12611,#1388),#4174,.T.);
#45192=ADVANCED_FACE('',(#12612),#4175,.F.);
#45193=ADVANCED_FACE('',(#12613,#1389),#4176,.T.);
#45194=ADVANCED_FACE('',(#12614),#4177,.F.);
#45195=ADVANCED_FACE('',(#12615,#1390),#4178,.T.);
#45196=ADVANCED_FACE('',(#12616),#4179,.F.);
#45197=ADVANCED_FACE('',(#12617,#1391),#4180,.T.);
#45198=ADVANCED_FACE('',(#12618),#4181,.F.);
#45199=ADVANCED_FACE('',(#12619,#1392),#4182,.T.);
#45200=ADVANCED_FACE('',(#12620),#4183,.F.);
#45201=ADVANCED_FACE('',(#12621,#1393),#4184,.T.);
#45202=ADVANCED_FACE('',(#12622),#4185,.F.);
#45203=ADVANCED_FACE('',(#12623,#1394),#4186,.T.);
#45204=ADVANCED_FACE('',(#12624),#4187,.F.);
#45205=ADVANCED_FACE('',(#12625,#1395),#4188,.T.);
#45206=ADVANCED_FACE('',(#12626),#4189,.F.);
#45207=ADVANCED_FACE('',(#12627,#1396),#4190,.T.);
#45208=ADVANCED_FACE('',(#12628),#4191,.F.);
#45209=ADVANCED_FACE('',(#12629,#1397),#4192,.T.);
#45210=ADVANCED_FACE('',(#12630),#4193,.F.);
#45211=ADVANCED_FACE('',(#12631,#1398),#1689,.T.);
#45212=ADVANCED_FACE('',(#12632),#4194,.F.);
#45213=ADVANCED_FACE('',(#12633,#1399),#1690,.T.);
#45214=ADVANCED_FACE('',(#12634),#4195,.F.);
#45215=ADVANCED_FACE('',(#12635,#1400),#1691,.T.);
#45216=ADVANCED_FACE('',(#12636),#4196,.F.);
#45217=ADVANCED_FACE('',(#12637,#1401),#1692,.T.);
#45218=ADVANCED_FACE('',(#12638),#4197,.F.);
#45219=ADVANCED_FACE('',(#12639,#1402),#1693,.T.);
#45220=ADVANCED_FACE('',(#12640),#4198,.F.);
#45221=ADVANCED_FACE('',(#12641,#1403),#1694,.T.);
#45222=ADVANCED_FACE('',(#12642),#4199,.F.);
#45223=ADVANCED_FACE('',(#12643,#1404),#1695,.T.);
#45224=ADVANCED_FACE('',(#12644),#4200,.F.);
#45225=ADVANCED_FACE('',(#12645,#1405),#1696,.T.);
#45226=ADVANCED_FACE('',(#12646),#4201,.F.);
#45227=ADVANCED_FACE('',(#12647,#1406),#1697,.T.);
#45228=ADVANCED_FACE('',(#12648),#4202,.F.);
#45229=ADVANCED_FACE('',(#12649,#1407),#1698,.T.);
#45230=ADVANCED_FACE('',(#12650),#4203,.F.);
#45231=ADVANCED_FACE('',(#12651,#1408),#1699,.T.);
#45232=ADVANCED_FACE('',(#12652),#4204,.F.);
#45233=ADVANCED_FACE('',(#12653,#1409),#1700,.T.);
#45234=ADVANCED_FACE('',(#12654),#4205,.F.);
#45235=ADVANCED_FACE('',(#12655,#1410),#1701,.T.);
#45236=ADVANCED_FACE('',(#12656),#4206,.F.);
#45237=ADVANCED_FACE('',(#12657,#1411),#1702,.T.);
#45238=ADVANCED_FACE('',(#12658),#4207,.F.);
#45239=ADVANCED_FACE('',(#12659,#1412),#1703,.T.);
#45240=ADVANCED_FACE('',(#12660),#4208,.F.);
#45241=ADVANCED_FACE('',(#12661,#1413),#1704,.T.);
#45242=ADVANCED_FACE('',(#12662),#4209,.F.);
#45243=ADVANCED_FACE('',(#12663,#1414),#1705,.T.);
#45244=ADVANCED_FACE('',(#12664),#4210,.F.);
#45245=ADVANCED_FACE('',(#12665,#1415),#1706,.T.);
#45246=ADVANCED_FACE('',(#12666),#4211,.F.);
#45247=ADVANCED_FACE('',(#12667,#1416),#1707,.T.);
#45248=ADVANCED_FACE('',(#12668),#4212,.F.);
#45249=ADVANCED_FACE('',(#12669,#1417),#1708,.T.);
#45250=ADVANCED_FACE('',(#12670),#4213,.F.);
#45251=ADVANCED_FACE('',(#12671,#1418),#1709,.T.);
#45252=ADVANCED_FACE('',(#12672),#4214,.F.);
#45253=ADVANCED_FACE('',(#12673,#1419),#1710,.T.);
#45254=ADVANCED_FACE('',(#12674),#4215,.F.);
#45255=ADVANCED_FACE('',(#12675,#1420),#1711,.T.);
#45256=ADVANCED_FACE('',(#12676),#4216,.F.);
#45257=ADVANCED_FACE('',(#12677,#1421),#1712,.T.);
#45258=ADVANCED_FACE('',(#12678),#4217,.F.);
#45259=ADVANCED_FACE('',(#12679,#1422),#1713,.T.);
#45260=ADVANCED_FACE('',(#12680),#4218,.F.);
#45261=ADVANCED_FACE('',(#12681,#1423),#1714,.T.);
#45262=ADVANCED_FACE('',(#12682),#4219,.F.);
#45263=ADVANCED_FACE('',(#12683,#1424),#1715,.T.);
#45264=ADVANCED_FACE('',(#12684),#4220,.F.);
#45265=ADVANCED_FACE('',(#12685,#1425),#1716,.T.);
#45266=ADVANCED_FACE('',(#12686),#4221,.F.);
#45267=ADVANCED_FACE('',(#12687,#1426),#1717,.T.);
#45268=ADVANCED_FACE('',(#12688),#4222,.F.);
#45269=ADVANCED_FACE('',(#12689,#1427),#1718,.T.);
#45270=ADVANCED_FACE('',(#12690),#4223,.F.);
#45271=ADVANCED_FACE('',(#12691,#1428),#1719,.T.);
#45272=ADVANCED_FACE('',(#12692),#4224,.F.);
#45273=ADVANCED_FACE('',(#12693,#1429),#1720,.T.);
#45274=ADVANCED_FACE('',(#12694),#4225,.F.);
#45275=ADVANCED_FACE('',(#12695,#1430),#1721,.T.);
#45276=ADVANCED_FACE('',(#12696),#4226,.F.);
#45277=ADVANCED_FACE('',(#12697,#1431),#1722,.T.);
#45278=ADVANCED_FACE('',(#12698),#4227,.F.);
#45279=ADVANCED_FACE('',(#12699,#1432),#1723,.T.);
#45280=ADVANCED_FACE('',(#12700),#4228,.F.);
#45281=ADVANCED_FACE('',(#12701,#1433),#1724,.T.);
#45282=ADVANCED_FACE('',(#12702),#4229,.F.);
#45283=ADVANCED_FACE('',(#12703,#1434),#1725,.T.);
#45284=ADVANCED_FACE('',(#12704),#4230,.F.);
#45285=ADVANCED_FACE('',(#12705,#1435),#1726,.T.);
#45286=ADVANCED_FACE('',(#12706),#4231,.F.);
#45287=ADVANCED_FACE('',(#12707,#1436),#1727,.T.);
#45288=ADVANCED_FACE('',(#12708),#4232,.F.);
#45289=ADVANCED_FACE('',(#12709,#1437),#1728,.T.);
#45290=ADVANCED_FACE('',(#12710),#4233,.F.);
#45291=ADVANCED_FACE('',(#12711,#1438),#1729,.T.);
#45292=ADVANCED_FACE('',(#12712),#4234,.F.);
#45293=ADVANCED_FACE('',(#12713,#1439),#1730,.T.);
#45294=ADVANCED_FACE('',(#12714),#4235,.F.);
#45295=ADVANCED_FACE('',(#12715,#1440),#1731,.T.);
#45296=ADVANCED_FACE('',(#12716),#4236,.F.);
#45297=ADVANCED_FACE('',(#12717,#1441),#1732,.T.);
#45298=ADVANCED_FACE('',(#12718),#4237,.F.);
#45299=ADVANCED_FACE('',(#12719,#1442),#1733,.T.);
#45300=ADVANCED_FACE('',(#12720),#4238,.F.);
#45301=ADVANCED_FACE('',(#12721,#1443),#1734,.T.);
#45302=ADVANCED_FACE('',(#12722),#4239,.F.);
#45303=ADVANCED_FACE('',(#12723,#1444),#1735,.T.);
#45304=ADVANCED_FACE('',(#12724),#4240,.F.);
#45305=ADVANCED_FACE('',(#12725,#1445),#1736,.T.);
#45306=ADVANCED_FACE('',(#12726),#4241,.F.);
#45307=ADVANCED_FACE('',(#12727,#1446),#1737,.T.);
#45308=ADVANCED_FACE('',(#12728),#4242,.F.);
#45309=ADVANCED_FACE('',(#12729,#1447),#1738,.T.);
#45310=ADVANCED_FACE('',(#12730),#4243,.F.);
#45311=ADVANCED_FACE('',(#12731,#1448),#1739,.T.);
#45312=ADVANCED_FACE('',(#12732),#4244,.F.);
#45313=ADVANCED_FACE('',(#12733,#1449),#1740,.T.);
#45314=ADVANCED_FACE('',(#12734),#4245,.F.);
#45315=ADVANCED_FACE('',(#12735,#1450),#1741,.T.);
#45316=ADVANCED_FACE('',(#12736),#4246,.F.);
#45317=ADVANCED_FACE('',(#12737,#1451),#1742,.T.);
#45318=ADVANCED_FACE('',(#12738),#4247,.F.);
#45319=ADVANCED_FACE('',(#12739,#1452),#1743,.T.);
#45320=ADVANCED_FACE('',(#12740),#4248,.F.);
#45321=ADVANCED_FACE('',(#12741,#1453),#1744,.T.);
#45322=ADVANCED_FACE('',(#12742),#4249,.F.);
#45323=ADVANCED_FACE('',(#12743,#1454),#1745,.T.);
#45324=ADVANCED_FACE('',(#12744),#4250,.F.);
#45325=ADVANCED_FACE('',(#12745,#1455),#1746,.T.);
#45326=ADVANCED_FACE('',(#12746),#4251,.F.);
#45327=ADVANCED_FACE('',(#12747,#1456),#1747,.T.);
#45328=ADVANCED_FACE('',(#12748),#4252,.F.);
#45329=ADVANCED_FACE('',(#12749,#1457),#1748,.T.);
#45330=ADVANCED_FACE('',(#12750),#4253,.F.);
#45331=ADVANCED_FACE('',(#12751,#1458),#1749,.T.);
#45332=ADVANCED_FACE('',(#12752),#4254,.F.);
#45333=ADVANCED_FACE('',(#12753,#1459),#1750,.T.);
#45334=ADVANCED_FACE('',(#12754),#4255,.F.);
#45335=ADVANCED_FACE('',(#12755,#1460),#1751,.T.);
#45336=ADVANCED_FACE('',(#12756),#4256,.F.);
#45337=ADVANCED_FACE('',(#12757,#1461),#1752,.T.);
#45338=ADVANCED_FACE('',(#12758),#4257,.F.);
#45339=ADVANCED_FACE('',(#12759,#1462),#1753,.T.);
#45340=ADVANCED_FACE('',(#12760),#4258,.F.);
#45341=ADVANCED_FACE('',(#12761,#1463),#1754,.T.);
#45342=ADVANCED_FACE('',(#12762),#4259,.F.);
#45343=ADVANCED_FACE('',(#12763,#1464),#1755,.T.);
#45344=ADVANCED_FACE('',(#12764),#4260,.F.);
#45345=ADVANCED_FACE('',(#12765,#1465),#1756,.T.);
#45346=ADVANCED_FACE('',(#12766),#4261,.F.);
#45347=ADVANCED_FACE('',(#12767,#1466),#1757,.T.);
#45348=ADVANCED_FACE('',(#12768),#4262,.F.);
#45349=ADVANCED_FACE('',(#12769,#1467),#1758,.T.);
#45350=ADVANCED_FACE('',(#12770),#4263,.F.);
#45351=ADVANCED_FACE('',(#12771,#1468),#1759,.T.);
#45352=ADVANCED_FACE('',(#12772),#4264,.F.);
#45353=ADVANCED_FACE('',(#12773,#1469),#1760,.T.);
#45354=ADVANCED_FACE('',(#12774),#4265,.F.);
#45355=ADVANCED_FACE('',(#12775,#1470),#1761,.T.);
#45356=ADVANCED_FACE('',(#12776),#4266,.F.);
#45357=ADVANCED_FACE('',(#12777,#1471),#1762,.T.);
#45358=ADVANCED_FACE('',(#12778),#4267,.F.);
#45359=ADVANCED_FACE('',(#12779,#1472),#1763,.T.);
#45360=ADVANCED_FACE('',(#12780),#4268,.F.);
#45361=ADVANCED_FACE('',(#12781,#1473),#1764,.T.);
#45362=ADVANCED_FACE('',(#12782),#4269,.F.);
#45363=ADVANCED_FACE('',(#12783,#1474),#1765,.T.);
#45364=ADVANCED_FACE('',(#12784),#4270,.F.);
#45365=ADVANCED_FACE('',(#12785,#1475),#1766,.T.);
#45366=ADVANCED_FACE('',(#12786),#4271,.F.);
#45367=ADVANCED_FACE('',(#12787,#1476),#1767,.T.);
#45368=ADVANCED_FACE('',(#12788),#4272,.F.);
#45369=ADVANCED_FACE('',(#12789,#1477),#1768,.T.);
#45370=ADVANCED_FACE('',(#12790),#4273,.F.);
#45371=ADVANCED_FACE('',(#12791,#1478),#1769,.T.);
#45372=ADVANCED_FACE('',(#12792),#4274,.F.);
#45373=ADVANCED_FACE('',(#12793,#1479),#1770,.T.);
#45374=ADVANCED_FACE('',(#12794),#4275,.F.);
#45375=ADVANCED_FACE('',(#12795,#1480),#1771,.T.);
#45376=ADVANCED_FACE('',(#12796),#4276,.F.);
#45377=ADVANCED_FACE('',(#12797,#1481),#1772,.T.);
#45378=ADVANCED_FACE('',(#12798),#4277,.F.);
#45379=ADVANCED_FACE('',(#12799,#1482),#1773,.T.);
#45380=ADVANCED_FACE('',(#12800),#4278,.F.);
#45381=ADVANCED_FACE('',(#12801,#1483),#1774,.T.);
#45382=ADVANCED_FACE('',(#12802),#4279,.F.);
#45383=ADVANCED_FACE('',(#12803,#1484),#1775,.T.);
#45384=ADVANCED_FACE('',(#12804),#4280,.F.);
#45385=ADVANCED_FACE('',(#12805,#1485),#1776,.T.);
#45386=ADVANCED_FACE('',(#12806),#4281,.F.);
#45387=ADVANCED_FACE('',(#12807,#1486),#1777,.T.);
#45388=ADVANCED_FACE('',(#12808),#4282,.F.);
#45389=ADVANCED_FACE('',(#12809,#1487),#1778,.T.);
#45390=ADVANCED_FACE('',(#12810),#4283,.F.);
#45391=ADVANCED_FACE('',(#12811,#1488),#1779,.T.);
#45392=ADVANCED_FACE('',(#12812),#4284,.F.);
#45393=ADVANCED_FACE('',(#12813,#1489),#1780,.T.);
#45394=ADVANCED_FACE('',(#12814),#4285,.F.);
#45395=ADVANCED_FACE('',(#12815,#1490),#1781,.T.);
#45396=ADVANCED_FACE('',(#12816),#4286,.F.);
#45397=ADVANCED_FACE('',(#12817,#1491),#1782,.T.);
#45398=ADVANCED_FACE('',(#12818),#4287,.F.);
#45399=ADVANCED_FACE('',(#12819,#1492),#1783,.T.);
#45400=ADVANCED_FACE('',(#12820),#4288,.F.);
#45401=ADVANCED_FACE('',(#12821,#1493),#1784,.T.);
#45402=ADVANCED_FACE('',(#12822),#4289,.F.);
#45403=ADVANCED_FACE('',(#12823,#1494),#1785,.T.);
#45404=ADVANCED_FACE('',(#12824),#4290,.F.);
#45405=ADVANCED_FACE('',(#12825,#1495),#1786,.T.);
#45406=ADVANCED_FACE('',(#12826),#4291,.F.);
#45407=ADVANCED_FACE('',(#12827,#1496),#1787,.T.);
#45408=ADVANCED_FACE('',(#12828),#4292,.F.);
#45409=ADVANCED_FACE('',(#12829,#1497),#1788,.T.);
#45410=ADVANCED_FACE('',(#12830),#4293,.F.);
#45411=ADVANCED_FACE('',(#12831,#1498),#1789,.T.);
#45412=ADVANCED_FACE('',(#12832),#4294,.F.);
#45413=ADVANCED_FACE('',(#12833,#1499),#1790,.T.);
#45414=ADVANCED_FACE('',(#12834),#4295,.F.);
#45415=ADVANCED_FACE('',(#12835,#1500),#1791,.T.);
#45416=ADVANCED_FACE('',(#12836),#4296,.F.);
#45417=ADVANCED_FACE('',(#12837,#1501),#1792,.T.);
#45418=ADVANCED_FACE('',(#12838),#4297,.F.);
#45419=ADVANCED_FACE('',(#12839,#1502),#1793,.T.);
#45420=ADVANCED_FACE('',(#12840),#4298,.F.);
#45421=ADVANCED_FACE('',(#12841,#1503),#1794,.T.);
#45422=ADVANCED_FACE('',(#12842),#4299,.F.);
#45423=ADVANCED_FACE('',(#12843,#1504),#1795,.T.);
#45424=ADVANCED_FACE('',(#12844),#4300,.F.);
#45425=ADVANCED_FACE('',(#12845,#1505),#1796,.T.);
#45426=ADVANCED_FACE('',(#12846),#4301,.F.);
#45427=ADVANCED_FACE('',(#12847,#1506),#1797,.T.);
#45428=ADVANCED_FACE('',(#12848),#4302,.F.);
#45429=ADVANCED_FACE('',(#12849,#1507),#1798,.T.);
#45430=ADVANCED_FACE('',(#12850),#4303,.F.);
#45431=ADVANCED_FACE('',(#12851,#1508),#1799,.T.);
#45432=ADVANCED_FACE('',(#12852),#4304,.F.);
#45433=ADVANCED_FACE('',(#12853,#1509),#1800,.T.);
#45434=ADVANCED_FACE('',(#12854),#4305,.F.);
#45435=ADVANCED_FACE('',(#12855,#1510),#1801,.T.);
#45436=ADVANCED_FACE('',(#12856),#4306,.F.);
#45437=ADVANCED_FACE('',(#12857,#1511),#1802,.T.);
#45438=ADVANCED_FACE('',(#12858),#4307,.F.);
#45439=ADVANCED_FACE('',(#12859,#1512),#1803,.T.);
#45440=ADVANCED_FACE('',(#12860),#4308,.F.);
#45441=ADVANCED_FACE('',(#12861,#1513),#1804,.T.);
#45442=ADVANCED_FACE('',(#12862),#4309,.F.);
#45443=ADVANCED_FACE('',(#12863,#1514),#1805,.T.);
#45444=ADVANCED_FACE('',(#12864),#4310,.F.);
#45445=ADVANCED_FACE('',(#12865,#1515),#1806,.T.);
#45446=ADVANCED_FACE('',(#12866),#4311,.F.);
#45447=ADVANCED_FACE('',(#12867,#1516),#1807,.T.);
#45459=CLOSED_SHELL('',(#43867,#43868,#43869,#43870,#43871,#43872,#43873,
#43874,#43875,#43876,#43877,#43878,#43879,#43880,#43881,#43882,#43883,#43884,
#43885,#43886,#43887,#43888,#43889,#43890,#43891,#43892,#43893,#43894,#43895,
#43896,#43897,#43898,#43899,#43900,#43901,#43902,#43903,#43904,#43905,#43906,
#43907,#43908,#43909,#43910,#43911,#43912,#43913,#43914,#43915,#43916,#43917,
#43918,#43919,#43920,#43921,#43922,#43923,#43924,#43925,#43926,#43927,#43928,
#43929,#43930,#43931,#43932,#43933,#43934,#43935,#43936,#43937,#43938,#43939,
#43940,#43941,#43942,#43943,#43944,#43945,#43946,#43947,#43948,#43949,#43950,
#43951,#43952,#43953,#43954,#43955,#43956,#43957,#43958,#43959,#43960,#43961,
#43962,#43963,#43964,#43965,#43966,#43967,#43968,#43969,#43970,#43971,#43972,
#43973,#43974,#43975,#43976,#43977,#43978,#43979,#43980,#43981,#43982,#43983,
#43984,#43985,#43986,#43987,#43988,#43989,#43990,#43991,#43992,#43993,#43994,
#43995,#43996,#43997,#43998,#43999,#44000,#44001,#44002,#44003,#44004,#44005,
#44006,#44007,#44008,#44009,#44010,#44011,#44012,#44013,#44014,#44015,#44016,
#44017,#44018,#44019,#44020,#44021,#44022,#44023,#44024,#44025,#44026,#44027,
#44028,#44029,#44030,#44031,#44032,#44033,#44034,#44035,#44036,#44037,#44038,
#44039,#44040,#44041,#44042,#44043,#44044,#44045,#44046,#44047,#44048,#44049,
#44050,#44051,#44052,#44053,#44054,#44055,#44056,#44057,#44058,#44059,#44060,
#44061,#44062,#44063,#44064,#44065,#44066,#44067,#44068,#44069,#44070,#44071,
#44072,#44073,#44074,#44075,#44076,#44077,#44078,#44079,#44080,#44081,#44082,
#44083,#44084,#44085,#44086,#44087,#44088,#44089,#44090,#44091,#44092,#44093,
#44094,#44095,#44096,#44097,#44098,#44099,#44100,#44101,#44102,#44103,#44104,
#44105,#44106,#44107,#44108,#44109,#44110,#44111,#44112,#44113,#44114,#44115,
#44116,#44117,#44118,#44119,#44120,#44121,#44122,#44123,#44124,#44125,#44126,
#44127,#44128,#44129,#44130,#44131,#44132,#44133,#44134,#44135,#44136,#44137,
#44138,#44139,#44140,#44141,#44142,#44143,#44144,#44145,#44146,#44147,#44148,
#44149,#44150,#44151,#44152,#44153,#44154,#44155,#44156,#44157,#44158,#44159,
#44160,#44161,#44162,#44163,#44164,#44165,#44166,#44167,#44168,#44169,#44170,
#44171,#44172,#44173,#44174,#44175,#44176,#44177,#44178,#44179,#44180,#44181,
#44182,#44183,#44184,#44185,#44186,#44187,#44188,#44189,#44190,#44191,#44192,
#44193,#44194,#44195,#44196,#44197,#44198,#44199,#44200,#44201,#44202,#44203,
#44204,#44205,#44206,#44207,#44208,#44209,#44210,#44211,#44212,#44213,#44214,
#44215,#44216,#44217,#44218,#44219,#44220,#44221,#44222,#44223,#44224,#44225,
#44226,#44227,#44228,#44229,#44230,#44231,#44232,#44233,#44234,#44235,#44236,
#44237,#44238,#44239,#44240,#44241,#44242,#44243,#44244,#44245,#44246,#44247,
#44248,#44249,#44250,#44251,#44252,#44253,#44254,#44255,#44256,#44257,#44258,
#44259,#44260,#44261,#44262,#44263,#44264,#44265,#44266,#44267,#44268,#44269,
#44270,#44271,#44272,#44273,#44274,#44275,#44276,#44277,#44278,#44279,#44280,
#44281,#44282,#44283,#44284,#44285,#44286,#44287,#44288,#44289,#44290,#44291,
#44292,#44293,#44294,#44295,#44296,#44297,#44298,#44299,#44300,#44301,#44302,
#44303,#44304,#44305,#44306,#44307,#44308,#44309,#44310,#44311,#44312,#44313,
#44314,#44315,#44316,#44317,#44318,#44319,#44320,#44321,#44322,#44323,#44324,
#44325,#44326,#44327,#44328,#44329,#44330,#44331,#44332,#44333,#44334,#44335,
#44336,#44337,#44338,#44339,#44340,#44341,#44342,#44343,#44344,#44345,#44346,
#44347,#44348,#44349,#44350,#44351,#44352,#44353,#44354,#44355,#44356,#44357,
#44358,#44359,#44360,#44361,#44362,#44363,#44364,#44365,#44366,#44367,#44368,
#44369,#44370,#44371,#44372,#44373,#44374,#44375,#44376,#44377,#44378,#44379,
#44380,#44381,#44382,#44383,#44384,#44385,#44386,#44387,#44388,#44389,#44390,
#44391,#44392,#44393,#44394,#44395,#44396,#44397,#44398,#44399,#44400,#44401,
#44402,#44403,#44404,#44405,#44406,#44407,#44408,#44409,#44410,#44411,#44412,
#44413,#44414,#44415,#44416,#44417,#44418,#44419,#44420,#44421,#44422,#44423,
#44424,#44425,#44426,#44427,#44428,#44429,#44430,#44431,#44432,#44433,#44434,
#44435,#44436,#44437,#44438,#44439,#44440,#44441,#44442,#44443,#44444,#44445,
#44446,#44447,#44448,#44449,#44450,#44451,#44452,#44453,#44454,#44455,#44456,
#44457,#44458,#44459,#44460,#44461,#44462,#44463,#44464,#44465,#44466,#44467,
#44468,#44469,#44470,#44471,#44472,#44473,#44474,#44475,#44476,#44477,#44478,
#44479,#44480,#44481,#44482,#44483,#44484,#44485,#44486,#44487,#44488,#44489,
#44490,#44491,#44492,#44493,#44494,#44495,#44496,#44497,#44498,#44499,#44500,
#44501,#44502,#44503,#44504,#44505,#44506,#44507,#44508,#44509,#44510,#44511,
#44512,#44513,#44514,#44515,#44516,#44517,#44518,#44519,#44520,#44521,#44522,
#44523,#44524,#44525,#44526,#44527,#44528,#44529,#44530,#44531,#44532,#44533,
#44534,#44535,#44536,#44537,#44538,#44539,#44540,#44541,#44542,#44543,#44544,
#44545,#44546,#44547,#44548,#44549,#44550,#44551,#44552,#44553,#44554,#44555,
#44556,#44557,#44558,#44559,#44560,#44561,#44562,#44563,#44564,#44565,#44566,
#44567,#44568,#44569,#44570,#44571,#44572,#44573,#44574,#44575,#44576,#44577,
#44578,#44579,#44580,#44581,#44582,#44583,#44584,#44585,#44586,#44587,#44588,
#44589,#44590,#44591,#44592,#44593,#44594,#44595,#44596,#44597,#44598,#44599,
#44600,#44601,#44602,#44603,#44604,#44605,#44606,#44607,#44608,#44609,#44610,
#44611,#44612,#44613,#44614,#44615,#44616,#44617,#44618,#44619,#44620,#44621,
#44622,#44623,#44624,#44625,#44626,#44627,#44628,#44629,#44630,#44631,#44632,
#44633,#44634,#44635,#44636,#44637,#44638,#44639,#44640,#44641,#44642,#44643,
#44644,#44645,#44646,#44647,#44648,#44649,#44650,#44651,#44652,#44653,#44654,
#44655,#44656,#44657,#44658,#44659,#44660,#44661,#44662,#44663,#44664,#44665,
#44666,#44667,#44668,#44669,#44670,#44671,#44672,#44673,#44674,#44675,#44676,
#44677,#44678,#44679,#44680,#44681,#44682,#44683,#44684,#44685,#44686,#44687,
#44688,#44689,#44690,#44691,#44692,#44693,#44694,#44695,#44696,#44697,#44698,
#44699,#44700,#44701,#44702,#44703,#44704,#44705,#44706,#44707,#44708,#44709,
#44710,#44711,#44712,#44713,#44714,#44715,#44716,#44717,#44718,#44719,#44720,
#44721,#44722,#44723,#44724,#44725,#44726,#44727,#44728,#44729,#44730,#44731,
#44732,#44733,#44734,#44735,#44736,#44737,#44738,#44739,#44740,#44741,#44742,
#44743,#44744,#44745,#44746,#44747,#44748,#44749,#44750,#44751,#44752,#44753,
#44754,#44755,#44756,#44757,#44758,#44759,#44760,#44761,#44762,#44763,#44764,
#44765,#44766,#44767,#44768,#44769,#44770,#44771,#44772,#44773,#44774,#44775,
#44776,#44777,#44778,#44779,#44780,#44781,#44782,#44783,#44784,#44785,#44786,
#44787,#44788,#44789,#44790,#44791,#44792,#44793,#44794,#44795,#44796,#44797,
#44798,#44799,#44800,#44801,#44802,#44803,#44804,#44805,#44806,#44807,#44808,
#44809,#44810,#44811,#44812,#44813,#44814,#44815,#44816,#44817,#44818,#44819,
#44820,#44821,#44822,#44823,#44824,#44825,#44826,#44827,#44828,#44829,#44830,
#44831,#44832,#44833,#44834,#44835,#44836,#44837,#44838,#44839,#44840,#44841,
#44842,#44843,#44844,#44845,#44846,#44847,#44848,#44849,#44850,#44851,#44852,
#44853,#44854,#44855,#44856,#44857,#44858,#44859,#44860,#44861,#44862,#44863,
#44864,#44865,#44866,#44867,#44868,#44869,#44870,#44871,#44872,#44873,#44874,
#44875,#44876,#44877,#44878,#44879,#44880,#44881,#44882,#44883,#44884,#44885,
#44886,#44887,#44888,#44889,#44890,#44891,#44892,#44893,#44894,#44895,#44896,
#44897,#44898,#44899,#44900,#44901,#44902,#44903,#44904,#44905,#44906,#44907,
#44908,#44909,#44910,#44911,#44912,#44913,#44914,#44915,#44916,#44917,#44918,
#44919,#44920,#44921,#44922,#44923,#44924,#44925,#44926,#44927,#44928,#44929,
#44930,#44931,#44932,#44933,#44934,#44935,#44936,#44937,#44938,#44939,#44940,
#44941,#44942,#44943,#44944,#44945,#44946,#44947,#44948,#44949,#44950,#44951,
#44952,#44953,#44954,#44955,#44956,#44957,#44958,#44959,#44960,#44961,#44962,
#44963,#44964,#44965,#44966,#44967,#44968,#44969,#44970,#44971,#44972,#44973,
#44974,#44975,#44976,#44977,#44978,#44979,#44980,#44981,#44982,#44983,#44984,
#44985,#44986,#44987,#44988,#44989,#44990,#44991,#44992,#44993,#44994,#44995,
#44996,#44997,#44998,#44999,#45000,#45001,#45002,#45003,#45004,#45005,#45006,
#45007,#45008,#45009,#45010,#45011,#45012,#45013,#45014,#45015,#45016,#45017,
#45018,#45019,#45020,#45021,#45022,#45023,#45024,#45025,#45026,#45027,#45028,
#45029,#45030,#45031,#45032,#45033,#45034,#45035,#45036,#45037,#45038,#45039,
#45040,#45041,#45042,#45043,#45044,#45045,#45046,#45047,#45048,#45049,#45050,
#45051,#45052,#45053,#45054,#45055,#45056,#45057,#45058,#45059,#45060,#45061,
#45062,#45063,#45064,#45065,#45066,#45067,#45068,#45069,#45070,#45071,#45072,
#45073,#45074,#45075,#45076,#45077,#45078,#45079,#45080,#45081,#45082,#45083,
#45084,#45085,#45086,#45087,#45088,#45089,#45090,#45091,#45092,#45093,#45094,
#45095,#45096,#45097,#45098,#45099,#45100,#45101,#45102,#45103,#45104,#45105,
#45106,#45107,#45108,#45109,#45110,#45111,#45112,#45113,#45114,#45115,#45116,
#45117,#45118,#45119,#45120,#45121,#45122,#45123,#45124,#45125,#45126,#45127,
#45128,#45129,#45130,#45131,#45132,#45133,#45134,#45135,#45136,#45137,#45138,
#45139,#45140,#45141,#45142,#45143,#45144,#45145,#45146,#45147,#45148,#45149,
#45150,#45151,#45152,#45153,#45154,#45155,#45156,#45157,#45158,#45159,#45160,
#45161,#45162,#45163,#45164,#45165,#45166,#45167,#45168,#45169,#45170,#45171,
#45172,#45173,#45174,#45175,#45176,#45177,#45178,#45179,#45180,#45181,#45182,
#45183,#45184,#45185,#45186,#45187,#45188,#45189,#45190,#45191,#45192,#45193,
#45194,#45195,#45196,#45197,#45198,#45199,#45200,#45201,#45202,#45203,#45204,
#45205,#45206,#45207,#45208,#45209,#45210,#45211,#45212,#45213,#45214,#45215,
#45216,#45217,#45218,#45219,#45220,#45221,#45222,#45223,#45224,#45225,#45226,
#45227,#45228,#45229,#45230,#45231,#45232,#45233,#45234,#45235,#45236,#45237,
#45238,#45239,#45240,#45241,#45242,#45243,#45244,#45245,#45246,#45247,#45248,
#45249,#45250,#45251,#45252,#45253,#45254,#45255,#45256,#45257,#45258,#45259,
#45260,#45261,#45262,#45263,#45264,#45265,#45266,#45267,#45268,#45269,#45270,
#45271,#45272,#45273,#45274,#45275,#45276,#45277,#45278,#45279,#45280,#45281,
#45282,#45283,#45284,#45285,#45286,#45287,#45288,#45289,#45290,#45291,#45292,
#45293,#45294,#45295,#45296,#45297,#45298,#45299,#45300,#45301,#45302,#45303,
#45304,#45305,#45306,#45307,#45308,#45309,#45310,#45311,#45312,#45313,#45314,
#45315,#45316,#45317,#45318,#45319,#45320,#45321,#45322,#45323,#45324,#45325,
#45326,#45327,#45328,#45329,#45330,#45331,#45332,#45333,#45334,#45335,#45336,
#45337,#45338,#45339,#45340,#45341,#45342,#45343,#45344,#45345,#45346,#45347,
#45348,#45349,#45350,#45351,#45352,#45353,#45354,#45355,#45356,#45357,#45358,
#45359,#45360,#45361,#45362,#45363,#45364,#45365,#45366,#45367,#45368,#45369,
#45370,#45371,#45372,#45373,#45374,#45375,#45376,#45377,#45378,#45379,#45380,
#45381,#45382,#45383,#45384,#45385,#45386,#45387,#45388,#45389,#45390,#45391,
#45392,#45393,#45394,#45395,#45396,#45397,#45398,#45399,#45400,#45401,#45402,
#45403,#45404,#45405,#45406,#45407,#45408,#45409,#45410,#45411,#45412,#45413,
#45414,#45415,#45416,#45417,#45418,#45419,#45420,#45421,#45422,#45423,#45424,
#45425,#45426,#45427,#45428,#45429,#45430,#45431,#45432,#45433,#45434,#45435,
#45436,#45437,#45438,#45439,#45440,#45441,#45442,#45443,#45444,#45445,#45446,
#45447));
#48902=AXIS2_PLACEMENT_3D('',#106591,#59297,#59298);
#48903=AXIS2_PLACEMENT_3D('',#106606,#59299,#59300);
#48904=AXIS2_PLACEMENT_3D('',#106612,#59301,#59302);
#48905=AXIS2_PLACEMENT_3D('',#110373,#59303,#59304);
#48906=AXIS2_PLACEMENT_3D('',#110375,#59305,#59306);
#48907=AXIS2_PLACEMENT_3D('',#110377,#59307,#59308);
#48908=AXIS2_PLACEMENT_3D('',#110378,#59309,#59310);
#48909=AXIS2_PLACEMENT_3D('',#110379,#59311,#59312);
#48910=AXIS2_PLACEMENT_3D('',#110420,#59314,#59315);
#48911=AXIS2_PLACEMENT_3D('',#110448,#59317,#59318);
#48912=AXIS2_PLACEMENT_3D('',#110469,#59319,#59320);
#48913=AXIS2_PLACEMENT_3D('',#110510,#59322,#59323);
#48914=AXIS2_PLACEMENT_3D('',#110537,#59325,#59326);
#48915=AXIS2_PLACEMENT_3D('',#110561,#59327,#59328);
#48916=AXIS2_PLACEMENT_3D('',#110602,#59330,#59331);
#48917=AXIS2_PLACEMENT_3D('',#110632,#59333,#59334);
#48918=AXIS2_PLACEMENT_3D('',#110653,#59335,#59336);
#48919=AXIS2_PLACEMENT_3D('',#110694,#59338,#59339);
#48920=AXIS2_PLACEMENT_3D('',#110721,#59341,#59342);
#48921=AXIS2_PLACEMENT_3D('',#110742,#59343,#59344);
#48922=AXIS2_PLACEMENT_3D('',#110781,#59346,#59347);
#48923=AXIS2_PLACEMENT_3D('',#110811,#59349,#59350);
#48924=AXIS2_PLACEMENT_3D('',#110830,#59351,#59352);
#48925=AXIS2_PLACEMENT_3D('',#110871,#59354,#59355);
#48926=AXIS2_PLACEMENT_3D('',#110898,#59357,#59358);
#48927=AXIS2_PLACEMENT_3D('',#110922,#59359,#59360);
#48928=AXIS2_PLACEMENT_3D('',#110963,#59362,#59363);
#48929=AXIS2_PLACEMENT_3D('',#110990,#59365,#59366);
#48930=AXIS2_PLACEMENT_3D('',#111014,#59367,#59368);
#48931=AXIS2_PLACEMENT_3D('',#111055,#59370,#59371);
#48932=AXIS2_PLACEMENT_3D('',#111085,#59373,#59374);
#48933=AXIS2_PLACEMENT_3D('',#111106,#59375,#59376);
#48934=AXIS2_PLACEMENT_3D('',#111145,#59378,#59379);
#48935=AXIS2_PLACEMENT_3D('',#111170,#59381,#59382);
#48936=AXIS2_PLACEMENT_3D('',#111192,#59383,#59384);
#48937=AXIS2_PLACEMENT_3D('',#111233,#59386,#59387);
#48938=AXIS2_PLACEMENT_3D('',#111260,#59389,#59390);
#48939=AXIS2_PLACEMENT_3D('',#111284,#59391,#59392);
#48940=AXIS2_PLACEMENT_3D('',#111325,#59394,#59395);
#48941=AXIS2_PLACEMENT_3D('',#111352,#59397,#59398);
#48942=AXIS2_PLACEMENT_3D('',#111376,#59399,#59400);
#48943=AXIS2_PLACEMENT_3D('',#111417,#59402,#59403);
#48944=AXIS2_PLACEMENT_3D('',#111444,#59405,#59406);
#48945=AXIS2_PLACEMENT_3D('',#111465,#59407,#59408);
#48946=AXIS2_PLACEMENT_3D('',#111504,#59410,#59411);
#48947=AXIS2_PLACEMENT_3D('',#111532,#59413,#59414);
#48948=AXIS2_PLACEMENT_3D('',#111553,#59415,#59416);
#48949=AXIS2_PLACEMENT_3D('',#111594,#59418,#59419);
#48950=AXIS2_PLACEMENT_3D('',#111624,#59421,#59422);
#48951=AXIS2_PLACEMENT_3D('',#111645,#59423,#59424);
#48952=AXIS2_PLACEMENT_3D('',#111686,#59426,#59427);
#48953=AXIS2_PLACEMENT_3D('',#111716,#59429,#59430);
#48954=AXIS2_PLACEMENT_3D('',#111737,#59431,#59432);
#48955=AXIS2_PLACEMENT_3D('',#111778,#59434,#59435);
#48956=AXIS2_PLACEMENT_3D('',#111803,#59437,#59438);
#48957=AXIS2_PLACEMENT_3D('',#111883,#59439,#59440);
#48958=AXIS2_PLACEMENT_3D('',#111922,#59442,#59443);
#48959=AXIS2_PLACEMENT_3D('',#111950,#59445,#59446);
#48960=AXIS2_PLACEMENT_3D('',#111971,#59447,#59448);
#48961=AXIS2_PLACEMENT_3D('',#112012,#59450,#59451);
#48962=AXIS2_PLACEMENT_3D('',#112039,#59453,#59454);
#48963=AXIS2_PLACEMENT_3D('',#112063,#59455,#59456);
#48964=AXIS2_PLACEMENT_3D('',#112102,#59458,#59459);
#48965=AXIS2_PLACEMENT_3D('',#112129,#59461,#59462);
#48966=AXIS2_PLACEMENT_3D('',#112151,#59463,#59464);
#48967=AXIS2_PLACEMENT_3D('',#112192,#59466,#59467);
#48968=AXIS2_PLACEMENT_3D('',#112219,#59469,#59470);
#48969=AXIS2_PLACEMENT_3D('',#112240,#59471,#59472);
#48970=AXIS2_PLACEMENT_3D('',#112279,#59474,#59475);
#48971=AXIS2_PLACEMENT_3D('',#112309,#59477,#59478);
#48972=AXIS2_PLACEMENT_3D('',#112330,#59479,#59480);
#48973=AXIS2_PLACEMENT_3D('',#112371,#59482,#59483);
#48974=AXIS2_PLACEMENT_3D('',#112398,#59485,#59486);
#48975=AXIS2_PLACEMENT_3D('',#112422,#59487,#59488);
#48976=AXIS2_PLACEMENT_3D('',#112461,#59490,#59491);
#48977=AXIS2_PLACEMENT_3D('',#112489,#59493,#59494);
#48978=AXIS2_PLACEMENT_3D('',#112508,#59495,#59496);
#48979=AXIS2_PLACEMENT_3D('',#112547,#59498,#59499);
#48980=AXIS2_PLACEMENT_3D('',#112574,#59501,#59502);
#48981=AXIS2_PLACEMENT_3D('',#112598,#59503,#59504);
#48982=AXIS2_PLACEMENT_3D('',#112637,#59506,#59507);
#48983=AXIS2_PLACEMENT_3D('',#112667,#59509,#59510);
#48984=AXIS2_PLACEMENT_3D('',#112688,#59511,#59512);
#48985=AXIS2_PLACEMENT_3D('',#112729,#59514,#59515);
#48986=AXIS2_PLACEMENT_3D('',#112756,#59517,#59518);
#48987=AXIS2_PLACEMENT_3D('',#112777,#59519,#59520);
#48988=AXIS2_PLACEMENT_3D('',#112818,#59522,#59523);
#48989=AXIS2_PLACEMENT_3D('',#112843,#59525,#59526);
#48990=AXIS2_PLACEMENT_3D('',#112864,#59527,#59528);
#48991=AXIS2_PLACEMENT_3D('',#113014,#59530,#59531);
#48992=AXIS2_PLACEMENT_3D('',#113041,#59533,#59534);
#48993=AXIS2_PLACEMENT_3D('',#113065,#59535,#59536);
#48994=AXIS2_PLACEMENT_3D('',#113104,#59538,#59539);
#48995=AXIS2_PLACEMENT_3D('',#113134,#59541,#59542);
#48996=AXIS2_PLACEMENT_3D('',#113155,#59543,#59544);
#48997=AXIS2_PLACEMENT_3D('',#113196,#59546,#59547);
#48998=AXIS2_PLACEMENT_3D('',#113223,#59549,#59550);
#48999=AXIS2_PLACEMENT_3D('',#113244,#59551,#59552);
#49000=AXIS2_PLACEMENT_3D('',#113283,#59554,#59555);
#49001=AXIS2_PLACEMENT_3D('',#113308,#59557,#59558);
#49002=AXIS2_PLACEMENT_3D('',#113329,#59559,#59560);
#49003=AXIS2_PLACEMENT_3D('',#113421,#59562,#59563);
#49004=AXIS2_PLACEMENT_3D('',#113448,#59565,#59566);
#49005=AXIS2_PLACEMENT_3D('',#113470,#59567,#59568);
#49006=AXIS2_PLACEMENT_3D('',#113562,#59570,#59571);
#49007=AXIS2_PLACEMENT_3D('',#113589,#59573,#59574);
#49008=AXIS2_PLACEMENT_3D('',#113610,#59575,#59576);
#49009=AXIS2_PLACEMENT_3D('',#113651,#59578,#59579);
#49010=AXIS2_PLACEMENT_3D('',#113678,#59581,#59582);
#49011=AXIS2_PLACEMENT_3D('',#113699,#59583,#59584);
#49012=AXIS2_PLACEMENT_3D('',#113738,#59586,#59587);
#49013=AXIS2_PLACEMENT_3D('',#113765,#59589,#59590);
#49014=AXIS2_PLACEMENT_3D('',#113786,#59591,#59592);
#49015=AXIS2_PLACEMENT_3D('',#113878,#59594,#59595);
#49016=AXIS2_PLACEMENT_3D('',#113903,#59597,#59598);
#49017=AXIS2_PLACEMENT_3D('',#113927,#59599,#59600);
#49018=AXIS2_PLACEMENT_3D('',#114021,#59602,#59603);
#49019=AXIS2_PLACEMENT_3D('',#114048,#59605,#59606);
#49020=AXIS2_PLACEMENT_3D('',#114069,#59607,#59608);
#49021=AXIS2_PLACEMENT_3D('',#114161,#59610,#59611);
#49022=AXIS2_PLACEMENT_3D('',#114188,#59613,#59614);
#49023=AXIS2_PLACEMENT_3D('',#114212,#59615,#59616);
#49024=AXIS2_PLACEMENT_3D('',#114304,#59618,#59619);
#49025=AXIS2_PLACEMENT_3D('',#114331,#59621,#59622);
#49026=AXIS2_PLACEMENT_3D('',#114352,#59623,#59624);
#49027=AXIS2_PLACEMENT_3D('',#114442,#59626,#59627);
#49028=AXIS2_PLACEMENT_3D('',#114467,#59629,#59630);
#49029=AXIS2_PLACEMENT_3D('',#114491,#59631,#59632);
#49030=AXIS2_PLACEMENT_3D('',#114587,#59634,#59635);
#49031=AXIS2_PLACEMENT_3D('',#114614,#59637,#59638);
#49032=AXIS2_PLACEMENT_3D('',#114635,#59639,#59640);
#49033=AXIS2_PLACEMENT_3D('',#114729,#59642,#59643);
#49034=AXIS2_PLACEMENT_3D('',#114756,#59645,#59646);
#49035=AXIS2_PLACEMENT_3D('',#114777,#59647,#59648);
#49036=AXIS2_PLACEMENT_3D('',#114871,#59650,#59651);
#49037=AXIS2_PLACEMENT_3D('',#114898,#59653,#59654);
#49038=AXIS2_PLACEMENT_3D('',#114919,#59655,#59656);
#49039=AXIS2_PLACEMENT_3D('',#115013,#59658,#59659);
#49040=AXIS2_PLACEMENT_3D('',#115038,#59661,#59662);
#49041=AXIS2_PLACEMENT_3D('',#115060,#59663,#59664);
#49042=AXIS2_PLACEMENT_3D('',#115156,#59666,#59667);
#49043=AXIS2_PLACEMENT_3D('',#115183,#59669,#59670);
#49044=AXIS2_PLACEMENT_3D('',#115207,#59671,#59672);
#49045=AXIS2_PLACEMENT_3D('',#115301,#59674,#59675);
#49046=AXIS2_PLACEMENT_3D('',#115329,#59677,#59678);
#49047=AXIS2_PLACEMENT_3D('',#115348,#59679,#59680);
#49048=AXIS2_PLACEMENT_3D('',#115444,#59682,#59683);
#49049=AXIS2_PLACEMENT_3D('',#115474,#59685,#59686);
#49050=AXIS2_PLACEMENT_3D('',#115495,#59687,#59688);
#49051=AXIS2_PLACEMENT_3D('',#115591,#59690,#59691);
#49052=AXIS2_PLACEMENT_3D('',#115614,#59693,#59694);
#49053=AXIS2_PLACEMENT_3D('',#115640,#59695,#59696);
#49054=AXIS2_PLACEMENT_3D('',#115736,#59698,#59699);
#49055=AXIS2_PLACEMENT_3D('',#115763,#59701,#59702);
#49056=AXIS2_PLACEMENT_3D('',#115784,#59703,#59704);
#49057=AXIS2_PLACEMENT_3D('',#115878,#59706,#59707);
#49058=AXIS2_PLACEMENT_3D('',#115903,#59709,#59710);
#49059=AXIS2_PLACEMENT_3D('',#115925,#59711,#59712);
#49060=AXIS2_PLACEMENT_3D('',#116023,#59714,#59715);
#49061=AXIS2_PLACEMENT_3D('',#116050,#59717,#59718);
#49062=AXIS2_PLACEMENT_3D('',#116071,#59719,#59720);
#49063=AXIS2_PLACEMENT_3D('',#116165,#59722,#59723);
#49064=AXIS2_PLACEMENT_3D('',#116188,#59725,#59726);
#49065=AXIS2_PLACEMENT_3D('',#116214,#59727,#59728);
#49066=AXIS2_PLACEMENT_3D('',#116310,#59730,#59731);
#49067=AXIS2_PLACEMENT_3D('',#116337,#59733,#59734);
#49068=AXIS2_PLACEMENT_3D('',#116361,#59735,#59736);
#49069=AXIS2_PLACEMENT_3D('',#116457,#59738,#59739);
#49070=AXIS2_PLACEMENT_3D('',#116482,#59741,#59742);
#49071=AXIS2_PLACEMENT_3D('',#116506,#59743,#59744);
#49072=AXIS2_PLACEMENT_3D('',#116604,#59746,#59747);
#49073=AXIS2_PLACEMENT_3D('',#116631,#59749,#59750);
#49074=AXIS2_PLACEMENT_3D('',#116655,#59751,#59752);
#49075=AXIS2_PLACEMENT_3D('',#116751,#59754,#59755);
#49076=AXIS2_PLACEMENT_3D('',#116774,#59757,#59758);
#49077=AXIS2_PLACEMENT_3D('',#116800,#59759,#59760);
#49078=AXIS2_PLACEMENT_3D('',#116896,#59762,#59763);
#49079=AXIS2_PLACEMENT_3D('',#116921,#59765,#59766);
#49080=AXIS2_PLACEMENT_3D('',#116947,#59767,#59768);
#49081=AXIS2_PLACEMENT_3D('',#117043,#59770,#59771);
#49082=AXIS2_PLACEMENT_3D('',#117069,#59773,#59774);
#49083=AXIS2_PLACEMENT_3D('',#117092,#59775,#59776);
#49084=AXIS2_PLACEMENT_3D('',#117190,#59778,#59779);
#49085=AXIS2_PLACEMENT_3D('',#117217,#59781,#59782);
#49086=AXIS2_PLACEMENT_3D('',#117241,#59783,#59784);
#49087=AXIS2_PLACEMENT_3D('',#117337,#59786,#59787);
#49088=AXIS2_PLACEMENT_3D('',#117362,#59789,#59790);
#49089=AXIS2_PLACEMENT_3D('',#117386,#59791,#59792);
#49090=AXIS2_PLACEMENT_3D('',#117480,#59794,#59795);
#49091=AXIS2_PLACEMENT_3D('',#117505,#59797,#59798);
#49092=AXIS2_PLACEMENT_3D('',#117531,#59799,#59800);
#49093=AXIS2_PLACEMENT_3D('',#117629,#59802,#59803);
#49094=AXIS2_PLACEMENT_3D('',#117659,#59805,#59806);
#49095=AXIS2_PLACEMENT_3D('',#117680,#59807,#59808);
#49096=AXIS2_PLACEMENT_3D('',#117778,#59810,#59811);
#49097=AXIS2_PLACEMENT_3D('',#117803,#59813,#59814);
#49098=AXIS2_PLACEMENT_3D('',#117829,#59815,#59816);
#49099=AXIS2_PLACEMENT_3D('',#118032,#59818,#59819);
#49100=AXIS2_PLACEMENT_3D('',#118059,#59821,#59822);
#49101=AXIS2_PLACEMENT_3D('',#118083,#59823,#59824);
#49102=AXIS2_PLACEMENT_3D('',#118179,#59826,#59827);
#49103=AXIS2_PLACEMENT_3D('',#118205,#59829,#59830);
#49104=AXIS2_PLACEMENT_3D('',#118228,#59831,#59832);
#49105=AXIS2_PLACEMENT_3D('',#118326,#59834,#59835);
#49106=AXIS2_PLACEMENT_3D('',#118351,#59837,#59838);
#49107=AXIS2_PLACEMENT_3D('',#118377,#59839,#59840);
#49108=AXIS2_PLACEMENT_3D('',#118475,#59842,#59843);
#49109=AXIS2_PLACEMENT_3D('',#118503,#59845,#59846);
#49110=AXIS2_PLACEMENT_3D('',#118526,#59847,#59848);
#49111=AXIS2_PLACEMENT_3D('',#118729,#59850,#59851);
#49112=AXIS2_PLACEMENT_3D('',#118754,#59853,#59854);
#49113=AXIS2_PLACEMENT_3D('',#118780,#59855,#59856);
#49114=AXIS2_PLACEMENT_3D('',#118872,#59858,#59859);
#49115=AXIS2_PLACEMENT_3D('',#118900,#59861,#59862);
#49116=AXIS2_PLACEMENT_3D('',#118921,#59863,#59864);
#49117=AXIS2_PLACEMENT_3D('',#119019,#59866,#59867);
#49118=AXIS2_PLACEMENT_3D('',#119049,#59869,#59870);
#49119=AXIS2_PLACEMENT_3D('',#119070,#59871,#59872);
#49120=AXIS2_PLACEMENT_3D('',#119168,#59874,#59875);
#49121=AXIS2_PLACEMENT_3D('',#119196,#59877,#59878);
#49122=AXIS2_PLACEMENT_3D('',#119219,#59879,#59880);
#49123=AXIS2_PLACEMENT_3D('',#119523,#59882,#59883);
#49124=AXIS2_PLACEMENT_3D('',#119550,#59885,#59886);
#49125=AXIS2_PLACEMENT_3D('',#119574,#59887,#59888);
#49126=AXIS2_PLACEMENT_3D('',#119668,#59890,#59891);
#49127=AXIS2_PLACEMENT_3D('',#119693,#59893,#59894);
#49128=AXIS2_PLACEMENT_3D('',#119719,#59895,#59896);
#49129=AXIS2_PLACEMENT_3D('',#119817,#59898,#59899);
#49130=AXIS2_PLACEMENT_3D('',#119842,#59901,#59902);
#49131=AXIS2_PLACEMENT_3D('',#119868,#59903,#59904);
#49132=AXIS2_PLACEMENT_3D('',#119964,#59906,#59907);
#49133=AXIS2_PLACEMENT_3D('',#119989,#59909,#59910);
#49134=AXIS2_PLACEMENT_3D('',#120013,#59911,#59912);
#49135=AXIS2_PLACEMENT_3D('',#120109,#59914,#59915);
#49136=AXIS2_PLACEMENT_3D('',#120134,#59917,#59918);
#49137=AXIS2_PLACEMENT_3D('',#120160,#59919,#59920);
#49138=AXIS2_PLACEMENT_3D('',#120254,#59922,#59923);
#49139=AXIS2_PLACEMENT_3D('',#120281,#59925,#59926);
#49140=AXIS2_PLACEMENT_3D('',#120303,#59927,#59928);
#49141=AXIS2_PLACEMENT_3D('',#120401,#59930,#59931);
#49142=AXIS2_PLACEMENT_3D('',#120431,#59933,#59934);
#49143=AXIS2_PLACEMENT_3D('',#120452,#59935,#59936);
#49144=AXIS2_PLACEMENT_3D('',#120548,#59938,#59939);
#49145=AXIS2_PLACEMENT_3D('',#120576,#59941,#59942);
#49146=AXIS2_PLACEMENT_3D('',#120599,#59943,#59944);
#49147=AXIS2_PLACEMENT_3D('',#120693,#59946,#59947);
#49148=AXIS2_PLACEMENT_3D('',#120720,#59949,#59950);
#49149=AXIS2_PLACEMENT_3D('',#120744,#59951,#59952);
#49150=AXIS2_PLACEMENT_3D('',#120838,#59954,#59955);
#49151=AXIS2_PLACEMENT_3D('',#120865,#59957,#59958);
#49152=AXIS2_PLACEMENT_3D('',#120887,#59959,#59960);
#49153=AXIS2_PLACEMENT_3D('',#120983,#59962,#59963);
#49154=AXIS2_PLACEMENT_3D('',#121013,#59965,#59966);
#49155=AXIS2_PLACEMENT_3D('',#121034,#59967,#59968);
#49156=AXIS2_PLACEMENT_3D('',#121126,#59970,#59971);
#49157=AXIS2_PLACEMENT_3D('',#121151,#59973,#59974);
#49158=AXIS2_PLACEMENT_3D('',#121175,#59975,#59976);
#49159=AXIS2_PLACEMENT_3D('',#121265,#59978,#59979);
#49160=AXIS2_PLACEMENT_3D('',#121288,#59981,#59982);
#49161=AXIS2_PLACEMENT_3D('',#121314,#59983,#59984);
#49162=AXIS2_PLACEMENT_3D('',#121406,#59986,#59987);
#49163=AXIS2_PLACEMENT_3D('',#121433,#59989,#59990);
#49164=AXIS2_PLACEMENT_3D('',#121455,#59991,#59992);
#49165=AXIS2_PLACEMENT_3D('',#121551,#59994,#59995);
#49166=AXIS2_PLACEMENT_3D('',#121578,#59997,#59998);
#49167=AXIS2_PLACEMENT_3D('',#121599,#59999,#60000);
#49168=AXIS2_PLACEMENT_3D('',#121693,#60002,#60003);
#49169=AXIS2_PLACEMENT_3D('',#121720,#60005,#60006);
#49170=AXIS2_PLACEMENT_3D('',#121739,#60007,#60008);
#49171=AXIS2_PLACEMENT_3D('',#121829,#60010,#60011);
#49172=AXIS2_PLACEMENT_3D('',#121854,#60013,#60014);
#49173=AXIS2_PLACEMENT_3D('',#121878,#60015,#60016);
#49174=AXIS2_PLACEMENT_3D('',#121972,#60018,#60019);
#49175=AXIS2_PLACEMENT_3D('',#121999,#60021,#60022);
#49176=AXIS2_PLACEMENT_3D('',#122020,#60023,#60024);
#49177=AXIS2_PLACEMENT_3D('',#122114,#60026,#60027);
#49178=AXIS2_PLACEMENT_3D('',#122141,#60029,#60030);
#49179=AXIS2_PLACEMENT_3D('',#122162,#60031,#60032);
#49180=AXIS2_PLACEMENT_3D('',#122256,#60034,#60035);
#49181=AXIS2_PLACEMENT_3D('',#122283,#60037,#60038);
#49182=AXIS2_PLACEMENT_3D('',#122302,#60039,#60040);
#49183=AXIS2_PLACEMENT_3D('',#122341,#60042,#60043);
#49184=AXIS2_PLACEMENT_3D('',#122366,#60045,#60046);
#49185=AXIS2_PLACEMENT_3D('',#122390,#60047,#60048);
#49186=AXIS2_PLACEMENT_3D('',#122431,#60050,#60051);
#49187=AXIS2_PLACEMENT_3D('',#122461,#60053,#60054);
#49188=AXIS2_PLACEMENT_3D('',#122482,#60055,#60056);
#49189=AXIS2_PLACEMENT_3D('',#122574,#60058,#60059);
#49190=AXIS2_PLACEMENT_3D('',#122601,#60061,#60062);
#49191=AXIS2_PLACEMENT_3D('',#122622,#60063,#60064);
#49192=AXIS2_PLACEMENT_3D('',#122716,#60066,#60067);
#49193=AXIS2_PLACEMENT_3D('',#122743,#60069,#60070);
#49194=AXIS2_PLACEMENT_3D('',#122764,#60071,#60072);
#49195=AXIS2_PLACEMENT_3D('',#122801,#60074,#60075);
#49196=AXIS2_PLACEMENT_3D('',#122826,#60077,#60078);
#49197=AXIS2_PLACEMENT_3D('',#122848,#60079,#60080);
#49198=AXIS2_PLACEMENT_3D('',#122889,#60082,#60083);
#49199=AXIS2_PLACEMENT_3D('',#122919,#60085,#60086);
#49200=AXIS2_PLACEMENT_3D('',#122940,#60087,#60088);
#49201=AXIS2_PLACEMENT_3D('',#122981,#60090,#60091);
#49202=AXIS2_PLACEMENT_3D('',#123008,#60093,#60094);
#49203=AXIS2_PLACEMENT_3D('',#123029,#60095,#60096);
#49204=AXIS2_PLACEMENT_3D('',#123070,#60098,#60099);
#49205=AXIS2_PLACEMENT_3D('',#123097,#60101,#60102);
#49206=AXIS2_PLACEMENT_3D('',#123118,#60103,#60104);
#49207=AXIS2_PLACEMENT_3D('',#123155,#60106,#60107);
#49208=AXIS2_PLACEMENT_3D('',#123180,#60109,#60110);
#49209=AXIS2_PLACEMENT_3D('',#123202,#60111,#60112);
#49210=AXIS2_PLACEMENT_3D('',#123243,#60114,#60115);
#49211=AXIS2_PLACEMENT_3D('',#123270,#60117,#60118);
#49212=AXIS2_PLACEMENT_3D('',#123291,#60119,#60120);
#49213=AXIS2_PLACEMENT_3D('',#123330,#60122,#60123);
#49214=AXIS2_PLACEMENT_3D('',#123355,#60125,#60126);
#49215=AXIS2_PLACEMENT_3D('',#123376,#60127,#60128);
#49216=AXIS2_PLACEMENT_3D('',#123417,#60130,#60131);
#49217=AXIS2_PLACEMENT_3D('',#123444,#60133,#60134);
#49218=AXIS2_PLACEMENT_3D('',#123465,#60135,#60136);
#49219=AXIS2_PLACEMENT_3D('',#123502,#60138,#60139);
#49220=AXIS2_PLACEMENT_3D('',#123527,#60141,#60142);
#49221=AXIS2_PLACEMENT_3D('',#123549,#60143,#60144);
#49222=AXIS2_PLACEMENT_3D('',#123590,#60146,#60147);
#49223=AXIS2_PLACEMENT_3D('',#123620,#60149,#60150);
#49224=AXIS2_PLACEMENT_3D('',#123641,#60151,#60152);
#49225=AXIS2_PLACEMENT_3D('',#123680,#60154,#60155);
#49226=AXIS2_PLACEMENT_3D('',#123705,#60157,#60158);
#49227=AXIS2_PLACEMENT_3D('',#123729,#60159,#60160);
#49228=AXIS2_PLACEMENT_3D('',#123770,#60162,#60163);
#49229=AXIS2_PLACEMENT_3D('',#123797,#60165,#60166);
#49230=AXIS2_PLACEMENT_3D('',#123821,#60167,#60168);
#49231=AXIS2_PLACEMENT_3D('',#123860,#60170,#60171);
#49232=AXIS2_PLACEMENT_3D('',#123887,#60173,#60174);
#49233=AXIS2_PLACEMENT_3D('',#123909,#60175,#60176);
#49234=AXIS2_PLACEMENT_3D('',#123950,#60178,#60179);
#49235=AXIS2_PLACEMENT_3D('',#123977,#60181,#60182);
#49236=AXIS2_PLACEMENT_3D('',#123998,#60183,#60184);
#49237=AXIS2_PLACEMENT_3D('',#124037,#60186,#60187);
#49238=AXIS2_PLACEMENT_3D('',#124067,#60189,#60190);
#49239=AXIS2_PLACEMENT_3D('',#124086,#60191,#60192);
#49240=AXIS2_PLACEMENT_3D('',#124127,#60194,#60195);
#49241=AXIS2_PLACEMENT_3D('',#124154,#60197,#60198);
#49242=AXIS2_PLACEMENT_3D('',#124175,#60199,#60200);
#49243=AXIS2_PLACEMENT_3D('',#124214,#60202,#60203);
#49244=AXIS2_PLACEMENT_3D('',#124241,#60205,#60206);
#49245=AXIS2_PLACEMENT_3D('',#124263,#60207,#60208);
#49246=AXIS2_PLACEMENT_3D('',#124304,#60210,#60211);
#49247=AXIS2_PLACEMENT_3D('',#124334,#60213,#60214);
#49248=AXIS2_PLACEMENT_3D('',#124355,#60215,#60216);
#49249=AXIS2_PLACEMENT_3D('',#124394,#60218,#60219);
#49250=AXIS2_PLACEMENT_3D('',#124424,#60221,#60222);
#49251=AXIS2_PLACEMENT_3D('',#124443,#60223,#60224);
#49252=AXIS2_PLACEMENT_3D('',#124484,#60226,#60227);
#49253=AXIS2_PLACEMENT_3D('',#124514,#60229,#60230);
#49254=AXIS2_PLACEMENT_3D('',#124535,#60231,#60232);
#49255=AXIS2_PLACEMENT_3D('',#124574,#60234,#60235);
#49256=AXIS2_PLACEMENT_3D('',#124601,#60237,#60238);
#49257=AXIS2_PLACEMENT_3D('',#124625,#60239,#60240);
#49258=AXIS2_PLACEMENT_3D('',#124666,#60242,#60243);
#49259=AXIS2_PLACEMENT_3D('',#124694,#60245,#60246);
#49260=AXIS2_PLACEMENT_3D('',#124715,#60247,#60248);
#49261=AXIS2_PLACEMENT_3D('',#124756,#60250,#60251);
#49262=AXIS2_PLACEMENT_3D('',#124786,#60253,#60254);
#49263=AXIS2_PLACEMENT_3D('',#124807,#60255,#60256);
#49264=AXIS2_PLACEMENT_3D('',#124846,#60258,#60259);
#49265=AXIS2_PLACEMENT_3D('',#124873,#60261,#60262);
#49266=AXIS2_PLACEMENT_3D('',#124897,#60263,#60264);
#49267=AXIS2_PLACEMENT_3D('',#124899,#60265,#60266);
#49268=AXIS2_PLACEMENT_3D('',#124902,#60268,#60269);
#49269=AXIS2_PLACEMENT_3D('',#124903,#60270,#60271);
#49270=AXIS2_PLACEMENT_3D('',#124905,#60272,#60273);
#49271=AXIS2_PLACEMENT_3D('',#124908,#60275,#60276);
#49272=AXIS2_PLACEMENT_3D('',#124909,#60277,#60278);
#49273=AXIS2_PLACEMENT_3D('',#124911,#60279,#60280);
#49274=AXIS2_PLACEMENT_3D('',#124914,#60282,#60283);
#49275=AXIS2_PLACEMENT_3D('',#124915,#60284,#60285);
#49276=AXIS2_PLACEMENT_3D('',#124917,#60286,#60287);
#49277=AXIS2_PLACEMENT_3D('',#124920,#60289,#60290);
#49278=AXIS2_PLACEMENT_3D('',#124921,#60291,#60292);
#49279=AXIS2_PLACEMENT_3D('',#124923,#60293,#60294);
#49280=AXIS2_PLACEMENT_3D('',#124926,#60296,#60297);
#49281=AXIS2_PLACEMENT_3D('',#124927,#60298,#60299);
#49282=AXIS2_PLACEMENT_3D('',#124929,#60300,#60301);
#49283=AXIS2_PLACEMENT_3D('',#124932,#60303,#60304);
#49284=AXIS2_PLACEMENT_3D('',#124933,#60305,#60306);
#49285=AXIS2_PLACEMENT_3D('',#124935,#60307,#60308);
#49286=AXIS2_PLACEMENT_3D('',#124938,#60310,#60311);
#49287=AXIS2_PLACEMENT_3D('',#124939,#60312,#60313);
#49288=AXIS2_PLACEMENT_3D('',#124941,#60314,#60315);
#49289=AXIS2_PLACEMENT_3D('',#124944,#60317,#60318);
#49290=AXIS2_PLACEMENT_3D('',#124945,#60319,#60320);
#49291=AXIS2_PLACEMENT_3D('',#124947,#60321,#60322);
#49292=AXIS2_PLACEMENT_3D('',#124950,#60324,#60325);
#49293=AXIS2_PLACEMENT_3D('',#124951,#60326,#60327);
#49294=AXIS2_PLACEMENT_3D('',#124953,#60328,#60329);
#49295=AXIS2_PLACEMENT_3D('',#124956,#60331,#60332);
#49296=AXIS2_PLACEMENT_3D('',#124957,#60333,#60334);
#49297=AXIS2_PLACEMENT_3D('',#124959,#60335,#60336);
#49298=AXIS2_PLACEMENT_3D('',#124962,#60338,#60339);
#49299=AXIS2_PLACEMENT_3D('',#124963,#60340,#60341);
#49300=AXIS2_PLACEMENT_3D('',#124965,#60342,#60343);
#49301=AXIS2_PLACEMENT_3D('',#124968,#60345,#60346);
#49302=AXIS2_PLACEMENT_3D('',#124969,#60347,#60348);
#49303=AXIS2_PLACEMENT_3D('',#124971,#60349,#60350);
#49304=AXIS2_PLACEMENT_3D('',#124974,#60352,#60353);
#49305=AXIS2_PLACEMENT_3D('',#124975,#60354,#60355);
#49306=AXIS2_PLACEMENT_3D('',#124977,#60356,#60357);
#49307=AXIS2_PLACEMENT_3D('',#124980,#60359,#60360);
#49308=AXIS2_PLACEMENT_3D('',#124981,#60361,#60362);
#49309=AXIS2_PLACEMENT_3D('',#124983,#60363,#60364);
#49310=AXIS2_PLACEMENT_3D('',#124986,#60366,#60367);
#49311=AXIS2_PLACEMENT_3D('',#124987,#60368,#60369);
#49312=AXIS2_PLACEMENT_3D('',#124989,#60370,#60371);
#49313=AXIS2_PLACEMENT_3D('',#124992,#60373,#60374);
#49314=AXIS2_PLACEMENT_3D('',#124993,#60375,#60376);
#49315=AXIS2_PLACEMENT_3D('',#124995,#60377,#60378);
#49316=AXIS2_PLACEMENT_3D('',#124998,#60380,#60381);
#49317=AXIS2_PLACEMENT_3D('',#124999,#60382,#60383);
#49318=AXIS2_PLACEMENT_3D('',#125001,#60384,#60385);
#49319=AXIS2_PLACEMENT_3D('',#125004,#60387,#60388);
#49320=AXIS2_PLACEMENT_3D('',#125005,#60389,#60390);
#49321=AXIS2_PLACEMENT_3D('',#125007,#60391,#60392);
#49322=AXIS2_PLACEMENT_3D('',#125010,#60394,#60395);
#49323=AXIS2_PLACEMENT_3D('',#125011,#60396,#60397);
#49324=AXIS2_PLACEMENT_3D('',#125013,#60398,#60399);
#49325=AXIS2_PLACEMENT_3D('',#125016,#60401,#60402);
#49326=AXIS2_PLACEMENT_3D('',#125017,#60403,#60404);
#49327=AXIS2_PLACEMENT_3D('',#125019,#60405,#60406);
#49328=AXIS2_PLACEMENT_3D('',#125022,#60408,#60409);
#49329=AXIS2_PLACEMENT_3D('',#125023,#60410,#60411);
#49330=AXIS2_PLACEMENT_3D('',#125025,#60412,#60413);
#49331=AXIS2_PLACEMENT_3D('',#125028,#60415,#60416);
#49332=AXIS2_PLACEMENT_3D('',#125029,#60417,#60418);
#49333=AXIS2_PLACEMENT_3D('',#125031,#60419,#60420);
#49334=AXIS2_PLACEMENT_3D('',#125034,#60422,#60423);
#49335=AXIS2_PLACEMENT_3D('',#125035,#60424,#60425);
#49336=AXIS2_PLACEMENT_3D('',#125037,#60426,#60427);
#49337=AXIS2_PLACEMENT_3D('',#125040,#60429,#60430);
#49338=AXIS2_PLACEMENT_3D('',#125041,#60431,#60432);
#49339=AXIS2_PLACEMENT_3D('',#125043,#60433,#60434);
#49340=AXIS2_PLACEMENT_3D('',#125046,#60436,#60437);
#49341=AXIS2_PLACEMENT_3D('',#125047,#60438,#60439);
#49342=AXIS2_PLACEMENT_3D('',#125049,#60440,#60441);
#49343=AXIS2_PLACEMENT_3D('',#125052,#60443,#60444);
#49344=AXIS2_PLACEMENT_3D('',#125053,#60445,#60446);
#49345=AXIS2_PLACEMENT_3D('',#125055,#60447,#60448);
#49346=AXIS2_PLACEMENT_3D('',#125058,#60450,#60451);
#49347=AXIS2_PLACEMENT_3D('',#125059,#60452,#60453);
#49348=AXIS2_PLACEMENT_3D('',#125061,#60454,#60455);
#49349=AXIS2_PLACEMENT_3D('',#125064,#60457,#60458);
#49350=AXIS2_PLACEMENT_3D('',#125065,#60459,#60460);
#49351=AXIS2_PLACEMENT_3D('',#125067,#60461,#60462);
#49352=AXIS2_PLACEMENT_3D('',#125070,#60464,#60465);
#49353=AXIS2_PLACEMENT_3D('',#125071,#60466,#60467);
#49354=AXIS2_PLACEMENT_3D('',#125073,#60468,#60469);
#49355=AXIS2_PLACEMENT_3D('',#125076,#60471,#60472);
#49356=AXIS2_PLACEMENT_3D('',#125077,#60473,#60474);
#49357=AXIS2_PLACEMENT_3D('',#125079,#60475,#60476);
#49358=AXIS2_PLACEMENT_3D('',#125082,#60478,#60479);
#49359=AXIS2_PLACEMENT_3D('',#125083,#60480,#60481);
#49360=AXIS2_PLACEMENT_3D('',#125085,#60482,#60483);
#49361=AXIS2_PLACEMENT_3D('',#125088,#60485,#60486);
#49362=AXIS2_PLACEMENT_3D('',#125089,#60487,#60488);
#49363=AXIS2_PLACEMENT_3D('',#125091,#60489,#60490);
#49364=AXIS2_PLACEMENT_3D('',#125094,#60492,#60493);
#49365=AXIS2_PLACEMENT_3D('',#125095,#60494,#60495);
#49366=AXIS2_PLACEMENT_3D('',#125097,#60496,#60497);
#49367=AXIS2_PLACEMENT_3D('',#125100,#60499,#60500);
#49368=AXIS2_PLACEMENT_3D('',#125101,#60501,#60502);
#49369=AXIS2_PLACEMENT_3D('',#125103,#60503,#60504);
#49370=AXIS2_PLACEMENT_3D('',#125106,#60506,#60507);
#49371=AXIS2_PLACEMENT_3D('',#125107,#60508,#60509);
#49372=AXIS2_PLACEMENT_3D('',#125109,#60510,#60511);
#49373=AXIS2_PLACEMENT_3D('',#125112,#60513,#60514);
#49374=AXIS2_PLACEMENT_3D('',#125113,#60515,#60516);
#49375=AXIS2_PLACEMENT_3D('',#125115,#60517,#60518);
#49376=AXIS2_PLACEMENT_3D('',#125118,#60520,#60521);
#49377=AXIS2_PLACEMENT_3D('',#125119,#60522,#60523);
#49378=AXIS2_PLACEMENT_3D('',#125121,#60524,#60525);
#49379=AXIS2_PLACEMENT_3D('',#125124,#60527,#60528);
#49380=AXIS2_PLACEMENT_3D('',#125125,#60529,#60530);
#49381=AXIS2_PLACEMENT_3D('',#125127,#60531,#60532);
#49382=AXIS2_PLACEMENT_3D('',#125130,#60534,#60535);
#49383=AXIS2_PLACEMENT_3D('',#125131,#60536,#60537);
#49384=AXIS2_PLACEMENT_3D('',#125133,#60538,#60539);
#49385=AXIS2_PLACEMENT_3D('',#125136,#60541,#60542);
#49386=AXIS2_PLACEMENT_3D('',#125137,#60543,#60544);
#49387=AXIS2_PLACEMENT_3D('',#125139,#60545,#60546);
#49388=AXIS2_PLACEMENT_3D('',#125142,#60548,#60549);
#49389=AXIS2_PLACEMENT_3D('',#125143,#60550,#60551);
#49390=AXIS2_PLACEMENT_3D('',#125145,#60552,#60553);
#49391=AXIS2_PLACEMENT_3D('',#125148,#60555,#60556);
#49392=AXIS2_PLACEMENT_3D('',#125149,#60557,#60558);
#49393=AXIS2_PLACEMENT_3D('',#125151,#60559,#60560);
#49394=AXIS2_PLACEMENT_3D('',#125154,#60562,#60563);
#49395=AXIS2_PLACEMENT_3D('',#125155,#60564,#60565);
#49396=AXIS2_PLACEMENT_3D('',#125157,#60566,#60567);
#49397=AXIS2_PLACEMENT_3D('',#125160,#60569,#60570);
#49398=AXIS2_PLACEMENT_3D('',#125161,#60571,#60572);
#49399=AXIS2_PLACEMENT_3D('',#125163,#60573,#60574);
#49400=AXIS2_PLACEMENT_3D('',#125166,#60576,#60577);
#49401=AXIS2_PLACEMENT_3D('',#125167,#60578,#60579);
#49402=AXIS2_PLACEMENT_3D('',#125169,#60580,#60581);
#49403=AXIS2_PLACEMENT_3D('',#125172,#60583,#60584);
#49404=AXIS2_PLACEMENT_3D('',#125173,#60585,#60586);
#49405=AXIS2_PLACEMENT_3D('',#125175,#60587,#60588);
#49406=AXIS2_PLACEMENT_3D('',#125178,#60590,#60591);
#49407=AXIS2_PLACEMENT_3D('',#125179,#60592,#60593);
#49408=AXIS2_PLACEMENT_3D('',#125181,#60594,#60595);
#49409=AXIS2_PLACEMENT_3D('',#125184,#60597,#60598);
#49410=AXIS2_PLACEMENT_3D('',#125185,#60599,#60600);
#49411=AXIS2_PLACEMENT_3D('',#125187,#60601,#60602);
#49412=AXIS2_PLACEMENT_3D('',#125190,#60604,#60605);
#49413=AXIS2_PLACEMENT_3D('',#125191,#60606,#60607);
#49414=AXIS2_PLACEMENT_3D('',#125193,#60608,#60609);
#49415=AXIS2_PLACEMENT_3D('',#125196,#60611,#60612);
#49416=AXIS2_PLACEMENT_3D('',#125197,#60613,#60614);
#49417=AXIS2_PLACEMENT_3D('',#125199,#60615,#60616);
#49418=AXIS2_PLACEMENT_3D('',#125202,#60618,#60619);
#49419=AXIS2_PLACEMENT_3D('',#125203,#60620,#60621);
#49420=AXIS2_PLACEMENT_3D('',#125205,#60622,#60623);
#49421=AXIS2_PLACEMENT_3D('',#125208,#60625,#60626);
#49422=AXIS2_PLACEMENT_3D('',#125209,#60627,#60628);
#49423=AXIS2_PLACEMENT_3D('',#125211,#60629,#60630);
#49424=AXIS2_PLACEMENT_3D('',#125214,#60632,#60633);
#49425=AXIS2_PLACEMENT_3D('',#125215,#60634,#60635);
#49426=AXIS2_PLACEMENT_3D('',#125217,#60636,#60637);
#49427=AXIS2_PLACEMENT_3D('',#125220,#60639,#60640);
#49428=AXIS2_PLACEMENT_3D('',#125221,#60641,#60642);
#49429=AXIS2_PLACEMENT_3D('',#125223,#60643,#60644);
#49430=AXIS2_PLACEMENT_3D('',#125226,#60646,#60647);
#49431=AXIS2_PLACEMENT_3D('',#125227,#60648,#60649);
#49432=AXIS2_PLACEMENT_3D('',#125229,#60650,#60651);
#49433=AXIS2_PLACEMENT_3D('',#125232,#60653,#60654);
#49434=AXIS2_PLACEMENT_3D('',#125233,#60655,#60656);
#49435=AXIS2_PLACEMENT_3D('',#125235,#60657,#60658);
#49436=AXIS2_PLACEMENT_3D('',#125238,#60660,#60661);
#49437=AXIS2_PLACEMENT_3D('',#125239,#60662,#60663);
#49438=AXIS2_PLACEMENT_3D('',#125241,#60664,#60665);
#49439=AXIS2_PLACEMENT_3D('',#125244,#60667,#60668);
#49440=AXIS2_PLACEMENT_3D('',#125245,#60669,#60670);
#49441=AXIS2_PLACEMENT_3D('',#125247,#60671,#60672);
#49442=AXIS2_PLACEMENT_3D('',#125250,#60674,#60675);
#49443=AXIS2_PLACEMENT_3D('',#125251,#60676,#60677);
#49444=AXIS2_PLACEMENT_3D('',#125253,#60678,#60679);
#49445=AXIS2_PLACEMENT_3D('',#125256,#60681,#60682);
#49446=AXIS2_PLACEMENT_3D('',#125257,#60683,#60684);
#49447=AXIS2_PLACEMENT_3D('',#125259,#60685,#60686);
#49448=AXIS2_PLACEMENT_3D('',#125262,#60688,#60689);
#49449=AXIS2_PLACEMENT_3D('',#125263,#60690,#60691);
#49450=AXIS2_PLACEMENT_3D('',#125265,#60692,#60693);
#49451=AXIS2_PLACEMENT_3D('',#125268,#60695,#60696);
#49452=AXIS2_PLACEMENT_3D('',#125269,#60697,#60698);
#49453=AXIS2_PLACEMENT_3D('',#125271,#60699,#60700);
#49454=AXIS2_PLACEMENT_3D('',#125274,#60702,#60703);
#49455=AXIS2_PLACEMENT_3D('',#125275,#60704,#60705);
#49456=AXIS2_PLACEMENT_3D('',#125277,#60706,#60707);
#49457=AXIS2_PLACEMENT_3D('',#125280,#60709,#60710);
#49458=AXIS2_PLACEMENT_3D('',#125281,#60711,#60712);
#49459=AXIS2_PLACEMENT_3D('',#125283,#60713,#60714);
#49460=AXIS2_PLACEMENT_3D('',#125286,#60716,#60717);
#49461=AXIS2_PLACEMENT_3D('',#125287,#60718,#60719);
#49462=AXIS2_PLACEMENT_3D('',#125289,#60720,#60721);
#49463=AXIS2_PLACEMENT_3D('',#125292,#60723,#60724);
#49464=AXIS2_PLACEMENT_3D('',#125293,#60725,#60726);
#49465=AXIS2_PLACEMENT_3D('',#125295,#60727,#60728);
#49466=AXIS2_PLACEMENT_3D('',#125298,#60730,#60731);
#49467=AXIS2_PLACEMENT_3D('',#125299,#60732,#60733);
#49468=AXIS2_PLACEMENT_3D('',#125301,#60734,#60735);
#49469=AXIS2_PLACEMENT_3D('',#125304,#60737,#60738);
#49470=AXIS2_PLACEMENT_3D('',#125305,#60739,#60740);
#49471=AXIS2_PLACEMENT_3D('',#125307,#60741,#60742);
#49472=AXIS2_PLACEMENT_3D('',#125310,#60744,#60745);
#49473=AXIS2_PLACEMENT_3D('',#125311,#60746,#60747);
#49474=AXIS2_PLACEMENT_3D('',#125313,#60748,#60749);
#49475=AXIS2_PLACEMENT_3D('',#125316,#60751,#60752);
#49476=AXIS2_PLACEMENT_3D('',#125317,#60753,#60754);
#49477=AXIS2_PLACEMENT_3D('',#125319,#60755,#60756);
#49478=AXIS2_PLACEMENT_3D('',#125322,#60758,#60759);
#49479=AXIS2_PLACEMENT_3D('',#125323,#60760,#60761);
#49480=AXIS2_PLACEMENT_3D('',#125325,#60762,#60763);
#49481=AXIS2_PLACEMENT_3D('',#125328,#60765,#60766);
#49482=AXIS2_PLACEMENT_3D('',#125329,#60767,#60768);
#49483=AXIS2_PLACEMENT_3D('',#125331,#60769,#60770);
#49484=AXIS2_PLACEMENT_3D('',#125334,#60772,#60773);
#49485=AXIS2_PLACEMENT_3D('',#125335,#60774,#60775);
#49486=AXIS2_PLACEMENT_3D('',#125337,#60776,#60777);
#49487=AXIS2_PLACEMENT_3D('',#125340,#60779,#60780);
#49488=AXIS2_PLACEMENT_3D('',#125341,#60781,#60782);
#49489=AXIS2_PLACEMENT_3D('',#125343,#60783,#60784);
#49490=AXIS2_PLACEMENT_3D('',#125346,#60786,#60787);
#49491=AXIS2_PLACEMENT_3D('',#125347,#60788,#60789);
#49492=AXIS2_PLACEMENT_3D('',#125349,#60790,#60791);
#49493=AXIS2_PLACEMENT_3D('',#125352,#60793,#60794);
#49494=AXIS2_PLACEMENT_3D('',#125353,#60795,#60796);
#49495=AXIS2_PLACEMENT_3D('',#125355,#60797,#60798);
#49496=AXIS2_PLACEMENT_3D('',#125358,#60800,#60801);
#49497=AXIS2_PLACEMENT_3D('',#125359,#60802,#60803);
#49498=AXIS2_PLACEMENT_3D('',#125361,#60804,#60805);
#49499=AXIS2_PLACEMENT_3D('',#125364,#60807,#60808);
#49500=AXIS2_PLACEMENT_3D('',#125365,#60809,#60810);
#49501=AXIS2_PLACEMENT_3D('',#125367,#60811,#60812);
#49502=AXIS2_PLACEMENT_3D('',#125370,#60814,#60815);
#49503=AXIS2_PLACEMENT_3D('',#125371,#60816,#60817);
#49504=AXIS2_PLACEMENT_3D('',#125373,#60818,#60819);
#49505=AXIS2_PLACEMENT_3D('',#125376,#60821,#60822);
#49506=AXIS2_PLACEMENT_3D('',#125377,#60823,#60824);
#49507=AXIS2_PLACEMENT_3D('',#125379,#60825,#60826);
#49508=AXIS2_PLACEMENT_3D('',#125382,#60828,#60829);
#49509=AXIS2_PLACEMENT_3D('',#125383,#60830,#60831);
#49510=AXIS2_PLACEMENT_3D('',#125385,#60832,#60833);
#49511=AXIS2_PLACEMENT_3D('',#125388,#60835,#60836);
#49512=AXIS2_PLACEMENT_3D('',#125389,#60837,#60838);
#49513=AXIS2_PLACEMENT_3D('',#125391,#60839,#60840);
#49514=AXIS2_PLACEMENT_3D('',#125394,#60842,#60843);
#49515=AXIS2_PLACEMENT_3D('',#125395,#60844,#60845);
#49516=AXIS2_PLACEMENT_3D('',#125397,#60846,#60847);
#49517=AXIS2_PLACEMENT_3D('',#125400,#60849,#60850);
#49518=AXIS2_PLACEMENT_3D('',#125401,#60851,#60852);
#49519=AXIS2_PLACEMENT_3D('',#125403,#60853,#60854);
#49520=AXIS2_PLACEMENT_3D('',#125406,#60856,#60857);
#49521=AXIS2_PLACEMENT_3D('',#125407,#60858,#60859);
#49522=AXIS2_PLACEMENT_3D('',#125409,#60860,#60861);
#49523=AXIS2_PLACEMENT_3D('',#125412,#60863,#60864);
#49524=AXIS2_PLACEMENT_3D('',#125413,#60865,#60866);
#49525=AXIS2_PLACEMENT_3D('',#125415,#60867,#60868);
#49526=AXIS2_PLACEMENT_3D('',#125418,#60870,#60871);
#49527=AXIS2_PLACEMENT_3D('',#125419,#60872,#60873);
#49528=AXIS2_PLACEMENT_3D('',#125421,#60874,#60875);
#49529=AXIS2_PLACEMENT_3D('',#125424,#60877,#60878);
#49530=AXIS2_PLACEMENT_3D('',#125425,#60879,#60880);
#49531=AXIS2_PLACEMENT_3D('',#125427,#60881,#60882);
#49532=AXIS2_PLACEMENT_3D('',#125430,#60884,#60885);
#49533=AXIS2_PLACEMENT_3D('',#125431,#60886,#60887);
#49534=AXIS2_PLACEMENT_3D('',#125433,#60888,#60889);
#49535=AXIS2_PLACEMENT_3D('',#125436,#60891,#60892);
#49536=AXIS2_PLACEMENT_3D('',#125437,#60893,#60894);
#49537=AXIS2_PLACEMENT_3D('',#125439,#60895,#60896);
#49538=AXIS2_PLACEMENT_3D('',#125442,#60898,#60899);
#49539=AXIS2_PLACEMENT_3D('',#125443,#60900,#60901);
#49540=AXIS2_PLACEMENT_3D('',#125445,#60902,#60903);
#49541=AXIS2_PLACEMENT_3D('',#125448,#60905,#60906);
#49542=AXIS2_PLACEMENT_3D('',#125449,#60907,#60908);
#49543=AXIS2_PLACEMENT_3D('',#125451,#60909,#60910);
#49544=AXIS2_PLACEMENT_3D('',#125454,#60912,#60913);
#49545=AXIS2_PLACEMENT_3D('',#125455,#60914,#60915);
#49546=AXIS2_PLACEMENT_3D('',#125457,#60916,#60917);
#49547=AXIS2_PLACEMENT_3D('',#125460,#60919,#60920);
#49548=AXIS2_PLACEMENT_3D('',#125461,#60921,#60922);
#49549=AXIS2_PLACEMENT_3D('',#125463,#60923,#60924);
#49550=AXIS2_PLACEMENT_3D('',#125466,#60926,#60927);
#49551=AXIS2_PLACEMENT_3D('',#125467,#60928,#60929);
#49552=AXIS2_PLACEMENT_3D('',#125469,#60930,#60931);
#49553=AXIS2_PLACEMENT_3D('',#125472,#60933,#60934);
#49554=AXIS2_PLACEMENT_3D('',#125473,#60935,#60936);
#49555=AXIS2_PLACEMENT_3D('',#125475,#60937,#60938);
#49556=AXIS2_PLACEMENT_3D('',#125478,#60940,#60941);
#49557=AXIS2_PLACEMENT_3D('',#125479,#60942,#60943);
#49558=AXIS2_PLACEMENT_3D('',#125481,#60944,#60945);
#49559=AXIS2_PLACEMENT_3D('',#125484,#60947,#60948);
#49560=AXIS2_PLACEMENT_3D('',#125485,#60949,#60950);
#49561=AXIS2_PLACEMENT_3D('',#125487,#60951,#60952);
#49562=AXIS2_PLACEMENT_3D('',#125490,#60954,#60955);
#49563=AXIS2_PLACEMENT_3D('',#125491,#60956,#60957);
#49564=AXIS2_PLACEMENT_3D('',#125493,#60958,#60959);
#49565=AXIS2_PLACEMENT_3D('',#125496,#60961,#60962);
#49566=AXIS2_PLACEMENT_3D('',#125497,#60963,#60964);
#49567=AXIS2_PLACEMENT_3D('',#125499,#60965,#60966);
#49568=AXIS2_PLACEMENT_3D('',#125502,#60968,#60969);
#49569=AXIS2_PLACEMENT_3D('',#125503,#60970,#60971);
#49570=AXIS2_PLACEMENT_3D('',#125505,#60972,#60973);
#49571=AXIS2_PLACEMENT_3D('',#125508,#60975,#60976);
#49572=AXIS2_PLACEMENT_3D('',#125509,#60977,#60978);
#49573=AXIS2_PLACEMENT_3D('',#125511,#60979,#60980);
#49574=AXIS2_PLACEMENT_3D('',#125514,#60982,#60983);
#49575=AXIS2_PLACEMENT_3D('',#125515,#60984,#60985);
#49576=AXIS2_PLACEMENT_3D('',#125517,#60986,#60987);
#49577=AXIS2_PLACEMENT_3D('',#125520,#60989,#60990);
#49578=AXIS2_PLACEMENT_3D('',#125521,#60991,#60992);
#49579=AXIS2_PLACEMENT_3D('',#125523,#60993,#60994);
#49580=AXIS2_PLACEMENT_3D('',#125526,#60996,#60997);
#49581=AXIS2_PLACEMENT_3D('',#125527,#60998,#60999);
#49582=AXIS2_PLACEMENT_3D('',#125529,#61000,#61001);
#49583=AXIS2_PLACEMENT_3D('',#125532,#61003,#61004);
#49584=AXIS2_PLACEMENT_3D('',#125533,#61005,#61006);
#49585=AXIS2_PLACEMENT_3D('',#125535,#61007,#61008);
#49586=AXIS2_PLACEMENT_3D('',#125538,#61010,#61011);
#49587=AXIS2_PLACEMENT_3D('',#125539,#61012,#61013);
#49588=AXIS2_PLACEMENT_3D('',#125541,#61014,#61015);
#49589=AXIS2_PLACEMENT_3D('',#125544,#61017,#61018);
#49590=AXIS2_PLACEMENT_3D('',#125545,#61019,#61020);
#49591=AXIS2_PLACEMENT_3D('',#125547,#61021,#61022);
#49592=AXIS2_PLACEMENT_3D('',#125550,#61024,#61025);
#49593=AXIS2_PLACEMENT_3D('',#125551,#61026,#61027);
#49594=AXIS2_PLACEMENT_3D('',#125553,#61028,#61029);
#49595=AXIS2_PLACEMENT_3D('',#125556,#61031,#61032);
#49596=AXIS2_PLACEMENT_3D('',#125557,#61033,#61034);
#49597=AXIS2_PLACEMENT_3D('',#125559,#61035,#61036);
#49598=AXIS2_PLACEMENT_3D('',#125562,#61038,#61039);
#49599=AXIS2_PLACEMENT_3D('',#125563,#61040,#61041);
#49600=AXIS2_PLACEMENT_3D('',#125565,#61042,#61043);
#49601=AXIS2_PLACEMENT_3D('',#125568,#61045,#61046);
#49602=AXIS2_PLACEMENT_3D('',#125569,#61047,#61048);
#49603=AXIS2_PLACEMENT_3D('',#125571,#61049,#61050);
#49604=AXIS2_PLACEMENT_3D('',#125574,#61052,#61053);
#49605=AXIS2_PLACEMENT_3D('',#125575,#61054,#61055);
#49606=AXIS2_PLACEMENT_3D('',#125577,#61056,#61057);
#49607=AXIS2_PLACEMENT_3D('',#125580,#61059,#61060);
#49608=AXIS2_PLACEMENT_3D('',#125581,#61061,#61062);
#49609=AXIS2_PLACEMENT_3D('',#125583,#61063,#61064);
#49610=AXIS2_PLACEMENT_3D('',#125586,#61066,#61067);
#49611=AXIS2_PLACEMENT_3D('',#125587,#61068,#61069);
#49612=AXIS2_PLACEMENT_3D('',#125589,#61070,#61071);
#49613=AXIS2_PLACEMENT_3D('',#125592,#61073,#61074);
#49614=AXIS2_PLACEMENT_3D('',#125593,#61075,#61076);
#49615=AXIS2_PLACEMENT_3D('',#125595,#61077,#61078);
#49616=AXIS2_PLACEMENT_3D('',#125598,#61080,#61081);
#49617=AXIS2_PLACEMENT_3D('',#125599,#61082,#61083);
#49618=AXIS2_PLACEMENT_3D('',#125601,#61084,#61085);
#49619=AXIS2_PLACEMENT_3D('',#125604,#61087,#61088);
#49620=AXIS2_PLACEMENT_3D('',#125605,#61089,#61090);
#49621=AXIS2_PLACEMENT_3D('',#125607,#61091,#61092);
#49622=AXIS2_PLACEMENT_3D('',#125610,#61094,#61095);
#49623=AXIS2_PLACEMENT_3D('',#125611,#61096,#61097);
#49624=AXIS2_PLACEMENT_3D('',#125613,#61098,#61099);
#49625=AXIS2_PLACEMENT_3D('',#125616,#61101,#61102);
#49626=AXIS2_PLACEMENT_3D('',#125617,#61103,#61104);
#49627=AXIS2_PLACEMENT_3D('',#125619,#61105,#61106);
#49628=AXIS2_PLACEMENT_3D('',#125622,#61108,#61109);
#49629=AXIS2_PLACEMENT_3D('',#125623,#61110,#61111);
#49630=AXIS2_PLACEMENT_3D('',#125625,#61112,#61113);
#49631=AXIS2_PLACEMENT_3D('',#125628,#61115,#61116);
#49632=AXIS2_PLACEMENT_3D('',#125629,#61117,#61118);
#49633=AXIS2_PLACEMENT_3D('',#125631,#61119,#61120);
#49634=AXIS2_PLACEMENT_3D('',#125634,#61122,#61123);
#49635=AXIS2_PLACEMENT_3D('',#125635,#61124,#61125);
#49636=AXIS2_PLACEMENT_3D('',#125637,#61126,#61127);
#49637=AXIS2_PLACEMENT_3D('',#125640,#61129,#61130);
#49638=AXIS2_PLACEMENT_3D('',#125641,#61131,#61132);
#49639=AXIS2_PLACEMENT_3D('',#125643,#61133,#61134);
#49640=AXIS2_PLACEMENT_3D('',#125646,#61136,#61137);
#49641=AXIS2_PLACEMENT_3D('',#125647,#61138,#61139);
#49642=AXIS2_PLACEMENT_3D('',#125649,#61140,#61141);
#49643=AXIS2_PLACEMENT_3D('',#125652,#61143,#61144);
#49644=AXIS2_PLACEMENT_3D('',#125653,#61145,#61146);
#49645=AXIS2_PLACEMENT_3D('',#125655,#61147,#61148);
#49646=AXIS2_PLACEMENT_3D('',#125658,#61150,#61151);
#49647=AXIS2_PLACEMENT_3D('',#125659,#61152,#61153);
#49648=AXIS2_PLACEMENT_3D('',#125661,#61154,#61155);
#49649=AXIS2_PLACEMENT_3D('',#125664,#61157,#61158);
#49650=AXIS2_PLACEMENT_3D('',#125665,#61159,#61160);
#49651=AXIS2_PLACEMENT_3D('',#125667,#61161,#61162);
#49652=AXIS2_PLACEMENT_3D('',#125670,#61164,#61165);
#49653=AXIS2_PLACEMENT_3D('',#125671,#61166,#61167);
#49654=AXIS2_PLACEMENT_3D('',#125673,#61168,#61169);
#49655=AXIS2_PLACEMENT_3D('',#125676,#61171,#61172);
#49656=AXIS2_PLACEMENT_3D('',#125677,#61173,#61174);
#49657=AXIS2_PLACEMENT_3D('',#125679,#61175,#61176);
#49658=AXIS2_PLACEMENT_3D('',#125682,#61178,#61179);
#49659=AXIS2_PLACEMENT_3D('',#125683,#61180,#61181);
#49660=AXIS2_PLACEMENT_3D('',#125685,#61182,#61183);
#49661=AXIS2_PLACEMENT_3D('',#125688,#61185,#61186);
#49662=AXIS2_PLACEMENT_3D('',#125689,#61187,#61188);
#49663=AXIS2_PLACEMENT_3D('',#125691,#61189,#61190);
#49664=AXIS2_PLACEMENT_3D('',#125694,#61192,#61193);
#49665=AXIS2_PLACEMENT_3D('',#125695,#61194,#61195);
#49666=AXIS2_PLACEMENT_3D('',#125697,#61196,#61197);
#49667=AXIS2_PLACEMENT_3D('',#125700,#61199,#61200);
#49668=AXIS2_PLACEMENT_3D('',#125701,#61201,#61202);
#49669=AXIS2_PLACEMENT_3D('',#125703,#61203,#61204);
#49670=AXIS2_PLACEMENT_3D('',#125706,#61206,#61207);
#49671=AXIS2_PLACEMENT_3D('',#125707,#61208,#61209);
#49672=AXIS2_PLACEMENT_3D('',#125709,#61210,#61211);
#49673=AXIS2_PLACEMENT_3D('',#125712,#61213,#61214);
#49674=AXIS2_PLACEMENT_3D('',#125713,#61215,#61216);
#49675=AXIS2_PLACEMENT_3D('',#125715,#61217,#61218);
#49676=AXIS2_PLACEMENT_3D('',#125718,#61220,#61221);
#49677=AXIS2_PLACEMENT_3D('',#125719,#61222,#61223);
#49678=AXIS2_PLACEMENT_3D('',#125721,#61224,#61225);
#49679=AXIS2_PLACEMENT_3D('',#125724,#61227,#61228);
#49680=AXIS2_PLACEMENT_3D('',#125725,#61229,#61230);
#49681=AXIS2_PLACEMENT_3D('',#125727,#61231,#61232);
#49682=AXIS2_PLACEMENT_3D('',#125730,#61234,#61235);
#49683=AXIS2_PLACEMENT_3D('',#125731,#61236,#61237);
#49684=AXIS2_PLACEMENT_3D('',#125733,#61238,#61239);
#49685=AXIS2_PLACEMENT_3D('',#125736,#61241,#61242);
#49686=AXIS2_PLACEMENT_3D('',#125737,#61243,#61244);
#49687=AXIS2_PLACEMENT_3D('',#125739,#61245,#61246);
#49688=AXIS2_PLACEMENT_3D('',#125742,#61248,#61249);
#49689=AXIS2_PLACEMENT_3D('',#125743,#61250,#61251);
#49690=AXIS2_PLACEMENT_3D('',#125745,#61252,#61253);
#49691=AXIS2_PLACEMENT_3D('',#125748,#61255,#61256);
#49692=AXIS2_PLACEMENT_3D('',#125749,#61257,#61258);
#49693=AXIS2_PLACEMENT_3D('',#125751,#61259,#61260);
#49694=AXIS2_PLACEMENT_3D('',#125754,#61262,#61263);
#49695=AXIS2_PLACEMENT_3D('',#125755,#61264,#61265);
#49696=AXIS2_PLACEMENT_3D('',#125757,#61266,#61267);
#49697=AXIS2_PLACEMENT_3D('',#125760,#61269,#61270);
#49698=AXIS2_PLACEMENT_3D('',#125761,#61271,#61272);
#49699=AXIS2_PLACEMENT_3D('',#125763,#61273,#61274);
#49700=AXIS2_PLACEMENT_3D('',#125766,#61276,#61277);
#49701=AXIS2_PLACEMENT_3D('',#125767,#61278,#61279);
#49702=AXIS2_PLACEMENT_3D('',#125769,#61280,#61281);
#49703=AXIS2_PLACEMENT_3D('',#125772,#61283,#61284);
#49704=AXIS2_PLACEMENT_3D('',#125773,#61285,#61286);
#49705=AXIS2_PLACEMENT_3D('',#125775,#61287,#61288);
#49706=AXIS2_PLACEMENT_3D('',#125778,#61290,#61291);
#49707=AXIS2_PLACEMENT_3D('',#125779,#61292,#61293);
#49708=AXIS2_PLACEMENT_3D('',#125781,#61294,#61295);
#49709=AXIS2_PLACEMENT_3D('',#125784,#61297,#61298);
#49710=AXIS2_PLACEMENT_3D('',#125785,#61299,#61300);
#49711=AXIS2_PLACEMENT_3D('',#125787,#61301,#61302);
#49712=AXIS2_PLACEMENT_3D('',#125790,#61304,#61305);
#49713=AXIS2_PLACEMENT_3D('',#125791,#61306,#61307);
#49714=AXIS2_PLACEMENT_3D('',#125793,#61308,#61309);
#49715=AXIS2_PLACEMENT_3D('',#125796,#61311,#61312);
#49716=AXIS2_PLACEMENT_3D('',#125797,#61313,#61314);
#49717=AXIS2_PLACEMENT_3D('',#125799,#61315,#61316);
#49718=AXIS2_PLACEMENT_3D('',#125802,#61318,#61319);
#49719=AXIS2_PLACEMENT_3D('',#125803,#61320,#61321);
#49720=AXIS2_PLACEMENT_3D('',#125805,#61322,#61323);
#49721=AXIS2_PLACEMENT_3D('',#125808,#61325,#61326);
#49722=AXIS2_PLACEMENT_3D('',#125809,#61327,#61328);
#49723=AXIS2_PLACEMENT_3D('',#125811,#61329,#61330);
#49724=AXIS2_PLACEMENT_3D('',#125814,#61332,#61333);
#49725=AXIS2_PLACEMENT_3D('',#125815,#61334,#61335);
#49726=AXIS2_PLACEMENT_3D('',#125817,#61336,#61337);
#49727=AXIS2_PLACEMENT_3D('',#125820,#61339,#61340);
#49728=AXIS2_PLACEMENT_3D('',#125821,#61341,#61342);
#49729=AXIS2_PLACEMENT_3D('',#125823,#61343,#61344);
#49730=AXIS2_PLACEMENT_3D('',#125826,#61346,#61347);
#49731=AXIS2_PLACEMENT_3D('',#125827,#61348,#61349);
#49732=AXIS2_PLACEMENT_3D('',#125829,#61350,#61351);
#49733=AXIS2_PLACEMENT_3D('',#125832,#61353,#61354);
#49734=AXIS2_PLACEMENT_3D('',#125833,#61355,#61356);
#49735=AXIS2_PLACEMENT_3D('',#125835,#61357,#61358);
#49736=AXIS2_PLACEMENT_3D('',#125838,#61360,#61361);
#49737=AXIS2_PLACEMENT_3D('',#125839,#61362,#61363);
#49738=AXIS2_PLACEMENT_3D('',#125841,#61364,#61365);
#49739=AXIS2_PLACEMENT_3D('',#125844,#61367,#61368);
#49740=AXIS2_PLACEMENT_3D('',#125845,#61369,#61370);
#49741=AXIS2_PLACEMENT_3D('',#125847,#61371,#61372);
#49742=AXIS2_PLACEMENT_3D('',#125850,#61374,#61375);
#49743=AXIS2_PLACEMENT_3D('',#125851,#61376,#61377);
#49744=AXIS2_PLACEMENT_3D('',#125853,#61378,#61379);
#49745=AXIS2_PLACEMENT_3D('',#125856,#61381,#61382);
#49746=AXIS2_PLACEMENT_3D('',#125857,#61383,#61384);
#49747=AXIS2_PLACEMENT_3D('',#125859,#61385,#61386);
#49748=AXIS2_PLACEMENT_3D('',#125862,#61388,#61389);
#49749=AXIS2_PLACEMENT_3D('',#125863,#61390,#61391);
#49750=AXIS2_PLACEMENT_3D('',#125865,#61392,#61393);
#49751=AXIS2_PLACEMENT_3D('',#125868,#61395,#61396);
#49752=AXIS2_PLACEMENT_3D('',#125869,#61397,#61398);
#49753=AXIS2_PLACEMENT_3D('',#125871,#61399,#61400);
#49754=AXIS2_PLACEMENT_3D('',#125874,#61402,#61403);
#49755=AXIS2_PLACEMENT_3D('',#125875,#61404,#61405);
#49756=AXIS2_PLACEMENT_3D('',#125877,#61406,#61407);
#49757=AXIS2_PLACEMENT_3D('',#125880,#61409,#61410);
#49758=AXIS2_PLACEMENT_3D('',#125881,#61411,#61412);
#49759=AXIS2_PLACEMENT_3D('',#125883,#61413,#61414);
#49760=AXIS2_PLACEMENT_3D('',#125886,#61416,#61417);
#49761=AXIS2_PLACEMENT_3D('',#125887,#61418,#61419);
#49762=AXIS2_PLACEMENT_3D('',#125889,#61420,#61421);
#49763=AXIS2_PLACEMENT_3D('',#125892,#61423,#61424);
#49764=AXIS2_PLACEMENT_3D('',#125893,#61425,#61426);
#49765=AXIS2_PLACEMENT_3D('',#125895,#61427,#61428);
#49766=AXIS2_PLACEMENT_3D('',#125898,#61430,#61431);
#49767=AXIS2_PLACEMENT_3D('',#125899,#61432,#61433);
#49768=AXIS2_PLACEMENT_3D('',#125901,#61434,#61435);
#49769=AXIS2_PLACEMENT_3D('',#125904,#61437,#61438);
#49770=AXIS2_PLACEMENT_3D('',#125905,#61439,#61440);
#49771=AXIS2_PLACEMENT_3D('',#125907,#61441,#61442);
#49772=AXIS2_PLACEMENT_3D('',#125910,#61444,#61445);
#49773=AXIS2_PLACEMENT_3D('',#125911,#61446,#61447);
#49774=AXIS2_PLACEMENT_3D('',#125913,#61448,#61449);
#49775=AXIS2_PLACEMENT_3D('',#125916,#61451,#61452);
#49776=AXIS2_PLACEMENT_3D('',#125917,#61453,#61454);
#49777=AXIS2_PLACEMENT_3D('',#125919,#61455,#61456);
#49778=AXIS2_PLACEMENT_3D('',#125922,#61458,#61459);
#49779=AXIS2_PLACEMENT_3D('',#125923,#61460,#61461);
#49780=AXIS2_PLACEMENT_3D('',#125925,#61462,#61463);
#49781=AXIS2_PLACEMENT_3D('',#125928,#61465,#61466);
#49782=AXIS2_PLACEMENT_3D('',#125929,#61467,#61468);
#49783=AXIS2_PLACEMENT_3D('',#125931,#61469,#61470);
#49784=AXIS2_PLACEMENT_3D('',#125934,#61472,#61473);
#49785=AXIS2_PLACEMENT_3D('',#125935,#61474,#61475);
#49786=AXIS2_PLACEMENT_3D('',#125937,#61476,#61477);
#49787=AXIS2_PLACEMENT_3D('',#125940,#61479,#61480);
#49788=AXIS2_PLACEMENT_3D('',#125941,#61481,#61482);
#49789=AXIS2_PLACEMENT_3D('',#125943,#61483,#61484);
#49790=AXIS2_PLACEMENT_3D('',#125946,#61486,#61487);
#49791=AXIS2_PLACEMENT_3D('',#125947,#61488,#61489);
#49792=AXIS2_PLACEMENT_3D('',#125949,#61490,#61491);
#49793=AXIS2_PLACEMENT_3D('',#125952,#61493,#61494);
#49794=AXIS2_PLACEMENT_3D('',#125953,#61495,#61496);
#49795=AXIS2_PLACEMENT_3D('',#125955,#61497,#61498);
#49796=AXIS2_PLACEMENT_3D('',#125958,#61500,#61501);
#49797=AXIS2_PLACEMENT_3D('',#125959,#61502,#61503);
#49798=AXIS2_PLACEMENT_3D('',#125961,#61504,#61505);
#49799=AXIS2_PLACEMENT_3D('',#125964,#61507,#61508);
#49800=AXIS2_PLACEMENT_3D('',#125965,#61509,#61510);
#49801=AXIS2_PLACEMENT_3D('',#125967,#61511,#61512);
#49802=AXIS2_PLACEMENT_3D('',#125970,#61514,#61515);
#49803=AXIS2_PLACEMENT_3D('',#125971,#61516,#61517);
#49804=AXIS2_PLACEMENT_3D('',#125973,#61518,#61519);
#49805=AXIS2_PLACEMENT_3D('',#125976,#61521,#61522);
#49806=AXIS2_PLACEMENT_3D('',#125977,#61523,#61524);
#49807=AXIS2_PLACEMENT_3D('',#125979,#61525,#61526);
#49808=AXIS2_PLACEMENT_3D('',#125982,#61528,#61529);
#49809=AXIS2_PLACEMENT_3D('',#125983,#61530,#61531);
#49810=AXIS2_PLACEMENT_3D('',#125985,#61532,#61533);
#49811=AXIS2_PLACEMENT_3D('',#125988,#61535,#61536);
#49812=AXIS2_PLACEMENT_3D('',#125989,#61537,#61538);
#49813=AXIS2_PLACEMENT_3D('',#125991,#61539,#61540);
#49814=AXIS2_PLACEMENT_3D('',#125994,#61542,#61543);
#49815=AXIS2_PLACEMENT_3D('',#125995,#61544,#61545);
#49816=AXIS2_PLACEMENT_3D('',#125997,#61546,#61547);
#49817=AXIS2_PLACEMENT_3D('',#126000,#61549,#61550);
#49818=AXIS2_PLACEMENT_3D('',#126001,#61551,#61552);
#49819=AXIS2_PLACEMENT_3D('',#126003,#61553,#61554);
#49820=AXIS2_PLACEMENT_3D('',#126006,#61556,#61557);
#49821=AXIS2_PLACEMENT_3D('',#126007,#61558,#61559);
#49822=AXIS2_PLACEMENT_3D('',#126009,#61560,#61561);
#49823=AXIS2_PLACEMENT_3D('',#126012,#61563,#61564);
#49824=AXIS2_PLACEMENT_3D('',#126013,#61565,#61566);
#49825=AXIS2_PLACEMENT_3D('',#126015,#61567,#61568);
#49826=AXIS2_PLACEMENT_3D('',#126018,#61570,#61571);
#49827=AXIS2_PLACEMENT_3D('',#126019,#61572,#61573);
#49828=AXIS2_PLACEMENT_3D('',#126021,#61574,#61575);
#49829=AXIS2_PLACEMENT_3D('',#126024,#61577,#61578);
#49830=AXIS2_PLACEMENT_3D('',#126025,#61579,#61580);
#49831=AXIS2_PLACEMENT_3D('',#126027,#61581,#61582);
#49832=AXIS2_PLACEMENT_3D('',#126030,#61584,#61585);
#49833=AXIS2_PLACEMENT_3D('',#126031,#61586,#61587);
#49834=AXIS2_PLACEMENT_3D('',#126033,#61588,#61589);
#49835=AXIS2_PLACEMENT_3D('',#126036,#61591,#61592);
#49836=AXIS2_PLACEMENT_3D('',#126037,#61593,#61594);
#49837=AXIS2_PLACEMENT_3D('',#126039,#61595,#61596);
#49838=AXIS2_PLACEMENT_3D('',#126042,#61598,#61599);
#49839=AXIS2_PLACEMENT_3D('',#126043,#61600,#61601);
#49840=AXIS2_PLACEMENT_3D('',#126045,#61602,#61603);
#49841=AXIS2_PLACEMENT_3D('',#126048,#61605,#61606);
#49842=AXIS2_PLACEMENT_3D('',#126049,#61607,#61608);
#49843=AXIS2_PLACEMENT_3D('',#126051,#61609,#61610);
#49844=AXIS2_PLACEMENT_3D('',#126054,#61612,#61613);
#49845=AXIS2_PLACEMENT_3D('',#126055,#61614,#61615);
#49846=AXIS2_PLACEMENT_3D('',#126057,#61616,#61617);
#49847=AXIS2_PLACEMENT_3D('',#126060,#61619,#61620);
#49848=AXIS2_PLACEMENT_3D('',#126061,#61621,#61622);
#49849=AXIS2_PLACEMENT_3D('',#126063,#61623,#61624);
#49850=AXIS2_PLACEMENT_3D('',#126066,#61626,#61627);
#49851=AXIS2_PLACEMENT_3D('',#126067,#61628,#61629);
#49852=AXIS2_PLACEMENT_3D('',#126069,#61630,#61631);
#49853=AXIS2_PLACEMENT_3D('',#126072,#61633,#61634);
#49854=AXIS2_PLACEMENT_3D('',#126073,#61635,#61636);
#49855=AXIS2_PLACEMENT_3D('',#126075,#61637,#61638);
#49856=AXIS2_PLACEMENT_3D('',#126078,#61640,#61641);
#49857=AXIS2_PLACEMENT_3D('',#126079,#61642,#61643);
#49858=AXIS2_PLACEMENT_3D('',#126081,#61644,#61645);
#49859=AXIS2_PLACEMENT_3D('',#126084,#61647,#61648);
#49860=AXIS2_PLACEMENT_3D('',#126085,#61649,#61650);
#49861=AXIS2_PLACEMENT_3D('',#126087,#61651,#61652);
#49862=AXIS2_PLACEMENT_3D('',#126090,#61654,#61655);
#49863=AXIS2_PLACEMENT_3D('',#126091,#61656,#61657);
#49864=AXIS2_PLACEMENT_3D('',#126093,#61658,#61659);
#49865=AXIS2_PLACEMENT_3D('',#126096,#61661,#61662);
#49866=AXIS2_PLACEMENT_3D('',#126097,#61663,#61664);
#49867=AXIS2_PLACEMENT_3D('',#126099,#61665,#61666);
#49868=AXIS2_PLACEMENT_3D('',#126102,#61668,#61669);
#49869=AXIS2_PLACEMENT_3D('',#126103,#61670,#61671);
#49870=AXIS2_PLACEMENT_3D('',#126105,#61672,#61673);
#49871=AXIS2_PLACEMENT_3D('',#126108,#61675,#61676);
#49872=AXIS2_PLACEMENT_3D('',#126109,#61677,#61678);
#49873=AXIS2_PLACEMENT_3D('',#126111,#61679,#61680);
#49874=AXIS2_PLACEMENT_3D('',#126114,#61682,#61683);
#49875=AXIS2_PLACEMENT_3D('',#126115,#61684,#61685);
#49876=AXIS2_PLACEMENT_3D('',#126117,#61686,#61687);
#49877=AXIS2_PLACEMENT_3D('',#126120,#61689,#61690);
#49878=AXIS2_PLACEMENT_3D('',#126121,#61691,#61692);
#49879=AXIS2_PLACEMENT_3D('',#126123,#61693,#61694);
#49880=AXIS2_PLACEMENT_3D('',#126126,#61696,#61697);
#49881=AXIS2_PLACEMENT_3D('',#126127,#61698,#61699);
#49882=AXIS2_PLACEMENT_3D('',#126129,#61700,#61701);
#49883=AXIS2_PLACEMENT_3D('',#126132,#61703,#61704);
#49884=AXIS2_PLACEMENT_3D('',#126133,#61705,#61706);
#49885=AXIS2_PLACEMENT_3D('',#126135,#61707,#61708);
#49886=AXIS2_PLACEMENT_3D('',#126138,#61710,#61711);
#49887=AXIS2_PLACEMENT_3D('',#126139,#61712,#61713);
#49888=AXIS2_PLACEMENT_3D('',#126141,#61714,#61715);
#49889=AXIS2_PLACEMENT_3D('',#126144,#61717,#61718);
#49890=AXIS2_PLACEMENT_3D('',#126145,#61719,#61720);
#49891=AXIS2_PLACEMENT_3D('',#126147,#61721,#61722);
#49892=AXIS2_PLACEMENT_3D('',#126150,#61724,#61725);
#49893=AXIS2_PLACEMENT_3D('',#126151,#61726,#61727);
#49894=AXIS2_PLACEMENT_3D('',#126153,#61728,#61729);
#49895=AXIS2_PLACEMENT_3D('',#126156,#61731,#61732);
#49896=AXIS2_PLACEMENT_3D('',#126157,#61733,#61734);
#49897=AXIS2_PLACEMENT_3D('',#126159,#61735,#61736);
#49898=AXIS2_PLACEMENT_3D('',#126162,#61738,#61739);
#49899=AXIS2_PLACEMENT_3D('',#126163,#61740,#61741);
#49900=AXIS2_PLACEMENT_3D('',#126165,#61742,#61743);
#49901=AXIS2_PLACEMENT_3D('',#126168,#61745,#61746);
#49902=AXIS2_PLACEMENT_3D('',#126169,#61747,#61748);
#49903=AXIS2_PLACEMENT_3D('',#126171,#61749,#61750);
#49904=AXIS2_PLACEMENT_3D('',#126174,#61752,#61753);
#49905=AXIS2_PLACEMENT_3D('',#126175,#61754,#61755);
#49906=AXIS2_PLACEMENT_3D('',#126177,#61756,#61757);
#49907=AXIS2_PLACEMENT_3D('',#126180,#61759,#61760);
#49908=AXIS2_PLACEMENT_3D('',#126181,#61761,#61762);
#49909=AXIS2_PLACEMENT_3D('',#126183,#61763,#61764);
#49910=AXIS2_PLACEMENT_3D('',#126186,#61766,#61767);
#49911=AXIS2_PLACEMENT_3D('',#126187,#61768,#61769);
#49912=AXIS2_PLACEMENT_3D('',#126189,#61770,#61771);
#49913=AXIS2_PLACEMENT_3D('',#126192,#61773,#61774);
#49914=AXIS2_PLACEMENT_3D('',#126193,#61775,#61776);
#49915=AXIS2_PLACEMENT_3D('',#126195,#61777,#61778);
#49916=AXIS2_PLACEMENT_3D('',#126198,#61780,#61781);
#49917=AXIS2_PLACEMENT_3D('',#126199,#61782,#61783);
#49918=AXIS2_PLACEMENT_3D('',#126201,#61784,#61785);
#49919=AXIS2_PLACEMENT_3D('',#126204,#61787,#61788);
#49920=AXIS2_PLACEMENT_3D('',#126205,#61789,#61790);
#49921=AXIS2_PLACEMENT_3D('',#126207,#61791,#61792);
#49922=AXIS2_PLACEMENT_3D('',#126210,#61794,#61795);
#49923=AXIS2_PLACEMENT_3D('',#126211,#61796,#61797);
#49924=AXIS2_PLACEMENT_3D('',#126213,#61798,#61799);
#49925=AXIS2_PLACEMENT_3D('',#126216,#61801,#61802);
#49926=AXIS2_PLACEMENT_3D('',#126217,#61803,#61804);
#49927=AXIS2_PLACEMENT_3D('',#126219,#61805,#61806);
#49928=AXIS2_PLACEMENT_3D('',#126222,#61808,#61809);
#49929=AXIS2_PLACEMENT_3D('',#126223,#61810,#61811);
#49930=AXIS2_PLACEMENT_3D('',#126225,#61812,#61813);
#49931=AXIS2_PLACEMENT_3D('',#126228,#61815,#61816);
#49932=AXIS2_PLACEMENT_3D('',#126229,#61817,#61818);
#49933=AXIS2_PLACEMENT_3D('',#126231,#61819,#61820);
#49934=AXIS2_PLACEMENT_3D('',#126234,#61822,#61823);
#49935=AXIS2_PLACEMENT_3D('',#126235,#61824,#61825);
#49936=AXIS2_PLACEMENT_3D('',#126237,#61826,#61827);
#49937=AXIS2_PLACEMENT_3D('',#126240,#61829,#61830);
#49938=AXIS2_PLACEMENT_3D('',#126241,#61831,#61832);
#49939=AXIS2_PLACEMENT_3D('',#126243,#61833,#61834);
#49940=AXIS2_PLACEMENT_3D('',#126246,#61836,#61837);
#49941=AXIS2_PLACEMENT_3D('',#126247,#61838,#61839);
#49942=AXIS2_PLACEMENT_3D('',#126249,#61840,#61841);
#49943=AXIS2_PLACEMENT_3D('',#126252,#61843,#61844);
#49944=AXIS2_PLACEMENT_3D('',#126253,#61845,#61846);
#49945=AXIS2_PLACEMENT_3D('',#126255,#61847,#61848);
#49946=AXIS2_PLACEMENT_3D('',#126258,#61850,#61851);
#49947=AXIS2_PLACEMENT_3D('',#126259,#61852,#61853);
#49948=AXIS2_PLACEMENT_3D('',#126261,#61854,#61855);
#49949=AXIS2_PLACEMENT_3D('',#126264,#61857,#61858);
#49950=AXIS2_PLACEMENT_3D('',#126265,#61859,#61860);
#49951=AXIS2_PLACEMENT_3D('',#126267,#61861,#61862);
#49952=AXIS2_PLACEMENT_3D('',#126270,#61864,#61865);
#49953=AXIS2_PLACEMENT_3D('',#126271,#61866,#61867);
#49954=AXIS2_PLACEMENT_3D('',#126273,#61868,#61869);
#49955=AXIS2_PLACEMENT_3D('',#126276,#61871,#61872);
#49956=AXIS2_PLACEMENT_3D('',#126277,#61873,#61874);
#49957=AXIS2_PLACEMENT_3D('',#126279,#61875,#61876);
#49958=AXIS2_PLACEMENT_3D('',#126282,#61878,#61879);
#49959=AXIS2_PLACEMENT_3D('',#126283,#61880,#61881);
#49960=AXIS2_PLACEMENT_3D('',#126285,#61882,#61883);
#49961=AXIS2_PLACEMENT_3D('',#126288,#61885,#61886);
#49962=AXIS2_PLACEMENT_3D('',#126289,#61887,#61888);
#49963=AXIS2_PLACEMENT_3D('',#126291,#61889,#61890);
#49964=AXIS2_PLACEMENT_3D('',#126294,#61892,#61893);
#49965=AXIS2_PLACEMENT_3D('',#126295,#61894,#61895);
#49966=AXIS2_PLACEMENT_3D('',#126297,#61896,#61897);
#49967=AXIS2_PLACEMENT_3D('',#126300,#61899,#61900);
#49968=AXIS2_PLACEMENT_3D('',#126301,#61901,#61902);
#49969=AXIS2_PLACEMENT_3D('',#126303,#61903,#61904);
#49970=AXIS2_PLACEMENT_3D('',#126306,#61906,#61907);
#49971=AXIS2_PLACEMENT_3D('',#126307,#61908,#61909);
#49972=AXIS2_PLACEMENT_3D('',#126309,#61910,#61911);
#49973=AXIS2_PLACEMENT_3D('',#126312,#61913,#61914);
#49974=AXIS2_PLACEMENT_3D('',#126313,#61915,#61916);
#49975=AXIS2_PLACEMENT_3D('',#126315,#61917,#61918);
#49976=AXIS2_PLACEMENT_3D('',#126318,#61920,#61921);
#49977=AXIS2_PLACEMENT_3D('',#126319,#61922,#61923);
#49978=AXIS2_PLACEMENT_3D('',#126321,#61924,#61925);
#49979=AXIS2_PLACEMENT_3D('',#126324,#61927,#61928);
#49980=AXIS2_PLACEMENT_3D('',#126325,#61929,#61930);
#49981=AXIS2_PLACEMENT_3D('',#126327,#61931,#61932);
#49982=AXIS2_PLACEMENT_3D('',#126330,#61934,#61935);
#49983=AXIS2_PLACEMENT_3D('',#126331,#61936,#61937);
#49984=AXIS2_PLACEMENT_3D('',#126333,#61938,#61939);
#49985=AXIS2_PLACEMENT_3D('',#126336,#61941,#61942);
#49986=AXIS2_PLACEMENT_3D('',#126337,#61943,#61944);
#49987=AXIS2_PLACEMENT_3D('',#126339,#61945,#61946);
#49988=AXIS2_PLACEMENT_3D('',#126342,#61948,#61949);
#49989=AXIS2_PLACEMENT_3D('',#126343,#61950,#61951);
#49990=AXIS2_PLACEMENT_3D('',#126345,#61952,#61953);
#49991=AXIS2_PLACEMENT_3D('',#126348,#61955,#61956);
#49992=AXIS2_PLACEMENT_3D('',#126349,#61957,#61958);
#49993=AXIS2_PLACEMENT_3D('',#126351,#61959,#61960);
#49994=AXIS2_PLACEMENT_3D('',#126354,#61962,#61963);
#49995=AXIS2_PLACEMENT_3D('',#126355,#61964,#61965);
#49996=AXIS2_PLACEMENT_3D('',#126357,#61966,#61967);
#49997=AXIS2_PLACEMENT_3D('',#126360,#61969,#61970);
#49998=AXIS2_PLACEMENT_3D('',#126361,#61971,#61972);
#49999=AXIS2_PLACEMENT_3D('',#126363,#61973,#61974);
#50000=AXIS2_PLACEMENT_3D('',#126366,#61976,#61977);
#50001=AXIS2_PLACEMENT_3D('',#126367,#61978,#61979);
#50002=AXIS2_PLACEMENT_3D('',#126369,#61980,#61981);
#50003=AXIS2_PLACEMENT_3D('',#126372,#61983,#61984);
#50004=AXIS2_PLACEMENT_3D('',#126373,#61985,#61986);
#50005=AXIS2_PLACEMENT_3D('',#126375,#61987,#61988);
#50006=AXIS2_PLACEMENT_3D('',#126378,#61990,#61991);
#50007=AXIS2_PLACEMENT_3D('',#126379,#61992,#61993);
#50008=AXIS2_PLACEMENT_3D('',#126381,#61994,#61995);
#50009=AXIS2_PLACEMENT_3D('',#126384,#61997,#61998);
#50010=AXIS2_PLACEMENT_3D('',#126385,#61999,#62000);
#50011=AXIS2_PLACEMENT_3D('',#126387,#62001,#62002);
#50012=AXIS2_PLACEMENT_3D('',#126390,#62004,#62005);
#50013=AXIS2_PLACEMENT_3D('',#126391,#62006,#62007);
#50014=AXIS2_PLACEMENT_3D('',#126393,#62008,#62009);
#50015=AXIS2_PLACEMENT_3D('',#126396,#62011,#62012);
#50016=AXIS2_PLACEMENT_3D('',#126397,#62013,#62014);
#50017=AXIS2_PLACEMENT_3D('',#126399,#62015,#62016);
#50018=AXIS2_PLACEMENT_3D('',#126402,#62018,#62019);
#50019=AXIS2_PLACEMENT_3D('',#126403,#62020,#62021);
#50020=AXIS2_PLACEMENT_3D('',#126405,#62022,#62023);
#50021=AXIS2_PLACEMENT_3D('',#126408,#62025,#62026);
#50022=AXIS2_PLACEMENT_3D('',#126409,#62027,#62028);
#50023=AXIS2_PLACEMENT_3D('',#126411,#62029,#62030);
#50024=AXIS2_PLACEMENT_3D('',#126414,#62032,#62033);
#50025=AXIS2_PLACEMENT_3D('',#126415,#62034,#62035);
#50026=AXIS2_PLACEMENT_3D('',#126417,#62036,#62037);
#50027=AXIS2_PLACEMENT_3D('',#126420,#62039,#62040);
#50028=AXIS2_PLACEMENT_3D('',#126421,#62041,#62042);
#50029=AXIS2_PLACEMENT_3D('',#126423,#62043,#62044);
#50030=AXIS2_PLACEMENT_3D('',#126426,#62046,#62047);
#50031=AXIS2_PLACEMENT_3D('',#126427,#62048,#62049);
#50032=AXIS2_PLACEMENT_3D('',#126429,#62050,#62051);
#50033=AXIS2_PLACEMENT_3D('',#126432,#62053,#62054);
#50034=AXIS2_PLACEMENT_3D('',#126433,#62055,#62056);
#50035=AXIS2_PLACEMENT_3D('',#126435,#62057,#62058);
#50036=AXIS2_PLACEMENT_3D('',#126438,#62060,#62061);
#50037=AXIS2_PLACEMENT_3D('',#126439,#62062,#62063);
#50038=AXIS2_PLACEMENT_3D('',#126441,#62064,#62065);
#50039=AXIS2_PLACEMENT_3D('',#126444,#62067,#62068);
#50040=AXIS2_PLACEMENT_3D('',#126445,#62069,#62070);
#50041=AXIS2_PLACEMENT_3D('',#126447,#62071,#62072);
#50042=AXIS2_PLACEMENT_3D('',#126450,#62074,#62075);
#50043=AXIS2_PLACEMENT_3D('',#126451,#62076,#62077);
#50044=AXIS2_PLACEMENT_3D('',#126453,#62078,#62079);
#50045=AXIS2_PLACEMENT_3D('',#126456,#62081,#62082);
#50046=AXIS2_PLACEMENT_3D('',#126457,#62083,#62084);
#50047=AXIS2_PLACEMENT_3D('',#126459,#62085,#62086);
#50048=AXIS2_PLACEMENT_3D('',#126462,#62088,#62089);
#50049=AXIS2_PLACEMENT_3D('',#126463,#62090,#62091);
#50050=AXIS2_PLACEMENT_3D('',#126465,#62092,#62093);
#50051=AXIS2_PLACEMENT_3D('',#126468,#62095,#62096);
#50052=AXIS2_PLACEMENT_3D('',#126469,#62097,#62098);
#50053=AXIS2_PLACEMENT_3D('',#126471,#62099,#62100);
#50054=AXIS2_PLACEMENT_3D('',#126474,#62102,#62103);
#50055=AXIS2_PLACEMENT_3D('',#126475,#62104,#62105);
#50056=AXIS2_PLACEMENT_3D('',#126477,#62106,#62107);
#50057=AXIS2_PLACEMENT_3D('',#126480,#62109,#62110);
#50058=AXIS2_PLACEMENT_3D('',#126481,#62111,#62112);
#50059=AXIS2_PLACEMENT_3D('',#126483,#62113,#62114);
#50060=AXIS2_PLACEMENT_3D('',#126486,#62116,#62117);
#50061=AXIS2_PLACEMENT_3D('',#126487,#62118,#62119);
#50062=AXIS2_PLACEMENT_3D('',#126489,#62120,#62121);
#50063=AXIS2_PLACEMENT_3D('',#126492,#62123,#62124);
#50064=AXIS2_PLACEMENT_3D('',#126493,#62125,#62126);
#50065=AXIS2_PLACEMENT_3D('',#126495,#62127,#62128);
#50066=AXIS2_PLACEMENT_3D('',#126498,#62130,#62131);
#50067=AXIS2_PLACEMENT_3D('',#126499,#62132,#62133);
#50068=AXIS2_PLACEMENT_3D('',#126501,#62134,#62135);
#50069=AXIS2_PLACEMENT_3D('',#126504,#62137,#62138);
#50070=AXIS2_PLACEMENT_3D('',#126505,#62139,#62140);
#50071=AXIS2_PLACEMENT_3D('',#126507,#62141,#62142);
#50072=AXIS2_PLACEMENT_3D('',#126510,#62144,#62145);
#50073=AXIS2_PLACEMENT_3D('',#126511,#62146,#62147);
#50074=AXIS2_PLACEMENT_3D('',#126513,#62148,#62149);
#50075=AXIS2_PLACEMENT_3D('',#126516,#62151,#62152);
#50076=AXIS2_PLACEMENT_3D('',#126517,#62153,#62154);
#50077=AXIS2_PLACEMENT_3D('',#126519,#62155,#62156);
#50078=AXIS2_PLACEMENT_3D('',#126522,#62158,#62159);
#50079=AXIS2_PLACEMENT_3D('',#126523,#62160,#62161);
#50080=AXIS2_PLACEMENT_3D('',#126525,#62162,#62163);
#50081=AXIS2_PLACEMENT_3D('',#126528,#62165,#62166);
#50082=AXIS2_PLACEMENT_3D('',#126529,#62167,#62168);
#50083=AXIS2_PLACEMENT_3D('',#126531,#62169,#62170);
#50084=AXIS2_PLACEMENT_3D('',#126534,#62172,#62173);
#50085=AXIS2_PLACEMENT_3D('',#126535,#62174,#62175);
#50086=AXIS2_PLACEMENT_3D('',#126537,#62176,#62177);
#50087=AXIS2_PLACEMENT_3D('',#126540,#62179,#62180);
#50088=AXIS2_PLACEMENT_3D('',#126541,#62181,#62182);
#50089=AXIS2_PLACEMENT_3D('',#126543,#62183,#62184);
#50090=AXIS2_PLACEMENT_3D('',#126546,#62186,#62187);
#50091=AXIS2_PLACEMENT_3D('',#126547,#62188,#62189);
#50092=AXIS2_PLACEMENT_3D('',#126549,#62190,#62191);
#50093=AXIS2_PLACEMENT_3D('',#126552,#62193,#62194);
#50094=AXIS2_PLACEMENT_3D('',#126553,#62195,#62196);
#50095=AXIS2_PLACEMENT_3D('',#126555,#62197,#62198);
#50096=AXIS2_PLACEMENT_3D('',#126558,#62200,#62201);
#50097=AXIS2_PLACEMENT_3D('',#126559,#62202,#62203);
#50098=AXIS2_PLACEMENT_3D('',#126561,#62204,#62205);
#50099=AXIS2_PLACEMENT_3D('',#126564,#62207,#62208);
#50100=AXIS2_PLACEMENT_3D('',#126565,#62209,#62210);
#50101=AXIS2_PLACEMENT_3D('',#126567,#62211,#62212);
#50102=AXIS2_PLACEMENT_3D('',#126570,#62214,#62215);
#50103=AXIS2_PLACEMENT_3D('',#126571,#62216,#62217);
#50104=AXIS2_PLACEMENT_3D('',#126573,#62218,#62219);
#50105=AXIS2_PLACEMENT_3D('',#126576,#62221,#62222);
#50106=AXIS2_PLACEMENT_3D('',#126577,#62223,#62224);
#50107=AXIS2_PLACEMENT_3D('',#126579,#62225,#62226);
#50108=AXIS2_PLACEMENT_3D('',#126582,#62228,#62229);
#50109=AXIS2_PLACEMENT_3D('',#126583,#62230,#62231);
#50110=AXIS2_PLACEMENT_3D('',#126585,#62232,#62233);
#50111=AXIS2_PLACEMENT_3D('',#126588,#62235,#62236);
#50112=AXIS2_PLACEMENT_3D('',#126589,#62237,#62238);
#50113=AXIS2_PLACEMENT_3D('',#126591,#62239,#62240);
#50114=AXIS2_PLACEMENT_3D('',#126594,#62242,#62243);
#50115=AXIS2_PLACEMENT_3D('',#126595,#62244,#62245);
#50116=AXIS2_PLACEMENT_3D('',#126597,#62246,#62247);
#50117=AXIS2_PLACEMENT_3D('',#126600,#62249,#62250);
#50118=AXIS2_PLACEMENT_3D('',#126601,#62251,#62252);
#50119=AXIS2_PLACEMENT_3D('',#126603,#62253,#62254);
#50120=AXIS2_PLACEMENT_3D('',#126606,#62256,#62257);
#50121=AXIS2_PLACEMENT_3D('',#126607,#62258,#62259);
#50122=AXIS2_PLACEMENT_3D('',#126609,#62260,#62261);
#50123=AXIS2_PLACEMENT_3D('',#126612,#62263,#62264);
#50124=AXIS2_PLACEMENT_3D('',#126613,#62265,#62266);
#50125=AXIS2_PLACEMENT_3D('',#126615,#62267,#62268);
#50126=AXIS2_PLACEMENT_3D('',#126618,#62270,#62271);
#50127=AXIS2_PLACEMENT_3D('',#126619,#62272,#62273);
#50128=AXIS2_PLACEMENT_3D('',#126621,#62274,#62275);
#50129=AXIS2_PLACEMENT_3D('',#126624,#62277,#62278);
#50130=AXIS2_PLACEMENT_3D('',#126625,#62279,#62280);
#50131=AXIS2_PLACEMENT_3D('',#126627,#62281,#62282);
#50132=AXIS2_PLACEMENT_3D('',#126630,#62284,#62285);
#50133=AXIS2_PLACEMENT_3D('',#126631,#62286,#62287);
#50134=AXIS2_PLACEMENT_3D('',#126633,#62288,#62289);
#50135=AXIS2_PLACEMENT_3D('',#126636,#62291,#62292);
#50136=AXIS2_PLACEMENT_3D('',#126637,#62293,#62294);
#50137=AXIS2_PLACEMENT_3D('',#126639,#62295,#62296);
#50138=AXIS2_PLACEMENT_3D('',#126642,#62298,#62299);
#50139=AXIS2_PLACEMENT_3D('',#126643,#62300,#62301);
#50140=AXIS2_PLACEMENT_3D('',#126645,#62302,#62303);
#50141=AXIS2_PLACEMENT_3D('',#126648,#62305,#62306);
#50142=AXIS2_PLACEMENT_3D('',#126649,#62307,#62308);
#50143=AXIS2_PLACEMENT_3D('',#126651,#62309,#62310);
#50144=AXIS2_PLACEMENT_3D('',#126654,#62312,#62313);
#50145=AXIS2_PLACEMENT_3D('',#126655,#62314,#62315);
#50146=AXIS2_PLACEMENT_3D('',#126657,#62316,#62317);
#50147=AXIS2_PLACEMENT_3D('',#126660,#62319,#62320);
#50148=AXIS2_PLACEMENT_3D('',#126661,#62321,#62322);
#50149=AXIS2_PLACEMENT_3D('',#126663,#62323,#62324);
#50150=AXIS2_PLACEMENT_3D('',#126666,#62326,#62327);
#50151=AXIS2_PLACEMENT_3D('',#126667,#62328,#62329);
#50152=AXIS2_PLACEMENT_3D('',#126669,#62330,#62331);
#50153=AXIS2_PLACEMENT_3D('',#126672,#62333,#62334);
#50154=AXIS2_PLACEMENT_3D('',#126673,#62335,#62336);
#50155=AXIS2_PLACEMENT_3D('',#126675,#62337,#62338);
#50156=AXIS2_PLACEMENT_3D('',#126678,#62340,#62341);
#50157=AXIS2_PLACEMENT_3D('',#126679,#62342,#62343);
#50158=AXIS2_PLACEMENT_3D('',#126681,#62344,#62345);
#50159=AXIS2_PLACEMENT_3D('',#126684,#62347,#62348);
#50160=AXIS2_PLACEMENT_3D('',#126685,#62349,#62350);
#50161=AXIS2_PLACEMENT_3D('',#126687,#62351,#62352);
#50162=AXIS2_PLACEMENT_3D('',#126690,#62354,#62355);
#50163=AXIS2_PLACEMENT_3D('',#126691,#62356,#62357);
#50164=AXIS2_PLACEMENT_3D('',#126693,#62358,#62359);
#50165=AXIS2_PLACEMENT_3D('',#126696,#62361,#62362);
#50166=AXIS2_PLACEMENT_3D('',#126697,#62363,#62364);
#50167=AXIS2_PLACEMENT_3D('',#126699,#62365,#62366);
#50168=AXIS2_PLACEMENT_3D('',#126702,#62368,#62369);
#50169=AXIS2_PLACEMENT_3D('',#126703,#62370,#62371);
#50170=AXIS2_PLACEMENT_3D('',#126705,#62372,#62373);
#50171=AXIS2_PLACEMENT_3D('',#126708,#62375,#62376);
#50172=AXIS2_PLACEMENT_3D('',#126709,#62377,#62378);
#50173=AXIS2_PLACEMENT_3D('',#126711,#62379,#62380);
#50174=AXIS2_PLACEMENT_3D('',#126714,#62382,#62383);
#50175=AXIS2_PLACEMENT_3D('',#126715,#62384,#62385);
#50176=AXIS2_PLACEMENT_3D('',#126717,#62386,#62387);
#50177=AXIS2_PLACEMENT_3D('',#126720,#62389,#62390);
#50178=AXIS2_PLACEMENT_3D('',#126721,#62391,#62392);
#50179=AXIS2_PLACEMENT_3D('',#126723,#62393,#62394);
#50180=AXIS2_PLACEMENT_3D('',#126726,#62396,#62397);
#50181=AXIS2_PLACEMENT_3D('',#126727,#62398,#62399);
#50182=AXIS2_PLACEMENT_3D('',#126729,#62400,#62401);
#50183=AXIS2_PLACEMENT_3D('',#126732,#62403,#62404);
#50184=AXIS2_PLACEMENT_3D('',#126733,#62405,#62406);
#50185=AXIS2_PLACEMENT_3D('',#126735,#62407,#62408);
#50186=AXIS2_PLACEMENT_3D('',#126738,#62410,#62411);
#50187=AXIS2_PLACEMENT_3D('',#126739,#62412,#62413);
#50188=AXIS2_PLACEMENT_3D('',#126741,#62414,#62415);
#50189=AXIS2_PLACEMENT_3D('',#126744,#62417,#62418);
#50190=AXIS2_PLACEMENT_3D('',#126745,#62419,#62420);
#50191=AXIS2_PLACEMENT_3D('',#126747,#62421,#62422);
#50192=AXIS2_PLACEMENT_3D('',#126750,#62424,#62425);
#50193=AXIS2_PLACEMENT_3D('',#126751,#62426,#62427);
#50194=AXIS2_PLACEMENT_3D('',#126753,#62428,#62429);
#50195=AXIS2_PLACEMENT_3D('',#126756,#62431,#62432);
#50196=AXIS2_PLACEMENT_3D('',#126757,#62433,#62434);
#50197=AXIS2_PLACEMENT_3D('',#126759,#62435,#62436);
#50198=AXIS2_PLACEMENT_3D('',#126762,#62438,#62439);
#50199=AXIS2_PLACEMENT_3D('',#126763,#62440,#62441);
#50200=AXIS2_PLACEMENT_3D('',#126765,#62442,#62443);
#50201=AXIS2_PLACEMENT_3D('',#126768,#62445,#62446);
#50202=AXIS2_PLACEMENT_3D('',#126769,#62447,#62448);
#50203=AXIS2_PLACEMENT_3D('',#126771,#62449,#62450);
#50204=AXIS2_PLACEMENT_3D('',#126774,#62452,#62453);
#50205=AXIS2_PLACEMENT_3D('',#126775,#62454,#62455);
#50206=AXIS2_PLACEMENT_3D('',#126777,#62456,#62457);
#50207=AXIS2_PLACEMENT_3D('',#126780,#62459,#62460);
#50208=AXIS2_PLACEMENT_3D('',#126781,#62461,#62462);
#50209=AXIS2_PLACEMENT_3D('',#126783,#62463,#62464);
#50210=AXIS2_PLACEMENT_3D('',#126786,#62466,#62467);
#50211=AXIS2_PLACEMENT_3D('',#126787,#62468,#62469);
#50212=AXIS2_PLACEMENT_3D('',#126789,#62470,#62471);
#50213=AXIS2_PLACEMENT_3D('',#126792,#62473,#62474);
#50214=AXIS2_PLACEMENT_3D('',#126793,#62475,#62476);
#50215=AXIS2_PLACEMENT_3D('',#126795,#62477,#62478);
#50216=AXIS2_PLACEMENT_3D('',#126798,#62480,#62481);
#50217=AXIS2_PLACEMENT_3D('',#126799,#62482,#62483);
#50218=AXIS2_PLACEMENT_3D('',#126801,#62484,#62485);
#50219=AXIS2_PLACEMENT_3D('',#126804,#62487,#62488);
#50220=AXIS2_PLACEMENT_3D('',#126805,#62489,#62490);
#50221=AXIS2_PLACEMENT_3D('',#126807,#62491,#62492);
#50222=AXIS2_PLACEMENT_3D('',#126810,#62494,#62495);
#50223=AXIS2_PLACEMENT_3D('',#126811,#62496,#62497);
#50224=AXIS2_PLACEMENT_3D('',#126813,#62498,#62499);
#50225=AXIS2_PLACEMENT_3D('',#126816,#62501,#62502);
#50226=AXIS2_PLACEMENT_3D('',#126817,#62503,#62504);
#50227=AXIS2_PLACEMENT_3D('',#126819,#62505,#62506);
#50228=AXIS2_PLACEMENT_3D('',#126822,#62508,#62509);
#50229=AXIS2_PLACEMENT_3D('',#126823,#62510,#62511);
#50230=AXIS2_PLACEMENT_3D('',#126825,#62512,#62513);
#50231=AXIS2_PLACEMENT_3D('',#126828,#62515,#62516);
#50232=AXIS2_PLACEMENT_3D('',#126829,#62517,#62518);
#50233=AXIS2_PLACEMENT_3D('',#126831,#62519,#62520);
#50234=AXIS2_PLACEMENT_3D('',#126834,#62522,#62523);
#50235=AXIS2_PLACEMENT_3D('',#126835,#62524,#62525);
#50236=AXIS2_PLACEMENT_3D('',#126837,#62526,#62527);
#50237=AXIS2_PLACEMENT_3D('',#126840,#62529,#62530);
#50238=AXIS2_PLACEMENT_3D('',#126841,#62531,#62532);
#50239=AXIS2_PLACEMENT_3D('',#126843,#62533,#62534);
#50240=AXIS2_PLACEMENT_3D('',#126846,#62536,#62537);
#50241=AXIS2_PLACEMENT_3D('',#126847,#62538,#62539);
#50242=AXIS2_PLACEMENT_3D('',#126849,#62540,#62541);
#50243=AXIS2_PLACEMENT_3D('',#126852,#62543,#62544);
#50244=AXIS2_PLACEMENT_3D('',#126853,#62545,#62546);
#50245=AXIS2_PLACEMENT_3D('',#126855,#62547,#62548);
#50246=AXIS2_PLACEMENT_3D('',#126858,#62550,#62551);
#50247=AXIS2_PLACEMENT_3D('',#126859,#62552,#62553);
#50248=AXIS2_PLACEMENT_3D('',#126861,#62554,#62555);
#50249=AXIS2_PLACEMENT_3D('',#126864,#62557,#62558);
#50250=AXIS2_PLACEMENT_3D('',#126865,#62559,#62560);
#50251=AXIS2_PLACEMENT_3D('',#126867,#62561,#62562);
#50252=AXIS2_PLACEMENT_3D('',#126870,#62564,#62565);
#50253=AXIS2_PLACEMENT_3D('',#126871,#62566,#62567);
#50254=AXIS2_PLACEMENT_3D('',#126873,#62568,#62569);
#50255=AXIS2_PLACEMENT_3D('',#126876,#62571,#62572);
#50256=AXIS2_PLACEMENT_3D('',#126877,#62573,#62574);
#50257=AXIS2_PLACEMENT_3D('',#126879,#62575,#62576);
#50258=AXIS2_PLACEMENT_3D('',#126882,#62578,#62579);
#50259=AXIS2_PLACEMENT_3D('',#126883,#62580,#62581);
#50260=AXIS2_PLACEMENT_3D('',#126885,#62582,#62583);
#50261=AXIS2_PLACEMENT_3D('',#126888,#62585,#62586);
#50262=AXIS2_PLACEMENT_3D('',#126889,#62587,#62588);
#50263=AXIS2_PLACEMENT_3D('',#126891,#62589,#62590);
#50264=AXIS2_PLACEMENT_3D('',#126894,#62592,#62593);
#50265=AXIS2_PLACEMENT_3D('',#126895,#62594,#62595);
#50266=AXIS2_PLACEMENT_3D('',#126897,#62596,#62597);
#50267=AXIS2_PLACEMENT_3D('',#126900,#62599,#62600);
#50268=AXIS2_PLACEMENT_3D('',#126901,#62601,#62602);
#50269=AXIS2_PLACEMENT_3D('',#126903,#62603,#62604);
#50270=AXIS2_PLACEMENT_3D('',#126906,#62606,#62607);
#50271=AXIS2_PLACEMENT_3D('',#126907,#62608,#62609);
#50272=AXIS2_PLACEMENT_3D('',#126909,#62610,#62611);
#50273=AXIS2_PLACEMENT_3D('',#126912,#62613,#62614);
#50274=AXIS2_PLACEMENT_3D('',#126913,#62615,#62616);
#50275=AXIS2_PLACEMENT_3D('',#126915,#62617,#62618);
#50276=AXIS2_PLACEMENT_3D('',#126918,#62620,#62621);
#50277=AXIS2_PLACEMENT_3D('',#126919,#62622,#62623);
#50278=AXIS2_PLACEMENT_3D('',#126921,#62624,#62625);
#50279=AXIS2_PLACEMENT_3D('',#126924,#62627,#62628);
#50280=AXIS2_PLACEMENT_3D('',#126925,#62629,#62630);
#50281=AXIS2_PLACEMENT_3D('',#126927,#62631,#62632);
#50282=AXIS2_PLACEMENT_3D('',#126930,#62634,#62635);
#50283=AXIS2_PLACEMENT_3D('',#126931,#62636,#62637);
#50284=AXIS2_PLACEMENT_3D('',#126933,#62638,#62639);
#50285=AXIS2_PLACEMENT_3D('',#126936,#62641,#62642);
#50286=AXIS2_PLACEMENT_3D('',#126937,#62643,#62644);
#50287=AXIS2_PLACEMENT_3D('',#126939,#62645,#62646);
#50288=AXIS2_PLACEMENT_3D('',#126942,#62648,#62649);
#50289=AXIS2_PLACEMENT_3D('',#126943,#62650,#62651);
#50290=AXIS2_PLACEMENT_3D('',#126945,#62652,#62653);
#50291=AXIS2_PLACEMENT_3D('',#126948,#62655,#62656);
#50292=AXIS2_PLACEMENT_3D('',#126949,#62657,#62658);
#50293=AXIS2_PLACEMENT_3D('',#126951,#62659,#62660);
#50294=AXIS2_PLACEMENT_3D('',#126954,#62662,#62663);
#50295=AXIS2_PLACEMENT_3D('',#126955,#62664,#62665);
#50296=AXIS2_PLACEMENT_3D('',#126957,#62666,#62667);
#50297=AXIS2_PLACEMENT_3D('',#126960,#62669,#62670);
#50298=AXIS2_PLACEMENT_3D('',#126961,#62671,#62672);
#50299=AXIS2_PLACEMENT_3D('',#126963,#62673,#62674);
#50300=AXIS2_PLACEMENT_3D('',#126966,#62676,#62677);
#50301=AXIS2_PLACEMENT_3D('',#126967,#62678,#62679);
#50302=AXIS2_PLACEMENT_3D('',#126969,#62680,#62681);
#50303=AXIS2_PLACEMENT_3D('',#126972,#62683,#62684);
#50304=AXIS2_PLACEMENT_3D('',#126973,#62685,#62686);
#50305=AXIS2_PLACEMENT_3D('',#126975,#62687,#62688);
#50306=AXIS2_PLACEMENT_3D('',#126978,#62690,#62691);
#50307=AXIS2_PLACEMENT_3D('',#126979,#62692,#62693);
#50308=AXIS2_PLACEMENT_3D('',#126981,#62694,#62695);
#50309=AXIS2_PLACEMENT_3D('',#126984,#62697,#62698);
#50310=AXIS2_PLACEMENT_3D('',#126985,#62699,#62700);
#50311=AXIS2_PLACEMENT_3D('',#126987,#62701,#62702);
#50312=AXIS2_PLACEMENT_3D('',#126990,#62704,#62705);
#50313=AXIS2_PLACEMENT_3D('',#126991,#62706,#62707);
#50314=AXIS2_PLACEMENT_3D('',#126993,#62708,#62709);
#50315=AXIS2_PLACEMENT_3D('',#126996,#62711,#62712);
#50316=AXIS2_PLACEMENT_3D('',#126997,#62713,#62714);
#50317=AXIS2_PLACEMENT_3D('',#126999,#62715,#62716);
#50318=AXIS2_PLACEMENT_3D('',#127002,#62718,#62719);
#50319=AXIS2_PLACEMENT_3D('',#127003,#62720,#62721);
#50320=AXIS2_PLACEMENT_3D('',#127005,#62722,#62723);
#50321=AXIS2_PLACEMENT_3D('',#127008,#62725,#62726);
#50322=AXIS2_PLACEMENT_3D('',#127009,#62727,#62728);
#50323=AXIS2_PLACEMENT_3D('',#127011,#62729,#62730);
#50324=AXIS2_PLACEMENT_3D('',#127014,#62732,#62733);
#50325=AXIS2_PLACEMENT_3D('',#127015,#62734,#62735);
#50326=AXIS2_PLACEMENT_3D('',#127017,#62736,#62737);
#50327=AXIS2_PLACEMENT_3D('',#127020,#62739,#62740);
#50328=AXIS2_PLACEMENT_3D('',#127021,#62741,#62742);
#50329=AXIS2_PLACEMENT_3D('',#127023,#62743,#62744);
#50330=AXIS2_PLACEMENT_3D('',#127026,#62746,#62747);
#50331=AXIS2_PLACEMENT_3D('',#127027,#62748,#62749);
#50332=AXIS2_PLACEMENT_3D('',#127029,#62750,#62751);
#50333=AXIS2_PLACEMENT_3D('',#127032,#62753,#62754);
#50334=AXIS2_PLACEMENT_3D('',#127033,#62755,#62756);
#50335=AXIS2_PLACEMENT_3D('',#127035,#62757,#62758);
#50336=AXIS2_PLACEMENT_3D('',#127038,#62760,#62761);
#50337=AXIS2_PLACEMENT_3D('',#127039,#62762,#62763);
#50338=AXIS2_PLACEMENT_3D('',#127041,#62764,#62765);
#50339=AXIS2_PLACEMENT_3D('',#127044,#62767,#62768);
#50340=AXIS2_PLACEMENT_3D('',#127045,#62769,#62770);
#50341=AXIS2_PLACEMENT_3D('',#127047,#62771,#62772);
#50342=AXIS2_PLACEMENT_3D('',#127050,#62774,#62775);
#50343=AXIS2_PLACEMENT_3D('',#127051,#62776,#62777);
#50344=AXIS2_PLACEMENT_3D('',#127053,#62778,#62779);
#50345=AXIS2_PLACEMENT_3D('',#127056,#62781,#62782);
#50346=AXIS2_PLACEMENT_3D('',#127057,#62783,#62784);
#50347=AXIS2_PLACEMENT_3D('',#127059,#62785,#62786);
#50348=AXIS2_PLACEMENT_3D('',#127062,#62788,#62789);
#50349=AXIS2_PLACEMENT_3D('',#127063,#62790,#62791);
#50350=AXIS2_PLACEMENT_3D('',#127065,#62792,#62793);
#50351=AXIS2_PLACEMENT_3D('',#127068,#62795,#62796);
#50352=AXIS2_PLACEMENT_3D('',#127069,#62797,#62798);
#50353=AXIS2_PLACEMENT_3D('',#127071,#62799,#62800);
#50354=AXIS2_PLACEMENT_3D('',#127074,#62802,#62803);
#50355=AXIS2_PLACEMENT_3D('',#127075,#62804,#62805);
#50356=AXIS2_PLACEMENT_3D('',#127077,#62806,#62807);
#50357=AXIS2_PLACEMENT_3D('',#127080,#62809,#62810);
#50358=AXIS2_PLACEMENT_3D('',#127081,#62811,#62812);
#50359=AXIS2_PLACEMENT_3D('',#127083,#62813,#62814);
#50360=AXIS2_PLACEMENT_3D('',#127086,#62816,#62817);
#50361=AXIS2_PLACEMENT_3D('',#127087,#62818,#62819);
#50362=AXIS2_PLACEMENT_3D('',#127089,#62820,#62821);
#50363=AXIS2_PLACEMENT_3D('',#127092,#62823,#62824);
#50364=AXIS2_PLACEMENT_3D('',#127093,#62825,#62826);
#50365=AXIS2_PLACEMENT_3D('',#127095,#62827,#62828);
#50366=AXIS2_PLACEMENT_3D('',#127098,#62830,#62831);
#50367=AXIS2_PLACEMENT_3D('',#127099,#62832,#62833);
#50368=AXIS2_PLACEMENT_3D('',#127101,#62834,#62835);
#50369=AXIS2_PLACEMENT_3D('',#127104,#62837,#62838);
#50370=AXIS2_PLACEMENT_3D('',#127105,#62839,#62840);
#50371=AXIS2_PLACEMENT_3D('',#127107,#62841,#62842);
#50372=AXIS2_PLACEMENT_3D('',#127110,#62844,#62845);
#50373=AXIS2_PLACEMENT_3D('',#127111,#62846,#62847);
#50374=AXIS2_PLACEMENT_3D('',#127113,#62848,#62849);
#50375=AXIS2_PLACEMENT_3D('',#127116,#62851,#62852);
#50376=AXIS2_PLACEMENT_3D('',#127117,#62853,#62854);
#50377=AXIS2_PLACEMENT_3D('',#127119,#62855,#62856);
#50378=AXIS2_PLACEMENT_3D('',#127122,#62858,#62859);
#50379=AXIS2_PLACEMENT_3D('',#127123,#62860,#62861);
#50380=AXIS2_PLACEMENT_3D('',#127125,#62862,#62863);
#50381=AXIS2_PLACEMENT_3D('',#127128,#62865,#62866);
#50382=AXIS2_PLACEMENT_3D('',#127129,#62867,#62868);
#50383=AXIS2_PLACEMENT_3D('',#127131,#62869,#62870);
#50384=AXIS2_PLACEMENT_3D('',#127134,#62872,#62873);
#50385=AXIS2_PLACEMENT_3D('',#127135,#62874,#62875);
#50386=AXIS2_PLACEMENT_3D('',#127137,#62876,#62877);
#50387=AXIS2_PLACEMENT_3D('',#127140,#62879,#62880);
#50388=AXIS2_PLACEMENT_3D('',#127141,#62881,#62882);
#50389=AXIS2_PLACEMENT_3D('',#127143,#62883,#62884);
#50390=AXIS2_PLACEMENT_3D('',#127146,#62886,#62887);
#50391=AXIS2_PLACEMENT_3D('',#127147,#62888,#62889);
#50392=AXIS2_PLACEMENT_3D('',#127149,#62890,#62891);
#50393=AXIS2_PLACEMENT_3D('',#127152,#62893,#62894);
#50394=AXIS2_PLACEMENT_3D('',#127153,#62895,#62896);
#50395=AXIS2_PLACEMENT_3D('',#127155,#62897,#62898);
#50396=AXIS2_PLACEMENT_3D('',#127158,#62900,#62901);
#50397=AXIS2_PLACEMENT_3D('',#127159,#62902,#62903);
#50398=AXIS2_PLACEMENT_3D('',#127161,#62904,#62905);
#50399=AXIS2_PLACEMENT_3D('',#127164,#62907,#62908);
#50400=AXIS2_PLACEMENT_3D('',#127165,#62909,#62910);
#50401=AXIS2_PLACEMENT_3D('',#127167,#62911,#62912);
#50402=AXIS2_PLACEMENT_3D('',#127170,#62914,#62915);
#50403=AXIS2_PLACEMENT_3D('',#127171,#62916,#62917);
#50404=AXIS2_PLACEMENT_3D('',#127173,#62918,#62919);
#50405=AXIS2_PLACEMENT_3D('',#127176,#62921,#62922);
#50406=AXIS2_PLACEMENT_3D('',#127177,#62923,#62924);
#50407=AXIS2_PLACEMENT_3D('',#127179,#62925,#62926);
#50408=AXIS2_PLACEMENT_3D('',#127182,#62928,#62929);
#50409=AXIS2_PLACEMENT_3D('',#127183,#62930,#62931);
#50410=AXIS2_PLACEMENT_3D('',#127185,#62932,#62933);
#50411=AXIS2_PLACEMENT_3D('',#127188,#62935,#62936);
#50412=AXIS2_PLACEMENT_3D('',#127189,#62937,#62938);
#50413=AXIS2_PLACEMENT_3D('',#127191,#62939,#62940);
#50414=AXIS2_PLACEMENT_3D('',#127194,#62942,#62943);
#50415=AXIS2_PLACEMENT_3D('',#127195,#62944,#62945);
#50416=AXIS2_PLACEMENT_3D('',#127197,#62946,#62947);
#50417=AXIS2_PLACEMENT_3D('',#127200,#62949,#62950);
#50418=AXIS2_PLACEMENT_3D('',#127201,#62951,#62952);
#50419=AXIS2_PLACEMENT_3D('',#127203,#62953,#62954);
#50420=AXIS2_PLACEMENT_3D('',#127206,#62956,#62957);
#50421=AXIS2_PLACEMENT_3D('',#127207,#62958,#62959);
#50422=AXIS2_PLACEMENT_3D('',#127209,#62960,#62961);
#50423=AXIS2_PLACEMENT_3D('',#127212,#62963,#62964);
#50424=AXIS2_PLACEMENT_3D('',#127213,#62965,#62966);
#50425=AXIS2_PLACEMENT_3D('',#127215,#62967,#62968);
#50426=AXIS2_PLACEMENT_3D('',#127218,#62970,#62971);
#50427=AXIS2_PLACEMENT_3D('',#127219,#62972,#62973);
#50428=AXIS2_PLACEMENT_3D('',#127221,#62974,#62975);
#50429=AXIS2_PLACEMENT_3D('',#127224,#62977,#62978);
#50430=AXIS2_PLACEMENT_3D('',#127225,#62979,#62980);
#50431=AXIS2_PLACEMENT_3D('',#127227,#62981,#62982);
#50432=AXIS2_PLACEMENT_3D('',#127230,#62984,#62985);
#50433=AXIS2_PLACEMENT_3D('',#127231,#62986,#62987);
#50434=AXIS2_PLACEMENT_3D('',#127233,#62988,#62989);
#50435=AXIS2_PLACEMENT_3D('',#127236,#62991,#62992);
#50436=AXIS2_PLACEMENT_3D('',#127237,#62993,#62994);
#50437=AXIS2_PLACEMENT_3D('',#127239,#62995,#62996);
#50438=AXIS2_PLACEMENT_3D('',#127242,#62998,#62999);
#50439=AXIS2_PLACEMENT_3D('',#127243,#63000,#63001);
#50440=AXIS2_PLACEMENT_3D('',#127245,#63002,#63003);
#50441=AXIS2_PLACEMENT_3D('',#127248,#63005,#63006);
#50442=AXIS2_PLACEMENT_3D('',#127249,#63007,#63008);
#50443=AXIS2_PLACEMENT_3D('',#127251,#63009,#63010);
#50444=AXIS2_PLACEMENT_3D('',#127254,#63012,#63013);
#50445=AXIS2_PLACEMENT_3D('',#127255,#63014,#63015);
#50446=AXIS2_PLACEMENT_3D('',#127257,#63016,#63017);
#50447=AXIS2_PLACEMENT_3D('',#127260,#63019,#63020);
#50448=AXIS2_PLACEMENT_3D('',#127261,#63021,#63022);
#50449=AXIS2_PLACEMENT_3D('',#127263,#63023,#63024);
#50450=AXIS2_PLACEMENT_3D('',#127266,#63026,#63027);
#50451=AXIS2_PLACEMENT_3D('',#127267,#63028,#63029);
#50452=AXIS2_PLACEMENT_3D('',#127269,#63030,#63031);
#50453=AXIS2_PLACEMENT_3D('',#127272,#63033,#63034);
#50454=AXIS2_PLACEMENT_3D('',#127273,#63035,#63036);
#50455=AXIS2_PLACEMENT_3D('',#127275,#63037,#63038);
#50456=AXIS2_PLACEMENT_3D('',#127278,#63040,#63041);
#50457=AXIS2_PLACEMENT_3D('',#127279,#63042,#63043);
#50458=AXIS2_PLACEMENT_3D('',#127281,#63044,#63045);
#50459=AXIS2_PLACEMENT_3D('',#127284,#63047,#63048);
#50460=AXIS2_PLACEMENT_3D('',#127285,#63049,#63050);
#50461=AXIS2_PLACEMENT_3D('',#127287,#63051,#63052);
#50462=AXIS2_PLACEMENT_3D('',#127290,#63054,#63055);
#50463=AXIS2_PLACEMENT_3D('',#127291,#63056,#63057);
#50464=AXIS2_PLACEMENT_3D('',#127293,#63058,#63059);
#50465=AXIS2_PLACEMENT_3D('',#127296,#63061,#63062);
#50466=AXIS2_PLACEMENT_3D('',#127297,#63063,#63064);
#50467=AXIS2_PLACEMENT_3D('',#127299,#63065,#63066);
#50468=AXIS2_PLACEMENT_3D('',#127302,#63068,#63069);
#50469=AXIS2_PLACEMENT_3D('',#127303,#63070,#63071);
#50470=AXIS2_PLACEMENT_3D('',#127305,#63072,#63073);
#50471=AXIS2_PLACEMENT_3D('',#127308,#63075,#63076);
#50472=AXIS2_PLACEMENT_3D('',#127309,#63077,#63078);
#50473=AXIS2_PLACEMENT_3D('',#127311,#63079,#63080);
#50474=AXIS2_PLACEMENT_3D('',#127314,#63082,#63083);
#50475=AXIS2_PLACEMENT_3D('',#127315,#63084,#63085);
#50476=AXIS2_PLACEMENT_3D('',#127317,#63086,#63087);
#50477=AXIS2_PLACEMENT_3D('',#127320,#63089,#63090);
#50478=AXIS2_PLACEMENT_3D('',#127321,#63091,#63092);
#50479=AXIS2_PLACEMENT_3D('',#127323,#63093,#63094);
#50480=AXIS2_PLACEMENT_3D('',#127326,#63096,#63097);
#50481=AXIS2_PLACEMENT_3D('',#127327,#63098,#63099);
#50482=AXIS2_PLACEMENT_3D('',#127329,#63100,#63101);
#50483=AXIS2_PLACEMENT_3D('',#127332,#63103,#63104);
#50484=AXIS2_PLACEMENT_3D('',#127333,#63105,#63106);
#50485=AXIS2_PLACEMENT_3D('',#127335,#63107,#63108);
#50486=AXIS2_PLACEMENT_3D('',#127338,#63110,#63111);
#50487=AXIS2_PLACEMENT_3D('',#127339,#63112,#63113);
#50488=AXIS2_PLACEMENT_3D('',#127341,#63114,#63115);
#50489=AXIS2_PLACEMENT_3D('',#127344,#63117,#63118);
#50490=AXIS2_PLACEMENT_3D('',#127345,#63119,#63120);
#50491=AXIS2_PLACEMENT_3D('',#127347,#63121,#63122);
#50492=AXIS2_PLACEMENT_3D('',#127350,#63124,#63125);
#50493=AXIS2_PLACEMENT_3D('',#127351,#63126,#63127);
#50494=AXIS2_PLACEMENT_3D('',#127353,#63128,#63129);
#50495=AXIS2_PLACEMENT_3D('',#127356,#63131,#63132);
#50496=AXIS2_PLACEMENT_3D('',#127357,#63133,#63134);
#50497=AXIS2_PLACEMENT_3D('',#127359,#63135,#63136);
#50498=AXIS2_PLACEMENT_3D('',#127362,#63138,#63139);
#50499=AXIS2_PLACEMENT_3D('',#127363,#63140,#63141);
#50500=AXIS2_PLACEMENT_3D('',#127365,#63142,#63143);
#50501=AXIS2_PLACEMENT_3D('',#127368,#63145,#63146);
#50502=AXIS2_PLACEMENT_3D('',#127369,#63147,#63148);
#50503=AXIS2_PLACEMENT_3D('',#127371,#63149,#63150);
#50504=AXIS2_PLACEMENT_3D('',#127374,#63152,#63153);
#50505=AXIS2_PLACEMENT_3D('',#127375,#63154,#63155);
#50506=AXIS2_PLACEMENT_3D('',#127377,#63156,#63157);
#50507=AXIS2_PLACEMENT_3D('',#127380,#63159,#63160);
#50508=AXIS2_PLACEMENT_3D('',#127381,#63161,#63162);
#50509=AXIS2_PLACEMENT_3D('',#127383,#63163,#63164);
#50510=AXIS2_PLACEMENT_3D('',#127386,#63166,#63167);
#50511=AXIS2_PLACEMENT_3D('',#127387,#63168,#63169);
#50512=AXIS2_PLACEMENT_3D('',#127389,#63170,#63171);
#50513=AXIS2_PLACEMENT_3D('',#127392,#63173,#63174);
#50514=AXIS2_PLACEMENT_3D('',#127393,#63175,#63176);
#50515=AXIS2_PLACEMENT_3D('',#127395,#63177,#63178);
#50516=AXIS2_PLACEMENT_3D('',#127398,#63180,#63181);
#50517=AXIS2_PLACEMENT_3D('',#127399,#63182,#63183);
#50518=AXIS2_PLACEMENT_3D('',#127401,#63184,#63185);
#50519=AXIS2_PLACEMENT_3D('',#127404,#63187,#63188);
#50520=AXIS2_PLACEMENT_3D('',#127405,#63189,#63190);
#50521=AXIS2_PLACEMENT_3D('',#127407,#63191,#63192);
#50522=AXIS2_PLACEMENT_3D('',#127410,#63194,#63195);
#50523=AXIS2_PLACEMENT_3D('',#127411,#63196,#63197);
#50524=AXIS2_PLACEMENT_3D('',#127413,#63198,#63199);
#50525=AXIS2_PLACEMENT_3D('',#127416,#63201,#63202);
#50526=AXIS2_PLACEMENT_3D('',#127417,#63203,#63204);
#50527=AXIS2_PLACEMENT_3D('',#127419,#63205,#63206);
#50528=AXIS2_PLACEMENT_3D('',#127422,#63208,#63209);
#50529=AXIS2_PLACEMENT_3D('',#127423,#63210,#63211);
#50530=AXIS2_PLACEMENT_3D('',#127425,#63212,#63213);
#50531=AXIS2_PLACEMENT_3D('',#127428,#63215,#63216);
#50532=AXIS2_PLACEMENT_3D('',#127429,#63217,#63218);
#50533=AXIS2_PLACEMENT_3D('',#127431,#63219,#63220);
#50534=AXIS2_PLACEMENT_3D('',#127434,#63222,#63223);
#50535=AXIS2_PLACEMENT_3D('',#127435,#63224,#63225);
#50536=AXIS2_PLACEMENT_3D('',#127437,#63226,#63227);
#50537=AXIS2_PLACEMENT_3D('',#127440,#63229,#63230);
#50538=AXIS2_PLACEMENT_3D('',#127441,#63231,#63232);
#50539=AXIS2_PLACEMENT_3D('',#127443,#63233,#63234);
#50540=AXIS2_PLACEMENT_3D('',#127446,#63236,#63237);
#50541=AXIS2_PLACEMENT_3D('',#127447,#63238,#63239);
#50542=AXIS2_PLACEMENT_3D('',#127449,#63240,#63241);
#50543=AXIS2_PLACEMENT_3D('',#127452,#63243,#63244);
#50544=AXIS2_PLACEMENT_3D('',#127453,#63245,#63246);
#50545=AXIS2_PLACEMENT_3D('',#127455,#63247,#63248);
#50546=AXIS2_PLACEMENT_3D('',#127458,#63250,#63251);
#50547=AXIS2_PLACEMENT_3D('',#127459,#63252,#63253);
#50548=AXIS2_PLACEMENT_3D('',#127461,#63254,#63255);
#50549=AXIS2_PLACEMENT_3D('',#127464,#63257,#63258);
#50550=AXIS2_PLACEMENT_3D('',#127465,#63259,#63260);
#50551=AXIS2_PLACEMENT_3D('',#127467,#63261,#63262);
#50552=AXIS2_PLACEMENT_3D('',#127470,#63264,#63265);
#50553=AXIS2_PLACEMENT_3D('',#127471,#63266,#63267);
#50554=AXIS2_PLACEMENT_3D('',#127473,#63268,#63269);
#50555=AXIS2_PLACEMENT_3D('',#127476,#63271,#63272);
#50556=AXIS2_PLACEMENT_3D('',#127477,#63273,#63274);
#50557=AXIS2_PLACEMENT_3D('',#127479,#63275,#63276);
#50558=AXIS2_PLACEMENT_3D('',#127482,#63278,#63279);
#50559=AXIS2_PLACEMENT_3D('',#127483,#63280,#63281);
#50560=AXIS2_PLACEMENT_3D('',#127485,#63282,#63283);
#50561=AXIS2_PLACEMENT_3D('',#127488,#63285,#63286);
#50562=AXIS2_PLACEMENT_3D('',#127489,#63287,#63288);
#50563=AXIS2_PLACEMENT_3D('',#127491,#63289,#63290);
#50564=AXIS2_PLACEMENT_3D('',#127494,#63292,#63293);
#50565=AXIS2_PLACEMENT_3D('',#127495,#63294,#63295);
#50566=AXIS2_PLACEMENT_3D('',#127497,#63296,#63297);
#50567=AXIS2_PLACEMENT_3D('',#127500,#63299,#63300);
#50568=AXIS2_PLACEMENT_3D('',#127501,#63301,#63302);
#50569=AXIS2_PLACEMENT_3D('',#127503,#63303,#63304);
#50570=AXIS2_PLACEMENT_3D('',#127506,#63306,#63307);
#50571=AXIS2_PLACEMENT_3D('',#127507,#63308,#63309);
#50572=AXIS2_PLACEMENT_3D('',#127509,#63310,#63311);
#50573=AXIS2_PLACEMENT_3D('',#127512,#63313,#63314);
#50574=AXIS2_PLACEMENT_3D('',#127513,#63315,#63316);
#50575=AXIS2_PLACEMENT_3D('',#127515,#63317,#63318);
#50576=AXIS2_PLACEMENT_3D('',#127518,#63320,#63321);
#50577=AXIS2_PLACEMENT_3D('',#127519,#63322,#63323);
#50578=AXIS2_PLACEMENT_3D('',#127521,#63324,#63325);
#50579=AXIS2_PLACEMENT_3D('',#127524,#63327,#63328);
#50580=AXIS2_PLACEMENT_3D('',#127525,#63329,#63330);
#50581=AXIS2_PLACEMENT_3D('',#127527,#63331,#63332);
#50582=AXIS2_PLACEMENT_3D('',#127530,#63334,#63335);
#50583=AXIS2_PLACEMENT_3D('',#127531,#63336,#63337);
#50584=AXIS2_PLACEMENT_3D('',#127533,#63338,#63339);
#50585=AXIS2_PLACEMENT_3D('',#127536,#63341,#63342);
#50586=AXIS2_PLACEMENT_3D('',#127537,#63343,#63344);
#50587=AXIS2_PLACEMENT_3D('',#127539,#63345,#63346);
#50588=AXIS2_PLACEMENT_3D('',#127542,#63348,#63349);
#50589=AXIS2_PLACEMENT_3D('',#127543,#63350,#63351);
#50590=AXIS2_PLACEMENT_3D('',#127545,#63352,#63353);
#50591=AXIS2_PLACEMENT_3D('',#127548,#63355,#63356);
#50592=AXIS2_PLACEMENT_3D('',#127549,#63357,#63358);
#50593=AXIS2_PLACEMENT_3D('',#127551,#63359,#63360);
#50594=AXIS2_PLACEMENT_3D('',#127554,#63362,#63363);
#50595=AXIS2_PLACEMENT_3D('',#127555,#63364,#63365);
#50596=AXIS2_PLACEMENT_3D('',#127557,#63366,#63367);
#50597=AXIS2_PLACEMENT_3D('',#127560,#63369,#63370);
#50598=AXIS2_PLACEMENT_3D('',#127561,#63371,#63372);
#50599=AXIS2_PLACEMENT_3D('',#127563,#63373,#63374);
#50600=AXIS2_PLACEMENT_3D('',#127566,#63376,#63377);
#50601=AXIS2_PLACEMENT_3D('',#127567,#63378,#63379);
#50602=AXIS2_PLACEMENT_3D('',#127569,#63380,#63381);
#50603=AXIS2_PLACEMENT_3D('',#127572,#63383,#63384);
#50604=AXIS2_PLACEMENT_3D('',#127573,#63385,#63386);
#50605=AXIS2_PLACEMENT_3D('',#127575,#63387,#63388);
#50606=AXIS2_PLACEMENT_3D('',#127578,#63390,#63391);
#50607=AXIS2_PLACEMENT_3D('',#127579,#63392,#63393);
#50608=AXIS2_PLACEMENT_3D('',#127581,#63394,#63395);
#50609=AXIS2_PLACEMENT_3D('',#127584,#63397,#63398);
#50610=AXIS2_PLACEMENT_3D('',#127585,#63399,#63400);
#50611=AXIS2_PLACEMENT_3D('',#127587,#63401,#63402);
#50612=AXIS2_PLACEMENT_3D('',#127590,#63404,#63405);
#50613=AXIS2_PLACEMENT_3D('',#127591,#63406,#63407);
#50614=AXIS2_PLACEMENT_3D('',#127593,#63408,#63409);
#50615=AXIS2_PLACEMENT_3D('',#127596,#63411,#63412);
#50616=AXIS2_PLACEMENT_3D('',#127597,#63413,#63414);
#50617=AXIS2_PLACEMENT_3D('',#127599,#63415,#63416);
#50618=AXIS2_PLACEMENT_3D('',#127602,#63418,#63419);
#50619=AXIS2_PLACEMENT_3D('',#127603,#63420,#63421);
#50620=AXIS2_PLACEMENT_3D('',#127605,#63422,#63423);
#50621=AXIS2_PLACEMENT_3D('',#127608,#63425,#63426);
#50622=AXIS2_PLACEMENT_3D('',#127609,#63427,#63428);
#50623=AXIS2_PLACEMENT_3D('',#127611,#63429,#63430);
#50624=AXIS2_PLACEMENT_3D('',#127614,#63432,#63433);
#50625=AXIS2_PLACEMENT_3D('',#127615,#63434,#63435);
#50626=AXIS2_PLACEMENT_3D('',#127617,#63436,#63437);
#50627=AXIS2_PLACEMENT_3D('',#127620,#63439,#63440);
#50628=AXIS2_PLACEMENT_3D('',#127621,#63441,#63442);
#50629=AXIS2_PLACEMENT_3D('',#127623,#63443,#63444);
#50630=AXIS2_PLACEMENT_3D('',#127626,#63446,#63447);
#50631=AXIS2_PLACEMENT_3D('',#127627,#63448,#63449);
#50632=AXIS2_PLACEMENT_3D('',#127629,#63450,#63451);
#50633=AXIS2_PLACEMENT_3D('',#127632,#63453,#63454);
#50634=AXIS2_PLACEMENT_3D('',#127633,#63455,#63456);
#50635=AXIS2_PLACEMENT_3D('',#127635,#63457,#63458);
#50636=AXIS2_PLACEMENT_3D('',#127638,#63460,#63461);
#50637=AXIS2_PLACEMENT_3D('',#127639,#63462,#63463);
#50638=AXIS2_PLACEMENT_3D('',#127641,#63464,#63465);
#50639=AXIS2_PLACEMENT_3D('',#127644,#63467,#63468);
#50640=AXIS2_PLACEMENT_3D('',#127645,#63469,#63470);
#50641=AXIS2_PLACEMENT_3D('',#127647,#63471,#63472);
#50642=AXIS2_PLACEMENT_3D('',#127650,#63474,#63475);
#50643=AXIS2_PLACEMENT_3D('',#127651,#63476,#63477);
#50644=AXIS2_PLACEMENT_3D('',#127653,#63478,#63479);
#50645=AXIS2_PLACEMENT_3D('',#127656,#63481,#63482);
#50646=AXIS2_PLACEMENT_3D('',#127657,#63483,#63484);
#50647=AXIS2_PLACEMENT_3D('',#127659,#63485,#63486);
#50648=AXIS2_PLACEMENT_3D('',#127662,#63488,#63489);
#50649=AXIS2_PLACEMENT_3D('',#127663,#63490,#63491);
#50650=AXIS2_PLACEMENT_3D('',#127665,#63492,#63493);
#50651=AXIS2_PLACEMENT_3D('',#127668,#63495,#63496);
#50652=AXIS2_PLACEMENT_3D('',#127669,#63497,#63498);
#50653=AXIS2_PLACEMENT_3D('',#127671,#63499,#63500);
#50654=AXIS2_PLACEMENT_3D('',#127674,#63502,#63503);
#50655=AXIS2_PLACEMENT_3D('',#127675,#63504,#63505);
#50656=AXIS2_PLACEMENT_3D('',#127677,#63506,#63507);
#50657=AXIS2_PLACEMENT_3D('',#127680,#63509,#63510);
#50658=AXIS2_PLACEMENT_3D('',#127681,#63511,#63512);
#50659=AXIS2_PLACEMENT_3D('',#127683,#63513,#63514);
#50660=AXIS2_PLACEMENT_3D('',#127686,#63516,#63517);
#50661=AXIS2_PLACEMENT_3D('',#127687,#63518,#63519);
#50662=AXIS2_PLACEMENT_3D('',#127689,#63520,#63521);
#50663=AXIS2_PLACEMENT_3D('',#127692,#63523,#63524);
#50664=AXIS2_PLACEMENT_3D('',#127693,#63525,#63526);
#50665=AXIS2_PLACEMENT_3D('',#127695,#63527,#63528);
#50666=AXIS2_PLACEMENT_3D('',#127698,#63530,#63531);
#50667=AXIS2_PLACEMENT_3D('',#127699,#63532,#63533);
#50668=AXIS2_PLACEMENT_3D('',#127701,#63534,#63535);
#50669=AXIS2_PLACEMENT_3D('',#127704,#63537,#63538);
#50670=AXIS2_PLACEMENT_3D('',#127705,#63539,#63540);
#50671=AXIS2_PLACEMENT_3D('',#127707,#63541,#63542);
#50672=AXIS2_PLACEMENT_3D('',#127710,#63544,#63545);
#50673=AXIS2_PLACEMENT_3D('',#127711,#63546,#63547);
#50674=AXIS2_PLACEMENT_3D('',#127713,#63548,#63549);
#50675=AXIS2_PLACEMENT_3D('',#127716,#63551,#63552);
#50676=AXIS2_PLACEMENT_3D('',#127717,#63553,#63554);
#50677=AXIS2_PLACEMENT_3D('',#127719,#63555,#63556);
#50678=AXIS2_PLACEMENT_3D('',#127722,#63558,#63559);
#50679=AXIS2_PLACEMENT_3D('',#127723,#63560,#63561);
#50680=AXIS2_PLACEMENT_3D('',#127725,#63562,#63563);
#50681=AXIS2_PLACEMENT_3D('',#127728,#63565,#63566);
#50682=AXIS2_PLACEMENT_3D('',#127729,#63567,#63568);
#50683=AXIS2_PLACEMENT_3D('',#127731,#63569,#63570);
#50684=AXIS2_PLACEMENT_3D('',#127734,#63572,#63573);
#50685=AXIS2_PLACEMENT_3D('',#127735,#63574,#63575);
#50686=AXIS2_PLACEMENT_3D('',#127737,#63576,#63577);
#50687=AXIS2_PLACEMENT_3D('',#127740,#63579,#63580);
#50688=AXIS2_PLACEMENT_3D('',#127741,#63581,#63582);
#50689=AXIS2_PLACEMENT_3D('',#127743,#63583,#63584);
#50690=AXIS2_PLACEMENT_3D('',#127746,#63586,#63587);
#50691=AXIS2_PLACEMENT_3D('',#127747,#63588,#63589);
#50692=AXIS2_PLACEMENT_3D('',#127749,#63590,#63591);
#50693=AXIS2_PLACEMENT_3D('',#127752,#63593,#63594);
#50694=AXIS2_PLACEMENT_3D('',#127753,#63595,#63596);
#50695=AXIS2_PLACEMENT_3D('',#127755,#63597,#63598);
#50696=AXIS2_PLACEMENT_3D('',#127758,#63600,#63601);
#50697=AXIS2_PLACEMENT_3D('',#127759,#63602,#63603);
#50698=AXIS2_PLACEMENT_3D('',#127761,#63604,#63605);
#50699=AXIS2_PLACEMENT_3D('',#127764,#63607,#63608);
#50700=AXIS2_PLACEMENT_3D('',#127765,#63609,#63610);
#50701=AXIS2_PLACEMENT_3D('',#127767,#63611,#63612);
#50702=AXIS2_PLACEMENT_3D('',#127770,#63614,#63615);
#50703=AXIS2_PLACEMENT_3D('',#127771,#63616,#63617);
#50704=AXIS2_PLACEMENT_3D('',#127773,#63618,#63619);
#50705=AXIS2_PLACEMENT_3D('',#127776,#63621,#63622);
#50706=AXIS2_PLACEMENT_3D('',#127777,#63623,#63624);
#50707=AXIS2_PLACEMENT_3D('',#127779,#63625,#63626);
#50708=AXIS2_PLACEMENT_3D('',#127782,#63628,#63629);
#50709=AXIS2_PLACEMENT_3D('',#127783,#63630,#63631);
#50710=AXIS2_PLACEMENT_3D('',#127785,#63632,#63633);
#50711=AXIS2_PLACEMENT_3D('',#127788,#63635,#63636);
#50712=AXIS2_PLACEMENT_3D('',#127789,#63637,#63638);
#50713=AXIS2_PLACEMENT_3D('',#127791,#63639,#63640);
#50714=AXIS2_PLACEMENT_3D('',#127794,#63642,#63643);
#50715=AXIS2_PLACEMENT_3D('',#127795,#63644,#63645);
#50716=AXIS2_PLACEMENT_3D('',#127797,#63646,#63647);
#50717=AXIS2_PLACEMENT_3D('',#127800,#63649,#63650);
#50718=AXIS2_PLACEMENT_3D('',#127801,#63651,#63652);
#50719=AXIS2_PLACEMENT_3D('',#127803,#63653,#63654);
#50720=AXIS2_PLACEMENT_3D('',#127806,#63656,#63657);
#50721=AXIS2_PLACEMENT_3D('',#127807,#63658,#63659);
#50722=AXIS2_PLACEMENT_3D('',#127809,#63660,#63661);
#50723=AXIS2_PLACEMENT_3D('',#127812,#63663,#63664);
#50724=AXIS2_PLACEMENT_3D('',#127813,#63665,#63666);
#50725=AXIS2_PLACEMENT_3D('',#127815,#63667,#63668);
#50726=AXIS2_PLACEMENT_3D('',#127818,#63670,#63671);
#50727=AXIS2_PLACEMENT_3D('',#127819,#63672,#63673);
#50728=AXIS2_PLACEMENT_3D('',#127821,#63674,#63675);
#50729=AXIS2_PLACEMENT_3D('',#127824,#63677,#63678);
#50730=AXIS2_PLACEMENT_3D('',#127825,#63679,#63680);
#50731=AXIS2_PLACEMENT_3D('',#127827,#63681,#63682);
#50732=AXIS2_PLACEMENT_3D('',#127830,#63684,#63685);
#50733=AXIS2_PLACEMENT_3D('',#127831,#63686,#63687);
#50734=AXIS2_PLACEMENT_3D('',#127833,#63688,#63689);
#50735=AXIS2_PLACEMENT_3D('',#127836,#63691,#63692);
#50736=AXIS2_PLACEMENT_3D('',#127837,#63693,#63694);
#50737=AXIS2_PLACEMENT_3D('',#127839,#63695,#63696);
#50738=AXIS2_PLACEMENT_3D('',#127842,#63698,#63699);
#50739=AXIS2_PLACEMENT_3D('',#127843,#63700,#63701);
#50740=AXIS2_PLACEMENT_3D('',#127845,#63702,#63703);
#50741=AXIS2_PLACEMENT_3D('',#127848,#63705,#63706);
#50742=AXIS2_PLACEMENT_3D('',#127849,#63707,#63708);
#50743=AXIS2_PLACEMENT_3D('',#127851,#63709,#63710);
#50744=AXIS2_PLACEMENT_3D('',#127854,#63712,#63713);
#50745=AXIS2_PLACEMENT_3D('',#127855,#63714,#63715);
#50746=AXIS2_PLACEMENT_3D('',#127857,#63716,#63717);
#50747=AXIS2_PLACEMENT_3D('',#127860,#63719,#63720);
#50748=AXIS2_PLACEMENT_3D('',#127861,#63721,#63722);
#50749=AXIS2_PLACEMENT_3D('',#127863,#63723,#63724);
#50750=AXIS2_PLACEMENT_3D('',#127866,#63726,#63727);
#50751=AXIS2_PLACEMENT_3D('',#127867,#63728,#63729);
#50752=AXIS2_PLACEMENT_3D('',#127869,#63730,#63731);
#50753=AXIS2_PLACEMENT_3D('',#127872,#63733,#63734);
#50754=AXIS2_PLACEMENT_3D('',#127873,#63735,#63736);
#50755=AXIS2_PLACEMENT_3D('',#127875,#63737,#63738);
#50756=AXIS2_PLACEMENT_3D('',#127878,#63740,#63741);
#50757=AXIS2_PLACEMENT_3D('',#127879,#63742,#63743);
#50758=AXIS2_PLACEMENT_3D('',#127881,#63744,#63745);
#50759=AXIS2_PLACEMENT_3D('',#127884,#63747,#63748);
#50760=AXIS2_PLACEMENT_3D('',#127885,#63749,#63750);
#50761=AXIS2_PLACEMENT_3D('',#127887,#63751,#63752);
#50762=AXIS2_PLACEMENT_3D('',#127890,#63754,#63755);
#50763=AXIS2_PLACEMENT_3D('',#127891,#63756,#63757);
#50764=AXIS2_PLACEMENT_3D('',#127893,#63758,#63759);
#50765=AXIS2_PLACEMENT_3D('',#127896,#63761,#63762);
#50766=AXIS2_PLACEMENT_3D('',#127897,#63763,#63764);
#50767=AXIS2_PLACEMENT_3D('',#127899,#63765,#63766);
#50768=AXIS2_PLACEMENT_3D('',#127902,#63768,#63769);
#50769=AXIS2_PLACEMENT_3D('',#127903,#63770,#63771);
#50770=AXIS2_PLACEMENT_3D('',#127905,#63772,#63773);
#50771=AXIS2_PLACEMENT_3D('',#127908,#63775,#63776);
#50772=AXIS2_PLACEMENT_3D('',#127909,#63777,#63778);
#50773=AXIS2_PLACEMENT_3D('',#127911,#63779,#63780);
#50774=AXIS2_PLACEMENT_3D('',#127914,#63782,#63783);
#50775=AXIS2_PLACEMENT_3D('',#127915,#63784,#63785);
#50776=AXIS2_PLACEMENT_3D('',#127917,#63786,#63787);
#50777=AXIS2_PLACEMENT_3D('',#127920,#63789,#63790);
#50778=AXIS2_PLACEMENT_3D('',#127921,#63791,#63792);
#50779=AXIS2_PLACEMENT_3D('',#127923,#63793,#63794);
#50780=AXIS2_PLACEMENT_3D('',#127926,#63796,#63797);
#50781=AXIS2_PLACEMENT_3D('',#127927,#63798,#63799);
#50782=AXIS2_PLACEMENT_3D('',#127929,#63800,#63801);
#50783=AXIS2_PLACEMENT_3D('',#127932,#63803,#63804);
#50784=AXIS2_PLACEMENT_3D('',#127933,#63805,#63806);
#50785=AXIS2_PLACEMENT_3D('',#127935,#63807,#63808);
#50786=AXIS2_PLACEMENT_3D('',#127938,#63810,#63811);
#50787=AXIS2_PLACEMENT_3D('',#127939,#63812,#63813);
#50788=AXIS2_PLACEMENT_3D('',#127941,#63814,#63815);
#50789=AXIS2_PLACEMENT_3D('',#127944,#63817,#63818);
#50790=AXIS2_PLACEMENT_3D('',#127945,#63819,#63820);
#50791=AXIS2_PLACEMENT_3D('',#127947,#63821,#63822);
#50792=AXIS2_PLACEMENT_3D('',#127950,#63824,#63825);
#50793=AXIS2_PLACEMENT_3D('',#127951,#63826,#63827);
#50794=AXIS2_PLACEMENT_3D('',#127953,#63828,#63829);
#50795=AXIS2_PLACEMENT_3D('',#127956,#63831,#63832);
#50796=AXIS2_PLACEMENT_3D('',#127957,#63833,#63834);
#50797=AXIS2_PLACEMENT_3D('',#127959,#63835,#63836);
#50798=AXIS2_PLACEMENT_3D('',#127962,#63838,#63839);
#50799=AXIS2_PLACEMENT_3D('',#127963,#63840,#63841);
#50800=AXIS2_PLACEMENT_3D('',#127965,#63842,#63843);
#50801=AXIS2_PLACEMENT_3D('',#127968,#63845,#63846);
#50802=AXIS2_PLACEMENT_3D('',#127969,#63847,#63848);
#50803=AXIS2_PLACEMENT_3D('',#127971,#63849,#63850);
#50804=AXIS2_PLACEMENT_3D('',#127974,#63852,#63853);
#50805=AXIS2_PLACEMENT_3D('',#127975,#63854,#63855);
#50806=AXIS2_PLACEMENT_3D('',#127977,#63856,#63857);
#50807=AXIS2_PLACEMENT_3D('',#127980,#63859,#63860);
#50808=AXIS2_PLACEMENT_3D('',#127981,#63861,#63862);
#50809=AXIS2_PLACEMENT_3D('',#127983,#63863,#63864);
#50810=AXIS2_PLACEMENT_3D('',#127986,#63866,#63867);
#50811=AXIS2_PLACEMENT_3D('',#127987,#63868,#63869);
#50812=AXIS2_PLACEMENT_3D('',#127989,#63870,#63871);
#50813=AXIS2_PLACEMENT_3D('',#127992,#63873,#63874);
#50814=AXIS2_PLACEMENT_3D('',#127993,#63875,#63876);
#50815=AXIS2_PLACEMENT_3D('',#127995,#63877,#63878);
#50816=AXIS2_PLACEMENT_3D('',#127998,#63880,#63881);
#50817=AXIS2_PLACEMENT_3D('',#127999,#63882,#63883);
#50818=AXIS2_PLACEMENT_3D('',#128001,#63884,#63885);
#50819=AXIS2_PLACEMENT_3D('',#128004,#63887,#63888);
#50820=AXIS2_PLACEMENT_3D('',#128005,#63889,#63890);
#50821=AXIS2_PLACEMENT_3D('',#128007,#63891,#63892);
#50822=AXIS2_PLACEMENT_3D('',#128010,#63894,#63895);
#50823=AXIS2_PLACEMENT_3D('',#128011,#63896,#63897);
#50824=AXIS2_PLACEMENT_3D('',#128013,#63898,#63899);
#50825=AXIS2_PLACEMENT_3D('',#128016,#63901,#63902);
#50826=AXIS2_PLACEMENT_3D('',#128017,#63903,#63904);
#50827=AXIS2_PLACEMENT_3D('',#128019,#63905,#63906);
#50828=AXIS2_PLACEMENT_3D('',#128022,#63908,#63909);
#50829=AXIS2_PLACEMENT_3D('',#128023,#63910,#63911);
#50830=AXIS2_PLACEMENT_3D('',#128025,#63912,#63913);
#50831=AXIS2_PLACEMENT_3D('',#128028,#63915,#63916);
#50832=AXIS2_PLACEMENT_3D('',#128029,#63917,#63918);
#50833=AXIS2_PLACEMENT_3D('',#128031,#63919,#63920);
#50834=AXIS2_PLACEMENT_3D('',#128034,#63922,#63923);
#50835=AXIS2_PLACEMENT_3D('',#128035,#63924,#63925);
#50836=AXIS2_PLACEMENT_3D('',#128037,#63926,#63927);
#50837=AXIS2_PLACEMENT_3D('',#128040,#63929,#63930);
#50838=AXIS2_PLACEMENT_3D('',#128041,#63931,#63932);
#50839=AXIS2_PLACEMENT_3D('',#128043,#63933,#63934);
#50840=AXIS2_PLACEMENT_3D('',#128046,#63936,#63937);
#50841=AXIS2_PLACEMENT_3D('',#128047,#63938,#63939);
#50842=AXIS2_PLACEMENT_3D('',#128049,#63940,#63941);
#50843=AXIS2_PLACEMENT_3D('',#128052,#63943,#63944);
#50844=AXIS2_PLACEMENT_3D('',#128053,#63945,#63946);
#50845=AXIS2_PLACEMENT_3D('',#128055,#63947,#63948);
#50846=AXIS2_PLACEMENT_3D('',#128058,#63950,#63951);
#50847=AXIS2_PLACEMENT_3D('',#128059,#63952,#63953);
#50848=AXIS2_PLACEMENT_3D('',#128061,#63954,#63955);
#50849=AXIS2_PLACEMENT_3D('',#128064,#63957,#63958);
#50850=AXIS2_PLACEMENT_3D('',#128065,#63959,#63960);
#50851=AXIS2_PLACEMENT_3D('',#128067,#63961,#63962);
#50852=AXIS2_PLACEMENT_3D('',#128070,#63964,#63965);
#50853=AXIS2_PLACEMENT_3D('',#128071,#63966,#63967);
#50854=AXIS2_PLACEMENT_3D('',#128073,#63968,#63969);
#50855=AXIS2_PLACEMENT_3D('',#128076,#63971,#63972);
#50856=AXIS2_PLACEMENT_3D('',#128077,#63973,#63974);
#50857=AXIS2_PLACEMENT_3D('',#128079,#63975,#63976);
#50858=AXIS2_PLACEMENT_3D('',#128082,#63978,#63979);
#50859=AXIS2_PLACEMENT_3D('',#128083,#63980,#63981);
#50860=AXIS2_PLACEMENT_3D('',#128085,#63982,#63983);
#50861=AXIS2_PLACEMENT_3D('',#128088,#63985,#63986);
#50862=AXIS2_PLACEMENT_3D('',#128089,#63987,#63988);
#50863=AXIS2_PLACEMENT_3D('',#128091,#63989,#63990);
#50864=AXIS2_PLACEMENT_3D('',#128094,#63992,#63993);
#50865=AXIS2_PLACEMENT_3D('',#128095,#63994,#63995);
#50866=AXIS2_PLACEMENT_3D('',#128097,#63996,#63997);
#50867=AXIS2_PLACEMENT_3D('',#128100,#63999,#64000);
#50868=AXIS2_PLACEMENT_3D('',#128101,#64001,#64002);
#50869=AXIS2_PLACEMENT_3D('',#128103,#64003,#64004);
#50870=AXIS2_PLACEMENT_3D('',#128106,#64006,#64007);
#50871=AXIS2_PLACEMENT_3D('',#128107,#64008,#64009);
#50872=AXIS2_PLACEMENT_3D('',#128109,#64010,#64011);
#50873=AXIS2_PLACEMENT_3D('',#128112,#64013,#64014);
#50874=AXIS2_PLACEMENT_3D('',#128113,#64015,#64016);
#50875=AXIS2_PLACEMENT_3D('',#128115,#64017,#64018);
#50876=AXIS2_PLACEMENT_3D('',#128118,#64020,#64021);
#50877=AXIS2_PLACEMENT_3D('',#128119,#64022,#64023);
#50878=AXIS2_PLACEMENT_3D('',#128121,#64024,#64025);
#50879=AXIS2_PLACEMENT_3D('',#128124,#64027,#64028);
#50880=AXIS2_PLACEMENT_3D('',#128125,#64029,#64030);
#50881=AXIS2_PLACEMENT_3D('',#128127,#64031,#64032);
#50882=AXIS2_PLACEMENT_3D('',#128130,#64034,#64035);
#50883=AXIS2_PLACEMENT_3D('',#128131,#64036,#64037);
#50884=AXIS2_PLACEMENT_3D('',#128133,#64038,#64039);
#50885=AXIS2_PLACEMENT_3D('',#128136,#64041,#64042);
#50886=AXIS2_PLACEMENT_3D('',#128137,#64043,#64044);
#50887=AXIS2_PLACEMENT_3D('',#128139,#64045,#64046);
#50888=AXIS2_PLACEMENT_3D('',#128140,#64047,#64048);
#50889=AXIS2_PLACEMENT_3D('',#128141,#64049,#64050);
#50890=AXIS2_PLACEMENT_3D('',#128142,#64051,#64052);
#50891=AXIS2_PLACEMENT_3D('',#128145,#64054,#64055);
#50892=AXIS2_PLACEMENT_3D('',#128146,#64056,#64057);
#50893=AXIS2_PLACEMENT_3D('',#128148,#64058,#64059);
#50894=AXIS2_PLACEMENT_3D('',#128150,#64060,#64061);
#50895=AXIS2_PLACEMENT_3D('',#128152,#64062,#64063);
#50896=AXIS2_PLACEMENT_3D('',#128153,#64064,#64065);
#50897=AXIS2_PLACEMENT_3D('',#128154,#64066,#64067);
#50898=AXIS2_PLACEMENT_3D('',#128156,#64068,#64069);
#50899=AXIS2_PLACEMENT_3D('',#128158,#64070,#64071);
#50900=AXIS2_PLACEMENT_3D('',#128159,#64072,#64073);
#50901=AXIS2_PLACEMENT_3D('',#128160,#64074,#64075);
#50902=AXIS2_PLACEMENT_3D('',#128162,#64077,#64078);
#50903=AXIS2_PLACEMENT_3D('',#128164,#64079,#64080);
#50904=AXIS2_PLACEMENT_3D('',#128165,#64081,#64082);
#50905=AXIS2_PLACEMENT_3D('',#128167,#64083,#64084);
#50906=AXIS2_PLACEMENT_3D('',#128169,#64085,#64086);
#50907=AXIS2_PLACEMENT_3D('',#128170,#64087,#64088);
#50908=AXIS2_PLACEMENT_3D('',#128171,#64089,#64090);
#50909=AXIS2_PLACEMENT_3D('',#128173,#64091,#64092);
#50910=AXIS2_PLACEMENT_3D('',#128175,#64093,#64094);
#50911=AXIS2_PLACEMENT_3D('',#128176,#64095,#64096);
#50912=AXIS2_PLACEMENT_3D('',#128177,#64097,#64098);
#50913=AXIS2_PLACEMENT_3D('',#128179,#64099,#64100);
#50914=AXIS2_PLACEMENT_3D('',#128180,#64101,#64102);
#50915=AXIS2_PLACEMENT_3D('',#128181,#64103,#64104);
#50916=AXIS2_PLACEMENT_3D('',#128183,#64105,#64106);
#50917=AXIS2_PLACEMENT_3D('',#128185,#64108,#64109);
#50918=AXIS2_PLACEMENT_3D('',#128188,#64110,#64111);
#50919=AXIS2_PLACEMENT_3D('',#128189,#64112,#64113);
#50920=AXIS2_PLACEMENT_3D('',#128191,#64114,#64115);
#50921=AXIS2_PLACEMENT_3D('',#128192,#64116,#64117);
#50922=AXIS2_PLACEMENT_3D('',#128193,#64118,#64119);
#50923=AXIS2_PLACEMENT_3D('',#128195,#64121,#64122);
#50924=AXIS2_PLACEMENT_3D('',#128222,#64124,#64125);
#50925=AXIS2_PLACEMENT_3D('',#128243,#64126,#64127);
#50926=AXIS2_PLACEMENT_3D('',#128300,#64129,#64130);
#50927=AXIS2_PLACEMENT_3D('',#128301,#64131,#64132);
#50928=AXIS2_PLACEMENT_3D('',#128302,#64133,#64134);
#50929=AXIS2_PLACEMENT_3D('',#128303,#64135,#64136);
#50930=AXIS2_PLACEMENT_3D('',#128304,#64137,#64138);
#50931=AXIS2_PLACEMENT_3D('',#128305,#64139,#64140);
#50932=AXIS2_PLACEMENT_3D('',#128306,#64141,#64142);
#50933=AXIS2_PLACEMENT_3D('',#128307,#64143,#64144);
#50934=AXIS2_PLACEMENT_3D('',#128320,#64145,#64146);
#50935=AXIS2_PLACEMENT_3D('',#128321,#64147,#64148);
#50936=AXIS2_PLACEMENT_3D('',#128322,#64149,#64150);
#50937=AXIS2_PLACEMENT_3D('',#128323,#64151,#64152);
#50938=AXIS2_PLACEMENT_3D('',#128324,#64153,#64154);
#50939=AXIS2_PLACEMENT_3D('',#128325,#64155,#64156);
#50940=AXIS2_PLACEMENT_3D('',#128326,#64157,#64158);
#50941=AXIS2_PLACEMENT_3D('',#128327,#64159,#64160);
#50942=AXIS2_PLACEMENT_3D('',#128328,#64161,#64162);
#50943=AXIS2_PLACEMENT_3D('',#128329,#64163,#64164);
#50944=AXIS2_PLACEMENT_3D('',#128330,#64165,#64166);
#50945=AXIS2_PLACEMENT_3D('',#128331,#64167,#64168);
#50946=AXIS2_PLACEMENT_3D('',#128332,#64169,#64170);
#50947=AXIS2_PLACEMENT_3D('',#128333,#64171,#64172);
#50948=AXIS2_PLACEMENT_3D('',#128334,#64173,#64174);
#50949=AXIS2_PLACEMENT_3D('',#128335,#64175,#64176);
#50950=AXIS2_PLACEMENT_3D('',#128336,#64177,#64178);
#50951=AXIS2_PLACEMENT_3D('',#128337,#64179,#64180);
#50952=AXIS2_PLACEMENT_3D('',#128338,#64181,#64182);
#50953=AXIS2_PLACEMENT_3D('',#128339,#64183,#64184);
#50954=AXIS2_PLACEMENT_3D('',#128340,#64185,#64186);
#50955=AXIS2_PLACEMENT_3D('',#128341,#64187,#64188);
#50956=AXIS2_PLACEMENT_3D('',#128342,#64189,#64190);
#50957=AXIS2_PLACEMENT_3D('',#128343,#64191,#64192);
#50958=AXIS2_PLACEMENT_3D('',#128344,#64193,#64194);
#50959=AXIS2_PLACEMENT_3D('',#128345,#64195,#64196);
#50960=AXIS2_PLACEMENT_3D('',#128346,#64197,#64198);
#50961=AXIS2_PLACEMENT_3D('',#128347,#64199,#64200);
#50962=AXIS2_PLACEMENT_3D('',#128348,#64201,#64202);
#50963=AXIS2_PLACEMENT_3D('',#128349,#64203,#64204);
#50964=AXIS2_PLACEMENT_3D('',#128350,#64205,#64206);
#50965=AXIS2_PLACEMENT_3D('',#128351,#64207,#64208);
#50966=AXIS2_PLACEMENT_3D('',#128352,#64209,#64210);
#50967=AXIS2_PLACEMENT_3D('',#128353,#64211,#64212);
#50968=AXIS2_PLACEMENT_3D('',#128354,#64213,#64214);
#50969=AXIS2_PLACEMENT_3D('',#128355,#64215,#64216);
#50970=AXIS2_PLACEMENT_3D('',#128356,#64217,#64218);
#50971=AXIS2_PLACEMENT_3D('',#128357,#64219,#64220);
#50972=AXIS2_PLACEMENT_3D('',#128358,#64221,#64222);
#50973=AXIS2_PLACEMENT_3D('',#128359,#64223,#64224);
#50974=AXIS2_PLACEMENT_3D('',#128360,#64225,#64226);
#50975=AXIS2_PLACEMENT_3D('',#128361,#64227,#64228);
#50976=AXIS2_PLACEMENT_3D('',#128362,#64229,#64230);
#50977=AXIS2_PLACEMENT_3D('',#128363,#64231,#64232);
#50978=AXIS2_PLACEMENT_3D('',#128364,#64233,#64234);
#50979=AXIS2_PLACEMENT_3D('',#128365,#64235,#64236);
#50980=AXIS2_PLACEMENT_3D('',#128366,#64237,#64238);
#50981=AXIS2_PLACEMENT_3D('',#128367,#64239,#64240);
#50982=AXIS2_PLACEMENT_3D('',#128368,#64241,#64242);
#50983=AXIS2_PLACEMENT_3D('',#128369,#64243,#64244);
#50984=AXIS2_PLACEMENT_3D('',#128370,#64245,#64246);
#50985=AXIS2_PLACEMENT_3D('',#128371,#64247,#64248);
#50986=AXIS2_PLACEMENT_3D('',#128372,#64249,#64250);
#50987=AXIS2_PLACEMENT_3D('',#128373,#64251,#64252);
#50988=AXIS2_PLACEMENT_3D('',#128374,#64253,#64254);
#50989=AXIS2_PLACEMENT_3D('',#128375,#64255,#64256);
#50990=AXIS2_PLACEMENT_3D('',#128376,#64257,#64258);
#50991=AXIS2_PLACEMENT_3D('',#128377,#64259,#64260);
#50992=AXIS2_PLACEMENT_3D('',#128378,#64261,#64262);
#50993=AXIS2_PLACEMENT_3D('',#128379,#64263,#64264);
#50994=AXIS2_PLACEMENT_3D('',#128380,#64265,#64266);
#50995=AXIS2_PLACEMENT_3D('',#128381,#64267,#64268);
#50996=AXIS2_PLACEMENT_3D('',#128382,#64269,#64270);
#50997=AXIS2_PLACEMENT_3D('',#128383,#64271,#64272);
#50998=AXIS2_PLACEMENT_3D('',#128384,#64273,#64274);
#50999=AXIS2_PLACEMENT_3D('',#128385,#64275,#64276);
#51000=AXIS2_PLACEMENT_3D('',#128386,#64277,#64278);
#51001=AXIS2_PLACEMENT_3D('',#128387,#64279,#64280);
#51002=AXIS2_PLACEMENT_3D('',#128388,#64281,#64282);
#51003=AXIS2_PLACEMENT_3D('',#128389,#64283,#64284);
#51004=AXIS2_PLACEMENT_3D('',#128390,#64285,#64286);
#51005=AXIS2_PLACEMENT_3D('',#128391,#64287,#64288);
#51006=AXIS2_PLACEMENT_3D('',#128392,#64289,#64290);
#51007=AXIS2_PLACEMENT_3D('',#128393,#64291,#64292);
#51008=AXIS2_PLACEMENT_3D('',#128394,#64293,#64294);
#51009=AXIS2_PLACEMENT_3D('',#128395,#64295,#64296);
#51010=AXIS2_PLACEMENT_3D('',#128396,#64297,#64298);
#51011=AXIS2_PLACEMENT_3D('',#128397,#64299,#64300);
#51012=AXIS2_PLACEMENT_3D('',#128398,#64301,#64302);
#51013=AXIS2_PLACEMENT_3D('',#128399,#64303,#64304);
#51014=AXIS2_PLACEMENT_3D('',#128400,#64305,#64306);
#51015=AXIS2_PLACEMENT_3D('',#128401,#64307,#64308);
#51016=AXIS2_PLACEMENT_3D('',#128402,#64309,#64310);
#51017=AXIS2_PLACEMENT_3D('',#128403,#64311,#64312);
#51018=AXIS2_PLACEMENT_3D('',#128404,#64313,#64314);
#51019=AXIS2_PLACEMENT_3D('',#128405,#64315,#64316);
#51020=AXIS2_PLACEMENT_3D('',#128406,#64317,#64318);
#51021=AXIS2_PLACEMENT_3D('',#128407,#64319,#64320);
#51022=AXIS2_PLACEMENT_3D('',#128408,#64321,#64322);
#51023=AXIS2_PLACEMENT_3D('',#128409,#64323,#64324);
#51024=AXIS2_PLACEMENT_3D('',#128410,#64325,#64326);
#51025=AXIS2_PLACEMENT_3D('',#128411,#64327,#64328);
#51026=AXIS2_PLACEMENT_3D('',#128412,#64329,#64330);
#51027=AXIS2_PLACEMENT_3D('',#128413,#64331,#64332);
#51028=AXIS2_PLACEMENT_3D('',#128414,#64333,#64334);
#51029=AXIS2_PLACEMENT_3D('',#128415,#64335,#64336);
#51030=AXIS2_PLACEMENT_3D('',#128416,#64337,#64338);
#51031=AXIS2_PLACEMENT_3D('',#128417,#64339,#64340);
#51032=AXIS2_PLACEMENT_3D('',#128418,#64341,#64342);
#51033=AXIS2_PLACEMENT_3D('',#128419,#64343,#64344);
#51034=AXIS2_PLACEMENT_3D('',#128420,#64345,#64346);
#51035=AXIS2_PLACEMENT_3D('',#128421,#64347,#64348);
#51036=AXIS2_PLACEMENT_3D('',#128422,#64349,#64350);
#51037=AXIS2_PLACEMENT_3D('',#128423,#64351,#64352);
#51038=AXIS2_PLACEMENT_3D('',#128424,#64353,#64354);
#51039=AXIS2_PLACEMENT_3D('',#128425,#64355,#64356);
#51040=AXIS2_PLACEMENT_3D('',#128426,#64357,#64358);
#51041=AXIS2_PLACEMENT_3D('',#128427,#64359,#64360);
#51042=AXIS2_PLACEMENT_3D('',#128428,#64361,#64362);
#51043=AXIS2_PLACEMENT_3D('',#128429,#64363,#64364);
#51044=AXIS2_PLACEMENT_3D('',#128430,#64365,#64366);
#51045=AXIS2_PLACEMENT_3D('',#128431,#64367,#64368);
#51046=AXIS2_PLACEMENT_3D('',#128432,#64369,#64370);
#51047=AXIS2_PLACEMENT_3D('',#128433,#64371,#64372);
#51048=AXIS2_PLACEMENT_3D('',#128434,#64373,#64374);
#51049=AXIS2_PLACEMENT_3D('',#128435,#64375,#64376);
#51050=AXIS2_PLACEMENT_3D('',#128436,#64377,#64378);
#51051=AXIS2_PLACEMENT_3D('',#128437,#64379,#64380);
#51052=AXIS2_PLACEMENT_3D('',#128438,#64381,#64382);
#51053=AXIS2_PLACEMENT_3D('',#128439,#64383,#64384);
#51054=AXIS2_PLACEMENT_3D('',#128440,#64385,#64386);
#51055=AXIS2_PLACEMENT_3D('',#128441,#64387,#64388);
#51056=AXIS2_PLACEMENT_3D('',#128442,#64389,#64390);
#51057=AXIS2_PLACEMENT_3D('',#128443,#64391,#64392);
#51058=AXIS2_PLACEMENT_3D('',#128444,#64393,#64394);
#51059=AXIS2_PLACEMENT_3D('',#128445,#64395,#64396);
#51060=AXIS2_PLACEMENT_3D('',#128446,#64397,#64398);
#51061=AXIS2_PLACEMENT_3D('',#128447,#64399,#64400);
#51062=AXIS2_PLACEMENT_3D('',#128448,#64401,#64402);
#51063=AXIS2_PLACEMENT_3D('',#128449,#64403,#64404);
#51064=AXIS2_PLACEMENT_3D('',#128450,#64405,#64406);
#51065=AXIS2_PLACEMENT_3D('',#128451,#64407,#64408);
#51066=AXIS2_PLACEMENT_3D('',#128452,#64409,#64410);
#51067=AXIS2_PLACEMENT_3D('',#128453,#64411,#64412);
#51068=AXIS2_PLACEMENT_3D('',#128454,#64413,#64414);
#51069=AXIS2_PLACEMENT_3D('',#128455,#64415,#64416);
#51070=AXIS2_PLACEMENT_3D('',#128456,#64417,#64418);
#51071=AXIS2_PLACEMENT_3D('',#128457,#64419,#64420);
#51072=AXIS2_PLACEMENT_3D('',#128458,#64421,#64422);
#51073=AXIS2_PLACEMENT_3D('',#128459,#64423,#64424);
#51074=AXIS2_PLACEMENT_3D('',#128460,#64425,#64426);
#51075=AXIS2_PLACEMENT_3D('',#128461,#64427,#64428);
#51076=AXIS2_PLACEMENT_3D('',#128462,#64429,#64430);
#51077=AXIS2_PLACEMENT_3D('',#128463,#64431,#64432);
#51078=AXIS2_PLACEMENT_3D('',#128464,#64433,#64434);
#51079=AXIS2_PLACEMENT_3D('',#128465,#64435,#64436);
#51080=AXIS2_PLACEMENT_3D('',#128466,#64437,#64438);
#51081=AXIS2_PLACEMENT_3D('',#128467,#64439,#64440);
#51082=AXIS2_PLACEMENT_3D('',#128468,#64441,#64442);
#51083=AXIS2_PLACEMENT_3D('',#128469,#64443,#64444);
#51084=AXIS2_PLACEMENT_3D('',#128470,#64445,#64446);
#51085=AXIS2_PLACEMENT_3D('',#128471,#64447,#64448);
#51086=AXIS2_PLACEMENT_3D('',#128472,#64449,#64450);
#51087=AXIS2_PLACEMENT_3D('',#128473,#64451,#64452);
#51088=AXIS2_PLACEMENT_3D('',#128474,#64453,#64454);
#51089=AXIS2_PLACEMENT_3D('',#128475,#64455,#64456);
#51090=AXIS2_PLACEMENT_3D('',#128476,#64457,#64458);
#51091=AXIS2_PLACEMENT_3D('',#128477,#64459,#64460);
#51092=AXIS2_PLACEMENT_3D('',#128478,#64461,#64462);
#51093=AXIS2_PLACEMENT_3D('',#128479,#64463,#64464);
#51094=AXIS2_PLACEMENT_3D('',#128480,#64465,#64466);
#51095=AXIS2_PLACEMENT_3D('',#128481,#64467,#64468);
#51096=AXIS2_PLACEMENT_3D('',#128482,#64469,#64470);
#51097=AXIS2_PLACEMENT_3D('',#128483,#64471,#64472);
#51098=AXIS2_PLACEMENT_3D('',#128484,#64473,#64474);
#51099=AXIS2_PLACEMENT_3D('',#128485,#64475,#64476);
#51100=AXIS2_PLACEMENT_3D('',#128486,#64477,#64478);
#51101=AXIS2_PLACEMENT_3D('',#128487,#64479,#64480);
#51102=AXIS2_PLACEMENT_3D('',#128488,#64481,#64482);
#51103=AXIS2_PLACEMENT_3D('',#128489,#64483,#64484);
#51104=AXIS2_PLACEMENT_3D('',#128490,#64485,#64486);
#51105=AXIS2_PLACEMENT_3D('',#128491,#64487,#64488);
#51106=AXIS2_PLACEMENT_3D('',#128492,#64489,#64490);
#51107=AXIS2_PLACEMENT_3D('',#128493,#64491,#64492);
#51108=AXIS2_PLACEMENT_3D('',#128494,#64493,#64494);
#51109=AXIS2_PLACEMENT_3D('',#128495,#64495,#64496);
#51110=AXIS2_PLACEMENT_3D('',#128496,#64497,#64498);
#51111=AXIS2_PLACEMENT_3D('',#128497,#64499,#64500);
#51112=AXIS2_PLACEMENT_3D('',#128498,#64501,#64502);
#51113=AXIS2_PLACEMENT_3D('',#128499,#64503,#64504);
#51114=AXIS2_PLACEMENT_3D('',#128500,#64505,#64506);
#51115=AXIS2_PLACEMENT_3D('',#128501,#64507,#64508);
#51116=AXIS2_PLACEMENT_3D('',#128502,#64509,#64510);
#51117=AXIS2_PLACEMENT_3D('',#128503,#64511,#64512);
#51118=AXIS2_PLACEMENT_3D('',#128504,#64513,#64514);
#51119=AXIS2_PLACEMENT_3D('',#128505,#64515,#64516);
#51120=AXIS2_PLACEMENT_3D('',#128506,#64517,#64518);
#51121=AXIS2_PLACEMENT_3D('',#128507,#64519,#64520);
#51122=AXIS2_PLACEMENT_3D('',#128508,#64521,#64522);
#51123=AXIS2_PLACEMENT_3D('',#128509,#64523,#64524);
#51124=AXIS2_PLACEMENT_3D('',#128510,#64525,#64526);
#51125=AXIS2_PLACEMENT_3D('',#128511,#64527,#64528);
#51126=AXIS2_PLACEMENT_3D('',#128512,#64529,#64530);
#51127=AXIS2_PLACEMENT_3D('',#128513,#64531,#64532);
#51128=AXIS2_PLACEMENT_3D('',#128514,#64533,#64534);
#51129=AXIS2_PLACEMENT_3D('',#128515,#64535,#64536);
#51130=AXIS2_PLACEMENT_3D('',#128516,#64537,#64538);
#51131=AXIS2_PLACEMENT_3D('',#128517,#64539,#64540);
#51132=AXIS2_PLACEMENT_3D('',#128518,#64541,#64542);
#51133=AXIS2_PLACEMENT_3D('',#128519,#64543,#64544);
#51134=AXIS2_PLACEMENT_3D('',#128520,#64545,#64546);
#51135=AXIS2_PLACEMENT_3D('',#128521,#64547,#64548);
#51136=AXIS2_PLACEMENT_3D('',#128522,#64549,#64550);
#51137=AXIS2_PLACEMENT_3D('',#128523,#64551,#64552);
#51138=AXIS2_PLACEMENT_3D('',#128524,#64553,#64554);
#51139=AXIS2_PLACEMENT_3D('',#128525,#64555,#64556);
#51140=AXIS2_PLACEMENT_3D('',#128526,#64557,#64558);
#51141=AXIS2_PLACEMENT_3D('',#128527,#64559,#64560);
#51142=AXIS2_PLACEMENT_3D('',#128528,#64561,#64562);
#51143=AXIS2_PLACEMENT_3D('',#128529,#64563,#64564);
#51144=AXIS2_PLACEMENT_3D('',#128530,#64565,#64566);
#51145=AXIS2_PLACEMENT_3D('',#128531,#64567,#64568);
#51146=AXIS2_PLACEMENT_3D('',#128532,#64569,#64570);
#51147=AXIS2_PLACEMENT_3D('',#128533,#64571,#64572);
#51148=AXIS2_PLACEMENT_3D('',#128534,#64573,#64574);
#51149=AXIS2_PLACEMENT_3D('',#128535,#64575,#64576);
#51150=AXIS2_PLACEMENT_3D('',#128536,#64577,#64578);
#51151=AXIS2_PLACEMENT_3D('',#128537,#64579,#64580);
#51152=AXIS2_PLACEMENT_3D('',#128538,#64581,#64582);
#51153=AXIS2_PLACEMENT_3D('',#128539,#64583,#64584);
#51154=AXIS2_PLACEMENT_3D('',#128540,#64585,#64586);
#51155=AXIS2_PLACEMENT_3D('',#128541,#64587,#64588);
#51156=AXIS2_PLACEMENT_3D('',#128542,#64589,#64590);
#51157=AXIS2_PLACEMENT_3D('',#128543,#64591,#64592);
#51158=AXIS2_PLACEMENT_3D('',#128544,#64593,#64594);
#51159=AXIS2_PLACEMENT_3D('',#128545,#64595,#64596);
#51160=AXIS2_PLACEMENT_3D('',#128546,#64597,#64598);
#51161=AXIS2_PLACEMENT_3D('',#128547,#64599,#64600);
#51162=AXIS2_PLACEMENT_3D('',#128548,#64601,#64602);
#51163=AXIS2_PLACEMENT_3D('',#128549,#64603,#64604);
#51164=AXIS2_PLACEMENT_3D('',#128550,#64605,#64606);
#51165=AXIS2_PLACEMENT_3D('',#128551,#64607,#64608);
#51166=AXIS2_PLACEMENT_3D('',#128552,#64609,#64610);
#51167=AXIS2_PLACEMENT_3D('',#128553,#64611,#64612);
#51168=AXIS2_PLACEMENT_3D('',#128554,#64613,#64614);
#51169=AXIS2_PLACEMENT_3D('',#128555,#64615,#64616);
#51170=AXIS2_PLACEMENT_3D('',#128556,#64617,#64618);
#51171=AXIS2_PLACEMENT_3D('',#128557,#64619,#64620);
#51172=AXIS2_PLACEMENT_3D('',#128558,#64621,#64622);
#51173=AXIS2_PLACEMENT_3D('',#128559,#64623,#64624);
#51174=AXIS2_PLACEMENT_3D('',#128560,#64625,#64626);
#51175=AXIS2_PLACEMENT_3D('',#128561,#64627,#64628);
#51176=AXIS2_PLACEMENT_3D('',#128562,#64629,#64630);
#51177=AXIS2_PLACEMENT_3D('',#128563,#64631,#64632);
#51178=AXIS2_PLACEMENT_3D('',#128564,#64633,#64634);
#51179=AXIS2_PLACEMENT_3D('',#128565,#64635,#64636);
#51180=AXIS2_PLACEMENT_3D('',#128566,#64637,#64638);
#51181=AXIS2_PLACEMENT_3D('',#128567,#64639,#64640);
#51182=AXIS2_PLACEMENT_3D('',#128568,#64641,#64642);
#51183=AXIS2_PLACEMENT_3D('',#128569,#64643,#64644);
#51184=AXIS2_PLACEMENT_3D('',#128570,#64645,#64646);
#51185=AXIS2_PLACEMENT_3D('',#128571,#64647,#64648);
#51186=AXIS2_PLACEMENT_3D('',#128572,#64649,#64650);
#51187=AXIS2_PLACEMENT_3D('',#128573,#64651,#64652);
#51188=AXIS2_PLACEMENT_3D('',#128574,#64653,#64654);
#51189=AXIS2_PLACEMENT_3D('',#128575,#64655,#64656);
#51190=AXIS2_PLACEMENT_3D('',#128576,#64657,#64658);
#51191=AXIS2_PLACEMENT_3D('',#128577,#64659,#64660);
#51192=AXIS2_PLACEMENT_3D('',#128578,#64661,#64662);
#51193=AXIS2_PLACEMENT_3D('',#128579,#64663,#64664);
#51194=AXIS2_PLACEMENT_3D('',#128580,#64665,#64666);
#51195=AXIS2_PLACEMENT_3D('',#128581,#64667,#64668);
#51196=AXIS2_PLACEMENT_3D('',#128582,#64669,#64670);
#51197=AXIS2_PLACEMENT_3D('',#128583,#64671,#64672);
#51198=AXIS2_PLACEMENT_3D('',#128584,#64673,#64674);
#51199=AXIS2_PLACEMENT_3D('',#128585,#64675,#64676);
#51200=AXIS2_PLACEMENT_3D('',#128586,#64677,#64678);
#51201=AXIS2_PLACEMENT_3D('',#128587,#64679,#64680);
#51202=AXIS2_PLACEMENT_3D('',#128588,#64681,#64682);
#51203=AXIS2_PLACEMENT_3D('',#128589,#64683,#64684);
#51204=AXIS2_PLACEMENT_3D('',#128590,#64685,#64686);
#51205=AXIS2_PLACEMENT_3D('',#128591,#64687,#64688);
#51206=AXIS2_PLACEMENT_3D('',#128592,#64689,#64690);
#51207=AXIS2_PLACEMENT_3D('',#128593,#64691,#64692);
#51208=AXIS2_PLACEMENT_3D('',#128594,#64693,#64694);
#51209=AXIS2_PLACEMENT_3D('',#128595,#64695,#64696);
#51210=AXIS2_PLACEMENT_3D('',#128596,#64697,#64698);
#51211=AXIS2_PLACEMENT_3D('',#128597,#64699,#64700);
#51212=AXIS2_PLACEMENT_3D('',#128598,#64701,#64702);
#51213=AXIS2_PLACEMENT_3D('',#128599,#64703,#64704);
#51214=AXIS2_PLACEMENT_3D('',#128600,#64705,#64706);
#51215=AXIS2_PLACEMENT_3D('',#128601,#64707,#64708);
#51216=AXIS2_PLACEMENT_3D('',#128602,#64709,#64710);
#51217=AXIS2_PLACEMENT_3D('',#128603,#64711,#64712);
#51218=AXIS2_PLACEMENT_3D('',#128604,#64713,#64714);
#51219=AXIS2_PLACEMENT_3D('',#128605,#64715,#64716);
#51220=AXIS2_PLACEMENT_3D('',#128606,#64717,#64718);
#51221=AXIS2_PLACEMENT_3D('',#128607,#64719,#64720);
#51222=AXIS2_PLACEMENT_3D('',#128608,#64721,#64722);
#51223=AXIS2_PLACEMENT_3D('',#128609,#64723,#64724);
#51224=AXIS2_PLACEMENT_3D('',#128610,#64725,#64726);
#51225=AXIS2_PLACEMENT_3D('',#128611,#64727,#64728);
#51226=AXIS2_PLACEMENT_3D('',#128612,#64729,#64730);
#51227=AXIS2_PLACEMENT_3D('',#128613,#64731,#64732);
#51228=AXIS2_PLACEMENT_3D('',#128614,#64733,#64734);
#51229=AXIS2_PLACEMENT_3D('',#128615,#64735,#64736);
#51230=AXIS2_PLACEMENT_3D('',#128616,#64737,#64738);
#51231=AXIS2_PLACEMENT_3D('',#128617,#64739,#64740);
#51232=AXIS2_PLACEMENT_3D('',#128618,#64741,#64742);
#51233=AXIS2_PLACEMENT_3D('',#128619,#64743,#64744);
#51234=AXIS2_PLACEMENT_3D('',#128620,#64745,#64746);
#51235=AXIS2_PLACEMENT_3D('',#128621,#64747,#64748);
#51236=AXIS2_PLACEMENT_3D('',#128622,#64749,#64750);
#51237=AXIS2_PLACEMENT_3D('',#128623,#64751,#64752);
#51238=AXIS2_PLACEMENT_3D('',#128624,#64753,#64754);
#51239=AXIS2_PLACEMENT_3D('',#128625,#64755,#64756);
#51240=AXIS2_PLACEMENT_3D('',#128626,#64757,#64758);
#51241=AXIS2_PLACEMENT_3D('',#128627,#64759,#64760);
#51242=AXIS2_PLACEMENT_3D('',#128628,#64761,#64762);
#51243=AXIS2_PLACEMENT_3D('',#128629,#64763,#64764);
#51244=AXIS2_PLACEMENT_3D('',#128630,#64765,#64766);
#51245=AXIS2_PLACEMENT_3D('',#128631,#64767,#64768);
#51246=AXIS2_PLACEMENT_3D('',#128632,#64769,#64770);
#51247=AXIS2_PLACEMENT_3D('',#128633,#64771,#64772);
#51248=AXIS2_PLACEMENT_3D('',#128634,#64773,#64774);
#51249=AXIS2_PLACEMENT_3D('',#128635,#64775,#64776);
#51250=AXIS2_PLACEMENT_3D('',#128636,#64777,#64778);
#51251=AXIS2_PLACEMENT_3D('',#128637,#64779,#64780);
#51252=AXIS2_PLACEMENT_3D('',#128638,#64781,#64782);
#51253=AXIS2_PLACEMENT_3D('',#128639,#64783,#64784);
#51254=AXIS2_PLACEMENT_3D('',#128640,#64785,#64786);
#51255=AXIS2_PLACEMENT_3D('',#128641,#64787,#64788);
#51256=AXIS2_PLACEMENT_3D('',#128642,#64789,#64790);
#51257=AXIS2_PLACEMENT_3D('',#128643,#64791,#64792);
#51258=AXIS2_PLACEMENT_3D('',#128644,#64793,#64794);
#51259=AXIS2_PLACEMENT_3D('',#128645,#64795,#64796);
#51260=AXIS2_PLACEMENT_3D('',#128646,#64797,#64798);
#51261=AXIS2_PLACEMENT_3D('',#128647,#64799,#64800);
#51262=AXIS2_PLACEMENT_3D('',#128648,#64801,#64802);
#51263=AXIS2_PLACEMENT_3D('',#128649,#64803,#64804);
#51264=AXIS2_PLACEMENT_3D('',#128650,#64805,#64806);
#51265=AXIS2_PLACEMENT_3D('',#128651,#64807,#64808);
#51266=AXIS2_PLACEMENT_3D('',#128652,#64809,#64810);
#51267=AXIS2_PLACEMENT_3D('',#128653,#64811,#64812);
#51268=AXIS2_PLACEMENT_3D('',#128654,#64813,#64814);
#51269=AXIS2_PLACEMENT_3D('',#128655,#64815,#64816);
#51270=AXIS2_PLACEMENT_3D('',#128656,#64817,#64818);
#51271=AXIS2_PLACEMENT_3D('',#128657,#64819,#64820);
#51272=AXIS2_PLACEMENT_3D('',#128658,#64821,#64822);
#51273=AXIS2_PLACEMENT_3D('',#128659,#64823,#64824);
#51274=AXIS2_PLACEMENT_3D('',#128660,#64825,#64826);
#51275=AXIS2_PLACEMENT_3D('',#128661,#64827,#64828);
#51276=AXIS2_PLACEMENT_3D('',#128662,#64829,#64830);
#51277=AXIS2_PLACEMENT_3D('',#128663,#64831,#64832);
#51278=AXIS2_PLACEMENT_3D('',#128664,#64833,#64834);
#51279=AXIS2_PLACEMENT_3D('',#128665,#64835,#64836);
#51280=AXIS2_PLACEMENT_3D('',#128666,#64837,#64838);
#51281=AXIS2_PLACEMENT_3D('',#128667,#64839,#64840);
#51282=AXIS2_PLACEMENT_3D('',#128668,#64841,#64842);
#51283=AXIS2_PLACEMENT_3D('',#128669,#64843,#64844);
#51284=AXIS2_PLACEMENT_3D('',#128670,#64845,#64846);
#51285=AXIS2_PLACEMENT_3D('',#128671,#64847,#64848);
#51286=AXIS2_PLACEMENT_3D('',#128672,#64849,#64850);
#51287=AXIS2_PLACEMENT_3D('',#128673,#64851,#64852);
#51288=AXIS2_PLACEMENT_3D('',#128674,#64853,#64854);
#51289=AXIS2_PLACEMENT_3D('',#128675,#64855,#64856);
#51290=AXIS2_PLACEMENT_3D('',#128676,#64857,#64858);
#51291=AXIS2_PLACEMENT_3D('',#128677,#64859,#64860);
#51292=AXIS2_PLACEMENT_3D('',#128678,#64861,#64862);
#51293=AXIS2_PLACEMENT_3D('',#128679,#64863,#64864);
#51294=AXIS2_PLACEMENT_3D('',#128680,#64865,#64866);
#51295=AXIS2_PLACEMENT_3D('',#128681,#64867,#64868);
#51296=AXIS2_PLACEMENT_3D('',#128682,#64869,#64870);
#51297=AXIS2_PLACEMENT_3D('',#128683,#64871,#64872);
#51298=AXIS2_PLACEMENT_3D('',#128684,#64873,#64874);
#51299=AXIS2_PLACEMENT_3D('',#128685,#64875,#64876);
#51300=AXIS2_PLACEMENT_3D('',#128686,#64877,#64878);
#51301=AXIS2_PLACEMENT_3D('',#128687,#64879,#64880);
#51302=AXIS2_PLACEMENT_3D('',#128688,#64881,#64882);
#51303=AXIS2_PLACEMENT_3D('',#128689,#64883,#64884);
#51304=AXIS2_PLACEMENT_3D('',#128690,#64885,#64886);
#51305=AXIS2_PLACEMENT_3D('',#128691,#64887,#64888);
#51306=AXIS2_PLACEMENT_3D('',#128692,#64889,#64890);
#51307=AXIS2_PLACEMENT_3D('',#128693,#64891,#64892);
#51308=AXIS2_PLACEMENT_3D('',#128694,#64893,#64894);
#51309=AXIS2_PLACEMENT_3D('',#128695,#64895,#64896);
#51310=AXIS2_PLACEMENT_3D('',#128696,#64897,#64898);
#51311=AXIS2_PLACEMENT_3D('',#128697,#64899,#64900);
#51312=AXIS2_PLACEMENT_3D('',#128698,#64901,#64902);
#51313=AXIS2_PLACEMENT_3D('',#128699,#64903,#64904);
#51314=AXIS2_PLACEMENT_3D('',#128700,#64905,#64906);
#51315=AXIS2_PLACEMENT_3D('',#128701,#64907,#64908);
#51316=AXIS2_PLACEMENT_3D('',#128702,#64909,#64910);
#51317=AXIS2_PLACEMENT_3D('',#128703,#64911,#64912);
#51318=AXIS2_PLACEMENT_3D('',#128704,#64913,#64914);
#51319=AXIS2_PLACEMENT_3D('',#128705,#64915,#64916);
#51320=AXIS2_PLACEMENT_3D('',#128706,#64917,#64918);
#51321=AXIS2_PLACEMENT_3D('',#128707,#64919,#64920);
#51322=AXIS2_PLACEMENT_3D('',#128708,#64921,#64922);
#51323=AXIS2_PLACEMENT_3D('',#128709,#64923,#64924);
#51324=AXIS2_PLACEMENT_3D('',#128710,#64925,#64926);
#51325=AXIS2_PLACEMENT_3D('',#128711,#64927,#64928);
#51326=AXIS2_PLACEMENT_3D('',#128712,#64929,#64930);
#51327=AXIS2_PLACEMENT_3D('',#128713,#64931,#64932);
#51328=AXIS2_PLACEMENT_3D('',#128714,#64933,#64934);
#51329=AXIS2_PLACEMENT_3D('',#128715,#64935,#64936);
#51330=AXIS2_PLACEMENT_3D('',#128716,#64937,#64938);
#51331=AXIS2_PLACEMENT_3D('',#128717,#64939,#64940);
#51332=AXIS2_PLACEMENT_3D('',#128718,#64941,#64942);
#51333=AXIS2_PLACEMENT_3D('',#128719,#64943,#64944);
#51334=AXIS2_PLACEMENT_3D('',#128720,#64945,#64946);
#51335=AXIS2_PLACEMENT_3D('',#128721,#64947,#64948);
#51336=AXIS2_PLACEMENT_3D('',#128722,#64949,#64950);
#51337=AXIS2_PLACEMENT_3D('',#128723,#64951,#64952);
#51338=AXIS2_PLACEMENT_3D('',#128724,#64953,#64954);
#51339=AXIS2_PLACEMENT_3D('',#128725,#64955,#64956);
#51340=AXIS2_PLACEMENT_3D('',#128726,#64957,#64958);
#51341=AXIS2_PLACEMENT_3D('',#128727,#64959,#64960);
#51342=AXIS2_PLACEMENT_3D('',#128728,#64961,#64962);
#51343=AXIS2_PLACEMENT_3D('',#128729,#64963,#64964);
#51344=AXIS2_PLACEMENT_3D('',#128730,#64965,#64966);
#51345=AXIS2_PLACEMENT_3D('',#128731,#64967,#64968);
#51346=AXIS2_PLACEMENT_3D('',#128732,#64969,#64970);
#51347=AXIS2_PLACEMENT_3D('',#128733,#64971,#64972);
#51348=AXIS2_PLACEMENT_3D('',#128734,#64973,#64974);
#51349=AXIS2_PLACEMENT_3D('',#128735,#64975,#64976);
#51350=AXIS2_PLACEMENT_3D('',#128736,#64977,#64978);
#51351=AXIS2_PLACEMENT_3D('',#128737,#64979,#64980);
#51352=AXIS2_PLACEMENT_3D('',#128738,#64981,#64982);
#51353=AXIS2_PLACEMENT_3D('',#128739,#64983,#64984);
#51354=AXIS2_PLACEMENT_3D('',#128740,#64985,#64986);
#51355=AXIS2_PLACEMENT_3D('',#128741,#64987,#64988);
#51356=AXIS2_PLACEMENT_3D('',#128742,#64989,#64990);
#51357=AXIS2_PLACEMENT_3D('',#128743,#64991,#64992);
#51358=AXIS2_PLACEMENT_3D('',#128744,#64993,#64994);
#51359=AXIS2_PLACEMENT_3D('',#128745,#64995,#64996);
#51360=AXIS2_PLACEMENT_3D('',#128746,#64997,#64998);
#51361=AXIS2_PLACEMENT_3D('',#128747,#64999,#65000);
#51362=AXIS2_PLACEMENT_3D('',#128748,#65001,#65002);
#51363=AXIS2_PLACEMENT_3D('',#128749,#65003,#65004);
#51364=AXIS2_PLACEMENT_3D('',#128750,#65005,#65006);
#51365=AXIS2_PLACEMENT_3D('',#128751,#65007,#65008);
#51366=AXIS2_PLACEMENT_3D('',#128752,#65009,#65010);
#51367=AXIS2_PLACEMENT_3D('',#128753,#65011,#65012);
#51368=AXIS2_PLACEMENT_3D('',#128754,#65013,#65014);
#51369=AXIS2_PLACEMENT_3D('',#128755,#65015,#65016);
#51370=AXIS2_PLACEMENT_3D('',#128756,#65017,#65018);
#51371=AXIS2_PLACEMENT_3D('',#128757,#65019,#65020);
#51372=AXIS2_PLACEMENT_3D('',#128758,#65021,#65022);
#51373=AXIS2_PLACEMENT_3D('',#128759,#65023,#65024);
#51374=AXIS2_PLACEMENT_3D('',#128760,#65025,#65026);
#51375=AXIS2_PLACEMENT_3D('',#128761,#65027,#65028);
#51376=AXIS2_PLACEMENT_3D('',#128762,#65029,#65030);
#51377=AXIS2_PLACEMENT_3D('',#128763,#65031,#65032);
#51378=AXIS2_PLACEMENT_3D('',#128764,#65033,#65034);
#51379=AXIS2_PLACEMENT_3D('',#128765,#65035,#65036);
#51380=AXIS2_PLACEMENT_3D('',#128766,#65037,#65038);
#51381=AXIS2_PLACEMENT_3D('',#128767,#65039,#65040);
#51382=AXIS2_PLACEMENT_3D('',#128768,#65041,#65042);
#51383=AXIS2_PLACEMENT_3D('',#128769,#65043,#65044);
#51384=AXIS2_PLACEMENT_3D('',#128770,#65045,#65046);
#51385=AXIS2_PLACEMENT_3D('',#128771,#65047,#65048);
#51386=AXIS2_PLACEMENT_3D('',#128772,#65049,#65050);
#51387=AXIS2_PLACEMENT_3D('',#128773,#65051,#65052);
#51388=AXIS2_PLACEMENT_3D('',#128774,#65053,#65054);
#51389=AXIS2_PLACEMENT_3D('',#128775,#65055,#65056);
#51390=AXIS2_PLACEMENT_3D('',#128776,#65057,#65058);
#51391=AXIS2_PLACEMENT_3D('',#128777,#65059,#65060);
#51392=AXIS2_PLACEMENT_3D('',#128778,#65061,#65062);
#51393=AXIS2_PLACEMENT_3D('',#128779,#65063,#65064);
#51394=AXIS2_PLACEMENT_3D('',#128780,#65065,#65066);
#51395=AXIS2_PLACEMENT_3D('',#128781,#65067,#65068);
#51396=AXIS2_PLACEMENT_3D('',#128782,#65069,#65070);
#51397=AXIS2_PLACEMENT_3D('',#128783,#65071,#65072);
#51398=AXIS2_PLACEMENT_3D('',#128784,#65073,#65074);
#51399=AXIS2_PLACEMENT_3D('',#128785,#65075,#65076);
#51400=AXIS2_PLACEMENT_3D('',#128786,#65077,#65078);
#51401=AXIS2_PLACEMENT_3D('',#128787,#65079,#65080);
#51402=AXIS2_PLACEMENT_3D('',#128788,#65081,#65082);
#51403=AXIS2_PLACEMENT_3D('',#128789,#65083,#65084);
#51404=AXIS2_PLACEMENT_3D('',#128790,#65085,#65086);
#51405=AXIS2_PLACEMENT_3D('',#128791,#65087,#65088);
#51406=AXIS2_PLACEMENT_3D('',#128792,#65089,#65090);
#51407=AXIS2_PLACEMENT_3D('',#128793,#65091,#65092);
#51408=AXIS2_PLACEMENT_3D('',#128794,#65093,#65094);
#51409=AXIS2_PLACEMENT_3D('',#128795,#65095,#65096);
#51410=AXIS2_PLACEMENT_3D('',#128796,#65097,#65098);
#51411=AXIS2_PLACEMENT_3D('',#128797,#65099,#65100);
#51412=AXIS2_PLACEMENT_3D('',#128798,#65101,#65102);
#51413=AXIS2_PLACEMENT_3D('',#128799,#65103,#65104);
#51414=AXIS2_PLACEMENT_3D('',#128800,#65105,#65106);
#51415=AXIS2_PLACEMENT_3D('',#128801,#65107,#65108);
#51416=AXIS2_PLACEMENT_3D('',#128802,#65109,#65110);
#51417=AXIS2_PLACEMENT_3D('',#128803,#65111,#65112);
#51418=AXIS2_PLACEMENT_3D('',#128804,#65113,#65114);
#51419=AXIS2_PLACEMENT_3D('',#128805,#65115,#65116);
#51420=AXIS2_PLACEMENT_3D('',#128806,#65117,#65118);
#51421=AXIS2_PLACEMENT_3D('',#128807,#65119,#65120);
#51422=AXIS2_PLACEMENT_3D('',#128808,#65121,#65122);
#51423=AXIS2_PLACEMENT_3D('',#128809,#65123,#65124);
#51424=AXIS2_PLACEMENT_3D('',#128810,#65125,#65126);
#51425=AXIS2_PLACEMENT_3D('',#128811,#65127,#65128);
#51426=AXIS2_PLACEMENT_3D('',#128812,#65129,#65130);
#51427=AXIS2_PLACEMENT_3D('',#128813,#65131,#65132);
#51428=AXIS2_PLACEMENT_3D('',#128814,#65133,#65134);
#51429=AXIS2_PLACEMENT_3D('',#128815,#65135,#65136);
#51430=AXIS2_PLACEMENT_3D('',#128816,#65137,#65138);
#51431=AXIS2_PLACEMENT_3D('',#128817,#65139,#65140);
#51432=AXIS2_PLACEMENT_3D('',#128818,#65141,#65142);
#51433=AXIS2_PLACEMENT_3D('',#128819,#65143,#65144);
#51434=AXIS2_PLACEMENT_3D('',#128820,#65145,#65146);
#51435=AXIS2_PLACEMENT_3D('',#128821,#65147,#65148);
#51436=AXIS2_PLACEMENT_3D('',#128822,#65149,#65150);
#51437=AXIS2_PLACEMENT_3D('',#128823,#65151,#65152);
#51438=AXIS2_PLACEMENT_3D('',#128824,#65153,#65154);
#51439=AXIS2_PLACEMENT_3D('',#128825,#65155,#65156);
#51440=AXIS2_PLACEMENT_3D('',#128826,#65157,#65158);
#51441=AXIS2_PLACEMENT_3D('',#128827,#65159,#65160);
#51442=AXIS2_PLACEMENT_3D('',#128828,#65161,#65162);
#51443=AXIS2_PLACEMENT_3D('',#128829,#65163,#65164);
#51444=AXIS2_PLACEMENT_3D('',#128830,#65165,#65166);
#51445=AXIS2_PLACEMENT_3D('',#128831,#65167,#65168);
#51446=AXIS2_PLACEMENT_3D('',#128832,#65169,#65170);
#51447=AXIS2_PLACEMENT_3D('',#128833,#65171,#65172);
#51448=AXIS2_PLACEMENT_3D('',#128834,#65173,#65174);
#51449=AXIS2_PLACEMENT_3D('',#128835,#65175,#65176);
#51450=AXIS2_PLACEMENT_3D('',#128836,#65177,#65178);
#51451=AXIS2_PLACEMENT_3D('',#128837,#65179,#65180);
#51452=AXIS2_PLACEMENT_3D('',#128838,#65181,#65182);
#51453=AXIS2_PLACEMENT_3D('',#128839,#65183,#65184);
#51454=AXIS2_PLACEMENT_3D('',#128840,#65185,#65186);
#51455=AXIS2_PLACEMENT_3D('',#128841,#65187,#65188);
#51456=AXIS2_PLACEMENT_3D('',#128842,#65189,#65190);
#51457=AXIS2_PLACEMENT_3D('',#128843,#65191,#65192);
#51458=AXIS2_PLACEMENT_3D('',#128844,#65193,#65194);
#51459=AXIS2_PLACEMENT_3D('',#128845,#65195,#65196);
#51460=AXIS2_PLACEMENT_3D('',#128846,#65197,#65198);
#51461=AXIS2_PLACEMENT_3D('',#128847,#65199,#65200);
#51462=AXIS2_PLACEMENT_3D('',#128848,#65201,#65202);
#51463=AXIS2_PLACEMENT_3D('',#128849,#65203,#65204);
#51464=AXIS2_PLACEMENT_3D('',#128850,#65205,#65206);
#51465=AXIS2_PLACEMENT_3D('',#128851,#65207,#65208);
#51466=AXIS2_PLACEMENT_3D('',#128852,#65209,#65210);
#51467=AXIS2_PLACEMENT_3D('',#128853,#65211,#65212);
#51468=AXIS2_PLACEMENT_3D('',#128854,#65213,#65214);
#51469=AXIS2_PLACEMENT_3D('',#128855,#65215,#65216);
#51470=AXIS2_PLACEMENT_3D('',#128856,#65217,#65218);
#51471=AXIS2_PLACEMENT_3D('',#128857,#65219,#65220);
#51472=AXIS2_PLACEMENT_3D('',#128858,#65221,#65222);
#51473=AXIS2_PLACEMENT_3D('',#128859,#65223,#65224);
#51474=AXIS2_PLACEMENT_3D('',#128860,#65225,#65226);
#51475=AXIS2_PLACEMENT_3D('',#128877,#65227,#65228);
#51476=AXIS2_PLACEMENT_3D('',#128894,#65229,#65230);
#51477=AXIS2_PLACEMENT_3D('',#128911,#65231,#65232);
#51478=AXIS2_PLACEMENT_3D('',#128928,#65233,#65234);
#51479=AXIS2_PLACEMENT_3D('',#128945,#65235,#65236);
#51480=AXIS2_PLACEMENT_3D('',#128962,#65237,#65238);
#51481=AXIS2_PLACEMENT_3D('',#128979,#65239,#65240);
#51482=AXIS2_PLACEMENT_3D('',#128996,#65241,#65242);
#51483=AXIS2_PLACEMENT_3D('',#129013,#65243,#65244);
#51484=AXIS2_PLACEMENT_3D('',#129030,#65245,#65246);
#51485=AXIS2_PLACEMENT_3D('',#129047,#65247,#65248);
#51486=AXIS2_PLACEMENT_3D('',#129064,#65249,#65250);
#51487=AXIS2_PLACEMENT_3D('',#129081,#65251,#65252);
#51488=AXIS2_PLACEMENT_3D('',#129098,#65253,#65254);
#51489=AXIS2_PLACEMENT_3D('',#129115,#65255,#65256);
#51490=AXIS2_PLACEMENT_3D('',#129132,#65257,#65258);
#51491=AXIS2_PLACEMENT_3D('',#129149,#65259,#65260);
#51492=AXIS2_PLACEMENT_3D('',#129166,#65261,#65262);
#51493=AXIS2_PLACEMENT_3D('',#129183,#65263,#65264);
#51494=AXIS2_PLACEMENT_3D('',#129200,#65265,#65266);
#51495=AXIS2_PLACEMENT_3D('',#129217,#65267,#65268);
#51496=AXIS2_PLACEMENT_3D('',#129234,#65269,#65270);
#51497=AXIS2_PLACEMENT_3D('',#129251,#65271,#65272);
#51498=AXIS2_PLACEMENT_3D('',#129268,#65273,#65274);
#51499=AXIS2_PLACEMENT_3D('',#129285,#65275,#65276);
#51500=AXIS2_PLACEMENT_3D('',#129302,#65277,#65278);
#51501=AXIS2_PLACEMENT_3D('',#129319,#65279,#65280);
#51502=AXIS2_PLACEMENT_3D('',#129336,#65281,#65282);
#51503=AXIS2_PLACEMENT_3D('',#129353,#65283,#65284);
#51504=AXIS2_PLACEMENT_3D('',#129370,#65285,#65286);
#51505=AXIS2_PLACEMENT_3D('',#129387,#65287,#65288);
#51506=AXIS2_PLACEMENT_3D('',#129404,#65289,#65290);
#51507=AXIS2_PLACEMENT_3D('',#129421,#65291,#65292);
#51508=AXIS2_PLACEMENT_3D('',#129438,#65293,#65294);
#51509=AXIS2_PLACEMENT_3D('',#129455,#65295,#65296);
#51510=AXIS2_PLACEMENT_3D('',#129472,#65297,#65298);
#51511=AXIS2_PLACEMENT_3D('',#129489,#65299,#65300);
#51512=AXIS2_PLACEMENT_3D('',#129506,#65301,#65302);
#51513=AXIS2_PLACEMENT_3D('',#129523,#65303,#65304);
#51514=AXIS2_PLACEMENT_3D('',#129540,#65305,#65306);
#51515=AXIS2_PLACEMENT_3D('',#129557,#65307,#65308);
#51516=AXIS2_PLACEMENT_3D('',#129574,#65309,#65310);
#51517=AXIS2_PLACEMENT_3D('',#129591,#65311,#65312);
#51518=AXIS2_PLACEMENT_3D('',#129608,#65313,#65314);
#51519=AXIS2_PLACEMENT_3D('',#129625,#65315,#65316);
#51520=AXIS2_PLACEMENT_3D('',#129642,#65317,#65318);
#51521=AXIS2_PLACEMENT_3D('',#129659,#65319,#65320);
#51522=AXIS2_PLACEMENT_3D('',#129676,#65321,#65322);
#51523=AXIS2_PLACEMENT_3D('',#129693,#65323,#65324);
#51524=AXIS2_PLACEMENT_3D('',#129710,#65325,#65326);
#51525=AXIS2_PLACEMENT_3D('',#129727,#65327,#65328);
#51526=AXIS2_PLACEMENT_3D('',#129744,#65329,#65330);
#51527=AXIS2_PLACEMENT_3D('',#129761,#65331,#65332);
#51528=AXIS2_PLACEMENT_3D('',#129778,#65333,#65334);
#51529=AXIS2_PLACEMENT_3D('',#129795,#65335,#65336);
#51530=AXIS2_PLACEMENT_3D('',#129812,#65337,#65338);
#51531=AXIS2_PLACEMENT_3D('',#129829,#65339,#65340);
#51532=AXIS2_PLACEMENT_3D('',#129846,#65341,#65342);
#51533=AXIS2_PLACEMENT_3D('',#129863,#65343,#65344);
#51534=AXIS2_PLACEMENT_3D('',#129880,#65345,#65346);
#51535=AXIS2_PLACEMENT_3D('',#129897,#65347,#65348);
#51536=AXIS2_PLACEMENT_3D('',#129914,#65349,#65350);
#51537=AXIS2_PLACEMENT_3D('',#129931,#65351,#65352);
#51538=AXIS2_PLACEMENT_3D('',#129948,#65353,#65354);
#51539=AXIS2_PLACEMENT_3D('',#129965,#65355,#65356);
#51540=AXIS2_PLACEMENT_3D('',#129982,#65357,#65358);
#51541=AXIS2_PLACEMENT_3D('',#129999,#65359,#65360);
#51542=AXIS2_PLACEMENT_3D('',#130016,#65361,#65362);
#51543=AXIS2_PLACEMENT_3D('',#130033,#65363,#65364);
#51544=AXIS2_PLACEMENT_3D('',#130050,#65365,#65366);
#51545=AXIS2_PLACEMENT_3D('',#130067,#65367,#65368);
#51546=AXIS2_PLACEMENT_3D('',#130084,#65369,#65370);
#51547=AXIS2_PLACEMENT_3D('',#130101,#65371,#65372);
#51548=AXIS2_PLACEMENT_3D('',#130118,#65373,#65374);
#51549=AXIS2_PLACEMENT_3D('',#130135,#65375,#65376);
#51550=AXIS2_PLACEMENT_3D('',#130152,#65377,#65378);
#51551=AXIS2_PLACEMENT_3D('',#130169,#65379,#65380);
#51552=AXIS2_PLACEMENT_3D('',#130186,#65381,#65382);
#51553=AXIS2_PLACEMENT_3D('',#130203,#65383,#65384);
#51554=AXIS2_PLACEMENT_3D('',#130220,#65385,#65386);
#51555=AXIS2_PLACEMENT_3D('',#130237,#65387,#65388);
#51556=AXIS2_PLACEMENT_3D('',#130254,#65389,#65390);
#51557=AXIS2_PLACEMENT_3D('',#130271,#65391,#65392);
#51558=AXIS2_PLACEMENT_3D('',#130288,#65393,#65394);
#51559=AXIS2_PLACEMENT_3D('',#130305,#65395,#65396);
#51560=AXIS2_PLACEMENT_3D('',#130322,#65397,#65398);
#51561=AXIS2_PLACEMENT_3D('',#130339,#65399,#65400);
#51562=AXIS2_PLACEMENT_3D('',#130356,#65401,#65402);
#51563=AXIS2_PLACEMENT_3D('',#130373,#65403,#65404);
#51564=AXIS2_PLACEMENT_3D('',#130390,#65405,#65406);
#51565=AXIS2_PLACEMENT_3D('',#130407,#65407,#65408);
#51566=AXIS2_PLACEMENT_3D('',#130424,#65409,#65410);
#51567=AXIS2_PLACEMENT_3D('',#130441,#65411,#65412);
#51568=AXIS2_PLACEMENT_3D('',#130458,#65413,#65414);
#51569=AXIS2_PLACEMENT_3D('',#130475,#65415,#65416);
#51570=AXIS2_PLACEMENT_3D('',#130492,#65417,#65418);
#51571=AXIS2_PLACEMENT_3D('',#130509,#65419,#65420);
#51572=AXIS2_PLACEMENT_3D('',#130526,#65421,#65422);
#51573=AXIS2_PLACEMENT_3D('',#130543,#65423,#65424);
#51574=AXIS2_PLACEMENT_3D('',#130560,#65425,#65426);
#51575=AXIS2_PLACEMENT_3D('',#130577,#65427,#65428);
#51576=AXIS2_PLACEMENT_3D('',#130594,#65429,#65430);
#51577=AXIS2_PLACEMENT_3D('',#130611,#65431,#65432);
#51578=AXIS2_PLACEMENT_3D('',#130628,#65433,#65434);
#51579=AXIS2_PLACEMENT_3D('',#130645,#65435,#65436);
#51580=AXIS2_PLACEMENT_3D('',#130662,#65437,#65438);
#51581=AXIS2_PLACEMENT_3D('',#130679,#65439,#65440);
#51582=AXIS2_PLACEMENT_3D('',#130696,#65441,#65442);
#51583=AXIS2_PLACEMENT_3D('',#130713,#65443,#65444);
#51584=AXIS2_PLACEMENT_3D('',#130730,#65445,#65446);
#51585=AXIS2_PLACEMENT_3D('',#130747,#65447,#65448);
#51586=AXIS2_PLACEMENT_3D('',#130764,#65449,#65450);
#51587=AXIS2_PLACEMENT_3D('',#130781,#65451,#65452);
#51588=AXIS2_PLACEMENT_3D('',#130798,#65453,#65454);
#51589=AXIS2_PLACEMENT_3D('',#130815,#65455,#65456);
#51590=AXIS2_PLACEMENT_3D('',#130832,#65457,#65458);
#51591=AXIS2_PLACEMENT_3D('',#130849,#65459,#65460);
#51592=AXIS2_PLACEMENT_3D('',#130866,#65461,#65462);
#59297=DIRECTION('axis',(0.,0.,1.));
#59298=DIRECTION('refdir',(1.,0.,0.));
#59299=DIRECTION('center_axis',(0.,1.,0.));
#59300=DIRECTION('ref_axis',(0.,0.,1.));
#59301=DIRECTION('center_axis',(0.,-1.,0.));
#59302=DIRECTION('ref_axis',(0.,0.,1.));
#59303=DIRECTION('center_axis',(0.,-1.,2.84598943930249E-15));
#59304=DIRECTION('ref_axis',(0.,0.,-1.));
#59305=DIRECTION('center_axis',(0.,-1.,2.84598943930249E-15));
#59306=DIRECTION('ref_axis',(0.,-2.84598943930249E-15,-1.));
#59307=DIRECTION('center_axis',(1.,3.48533185724896E-31,1.22464679914735E-16));
#59308=DIRECTION('ref_axis',(-1.22464679914735E-16,0.,1.));
#59309=DIRECTION('center_axis',(0.,1.,-2.84598943930249E-15));
#59310=DIRECTION('ref_axis',(0.,-2.84598943930249E-15,-1.));
#59311=DIRECTION('center_axis',(0.,1.,0.));
#59312=DIRECTION('ref_axis',(0.,0.,1.));
#59313=DIRECTION('',(0.,-1.,0.));
#59314=DIRECTION('center_axis',(0.,1.,0.));
#59315=DIRECTION('ref_axis',(0.,0.,1.));
#59316=DIRECTION('',(0.,1.,0.));
#59317=DIRECTION('center_axis',(0.,-1.,0.));
#59318=DIRECTION('ref_axis',(0.,0.,-1.));
#59319=DIRECTION('center_axis',(0.,1.,0.));
#59320=DIRECTION('ref_axis',(0.,0.,1.));
#59321=DIRECTION('',(0.,-1.,0.));
#59322=DIRECTION('center_axis',(0.,1.,0.));
#59323=DIRECTION('ref_axis',(0.,0.,1.));
#59324=DIRECTION('',(0.,1.,0.));
#59325=DIRECTION('center_axis',(0.,-1.,0.));
#59326=DIRECTION('ref_axis',(0.,0.,-1.));
#59327=DIRECTION('center_axis',(0.,1.,0.));
#59328=DIRECTION('ref_axis',(0.,0.,1.));
#59329=DIRECTION('',(0.,-1.,0.));
#59330=DIRECTION('center_axis',(0.,1.,0.));
#59331=DIRECTION('ref_axis',(0.,0.,1.));
#59332=DIRECTION('',(0.,1.,0.));
#59333=DIRECTION('center_axis',(0.,-1.,0.));
#59334=DIRECTION('ref_axis',(0.,0.,-1.));
#59335=DIRECTION('center_axis',(0.,1.,0.));
#59336=DIRECTION('ref_axis',(0.,0.,1.));
#59337=DIRECTION('',(0.,-1.,0.));
#59338=DIRECTION('center_axis',(0.,1.,0.));
#59339=DIRECTION('ref_axis',(0.,0.,1.));
#59340=DIRECTION('',(0.,1.,0.));
#59341=DIRECTION('center_axis',(0.,-1.,0.));
#59342=DIRECTION('ref_axis',(0.,0.,-1.));
#59343=DIRECTION('center_axis',(0.,1.,0.));
#59344=DIRECTION('ref_axis',(0.,0.,1.));
#59345=DIRECTION('',(0.,-1.,0.));
#59346=DIRECTION('center_axis',(0.,1.,0.));
#59347=DIRECTION('ref_axis',(0.,0.,1.));
#59348=DIRECTION('',(0.,1.,0.));
#59349=DIRECTION('center_axis',(0.,-1.,0.));
#59350=DIRECTION('ref_axis',(0.,0.,-1.));
#59351=DIRECTION('center_axis',(0.,1.,0.));
#59352=DIRECTION('ref_axis',(0.,0.,1.));
#59353=DIRECTION('',(0.,-1.,0.));
#59354=DIRECTION('center_axis',(0.,1.,0.));
#59355=DIRECTION('ref_axis',(0.,0.,1.));
#59356=DIRECTION('',(0.,1.,0.));
#59357=DIRECTION('center_axis',(0.,-1.,0.));
#59358=DIRECTION('ref_axis',(0.,0.,-1.));
#59359=DIRECTION('center_axis',(0.,1.,0.));
#59360=DIRECTION('ref_axis',(0.,0.,1.));
#59361=DIRECTION('',(0.,-1.,0.));
#59362=DIRECTION('center_axis',(0.,1.,0.));
#59363=DIRECTION('ref_axis',(0.,0.,1.));
#59364=DIRECTION('',(0.,1.,0.));
#59365=DIRECTION('center_axis',(0.,-1.,0.));
#59366=DIRECTION('ref_axis',(0.,0.,-1.));
#59367=DIRECTION('center_axis',(0.,1.,0.));
#59368=DIRECTION('ref_axis',(0.,0.,1.));
#59369=DIRECTION('',(0.,-1.,0.));
#59370=DIRECTION('center_axis',(0.,1.,0.));
#59371=DIRECTION('ref_axis',(0.,0.,1.));
#59372=DIRECTION('',(0.,1.,0.));
#59373=DIRECTION('center_axis',(0.,-1.,0.));
#59374=DIRECTION('ref_axis',(0.,0.,-1.));
#59375=DIRECTION('center_axis',(0.,1.,0.));
#59376=DIRECTION('ref_axis',(0.,0.,1.));
#59377=DIRECTION('',(0.,-1.,0.));
#59378=DIRECTION('center_axis',(0.,1.,0.));
#59379=DIRECTION('ref_axis',(0.,0.,1.));
#59380=DIRECTION('',(0.,1.,0.));
#59381=DIRECTION('center_axis',(0.,-1.,0.));
#59382=DIRECTION('ref_axis',(0.,0.,-1.));
#59383=DIRECTION('center_axis',(0.,1.,0.));
#59384=DIRECTION('ref_axis',(0.,0.,1.));
#59385=DIRECTION('',(0.,-1.,0.));
#59386=DIRECTION('center_axis',(0.,1.,0.));
#59387=DIRECTION('ref_axis',(0.,0.,1.));
#59388=DIRECTION('',(0.,1.,0.));
#59389=DIRECTION('center_axis',(0.,-1.,0.));
#59390=DIRECTION('ref_axis',(0.,0.,-1.));
#59391=DIRECTION('center_axis',(0.,1.,0.));
#59392=DIRECTION('ref_axis',(0.,0.,1.));
#59393=DIRECTION('',(0.,-1.,0.));
#59394=DIRECTION('center_axis',(0.,1.,0.));
#59395=DIRECTION('ref_axis',(0.,0.,1.));
#59396=DIRECTION('',(0.,1.,0.));
#59397=DIRECTION('center_axis',(0.,-1.,0.));
#59398=DIRECTION('ref_axis',(0.,0.,-1.));
#59399=DIRECTION('center_axis',(0.,1.,0.));
#59400=DIRECTION('ref_axis',(0.,0.,1.));
#59401=DIRECTION('',(0.,-1.,0.));
#59402=DIRECTION('center_axis',(0.,1.,0.));
#59403=DIRECTION('ref_axis',(0.,0.,1.));
#59404=DIRECTION('',(0.,1.,0.));
#59405=DIRECTION('center_axis',(0.,-1.,0.));
#59406=DIRECTION('ref_axis',(0.,0.,-1.));
#59407=DIRECTION('center_axis',(0.,1.,0.));
#59408=DIRECTION('ref_axis',(0.,0.,1.));
#59409=DIRECTION('',(0.,-1.,0.));
#59410=DIRECTION('center_axis',(0.,1.,0.));
#59411=DIRECTION('ref_axis',(0.,0.,1.));
#59412=DIRECTION('',(0.,1.,0.));
#59413=DIRECTION('center_axis',(0.,-1.,0.));
#59414=DIRECTION('ref_axis',(0.,0.,-1.));
#59415=DIRECTION('center_axis',(0.,1.,0.));
#59416=DIRECTION('ref_axis',(0.,0.,1.));
#59417=DIRECTION('',(0.,-1.,0.));
#59418=DIRECTION('center_axis',(0.,1.,0.));
#59419=DIRECTION('ref_axis',(0.,0.,1.));
#59420=DIRECTION('',(0.,1.,0.));
#59421=DIRECTION('center_axis',(0.,-1.,0.));
#59422=DIRECTION('ref_axis',(0.,0.,-1.));
#59423=DIRECTION('center_axis',(0.,1.,0.));
#59424=DIRECTION('ref_axis',(0.,0.,1.));
#59425=DIRECTION('',(0.,-1.,0.));
#59426=DIRECTION('center_axis',(0.,1.,0.));
#59427=DIRECTION('ref_axis',(0.,0.,1.));
#59428=DIRECTION('',(0.,1.,0.));
#59429=DIRECTION('center_axis',(0.,-1.,0.));
#59430=DIRECTION('ref_axis',(0.,0.,-1.));
#59431=DIRECTION('center_axis',(0.,1.,0.));
#59432=DIRECTION('ref_axis',(0.,0.,1.));
#59433=DIRECTION('',(0.,-1.,0.));
#59434=DIRECTION('center_axis',(0.,1.,0.));
#59435=DIRECTION('ref_axis',(0.,0.,1.));
#59436=DIRECTION('',(0.,1.,0.));
#59437=DIRECTION('center_axis',(0.,-1.,0.));
#59438=DIRECTION('ref_axis',(0.,0.,-1.));
#59439=DIRECTION('center_axis',(0.,1.,0.));
#59440=DIRECTION('ref_axis',(0.,0.,1.));
#59441=DIRECTION('',(0.,-1.,0.));
#59442=DIRECTION('center_axis',(0.,1.,0.));
#59443=DIRECTION('ref_axis',(0.,0.,1.));
#59444=DIRECTION('',(0.,1.,0.));
#59445=DIRECTION('center_axis',(0.,-1.,0.));
#59446=DIRECTION('ref_axis',(0.,0.,-1.));
#59447=DIRECTION('center_axis',(0.,1.,0.));
#59448=DIRECTION('ref_axis',(0.,0.,1.));
#59449=DIRECTION('',(0.,-1.,0.));
#59450=DIRECTION('center_axis',(0.,1.,0.));
#59451=DIRECTION('ref_axis',(0.,0.,1.));
#59452=DIRECTION('',(0.,1.,0.));
#59453=DIRECTION('center_axis',(0.,-1.,0.));
#59454=DIRECTION('ref_axis',(0.,0.,-1.));
#59455=DIRECTION('center_axis',(0.,1.,0.));
#59456=DIRECTION('ref_axis',(0.,0.,1.));
#59457=DIRECTION('',(0.,-1.,0.));
#59458=DIRECTION('center_axis',(0.,1.,0.));
#59459=DIRECTION('ref_axis',(0.,0.,1.));
#59460=DIRECTION('',(0.,1.,0.));
#59461=DIRECTION('center_axis',(0.,-1.,0.));
#59462=DIRECTION('ref_axis',(0.,0.,-1.));
#59463=DIRECTION('center_axis',(0.,1.,0.));
#59464=DIRECTION('ref_axis',(0.,0.,1.));
#59465=DIRECTION('',(0.,-1.,0.));
#59466=DIRECTION('center_axis',(0.,1.,0.));
#59467=DIRECTION('ref_axis',(0.,0.,1.));
#59468=DIRECTION('',(0.,1.,0.));
#59469=DIRECTION('center_axis',(0.,-1.,0.));
#59470=DIRECTION('ref_axis',(0.,0.,-1.));
#59471=DIRECTION('center_axis',(0.,1.,0.));
#59472=DIRECTION('ref_axis',(0.,0.,1.));
#59473=DIRECTION('',(0.,-1.,0.));
#59474=DIRECTION('center_axis',(0.,1.,0.));
#59475=DIRECTION('ref_axis',(0.,0.,1.));
#59476=DIRECTION('',(0.,1.,0.));
#59477=DIRECTION('center_axis',(0.,-1.,0.));
#59478=DIRECTION('ref_axis',(0.,0.,-1.));
#59479=DIRECTION('center_axis',(0.,1.,0.));
#59480=DIRECTION('ref_axis',(0.,0.,1.));
#59481=DIRECTION('',(0.,-1.,0.));
#59482=DIRECTION('center_axis',(0.,1.,0.));
#59483=DIRECTION('ref_axis',(0.,0.,1.));
#59484=DIRECTION('',(0.,1.,0.));
#59485=DIRECTION('center_axis',(0.,-1.,0.));
#59486=DIRECTION('ref_axis',(0.,0.,-1.));
#59487=DIRECTION('center_axis',(0.,1.,0.));
#59488=DIRECTION('ref_axis',(0.,0.,1.));
#59489=DIRECTION('',(0.,-1.,0.));
#59490=DIRECTION('center_axis',(0.,1.,0.));
#59491=DIRECTION('ref_axis',(0.,0.,1.));
#59492=DIRECTION('',(0.,1.,0.));
#59493=DIRECTION('center_axis',(0.,-1.,0.));
#59494=DIRECTION('ref_axis',(0.,0.,-1.));
#59495=DIRECTION('center_axis',(0.,1.,0.));
#59496=DIRECTION('ref_axis',(0.,0.,1.));
#59497=DIRECTION('',(0.,-1.,0.));
#59498=DIRECTION('center_axis',(0.,1.,0.));
#59499=DIRECTION('ref_axis',(0.,0.,1.));
#59500=DIRECTION('',(0.,1.,0.));
#59501=DIRECTION('center_axis',(0.,-1.,0.));
#59502=DIRECTION('ref_axis',(0.,0.,-1.));
#59503=DIRECTION('center_axis',(0.,1.,0.));
#59504=DIRECTION('ref_axis',(0.,0.,1.));
#59505=DIRECTION('',(0.,-1.,0.));
#59506=DIRECTION('center_axis',(0.,1.,0.));
#59507=DIRECTION('ref_axis',(0.,0.,1.));
#59508=DIRECTION('',(0.,1.,0.));
#59509=DIRECTION('center_axis',(0.,-1.,0.));
#59510=DIRECTION('ref_axis',(0.,0.,-1.));
#59511=DIRECTION('center_axis',(0.,1.,0.));
#59512=DIRECTION('ref_axis',(0.,0.,1.));
#59513=DIRECTION('',(0.,-1.,0.));
#59514=DIRECTION('center_axis',(0.,1.,0.));
#59515=DIRECTION('ref_axis',(0.,0.,1.));
#59516=DIRECTION('',(0.,1.,0.));
#59517=DIRECTION('center_axis',(0.,-1.,0.));
#59518=DIRECTION('ref_axis',(0.,0.,-1.));
#59519=DIRECTION('center_axis',(0.,1.,0.));
#59520=DIRECTION('ref_axis',(0.,0.,1.));
#59521=DIRECTION('',(0.,-1.,0.));
#59522=DIRECTION('center_axis',(0.,1.,0.));
#59523=DIRECTION('ref_axis',(0.,0.,1.));
#59524=DIRECTION('',(0.,1.,0.));
#59525=DIRECTION('center_axis',(0.,-1.,0.));
#59526=DIRECTION('ref_axis',(0.,0.,-1.));
#59527=DIRECTION('center_axis',(0.,1.,0.));
#59528=DIRECTION('ref_axis',(0.,0.,1.));
#59529=DIRECTION('',(0.,-1.,0.));
#59530=DIRECTION('center_axis',(0.,1.,0.));
#59531=DIRECTION('ref_axis',(0.,0.,1.));
#59532=DIRECTION('',(0.,1.,0.));
#59533=DIRECTION('center_axis',(0.,-1.,0.));
#59534=DIRECTION('ref_axis',(0.,0.,-1.));
#59535=DIRECTION('center_axis',(0.,1.,0.));
#59536=DIRECTION('ref_axis',(0.,0.,1.));
#59537=DIRECTION('',(0.,-1.,0.));
#59538=DIRECTION('center_axis',(0.,1.,0.));
#59539=DIRECTION('ref_axis',(0.,0.,1.));
#59540=DIRECTION('',(0.,1.,0.));
#59541=DIRECTION('center_axis',(0.,-1.,0.));
#59542=DIRECTION('ref_axis',(0.,0.,-1.));
#59543=DIRECTION('center_axis',(0.,1.,0.));
#59544=DIRECTION('ref_axis',(0.,0.,1.));
#59545=DIRECTION('',(0.,-1.,0.));
#59546=DIRECTION('center_axis',(0.,1.,0.));
#59547=DIRECTION('ref_axis',(0.,0.,1.));
#59548=DIRECTION('',(0.,1.,0.));
#59549=DIRECTION('center_axis',(0.,-1.,0.));
#59550=DIRECTION('ref_axis',(0.,0.,-1.));
#59551=DIRECTION('center_axis',(0.,1.,0.));
#59552=DIRECTION('ref_axis',(0.,0.,1.));
#59553=DIRECTION('',(0.,-1.,0.));
#59554=DIRECTION('center_axis',(0.,1.,0.));
#59555=DIRECTION('ref_axis',(0.,0.,1.));
#59556=DIRECTION('',(0.,1.,0.));
#59557=DIRECTION('center_axis',(0.,-1.,0.));
#59558=DIRECTION('ref_axis',(0.,0.,-1.));
#59559=DIRECTION('center_axis',(0.,1.,0.));
#59560=DIRECTION('ref_axis',(0.,0.,1.));
#59561=DIRECTION('',(0.,-1.,0.));
#59562=DIRECTION('center_axis',(0.,1.,0.));
#59563=DIRECTION('ref_axis',(0.,0.,1.));
#59564=DIRECTION('',(0.,1.,0.));
#59565=DIRECTION('center_axis',(0.,-1.,0.));
#59566=DIRECTION('ref_axis',(0.,0.,-1.));
#59567=DIRECTION('center_axis',(0.,1.,0.));
#59568=DIRECTION('ref_axis',(0.,0.,1.));
#59569=DIRECTION('',(0.,-1.,0.));
#59570=DIRECTION('center_axis',(0.,1.,0.));
#59571=DIRECTION('ref_axis',(0.,0.,1.));
#59572=DIRECTION('',(0.,1.,0.));
#59573=DIRECTION('center_axis',(0.,-1.,0.));
#59574=DIRECTION('ref_axis',(0.,0.,-1.));
#59575=DIRECTION('center_axis',(0.,1.,0.));
#59576=DIRECTION('ref_axis',(0.,0.,1.));
#59577=DIRECTION('',(0.,-1.,0.));
#59578=DIRECTION('center_axis',(0.,1.,0.));
#59579=DIRECTION('ref_axis',(0.,0.,1.));
#59580=DIRECTION('',(0.,1.,0.));
#59581=DIRECTION('center_axis',(0.,-1.,0.));
#59582=DIRECTION('ref_axis',(0.,0.,-1.));
#59583=DIRECTION('center_axis',(0.,1.,0.));
#59584=DIRECTION('ref_axis',(0.,0.,1.));
#59585=DIRECTION('',(0.,-1.,0.));
#59586=DIRECTION('center_axis',(0.,1.,0.));
#59587=DIRECTION('ref_axis',(0.,0.,1.));
#59588=DIRECTION('',(0.,1.,0.));
#59589=DIRECTION('center_axis',(0.,-1.,0.));
#59590=DIRECTION('ref_axis',(0.,0.,-1.));
#59591=DIRECTION('center_axis',(0.,1.,0.));
#59592=DIRECTION('ref_axis',(0.,0.,1.));
#59593=DIRECTION('',(0.,-1.,0.));
#59594=DIRECTION('center_axis',(0.,1.,0.));
#59595=DIRECTION('ref_axis',(0.,0.,1.));
#59596=DIRECTION('',(0.,1.,0.));
#59597=DIRECTION('center_axis',(0.,-1.,0.));
#59598=DIRECTION('ref_axis',(0.,0.,-1.));
#59599=DIRECTION('center_axis',(0.,1.,0.));
#59600=DIRECTION('ref_axis',(0.,0.,1.));
#59601=DIRECTION('',(0.,-1.,0.));
#59602=DIRECTION('center_axis',(0.,1.,0.));
#59603=DIRECTION('ref_axis',(0.,0.,1.));
#59604=DIRECTION('',(0.,1.,0.));
#59605=DIRECTION('center_axis',(0.,-1.,0.));
#59606=DIRECTION('ref_axis',(0.,0.,-1.));
#59607=DIRECTION('center_axis',(0.,1.,0.));
#59608=DIRECTION('ref_axis',(0.,0.,1.));
#59609=DIRECTION('',(0.,-1.,0.));
#59610=DIRECTION('center_axis',(0.,1.,0.));
#59611=DIRECTION('ref_axis',(0.,0.,1.));
#59612=DIRECTION('',(0.,1.,0.));
#59613=DIRECTION('center_axis',(0.,-1.,0.));
#59614=DIRECTION('ref_axis',(0.,0.,-1.));
#59615=DIRECTION('center_axis',(0.,1.,0.));
#59616=DIRECTION('ref_axis',(0.,0.,1.));
#59617=DIRECTION('',(0.,-1.,0.));
#59618=DIRECTION('center_axis',(0.,1.,0.));
#59619=DIRECTION('ref_axis',(0.,0.,1.));
#59620=DIRECTION('',(0.,1.,0.));
#59621=DIRECTION('center_axis',(0.,-1.,0.));
#59622=DIRECTION('ref_axis',(0.,0.,-1.));
#59623=DIRECTION('center_axis',(0.,1.,0.));
#59624=DIRECTION('ref_axis',(0.,0.,1.));
#59625=DIRECTION('',(0.,-1.,0.));
#59626=DIRECTION('center_axis',(0.,1.,0.));
#59627=DIRECTION('ref_axis',(0.,0.,1.));
#59628=DIRECTION('',(0.,1.,0.));
#59629=DIRECTION('center_axis',(0.,-1.,0.));
#59630=DIRECTION('ref_axis',(0.,0.,-1.));
#59631=DIRECTION('center_axis',(0.,1.,0.));
#59632=DIRECTION('ref_axis',(0.,0.,1.));
#59633=DIRECTION('',(0.,-1.,0.));
#59634=DIRECTION('center_axis',(0.,1.,0.));
#59635=DIRECTION('ref_axis',(0.,0.,1.));
#59636=DIRECTION('',(0.,1.,0.));
#59637=DIRECTION('center_axis',(0.,-1.,0.));
#59638=DIRECTION('ref_axis',(0.,0.,-1.));
#59639=DIRECTION('center_axis',(0.,1.,0.));
#59640=DIRECTION('ref_axis',(0.,0.,1.));
#59641=DIRECTION('',(0.,-1.,0.));
#59642=DIRECTION('center_axis',(0.,1.,0.));
#59643=DIRECTION('ref_axis',(0.,0.,1.));
#59644=DIRECTION('',(0.,1.,0.));
#59645=DIRECTION('center_axis',(0.,-1.,0.));
#59646=DIRECTION('ref_axis',(0.,0.,-1.));
#59647=DIRECTION('center_axis',(0.,1.,0.));
#59648=DIRECTION('ref_axis',(0.,0.,1.));
#59649=DIRECTION('',(0.,-1.,0.));
#59650=DIRECTION('center_axis',(0.,1.,0.));
#59651=DIRECTION('ref_axis',(0.,0.,1.));
#59652=DIRECTION('',(0.,1.,0.));
#59653=DIRECTION('center_axis',(0.,-1.,0.));
#59654=DIRECTION('ref_axis',(0.,0.,-1.));
#59655=DIRECTION('center_axis',(0.,1.,0.));
#59656=DIRECTION('ref_axis',(0.,0.,1.));
#59657=DIRECTION('',(0.,-1.,0.));
#59658=DIRECTION('center_axis',(0.,1.,0.));
#59659=DIRECTION('ref_axis',(0.,0.,1.));
#59660=DIRECTION('',(0.,1.,0.));
#59661=DIRECTION('center_axis',(0.,-1.,0.));
#59662=DIRECTION('ref_axis',(0.,0.,-1.));
#59663=DIRECTION('center_axis',(0.,1.,0.));
#59664=DIRECTION('ref_axis',(0.,0.,1.));
#59665=DIRECTION('',(0.,-1.,0.));
#59666=DIRECTION('center_axis',(0.,1.,0.));
#59667=DIRECTION('ref_axis',(0.,0.,1.));
#59668=DIRECTION('',(0.,1.,0.));
#59669=DIRECTION('center_axis',(0.,-1.,0.));
#59670=DIRECTION('ref_axis',(0.,0.,-1.));
#59671=DIRECTION('center_axis',(0.,1.,0.));
#59672=DIRECTION('ref_axis',(0.,0.,1.));
#59673=DIRECTION('',(0.,-1.,0.));
#59674=DIRECTION('center_axis',(0.,1.,0.));
#59675=DIRECTION('ref_axis',(0.,0.,1.));
#59676=DIRECTION('',(0.,1.,0.));
#59677=DIRECTION('center_axis',(0.,-1.,0.));
#59678=DIRECTION('ref_axis',(0.,0.,-1.));
#59679=DIRECTION('center_axis',(0.,1.,0.));
#59680=DIRECTION('ref_axis',(0.,0.,1.));
#59681=DIRECTION('',(0.,-1.,0.));
#59682=DIRECTION('center_axis',(0.,1.,0.));
#59683=DIRECTION('ref_axis',(0.,0.,1.));
#59684=DIRECTION('',(0.,1.,0.));
#59685=DIRECTION('center_axis',(0.,-1.,0.));
#59686=DIRECTION('ref_axis',(0.,0.,-1.));
#59687=DIRECTION('center_axis',(0.,1.,0.));
#59688=DIRECTION('ref_axis',(0.,0.,1.));
#59689=DIRECTION('',(0.,-1.,0.));
#59690=DIRECTION('center_axis',(0.,1.,0.));
#59691=DIRECTION('ref_axis',(0.,0.,1.));
#59692=DIRECTION('',(0.,1.,0.));
#59693=DIRECTION('center_axis',(0.,-1.,0.));
#59694=DIRECTION('ref_axis',(0.,0.,-1.));
#59695=DIRECTION('center_axis',(0.,1.,0.));
#59696=DIRECTION('ref_axis',(0.,0.,1.));
#59697=DIRECTION('',(0.,-1.,0.));
#59698=DIRECTION('center_axis',(0.,1.,0.));
#59699=DIRECTION('ref_axis',(0.,0.,1.));
#59700=DIRECTION('',(0.,1.,0.));
#59701=DIRECTION('center_axis',(0.,-1.,0.));
#59702=DIRECTION('ref_axis',(0.,0.,-1.));
#59703=DIRECTION('center_axis',(0.,1.,0.));
#59704=DIRECTION('ref_axis',(0.,0.,1.));
#59705=DIRECTION('',(0.,-1.,0.));
#59706=DIRECTION('center_axis',(0.,1.,0.));
#59707=DIRECTION('ref_axis',(0.,0.,1.));
#59708=DIRECTION('',(0.,1.,0.));
#59709=DIRECTION('center_axis',(0.,-1.,0.));
#59710=DIRECTION('ref_axis',(0.,0.,-1.));
#59711=DIRECTION('center_axis',(0.,1.,0.));
#59712=DIRECTION('ref_axis',(0.,0.,1.));
#59713=DIRECTION('',(0.,-1.,0.));
#59714=DIRECTION('center_axis',(0.,1.,0.));
#59715=DIRECTION('ref_axis',(0.,0.,1.));
#59716=DIRECTION('',(0.,1.,0.));
#59717=DIRECTION('center_axis',(0.,-1.,0.));
#59718=DIRECTION('ref_axis',(0.,0.,-1.));
#59719=DIRECTION('center_axis',(0.,1.,0.));
#59720=DIRECTION('ref_axis',(0.,0.,1.));
#59721=DIRECTION('',(0.,-1.,0.));
#59722=DIRECTION('center_axis',(0.,1.,0.));
#59723=DIRECTION('ref_axis',(0.,0.,1.));
#59724=DIRECTION('',(0.,1.,0.));
#59725=DIRECTION('center_axis',(0.,-1.,0.));
#59726=DIRECTION('ref_axis',(0.,0.,-1.));
#59727=DIRECTION('center_axis',(0.,1.,0.));
#59728=DIRECTION('ref_axis',(0.,0.,1.));
#59729=DIRECTION('',(0.,-1.,0.));
#59730=DIRECTION('center_axis',(0.,1.,0.));
#59731=DIRECTION('ref_axis',(0.,0.,1.));
#59732=DIRECTION('',(0.,1.,0.));
#59733=DIRECTION('center_axis',(0.,-1.,0.));
#59734=DIRECTION('ref_axis',(0.,0.,-1.));
#59735=DIRECTION('center_axis',(0.,1.,0.));
#59736=DIRECTION('ref_axis',(0.,0.,1.));
#59737=DIRECTION('',(0.,-1.,0.));
#59738=DIRECTION('center_axis',(0.,1.,0.));
#59739=DIRECTION('ref_axis',(0.,0.,1.));
#59740=DIRECTION('',(0.,1.,0.));
#59741=DIRECTION('center_axis',(0.,-1.,0.));
#59742=DIRECTION('ref_axis',(0.,0.,-1.));
#59743=DIRECTION('center_axis',(0.,1.,0.));
#59744=DIRECTION('ref_axis',(0.,0.,1.));
#59745=DIRECTION('',(0.,-1.,0.));
#59746=DIRECTION('center_axis',(0.,1.,0.));
#59747=DIRECTION('ref_axis',(0.,0.,1.));
#59748=DIRECTION('',(0.,1.,0.));
#59749=DIRECTION('center_axis',(0.,-1.,0.));
#59750=DIRECTION('ref_axis',(0.,0.,-1.));
#59751=DIRECTION('center_axis',(0.,1.,0.));
#59752=DIRECTION('ref_axis',(0.,0.,1.));
#59753=DIRECTION('',(0.,-1.,0.));
#59754=DIRECTION('center_axis',(0.,1.,0.));
#59755=DIRECTION('ref_axis',(0.,0.,1.));
#59756=DIRECTION('',(0.,1.,0.));
#59757=DIRECTION('center_axis',(0.,-1.,0.));
#59758=DIRECTION('ref_axis',(0.,0.,-1.));
#59759=DIRECTION('center_axis',(0.,1.,0.));
#59760=DIRECTION('ref_axis',(0.,0.,1.));
#59761=DIRECTION('',(0.,-1.,0.));
#59762=DIRECTION('center_axis',(0.,1.,0.));
#59763=DIRECTION('ref_axis',(0.,0.,1.));
#59764=DIRECTION('',(0.,1.,0.));
#59765=DIRECTION('center_axis',(0.,-1.,0.));
#59766=DIRECTION('ref_axis',(0.,0.,-1.));
#59767=DIRECTION('center_axis',(0.,1.,0.));
#59768=DIRECTION('ref_axis',(0.,0.,1.));
#59769=DIRECTION('',(0.,-1.,0.));
#59770=DIRECTION('center_axis',(0.,1.,0.));
#59771=DIRECTION('ref_axis',(0.,0.,1.));
#59772=DIRECTION('',(0.,1.,0.));
#59773=DIRECTION('center_axis',(0.,-1.,0.));
#59774=DIRECTION('ref_axis',(0.,0.,-1.));
#59775=DIRECTION('center_axis',(0.,1.,0.));
#59776=DIRECTION('ref_axis',(0.,0.,1.));
#59777=DIRECTION('',(0.,-1.,0.));
#59778=DIRECTION('center_axis',(0.,1.,0.));
#59779=DIRECTION('ref_axis',(0.,0.,1.));
#59780=DIRECTION('',(0.,1.,0.));
#59781=DIRECTION('center_axis',(0.,-1.,0.));
#59782=DIRECTION('ref_axis',(0.,0.,-1.));
#59783=DIRECTION('center_axis',(0.,1.,0.));
#59784=DIRECTION('ref_axis',(0.,0.,1.));
#59785=DIRECTION('',(0.,-1.,0.));
#59786=DIRECTION('center_axis',(0.,1.,0.));
#59787=DIRECTION('ref_axis',(0.,0.,1.));
#59788=DIRECTION('',(0.,1.,0.));
#59789=DIRECTION('center_axis',(0.,-1.,0.));
#59790=DIRECTION('ref_axis',(0.,0.,-1.));
#59791=DIRECTION('center_axis',(0.,1.,0.));
#59792=DIRECTION('ref_axis',(0.,0.,1.));
#59793=DIRECTION('',(0.,-1.,0.));
#59794=DIRECTION('center_axis',(0.,1.,0.));
#59795=DIRECTION('ref_axis',(0.,0.,1.));
#59796=DIRECTION('',(0.,1.,0.));
#59797=DIRECTION('center_axis',(0.,-1.,0.));
#59798=DIRECTION('ref_axis',(0.,0.,-1.));
#59799=DIRECTION('center_axis',(0.,1.,0.));
#59800=DIRECTION('ref_axis',(0.,0.,1.));
#59801=DIRECTION('',(0.,-1.,0.));
#59802=DIRECTION('center_axis',(0.,1.,0.));
#59803=DIRECTION('ref_axis',(0.,0.,1.));
#59804=DIRECTION('',(0.,1.,0.));
#59805=DIRECTION('center_axis',(0.,-1.,0.));
#59806=DIRECTION('ref_axis',(0.,0.,-1.));
#59807=DIRECTION('center_axis',(0.,1.,0.));
#59808=DIRECTION('ref_axis',(0.,0.,1.));
#59809=DIRECTION('',(0.,-1.,0.));
#59810=DIRECTION('center_axis',(0.,1.,0.));
#59811=DIRECTION('ref_axis',(0.,0.,1.));
#59812=DIRECTION('',(0.,1.,0.));
#59813=DIRECTION('center_axis',(0.,-1.,0.));
#59814=DIRECTION('ref_axis',(0.,0.,-1.));
#59815=DIRECTION('center_axis',(0.,1.,0.));
#59816=DIRECTION('ref_axis',(0.,0.,1.));
#59817=DIRECTION('',(0.,-1.,0.));
#59818=DIRECTION('center_axis',(0.,1.,0.));
#59819=DIRECTION('ref_axis',(0.,0.,1.));
#59820=DIRECTION('',(0.,1.,0.));
#59821=DIRECTION('center_axis',(0.,-1.,0.));
#59822=DIRECTION('ref_axis',(0.,0.,-1.));
#59823=DIRECTION('center_axis',(0.,1.,0.));
#59824=DIRECTION('ref_axis',(0.,0.,1.));
#59825=DIRECTION('',(0.,-1.,0.));
#59826=DIRECTION('center_axis',(0.,1.,0.));
#59827=DIRECTION('ref_axis',(0.,0.,1.));
#59828=DIRECTION('',(0.,1.,0.));
#59829=DIRECTION('center_axis',(0.,-1.,0.));
#59830=DIRECTION('ref_axis',(0.,0.,-1.));
#59831=DIRECTION('center_axis',(0.,1.,0.));
#59832=DIRECTION('ref_axis',(0.,0.,1.));
#59833=DIRECTION('',(0.,-1.,0.));
#59834=DIRECTION('center_axis',(0.,1.,0.));
#59835=DIRECTION('ref_axis',(0.,0.,1.));
#59836=DIRECTION('',(0.,1.,0.));
#59837=DIRECTION('center_axis',(0.,-1.,0.));
#59838=DIRECTION('ref_axis',(0.,0.,-1.));
#59839=DIRECTION('center_axis',(0.,1.,0.));
#59840=DIRECTION('ref_axis',(0.,0.,1.));
#59841=DIRECTION('',(0.,-1.,0.));
#59842=DIRECTION('center_axis',(0.,1.,0.));
#59843=DIRECTION('ref_axis',(0.,0.,1.));
#59844=DIRECTION('',(0.,1.,0.));
#59845=DIRECTION('center_axis',(0.,-1.,0.));
#59846=DIRECTION('ref_axis',(0.,0.,-1.));
#59847=DIRECTION('center_axis',(0.,1.,0.));
#59848=DIRECTION('ref_axis',(0.,0.,1.));
#59849=DIRECTION('',(0.,-1.,0.));
#59850=DIRECTION('center_axis',(0.,1.,0.));
#59851=DIRECTION('ref_axis',(0.,0.,1.));
#59852=DIRECTION('',(0.,1.,0.));
#59853=DIRECTION('center_axis',(0.,-1.,0.));
#59854=DIRECTION('ref_axis',(0.,0.,-1.));
#59855=DIRECTION('center_axis',(0.,1.,0.));
#59856=DIRECTION('ref_axis',(0.,0.,1.));
#59857=DIRECTION('',(0.,-1.,0.));
#59858=DIRECTION('center_axis',(0.,1.,0.));
#59859=DIRECTION('ref_axis',(0.,0.,1.));
#59860=DIRECTION('',(0.,1.,0.));
#59861=DIRECTION('center_axis',(0.,-1.,0.));
#59862=DIRECTION('ref_axis',(0.,0.,-1.));
#59863=DIRECTION('center_axis',(0.,1.,0.));
#59864=DIRECTION('ref_axis',(0.,0.,1.));
#59865=DIRECTION('',(0.,-1.,0.));
#59866=DIRECTION('center_axis',(0.,1.,0.));
#59867=DIRECTION('ref_axis',(0.,0.,1.));
#59868=DIRECTION('',(0.,1.,0.));
#59869=DIRECTION('center_axis',(0.,-1.,0.));
#59870=DIRECTION('ref_axis',(0.,0.,-1.));
#59871=DIRECTION('center_axis',(0.,1.,0.));
#59872=DIRECTION('ref_axis',(0.,0.,1.));
#59873=DIRECTION('',(0.,-1.,0.));
#59874=DIRECTION('center_axis',(0.,1.,0.));
#59875=DIRECTION('ref_axis',(0.,0.,1.));
#59876=DIRECTION('',(0.,1.,0.));
#59877=DIRECTION('center_axis',(0.,-1.,0.));
#59878=DIRECTION('ref_axis',(0.,0.,-1.));
#59879=DIRECTION('center_axis',(0.,1.,0.));
#59880=DIRECTION('ref_axis',(0.,0.,1.));
#59881=DIRECTION('',(0.,-1.,0.));
#59882=DIRECTION('center_axis',(0.,1.,0.));
#59883=DIRECTION('ref_axis',(0.,0.,1.));
#59884=DIRECTION('',(0.,1.,0.));
#59885=DIRECTION('center_axis',(0.,-1.,0.));
#59886=DIRECTION('ref_axis',(0.,0.,-1.));
#59887=DIRECTION('center_axis',(0.,1.,0.));
#59888=DIRECTION('ref_axis',(0.,0.,1.));
#59889=DIRECTION('',(0.,-1.,0.));
#59890=DIRECTION('center_axis',(0.,1.,0.));
#59891=DIRECTION('ref_axis',(0.,0.,1.));
#59892=DIRECTION('',(0.,1.,0.));
#59893=DIRECTION('center_axis',(0.,-1.,0.));
#59894=DIRECTION('ref_axis',(0.,0.,-1.));
#59895=DIRECTION('center_axis',(0.,1.,0.));
#59896=DIRECTION('ref_axis',(0.,0.,1.));
#59897=DIRECTION('',(0.,-1.,0.));
#59898=DIRECTION('center_axis',(0.,1.,0.));
#59899=DIRECTION('ref_axis',(0.,0.,1.));
#59900=DIRECTION('',(0.,1.,0.));
#59901=DIRECTION('center_axis',(0.,-1.,0.));
#59902=DIRECTION('ref_axis',(0.,0.,-1.));
#59903=DIRECTION('center_axis',(0.,1.,0.));
#59904=DIRECTION('ref_axis',(0.,0.,1.));
#59905=DIRECTION('',(0.,-1.,0.));
#59906=DIRECTION('center_axis',(0.,1.,0.));
#59907=DIRECTION('ref_axis',(0.,0.,1.));
#59908=DIRECTION('',(0.,1.,0.));
#59909=DIRECTION('center_axis',(0.,-1.,0.));
#59910=DIRECTION('ref_axis',(0.,0.,-1.));
#59911=DIRECTION('center_axis',(0.,1.,0.));
#59912=DIRECTION('ref_axis',(0.,0.,1.));
#59913=DIRECTION('',(0.,-1.,0.));
#59914=DIRECTION('center_axis',(0.,1.,0.));
#59915=DIRECTION('ref_axis',(0.,0.,1.));
#59916=DIRECTION('',(0.,1.,0.));
#59917=DIRECTION('center_axis',(0.,-1.,0.));
#59918=DIRECTION('ref_axis',(0.,0.,-1.));
#59919=DIRECTION('center_axis',(0.,1.,0.));
#59920=DIRECTION('ref_axis',(0.,0.,1.));
#59921=DIRECTION('',(0.,-1.,0.));
#59922=DIRECTION('center_axis',(0.,1.,0.));
#59923=DIRECTION('ref_axis',(0.,0.,1.));
#59924=DIRECTION('',(0.,1.,0.));
#59925=DIRECTION('center_axis',(0.,-1.,0.));
#59926=DIRECTION('ref_axis',(0.,0.,-1.));
#59927=DIRECTION('center_axis',(0.,1.,0.));
#59928=DIRECTION('ref_axis',(0.,0.,1.));
#59929=DIRECTION('',(0.,-1.,0.));
#59930=DIRECTION('center_axis',(0.,1.,0.));
#59931=DIRECTION('ref_axis',(0.,0.,1.));
#59932=DIRECTION('',(0.,1.,0.));
#59933=DIRECTION('center_axis',(0.,-1.,0.));
#59934=DIRECTION('ref_axis',(0.,0.,-1.));
#59935=DIRECTION('center_axis',(0.,1.,0.));
#59936=DIRECTION('ref_axis',(0.,0.,1.));
#59937=DIRECTION('',(0.,-1.,0.));
#59938=DIRECTION('center_axis',(0.,1.,0.));
#59939=DIRECTION('ref_axis',(0.,0.,1.));
#59940=DIRECTION('',(0.,1.,0.));
#59941=DIRECTION('center_axis',(0.,-1.,0.));
#59942=DIRECTION('ref_axis',(0.,0.,-1.));
#59943=DIRECTION('center_axis',(0.,1.,0.));
#59944=DIRECTION('ref_axis',(0.,0.,1.));
#59945=DIRECTION('',(0.,-1.,0.));
#59946=DIRECTION('center_axis',(0.,1.,0.));
#59947=DIRECTION('ref_axis',(0.,0.,1.));
#59948=DIRECTION('',(0.,1.,0.));
#59949=DIRECTION('center_axis',(0.,-1.,0.));
#59950=DIRECTION('ref_axis',(0.,0.,-1.));
#59951=DIRECTION('center_axis',(0.,1.,0.));
#59952=DIRECTION('ref_axis',(0.,0.,1.));
#59953=DIRECTION('',(0.,-1.,0.));
#59954=DIRECTION('center_axis',(0.,1.,0.));
#59955=DIRECTION('ref_axis',(0.,0.,1.));
#59956=DIRECTION('',(0.,1.,0.));
#59957=DIRECTION('center_axis',(0.,-1.,0.));
#59958=DIRECTION('ref_axis',(0.,0.,-1.));
#59959=DIRECTION('center_axis',(0.,1.,0.));
#59960=DIRECTION('ref_axis',(0.,0.,1.));
#59961=DIRECTION('',(0.,-1.,0.));
#59962=DIRECTION('center_axis',(0.,1.,0.));
#59963=DIRECTION('ref_axis',(0.,0.,1.));
#59964=DIRECTION('',(0.,1.,0.));
#59965=DIRECTION('center_axis',(0.,-1.,0.));
#59966=DIRECTION('ref_axis',(0.,0.,-1.));
#59967=DIRECTION('center_axis',(0.,1.,0.));
#59968=DIRECTION('ref_axis',(0.,0.,1.));
#59969=DIRECTION('',(0.,-1.,0.));
#59970=DIRECTION('center_axis',(0.,1.,0.));
#59971=DIRECTION('ref_axis',(0.,0.,1.));
#59972=DIRECTION('',(0.,1.,0.));
#59973=DIRECTION('center_axis',(0.,-1.,0.));
#59974=DIRECTION('ref_axis',(0.,0.,-1.));
#59975=DIRECTION('center_axis',(0.,1.,0.));
#59976=DIRECTION('ref_axis',(0.,0.,1.));
#59977=DIRECTION('',(0.,-1.,0.));
#59978=DIRECTION('center_axis',(0.,1.,0.));
#59979=DIRECTION('ref_axis',(0.,0.,1.));
#59980=DIRECTION('',(0.,1.,0.));
#59981=DIRECTION('center_axis',(0.,-1.,0.));
#59982=DIRECTION('ref_axis',(0.,0.,-1.));
#59983=DIRECTION('center_axis',(0.,1.,0.));
#59984=DIRECTION('ref_axis',(0.,0.,1.));
#59985=DIRECTION('',(0.,-1.,0.));
#59986=DIRECTION('center_axis',(0.,1.,0.));
#59987=DIRECTION('ref_axis',(0.,0.,1.));
#59988=DIRECTION('',(0.,1.,0.));
#59989=DIRECTION('center_axis',(0.,-1.,0.));
#59990=DIRECTION('ref_axis',(0.,0.,-1.));
#59991=DIRECTION('center_axis',(0.,1.,0.));
#59992=DIRECTION('ref_axis',(0.,0.,1.));
#59993=DIRECTION('',(0.,-1.,0.));
#59994=DIRECTION('center_axis',(0.,1.,0.));
#59995=DIRECTION('ref_axis',(0.,0.,1.));
#59996=DIRECTION('',(0.,1.,0.));
#59997=DIRECTION('center_axis',(0.,-1.,0.));
#59998=DIRECTION('ref_axis',(0.,0.,-1.));
#59999=DIRECTION('center_axis',(0.,1.,0.));
#60000=DIRECTION('ref_axis',(0.,0.,1.));
#60001=DIRECTION('',(0.,-1.,0.));
#60002=DIRECTION('center_axis',(0.,1.,0.));
#60003=DIRECTION('ref_axis',(0.,0.,1.));
#60004=DIRECTION('',(0.,1.,0.));
#60005=DIRECTION('center_axis',(0.,-1.,0.));
#60006=DIRECTION('ref_axis',(0.,0.,-1.));
#60007=DIRECTION('center_axis',(0.,1.,0.));
#60008=DIRECTION('ref_axis',(0.,0.,1.));
#60009=DIRECTION('',(0.,-1.,0.));
#60010=DIRECTION('center_axis',(0.,1.,0.));
#60011=DIRECTION('ref_axis',(0.,0.,1.));
#60012=DIRECTION('',(0.,1.,0.));
#60013=DIRECTION('center_axis',(0.,-1.,0.));
#60014=DIRECTION('ref_axis',(0.,0.,-1.));
#60015=DIRECTION('center_axis',(0.,1.,0.));
#60016=DIRECTION('ref_axis',(0.,0.,1.));
#60017=DIRECTION('',(0.,-1.,0.));
#60018=DIRECTION('center_axis',(0.,1.,0.));
#60019=DIRECTION('ref_axis',(0.,0.,1.));
#60020=DIRECTION('',(0.,1.,0.));
#60021=DIRECTION('center_axis',(0.,-1.,0.));
#60022=DIRECTION('ref_axis',(0.,0.,-1.));
#60023=DIRECTION('center_axis',(0.,1.,0.));
#60024=DIRECTION('ref_axis',(0.,0.,1.));
#60025=DIRECTION('',(0.,-1.,0.));
#60026=DIRECTION('center_axis',(0.,1.,0.));
#60027=DIRECTION('ref_axis',(0.,0.,1.));
#60028=DIRECTION('',(0.,1.,0.));
#60029=DIRECTION('center_axis',(0.,-1.,0.));
#60030=DIRECTION('ref_axis',(0.,0.,-1.));
#60031=DIRECTION('center_axis',(0.,1.,0.));
#60032=DIRECTION('ref_axis',(0.,0.,1.));
#60033=DIRECTION('',(0.,-1.,0.));
#60034=DIRECTION('center_axis',(0.,1.,0.));
#60035=DIRECTION('ref_axis',(0.,0.,1.));
#60036=DIRECTION('',(0.,1.,0.));
#60037=DIRECTION('center_axis',(0.,-1.,0.));
#60038=DIRECTION('ref_axis',(0.,0.,-1.));
#60039=DIRECTION('center_axis',(0.,1.,0.));
#60040=DIRECTION('ref_axis',(0.,0.,1.));
#60041=DIRECTION('',(0.,-1.,0.));
#60042=DIRECTION('center_axis',(0.,1.,0.));
#60043=DIRECTION('ref_axis',(0.,0.,1.));
#60044=DIRECTION('',(0.,1.,0.));
#60045=DIRECTION('center_axis',(0.,-1.,0.));
#60046=DIRECTION('ref_axis',(0.,0.,-1.));
#60047=DIRECTION('center_axis',(0.,1.,0.));
#60048=DIRECTION('ref_axis',(0.,0.,1.));
#60049=DIRECTION('',(0.,-1.,0.));
#60050=DIRECTION('center_axis',(0.,1.,0.));
#60051=DIRECTION('ref_axis',(0.,0.,1.));
#60052=DIRECTION('',(0.,1.,0.));
#60053=DIRECTION('center_axis',(0.,-1.,0.));
#60054=DIRECTION('ref_axis',(0.,0.,-1.));
#60055=DIRECTION('center_axis',(0.,1.,0.));
#60056=DIRECTION('ref_axis',(0.,0.,1.));
#60057=DIRECTION('',(0.,-1.,0.));
#60058=DIRECTION('center_axis',(0.,1.,0.));
#60059=DIRECTION('ref_axis',(0.,0.,1.));
#60060=DIRECTION('',(0.,1.,0.));
#60061=DIRECTION('center_axis',(0.,-1.,0.));
#60062=DIRECTION('ref_axis',(0.,0.,-1.));
#60063=DIRECTION('center_axis',(0.,1.,0.));
#60064=DIRECTION('ref_axis',(0.,0.,1.));
#60065=DIRECTION('',(0.,-1.,0.));
#60066=DIRECTION('center_axis',(0.,1.,0.));
#60067=DIRECTION('ref_axis',(0.,0.,1.));
#60068=DIRECTION('',(0.,1.,0.));
#60069=DIRECTION('center_axis',(0.,-1.,0.));
#60070=DIRECTION('ref_axis',(0.,0.,-1.));
#60071=DIRECTION('center_axis',(0.,1.,0.));
#60072=DIRECTION('ref_axis',(0.,0.,1.));
#60073=DIRECTION('',(0.,-1.,0.));
#60074=DIRECTION('center_axis',(0.,1.,0.));
#60075=DIRECTION('ref_axis',(0.,0.,1.));
#60076=DIRECTION('',(0.,1.,0.));
#60077=DIRECTION('center_axis',(0.,-1.,0.));
#60078=DIRECTION('ref_axis',(0.,0.,-1.));
#60079=DIRECTION('center_axis',(0.,1.,0.));
#60080=DIRECTION('ref_axis',(0.,0.,1.));
#60081=DIRECTION('',(0.,-1.,0.));
#60082=DIRECTION('center_axis',(0.,1.,0.));
#60083=DIRECTION('ref_axis',(0.,0.,1.));
#60084=DIRECTION('',(0.,1.,0.));
#60085=DIRECTION('center_axis',(0.,-1.,0.));
#60086=DIRECTION('ref_axis',(0.,0.,-1.));
#60087=DIRECTION('center_axis',(0.,1.,0.));
#60088=DIRECTION('ref_axis',(0.,0.,1.));
#60089=DIRECTION('',(0.,-1.,0.));
#60090=DIRECTION('center_axis',(0.,1.,0.));
#60091=DIRECTION('ref_axis',(0.,0.,1.));
#60092=DIRECTION('',(0.,1.,0.));
#60093=DIRECTION('center_axis',(0.,-1.,0.));
#60094=DIRECTION('ref_axis',(0.,0.,-1.));
#60095=DIRECTION('center_axis',(0.,1.,0.));
#60096=DIRECTION('ref_axis',(0.,0.,1.));
#60097=DIRECTION('',(0.,-1.,0.));
#60098=DIRECTION('center_axis',(0.,1.,0.));
#60099=DIRECTION('ref_axis',(0.,0.,1.));
#60100=DIRECTION('',(0.,1.,0.));
#60101=DIRECTION('center_axis',(0.,-1.,0.));
#60102=DIRECTION('ref_axis',(0.,0.,-1.));
#60103=DIRECTION('center_axis',(0.,1.,0.));
#60104=DIRECTION('ref_axis',(0.,0.,1.));
#60105=DIRECTION('',(0.,-1.,0.));
#60106=DIRECTION('center_axis',(0.,1.,0.));
#60107=DIRECTION('ref_axis',(0.,0.,1.));
#60108=DIRECTION('',(0.,1.,0.));
#60109=DIRECTION('center_axis',(0.,-1.,0.));
#60110=DIRECTION('ref_axis',(0.,0.,-1.));
#60111=DIRECTION('center_axis',(0.,1.,0.));
#60112=DIRECTION('ref_axis',(0.,0.,1.));
#60113=DIRECTION('',(0.,-1.,0.));
#60114=DIRECTION('center_axis',(0.,1.,0.));
#60115=DIRECTION('ref_axis',(0.,0.,1.));
#60116=DIRECTION('',(0.,1.,0.));
#60117=DIRECTION('center_axis',(0.,-1.,0.));
#60118=DIRECTION('ref_axis',(0.,0.,-1.));
#60119=DIRECTION('center_axis',(0.,1.,0.));
#60120=DIRECTION('ref_axis',(0.,0.,1.));
#60121=DIRECTION('',(0.,-1.,0.));
#60122=DIRECTION('center_axis',(0.,1.,0.));
#60123=DIRECTION('ref_axis',(0.,0.,1.));
#60124=DIRECTION('',(0.,1.,0.));
#60125=DIRECTION('center_axis',(0.,-1.,0.));
#60126=DIRECTION('ref_axis',(0.,0.,-1.));
#60127=DIRECTION('center_axis',(0.,1.,0.));
#60128=DIRECTION('ref_axis',(0.,0.,1.));
#60129=DIRECTION('',(0.,-1.,0.));
#60130=DIRECTION('center_axis',(0.,1.,0.));
#60131=DIRECTION('ref_axis',(0.,0.,1.));
#60132=DIRECTION('',(0.,1.,0.));
#60133=DIRECTION('center_axis',(0.,-1.,0.));
#60134=DIRECTION('ref_axis',(0.,0.,-1.));
#60135=DIRECTION('center_axis',(0.,1.,0.));
#60136=DIRECTION('ref_axis',(0.,0.,1.));
#60137=DIRECTION('',(0.,-1.,0.));
#60138=DIRECTION('center_axis',(0.,1.,0.));
#60139=DIRECTION('ref_axis',(0.,0.,1.));
#60140=DIRECTION('',(0.,1.,0.));
#60141=DIRECTION('center_axis',(0.,-1.,0.));
#60142=DIRECTION('ref_axis',(0.,0.,-1.));
#60143=DIRECTION('center_axis',(0.,1.,0.));
#60144=DIRECTION('ref_axis',(0.,0.,1.));
#60145=DIRECTION('',(0.,-1.,0.));
#60146=DIRECTION('center_axis',(0.,1.,0.));
#60147=DIRECTION('ref_axis',(0.,0.,1.));
#60148=DIRECTION('',(0.,1.,0.));
#60149=DIRECTION('center_axis',(0.,-1.,0.));
#60150=DIRECTION('ref_axis',(0.,0.,-1.));
#60151=DIRECTION('center_axis',(0.,1.,0.));
#60152=DIRECTION('ref_axis',(0.,0.,1.));
#60153=DIRECTION('',(0.,-1.,0.));
#60154=DIRECTION('center_axis',(0.,1.,0.));
#60155=DIRECTION('ref_axis',(0.,0.,1.));
#60156=DIRECTION('',(0.,1.,0.));
#60157=DIRECTION('center_axis',(0.,-1.,0.));
#60158=DIRECTION('ref_axis',(0.,0.,-1.));
#60159=DIRECTION('center_axis',(0.,1.,0.));
#60160=DIRECTION('ref_axis',(0.,0.,1.));
#60161=DIRECTION('',(0.,-1.,0.));
#60162=DIRECTION('center_axis',(0.,1.,0.));
#60163=DIRECTION('ref_axis',(0.,0.,1.));
#60164=DIRECTION('',(0.,1.,0.));
#60165=DIRECTION('center_axis',(0.,-1.,0.));
#60166=DIRECTION('ref_axis',(0.,0.,-1.));
#60167=DIRECTION('center_axis',(0.,1.,0.));
#60168=DIRECTION('ref_axis',(0.,0.,1.));
#60169=DIRECTION('',(0.,-1.,0.));
#60170=DIRECTION('center_axis',(0.,1.,0.));
#60171=DIRECTION('ref_axis',(0.,0.,1.));
#60172=DIRECTION('',(0.,1.,0.));
#60173=DIRECTION('center_axis',(0.,-1.,0.));
#60174=DIRECTION('ref_axis',(0.,0.,-1.));
#60175=DIRECTION('center_axis',(0.,1.,0.));
#60176=DIRECTION('ref_axis',(0.,0.,1.));
#60177=DIRECTION('',(0.,-1.,0.));
#60178=DIRECTION('center_axis',(0.,1.,0.));
#60179=DIRECTION('ref_axis',(0.,0.,1.));
#60180=DIRECTION('',(0.,1.,0.));
#60181=DIRECTION('center_axis',(0.,-1.,0.));
#60182=DIRECTION('ref_axis',(0.,0.,-1.));
#60183=DIRECTION('center_axis',(0.,1.,0.));
#60184=DIRECTION('ref_axis',(0.,0.,1.));
#60185=DIRECTION('',(0.,-1.,0.));
#60186=DIRECTION('center_axis',(0.,1.,0.));
#60187=DIRECTION('ref_axis',(0.,0.,1.));
#60188=DIRECTION('',(0.,1.,0.));
#60189=DIRECTION('center_axis',(0.,-1.,0.));
#60190=DIRECTION('ref_axis',(0.,0.,-1.));
#60191=DIRECTION('center_axis',(0.,1.,0.));
#60192=DIRECTION('ref_axis',(0.,0.,1.));
#60193=DIRECTION('',(0.,-1.,0.));
#60194=DIRECTION('center_axis',(0.,1.,0.));
#60195=DIRECTION('ref_axis',(0.,0.,1.));
#60196=DIRECTION('',(0.,1.,0.));
#60197=DIRECTION('center_axis',(0.,-1.,0.));
#60198=DIRECTION('ref_axis',(0.,0.,-1.));
#60199=DIRECTION('center_axis',(0.,1.,0.));
#60200=DIRECTION('ref_axis',(0.,0.,1.));
#60201=DIRECTION('',(0.,-1.,0.));
#60202=DIRECTION('center_axis',(0.,1.,0.));
#60203=DIRECTION('ref_axis',(0.,0.,1.));
#60204=DIRECTION('',(0.,1.,0.));
#60205=DIRECTION('center_axis',(0.,-1.,0.));
#60206=DIRECTION('ref_axis',(0.,0.,-1.));
#60207=DIRECTION('center_axis',(0.,1.,0.));
#60208=DIRECTION('ref_axis',(0.,0.,1.));
#60209=DIRECTION('',(0.,-1.,0.));
#60210=DIRECTION('center_axis',(0.,1.,0.));
#60211=DIRECTION('ref_axis',(0.,0.,1.));
#60212=DIRECTION('',(0.,1.,0.));
#60213=DIRECTION('center_axis',(0.,-1.,0.));
#60214=DIRECTION('ref_axis',(0.,0.,-1.));
#60215=DIRECTION('center_axis',(0.,1.,0.));
#60216=DIRECTION('ref_axis',(0.,0.,1.));
#60217=DIRECTION('',(0.,-1.,0.));
#60218=DIRECTION('center_axis',(0.,1.,0.));
#60219=DIRECTION('ref_axis',(0.,0.,1.));
#60220=DIRECTION('',(0.,1.,0.));
#60221=DIRECTION('center_axis',(0.,-1.,0.));
#60222=DIRECTION('ref_axis',(0.,0.,-1.));
#60223=DIRECTION('center_axis',(0.,1.,0.));
#60224=DIRECTION('ref_axis',(0.,0.,1.));
#60225=DIRECTION('',(0.,-1.,0.));
#60226=DIRECTION('center_axis',(0.,1.,0.));
#60227=DIRECTION('ref_axis',(0.,0.,1.));
#60228=DIRECTION('',(0.,1.,0.));
#60229=DIRECTION('center_axis',(0.,-1.,0.));
#60230=DIRECTION('ref_axis',(0.,0.,-1.));
#60231=DIRECTION('center_axis',(0.,1.,0.));
#60232=DIRECTION('ref_axis',(0.,0.,1.));
#60233=DIRECTION('',(0.,-1.,0.));
#60234=DIRECTION('center_axis',(0.,1.,0.));
#60235=DIRECTION('ref_axis',(0.,0.,1.));
#60236=DIRECTION('',(0.,1.,0.));
#60237=DIRECTION('center_axis',(0.,-1.,0.));
#60238=DIRECTION('ref_axis',(0.,0.,-1.));
#60239=DIRECTION('center_axis',(0.,1.,0.));
#60240=DIRECTION('ref_axis',(0.,0.,1.));
#60241=DIRECTION('',(0.,-1.,0.));
#60242=DIRECTION('center_axis',(0.,1.,0.));
#60243=DIRECTION('ref_axis',(0.,0.,1.));
#60244=DIRECTION('',(0.,1.,0.));
#60245=DIRECTION('center_axis',(0.,-1.,0.));
#60246=DIRECTION('ref_axis',(0.,0.,-1.));
#60247=DIRECTION('center_axis',(0.,1.,0.));
#60248=DIRECTION('ref_axis',(0.,0.,1.));
#60249=DIRECTION('',(0.,-1.,0.));
#60250=DIRECTION('center_axis',(0.,1.,0.));
#60251=DIRECTION('ref_axis',(0.,0.,1.));
#60252=DIRECTION('',(0.,1.,0.));
#60253=DIRECTION('center_axis',(0.,-1.,0.));
#60254=DIRECTION('ref_axis',(0.,0.,-1.));
#60255=DIRECTION('center_axis',(0.,1.,0.));
#60256=DIRECTION('ref_axis',(0.,0.,1.));
#60257=DIRECTION('',(0.,-1.,0.));
#60258=DIRECTION('center_axis',(0.,1.,0.));
#60259=DIRECTION('ref_axis',(0.,0.,1.));
#60260=DIRECTION('',(0.,1.,0.));
#60261=DIRECTION('center_axis',(0.,-1.,0.));
#60262=DIRECTION('ref_axis',(0.,0.,-1.));
#60263=DIRECTION('center_axis',(0.,1.,0.));
#60264=DIRECTION('ref_axis',(0.,0.,1.));
#60265=DIRECTION('center_axis',(0.,1.,0.));
#60266=DIRECTION('ref_axis',(0.,0.,1.));
#60267=DIRECTION('',(0.,-1.,0.));
#60268=DIRECTION('center_axis',(0.,-1.,0.));
#60269=DIRECTION('ref_axis',(0.,0.,-1.));
#60270=DIRECTION('center_axis',(0.,1.,0.));
#60271=DIRECTION('ref_axis',(0.,0.,1.));
#60272=DIRECTION('center_axis',(0.,-1.,0.));
#60273=DIRECTION('ref_axis',(0.,0.,-1.));
#60274=DIRECTION('',(0.,1.,0.));
#60275=DIRECTION('center_axis',(0.,-1.,0.));
#60276=DIRECTION('ref_axis',(0.,0.,-1.));
#60277=DIRECTION('center_axis',(0.,1.,0.));
#60278=DIRECTION('ref_axis',(0.,0.,1.));
#60279=DIRECTION('center_axis',(0.,1.,0.));
#60280=DIRECTION('ref_axis',(0.,0.,1.));
#60281=DIRECTION('',(0.,-1.,0.));
#60282=DIRECTION('center_axis',(0.,-1.,0.));
#60283=DIRECTION('ref_axis',(0.,0.,-1.));
#60284=DIRECTION('center_axis',(0.,1.,0.));
#60285=DIRECTION('ref_axis',(0.,0.,1.));
#60286=DIRECTION('center_axis',(0.,-1.,0.));
#60287=DIRECTION('ref_axis',(0.,0.,-1.));
#60288=DIRECTION('',(0.,1.,0.));
#60289=DIRECTION('center_axis',(0.,-1.,0.));
#60290=DIRECTION('ref_axis',(0.,0.,-1.));
#60291=DIRECTION('center_axis',(0.,1.,0.));
#60292=DIRECTION('ref_axis',(0.,0.,1.));
#60293=DIRECTION('center_axis',(0.,1.,0.));
#60294=DIRECTION('ref_axis',(0.,0.,1.));
#60295=DIRECTION('',(0.,-1.,0.));
#60296=DIRECTION('center_axis',(0.,-1.,0.));
#60297=DIRECTION('ref_axis',(0.,0.,-1.));
#60298=DIRECTION('center_axis',(0.,1.,0.));
#60299=DIRECTION('ref_axis',(0.,0.,1.));
#60300=DIRECTION('center_axis',(0.,-1.,0.));
#60301=DIRECTION('ref_axis',(0.,0.,-1.));
#60302=DIRECTION('',(0.,1.,0.));
#60303=DIRECTION('center_axis',(0.,-1.,0.));
#60304=DIRECTION('ref_axis',(0.,0.,-1.));
#60305=DIRECTION('center_axis',(0.,1.,0.));
#60306=DIRECTION('ref_axis',(0.,0.,1.));
#60307=DIRECTION('center_axis',(0.,1.,0.));
#60308=DIRECTION('ref_axis',(0.,0.,1.));
#60309=DIRECTION('',(0.,-1.,0.));
#60310=DIRECTION('center_axis',(0.,-1.,0.));
#60311=DIRECTION('ref_axis',(0.,0.,-1.));
#60312=DIRECTION('center_axis',(0.,1.,0.));
#60313=DIRECTION('ref_axis',(0.,0.,1.));
#60314=DIRECTION('center_axis',(0.,-1.,0.));
#60315=DIRECTION('ref_axis',(0.,0.,-1.));
#60316=DIRECTION('',(0.,1.,0.));
#60317=DIRECTION('center_axis',(0.,-1.,0.));
#60318=DIRECTION('ref_axis',(0.,0.,-1.));
#60319=DIRECTION('center_axis',(0.,1.,0.));
#60320=DIRECTION('ref_axis',(0.,0.,1.));
#60321=DIRECTION('center_axis',(0.,1.,0.));
#60322=DIRECTION('ref_axis',(0.,0.,1.));
#60323=DIRECTION('',(0.,-1.,0.));
#60324=DIRECTION('center_axis',(0.,-1.,0.));
#60325=DIRECTION('ref_axis',(0.,0.,-1.));
#60326=DIRECTION('center_axis',(0.,1.,0.));
#60327=DIRECTION('ref_axis',(0.,0.,1.));
#60328=DIRECTION('center_axis',(0.,-1.,0.));
#60329=DIRECTION('ref_axis',(0.,0.,-1.));
#60330=DIRECTION('',(0.,1.,0.));
#60331=DIRECTION('center_axis',(0.,-1.,0.));
#60332=DIRECTION('ref_axis',(0.,0.,-1.));
#60333=DIRECTION('center_axis',(0.,1.,0.));
#60334=DIRECTION('ref_axis',(0.,0.,1.));
#60335=DIRECTION('center_axis',(0.,1.,0.));
#60336=DIRECTION('ref_axis',(0.,0.,1.));
#60337=DIRECTION('',(0.,-1.,0.));
#60338=DIRECTION('center_axis',(0.,-1.,0.));
#60339=DIRECTION('ref_axis',(0.,0.,-1.));
#60340=DIRECTION('center_axis',(0.,1.,0.));
#60341=DIRECTION('ref_axis',(0.,0.,1.));
#60342=DIRECTION('center_axis',(0.,-1.,0.));
#60343=DIRECTION('ref_axis',(0.,0.,-1.));
#60344=DIRECTION('',(0.,1.,0.));
#60345=DIRECTION('center_axis',(0.,-1.,0.));
#60346=DIRECTION('ref_axis',(0.,0.,-1.));
#60347=DIRECTION('center_axis',(0.,1.,0.));
#60348=DIRECTION('ref_axis',(0.,0.,1.));
#60349=DIRECTION('center_axis',(0.,1.,0.));
#60350=DIRECTION('ref_axis',(0.,0.,1.));
#60351=DIRECTION('',(0.,-1.,0.));
#60352=DIRECTION('center_axis',(0.,-1.,0.));
#60353=DIRECTION('ref_axis',(0.,0.,-1.));
#60354=DIRECTION('center_axis',(0.,1.,0.));
#60355=DIRECTION('ref_axis',(0.,0.,1.));
#60356=DIRECTION('center_axis',(0.,-1.,0.));
#60357=DIRECTION('ref_axis',(0.,0.,-1.));
#60358=DIRECTION('',(0.,1.,0.));
#60359=DIRECTION('center_axis',(0.,-1.,0.));
#60360=DIRECTION('ref_axis',(0.,0.,-1.));
#60361=DIRECTION('center_axis',(0.,1.,0.));
#60362=DIRECTION('ref_axis',(0.,0.,1.));
#60363=DIRECTION('center_axis',(0.,1.,0.));
#60364=DIRECTION('ref_axis',(0.,0.,1.));
#60365=DIRECTION('',(0.,-1.,0.));
#60366=DIRECTION('center_axis',(0.,-1.,0.));
#60367=DIRECTION('ref_axis',(0.,0.,-1.));
#60368=DIRECTION('center_axis',(0.,1.,0.));
#60369=DIRECTION('ref_axis',(0.,0.,1.));
#60370=DIRECTION('center_axis',(0.,-1.,0.));
#60371=DIRECTION('ref_axis',(0.,0.,-1.));
#60372=DIRECTION('',(0.,1.,0.));
#60373=DIRECTION('center_axis',(0.,-1.,0.));
#60374=DIRECTION('ref_axis',(0.,0.,-1.));
#60375=DIRECTION('center_axis',(0.,1.,0.));
#60376=DIRECTION('ref_axis',(0.,0.,1.));
#60377=DIRECTION('center_axis',(0.,1.,0.));
#60378=DIRECTION('ref_axis',(0.,0.,1.));
#60379=DIRECTION('',(0.,-1.,0.));
#60380=DIRECTION('center_axis',(0.,-1.,0.));
#60381=DIRECTION('ref_axis',(0.,0.,-1.));
#60382=DIRECTION('center_axis',(0.,1.,0.));
#60383=DIRECTION('ref_axis',(0.,0.,1.));
#60384=DIRECTION('center_axis',(0.,-1.,0.));
#60385=DIRECTION('ref_axis',(0.,0.,-1.));
#60386=DIRECTION('',(0.,1.,0.));
#60387=DIRECTION('center_axis',(0.,-1.,0.));
#60388=DIRECTION('ref_axis',(0.,0.,-1.));
#60389=DIRECTION('center_axis',(0.,1.,0.));
#60390=DIRECTION('ref_axis',(0.,0.,1.));
#60391=DIRECTION('center_axis',(0.,1.,0.));
#60392=DIRECTION('ref_axis',(0.,0.,1.));
#60393=DIRECTION('',(0.,-1.,0.));
#60394=DIRECTION('center_axis',(0.,-1.,0.));
#60395=DIRECTION('ref_axis',(0.,0.,-1.));
#60396=DIRECTION('center_axis',(0.,1.,0.));
#60397=DIRECTION('ref_axis',(0.,0.,1.));
#60398=DIRECTION('center_axis',(0.,-1.,0.));
#60399=DIRECTION('ref_axis',(0.,0.,-1.));
#60400=DIRECTION('',(0.,1.,0.));
#60401=DIRECTION('center_axis',(0.,-1.,0.));
#60402=DIRECTION('ref_axis',(0.,0.,-1.));
#60403=DIRECTION('center_axis',(0.,1.,0.));
#60404=DIRECTION('ref_axis',(0.,0.,1.));
#60405=DIRECTION('center_axis',(0.,1.,0.));
#60406=DIRECTION('ref_axis',(0.,0.,1.));
#60407=DIRECTION('',(0.,-1.,0.));
#60408=DIRECTION('center_axis',(0.,-1.,0.));
#60409=DIRECTION('ref_axis',(0.,0.,-1.));
#60410=DIRECTION('center_axis',(0.,1.,0.));
#60411=DIRECTION('ref_axis',(0.,0.,1.));
#60412=DIRECTION('center_axis',(0.,-1.,0.));
#60413=DIRECTION('ref_axis',(0.,0.,-1.));
#60414=DIRECTION('',(0.,1.,0.));
#60415=DIRECTION('center_axis',(0.,-1.,0.));
#60416=DIRECTION('ref_axis',(0.,0.,-1.));
#60417=DIRECTION('center_axis',(0.,1.,0.));
#60418=DIRECTION('ref_axis',(0.,0.,1.));
#60419=DIRECTION('center_axis',(0.,1.,0.));
#60420=DIRECTION('ref_axis',(0.,0.,1.));
#60421=DIRECTION('',(0.,-1.,0.));
#60422=DIRECTION('center_axis',(0.,-1.,0.));
#60423=DIRECTION('ref_axis',(0.,0.,-1.));
#60424=DIRECTION('center_axis',(0.,1.,0.));
#60425=DIRECTION('ref_axis',(0.,0.,1.));
#60426=DIRECTION('center_axis',(0.,-1.,0.));
#60427=DIRECTION('ref_axis',(0.,0.,-1.));
#60428=DIRECTION('',(0.,1.,0.));
#60429=DIRECTION('center_axis',(0.,-1.,0.));
#60430=DIRECTION('ref_axis',(0.,0.,-1.));
#60431=DIRECTION('center_axis',(0.,1.,0.));
#60432=DIRECTION('ref_axis',(0.,0.,1.));
#60433=DIRECTION('center_axis',(0.,1.,0.));
#60434=DIRECTION('ref_axis',(0.,0.,1.));
#60435=DIRECTION('',(0.,-1.,0.));
#60436=DIRECTION('center_axis',(0.,-1.,0.));
#60437=DIRECTION('ref_axis',(0.,0.,-1.));
#60438=DIRECTION('center_axis',(0.,1.,0.));
#60439=DIRECTION('ref_axis',(0.,0.,1.));
#60440=DIRECTION('center_axis',(0.,-1.,0.));
#60441=DIRECTION('ref_axis',(0.,0.,-1.));
#60442=DIRECTION('',(0.,1.,0.));
#60443=DIRECTION('center_axis',(0.,-1.,0.));
#60444=DIRECTION('ref_axis',(0.,0.,-1.));
#60445=DIRECTION('center_axis',(0.,1.,0.));
#60446=DIRECTION('ref_axis',(0.,0.,1.));
#60447=DIRECTION('center_axis',(0.,1.,0.));
#60448=DIRECTION('ref_axis',(0.,0.,1.));
#60449=DIRECTION('',(0.,-1.,0.));
#60450=DIRECTION('center_axis',(0.,-1.,0.));
#60451=DIRECTION('ref_axis',(0.,0.,-1.));
#60452=DIRECTION('center_axis',(0.,1.,0.));
#60453=DIRECTION('ref_axis',(0.,0.,1.));
#60454=DIRECTION('center_axis',(0.,-1.,0.));
#60455=DIRECTION('ref_axis',(0.,0.,-1.));
#60456=DIRECTION('',(0.,1.,0.));
#60457=DIRECTION('center_axis',(0.,-1.,0.));
#60458=DIRECTION('ref_axis',(0.,0.,-1.));
#60459=DIRECTION('center_axis',(0.,1.,0.));
#60460=DIRECTION('ref_axis',(0.,0.,1.));
#60461=DIRECTION('center_axis',(0.,1.,0.));
#60462=DIRECTION('ref_axis',(0.,0.,1.));
#60463=DIRECTION('',(0.,-1.,0.));
#60464=DIRECTION('center_axis',(0.,-1.,0.));
#60465=DIRECTION('ref_axis',(0.,0.,-1.));
#60466=DIRECTION('center_axis',(0.,1.,0.));
#60467=DIRECTION('ref_axis',(0.,0.,1.));
#60468=DIRECTION('center_axis',(0.,-1.,0.));
#60469=DIRECTION('ref_axis',(0.,0.,-1.));
#60470=DIRECTION('',(0.,1.,0.));
#60471=DIRECTION('center_axis',(0.,-1.,0.));
#60472=DIRECTION('ref_axis',(0.,0.,-1.));
#60473=DIRECTION('center_axis',(0.,1.,0.));
#60474=DIRECTION('ref_axis',(0.,0.,1.));
#60475=DIRECTION('center_axis',(0.,1.,0.));
#60476=DIRECTION('ref_axis',(0.,0.,1.));
#60477=DIRECTION('',(0.,-1.,0.));
#60478=DIRECTION('center_axis',(0.,-1.,0.));
#60479=DIRECTION('ref_axis',(0.,0.,-1.));
#60480=DIRECTION('center_axis',(0.,1.,0.));
#60481=DIRECTION('ref_axis',(0.,0.,1.));
#60482=DIRECTION('center_axis',(0.,-1.,0.));
#60483=DIRECTION('ref_axis',(0.,0.,-1.));
#60484=DIRECTION('',(0.,1.,0.));
#60485=DIRECTION('center_axis',(0.,-1.,0.));
#60486=DIRECTION('ref_axis',(0.,0.,-1.));
#60487=DIRECTION('center_axis',(0.,1.,0.));
#60488=DIRECTION('ref_axis',(0.,0.,1.));
#60489=DIRECTION('center_axis',(0.,1.,0.));
#60490=DIRECTION('ref_axis',(0.,0.,1.));
#60491=DIRECTION('',(0.,-1.,0.));
#60492=DIRECTION('center_axis',(0.,-1.,0.));
#60493=DIRECTION('ref_axis',(0.,0.,-1.));
#60494=DIRECTION('center_axis',(0.,1.,0.));
#60495=DIRECTION('ref_axis',(0.,0.,1.));
#60496=DIRECTION('center_axis',(0.,-1.,0.));
#60497=DIRECTION('ref_axis',(0.,0.,-1.));
#60498=DIRECTION('',(0.,1.,0.));
#60499=DIRECTION('center_axis',(0.,-1.,0.));
#60500=DIRECTION('ref_axis',(0.,0.,-1.));
#60501=DIRECTION('center_axis',(0.,1.,0.));
#60502=DIRECTION('ref_axis',(0.,0.,1.));
#60503=DIRECTION('center_axis',(0.,1.,0.));
#60504=DIRECTION('ref_axis',(0.,0.,1.));
#60505=DIRECTION('',(0.,-1.,0.));
#60506=DIRECTION('center_axis',(0.,-1.,0.));
#60507=DIRECTION('ref_axis',(0.,0.,-1.));
#60508=DIRECTION('center_axis',(0.,1.,0.));
#60509=DIRECTION('ref_axis',(0.,0.,1.));
#60510=DIRECTION('center_axis',(0.,-1.,0.));
#60511=DIRECTION('ref_axis',(0.,0.,-1.));
#60512=DIRECTION('',(0.,1.,0.));
#60513=DIRECTION('center_axis',(0.,-1.,0.));
#60514=DIRECTION('ref_axis',(0.,0.,-1.));
#60515=DIRECTION('center_axis',(0.,1.,0.));
#60516=DIRECTION('ref_axis',(0.,0.,1.));
#60517=DIRECTION('center_axis',(0.,1.,0.));
#60518=DIRECTION('ref_axis',(0.,0.,1.));
#60519=DIRECTION('',(0.,-1.,0.));
#60520=DIRECTION('center_axis',(0.,-1.,0.));
#60521=DIRECTION('ref_axis',(0.,0.,-1.));
#60522=DIRECTION('center_axis',(0.,1.,0.));
#60523=DIRECTION('ref_axis',(0.,0.,1.));
#60524=DIRECTION('center_axis',(0.,-1.,0.));
#60525=DIRECTION('ref_axis',(0.,0.,-1.));
#60526=DIRECTION('',(0.,1.,0.));
#60527=DIRECTION('center_axis',(0.,-1.,0.));
#60528=DIRECTION('ref_axis',(0.,0.,-1.));
#60529=DIRECTION('center_axis',(0.,1.,0.));
#60530=DIRECTION('ref_axis',(0.,0.,1.));
#60531=DIRECTION('center_axis',(0.,1.,0.));
#60532=DIRECTION('ref_axis',(0.,0.,1.));
#60533=DIRECTION('',(0.,-1.,0.));
#60534=DIRECTION('center_axis',(0.,-1.,0.));
#60535=DIRECTION('ref_axis',(0.,0.,-1.));
#60536=DIRECTION('center_axis',(0.,1.,0.));
#60537=DIRECTION('ref_axis',(0.,0.,1.));
#60538=DIRECTION('center_axis',(0.,-1.,0.));
#60539=DIRECTION('ref_axis',(0.,0.,-1.));
#60540=DIRECTION('',(0.,1.,0.));
#60541=DIRECTION('center_axis',(0.,-1.,0.));
#60542=DIRECTION('ref_axis',(0.,0.,-1.));
#60543=DIRECTION('center_axis',(0.,1.,0.));
#60544=DIRECTION('ref_axis',(0.,0.,1.));
#60545=DIRECTION('center_axis',(0.,1.,0.));
#60546=DIRECTION('ref_axis',(0.,0.,1.));
#60547=DIRECTION('',(0.,-1.,0.));
#60548=DIRECTION('center_axis',(0.,-1.,0.));
#60549=DIRECTION('ref_axis',(0.,0.,-1.));
#60550=DIRECTION('center_axis',(0.,1.,0.));
#60551=DIRECTION('ref_axis',(0.,0.,1.));
#60552=DIRECTION('center_axis',(0.,-1.,0.));
#60553=DIRECTION('ref_axis',(0.,0.,-1.));
#60554=DIRECTION('',(0.,1.,0.));
#60555=DIRECTION('center_axis',(0.,-1.,0.));
#60556=DIRECTION('ref_axis',(0.,0.,-1.));
#60557=DIRECTION('center_axis',(0.,1.,0.));
#60558=DIRECTION('ref_axis',(0.,0.,1.));
#60559=DIRECTION('center_axis',(0.,1.,0.));
#60560=DIRECTION('ref_axis',(0.,0.,1.));
#60561=DIRECTION('',(0.,-1.,0.));
#60562=DIRECTION('center_axis',(0.,-1.,0.));
#60563=DIRECTION('ref_axis',(0.,0.,-1.));
#60564=DIRECTION('center_axis',(0.,1.,0.));
#60565=DIRECTION('ref_axis',(0.,0.,1.));
#60566=DIRECTION('center_axis',(0.,-1.,0.));
#60567=DIRECTION('ref_axis',(0.,0.,-1.));
#60568=DIRECTION('',(0.,1.,0.));
#60569=DIRECTION('center_axis',(0.,-1.,0.));
#60570=DIRECTION('ref_axis',(0.,0.,-1.));
#60571=DIRECTION('center_axis',(0.,1.,0.));
#60572=DIRECTION('ref_axis',(0.,0.,1.));
#60573=DIRECTION('center_axis',(0.,1.,0.));
#60574=DIRECTION('ref_axis',(0.,0.,1.));
#60575=DIRECTION('',(0.,-1.,0.));
#60576=DIRECTION('center_axis',(0.,-1.,0.));
#60577=DIRECTION('ref_axis',(0.,0.,-1.));
#60578=DIRECTION('center_axis',(0.,1.,0.));
#60579=DIRECTION('ref_axis',(0.,0.,1.));
#60580=DIRECTION('center_axis',(0.,-1.,0.));
#60581=DIRECTION('ref_axis',(0.,0.,-1.));
#60582=DIRECTION('',(0.,1.,0.));
#60583=DIRECTION('center_axis',(0.,-1.,0.));
#60584=DIRECTION('ref_axis',(0.,0.,-1.));
#60585=DIRECTION('center_axis',(0.,1.,0.));
#60586=DIRECTION('ref_axis',(0.,0.,1.));
#60587=DIRECTION('center_axis',(0.,1.,0.));
#60588=DIRECTION('ref_axis',(0.,0.,1.));
#60589=DIRECTION('',(0.,-1.,0.));
#60590=DIRECTION('center_axis',(0.,-1.,0.));
#60591=DIRECTION('ref_axis',(0.,0.,-1.));
#60592=DIRECTION('center_axis',(0.,1.,0.));
#60593=DIRECTION('ref_axis',(0.,0.,1.));
#60594=DIRECTION('center_axis',(0.,-1.,0.));
#60595=DIRECTION('ref_axis',(0.,0.,-1.));
#60596=DIRECTION('',(0.,1.,0.));
#60597=DIRECTION('center_axis',(0.,-1.,0.));
#60598=DIRECTION('ref_axis',(0.,0.,-1.));
#60599=DIRECTION('center_axis',(0.,1.,0.));
#60600=DIRECTION('ref_axis',(0.,0.,1.));
#60601=DIRECTION('center_axis',(0.,1.,0.));
#60602=DIRECTION('ref_axis',(0.,0.,1.));
#60603=DIRECTION('',(0.,-1.,0.));
#60604=DIRECTION('center_axis',(0.,-1.,0.));
#60605=DIRECTION('ref_axis',(0.,0.,-1.));
#60606=DIRECTION('center_axis',(0.,1.,0.));
#60607=DIRECTION('ref_axis',(0.,0.,1.));
#60608=DIRECTION('center_axis',(0.,-1.,0.));
#60609=DIRECTION('ref_axis',(0.,0.,-1.));
#60610=DIRECTION('',(0.,1.,0.));
#60611=DIRECTION('center_axis',(0.,-1.,0.));
#60612=DIRECTION('ref_axis',(0.,0.,-1.));
#60613=DIRECTION('center_axis',(0.,1.,0.));
#60614=DIRECTION('ref_axis',(0.,0.,1.));
#60615=DIRECTION('center_axis',(0.,1.,0.));
#60616=DIRECTION('ref_axis',(0.,0.,1.));
#60617=DIRECTION('',(0.,-1.,0.));
#60618=DIRECTION('center_axis',(0.,-1.,0.));
#60619=DIRECTION('ref_axis',(0.,0.,-1.));
#60620=DIRECTION('center_axis',(0.,1.,0.));
#60621=DIRECTION('ref_axis',(0.,0.,1.));
#60622=DIRECTION('center_axis',(0.,-1.,0.));
#60623=DIRECTION('ref_axis',(0.,0.,-1.));
#60624=DIRECTION('',(0.,1.,0.));
#60625=DIRECTION('center_axis',(0.,-1.,0.));
#60626=DIRECTION('ref_axis',(0.,0.,-1.));
#60627=DIRECTION('center_axis',(0.,1.,0.));
#60628=DIRECTION('ref_axis',(0.,0.,1.));
#60629=DIRECTION('center_axis',(0.,1.,0.));
#60630=DIRECTION('ref_axis',(0.,0.,1.));
#60631=DIRECTION('',(0.,-1.,0.));
#60632=DIRECTION('center_axis',(0.,-1.,0.));
#60633=DIRECTION('ref_axis',(0.,0.,-1.));
#60634=DIRECTION('center_axis',(0.,1.,0.));
#60635=DIRECTION('ref_axis',(0.,0.,1.));
#60636=DIRECTION('center_axis',(0.,-1.,0.));
#60637=DIRECTION('ref_axis',(0.,0.,-1.));
#60638=DIRECTION('',(0.,1.,0.));
#60639=DIRECTION('center_axis',(0.,-1.,0.));
#60640=DIRECTION('ref_axis',(0.,0.,-1.));
#60641=DIRECTION('center_axis',(0.,1.,0.));
#60642=DIRECTION('ref_axis',(0.,0.,1.));
#60643=DIRECTION('center_axis',(0.,1.,0.));
#60644=DIRECTION('ref_axis',(0.,0.,1.));
#60645=DIRECTION('',(0.,-1.,0.));
#60646=DIRECTION('center_axis',(0.,-1.,0.));
#60647=DIRECTION('ref_axis',(0.,0.,-1.));
#60648=DIRECTION('center_axis',(0.,1.,0.));
#60649=DIRECTION('ref_axis',(0.,0.,1.));
#60650=DIRECTION('center_axis',(0.,-1.,0.));
#60651=DIRECTION('ref_axis',(0.,0.,-1.));
#60652=DIRECTION('',(0.,1.,0.));
#60653=DIRECTION('center_axis',(0.,-1.,0.));
#60654=DIRECTION('ref_axis',(0.,0.,-1.));
#60655=DIRECTION('center_axis',(0.,1.,0.));
#60656=DIRECTION('ref_axis',(0.,0.,1.));
#60657=DIRECTION('center_axis',(0.,1.,0.));
#60658=DIRECTION('ref_axis',(0.,0.,1.));
#60659=DIRECTION('',(0.,-1.,0.));
#60660=DIRECTION('center_axis',(0.,-1.,0.));
#60661=DIRECTION('ref_axis',(0.,0.,-1.));
#60662=DIRECTION('center_axis',(0.,1.,0.));
#60663=DIRECTION('ref_axis',(0.,0.,1.));
#60664=DIRECTION('center_axis',(0.,-1.,0.));
#60665=DIRECTION('ref_axis',(0.,0.,-1.));
#60666=DIRECTION('',(0.,1.,0.));
#60667=DIRECTION('center_axis',(0.,-1.,0.));
#60668=DIRECTION('ref_axis',(0.,0.,-1.));
#60669=DIRECTION('center_axis',(0.,1.,0.));
#60670=DIRECTION('ref_axis',(0.,0.,1.));
#60671=DIRECTION('center_axis',(0.,1.,0.));
#60672=DIRECTION('ref_axis',(0.,0.,1.));
#60673=DIRECTION('',(0.,-1.,0.));
#60674=DIRECTION('center_axis',(0.,-1.,0.));
#60675=DIRECTION('ref_axis',(0.,0.,-1.));
#60676=DIRECTION('center_axis',(0.,1.,0.));
#60677=DIRECTION('ref_axis',(0.,0.,1.));
#60678=DIRECTION('center_axis',(0.,-1.,0.));
#60679=DIRECTION('ref_axis',(0.,0.,-1.));
#60680=DIRECTION('',(0.,1.,0.));
#60681=DIRECTION('center_axis',(0.,-1.,0.));
#60682=DIRECTION('ref_axis',(0.,0.,-1.));
#60683=DIRECTION('center_axis',(0.,1.,0.));
#60684=DIRECTION('ref_axis',(0.,0.,1.));
#60685=DIRECTION('center_axis',(0.,1.,0.));
#60686=DIRECTION('ref_axis',(0.,0.,1.));
#60687=DIRECTION('',(0.,-1.,0.));
#60688=DIRECTION('center_axis',(0.,-1.,0.));
#60689=DIRECTION('ref_axis',(0.,0.,-1.));
#60690=DIRECTION('center_axis',(0.,1.,0.));
#60691=DIRECTION('ref_axis',(0.,0.,1.));
#60692=DIRECTION('center_axis',(0.,-1.,0.));
#60693=DIRECTION('ref_axis',(0.,0.,-1.));
#60694=DIRECTION('',(0.,1.,0.));
#60695=DIRECTION('center_axis',(0.,-1.,0.));
#60696=DIRECTION('ref_axis',(0.,0.,-1.));
#60697=DIRECTION('center_axis',(0.,1.,0.));
#60698=DIRECTION('ref_axis',(0.,0.,1.));
#60699=DIRECTION('center_axis',(0.,1.,0.));
#60700=DIRECTION('ref_axis',(0.,0.,1.));
#60701=DIRECTION('',(0.,-1.,0.));
#60702=DIRECTION('center_axis',(0.,-1.,0.));
#60703=DIRECTION('ref_axis',(0.,0.,-1.));
#60704=DIRECTION('center_axis',(0.,1.,0.));
#60705=DIRECTION('ref_axis',(0.,0.,1.));
#60706=DIRECTION('center_axis',(0.,-1.,0.));
#60707=DIRECTION('ref_axis',(0.,0.,-1.));
#60708=DIRECTION('',(0.,1.,0.));
#60709=DIRECTION('center_axis',(0.,-1.,0.));
#60710=DIRECTION('ref_axis',(0.,0.,-1.));
#60711=DIRECTION('center_axis',(0.,1.,0.));
#60712=DIRECTION('ref_axis',(0.,0.,1.));
#60713=DIRECTION('center_axis',(0.,1.,0.));
#60714=DIRECTION('ref_axis',(0.,0.,1.));
#60715=DIRECTION('',(0.,-1.,0.));
#60716=DIRECTION('center_axis',(0.,-1.,0.));
#60717=DIRECTION('ref_axis',(0.,0.,-1.));
#60718=DIRECTION('center_axis',(0.,1.,0.));
#60719=DIRECTION('ref_axis',(0.,0.,1.));
#60720=DIRECTION('center_axis',(0.,-1.,0.));
#60721=DIRECTION('ref_axis',(0.,0.,-1.));
#60722=DIRECTION('',(0.,1.,0.));
#60723=DIRECTION('center_axis',(0.,-1.,0.));
#60724=DIRECTION('ref_axis',(0.,0.,-1.));
#60725=DIRECTION('center_axis',(0.,1.,0.));
#60726=DIRECTION('ref_axis',(0.,0.,1.));
#60727=DIRECTION('center_axis',(0.,1.,0.));
#60728=DIRECTION('ref_axis',(0.,0.,1.));
#60729=DIRECTION('',(0.,-1.,0.));
#60730=DIRECTION('center_axis',(0.,-1.,0.));
#60731=DIRECTION('ref_axis',(0.,0.,-1.));
#60732=DIRECTION('center_axis',(0.,1.,0.));
#60733=DIRECTION('ref_axis',(0.,0.,1.));
#60734=DIRECTION('center_axis',(0.,-1.,0.));
#60735=DIRECTION('ref_axis',(0.,0.,-1.));
#60736=DIRECTION('',(0.,1.,0.));
#60737=DIRECTION('center_axis',(0.,-1.,0.));
#60738=DIRECTION('ref_axis',(0.,0.,-1.));
#60739=DIRECTION('center_axis',(0.,1.,0.));
#60740=DIRECTION('ref_axis',(0.,0.,1.));
#60741=DIRECTION('center_axis',(0.,1.,0.));
#60742=DIRECTION('ref_axis',(0.,0.,1.));
#60743=DIRECTION('',(0.,-1.,0.));
#60744=DIRECTION('center_axis',(0.,-1.,0.));
#60745=DIRECTION('ref_axis',(0.,0.,-1.));
#60746=DIRECTION('center_axis',(0.,1.,0.));
#60747=DIRECTION('ref_axis',(0.,0.,1.));
#60748=DIRECTION('center_axis',(0.,-1.,0.));
#60749=DIRECTION('ref_axis',(0.,0.,-1.));
#60750=DIRECTION('',(0.,1.,0.));
#60751=DIRECTION('center_axis',(0.,-1.,0.));
#60752=DIRECTION('ref_axis',(0.,0.,-1.));
#60753=DIRECTION('center_axis',(0.,1.,0.));
#60754=DIRECTION('ref_axis',(0.,0.,1.));
#60755=DIRECTION('center_axis',(0.,1.,0.));
#60756=DIRECTION('ref_axis',(0.,0.,1.));
#60757=DIRECTION('',(0.,-1.,0.));
#60758=DIRECTION('center_axis',(0.,-1.,0.));
#60759=DIRECTION('ref_axis',(0.,0.,-1.));
#60760=DIRECTION('center_axis',(0.,1.,0.));
#60761=DIRECTION('ref_axis',(0.,0.,1.));
#60762=DIRECTION('center_axis',(0.,-1.,0.));
#60763=DIRECTION('ref_axis',(0.,0.,-1.));
#60764=DIRECTION('',(0.,1.,0.));
#60765=DIRECTION('center_axis',(0.,-1.,0.));
#60766=DIRECTION('ref_axis',(0.,0.,-1.));
#60767=DIRECTION('center_axis',(0.,1.,0.));
#60768=DIRECTION('ref_axis',(0.,0.,1.));
#60769=DIRECTION('center_axis',(0.,1.,0.));
#60770=DIRECTION('ref_axis',(0.,0.,1.));
#60771=DIRECTION('',(0.,-1.,0.));
#60772=DIRECTION('center_axis',(0.,-1.,0.));
#60773=DIRECTION('ref_axis',(0.,0.,-1.));
#60774=DIRECTION('center_axis',(0.,1.,0.));
#60775=DIRECTION('ref_axis',(0.,0.,1.));
#60776=DIRECTION('center_axis',(0.,-1.,0.));
#60777=DIRECTION('ref_axis',(0.,0.,-1.));
#60778=DIRECTION('',(0.,1.,0.));
#60779=DIRECTION('center_axis',(0.,-1.,0.));
#60780=DIRECTION('ref_axis',(0.,0.,-1.));
#60781=DIRECTION('center_axis',(0.,1.,0.));
#60782=DIRECTION('ref_axis',(0.,0.,1.));
#60783=DIRECTION('center_axis',(0.,1.,0.));
#60784=DIRECTION('ref_axis',(0.,0.,1.));
#60785=DIRECTION('',(0.,-1.,0.));
#60786=DIRECTION('center_axis',(0.,-1.,0.));
#60787=DIRECTION('ref_axis',(0.,0.,-1.));
#60788=DIRECTION('center_axis',(0.,1.,0.));
#60789=DIRECTION('ref_axis',(0.,0.,1.));
#60790=DIRECTION('center_axis',(0.,-1.,0.));
#60791=DIRECTION('ref_axis',(0.,0.,-1.));
#60792=DIRECTION('',(0.,1.,0.));
#60793=DIRECTION('center_axis',(0.,-1.,0.));
#60794=DIRECTION('ref_axis',(0.,0.,-1.));
#60795=DIRECTION('center_axis',(0.,1.,0.));
#60796=DIRECTION('ref_axis',(0.,0.,1.));
#60797=DIRECTION('center_axis',(0.,1.,0.));
#60798=DIRECTION('ref_axis',(0.,0.,1.));
#60799=DIRECTION('',(0.,-1.,0.));
#60800=DIRECTION('center_axis',(0.,-1.,0.));
#60801=DIRECTION('ref_axis',(0.,0.,-1.));
#60802=DIRECTION('center_axis',(0.,1.,0.));
#60803=DIRECTION('ref_axis',(0.,0.,1.));
#60804=DIRECTION('center_axis',(0.,-1.,0.));
#60805=DIRECTION('ref_axis',(0.,0.,-1.));
#60806=DIRECTION('',(0.,1.,0.));
#60807=DIRECTION('center_axis',(0.,-1.,0.));
#60808=DIRECTION('ref_axis',(0.,0.,-1.));
#60809=DIRECTION('center_axis',(0.,1.,0.));
#60810=DIRECTION('ref_axis',(0.,0.,1.));
#60811=DIRECTION('center_axis',(0.,1.,0.));
#60812=DIRECTION('ref_axis',(0.,0.,1.));
#60813=DIRECTION('',(0.,-1.,0.));
#60814=DIRECTION('center_axis',(0.,-1.,0.));
#60815=DIRECTION('ref_axis',(0.,0.,-1.));
#60816=DIRECTION('center_axis',(0.,1.,0.));
#60817=DIRECTION('ref_axis',(0.,0.,1.));
#60818=DIRECTION('center_axis',(0.,-1.,0.));
#60819=DIRECTION('ref_axis',(0.,0.,-1.));
#60820=DIRECTION('',(0.,1.,0.));
#60821=DIRECTION('center_axis',(0.,-1.,0.));
#60822=DIRECTION('ref_axis',(0.,0.,-1.));
#60823=DIRECTION('center_axis',(0.,1.,0.));
#60824=DIRECTION('ref_axis',(0.,0.,1.));
#60825=DIRECTION('center_axis',(0.,1.,0.));
#60826=DIRECTION('ref_axis',(0.,0.,1.));
#60827=DIRECTION('',(0.,-1.,0.));
#60828=DIRECTION('center_axis',(0.,-1.,0.));
#60829=DIRECTION('ref_axis',(0.,0.,-1.));
#60830=DIRECTION('center_axis',(0.,1.,0.));
#60831=DIRECTION('ref_axis',(0.,0.,1.));
#60832=DIRECTION('center_axis',(0.,-1.,0.));
#60833=DIRECTION('ref_axis',(0.,0.,-1.));
#60834=DIRECTION('',(0.,1.,0.));
#60835=DIRECTION('center_axis',(0.,-1.,0.));
#60836=DIRECTION('ref_axis',(0.,0.,-1.));
#60837=DIRECTION('center_axis',(0.,1.,0.));
#60838=DIRECTION('ref_axis',(0.,0.,1.));
#60839=DIRECTION('center_axis',(0.,1.,0.));
#60840=DIRECTION('ref_axis',(0.,0.,1.));
#60841=DIRECTION('',(0.,-1.,0.));
#60842=DIRECTION('center_axis',(0.,-1.,0.));
#60843=DIRECTION('ref_axis',(0.,0.,-1.));
#60844=DIRECTION('center_axis',(0.,1.,0.));
#60845=DIRECTION('ref_axis',(0.,0.,1.));
#60846=DIRECTION('center_axis',(0.,-1.,0.));
#60847=DIRECTION('ref_axis',(0.,0.,-1.));
#60848=DIRECTION('',(0.,1.,0.));
#60849=DIRECTION('center_axis',(0.,-1.,0.));
#60850=DIRECTION('ref_axis',(0.,0.,-1.));
#60851=DIRECTION('center_axis',(0.,1.,0.));
#60852=DIRECTION('ref_axis',(0.,0.,1.));
#60853=DIRECTION('center_axis',(0.,1.,0.));
#60854=DIRECTION('ref_axis',(0.,0.,1.));
#60855=DIRECTION('',(0.,-1.,0.));
#60856=DIRECTION('center_axis',(0.,-1.,0.));
#60857=DIRECTION('ref_axis',(0.,0.,-1.));
#60858=DIRECTION('center_axis',(0.,1.,0.));
#60859=DIRECTION('ref_axis',(0.,0.,1.));
#60860=DIRECTION('center_axis',(0.,-1.,0.));
#60861=DIRECTION('ref_axis',(0.,0.,-1.));
#60862=DIRECTION('',(0.,1.,0.));
#60863=DIRECTION('center_axis',(0.,-1.,0.));
#60864=DIRECTION('ref_axis',(0.,0.,-1.));
#60865=DIRECTION('center_axis',(0.,1.,0.));
#60866=DIRECTION('ref_axis',(0.,0.,1.));
#60867=DIRECTION('center_axis',(0.,1.,0.));
#60868=DIRECTION('ref_axis',(0.,0.,1.));
#60869=DIRECTION('',(0.,-1.,0.));
#60870=DIRECTION('center_axis',(0.,-1.,0.));
#60871=DIRECTION('ref_axis',(0.,0.,-1.));
#60872=DIRECTION('center_axis',(0.,1.,0.));
#60873=DIRECTION('ref_axis',(0.,0.,1.));
#60874=DIRECTION('center_axis',(0.,-1.,0.));
#60875=DIRECTION('ref_axis',(0.,0.,-1.));
#60876=DIRECTION('',(0.,1.,0.));
#60877=DIRECTION('center_axis',(0.,-1.,0.));
#60878=DIRECTION('ref_axis',(0.,0.,-1.));
#60879=DIRECTION('center_axis',(0.,1.,0.));
#60880=DIRECTION('ref_axis',(0.,0.,1.));
#60881=DIRECTION('center_axis',(0.,1.,0.));
#60882=DIRECTION('ref_axis',(0.,0.,1.));
#60883=DIRECTION('',(0.,-1.,0.));
#60884=DIRECTION('center_axis',(0.,-1.,0.));
#60885=DIRECTION('ref_axis',(0.,0.,-1.));
#60886=DIRECTION('center_axis',(0.,1.,0.));
#60887=DIRECTION('ref_axis',(0.,0.,1.));
#60888=DIRECTION('center_axis',(0.,-1.,0.));
#60889=DIRECTION('ref_axis',(0.,0.,-1.));
#60890=DIRECTION('',(0.,1.,0.));
#60891=DIRECTION('center_axis',(0.,-1.,0.));
#60892=DIRECTION('ref_axis',(0.,0.,-1.));
#60893=DIRECTION('center_axis',(0.,1.,0.));
#60894=DIRECTION('ref_axis',(0.,0.,1.));
#60895=DIRECTION('center_axis',(0.,1.,0.));
#60896=DIRECTION('ref_axis',(0.,0.,1.));
#60897=DIRECTION('',(0.,-1.,0.));
#60898=DIRECTION('center_axis',(0.,-1.,0.));
#60899=DIRECTION('ref_axis',(0.,0.,-1.));
#60900=DIRECTION('center_axis',(0.,1.,0.));
#60901=DIRECTION('ref_axis',(0.,0.,1.));
#60902=DIRECTION('center_axis',(0.,-1.,0.));
#60903=DIRECTION('ref_axis',(0.,0.,-1.));
#60904=DIRECTION('',(0.,1.,0.));
#60905=DIRECTION('center_axis',(0.,-1.,0.));
#60906=DIRECTION('ref_axis',(0.,0.,-1.));
#60907=DIRECTION('center_axis',(0.,1.,0.));
#60908=DIRECTION('ref_axis',(0.,0.,1.));
#60909=DIRECTION('center_axis',(0.,1.,0.));
#60910=DIRECTION('ref_axis',(0.,0.,1.));
#60911=DIRECTION('',(0.,-1.,0.));
#60912=DIRECTION('center_axis',(0.,-1.,0.));
#60913=DIRECTION('ref_axis',(0.,0.,-1.));
#60914=DIRECTION('center_axis',(0.,1.,0.));
#60915=DIRECTION('ref_axis',(0.,0.,1.));
#60916=DIRECTION('center_axis',(0.,-1.,0.));
#60917=DIRECTION('ref_axis',(0.,0.,-1.));
#60918=DIRECTION('',(0.,1.,0.));
#60919=DIRECTION('center_axis',(0.,-1.,0.));
#60920=DIRECTION('ref_axis',(0.,0.,-1.));
#60921=DIRECTION('center_axis',(0.,1.,0.));
#60922=DIRECTION('ref_axis',(0.,0.,1.));
#60923=DIRECTION('center_axis',(0.,1.,0.));
#60924=DIRECTION('ref_axis',(0.,0.,1.));
#60925=DIRECTION('',(0.,-1.,0.));
#60926=DIRECTION('center_axis',(0.,-1.,0.));
#60927=DIRECTION('ref_axis',(0.,0.,-1.));
#60928=DIRECTION('center_axis',(0.,1.,0.));
#60929=DIRECTION('ref_axis',(0.,0.,1.));
#60930=DIRECTION('center_axis',(0.,-1.,0.));
#60931=DIRECTION('ref_axis',(0.,0.,-1.));
#60932=DIRECTION('',(0.,1.,0.));
#60933=DIRECTION('center_axis',(0.,-1.,0.));
#60934=DIRECTION('ref_axis',(0.,0.,-1.));
#60935=DIRECTION('center_axis',(0.,1.,0.));
#60936=DIRECTION('ref_axis',(0.,0.,1.));
#60937=DIRECTION('center_axis',(0.,1.,0.));
#60938=DIRECTION('ref_axis',(0.,0.,1.));
#60939=DIRECTION('',(0.,-1.,0.));
#60940=DIRECTION('center_axis',(0.,-1.,0.));
#60941=DIRECTION('ref_axis',(0.,0.,-1.));
#60942=DIRECTION('center_axis',(0.,1.,0.));
#60943=DIRECTION('ref_axis',(0.,0.,1.));
#60944=DIRECTION('center_axis',(0.,-1.,0.));
#60945=DIRECTION('ref_axis',(0.,0.,-1.));
#60946=DIRECTION('',(0.,1.,0.));
#60947=DIRECTION('center_axis',(0.,-1.,0.));
#60948=DIRECTION('ref_axis',(0.,0.,-1.));
#60949=DIRECTION('center_axis',(0.,1.,0.));
#60950=DIRECTION('ref_axis',(0.,0.,1.));
#60951=DIRECTION('center_axis',(0.,1.,0.));
#60952=DIRECTION('ref_axis',(0.,0.,1.));
#60953=DIRECTION('',(0.,-1.,0.));
#60954=DIRECTION('center_axis',(0.,-1.,0.));
#60955=DIRECTION('ref_axis',(0.,0.,-1.));
#60956=DIRECTION('center_axis',(0.,1.,0.));
#60957=DIRECTION('ref_axis',(0.,0.,1.));
#60958=DIRECTION('center_axis',(0.,-1.,0.));
#60959=DIRECTION('ref_axis',(0.,0.,-1.));
#60960=DIRECTION('',(0.,1.,0.));
#60961=DIRECTION('center_axis',(0.,-1.,0.));
#60962=DIRECTION('ref_axis',(0.,0.,-1.));
#60963=DIRECTION('center_axis',(0.,1.,0.));
#60964=DIRECTION('ref_axis',(0.,0.,1.));
#60965=DIRECTION('center_axis',(0.,1.,0.));
#60966=DIRECTION('ref_axis',(0.,0.,1.));
#60967=DIRECTION('',(0.,-1.,0.));
#60968=DIRECTION('center_axis',(0.,-1.,0.));
#60969=DIRECTION('ref_axis',(0.,0.,-1.));
#60970=DIRECTION('center_axis',(0.,1.,0.));
#60971=DIRECTION('ref_axis',(0.,0.,1.));
#60972=DIRECTION('center_axis',(0.,-1.,0.));
#60973=DIRECTION('ref_axis',(0.,0.,-1.));
#60974=DIRECTION('',(0.,1.,0.));
#60975=DIRECTION('center_axis',(0.,-1.,0.));
#60976=DIRECTION('ref_axis',(0.,0.,-1.));
#60977=DIRECTION('center_axis',(0.,1.,0.));
#60978=DIRECTION('ref_axis',(0.,0.,1.));
#60979=DIRECTION('center_axis',(0.,1.,0.));
#60980=DIRECTION('ref_axis',(0.,0.,1.));
#60981=DIRECTION('',(0.,-1.,0.));
#60982=DIRECTION('center_axis',(0.,-1.,0.));
#60983=DIRECTION('ref_axis',(0.,0.,-1.));
#60984=DIRECTION('center_axis',(0.,1.,0.));
#60985=DIRECTION('ref_axis',(0.,0.,1.));
#60986=DIRECTION('center_axis',(0.,-1.,0.));
#60987=DIRECTION('ref_axis',(0.,0.,-1.));
#60988=DIRECTION('',(0.,1.,0.));
#60989=DIRECTION('center_axis',(0.,-1.,0.));
#60990=DIRECTION('ref_axis',(0.,0.,-1.));
#60991=DIRECTION('center_axis',(0.,1.,0.));
#60992=DIRECTION('ref_axis',(0.,0.,1.));
#60993=DIRECTION('center_axis',(0.,1.,0.));
#60994=DIRECTION('ref_axis',(0.,0.,1.));
#60995=DIRECTION('',(0.,-1.,0.));
#60996=DIRECTION('center_axis',(0.,-1.,0.));
#60997=DIRECTION('ref_axis',(0.,0.,-1.));
#60998=DIRECTION('center_axis',(0.,1.,0.));
#60999=DIRECTION('ref_axis',(0.,0.,1.));
#61000=DIRECTION('center_axis',(0.,-1.,0.));
#61001=DIRECTION('ref_axis',(0.,0.,-1.));
#61002=DIRECTION('',(0.,1.,0.));
#61003=DIRECTION('center_axis',(0.,-1.,0.));
#61004=DIRECTION('ref_axis',(0.,0.,-1.));
#61005=DIRECTION('center_axis',(0.,1.,0.));
#61006=DIRECTION('ref_axis',(0.,0.,1.));
#61007=DIRECTION('center_axis',(0.,1.,0.));
#61008=DIRECTION('ref_axis',(0.,0.,1.));
#61009=DIRECTION('',(0.,-1.,0.));
#61010=DIRECTION('center_axis',(0.,-1.,0.));
#61011=DIRECTION('ref_axis',(0.,0.,-1.));
#61012=DIRECTION('center_axis',(0.,1.,0.));
#61013=DIRECTION('ref_axis',(0.,0.,1.));
#61014=DIRECTION('center_axis',(0.,-1.,0.));
#61015=DIRECTION('ref_axis',(0.,0.,-1.));
#61016=DIRECTION('',(0.,1.,0.));
#61017=DIRECTION('center_axis',(0.,-1.,0.));
#61018=DIRECTION('ref_axis',(0.,0.,-1.));
#61019=DIRECTION('center_axis',(0.,1.,0.));
#61020=DIRECTION('ref_axis',(0.,0.,1.));
#61021=DIRECTION('center_axis',(0.,1.,0.));
#61022=DIRECTION('ref_axis',(0.,0.,1.));
#61023=DIRECTION('',(0.,-1.,0.));
#61024=DIRECTION('center_axis',(0.,-1.,0.));
#61025=DIRECTION('ref_axis',(0.,0.,-1.));
#61026=DIRECTION('center_axis',(0.,1.,0.));
#61027=DIRECTION('ref_axis',(0.,0.,1.));
#61028=DIRECTION('center_axis',(0.,-1.,0.));
#61029=DIRECTION('ref_axis',(0.,0.,-1.));
#61030=DIRECTION('',(0.,1.,0.));
#61031=DIRECTION('center_axis',(0.,-1.,0.));
#61032=DIRECTION('ref_axis',(0.,0.,-1.));
#61033=DIRECTION('center_axis',(0.,1.,0.));
#61034=DIRECTION('ref_axis',(0.,0.,1.));
#61035=DIRECTION('center_axis',(0.,1.,0.));
#61036=DIRECTION('ref_axis',(0.,0.,1.));
#61037=DIRECTION('',(0.,-1.,0.));
#61038=DIRECTION('center_axis',(0.,-1.,0.));
#61039=DIRECTION('ref_axis',(0.,0.,-1.));
#61040=DIRECTION('center_axis',(0.,1.,0.));
#61041=DIRECTION('ref_axis',(0.,0.,1.));
#61042=DIRECTION('center_axis',(0.,-1.,0.));
#61043=DIRECTION('ref_axis',(0.,0.,-1.));
#61044=DIRECTION('',(0.,1.,0.));
#61045=DIRECTION('center_axis',(0.,-1.,0.));
#61046=DIRECTION('ref_axis',(0.,0.,-1.));
#61047=DIRECTION('center_axis',(0.,1.,0.));
#61048=DIRECTION('ref_axis',(0.,0.,1.));
#61049=DIRECTION('center_axis',(0.,1.,0.));
#61050=DIRECTION('ref_axis',(0.,0.,1.));
#61051=DIRECTION('',(0.,-1.,0.));
#61052=DIRECTION('center_axis',(0.,-1.,0.));
#61053=DIRECTION('ref_axis',(0.,0.,-1.));
#61054=DIRECTION('center_axis',(0.,1.,0.));
#61055=DIRECTION('ref_axis',(0.,0.,1.));
#61056=DIRECTION('center_axis',(0.,-1.,0.));
#61057=DIRECTION('ref_axis',(0.,0.,-1.));
#61058=DIRECTION('',(0.,1.,0.));
#61059=DIRECTION('center_axis',(0.,-1.,0.));
#61060=DIRECTION('ref_axis',(0.,0.,-1.));
#61061=DIRECTION('center_axis',(0.,1.,0.));
#61062=DIRECTION('ref_axis',(0.,0.,1.));
#61063=DIRECTION('center_axis',(0.,1.,0.));
#61064=DIRECTION('ref_axis',(0.,0.,1.));
#61065=DIRECTION('',(0.,-1.,0.));
#61066=DIRECTION('center_axis',(0.,-1.,0.));
#61067=DIRECTION('ref_axis',(0.,0.,-1.));
#61068=DIRECTION('center_axis',(0.,1.,0.));
#61069=DIRECTION('ref_axis',(0.,0.,1.));
#61070=DIRECTION('center_axis',(0.,-1.,0.));
#61071=DIRECTION('ref_axis',(0.,0.,-1.));
#61072=DIRECTION('',(0.,1.,0.));
#61073=DIRECTION('center_axis',(0.,-1.,0.));
#61074=DIRECTION('ref_axis',(0.,0.,-1.));
#61075=DIRECTION('center_axis',(0.,1.,0.));
#61076=DIRECTION('ref_axis',(0.,0.,1.));
#61077=DIRECTION('center_axis',(0.,1.,0.));
#61078=DIRECTION('ref_axis',(0.,0.,1.));
#61079=DIRECTION('',(0.,-1.,0.));
#61080=DIRECTION('center_axis',(0.,-1.,0.));
#61081=DIRECTION('ref_axis',(0.,0.,-1.));
#61082=DIRECTION('center_axis',(0.,1.,0.));
#61083=DIRECTION('ref_axis',(0.,0.,1.));
#61084=DIRECTION('center_axis',(0.,-1.,0.));
#61085=DIRECTION('ref_axis',(0.,0.,-1.));
#61086=DIRECTION('',(0.,1.,0.));
#61087=DIRECTION('center_axis',(0.,-1.,0.));
#61088=DIRECTION('ref_axis',(0.,0.,-1.));
#61089=DIRECTION('center_axis',(0.,1.,0.));
#61090=DIRECTION('ref_axis',(0.,0.,1.));
#61091=DIRECTION('center_axis',(0.,1.,0.));
#61092=DIRECTION('ref_axis',(0.,0.,1.));
#61093=DIRECTION('',(0.,-1.,0.));
#61094=DIRECTION('center_axis',(0.,-1.,0.));
#61095=DIRECTION('ref_axis',(0.,0.,-1.));
#61096=DIRECTION('center_axis',(0.,1.,0.));
#61097=DIRECTION('ref_axis',(0.,0.,1.));
#61098=DIRECTION('center_axis',(0.,-1.,0.));
#61099=DIRECTION('ref_axis',(0.,0.,-1.));
#61100=DIRECTION('',(0.,1.,0.));
#61101=DIRECTION('center_axis',(0.,-1.,0.));
#61102=DIRECTION('ref_axis',(0.,0.,-1.));
#61103=DIRECTION('center_axis',(0.,1.,0.));
#61104=DIRECTION('ref_axis',(0.,0.,1.));
#61105=DIRECTION('center_axis',(0.,1.,0.));
#61106=DIRECTION('ref_axis',(0.,0.,1.));
#61107=DIRECTION('',(0.,-1.,0.));
#61108=DIRECTION('center_axis',(0.,-1.,0.));
#61109=DIRECTION('ref_axis',(0.,0.,-1.));
#61110=DIRECTION('center_axis',(0.,1.,0.));
#61111=DIRECTION('ref_axis',(0.,0.,1.));
#61112=DIRECTION('center_axis',(0.,-1.,0.));
#61113=DIRECTION('ref_axis',(0.,0.,-1.));
#61114=DIRECTION('',(0.,1.,0.));
#61115=DIRECTION('center_axis',(0.,-1.,0.));
#61116=DIRECTION('ref_axis',(0.,0.,-1.));
#61117=DIRECTION('center_axis',(0.,1.,0.));
#61118=DIRECTION('ref_axis',(0.,0.,1.));
#61119=DIRECTION('center_axis',(0.,1.,0.));
#61120=DIRECTION('ref_axis',(0.,0.,1.));
#61121=DIRECTION('',(0.,-1.,0.));
#61122=DIRECTION('center_axis',(0.,-1.,0.));
#61123=DIRECTION('ref_axis',(0.,0.,-1.));
#61124=DIRECTION('center_axis',(0.,1.,0.));
#61125=DIRECTION('ref_axis',(0.,0.,1.));
#61126=DIRECTION('center_axis',(0.,-1.,0.));
#61127=DIRECTION('ref_axis',(0.,0.,-1.));
#61128=DIRECTION('',(0.,1.,0.));
#61129=DIRECTION('center_axis',(0.,-1.,0.));
#61130=DIRECTION('ref_axis',(0.,0.,-1.));
#61131=DIRECTION('center_axis',(0.,1.,0.));
#61132=DIRECTION('ref_axis',(0.,0.,1.));
#61133=DIRECTION('center_axis',(0.,1.,0.));
#61134=DIRECTION('ref_axis',(0.,0.,1.));
#61135=DIRECTION('',(0.,-1.,0.));
#61136=DIRECTION('center_axis',(0.,-1.,0.));
#61137=DIRECTION('ref_axis',(0.,0.,-1.));
#61138=DIRECTION('center_axis',(0.,1.,0.));
#61139=DIRECTION('ref_axis',(0.,0.,1.));
#61140=DIRECTION('center_axis',(0.,-1.,0.));
#61141=DIRECTION('ref_axis',(0.,0.,-1.));
#61142=DIRECTION('',(0.,1.,0.));
#61143=DIRECTION('center_axis',(0.,-1.,0.));
#61144=DIRECTION('ref_axis',(0.,0.,-1.));
#61145=DIRECTION('center_axis',(0.,1.,0.));
#61146=DIRECTION('ref_axis',(0.,0.,1.));
#61147=DIRECTION('center_axis',(0.,1.,0.));
#61148=DIRECTION('ref_axis',(0.,0.,1.));
#61149=DIRECTION('',(0.,-1.,0.));
#61150=DIRECTION('center_axis',(0.,-1.,0.));
#61151=DIRECTION('ref_axis',(0.,0.,-1.));
#61152=DIRECTION('center_axis',(0.,1.,0.));
#61153=DIRECTION('ref_axis',(0.,0.,1.));
#61154=DIRECTION('center_axis',(0.,-1.,0.));
#61155=DIRECTION('ref_axis',(0.,0.,-1.));
#61156=DIRECTION('',(0.,1.,0.));
#61157=DIRECTION('center_axis',(0.,-1.,0.));
#61158=DIRECTION('ref_axis',(0.,0.,-1.));
#61159=DIRECTION('center_axis',(0.,1.,0.));
#61160=DIRECTION('ref_axis',(0.,0.,1.));
#61161=DIRECTION('center_axis',(0.,1.,0.));
#61162=DIRECTION('ref_axis',(0.,0.,1.));
#61163=DIRECTION('',(0.,-1.,0.));
#61164=DIRECTION('center_axis',(0.,-1.,0.));
#61165=DIRECTION('ref_axis',(0.,0.,-1.));
#61166=DIRECTION('center_axis',(0.,1.,0.));
#61167=DIRECTION('ref_axis',(0.,0.,1.));
#61168=DIRECTION('center_axis',(0.,-1.,0.));
#61169=DIRECTION('ref_axis',(0.,0.,-1.));
#61170=DIRECTION('',(0.,1.,0.));
#61171=DIRECTION('center_axis',(0.,-1.,0.));
#61172=DIRECTION('ref_axis',(0.,0.,-1.));
#61173=DIRECTION('center_axis',(0.,1.,0.));
#61174=DIRECTION('ref_axis',(0.,0.,1.));
#61175=DIRECTION('center_axis',(0.,1.,0.));
#61176=DIRECTION('ref_axis',(0.,0.,1.));
#61177=DIRECTION('',(0.,-1.,0.));
#61178=DIRECTION('center_axis',(0.,-1.,0.));
#61179=DIRECTION('ref_axis',(0.,0.,-1.));
#61180=DIRECTION('center_axis',(0.,1.,0.));
#61181=DIRECTION('ref_axis',(0.,0.,1.));
#61182=DIRECTION('center_axis',(0.,-1.,0.));
#61183=DIRECTION('ref_axis',(0.,0.,-1.));
#61184=DIRECTION('',(0.,1.,0.));
#61185=DIRECTION('center_axis',(0.,-1.,0.));
#61186=DIRECTION('ref_axis',(0.,0.,-1.));
#61187=DIRECTION('center_axis',(0.,1.,0.));
#61188=DIRECTION('ref_axis',(0.,0.,1.));
#61189=DIRECTION('center_axis',(0.,1.,0.));
#61190=DIRECTION('ref_axis',(0.,0.,1.));
#61191=DIRECTION('',(0.,-1.,0.));
#61192=DIRECTION('center_axis',(0.,-1.,0.));
#61193=DIRECTION('ref_axis',(0.,0.,-1.));
#61194=DIRECTION('center_axis',(0.,1.,0.));
#61195=DIRECTION('ref_axis',(0.,0.,1.));
#61196=DIRECTION('center_axis',(0.,-1.,0.));
#61197=DIRECTION('ref_axis',(0.,0.,-1.));
#61198=DIRECTION('',(0.,1.,0.));
#61199=DIRECTION('center_axis',(0.,-1.,0.));
#61200=DIRECTION('ref_axis',(0.,0.,-1.));
#61201=DIRECTION('center_axis',(0.,1.,0.));
#61202=DIRECTION('ref_axis',(0.,0.,1.));
#61203=DIRECTION('center_axis',(0.,1.,0.));
#61204=DIRECTION('ref_axis',(0.,0.,1.));
#61205=DIRECTION('',(0.,-1.,0.));
#61206=DIRECTION('center_axis',(0.,-1.,0.));
#61207=DIRECTION('ref_axis',(0.,0.,-1.));
#61208=DIRECTION('center_axis',(0.,1.,0.));
#61209=DIRECTION('ref_axis',(0.,0.,1.));
#61210=DIRECTION('center_axis',(0.,-1.,0.));
#61211=DIRECTION('ref_axis',(0.,0.,-1.));
#61212=DIRECTION('',(0.,1.,0.));
#61213=DIRECTION('center_axis',(0.,-1.,0.));
#61214=DIRECTION('ref_axis',(0.,0.,-1.));
#61215=DIRECTION('center_axis',(0.,1.,0.));
#61216=DIRECTION('ref_axis',(0.,0.,1.));
#61217=DIRECTION('center_axis',(0.,1.,0.));
#61218=DIRECTION('ref_axis',(0.,0.,1.));
#61219=DIRECTION('',(0.,-1.,0.));
#61220=DIRECTION('center_axis',(0.,-1.,0.));
#61221=DIRECTION('ref_axis',(0.,0.,-1.));
#61222=DIRECTION('center_axis',(0.,1.,0.));
#61223=DIRECTION('ref_axis',(0.,0.,1.));
#61224=DIRECTION('center_axis',(0.,-1.,0.));
#61225=DIRECTION('ref_axis',(0.,0.,-1.));
#61226=DIRECTION('',(0.,1.,0.));
#61227=DIRECTION('center_axis',(0.,-1.,0.));
#61228=DIRECTION('ref_axis',(0.,0.,-1.));
#61229=DIRECTION('center_axis',(0.,1.,0.));
#61230=DIRECTION('ref_axis',(0.,0.,1.));
#61231=DIRECTION('center_axis',(0.,1.,0.));
#61232=DIRECTION('ref_axis',(0.,0.,1.));
#61233=DIRECTION('',(0.,-1.,0.));
#61234=DIRECTION('center_axis',(0.,-1.,0.));
#61235=DIRECTION('ref_axis',(0.,0.,-1.));
#61236=DIRECTION('center_axis',(0.,1.,0.));
#61237=DIRECTION('ref_axis',(0.,0.,1.));
#61238=DIRECTION('center_axis',(0.,-1.,0.));
#61239=DIRECTION('ref_axis',(0.,0.,-1.));
#61240=DIRECTION('',(0.,1.,0.));
#61241=DIRECTION('center_axis',(0.,-1.,0.));
#61242=DIRECTION('ref_axis',(0.,0.,-1.));
#61243=DIRECTION('center_axis',(0.,1.,0.));
#61244=DIRECTION('ref_axis',(0.,0.,1.));
#61245=DIRECTION('center_axis',(0.,1.,0.));
#61246=DIRECTION('ref_axis',(0.,0.,1.));
#61247=DIRECTION('',(0.,-1.,0.));
#61248=DIRECTION('center_axis',(0.,-1.,0.));
#61249=DIRECTION('ref_axis',(0.,0.,-1.));
#61250=DIRECTION('center_axis',(0.,1.,0.));
#61251=DIRECTION('ref_axis',(0.,0.,1.));
#61252=DIRECTION('center_axis',(0.,-1.,0.));
#61253=DIRECTION('ref_axis',(0.,0.,-1.));
#61254=DIRECTION('',(0.,1.,0.));
#61255=DIRECTION('center_axis',(0.,-1.,0.));
#61256=DIRECTION('ref_axis',(0.,0.,-1.));
#61257=DIRECTION('center_axis',(0.,1.,0.));
#61258=DIRECTION('ref_axis',(0.,0.,1.));
#61259=DIRECTION('center_axis',(0.,1.,0.));
#61260=DIRECTION('ref_axis',(0.,0.,1.));
#61261=DIRECTION('',(0.,-1.,0.));
#61262=DIRECTION('center_axis',(0.,-1.,0.));
#61263=DIRECTION('ref_axis',(0.,0.,-1.));
#61264=DIRECTION('center_axis',(0.,1.,0.));
#61265=DIRECTION('ref_axis',(0.,0.,1.));
#61266=DIRECTION('center_axis',(0.,-1.,0.));
#61267=DIRECTION('ref_axis',(0.,0.,-1.));
#61268=DIRECTION('',(0.,1.,0.));
#61269=DIRECTION('center_axis',(0.,-1.,0.));
#61270=DIRECTION('ref_axis',(0.,0.,-1.));
#61271=DIRECTION('center_axis',(0.,1.,0.));
#61272=DIRECTION('ref_axis',(0.,0.,1.));
#61273=DIRECTION('center_axis',(0.,1.,0.));
#61274=DIRECTION('ref_axis',(0.,0.,1.));
#61275=DIRECTION('',(0.,-1.,0.));
#61276=DIRECTION('center_axis',(0.,-1.,0.));
#61277=DIRECTION('ref_axis',(0.,0.,-1.));
#61278=DIRECTION('center_axis',(0.,1.,0.));
#61279=DIRECTION('ref_axis',(0.,0.,1.));
#61280=DIRECTION('center_axis',(0.,-1.,0.));
#61281=DIRECTION('ref_axis',(0.,0.,-1.));
#61282=DIRECTION('',(0.,1.,0.));
#61283=DIRECTION('center_axis',(0.,-1.,0.));
#61284=DIRECTION('ref_axis',(0.,0.,-1.));
#61285=DIRECTION('center_axis',(0.,1.,0.));
#61286=DIRECTION('ref_axis',(0.,0.,1.));
#61287=DIRECTION('center_axis',(0.,1.,0.));
#61288=DIRECTION('ref_axis',(0.,0.,1.));
#61289=DIRECTION('',(0.,-1.,0.));
#61290=DIRECTION('center_axis',(0.,-1.,0.));
#61291=DIRECTION('ref_axis',(0.,0.,-1.));
#61292=DIRECTION('center_axis',(0.,1.,0.));
#61293=DIRECTION('ref_axis',(0.,0.,1.));
#61294=DIRECTION('center_axis',(0.,-1.,0.));
#61295=DIRECTION('ref_axis',(0.,0.,-1.));
#61296=DIRECTION('',(0.,1.,0.));
#61297=DIRECTION('center_axis',(0.,-1.,0.));
#61298=DIRECTION('ref_axis',(0.,0.,-1.));
#61299=DIRECTION('center_axis',(0.,1.,0.));
#61300=DIRECTION('ref_axis',(0.,0.,1.));
#61301=DIRECTION('center_axis',(0.,1.,0.));
#61302=DIRECTION('ref_axis',(0.,0.,1.));
#61303=DIRECTION('',(0.,-1.,0.));
#61304=DIRECTION('center_axis',(0.,-1.,0.));
#61305=DIRECTION('ref_axis',(0.,0.,-1.));
#61306=DIRECTION('center_axis',(0.,1.,0.));
#61307=DIRECTION('ref_axis',(0.,0.,1.));
#61308=DIRECTION('center_axis',(0.,-1.,0.));
#61309=DIRECTION('ref_axis',(0.,0.,-1.));
#61310=DIRECTION('',(0.,1.,0.));
#61311=DIRECTION('center_axis',(0.,-1.,0.));
#61312=DIRECTION('ref_axis',(0.,0.,-1.));
#61313=DIRECTION('center_axis',(0.,1.,0.));
#61314=DIRECTION('ref_axis',(0.,0.,1.));
#61315=DIRECTION('center_axis',(0.,1.,0.));
#61316=DIRECTION('ref_axis',(0.,0.,1.));
#61317=DIRECTION('',(0.,-1.,0.));
#61318=DIRECTION('center_axis',(0.,-1.,0.));
#61319=DIRECTION('ref_axis',(0.,0.,-1.));
#61320=DIRECTION('center_axis',(0.,1.,0.));
#61321=DIRECTION('ref_axis',(0.,0.,1.));
#61322=DIRECTION('center_axis',(0.,-1.,0.));
#61323=DIRECTION('ref_axis',(0.,0.,-1.));
#61324=DIRECTION('',(0.,1.,0.));
#61325=DIRECTION('center_axis',(0.,-1.,0.));
#61326=DIRECTION('ref_axis',(0.,0.,-1.));
#61327=DIRECTION('center_axis',(0.,1.,0.));
#61328=DIRECTION('ref_axis',(0.,0.,1.));
#61329=DIRECTION('center_axis',(0.,1.,0.));
#61330=DIRECTION('ref_axis',(0.,0.,1.));
#61331=DIRECTION('',(0.,-1.,0.));
#61332=DIRECTION('center_axis',(0.,-1.,0.));
#61333=DIRECTION('ref_axis',(0.,0.,-1.));
#61334=DIRECTION('center_axis',(0.,1.,0.));
#61335=DIRECTION('ref_axis',(0.,0.,1.));
#61336=DIRECTION('center_axis',(0.,-1.,0.));
#61337=DIRECTION('ref_axis',(0.,0.,-1.));
#61338=DIRECTION('',(0.,1.,0.));
#61339=DIRECTION('center_axis',(0.,-1.,0.));
#61340=DIRECTION('ref_axis',(0.,0.,-1.));
#61341=DIRECTION('center_axis',(0.,1.,0.));
#61342=DIRECTION('ref_axis',(0.,0.,1.));
#61343=DIRECTION('center_axis',(0.,1.,0.));
#61344=DIRECTION('ref_axis',(0.,0.,1.));
#61345=DIRECTION('',(0.,-1.,0.));
#61346=DIRECTION('center_axis',(0.,-1.,0.));
#61347=DIRECTION('ref_axis',(0.,0.,-1.));
#61348=DIRECTION('center_axis',(0.,1.,0.));
#61349=DIRECTION('ref_axis',(0.,0.,1.));
#61350=DIRECTION('center_axis',(0.,-1.,0.));
#61351=DIRECTION('ref_axis',(0.,0.,-1.));
#61352=DIRECTION('',(0.,1.,0.));
#61353=DIRECTION('center_axis',(0.,-1.,0.));
#61354=DIRECTION('ref_axis',(0.,0.,-1.));
#61355=DIRECTION('center_axis',(0.,1.,0.));
#61356=DIRECTION('ref_axis',(0.,0.,1.));
#61357=DIRECTION('center_axis',(0.,1.,0.));
#61358=DIRECTION('ref_axis',(0.,0.,1.));
#61359=DIRECTION('',(0.,-1.,0.));
#61360=DIRECTION('center_axis',(0.,-1.,0.));
#61361=DIRECTION('ref_axis',(0.,0.,-1.));
#61362=DIRECTION('center_axis',(0.,1.,0.));
#61363=DIRECTION('ref_axis',(0.,0.,1.));
#61364=DIRECTION('center_axis',(0.,-1.,0.));
#61365=DIRECTION('ref_axis',(0.,0.,-1.));
#61366=DIRECTION('',(0.,1.,0.));
#61367=DIRECTION('center_axis',(0.,-1.,0.));
#61368=DIRECTION('ref_axis',(0.,0.,-1.));
#61369=DIRECTION('center_axis',(0.,1.,0.));
#61370=DIRECTION('ref_axis',(0.,0.,1.));
#61371=DIRECTION('center_axis',(0.,1.,0.));
#61372=DIRECTION('ref_axis',(0.,0.,1.));
#61373=DIRECTION('',(0.,-1.,0.));
#61374=DIRECTION('center_axis',(0.,-1.,0.));
#61375=DIRECTION('ref_axis',(0.,0.,-1.));
#61376=DIRECTION('center_axis',(0.,1.,0.));
#61377=DIRECTION('ref_axis',(0.,0.,1.));
#61378=DIRECTION('center_axis',(0.,-1.,0.));
#61379=DIRECTION('ref_axis',(0.,0.,-1.));
#61380=DIRECTION('',(0.,1.,0.));
#61381=DIRECTION('center_axis',(0.,-1.,0.));
#61382=DIRECTION('ref_axis',(0.,0.,-1.));
#61383=DIRECTION('center_axis',(0.,1.,0.));
#61384=DIRECTION('ref_axis',(0.,0.,1.));
#61385=DIRECTION('center_axis',(0.,1.,0.));
#61386=DIRECTION('ref_axis',(0.,0.,1.));
#61387=DIRECTION('',(0.,-1.,0.));
#61388=DIRECTION('center_axis',(0.,-1.,0.));
#61389=DIRECTION('ref_axis',(0.,0.,-1.));
#61390=DIRECTION('center_axis',(0.,1.,0.));
#61391=DIRECTION('ref_axis',(0.,0.,1.));
#61392=DIRECTION('center_axis',(0.,-1.,0.));
#61393=DIRECTION('ref_axis',(0.,0.,-1.));
#61394=DIRECTION('',(0.,1.,0.));
#61395=DIRECTION('center_axis',(0.,-1.,0.));
#61396=DIRECTION('ref_axis',(0.,0.,-1.));
#61397=DIRECTION('center_axis',(0.,1.,0.));
#61398=DIRECTION('ref_axis',(0.,0.,1.));
#61399=DIRECTION('center_axis',(0.,1.,0.));
#61400=DIRECTION('ref_axis',(0.,0.,1.));
#61401=DIRECTION('',(0.,-1.,0.));
#61402=DIRECTION('center_axis',(0.,-1.,0.));
#61403=DIRECTION('ref_axis',(0.,0.,-1.));
#61404=DIRECTION('center_axis',(0.,1.,0.));
#61405=DIRECTION('ref_axis',(0.,0.,1.));
#61406=DIRECTION('center_axis',(0.,-1.,0.));
#61407=DIRECTION('ref_axis',(0.,0.,-1.));
#61408=DIRECTION('',(0.,1.,0.));
#61409=DIRECTION('center_axis',(0.,-1.,0.));
#61410=DIRECTION('ref_axis',(0.,0.,-1.));
#61411=DIRECTION('center_axis',(0.,1.,0.));
#61412=DIRECTION('ref_axis',(0.,0.,1.));
#61413=DIRECTION('center_axis',(0.,1.,0.));
#61414=DIRECTION('ref_axis',(0.,0.,1.));
#61415=DIRECTION('',(0.,-1.,0.));
#61416=DIRECTION('center_axis',(0.,-1.,0.));
#61417=DIRECTION('ref_axis',(0.,0.,-1.));
#61418=DIRECTION('center_axis',(0.,1.,0.));
#61419=DIRECTION('ref_axis',(0.,0.,1.));
#61420=DIRECTION('center_axis',(0.,-1.,0.));
#61421=DIRECTION('ref_axis',(0.,0.,-1.));
#61422=DIRECTION('',(0.,1.,0.));
#61423=DIRECTION('center_axis',(0.,-1.,0.));
#61424=DIRECTION('ref_axis',(0.,0.,-1.));
#61425=DIRECTION('center_axis',(0.,1.,0.));
#61426=DIRECTION('ref_axis',(0.,0.,1.));
#61427=DIRECTION('center_axis',(0.,1.,0.));
#61428=DIRECTION('ref_axis',(0.,0.,1.));
#61429=DIRECTION('',(0.,-1.,0.));
#61430=DIRECTION('center_axis',(0.,-1.,0.));
#61431=DIRECTION('ref_axis',(0.,0.,-1.));
#61432=DIRECTION('center_axis',(0.,1.,0.));
#61433=DIRECTION('ref_axis',(0.,0.,1.));
#61434=DIRECTION('center_axis',(0.,-1.,0.));
#61435=DIRECTION('ref_axis',(0.,0.,-1.));
#61436=DIRECTION('',(0.,1.,0.));
#61437=DIRECTION('center_axis',(0.,-1.,0.));
#61438=DIRECTION('ref_axis',(0.,0.,-1.));
#61439=DIRECTION('center_axis',(0.,1.,0.));
#61440=DIRECTION('ref_axis',(0.,0.,1.));
#61441=DIRECTION('center_axis',(0.,1.,0.));
#61442=DIRECTION('ref_axis',(0.,0.,1.));
#61443=DIRECTION('',(0.,-1.,0.));
#61444=DIRECTION('center_axis',(0.,-1.,0.));
#61445=DIRECTION('ref_axis',(0.,0.,-1.));
#61446=DIRECTION('center_axis',(0.,1.,0.));
#61447=DIRECTION('ref_axis',(0.,0.,1.));
#61448=DIRECTION('center_axis',(0.,-1.,0.));
#61449=DIRECTION('ref_axis',(0.,0.,-1.));
#61450=DIRECTION('',(0.,1.,0.));
#61451=DIRECTION('center_axis',(0.,-1.,0.));
#61452=DIRECTION('ref_axis',(0.,0.,-1.));
#61453=DIRECTION('center_axis',(0.,1.,0.));
#61454=DIRECTION('ref_axis',(0.,0.,1.));
#61455=DIRECTION('center_axis',(0.,1.,0.));
#61456=DIRECTION('ref_axis',(0.,0.,1.));
#61457=DIRECTION('',(0.,-1.,0.));
#61458=DIRECTION('center_axis',(0.,-1.,0.));
#61459=DIRECTION('ref_axis',(0.,0.,-1.));
#61460=DIRECTION('center_axis',(0.,1.,0.));
#61461=DIRECTION('ref_axis',(0.,0.,1.));
#61462=DIRECTION('center_axis',(0.,-1.,0.));
#61463=DIRECTION('ref_axis',(0.,0.,-1.));
#61464=DIRECTION('',(0.,1.,0.));
#61465=DIRECTION('center_axis',(0.,-1.,0.));
#61466=DIRECTION('ref_axis',(0.,0.,-1.));
#61467=DIRECTION('center_axis',(0.,1.,0.));
#61468=DIRECTION('ref_axis',(0.,0.,1.));
#61469=DIRECTION('center_axis',(0.,1.,0.));
#61470=DIRECTION('ref_axis',(0.,0.,1.));
#61471=DIRECTION('',(0.,-1.,0.));
#61472=DIRECTION('center_axis',(0.,-1.,0.));
#61473=DIRECTION('ref_axis',(0.,0.,-1.));
#61474=DIRECTION('center_axis',(0.,1.,0.));
#61475=DIRECTION('ref_axis',(0.,0.,1.));
#61476=DIRECTION('center_axis',(0.,-1.,0.));
#61477=DIRECTION('ref_axis',(0.,0.,-1.));
#61478=DIRECTION('',(0.,1.,0.));
#61479=DIRECTION('center_axis',(0.,-1.,0.));
#61480=DIRECTION('ref_axis',(0.,0.,-1.));
#61481=DIRECTION('center_axis',(0.,1.,0.));
#61482=DIRECTION('ref_axis',(0.,0.,1.));
#61483=DIRECTION('center_axis',(0.,1.,0.));
#61484=DIRECTION('ref_axis',(0.,0.,1.));
#61485=DIRECTION('',(0.,-1.,0.));
#61486=DIRECTION('center_axis',(0.,-1.,0.));
#61487=DIRECTION('ref_axis',(0.,0.,-1.));
#61488=DIRECTION('center_axis',(0.,1.,0.));
#61489=DIRECTION('ref_axis',(0.,0.,1.));
#61490=DIRECTION('center_axis',(0.,-1.,0.));
#61491=DIRECTION('ref_axis',(0.,0.,-1.));
#61492=DIRECTION('',(0.,1.,0.));
#61493=DIRECTION('center_axis',(0.,-1.,0.));
#61494=DIRECTION('ref_axis',(0.,0.,-1.));
#61495=DIRECTION('center_axis',(0.,1.,0.));
#61496=DIRECTION('ref_axis',(0.,0.,1.));
#61497=DIRECTION('center_axis',(0.,1.,0.));
#61498=DIRECTION('ref_axis',(0.,0.,1.));
#61499=DIRECTION('',(0.,-1.,0.));
#61500=DIRECTION('center_axis',(0.,-1.,0.));
#61501=DIRECTION('ref_axis',(0.,0.,-1.));
#61502=DIRECTION('center_axis',(0.,1.,0.));
#61503=DIRECTION('ref_axis',(0.,0.,1.));
#61504=DIRECTION('center_axis',(0.,-1.,0.));
#61505=DIRECTION('ref_axis',(0.,0.,-1.));
#61506=DIRECTION('',(0.,1.,0.));
#61507=DIRECTION('center_axis',(0.,-1.,0.));
#61508=DIRECTION('ref_axis',(0.,0.,-1.));
#61509=DIRECTION('center_axis',(0.,1.,0.));
#61510=DIRECTION('ref_axis',(0.,0.,1.));
#61511=DIRECTION('center_axis',(0.,1.,0.));
#61512=DIRECTION('ref_axis',(0.,0.,1.));
#61513=DIRECTION('',(0.,-1.,0.));
#61514=DIRECTION('center_axis',(0.,-1.,0.));
#61515=DIRECTION('ref_axis',(0.,0.,-1.));
#61516=DIRECTION('center_axis',(0.,1.,0.));
#61517=DIRECTION('ref_axis',(0.,0.,1.));
#61518=DIRECTION('center_axis',(0.,-1.,0.));
#61519=DIRECTION('ref_axis',(0.,0.,-1.));
#61520=DIRECTION('',(0.,1.,0.));
#61521=DIRECTION('center_axis',(0.,-1.,0.));
#61522=DIRECTION('ref_axis',(0.,0.,-1.));
#61523=DIRECTION('center_axis',(0.,1.,0.));
#61524=DIRECTION('ref_axis',(0.,0.,1.));
#61525=DIRECTION('center_axis',(0.,1.,0.));
#61526=DIRECTION('ref_axis',(0.,0.,1.));
#61527=DIRECTION('',(0.,-1.,0.));
#61528=DIRECTION('center_axis',(0.,-1.,0.));
#61529=DIRECTION('ref_axis',(0.,0.,-1.));
#61530=DIRECTION('center_axis',(0.,1.,0.));
#61531=DIRECTION('ref_axis',(0.,0.,1.));
#61532=DIRECTION('center_axis',(0.,-1.,0.));
#61533=DIRECTION('ref_axis',(0.,0.,-1.));
#61534=DIRECTION('',(0.,1.,0.));
#61535=DIRECTION('center_axis',(0.,-1.,0.));
#61536=DIRECTION('ref_axis',(0.,0.,-1.));
#61537=DIRECTION('center_axis',(0.,1.,0.));
#61538=DIRECTION('ref_axis',(0.,0.,1.));
#61539=DIRECTION('center_axis',(0.,1.,0.));
#61540=DIRECTION('ref_axis',(0.,0.,1.));
#61541=DIRECTION('',(0.,-1.,0.));
#61542=DIRECTION('center_axis',(0.,-1.,0.));
#61543=DIRECTION('ref_axis',(0.,0.,-1.));
#61544=DIRECTION('center_axis',(0.,1.,0.));
#61545=DIRECTION('ref_axis',(0.,0.,1.));
#61546=DIRECTION('center_axis',(0.,-1.,0.));
#61547=DIRECTION('ref_axis',(0.,0.,-1.));
#61548=DIRECTION('',(0.,1.,0.));
#61549=DIRECTION('center_axis',(0.,-1.,0.));
#61550=DIRECTION('ref_axis',(0.,0.,-1.));
#61551=DIRECTION('center_axis',(0.,1.,0.));
#61552=DIRECTION('ref_axis',(0.,0.,1.));
#61553=DIRECTION('center_axis',(0.,1.,0.));
#61554=DIRECTION('ref_axis',(0.,0.,1.));
#61555=DIRECTION('',(0.,-1.,0.));
#61556=DIRECTION('center_axis',(0.,-1.,0.));
#61557=DIRECTION('ref_axis',(0.,0.,-1.));
#61558=DIRECTION('center_axis',(0.,1.,0.));
#61559=DIRECTION('ref_axis',(0.,0.,1.));
#61560=DIRECTION('center_axis',(0.,-1.,0.));
#61561=DIRECTION('ref_axis',(0.,0.,-1.));
#61562=DIRECTION('',(0.,1.,0.));
#61563=DIRECTION('center_axis',(0.,-1.,0.));
#61564=DIRECTION('ref_axis',(0.,0.,-1.));
#61565=DIRECTION('center_axis',(0.,1.,0.));
#61566=DIRECTION('ref_axis',(0.,0.,1.));
#61567=DIRECTION('center_axis',(0.,1.,0.));
#61568=DIRECTION('ref_axis',(0.,0.,1.));
#61569=DIRECTION('',(0.,-1.,0.));
#61570=DIRECTION('center_axis',(0.,-1.,0.));
#61571=DIRECTION('ref_axis',(0.,0.,-1.));
#61572=DIRECTION('center_axis',(0.,1.,0.));
#61573=DIRECTION('ref_axis',(0.,0.,1.));
#61574=DIRECTION('center_axis',(0.,-1.,0.));
#61575=DIRECTION('ref_axis',(0.,0.,-1.));
#61576=DIRECTION('',(0.,1.,0.));
#61577=DIRECTION('center_axis',(0.,-1.,0.));
#61578=DIRECTION('ref_axis',(0.,0.,-1.));
#61579=DIRECTION('center_axis',(0.,1.,0.));
#61580=DIRECTION('ref_axis',(0.,0.,1.));
#61581=DIRECTION('center_axis',(0.,1.,0.));
#61582=DIRECTION('ref_axis',(0.,0.,1.));
#61583=DIRECTION('',(0.,-1.,0.));
#61584=DIRECTION('center_axis',(0.,-1.,0.));
#61585=DIRECTION('ref_axis',(0.,0.,-1.));
#61586=DIRECTION('center_axis',(0.,1.,0.));
#61587=DIRECTION('ref_axis',(0.,0.,1.));
#61588=DIRECTION('center_axis',(0.,-1.,0.));
#61589=DIRECTION('ref_axis',(0.,0.,-1.));
#61590=DIRECTION('',(0.,1.,0.));
#61591=DIRECTION('center_axis',(0.,-1.,0.));
#61592=DIRECTION('ref_axis',(0.,0.,-1.));
#61593=DIRECTION('center_axis',(0.,1.,0.));
#61594=DIRECTION('ref_axis',(0.,0.,1.));
#61595=DIRECTION('center_axis',(0.,1.,0.));
#61596=DIRECTION('ref_axis',(0.,0.,1.));
#61597=DIRECTION('',(0.,-1.,0.));
#61598=DIRECTION('center_axis',(0.,-1.,0.));
#61599=DIRECTION('ref_axis',(0.,0.,-1.));
#61600=DIRECTION('center_axis',(0.,1.,0.));
#61601=DIRECTION('ref_axis',(0.,0.,1.));
#61602=DIRECTION('center_axis',(0.,-1.,0.));
#61603=DIRECTION('ref_axis',(0.,0.,-1.));
#61604=DIRECTION('',(0.,1.,0.));
#61605=DIRECTION('center_axis',(0.,-1.,0.));
#61606=DIRECTION('ref_axis',(0.,0.,-1.));
#61607=DIRECTION('center_axis',(0.,1.,0.));
#61608=DIRECTION('ref_axis',(0.,0.,1.));
#61609=DIRECTION('center_axis',(0.,1.,0.));
#61610=DIRECTION('ref_axis',(0.,0.,1.));
#61611=DIRECTION('',(0.,-1.,0.));
#61612=DIRECTION('center_axis',(0.,-1.,0.));
#61613=DIRECTION('ref_axis',(0.,0.,-1.));
#61614=DIRECTION('center_axis',(0.,1.,0.));
#61615=DIRECTION('ref_axis',(0.,0.,1.));
#61616=DIRECTION('center_axis',(0.,-1.,0.));
#61617=DIRECTION('ref_axis',(0.,0.,-1.));
#61618=DIRECTION('',(0.,1.,0.));
#61619=DIRECTION('center_axis',(0.,-1.,0.));
#61620=DIRECTION('ref_axis',(0.,0.,-1.));
#61621=DIRECTION('center_axis',(0.,1.,0.));
#61622=DIRECTION('ref_axis',(0.,0.,1.));
#61623=DIRECTION('center_axis',(0.,1.,0.));
#61624=DIRECTION('ref_axis',(0.,0.,1.));
#61625=DIRECTION('',(0.,-1.,0.));
#61626=DIRECTION('center_axis',(0.,-1.,0.));
#61627=DIRECTION('ref_axis',(0.,0.,-1.));
#61628=DIRECTION('center_axis',(0.,1.,0.));
#61629=DIRECTION('ref_axis',(0.,0.,1.));
#61630=DIRECTION('center_axis',(0.,-1.,0.));
#61631=DIRECTION('ref_axis',(0.,0.,-1.));
#61632=DIRECTION('',(0.,1.,0.));
#61633=DIRECTION('center_axis',(0.,-1.,0.));
#61634=DIRECTION('ref_axis',(0.,0.,-1.));
#61635=DIRECTION('center_axis',(0.,1.,0.));
#61636=DIRECTION('ref_axis',(0.,0.,1.));
#61637=DIRECTION('center_axis',(0.,1.,0.));
#61638=DIRECTION('ref_axis',(0.,0.,1.));
#61639=DIRECTION('',(0.,-1.,0.));
#61640=DIRECTION('center_axis',(0.,-1.,0.));
#61641=DIRECTION('ref_axis',(0.,0.,-1.));
#61642=DIRECTION('center_axis',(0.,1.,0.));
#61643=DIRECTION('ref_axis',(0.,0.,1.));
#61644=DIRECTION('center_axis',(0.,-1.,0.));
#61645=DIRECTION('ref_axis',(0.,0.,-1.));
#61646=DIRECTION('',(0.,1.,0.));
#61647=DIRECTION('center_axis',(0.,-1.,0.));
#61648=DIRECTION('ref_axis',(0.,0.,-1.));
#61649=DIRECTION('center_axis',(0.,1.,0.));
#61650=DIRECTION('ref_axis',(0.,0.,1.));
#61651=DIRECTION('center_axis',(0.,1.,0.));
#61652=DIRECTION('ref_axis',(0.,0.,1.));
#61653=DIRECTION('',(0.,-1.,0.));
#61654=DIRECTION('center_axis',(0.,-1.,0.));
#61655=DIRECTION('ref_axis',(0.,0.,-1.));
#61656=DIRECTION('center_axis',(0.,1.,0.));
#61657=DIRECTION('ref_axis',(0.,0.,1.));
#61658=DIRECTION('center_axis',(0.,-1.,0.));
#61659=DIRECTION('ref_axis',(0.,0.,-1.));
#61660=DIRECTION('',(0.,1.,0.));
#61661=DIRECTION('center_axis',(0.,-1.,0.));
#61662=DIRECTION('ref_axis',(0.,0.,-1.));
#61663=DIRECTION('center_axis',(0.,1.,0.));
#61664=DIRECTION('ref_axis',(0.,0.,1.));
#61665=DIRECTION('center_axis',(0.,1.,0.));
#61666=DIRECTION('ref_axis',(0.,0.,1.));
#61667=DIRECTION('',(0.,-1.,0.));
#61668=DIRECTION('center_axis',(0.,-1.,0.));
#61669=DIRECTION('ref_axis',(0.,0.,-1.));
#61670=DIRECTION('center_axis',(0.,1.,0.));
#61671=DIRECTION('ref_axis',(0.,0.,1.));
#61672=DIRECTION('center_axis',(0.,-1.,0.));
#61673=DIRECTION('ref_axis',(0.,0.,-1.));
#61674=DIRECTION('',(0.,1.,0.));
#61675=DIRECTION('center_axis',(0.,-1.,0.));
#61676=DIRECTION('ref_axis',(0.,0.,-1.));
#61677=DIRECTION('center_axis',(0.,1.,0.));
#61678=DIRECTION('ref_axis',(0.,0.,1.));
#61679=DIRECTION('center_axis',(0.,1.,0.));
#61680=DIRECTION('ref_axis',(0.,0.,1.));
#61681=DIRECTION('',(0.,-1.,0.));
#61682=DIRECTION('center_axis',(0.,-1.,0.));
#61683=DIRECTION('ref_axis',(0.,0.,-1.));
#61684=DIRECTION('center_axis',(0.,1.,0.));
#61685=DIRECTION('ref_axis',(0.,0.,1.));
#61686=DIRECTION('center_axis',(0.,-1.,0.));
#61687=DIRECTION('ref_axis',(0.,0.,-1.));
#61688=DIRECTION('',(0.,1.,0.));
#61689=DIRECTION('center_axis',(0.,-1.,0.));
#61690=DIRECTION('ref_axis',(0.,0.,-1.));
#61691=DIRECTION('center_axis',(0.,1.,0.));
#61692=DIRECTION('ref_axis',(0.,0.,1.));
#61693=DIRECTION('center_axis',(0.,1.,0.));
#61694=DIRECTION('ref_axis',(0.,0.,1.));
#61695=DIRECTION('',(0.,-1.,0.));
#61696=DIRECTION('center_axis',(0.,-1.,0.));
#61697=DIRECTION('ref_axis',(0.,0.,-1.));
#61698=DIRECTION('center_axis',(0.,1.,0.));
#61699=DIRECTION('ref_axis',(0.,0.,1.));
#61700=DIRECTION('center_axis',(0.,-1.,0.));
#61701=DIRECTION('ref_axis',(0.,0.,-1.));
#61702=DIRECTION('',(0.,1.,0.));
#61703=DIRECTION('center_axis',(0.,-1.,0.));
#61704=DIRECTION('ref_axis',(0.,0.,-1.));
#61705=DIRECTION('center_axis',(0.,1.,0.));
#61706=DIRECTION('ref_axis',(0.,0.,1.));
#61707=DIRECTION('center_axis',(0.,1.,0.));
#61708=DIRECTION('ref_axis',(0.,0.,1.));
#61709=DIRECTION('',(0.,-1.,0.));
#61710=DIRECTION('center_axis',(0.,-1.,0.));
#61711=DIRECTION('ref_axis',(0.,0.,-1.));
#61712=DIRECTION('center_axis',(0.,1.,0.));
#61713=DIRECTION('ref_axis',(0.,0.,1.));
#61714=DIRECTION('center_axis',(0.,-1.,0.));
#61715=DIRECTION('ref_axis',(0.,0.,-1.));
#61716=DIRECTION('',(0.,1.,0.));
#61717=DIRECTION('center_axis',(0.,-1.,0.));
#61718=DIRECTION('ref_axis',(0.,0.,-1.));
#61719=DIRECTION('center_axis',(0.,1.,0.));
#61720=DIRECTION('ref_axis',(0.,0.,1.));
#61721=DIRECTION('center_axis',(0.,1.,0.));
#61722=DIRECTION('ref_axis',(0.,0.,1.));
#61723=DIRECTION('',(0.,-1.,0.));
#61724=DIRECTION('center_axis',(0.,-1.,0.));
#61725=DIRECTION('ref_axis',(0.,0.,-1.));
#61726=DIRECTION('center_axis',(0.,1.,0.));
#61727=DIRECTION('ref_axis',(0.,0.,1.));
#61728=DIRECTION('center_axis',(0.,-1.,0.));
#61729=DIRECTION('ref_axis',(0.,0.,-1.));
#61730=DIRECTION('',(0.,1.,0.));
#61731=DIRECTION('center_axis',(0.,-1.,0.));
#61732=DIRECTION('ref_axis',(0.,0.,-1.));
#61733=DIRECTION('center_axis',(0.,1.,0.));
#61734=DIRECTION('ref_axis',(0.,0.,1.));
#61735=DIRECTION('center_axis',(0.,1.,0.));
#61736=DIRECTION('ref_axis',(0.,0.,1.));
#61737=DIRECTION('',(0.,-1.,0.));
#61738=DIRECTION('center_axis',(0.,-1.,0.));
#61739=DIRECTION('ref_axis',(0.,0.,-1.));
#61740=DIRECTION('center_axis',(0.,1.,0.));
#61741=DIRECTION('ref_axis',(0.,0.,1.));
#61742=DIRECTION('center_axis',(0.,-1.,0.));
#61743=DIRECTION('ref_axis',(0.,0.,-1.));
#61744=DIRECTION('',(0.,1.,0.));
#61745=DIRECTION('center_axis',(0.,-1.,0.));
#61746=DIRECTION('ref_axis',(0.,0.,-1.));
#61747=DIRECTION('center_axis',(0.,1.,0.));
#61748=DIRECTION('ref_axis',(0.,0.,1.));
#61749=DIRECTION('center_axis',(0.,1.,0.));
#61750=DIRECTION('ref_axis',(0.,0.,1.));
#61751=DIRECTION('',(0.,-1.,0.));
#61752=DIRECTION('center_axis',(0.,-1.,0.));
#61753=DIRECTION('ref_axis',(0.,0.,-1.));
#61754=DIRECTION('center_axis',(0.,1.,0.));
#61755=DIRECTION('ref_axis',(0.,0.,1.));
#61756=DIRECTION('center_axis',(0.,-1.,0.));
#61757=DIRECTION('ref_axis',(0.,0.,-1.));
#61758=DIRECTION('',(0.,1.,0.));
#61759=DIRECTION('center_axis',(0.,-1.,0.));
#61760=DIRECTION('ref_axis',(0.,0.,-1.));
#61761=DIRECTION('center_axis',(0.,1.,0.));
#61762=DIRECTION('ref_axis',(0.,0.,1.));
#61763=DIRECTION('center_axis',(0.,1.,0.));
#61764=DIRECTION('ref_axis',(0.,0.,1.));
#61765=DIRECTION('',(0.,-1.,0.));
#61766=DIRECTION('center_axis',(0.,-1.,0.));
#61767=DIRECTION('ref_axis',(0.,0.,-1.));
#61768=DIRECTION('center_axis',(0.,1.,0.));
#61769=DIRECTION('ref_axis',(0.,0.,1.));
#61770=DIRECTION('center_axis',(0.,-1.,0.));
#61771=DIRECTION('ref_axis',(0.,0.,-1.));
#61772=DIRECTION('',(0.,1.,0.));
#61773=DIRECTION('center_axis',(0.,-1.,0.));
#61774=DIRECTION('ref_axis',(0.,0.,-1.));
#61775=DIRECTION('center_axis',(0.,1.,0.));
#61776=DIRECTION('ref_axis',(0.,0.,1.));
#61777=DIRECTION('center_axis',(0.,1.,0.));
#61778=DIRECTION('ref_axis',(0.,0.,1.));
#61779=DIRECTION('',(0.,-1.,0.));
#61780=DIRECTION('center_axis',(0.,-1.,0.));
#61781=DIRECTION('ref_axis',(0.,0.,-1.));
#61782=DIRECTION('center_axis',(0.,1.,0.));
#61783=DIRECTION('ref_axis',(0.,0.,1.));
#61784=DIRECTION('center_axis',(0.,-1.,0.));
#61785=DIRECTION('ref_axis',(0.,0.,-1.));
#61786=DIRECTION('',(0.,1.,0.));
#61787=DIRECTION('center_axis',(0.,-1.,0.));
#61788=DIRECTION('ref_axis',(0.,0.,-1.));
#61789=DIRECTION('center_axis',(0.,1.,0.));
#61790=DIRECTION('ref_axis',(0.,0.,1.));
#61791=DIRECTION('center_axis',(0.,1.,0.));
#61792=DIRECTION('ref_axis',(0.,0.,1.));
#61793=DIRECTION('',(0.,-1.,0.));
#61794=DIRECTION('center_axis',(0.,-1.,0.));
#61795=DIRECTION('ref_axis',(0.,0.,-1.));
#61796=DIRECTION('center_axis',(0.,1.,0.));
#61797=DIRECTION('ref_axis',(0.,0.,1.));
#61798=DIRECTION('center_axis',(0.,-1.,0.));
#61799=DIRECTION('ref_axis',(0.,0.,-1.));
#61800=DIRECTION('',(0.,1.,0.));
#61801=DIRECTION('center_axis',(0.,-1.,0.));
#61802=DIRECTION('ref_axis',(0.,0.,-1.));
#61803=DIRECTION('center_axis',(0.,1.,0.));
#61804=DIRECTION('ref_axis',(0.,0.,1.));
#61805=DIRECTION('center_axis',(0.,1.,0.));
#61806=DIRECTION('ref_axis',(0.,0.,1.));
#61807=DIRECTION('',(0.,-1.,0.));
#61808=DIRECTION('center_axis',(0.,-1.,0.));
#61809=DIRECTION('ref_axis',(0.,0.,-1.));
#61810=DIRECTION('center_axis',(0.,1.,0.));
#61811=DIRECTION('ref_axis',(0.,0.,1.));
#61812=DIRECTION('center_axis',(0.,-1.,0.));
#61813=DIRECTION('ref_axis',(0.,0.,-1.));
#61814=DIRECTION('',(0.,1.,0.));
#61815=DIRECTION('center_axis',(0.,-1.,0.));
#61816=DIRECTION('ref_axis',(0.,0.,-1.));
#61817=DIRECTION('center_axis',(0.,1.,0.));
#61818=DIRECTION('ref_axis',(0.,0.,1.));
#61819=DIRECTION('center_axis',(0.,1.,0.));
#61820=DIRECTION('ref_axis',(0.,0.,1.));
#61821=DIRECTION('',(0.,-1.,0.));
#61822=DIRECTION('center_axis',(0.,-1.,0.));
#61823=DIRECTION('ref_axis',(0.,0.,-1.));
#61824=DIRECTION('center_axis',(0.,1.,0.));
#61825=DIRECTION('ref_axis',(0.,0.,1.));
#61826=DIRECTION('center_axis',(0.,-1.,0.));
#61827=DIRECTION('ref_axis',(0.,0.,-1.));
#61828=DIRECTION('',(0.,1.,0.));
#61829=DIRECTION('center_axis',(0.,-1.,0.));
#61830=DIRECTION('ref_axis',(0.,0.,-1.));
#61831=DIRECTION('center_axis',(0.,1.,0.));
#61832=DIRECTION('ref_axis',(0.,0.,1.));
#61833=DIRECTION('center_axis',(0.,1.,0.));
#61834=DIRECTION('ref_axis',(0.,0.,1.));
#61835=DIRECTION('',(0.,-1.,0.));
#61836=DIRECTION('center_axis',(0.,-1.,0.));
#61837=DIRECTION('ref_axis',(0.,0.,-1.));
#61838=DIRECTION('center_axis',(0.,1.,0.));
#61839=DIRECTION('ref_axis',(0.,0.,1.));
#61840=DIRECTION('center_axis',(0.,-1.,0.));
#61841=DIRECTION('ref_axis',(0.,0.,-1.));
#61842=DIRECTION('',(0.,1.,0.));
#61843=DIRECTION('center_axis',(0.,-1.,0.));
#61844=DIRECTION('ref_axis',(0.,0.,-1.));
#61845=DIRECTION('center_axis',(0.,1.,0.));
#61846=DIRECTION('ref_axis',(0.,0.,1.));
#61847=DIRECTION('center_axis',(0.,1.,0.));
#61848=DIRECTION('ref_axis',(0.,0.,1.));
#61849=DIRECTION('',(0.,-1.,0.));
#61850=DIRECTION('center_axis',(0.,-1.,0.));
#61851=DIRECTION('ref_axis',(0.,0.,-1.));
#61852=DIRECTION('center_axis',(0.,1.,0.));
#61853=DIRECTION('ref_axis',(0.,0.,1.));
#61854=DIRECTION('center_axis',(0.,-1.,0.));
#61855=DIRECTION('ref_axis',(0.,0.,-1.));
#61856=DIRECTION('',(0.,1.,0.));
#61857=DIRECTION('center_axis',(0.,-1.,0.));
#61858=DIRECTION('ref_axis',(0.,0.,-1.));
#61859=DIRECTION('center_axis',(0.,1.,0.));
#61860=DIRECTION('ref_axis',(0.,0.,1.));
#61861=DIRECTION('center_axis',(0.,1.,0.));
#61862=DIRECTION('ref_axis',(0.,0.,1.));
#61863=DIRECTION('',(0.,-1.,0.));
#61864=DIRECTION('center_axis',(0.,-1.,0.));
#61865=DIRECTION('ref_axis',(0.,0.,-1.));
#61866=DIRECTION('center_axis',(0.,1.,0.));
#61867=DIRECTION('ref_axis',(0.,0.,1.));
#61868=DIRECTION('center_axis',(0.,-1.,0.));
#61869=DIRECTION('ref_axis',(0.,0.,-1.));
#61870=DIRECTION('',(0.,1.,0.));
#61871=DIRECTION('center_axis',(0.,-1.,0.));
#61872=DIRECTION('ref_axis',(0.,0.,-1.));
#61873=DIRECTION('center_axis',(0.,1.,0.));
#61874=DIRECTION('ref_axis',(0.,0.,1.));
#61875=DIRECTION('center_axis',(0.,1.,0.));
#61876=DIRECTION('ref_axis',(0.,0.,1.));
#61877=DIRECTION('',(0.,-1.,0.));
#61878=DIRECTION('center_axis',(0.,-1.,0.));
#61879=DIRECTION('ref_axis',(0.,0.,-1.));
#61880=DIRECTION('center_axis',(0.,1.,0.));
#61881=DIRECTION('ref_axis',(0.,0.,1.));
#61882=DIRECTION('center_axis',(0.,-1.,0.));
#61883=DIRECTION('ref_axis',(0.,0.,-1.));
#61884=DIRECTION('',(0.,1.,0.));
#61885=DIRECTION('center_axis',(0.,-1.,0.));
#61886=DIRECTION('ref_axis',(0.,0.,-1.));
#61887=DIRECTION('center_axis',(0.,1.,0.));
#61888=DIRECTION('ref_axis',(0.,0.,1.));
#61889=DIRECTION('center_axis',(0.,1.,0.));
#61890=DIRECTION('ref_axis',(0.,0.,1.));
#61891=DIRECTION('',(0.,-1.,0.));
#61892=DIRECTION('center_axis',(0.,-1.,0.));
#61893=DIRECTION('ref_axis',(0.,0.,-1.));
#61894=DIRECTION('center_axis',(0.,1.,0.));
#61895=DIRECTION('ref_axis',(0.,0.,1.));
#61896=DIRECTION('center_axis',(0.,-1.,0.));
#61897=DIRECTION('ref_axis',(0.,0.,-1.));
#61898=DIRECTION('',(0.,1.,0.));
#61899=DIRECTION('center_axis',(0.,-1.,0.));
#61900=DIRECTION('ref_axis',(0.,0.,-1.));
#61901=DIRECTION('center_axis',(0.,1.,0.));
#61902=DIRECTION('ref_axis',(0.,0.,1.));
#61903=DIRECTION('center_axis',(0.,1.,0.));
#61904=DIRECTION('ref_axis',(0.,0.,1.));
#61905=DIRECTION('',(0.,-1.,0.));
#61906=DIRECTION('center_axis',(0.,-1.,0.));
#61907=DIRECTION('ref_axis',(0.,0.,-1.));
#61908=DIRECTION('center_axis',(0.,1.,0.));
#61909=DIRECTION('ref_axis',(0.,0.,1.));
#61910=DIRECTION('center_axis',(0.,-1.,0.));
#61911=DIRECTION('ref_axis',(0.,0.,-1.));
#61912=DIRECTION('',(0.,1.,0.));
#61913=DIRECTION('center_axis',(0.,-1.,0.));
#61914=DIRECTION('ref_axis',(0.,0.,-1.));
#61915=DIRECTION('center_axis',(0.,1.,0.));
#61916=DIRECTION('ref_axis',(0.,0.,1.));
#61917=DIRECTION('center_axis',(0.,1.,0.));
#61918=DIRECTION('ref_axis',(0.,0.,1.));
#61919=DIRECTION('',(0.,-1.,0.));
#61920=DIRECTION('center_axis',(0.,-1.,0.));
#61921=DIRECTION('ref_axis',(0.,0.,-1.));
#61922=DIRECTION('center_axis',(0.,1.,0.));
#61923=DIRECTION('ref_axis',(0.,0.,1.));
#61924=DIRECTION('center_axis',(0.,-1.,0.));
#61925=DIRECTION('ref_axis',(0.,0.,-1.));
#61926=DIRECTION('',(0.,1.,0.));
#61927=DIRECTION('center_axis',(0.,-1.,0.));
#61928=DIRECTION('ref_axis',(0.,0.,-1.));
#61929=DIRECTION('center_axis',(0.,1.,0.));
#61930=DIRECTION('ref_axis',(0.,0.,1.));
#61931=DIRECTION('center_axis',(0.,1.,0.));
#61932=DIRECTION('ref_axis',(0.,0.,1.));
#61933=DIRECTION('',(0.,-1.,0.));
#61934=DIRECTION('center_axis',(0.,-1.,0.));
#61935=DIRECTION('ref_axis',(0.,0.,-1.));
#61936=DIRECTION('center_axis',(0.,1.,0.));
#61937=DIRECTION('ref_axis',(0.,0.,1.));
#61938=DIRECTION('center_axis',(0.,-1.,0.));
#61939=DIRECTION('ref_axis',(0.,0.,-1.));
#61940=DIRECTION('',(0.,1.,0.));
#61941=DIRECTION('center_axis',(0.,-1.,0.));
#61942=DIRECTION('ref_axis',(0.,0.,-1.));
#61943=DIRECTION('center_axis',(0.,1.,0.));
#61944=DIRECTION('ref_axis',(0.,0.,1.));
#61945=DIRECTION('center_axis',(0.,1.,0.));
#61946=DIRECTION('ref_axis',(0.,0.,1.));
#61947=DIRECTION('',(0.,-1.,0.));
#61948=DIRECTION('center_axis',(0.,-1.,0.));
#61949=DIRECTION('ref_axis',(0.,0.,-1.));
#61950=DIRECTION('center_axis',(0.,1.,0.));
#61951=DIRECTION('ref_axis',(0.,0.,1.));
#61952=DIRECTION('center_axis',(0.,-1.,0.));
#61953=DIRECTION('ref_axis',(0.,0.,-1.));
#61954=DIRECTION('',(0.,1.,0.));
#61955=DIRECTION('center_axis',(0.,-1.,0.));
#61956=DIRECTION('ref_axis',(0.,0.,-1.));
#61957=DIRECTION('center_axis',(0.,1.,0.));
#61958=DIRECTION('ref_axis',(0.,0.,1.));
#61959=DIRECTION('center_axis',(0.,1.,0.));
#61960=DIRECTION('ref_axis',(0.,0.,1.));
#61961=DIRECTION('',(0.,-1.,0.));
#61962=DIRECTION('center_axis',(0.,-1.,0.));
#61963=DIRECTION('ref_axis',(0.,0.,-1.));
#61964=DIRECTION('center_axis',(0.,1.,0.));
#61965=DIRECTION('ref_axis',(0.,0.,1.));
#61966=DIRECTION('center_axis',(0.,-1.,0.));
#61967=DIRECTION('ref_axis',(0.,0.,-1.));
#61968=DIRECTION('',(0.,1.,0.));
#61969=DIRECTION('center_axis',(0.,-1.,0.));
#61970=DIRECTION('ref_axis',(0.,0.,-1.));
#61971=DIRECTION('center_axis',(0.,1.,0.));
#61972=DIRECTION('ref_axis',(0.,0.,1.));
#61973=DIRECTION('center_axis',(0.,1.,0.));
#61974=DIRECTION('ref_axis',(0.,0.,1.));
#61975=DIRECTION('',(0.,-1.,0.));
#61976=DIRECTION('center_axis',(0.,-1.,0.));
#61977=DIRECTION('ref_axis',(0.,0.,-1.));
#61978=DIRECTION('center_axis',(0.,1.,0.));
#61979=DIRECTION('ref_axis',(0.,0.,1.));
#61980=DIRECTION('center_axis',(0.,-1.,0.));
#61981=DIRECTION('ref_axis',(0.,0.,-1.));
#61982=DIRECTION('',(0.,1.,0.));
#61983=DIRECTION('center_axis',(0.,-1.,0.));
#61984=DIRECTION('ref_axis',(0.,0.,-1.));
#61985=DIRECTION('center_axis',(0.,1.,0.));
#61986=DIRECTION('ref_axis',(0.,0.,1.));
#61987=DIRECTION('center_axis',(0.,1.,0.));
#61988=DIRECTION('ref_axis',(0.,0.,1.));
#61989=DIRECTION('',(0.,-1.,0.));
#61990=DIRECTION('center_axis',(0.,-1.,0.));
#61991=DIRECTION('ref_axis',(0.,0.,-1.));
#61992=DIRECTION('center_axis',(0.,1.,0.));
#61993=DIRECTION('ref_axis',(0.,0.,1.));
#61994=DIRECTION('center_axis',(0.,-1.,0.));
#61995=DIRECTION('ref_axis',(0.,0.,-1.));
#61996=DIRECTION('',(0.,1.,0.));
#61997=DIRECTION('center_axis',(0.,-1.,0.));
#61998=DIRECTION('ref_axis',(0.,0.,-1.));
#61999=DIRECTION('center_axis',(0.,1.,0.));
#62000=DIRECTION('ref_axis',(0.,0.,1.));
#62001=DIRECTION('center_axis',(0.,1.,0.));
#62002=DIRECTION('ref_axis',(0.,0.,1.));
#62003=DIRECTION('',(0.,-1.,0.));
#62004=DIRECTION('center_axis',(0.,-1.,0.));
#62005=DIRECTION('ref_axis',(0.,0.,-1.));
#62006=DIRECTION('center_axis',(0.,1.,0.));
#62007=DIRECTION('ref_axis',(0.,0.,1.));
#62008=DIRECTION('center_axis',(0.,-1.,0.));
#62009=DIRECTION('ref_axis',(0.,0.,-1.));
#62010=DIRECTION('',(0.,1.,0.));
#62011=DIRECTION('center_axis',(0.,-1.,0.));
#62012=DIRECTION('ref_axis',(0.,0.,-1.));
#62013=DIRECTION('center_axis',(0.,1.,0.));
#62014=DIRECTION('ref_axis',(0.,0.,1.));
#62015=DIRECTION('center_axis',(0.,1.,0.));
#62016=DIRECTION('ref_axis',(0.,0.,1.));
#62017=DIRECTION('',(0.,-1.,0.));
#62018=DIRECTION('center_axis',(0.,-1.,0.));
#62019=DIRECTION('ref_axis',(0.,0.,-1.));
#62020=DIRECTION('center_axis',(0.,1.,0.));
#62021=DIRECTION('ref_axis',(0.,0.,1.));
#62022=DIRECTION('center_axis',(0.,-1.,0.));
#62023=DIRECTION('ref_axis',(0.,0.,-1.));
#62024=DIRECTION('',(0.,1.,0.));
#62025=DIRECTION('center_axis',(0.,-1.,0.));
#62026=DIRECTION('ref_axis',(0.,0.,-1.));
#62027=DIRECTION('center_axis',(0.,1.,0.));
#62028=DIRECTION('ref_axis',(0.,0.,1.));
#62029=DIRECTION('center_axis',(0.,1.,0.));
#62030=DIRECTION('ref_axis',(0.,0.,1.));
#62031=DIRECTION('',(0.,-1.,0.));
#62032=DIRECTION('center_axis',(0.,-1.,0.));
#62033=DIRECTION('ref_axis',(0.,0.,-1.));
#62034=DIRECTION('center_axis',(0.,1.,0.));
#62035=DIRECTION('ref_axis',(0.,0.,1.));
#62036=DIRECTION('center_axis',(0.,-1.,0.));
#62037=DIRECTION('ref_axis',(0.,0.,-1.));
#62038=DIRECTION('',(0.,1.,0.));
#62039=DIRECTION('center_axis',(0.,-1.,0.));
#62040=DIRECTION('ref_axis',(0.,0.,-1.));
#62041=DIRECTION('center_axis',(0.,1.,0.));
#62042=DIRECTION('ref_axis',(0.,0.,1.));
#62043=DIRECTION('center_axis',(0.,1.,0.));
#62044=DIRECTION('ref_axis',(0.,0.,1.));
#62045=DIRECTION('',(0.,-1.,0.));
#62046=DIRECTION('center_axis',(0.,-1.,0.));
#62047=DIRECTION('ref_axis',(0.,0.,-1.));
#62048=DIRECTION('center_axis',(0.,1.,0.));
#62049=DIRECTION('ref_axis',(0.,0.,1.));
#62050=DIRECTION('center_axis',(0.,-1.,0.));
#62051=DIRECTION('ref_axis',(0.,0.,-1.));
#62052=DIRECTION('',(0.,1.,0.));
#62053=DIRECTION('center_axis',(0.,-1.,0.));
#62054=DIRECTION('ref_axis',(0.,0.,-1.));
#62055=DIRECTION('center_axis',(0.,1.,0.));
#62056=DIRECTION('ref_axis',(0.,0.,1.));
#62057=DIRECTION('center_axis',(0.,1.,0.));
#62058=DIRECTION('ref_axis',(0.,0.,1.));
#62059=DIRECTION('',(0.,-1.,0.));
#62060=DIRECTION('center_axis',(0.,-1.,0.));
#62061=DIRECTION('ref_axis',(0.,0.,-1.));
#62062=DIRECTION('center_axis',(0.,1.,0.));
#62063=DIRECTION('ref_axis',(0.,0.,1.));
#62064=DIRECTION('center_axis',(0.,-1.,0.));
#62065=DIRECTION('ref_axis',(0.,0.,-1.));
#62066=DIRECTION('',(0.,1.,0.));
#62067=DIRECTION('center_axis',(0.,-1.,0.));
#62068=DIRECTION('ref_axis',(0.,0.,-1.));
#62069=DIRECTION('center_axis',(0.,1.,0.));
#62070=DIRECTION('ref_axis',(0.,0.,1.));
#62071=DIRECTION('center_axis',(0.,1.,0.));
#62072=DIRECTION('ref_axis',(0.,0.,1.));
#62073=DIRECTION('',(0.,-1.,0.));
#62074=DIRECTION('center_axis',(0.,-1.,0.));
#62075=DIRECTION('ref_axis',(0.,0.,-1.));
#62076=DIRECTION('center_axis',(0.,1.,0.));
#62077=DIRECTION('ref_axis',(0.,0.,1.));
#62078=DIRECTION('center_axis',(0.,-1.,0.));
#62079=DIRECTION('ref_axis',(0.,0.,-1.));
#62080=DIRECTION('',(0.,1.,0.));
#62081=DIRECTION('center_axis',(0.,-1.,0.));
#62082=DIRECTION('ref_axis',(0.,0.,-1.));
#62083=DIRECTION('center_axis',(0.,1.,0.));
#62084=DIRECTION('ref_axis',(0.,0.,1.));
#62085=DIRECTION('center_axis',(0.,1.,0.));
#62086=DIRECTION('ref_axis',(0.,0.,1.));
#62087=DIRECTION('',(0.,-1.,0.));
#62088=DIRECTION('center_axis',(0.,-1.,0.));
#62089=DIRECTION('ref_axis',(0.,0.,-1.));
#62090=DIRECTION('center_axis',(0.,1.,0.));
#62091=DIRECTION('ref_axis',(0.,0.,1.));
#62092=DIRECTION('center_axis',(0.,-1.,0.));
#62093=DIRECTION('ref_axis',(0.,0.,-1.));
#62094=DIRECTION('',(0.,1.,0.));
#62095=DIRECTION('center_axis',(0.,-1.,0.));
#62096=DIRECTION('ref_axis',(0.,0.,-1.));
#62097=DIRECTION('center_axis',(0.,1.,0.));
#62098=DIRECTION('ref_axis',(0.,0.,1.));
#62099=DIRECTION('center_axis',(0.,1.,0.));
#62100=DIRECTION('ref_axis',(0.,0.,1.));
#62101=DIRECTION('',(0.,-1.,0.));
#62102=DIRECTION('center_axis',(0.,-1.,0.));
#62103=DIRECTION('ref_axis',(0.,0.,-1.));
#62104=DIRECTION('center_axis',(0.,1.,0.));
#62105=DIRECTION('ref_axis',(0.,0.,1.));
#62106=DIRECTION('center_axis',(0.,-1.,0.));
#62107=DIRECTION('ref_axis',(0.,0.,-1.));
#62108=DIRECTION('',(0.,1.,0.));
#62109=DIRECTION('center_axis',(0.,-1.,0.));
#62110=DIRECTION('ref_axis',(0.,0.,-1.));
#62111=DIRECTION('center_axis',(0.,1.,0.));
#62112=DIRECTION('ref_axis',(0.,0.,1.));
#62113=DIRECTION('center_axis',(0.,1.,0.));
#62114=DIRECTION('ref_axis',(0.,0.,1.));
#62115=DIRECTION('',(0.,-1.,0.));
#62116=DIRECTION('center_axis',(0.,-1.,0.));
#62117=DIRECTION('ref_axis',(0.,0.,-1.));
#62118=DIRECTION('center_axis',(0.,1.,0.));
#62119=DIRECTION('ref_axis',(0.,0.,1.));
#62120=DIRECTION('center_axis',(0.,-1.,0.));
#62121=DIRECTION('ref_axis',(0.,0.,-1.));
#62122=DIRECTION('',(0.,1.,0.));
#62123=DIRECTION('center_axis',(0.,-1.,0.));
#62124=DIRECTION('ref_axis',(0.,0.,-1.));
#62125=DIRECTION('center_axis',(0.,1.,0.));
#62126=DIRECTION('ref_axis',(0.,0.,1.));
#62127=DIRECTION('center_axis',(0.,1.,0.));
#62128=DIRECTION('ref_axis',(0.,0.,1.));
#62129=DIRECTION('',(0.,-1.,0.));
#62130=DIRECTION('center_axis',(0.,-1.,0.));
#62131=DIRECTION('ref_axis',(0.,0.,-1.));
#62132=DIRECTION('center_axis',(0.,1.,0.));
#62133=DIRECTION('ref_axis',(0.,0.,1.));
#62134=DIRECTION('center_axis',(0.,-1.,0.));
#62135=DIRECTION('ref_axis',(0.,0.,-1.));
#62136=DIRECTION('',(0.,1.,0.));
#62137=DIRECTION('center_axis',(0.,-1.,0.));
#62138=DIRECTION('ref_axis',(0.,0.,-1.));
#62139=DIRECTION('center_axis',(0.,1.,0.));
#62140=DIRECTION('ref_axis',(0.,0.,1.));
#62141=DIRECTION('center_axis',(0.,1.,0.));
#62142=DIRECTION('ref_axis',(0.,0.,1.));
#62143=DIRECTION('',(0.,-1.,0.));
#62144=DIRECTION('center_axis',(0.,-1.,0.));
#62145=DIRECTION('ref_axis',(0.,0.,-1.));
#62146=DIRECTION('center_axis',(0.,1.,0.));
#62147=DIRECTION('ref_axis',(0.,0.,1.));
#62148=DIRECTION('center_axis',(0.,-1.,0.));
#62149=DIRECTION('ref_axis',(0.,0.,-1.));
#62150=DIRECTION('',(0.,1.,0.));
#62151=DIRECTION('center_axis',(0.,-1.,0.));
#62152=DIRECTION('ref_axis',(0.,0.,-1.));
#62153=DIRECTION('center_axis',(0.,1.,0.));
#62154=DIRECTION('ref_axis',(0.,0.,1.));
#62155=DIRECTION('center_axis',(0.,1.,0.));
#62156=DIRECTION('ref_axis',(0.,0.,1.));
#62157=DIRECTION('',(0.,-1.,0.));
#62158=DIRECTION('center_axis',(0.,-1.,0.));
#62159=DIRECTION('ref_axis',(0.,0.,-1.));
#62160=DIRECTION('center_axis',(0.,1.,0.));
#62161=DIRECTION('ref_axis',(0.,0.,1.));
#62162=DIRECTION('center_axis',(0.,-1.,0.));
#62163=DIRECTION('ref_axis',(0.,0.,-1.));
#62164=DIRECTION('',(0.,1.,0.));
#62165=DIRECTION('center_axis',(0.,-1.,0.));
#62166=DIRECTION('ref_axis',(0.,0.,-1.));
#62167=DIRECTION('center_axis',(0.,1.,0.));
#62168=DIRECTION('ref_axis',(0.,0.,1.));
#62169=DIRECTION('center_axis',(0.,1.,0.));
#62170=DIRECTION('ref_axis',(0.,0.,1.));
#62171=DIRECTION('',(0.,-1.,0.));
#62172=DIRECTION('center_axis',(0.,-1.,0.));
#62173=DIRECTION('ref_axis',(0.,0.,-1.));
#62174=DIRECTION('center_axis',(0.,1.,0.));
#62175=DIRECTION('ref_axis',(0.,0.,1.));
#62176=DIRECTION('center_axis',(0.,-1.,0.));
#62177=DIRECTION('ref_axis',(0.,0.,-1.));
#62178=DIRECTION('',(0.,1.,0.));
#62179=DIRECTION('center_axis',(0.,-1.,0.));
#62180=DIRECTION('ref_axis',(0.,0.,-1.));
#62181=DIRECTION('center_axis',(0.,1.,0.));
#62182=DIRECTION('ref_axis',(0.,0.,1.));
#62183=DIRECTION('center_axis',(0.,1.,0.));
#62184=DIRECTION('ref_axis',(0.,0.,1.));
#62185=DIRECTION('',(0.,-1.,0.));
#62186=DIRECTION('center_axis',(0.,-1.,0.));
#62187=DIRECTION('ref_axis',(0.,0.,-1.));
#62188=DIRECTION('center_axis',(0.,1.,0.));
#62189=DIRECTION('ref_axis',(0.,0.,1.));
#62190=DIRECTION('center_axis',(0.,-1.,0.));
#62191=DIRECTION('ref_axis',(0.,0.,-1.));
#62192=DIRECTION('',(0.,1.,0.));
#62193=DIRECTION('center_axis',(0.,-1.,0.));
#62194=DIRECTION('ref_axis',(0.,0.,-1.));
#62195=DIRECTION('center_axis',(0.,1.,0.));
#62196=DIRECTION('ref_axis',(0.,0.,1.));
#62197=DIRECTION('center_axis',(0.,1.,0.));
#62198=DIRECTION('ref_axis',(0.,0.,1.));
#62199=DIRECTION('',(0.,-1.,0.));
#62200=DIRECTION('center_axis',(0.,-1.,0.));
#62201=DIRECTION('ref_axis',(0.,0.,-1.));
#62202=DIRECTION('center_axis',(0.,1.,0.));
#62203=DIRECTION('ref_axis',(0.,0.,1.));
#62204=DIRECTION('center_axis',(0.,-1.,0.));
#62205=DIRECTION('ref_axis',(0.,0.,-1.));
#62206=DIRECTION('',(0.,1.,0.));
#62207=DIRECTION('center_axis',(0.,-1.,0.));
#62208=DIRECTION('ref_axis',(0.,0.,-1.));
#62209=DIRECTION('center_axis',(0.,1.,0.));
#62210=DIRECTION('ref_axis',(0.,0.,1.));
#62211=DIRECTION('center_axis',(0.,1.,0.));
#62212=DIRECTION('ref_axis',(0.,0.,1.));
#62213=DIRECTION('',(0.,-1.,0.));
#62214=DIRECTION('center_axis',(0.,-1.,0.));
#62215=DIRECTION('ref_axis',(0.,0.,-1.));
#62216=DIRECTION('center_axis',(0.,1.,0.));
#62217=DIRECTION('ref_axis',(0.,0.,1.));
#62218=DIRECTION('center_axis',(0.,-1.,0.));
#62219=DIRECTION('ref_axis',(0.,0.,-1.));
#62220=DIRECTION('',(0.,1.,0.));
#62221=DIRECTION('center_axis',(0.,-1.,0.));
#62222=DIRECTION('ref_axis',(0.,0.,-1.));
#62223=DIRECTION('center_axis',(0.,1.,0.));
#62224=DIRECTION('ref_axis',(0.,0.,1.));
#62225=DIRECTION('center_axis',(0.,1.,0.));
#62226=DIRECTION('ref_axis',(0.,0.,1.));
#62227=DIRECTION('',(0.,-1.,0.));
#62228=DIRECTION('center_axis',(0.,-1.,0.));
#62229=DIRECTION('ref_axis',(0.,0.,-1.));
#62230=DIRECTION('center_axis',(0.,1.,0.));
#62231=DIRECTION('ref_axis',(0.,0.,1.));
#62232=DIRECTION('center_axis',(0.,-1.,0.));
#62233=DIRECTION('ref_axis',(0.,0.,-1.));
#62234=DIRECTION('',(0.,1.,0.));
#62235=DIRECTION('center_axis',(0.,-1.,0.));
#62236=DIRECTION('ref_axis',(0.,0.,-1.));
#62237=DIRECTION('center_axis',(0.,1.,0.));
#62238=DIRECTION('ref_axis',(0.,0.,1.));
#62239=DIRECTION('center_axis',(0.,1.,0.));
#62240=DIRECTION('ref_axis',(0.,0.,1.));
#62241=DIRECTION('',(0.,-1.,0.));
#62242=DIRECTION('center_axis',(0.,-1.,0.));
#62243=DIRECTION('ref_axis',(0.,0.,-1.));
#62244=DIRECTION('center_axis',(0.,1.,0.));
#62245=DIRECTION('ref_axis',(0.,0.,1.));
#62246=DIRECTION('center_axis',(0.,-1.,0.));
#62247=DIRECTION('ref_axis',(0.,0.,-1.));
#62248=DIRECTION('',(0.,1.,0.));
#62249=DIRECTION('center_axis',(0.,-1.,0.));
#62250=DIRECTION('ref_axis',(0.,0.,-1.));
#62251=DIRECTION('center_axis',(0.,1.,0.));
#62252=DIRECTION('ref_axis',(0.,0.,1.));
#62253=DIRECTION('center_axis',(0.,1.,0.));
#62254=DIRECTION('ref_axis',(0.,0.,1.));
#62255=DIRECTION('',(0.,-1.,0.));
#62256=DIRECTION('center_axis',(0.,-1.,0.));
#62257=DIRECTION('ref_axis',(0.,0.,-1.));
#62258=DIRECTION('center_axis',(0.,1.,0.));
#62259=DIRECTION('ref_axis',(0.,0.,1.));
#62260=DIRECTION('center_axis',(0.,-1.,0.));
#62261=DIRECTION('ref_axis',(0.,0.,-1.));
#62262=DIRECTION('',(0.,1.,0.));
#62263=DIRECTION('center_axis',(0.,-1.,0.));
#62264=DIRECTION('ref_axis',(0.,0.,-1.));
#62265=DIRECTION('center_axis',(0.,1.,0.));
#62266=DIRECTION('ref_axis',(0.,0.,1.));
#62267=DIRECTION('center_axis',(0.,1.,0.));
#62268=DIRECTION('ref_axis',(0.,0.,1.));
#62269=DIRECTION('',(0.,-1.,0.));
#62270=DIRECTION('center_axis',(0.,-1.,0.));
#62271=DIRECTION('ref_axis',(0.,0.,-1.));
#62272=DIRECTION('center_axis',(0.,1.,0.));
#62273=DIRECTION('ref_axis',(0.,0.,1.));
#62274=DIRECTION('center_axis',(0.,-1.,0.));
#62275=DIRECTION('ref_axis',(0.,0.,-1.));
#62276=DIRECTION('',(0.,1.,0.));
#62277=DIRECTION('center_axis',(0.,-1.,0.));
#62278=DIRECTION('ref_axis',(0.,0.,-1.));
#62279=DIRECTION('center_axis',(0.,1.,0.));
#62280=DIRECTION('ref_axis',(0.,0.,1.));
#62281=DIRECTION('center_axis',(0.,1.,0.));
#62282=DIRECTION('ref_axis',(0.,0.,1.));
#62283=DIRECTION('',(0.,-1.,0.));
#62284=DIRECTION('center_axis',(0.,-1.,0.));
#62285=DIRECTION('ref_axis',(0.,0.,-1.));
#62286=DIRECTION('center_axis',(0.,1.,0.));
#62287=DIRECTION('ref_axis',(0.,0.,1.));
#62288=DIRECTION('center_axis',(0.,-1.,0.));
#62289=DIRECTION('ref_axis',(0.,0.,-1.));
#62290=DIRECTION('',(0.,1.,0.));
#62291=DIRECTION('center_axis',(0.,-1.,0.));
#62292=DIRECTION('ref_axis',(0.,0.,-1.));
#62293=DIRECTION('center_axis',(0.,1.,0.));
#62294=DIRECTION('ref_axis',(0.,0.,1.));
#62295=DIRECTION('center_axis',(0.,1.,0.));
#62296=DIRECTION('ref_axis',(0.,0.,1.));
#62297=DIRECTION('',(0.,-1.,0.));
#62298=DIRECTION('center_axis',(0.,-1.,0.));
#62299=DIRECTION('ref_axis',(0.,0.,-1.));
#62300=DIRECTION('center_axis',(0.,1.,0.));
#62301=DIRECTION('ref_axis',(0.,0.,1.));
#62302=DIRECTION('center_axis',(0.,-1.,0.));
#62303=DIRECTION('ref_axis',(0.,0.,-1.));
#62304=DIRECTION('',(0.,1.,0.));
#62305=DIRECTION('center_axis',(0.,-1.,0.));
#62306=DIRECTION('ref_axis',(0.,0.,-1.));
#62307=DIRECTION('center_axis',(0.,1.,0.));
#62308=DIRECTION('ref_axis',(0.,0.,1.));
#62309=DIRECTION('center_axis',(0.,1.,0.));
#62310=DIRECTION('ref_axis',(0.,0.,1.));
#62311=DIRECTION('',(0.,-1.,0.));
#62312=DIRECTION('center_axis',(0.,-1.,0.));
#62313=DIRECTION('ref_axis',(0.,0.,-1.));
#62314=DIRECTION('center_axis',(0.,1.,0.));
#62315=DIRECTION('ref_axis',(0.,0.,1.));
#62316=DIRECTION('center_axis',(0.,-1.,0.));
#62317=DIRECTION('ref_axis',(0.,0.,-1.));
#62318=DIRECTION('',(0.,1.,0.));
#62319=DIRECTION('center_axis',(0.,-1.,0.));
#62320=DIRECTION('ref_axis',(0.,0.,-1.));
#62321=DIRECTION('center_axis',(0.,1.,0.));
#62322=DIRECTION('ref_axis',(0.,0.,1.));
#62323=DIRECTION('center_axis',(0.,1.,0.));
#62324=DIRECTION('ref_axis',(0.,0.,1.));
#62325=DIRECTION('',(0.,-1.,0.));
#62326=DIRECTION('center_axis',(0.,-1.,0.));
#62327=DIRECTION('ref_axis',(0.,0.,-1.));
#62328=DIRECTION('center_axis',(0.,1.,0.));
#62329=DIRECTION('ref_axis',(0.,0.,1.));
#62330=DIRECTION('center_axis',(0.,-1.,0.));
#62331=DIRECTION('ref_axis',(0.,0.,-1.));
#62332=DIRECTION('',(0.,1.,0.));
#62333=DIRECTION('center_axis',(0.,-1.,0.));
#62334=DIRECTION('ref_axis',(0.,0.,-1.));
#62335=DIRECTION('center_axis',(0.,1.,0.));
#62336=DIRECTION('ref_axis',(0.,0.,1.));
#62337=DIRECTION('center_axis',(0.,1.,0.));
#62338=DIRECTION('ref_axis',(0.,0.,1.));
#62339=DIRECTION('',(0.,-1.,0.));
#62340=DIRECTION('center_axis',(0.,-1.,0.));
#62341=DIRECTION('ref_axis',(0.,0.,-1.));
#62342=DIRECTION('center_axis',(0.,1.,0.));
#62343=DIRECTION('ref_axis',(0.,0.,1.));
#62344=DIRECTION('center_axis',(0.,-1.,0.));
#62345=DIRECTION('ref_axis',(0.,0.,-1.));
#62346=DIRECTION('',(0.,1.,0.));
#62347=DIRECTION('center_axis',(0.,-1.,0.));
#62348=DIRECTION('ref_axis',(0.,0.,-1.));
#62349=DIRECTION('center_axis',(0.,1.,0.));
#62350=DIRECTION('ref_axis',(0.,0.,1.));
#62351=DIRECTION('center_axis',(0.,1.,0.));
#62352=DIRECTION('ref_axis',(0.,0.,1.));
#62353=DIRECTION('',(0.,-1.,0.));
#62354=DIRECTION('center_axis',(0.,-1.,0.));
#62355=DIRECTION('ref_axis',(0.,0.,-1.));
#62356=DIRECTION('center_axis',(0.,1.,0.));
#62357=DIRECTION('ref_axis',(0.,0.,1.));
#62358=DIRECTION('center_axis',(0.,-1.,0.));
#62359=DIRECTION('ref_axis',(0.,0.,-1.));
#62360=DIRECTION('',(0.,1.,0.));
#62361=DIRECTION('center_axis',(0.,-1.,0.));
#62362=DIRECTION('ref_axis',(0.,0.,-1.));
#62363=DIRECTION('center_axis',(0.,1.,0.));
#62364=DIRECTION('ref_axis',(0.,0.,1.));
#62365=DIRECTION('center_axis',(0.,1.,0.));
#62366=DIRECTION('ref_axis',(0.,0.,1.));
#62367=DIRECTION('',(0.,-1.,0.));
#62368=DIRECTION('center_axis',(0.,-1.,0.));
#62369=DIRECTION('ref_axis',(0.,0.,-1.));
#62370=DIRECTION('center_axis',(0.,1.,0.));
#62371=DIRECTION('ref_axis',(0.,0.,1.));
#62372=DIRECTION('center_axis',(0.,-1.,0.));
#62373=DIRECTION('ref_axis',(0.,0.,-1.));
#62374=DIRECTION('',(0.,1.,0.));
#62375=DIRECTION('center_axis',(0.,-1.,0.));
#62376=DIRECTION('ref_axis',(0.,0.,-1.));
#62377=DIRECTION('center_axis',(0.,1.,0.));
#62378=DIRECTION('ref_axis',(0.,0.,1.));
#62379=DIRECTION('center_axis',(0.,1.,0.));
#62380=DIRECTION('ref_axis',(0.,0.,1.));
#62381=DIRECTION('',(0.,-1.,0.));
#62382=DIRECTION('center_axis',(0.,-1.,0.));
#62383=DIRECTION('ref_axis',(0.,0.,-1.));
#62384=DIRECTION('center_axis',(0.,1.,0.));
#62385=DIRECTION('ref_axis',(0.,0.,1.));
#62386=DIRECTION('center_axis',(0.,-1.,0.));
#62387=DIRECTION('ref_axis',(0.,0.,-1.));
#62388=DIRECTION('',(0.,1.,0.));
#62389=DIRECTION('center_axis',(0.,-1.,0.));
#62390=DIRECTION('ref_axis',(0.,0.,-1.));
#62391=DIRECTION('center_axis',(0.,1.,0.));
#62392=DIRECTION('ref_axis',(0.,0.,1.));
#62393=DIRECTION('center_axis',(0.,1.,0.));
#62394=DIRECTION('ref_axis',(0.,0.,1.));
#62395=DIRECTION('',(0.,-1.,0.));
#62396=DIRECTION('center_axis',(0.,-1.,0.));
#62397=DIRECTION('ref_axis',(0.,0.,-1.));
#62398=DIRECTION('center_axis',(0.,1.,0.));
#62399=DIRECTION('ref_axis',(0.,0.,1.));
#62400=DIRECTION('center_axis',(0.,-1.,0.));
#62401=DIRECTION('ref_axis',(0.,0.,-1.));
#62402=DIRECTION('',(0.,1.,0.));
#62403=DIRECTION('center_axis',(0.,-1.,0.));
#62404=DIRECTION('ref_axis',(0.,0.,-1.));
#62405=DIRECTION('center_axis',(0.,1.,0.));
#62406=DIRECTION('ref_axis',(0.,0.,1.));
#62407=DIRECTION('center_axis',(0.,1.,0.));
#62408=DIRECTION('ref_axis',(0.,0.,1.));
#62409=DIRECTION('',(0.,-1.,0.));
#62410=DIRECTION('center_axis',(0.,-1.,0.));
#62411=DIRECTION('ref_axis',(0.,0.,-1.));
#62412=DIRECTION('center_axis',(0.,1.,0.));
#62413=DIRECTION('ref_axis',(0.,0.,1.));
#62414=DIRECTION('center_axis',(0.,-1.,0.));
#62415=DIRECTION('ref_axis',(0.,0.,-1.));
#62416=DIRECTION('',(0.,1.,0.));
#62417=DIRECTION('center_axis',(0.,-1.,0.));
#62418=DIRECTION('ref_axis',(0.,0.,-1.));
#62419=DIRECTION('center_axis',(0.,1.,0.));
#62420=DIRECTION('ref_axis',(0.,0.,1.));
#62421=DIRECTION('center_axis',(0.,1.,0.));
#62422=DIRECTION('ref_axis',(0.,0.,1.));
#62423=DIRECTION('',(0.,-1.,0.));
#62424=DIRECTION('center_axis',(0.,-1.,0.));
#62425=DIRECTION('ref_axis',(0.,0.,-1.));
#62426=DIRECTION('center_axis',(0.,1.,0.));
#62427=DIRECTION('ref_axis',(0.,0.,1.));
#62428=DIRECTION('center_axis',(0.,-1.,0.));
#62429=DIRECTION('ref_axis',(0.,0.,-1.));
#62430=DIRECTION('',(0.,1.,0.));
#62431=DIRECTION('center_axis',(0.,-1.,0.));
#62432=DIRECTION('ref_axis',(0.,0.,-1.));
#62433=DIRECTION('center_axis',(0.,1.,0.));
#62434=DIRECTION('ref_axis',(0.,0.,1.));
#62435=DIRECTION('center_axis',(0.,1.,0.));
#62436=DIRECTION('ref_axis',(0.,0.,1.));
#62437=DIRECTION('',(0.,-1.,0.));
#62438=DIRECTION('center_axis',(0.,-1.,0.));
#62439=DIRECTION('ref_axis',(0.,0.,-1.));
#62440=DIRECTION('center_axis',(0.,1.,0.));
#62441=DIRECTION('ref_axis',(0.,0.,1.));
#62442=DIRECTION('center_axis',(0.,-1.,0.));
#62443=DIRECTION('ref_axis',(0.,0.,-1.));
#62444=DIRECTION('',(0.,1.,0.));
#62445=DIRECTION('center_axis',(0.,-1.,0.));
#62446=DIRECTION('ref_axis',(0.,0.,-1.));
#62447=DIRECTION('center_axis',(0.,1.,0.));
#62448=DIRECTION('ref_axis',(0.,0.,1.));
#62449=DIRECTION('center_axis',(0.,1.,0.));
#62450=DIRECTION('ref_axis',(0.,0.,1.));
#62451=DIRECTION('',(0.,-1.,0.));
#62452=DIRECTION('center_axis',(0.,-1.,0.));
#62453=DIRECTION('ref_axis',(0.,0.,-1.));
#62454=DIRECTION('center_axis',(0.,1.,0.));
#62455=DIRECTION('ref_axis',(0.,0.,1.));
#62456=DIRECTION('center_axis',(0.,-1.,0.));
#62457=DIRECTION('ref_axis',(0.,0.,-1.));
#62458=DIRECTION('',(0.,1.,0.));
#62459=DIRECTION('center_axis',(0.,-1.,0.));
#62460=DIRECTION('ref_axis',(0.,0.,-1.));
#62461=DIRECTION('center_axis',(0.,1.,0.));
#62462=DIRECTION('ref_axis',(0.,0.,1.));
#62463=DIRECTION('center_axis',(0.,1.,0.));
#62464=DIRECTION('ref_axis',(0.,0.,1.));
#62465=DIRECTION('',(0.,-1.,0.));
#62466=DIRECTION('center_axis',(0.,-1.,0.));
#62467=DIRECTION('ref_axis',(0.,0.,-1.));
#62468=DIRECTION('center_axis',(0.,1.,0.));
#62469=DIRECTION('ref_axis',(0.,0.,1.));
#62470=DIRECTION('center_axis',(0.,-1.,0.));
#62471=DIRECTION('ref_axis',(0.,0.,-1.));
#62472=DIRECTION('',(0.,1.,0.));
#62473=DIRECTION('center_axis',(0.,-1.,0.));
#62474=DIRECTION('ref_axis',(0.,0.,-1.));
#62475=DIRECTION('center_axis',(0.,1.,0.));
#62476=DIRECTION('ref_axis',(0.,0.,1.));
#62477=DIRECTION('center_axis',(0.,1.,0.));
#62478=DIRECTION('ref_axis',(0.,0.,1.));
#62479=DIRECTION('',(0.,-1.,0.));
#62480=DIRECTION('center_axis',(0.,-1.,0.));
#62481=DIRECTION('ref_axis',(0.,0.,-1.));
#62482=DIRECTION('center_axis',(0.,1.,0.));
#62483=DIRECTION('ref_axis',(0.,0.,1.));
#62484=DIRECTION('center_axis',(0.,-1.,0.));
#62485=DIRECTION('ref_axis',(0.,0.,-1.));
#62486=DIRECTION('',(0.,1.,0.));
#62487=DIRECTION('center_axis',(0.,-1.,0.));
#62488=DIRECTION('ref_axis',(0.,0.,-1.));
#62489=DIRECTION('center_axis',(0.,1.,0.));
#62490=DIRECTION('ref_axis',(0.,0.,1.));
#62491=DIRECTION('center_axis',(0.,1.,0.));
#62492=DIRECTION('ref_axis',(0.,0.,1.));
#62493=DIRECTION('',(0.,-1.,0.));
#62494=DIRECTION('center_axis',(0.,-1.,0.));
#62495=DIRECTION('ref_axis',(0.,0.,-1.));
#62496=DIRECTION('center_axis',(0.,1.,0.));
#62497=DIRECTION('ref_axis',(0.,0.,1.));
#62498=DIRECTION('center_axis',(0.,-1.,0.));
#62499=DIRECTION('ref_axis',(0.,0.,-1.));
#62500=DIRECTION('',(0.,1.,0.));
#62501=DIRECTION('center_axis',(0.,-1.,0.));
#62502=DIRECTION('ref_axis',(0.,0.,-1.));
#62503=DIRECTION('center_axis',(0.,1.,0.));
#62504=DIRECTION('ref_axis',(0.,0.,1.));
#62505=DIRECTION('center_axis',(0.,1.,0.));
#62506=DIRECTION('ref_axis',(0.,0.,1.));
#62507=DIRECTION('',(0.,-1.,0.));
#62508=DIRECTION('center_axis',(0.,-1.,0.));
#62509=DIRECTION('ref_axis',(0.,0.,-1.));
#62510=DIRECTION('center_axis',(0.,1.,0.));
#62511=DIRECTION('ref_axis',(0.,0.,1.));
#62512=DIRECTION('center_axis',(0.,-1.,0.));
#62513=DIRECTION('ref_axis',(0.,0.,-1.));
#62514=DIRECTION('',(0.,1.,0.));
#62515=DIRECTION('center_axis',(0.,-1.,0.));
#62516=DIRECTION('ref_axis',(0.,0.,-1.));
#62517=DIRECTION('center_axis',(0.,1.,0.));
#62518=DIRECTION('ref_axis',(0.,0.,1.));
#62519=DIRECTION('center_axis',(0.,1.,0.));
#62520=DIRECTION('ref_axis',(0.,0.,1.));
#62521=DIRECTION('',(0.,-1.,0.));
#62522=DIRECTION('center_axis',(0.,-1.,0.));
#62523=DIRECTION('ref_axis',(0.,0.,-1.));
#62524=DIRECTION('center_axis',(0.,1.,0.));
#62525=DIRECTION('ref_axis',(0.,0.,1.));
#62526=DIRECTION('center_axis',(0.,-1.,0.));
#62527=DIRECTION('ref_axis',(0.,0.,-1.));
#62528=DIRECTION('',(0.,1.,0.));
#62529=DIRECTION('center_axis',(0.,-1.,0.));
#62530=DIRECTION('ref_axis',(0.,0.,-1.));
#62531=DIRECTION('center_axis',(0.,1.,0.));
#62532=DIRECTION('ref_axis',(0.,0.,1.));
#62533=DIRECTION('center_axis',(0.,1.,0.));
#62534=DIRECTION('ref_axis',(0.,0.,1.));
#62535=DIRECTION('',(0.,-1.,0.));
#62536=DIRECTION('center_axis',(0.,-1.,0.));
#62537=DIRECTION('ref_axis',(0.,0.,-1.));
#62538=DIRECTION('center_axis',(0.,1.,0.));
#62539=DIRECTION('ref_axis',(0.,0.,1.));
#62540=DIRECTION('center_axis',(0.,-1.,0.));
#62541=DIRECTION('ref_axis',(0.,0.,-1.));
#62542=DIRECTION('',(0.,1.,0.));
#62543=DIRECTION('center_axis',(0.,-1.,0.));
#62544=DIRECTION('ref_axis',(0.,0.,-1.));
#62545=DIRECTION('center_axis',(0.,1.,0.));
#62546=DIRECTION('ref_axis',(0.,0.,1.));
#62547=DIRECTION('center_axis',(0.,1.,0.));
#62548=DIRECTION('ref_axis',(0.,0.,1.));
#62549=DIRECTION('',(0.,-1.,0.));
#62550=DIRECTION('center_axis',(0.,-1.,0.));
#62551=DIRECTION('ref_axis',(0.,0.,-1.));
#62552=DIRECTION('center_axis',(0.,1.,0.));
#62553=DIRECTION('ref_axis',(0.,0.,1.));
#62554=DIRECTION('center_axis',(0.,-1.,0.));
#62555=DIRECTION('ref_axis',(0.,0.,-1.));
#62556=DIRECTION('',(0.,1.,0.));
#62557=DIRECTION('center_axis',(0.,-1.,0.));
#62558=DIRECTION('ref_axis',(0.,0.,-1.));
#62559=DIRECTION('center_axis',(0.,1.,0.));
#62560=DIRECTION('ref_axis',(0.,0.,1.));
#62561=DIRECTION('center_axis',(0.,1.,0.));
#62562=DIRECTION('ref_axis',(0.,0.,1.));
#62563=DIRECTION('',(0.,-1.,0.));
#62564=DIRECTION('center_axis',(0.,-1.,0.));
#62565=DIRECTION('ref_axis',(0.,0.,-1.));
#62566=DIRECTION('center_axis',(0.,1.,0.));
#62567=DIRECTION('ref_axis',(0.,0.,1.));
#62568=DIRECTION('center_axis',(0.,-1.,0.));
#62569=DIRECTION('ref_axis',(0.,0.,-1.));
#62570=DIRECTION('',(0.,1.,0.));
#62571=DIRECTION('center_axis',(0.,-1.,0.));
#62572=DIRECTION('ref_axis',(0.,0.,-1.));
#62573=DIRECTION('center_axis',(0.,1.,0.));
#62574=DIRECTION('ref_axis',(0.,0.,1.));
#62575=DIRECTION('center_axis',(0.,1.,0.));
#62576=DIRECTION('ref_axis',(0.,0.,1.));
#62577=DIRECTION('',(0.,-1.,0.));
#62578=DIRECTION('center_axis',(0.,-1.,0.));
#62579=DIRECTION('ref_axis',(0.,0.,-1.));
#62580=DIRECTION('center_axis',(0.,1.,0.));
#62581=DIRECTION('ref_axis',(0.,0.,1.));
#62582=DIRECTION('center_axis',(0.,-1.,0.));
#62583=DIRECTION('ref_axis',(0.,0.,-1.));
#62584=DIRECTION('',(0.,1.,0.));
#62585=DIRECTION('center_axis',(0.,-1.,0.));
#62586=DIRECTION('ref_axis',(0.,0.,-1.));
#62587=DIRECTION('center_axis',(0.,1.,0.));
#62588=DIRECTION('ref_axis',(0.,0.,1.));
#62589=DIRECTION('center_axis',(0.,1.,0.));
#62590=DIRECTION('ref_axis',(0.,0.,1.));
#62591=DIRECTION('',(0.,-1.,0.));
#62592=DIRECTION('center_axis',(0.,-1.,0.));
#62593=DIRECTION('ref_axis',(0.,0.,-1.));
#62594=DIRECTION('center_axis',(0.,1.,0.));
#62595=DIRECTION('ref_axis',(0.,0.,1.));
#62596=DIRECTION('center_axis',(0.,-1.,0.));
#62597=DIRECTION('ref_axis',(0.,0.,-1.));
#62598=DIRECTION('',(0.,1.,0.));
#62599=DIRECTION('center_axis',(0.,-1.,0.));
#62600=DIRECTION('ref_axis',(0.,0.,-1.));
#62601=DIRECTION('center_axis',(0.,1.,0.));
#62602=DIRECTION('ref_axis',(0.,0.,1.));
#62603=DIRECTION('center_axis',(0.,1.,0.));
#62604=DIRECTION('ref_axis',(0.,0.,1.));
#62605=DIRECTION('',(0.,-1.,0.));
#62606=DIRECTION('center_axis',(0.,-1.,0.));
#62607=DIRECTION('ref_axis',(0.,0.,-1.));
#62608=DIRECTION('center_axis',(0.,1.,0.));
#62609=DIRECTION('ref_axis',(0.,0.,1.));
#62610=DIRECTION('center_axis',(0.,-1.,0.));
#62611=DIRECTION('ref_axis',(0.,0.,-1.));
#62612=DIRECTION('',(0.,1.,0.));
#62613=DIRECTION('center_axis',(0.,-1.,0.));
#62614=DIRECTION('ref_axis',(0.,0.,-1.));
#62615=DIRECTION('center_axis',(0.,1.,0.));
#62616=DIRECTION('ref_axis',(0.,0.,1.));
#62617=DIRECTION('center_axis',(0.,1.,0.));
#62618=DIRECTION('ref_axis',(0.,0.,1.));
#62619=DIRECTION('',(0.,-1.,0.));
#62620=DIRECTION('center_axis',(0.,-1.,0.));
#62621=DIRECTION('ref_axis',(0.,0.,-1.));
#62622=DIRECTION('center_axis',(0.,1.,0.));
#62623=DIRECTION('ref_axis',(0.,0.,1.));
#62624=DIRECTION('center_axis',(0.,-1.,0.));
#62625=DIRECTION('ref_axis',(0.,0.,-1.));
#62626=DIRECTION('',(0.,1.,0.));
#62627=DIRECTION('center_axis',(0.,-1.,0.));
#62628=DIRECTION('ref_axis',(0.,0.,-1.));
#62629=DIRECTION('center_axis',(0.,1.,0.));
#62630=DIRECTION('ref_axis',(0.,0.,1.));
#62631=DIRECTION('center_axis',(0.,1.,0.));
#62632=DIRECTION('ref_axis',(0.,0.,1.));
#62633=DIRECTION('',(0.,-1.,0.));
#62634=DIRECTION('center_axis',(0.,-1.,0.));
#62635=DIRECTION('ref_axis',(0.,0.,-1.));
#62636=DIRECTION('center_axis',(0.,1.,0.));
#62637=DIRECTION('ref_axis',(0.,0.,1.));
#62638=DIRECTION('center_axis',(0.,-1.,0.));
#62639=DIRECTION('ref_axis',(0.,0.,-1.));
#62640=DIRECTION('',(0.,1.,0.));
#62641=DIRECTION('center_axis',(0.,-1.,0.));
#62642=DIRECTION('ref_axis',(0.,0.,-1.));
#62643=DIRECTION('center_axis',(0.,1.,0.));
#62644=DIRECTION('ref_axis',(0.,0.,1.));
#62645=DIRECTION('center_axis',(0.,1.,0.));
#62646=DIRECTION('ref_axis',(0.,0.,1.));
#62647=DIRECTION('',(0.,-1.,0.));
#62648=DIRECTION('center_axis',(0.,-1.,0.));
#62649=DIRECTION('ref_axis',(0.,0.,-1.));
#62650=DIRECTION('center_axis',(0.,1.,0.));
#62651=DIRECTION('ref_axis',(0.,0.,1.));
#62652=DIRECTION('center_axis',(0.,-1.,0.));
#62653=DIRECTION('ref_axis',(0.,0.,-1.));
#62654=DIRECTION('',(0.,1.,0.));
#62655=DIRECTION('center_axis',(0.,-1.,0.));
#62656=DIRECTION('ref_axis',(0.,0.,-1.));
#62657=DIRECTION('center_axis',(0.,1.,0.));
#62658=DIRECTION('ref_axis',(0.,0.,1.));
#62659=DIRECTION('center_axis',(0.,1.,0.));
#62660=DIRECTION('ref_axis',(0.,0.,1.));
#62661=DIRECTION('',(0.,-1.,0.));
#62662=DIRECTION('center_axis',(0.,-1.,0.));
#62663=DIRECTION('ref_axis',(0.,0.,-1.));
#62664=DIRECTION('center_axis',(0.,1.,0.));
#62665=DIRECTION('ref_axis',(0.,0.,1.));
#62666=DIRECTION('center_axis',(0.,-1.,0.));
#62667=DIRECTION('ref_axis',(0.,0.,-1.));
#62668=DIRECTION('',(0.,1.,0.));
#62669=DIRECTION('center_axis',(0.,-1.,0.));
#62670=DIRECTION('ref_axis',(0.,0.,-1.));
#62671=DIRECTION('center_axis',(0.,1.,0.));
#62672=DIRECTION('ref_axis',(0.,0.,1.));
#62673=DIRECTION('center_axis',(0.,1.,0.));
#62674=DIRECTION('ref_axis',(0.,0.,1.));
#62675=DIRECTION('',(0.,-1.,0.));
#62676=DIRECTION('center_axis',(0.,-1.,0.));
#62677=DIRECTION('ref_axis',(0.,0.,-1.));
#62678=DIRECTION('center_axis',(0.,1.,0.));
#62679=DIRECTION('ref_axis',(0.,0.,1.));
#62680=DIRECTION('center_axis',(0.,-1.,0.));
#62681=DIRECTION('ref_axis',(0.,0.,-1.));
#62682=DIRECTION('',(0.,1.,0.));
#62683=DIRECTION('center_axis',(0.,-1.,0.));
#62684=DIRECTION('ref_axis',(0.,0.,-1.));
#62685=DIRECTION('center_axis',(0.,1.,0.));
#62686=DIRECTION('ref_axis',(0.,0.,1.));
#62687=DIRECTION('center_axis',(0.,1.,0.));
#62688=DIRECTION('ref_axis',(0.,0.,1.));
#62689=DIRECTION('',(0.,-1.,0.));
#62690=DIRECTION('center_axis',(0.,-1.,0.));
#62691=DIRECTION('ref_axis',(0.,0.,-1.));
#62692=DIRECTION('center_axis',(0.,1.,0.));
#62693=DIRECTION('ref_axis',(0.,0.,1.));
#62694=DIRECTION('center_axis',(0.,-1.,0.));
#62695=DIRECTION('ref_axis',(0.,0.,-1.));
#62696=DIRECTION('',(0.,1.,0.));
#62697=DIRECTION('center_axis',(0.,-1.,0.));
#62698=DIRECTION('ref_axis',(0.,0.,-1.));
#62699=DIRECTION('center_axis',(0.,1.,0.));
#62700=DIRECTION('ref_axis',(0.,0.,1.));
#62701=DIRECTION('center_axis',(0.,1.,0.));
#62702=DIRECTION('ref_axis',(0.,0.,1.));
#62703=DIRECTION('',(0.,-1.,0.));
#62704=DIRECTION('center_axis',(0.,-1.,0.));
#62705=DIRECTION('ref_axis',(0.,0.,-1.));
#62706=DIRECTION('center_axis',(0.,1.,0.));
#62707=DIRECTION('ref_axis',(0.,0.,1.));
#62708=DIRECTION('center_axis',(0.,-1.,0.));
#62709=DIRECTION('ref_axis',(0.,0.,-1.));
#62710=DIRECTION('',(0.,1.,0.));
#62711=DIRECTION('center_axis',(0.,-1.,0.));
#62712=DIRECTION('ref_axis',(0.,0.,-1.));
#62713=DIRECTION('center_axis',(0.,1.,0.));
#62714=DIRECTION('ref_axis',(0.,0.,1.));
#62715=DIRECTION('center_axis',(0.,1.,0.));
#62716=DIRECTION('ref_axis',(0.,0.,1.));
#62717=DIRECTION('',(0.,-1.,0.));
#62718=DIRECTION('center_axis',(0.,-1.,0.));
#62719=DIRECTION('ref_axis',(0.,0.,-1.));
#62720=DIRECTION('center_axis',(0.,1.,0.));
#62721=DIRECTION('ref_axis',(0.,0.,1.));
#62722=DIRECTION('center_axis',(0.,-1.,0.));
#62723=DIRECTION('ref_axis',(0.,0.,-1.));
#62724=DIRECTION('',(0.,1.,0.));
#62725=DIRECTION('center_axis',(0.,-1.,0.));
#62726=DIRECTION('ref_axis',(0.,0.,-1.));
#62727=DIRECTION('center_axis',(0.,1.,0.));
#62728=DIRECTION('ref_axis',(0.,0.,1.));
#62729=DIRECTION('center_axis',(0.,1.,0.));
#62730=DIRECTION('ref_axis',(0.,0.,1.));
#62731=DIRECTION('',(0.,-1.,0.));
#62732=DIRECTION('center_axis',(0.,-1.,0.));
#62733=DIRECTION('ref_axis',(0.,0.,-1.));
#62734=DIRECTION('center_axis',(0.,1.,0.));
#62735=DIRECTION('ref_axis',(0.,0.,1.));
#62736=DIRECTION('center_axis',(0.,-1.,0.));
#62737=DIRECTION('ref_axis',(0.,0.,-1.));
#62738=DIRECTION('',(0.,1.,0.));
#62739=DIRECTION('center_axis',(0.,-1.,0.));
#62740=DIRECTION('ref_axis',(0.,0.,-1.));
#62741=DIRECTION('center_axis',(0.,1.,0.));
#62742=DIRECTION('ref_axis',(0.,0.,1.));
#62743=DIRECTION('center_axis',(0.,1.,0.));
#62744=DIRECTION('ref_axis',(0.,0.,1.));
#62745=DIRECTION('',(0.,-1.,0.));
#62746=DIRECTION('center_axis',(0.,-1.,0.));
#62747=DIRECTION('ref_axis',(0.,0.,-1.));
#62748=DIRECTION('center_axis',(0.,1.,0.));
#62749=DIRECTION('ref_axis',(0.,0.,1.));
#62750=DIRECTION('center_axis',(0.,-1.,0.));
#62751=DIRECTION('ref_axis',(0.,0.,-1.));
#62752=DIRECTION('',(0.,1.,0.));
#62753=DIRECTION('center_axis',(0.,-1.,0.));
#62754=DIRECTION('ref_axis',(0.,0.,-1.));
#62755=DIRECTION('center_axis',(0.,1.,0.));
#62756=DIRECTION('ref_axis',(0.,0.,1.));
#62757=DIRECTION('center_axis',(0.,1.,0.));
#62758=DIRECTION('ref_axis',(0.,0.,1.));
#62759=DIRECTION('',(0.,-1.,0.));
#62760=DIRECTION('center_axis',(0.,-1.,0.));
#62761=DIRECTION('ref_axis',(0.,0.,-1.));
#62762=DIRECTION('center_axis',(0.,1.,0.));
#62763=DIRECTION('ref_axis',(0.,0.,1.));
#62764=DIRECTION('center_axis',(0.,-1.,0.));
#62765=DIRECTION('ref_axis',(0.,0.,-1.));
#62766=DIRECTION('',(0.,1.,0.));
#62767=DIRECTION('center_axis',(0.,-1.,0.));
#62768=DIRECTION('ref_axis',(0.,0.,-1.));
#62769=DIRECTION('center_axis',(0.,1.,0.));
#62770=DIRECTION('ref_axis',(0.,0.,1.));
#62771=DIRECTION('center_axis',(0.,1.,0.));
#62772=DIRECTION('ref_axis',(0.,0.,1.));
#62773=DIRECTION('',(0.,-1.,0.));
#62774=DIRECTION('center_axis',(0.,-1.,0.));
#62775=DIRECTION('ref_axis',(0.,0.,-1.));
#62776=DIRECTION('center_axis',(0.,1.,0.));
#62777=DIRECTION('ref_axis',(0.,0.,1.));
#62778=DIRECTION('center_axis',(0.,-1.,0.));
#62779=DIRECTION('ref_axis',(0.,0.,-1.));
#62780=DIRECTION('',(0.,1.,0.));
#62781=DIRECTION('center_axis',(0.,-1.,0.));
#62782=DIRECTION('ref_axis',(0.,0.,-1.));
#62783=DIRECTION('center_axis',(0.,1.,0.));
#62784=DIRECTION('ref_axis',(0.,0.,1.));
#62785=DIRECTION('center_axis',(0.,1.,0.));
#62786=DIRECTION('ref_axis',(0.,0.,1.));
#62787=DIRECTION('',(0.,-1.,0.));
#62788=DIRECTION('center_axis',(0.,-1.,0.));
#62789=DIRECTION('ref_axis',(0.,0.,-1.));
#62790=DIRECTION('center_axis',(0.,1.,0.));
#62791=DIRECTION('ref_axis',(0.,0.,1.));
#62792=DIRECTION('center_axis',(0.,-1.,0.));
#62793=DIRECTION('ref_axis',(0.,0.,-1.));
#62794=DIRECTION('',(0.,1.,0.));
#62795=DIRECTION('center_axis',(0.,-1.,0.));
#62796=DIRECTION('ref_axis',(0.,0.,-1.));
#62797=DIRECTION('center_axis',(0.,1.,0.));
#62798=DIRECTION('ref_axis',(0.,0.,1.));
#62799=DIRECTION('center_axis',(0.,1.,0.));
#62800=DIRECTION('ref_axis',(0.,0.,1.));
#62801=DIRECTION('',(0.,-1.,0.));
#62802=DIRECTION('center_axis',(0.,-1.,0.));
#62803=DIRECTION('ref_axis',(0.,0.,-1.));
#62804=DIRECTION('center_axis',(0.,1.,0.));
#62805=DIRECTION('ref_axis',(0.,0.,1.));
#62806=DIRECTION('center_axis',(0.,-1.,0.));
#62807=DIRECTION('ref_axis',(0.,0.,-1.));
#62808=DIRECTION('',(0.,1.,0.));
#62809=DIRECTION('center_axis',(0.,-1.,0.));
#62810=DIRECTION('ref_axis',(0.,0.,-1.));
#62811=DIRECTION('center_axis',(0.,1.,0.));
#62812=DIRECTION('ref_axis',(0.,0.,1.));
#62813=DIRECTION('center_axis',(0.,1.,0.));
#62814=DIRECTION('ref_axis',(0.,0.,1.));
#62815=DIRECTION('',(0.,-1.,0.));
#62816=DIRECTION('center_axis',(0.,-1.,0.));
#62817=DIRECTION('ref_axis',(0.,0.,-1.));
#62818=DIRECTION('center_axis',(0.,1.,0.));
#62819=DIRECTION('ref_axis',(0.,0.,1.));
#62820=DIRECTION('center_axis',(0.,-1.,0.));
#62821=DIRECTION('ref_axis',(0.,0.,-1.));
#62822=DIRECTION('',(0.,1.,0.));
#62823=DIRECTION('center_axis',(0.,-1.,0.));
#62824=DIRECTION('ref_axis',(0.,0.,-1.));
#62825=DIRECTION('center_axis',(0.,1.,0.));
#62826=DIRECTION('ref_axis',(0.,0.,1.));
#62827=DIRECTION('center_axis',(0.,1.,0.));
#62828=DIRECTION('ref_axis',(0.,0.,1.));
#62829=DIRECTION('',(0.,-1.,0.));
#62830=DIRECTION('center_axis',(0.,-1.,0.));
#62831=DIRECTION('ref_axis',(0.,0.,-1.));
#62832=DIRECTION('center_axis',(0.,1.,0.));
#62833=DIRECTION('ref_axis',(0.,0.,1.));
#62834=DIRECTION('center_axis',(0.,-1.,0.));
#62835=DIRECTION('ref_axis',(0.,0.,-1.));
#62836=DIRECTION('',(0.,1.,0.));
#62837=DIRECTION('center_axis',(0.,-1.,0.));
#62838=DIRECTION('ref_axis',(0.,0.,-1.));
#62839=DIRECTION('center_axis',(0.,1.,0.));
#62840=DIRECTION('ref_axis',(0.,0.,1.));
#62841=DIRECTION('center_axis',(0.,1.,0.));
#62842=DIRECTION('ref_axis',(0.,0.,1.));
#62843=DIRECTION('',(0.,-1.,0.));
#62844=DIRECTION('center_axis',(0.,-1.,0.));
#62845=DIRECTION('ref_axis',(0.,0.,-1.));
#62846=DIRECTION('center_axis',(0.,1.,0.));
#62847=DIRECTION('ref_axis',(0.,0.,1.));
#62848=DIRECTION('center_axis',(0.,-1.,0.));
#62849=DIRECTION('ref_axis',(0.,0.,-1.));
#62850=DIRECTION('',(0.,1.,0.));
#62851=DIRECTION('center_axis',(0.,-1.,0.));
#62852=DIRECTION('ref_axis',(0.,0.,-1.));
#62853=DIRECTION('center_axis',(0.,1.,0.));
#62854=DIRECTION('ref_axis',(0.,0.,1.));
#62855=DIRECTION('center_axis',(0.,1.,0.));
#62856=DIRECTION('ref_axis',(0.,0.,1.));
#62857=DIRECTION('',(0.,-1.,0.));
#62858=DIRECTION('center_axis',(0.,-1.,0.));
#62859=DIRECTION('ref_axis',(0.,0.,-1.));
#62860=DIRECTION('center_axis',(0.,1.,0.));
#62861=DIRECTION('ref_axis',(0.,0.,1.));
#62862=DIRECTION('center_axis',(0.,-1.,0.));
#62863=DIRECTION('ref_axis',(0.,0.,-1.));
#62864=DIRECTION('',(0.,1.,0.));
#62865=DIRECTION('center_axis',(0.,-1.,0.));
#62866=DIRECTION('ref_axis',(0.,0.,-1.));
#62867=DIRECTION('center_axis',(0.,1.,0.));
#62868=DIRECTION('ref_axis',(0.,0.,1.));
#62869=DIRECTION('center_axis',(0.,1.,0.));
#62870=DIRECTION('ref_axis',(0.,0.,1.));
#62871=DIRECTION('',(0.,-1.,0.));
#62872=DIRECTION('center_axis',(0.,-1.,0.));
#62873=DIRECTION('ref_axis',(0.,0.,-1.));
#62874=DIRECTION('center_axis',(0.,1.,0.));
#62875=DIRECTION('ref_axis',(0.,0.,1.));
#62876=DIRECTION('center_axis',(0.,-1.,0.));
#62877=DIRECTION('ref_axis',(0.,0.,-1.));
#62878=DIRECTION('',(0.,1.,0.));
#62879=DIRECTION('center_axis',(0.,-1.,0.));
#62880=DIRECTION('ref_axis',(0.,0.,-1.));
#62881=DIRECTION('center_axis',(0.,1.,0.));
#62882=DIRECTION('ref_axis',(0.,0.,1.));
#62883=DIRECTION('center_axis',(0.,1.,0.));
#62884=DIRECTION('ref_axis',(0.,0.,1.));
#62885=DIRECTION('',(0.,-1.,0.));
#62886=DIRECTION('center_axis',(0.,-1.,0.));
#62887=DIRECTION('ref_axis',(0.,0.,-1.));
#62888=DIRECTION('center_axis',(0.,1.,0.));
#62889=DIRECTION('ref_axis',(0.,0.,1.));
#62890=DIRECTION('center_axis',(0.,-1.,0.));
#62891=DIRECTION('ref_axis',(0.,0.,-1.));
#62892=DIRECTION('',(0.,1.,0.));
#62893=DIRECTION('center_axis',(0.,-1.,0.));
#62894=DIRECTION('ref_axis',(0.,0.,-1.));
#62895=DIRECTION('center_axis',(0.,1.,0.));
#62896=DIRECTION('ref_axis',(0.,0.,1.));
#62897=DIRECTION('center_axis',(0.,1.,0.));
#62898=DIRECTION('ref_axis',(0.,0.,1.));
#62899=DIRECTION('',(0.,-1.,0.));
#62900=DIRECTION('center_axis',(0.,-1.,0.));
#62901=DIRECTION('ref_axis',(0.,0.,-1.));
#62902=DIRECTION('center_axis',(0.,1.,0.));
#62903=DIRECTION('ref_axis',(0.,0.,1.));
#62904=DIRECTION('center_axis',(0.,-1.,0.));
#62905=DIRECTION('ref_axis',(0.,0.,-1.));
#62906=DIRECTION('',(0.,1.,0.));
#62907=DIRECTION('center_axis',(0.,-1.,0.));
#62908=DIRECTION('ref_axis',(0.,0.,-1.));
#62909=DIRECTION('center_axis',(0.,1.,0.));
#62910=DIRECTION('ref_axis',(0.,0.,1.));
#62911=DIRECTION('center_axis',(0.,1.,0.));
#62912=DIRECTION('ref_axis',(0.,0.,1.));
#62913=DIRECTION('',(0.,-1.,0.));
#62914=DIRECTION('center_axis',(0.,-1.,0.));
#62915=DIRECTION('ref_axis',(0.,0.,-1.));
#62916=DIRECTION('center_axis',(0.,1.,0.));
#62917=DIRECTION('ref_axis',(0.,0.,1.));
#62918=DIRECTION('center_axis',(0.,-1.,0.));
#62919=DIRECTION('ref_axis',(0.,0.,-1.));
#62920=DIRECTION('',(0.,1.,0.));
#62921=DIRECTION('center_axis',(0.,-1.,0.));
#62922=DIRECTION('ref_axis',(0.,0.,-1.));
#62923=DIRECTION('center_axis',(0.,1.,0.));
#62924=DIRECTION('ref_axis',(0.,0.,1.));
#62925=DIRECTION('center_axis',(0.,1.,0.));
#62926=DIRECTION('ref_axis',(0.,0.,1.));
#62927=DIRECTION('',(0.,-1.,0.));
#62928=DIRECTION('center_axis',(0.,-1.,0.));
#62929=DIRECTION('ref_axis',(0.,0.,-1.));
#62930=DIRECTION('center_axis',(0.,1.,0.));
#62931=DIRECTION('ref_axis',(0.,0.,1.));
#62932=DIRECTION('center_axis',(0.,-1.,0.));
#62933=DIRECTION('ref_axis',(0.,0.,-1.));
#62934=DIRECTION('',(0.,1.,0.));
#62935=DIRECTION('center_axis',(0.,-1.,0.));
#62936=DIRECTION('ref_axis',(0.,0.,-1.));
#62937=DIRECTION('center_axis',(0.,1.,0.));
#62938=DIRECTION('ref_axis',(0.,0.,1.));
#62939=DIRECTION('center_axis',(0.,1.,0.));
#62940=DIRECTION('ref_axis',(0.,0.,1.));
#62941=DIRECTION('',(0.,-1.,0.));
#62942=DIRECTION('center_axis',(0.,-1.,0.));
#62943=DIRECTION('ref_axis',(0.,0.,-1.));
#62944=DIRECTION('center_axis',(0.,1.,0.));
#62945=DIRECTION('ref_axis',(0.,0.,1.));
#62946=DIRECTION('center_axis',(0.,-1.,0.));
#62947=DIRECTION('ref_axis',(0.,0.,-1.));
#62948=DIRECTION('',(0.,1.,0.));
#62949=DIRECTION('center_axis',(0.,-1.,0.));
#62950=DIRECTION('ref_axis',(0.,0.,-1.));
#62951=DIRECTION('center_axis',(0.,1.,0.));
#62952=DIRECTION('ref_axis',(0.,0.,1.));
#62953=DIRECTION('center_axis',(0.,1.,0.));
#62954=DIRECTION('ref_axis',(0.,0.,1.));
#62955=DIRECTION('',(0.,-1.,0.));
#62956=DIRECTION('center_axis',(0.,-1.,0.));
#62957=DIRECTION('ref_axis',(0.,0.,-1.));
#62958=DIRECTION('center_axis',(0.,1.,0.));
#62959=DIRECTION('ref_axis',(0.,0.,1.));
#62960=DIRECTION('center_axis',(0.,-1.,0.));
#62961=DIRECTION('ref_axis',(0.,0.,-1.));
#62962=DIRECTION('',(0.,1.,0.));
#62963=DIRECTION('center_axis',(0.,-1.,0.));
#62964=DIRECTION('ref_axis',(0.,0.,-1.));
#62965=DIRECTION('center_axis',(0.,1.,0.));
#62966=DIRECTION('ref_axis',(0.,0.,1.));
#62967=DIRECTION('center_axis',(0.,1.,0.));
#62968=DIRECTION('ref_axis',(0.,0.,1.));
#62969=DIRECTION('',(0.,-1.,0.));
#62970=DIRECTION('center_axis',(0.,-1.,0.));
#62971=DIRECTION('ref_axis',(0.,0.,-1.));
#62972=DIRECTION('center_axis',(0.,1.,0.));
#62973=DIRECTION('ref_axis',(0.,0.,1.));
#62974=DIRECTION('center_axis',(0.,-1.,0.));
#62975=DIRECTION('ref_axis',(0.,0.,-1.));
#62976=DIRECTION('',(0.,1.,0.));
#62977=DIRECTION('center_axis',(0.,-1.,0.));
#62978=DIRECTION('ref_axis',(0.,0.,-1.));
#62979=DIRECTION('center_axis',(0.,1.,0.));
#62980=DIRECTION('ref_axis',(0.,0.,1.));
#62981=DIRECTION('center_axis',(0.,1.,0.));
#62982=DIRECTION('ref_axis',(0.,0.,1.));
#62983=DIRECTION('',(0.,-1.,0.));
#62984=DIRECTION('center_axis',(0.,-1.,0.));
#62985=DIRECTION('ref_axis',(0.,0.,-1.));
#62986=DIRECTION('center_axis',(0.,1.,0.));
#62987=DIRECTION('ref_axis',(0.,0.,1.));
#62988=DIRECTION('center_axis',(0.,-1.,0.));
#62989=DIRECTION('ref_axis',(0.,0.,-1.));
#62990=DIRECTION('',(0.,1.,0.));
#62991=DIRECTION('center_axis',(0.,-1.,0.));
#62992=DIRECTION('ref_axis',(0.,0.,-1.));
#62993=DIRECTION('center_axis',(0.,1.,0.));
#62994=DIRECTION('ref_axis',(0.,0.,1.));
#62995=DIRECTION('center_axis',(0.,1.,0.));
#62996=DIRECTION('ref_axis',(0.,0.,1.));
#62997=DIRECTION('',(0.,-1.,0.));
#62998=DIRECTION('center_axis',(0.,-1.,0.));
#62999=DIRECTION('ref_axis',(0.,0.,-1.));
#63000=DIRECTION('center_axis',(0.,1.,0.));
#63001=DIRECTION('ref_axis',(0.,0.,1.));
#63002=DIRECTION('center_axis',(0.,-1.,0.));
#63003=DIRECTION('ref_axis',(0.,0.,-1.));
#63004=DIRECTION('',(0.,1.,0.));
#63005=DIRECTION('center_axis',(0.,-1.,0.));
#63006=DIRECTION('ref_axis',(0.,0.,-1.));
#63007=DIRECTION('center_axis',(0.,1.,0.));
#63008=DIRECTION('ref_axis',(0.,0.,1.));
#63009=DIRECTION('center_axis',(0.,1.,0.));
#63010=DIRECTION('ref_axis',(0.,0.,1.));
#63011=DIRECTION('',(0.,-1.,0.));
#63012=DIRECTION('center_axis',(0.,-1.,0.));
#63013=DIRECTION('ref_axis',(0.,0.,-1.));
#63014=DIRECTION('center_axis',(0.,1.,0.));
#63015=DIRECTION('ref_axis',(0.,0.,1.));
#63016=DIRECTION('center_axis',(0.,-1.,0.));
#63017=DIRECTION('ref_axis',(0.,0.,-1.));
#63018=DIRECTION('',(0.,1.,0.));
#63019=DIRECTION('center_axis',(0.,-1.,0.));
#63020=DIRECTION('ref_axis',(0.,0.,-1.));
#63021=DIRECTION('center_axis',(0.,1.,0.));
#63022=DIRECTION('ref_axis',(0.,0.,1.));
#63023=DIRECTION('center_axis',(0.,1.,0.));
#63024=DIRECTION('ref_axis',(0.,0.,1.));
#63025=DIRECTION('',(0.,-1.,0.));
#63026=DIRECTION('center_axis',(0.,-1.,0.));
#63027=DIRECTION('ref_axis',(0.,0.,-1.));
#63028=DIRECTION('center_axis',(0.,1.,0.));
#63029=DIRECTION('ref_axis',(0.,0.,1.));
#63030=DIRECTION('center_axis',(0.,-1.,0.));
#63031=DIRECTION('ref_axis',(0.,0.,-1.));
#63032=DIRECTION('',(0.,1.,0.));
#63033=DIRECTION('center_axis',(0.,-1.,0.));
#63034=DIRECTION('ref_axis',(0.,0.,-1.));
#63035=DIRECTION('center_axis',(0.,1.,0.));
#63036=DIRECTION('ref_axis',(0.,0.,1.));
#63037=DIRECTION('center_axis',(0.,1.,0.));
#63038=DIRECTION('ref_axis',(0.,0.,1.));
#63039=DIRECTION('',(0.,-1.,0.));
#63040=DIRECTION('center_axis',(0.,-1.,0.));
#63041=DIRECTION('ref_axis',(0.,0.,-1.));
#63042=DIRECTION('center_axis',(0.,1.,0.));
#63043=DIRECTION('ref_axis',(0.,0.,1.));
#63044=DIRECTION('center_axis',(0.,-1.,0.));
#63045=DIRECTION('ref_axis',(0.,0.,-1.));
#63046=DIRECTION('',(0.,1.,0.));
#63047=DIRECTION('center_axis',(0.,-1.,0.));
#63048=DIRECTION('ref_axis',(0.,0.,-1.));
#63049=DIRECTION('center_axis',(0.,1.,0.));
#63050=DIRECTION('ref_axis',(0.,0.,1.));
#63051=DIRECTION('center_axis',(0.,1.,0.));
#63052=DIRECTION('ref_axis',(0.,0.,1.));
#63053=DIRECTION('',(0.,-1.,0.));
#63054=DIRECTION('center_axis',(0.,-1.,0.));
#63055=DIRECTION('ref_axis',(0.,0.,-1.));
#63056=DIRECTION('center_axis',(0.,1.,0.));
#63057=DIRECTION('ref_axis',(0.,0.,1.));
#63058=DIRECTION('center_axis',(0.,-1.,0.));
#63059=DIRECTION('ref_axis',(0.,0.,-1.));
#63060=DIRECTION('',(0.,1.,0.));
#63061=DIRECTION('center_axis',(0.,-1.,0.));
#63062=DIRECTION('ref_axis',(0.,0.,-1.));
#63063=DIRECTION('center_axis',(0.,1.,0.));
#63064=DIRECTION('ref_axis',(0.,0.,1.));
#63065=DIRECTION('center_axis',(0.,1.,0.));
#63066=DIRECTION('ref_axis',(0.,0.,1.));
#63067=DIRECTION('',(0.,-1.,0.));
#63068=DIRECTION('center_axis',(0.,-1.,0.));
#63069=DIRECTION('ref_axis',(0.,0.,-1.));
#63070=DIRECTION('center_axis',(0.,1.,0.));
#63071=DIRECTION('ref_axis',(0.,0.,1.));
#63072=DIRECTION('center_axis',(0.,-1.,0.));
#63073=DIRECTION('ref_axis',(0.,0.,-1.));
#63074=DIRECTION('',(0.,1.,0.));
#63075=DIRECTION('center_axis',(0.,-1.,0.));
#63076=DIRECTION('ref_axis',(0.,0.,-1.));
#63077=DIRECTION('center_axis',(0.,1.,0.));
#63078=DIRECTION('ref_axis',(0.,0.,1.));
#63079=DIRECTION('center_axis',(0.,1.,0.));
#63080=DIRECTION('ref_axis',(0.,0.,1.));
#63081=DIRECTION('',(0.,-1.,0.));
#63082=DIRECTION('center_axis',(0.,-1.,0.));
#63083=DIRECTION('ref_axis',(0.,0.,-1.));
#63084=DIRECTION('center_axis',(0.,1.,0.));
#63085=DIRECTION('ref_axis',(0.,0.,1.));
#63086=DIRECTION('center_axis',(0.,-1.,0.));
#63087=DIRECTION('ref_axis',(0.,0.,-1.));
#63088=DIRECTION('',(0.,1.,0.));
#63089=DIRECTION('center_axis',(0.,-1.,0.));
#63090=DIRECTION('ref_axis',(0.,0.,-1.));
#63091=DIRECTION('center_axis',(0.,1.,0.));
#63092=DIRECTION('ref_axis',(0.,0.,1.));
#63093=DIRECTION('center_axis',(0.,1.,0.));
#63094=DIRECTION('ref_axis',(0.,0.,1.));
#63095=DIRECTION('',(0.,-1.,0.));
#63096=DIRECTION('center_axis',(0.,-1.,0.));
#63097=DIRECTION('ref_axis',(0.,0.,-1.));
#63098=DIRECTION('center_axis',(0.,1.,0.));
#63099=DIRECTION('ref_axis',(0.,0.,1.));
#63100=DIRECTION('center_axis',(0.,-1.,0.));
#63101=DIRECTION('ref_axis',(0.,0.,-1.));
#63102=DIRECTION('',(0.,1.,0.));
#63103=DIRECTION('center_axis',(0.,-1.,0.));
#63104=DIRECTION('ref_axis',(0.,0.,-1.));
#63105=DIRECTION('center_axis',(0.,1.,0.));
#63106=DIRECTION('ref_axis',(0.,0.,1.));
#63107=DIRECTION('center_axis',(0.,1.,0.));
#63108=DIRECTION('ref_axis',(0.,0.,1.));
#63109=DIRECTION('',(0.,-1.,0.));
#63110=DIRECTION('center_axis',(0.,-1.,0.));
#63111=DIRECTION('ref_axis',(0.,0.,-1.));
#63112=DIRECTION('center_axis',(0.,1.,0.));
#63113=DIRECTION('ref_axis',(0.,0.,1.));
#63114=DIRECTION('center_axis',(0.,-1.,0.));
#63115=DIRECTION('ref_axis',(0.,0.,-1.));
#63116=DIRECTION('',(0.,1.,0.));
#63117=DIRECTION('center_axis',(0.,-1.,0.));
#63118=DIRECTION('ref_axis',(0.,0.,-1.));
#63119=DIRECTION('center_axis',(0.,1.,0.));
#63120=DIRECTION('ref_axis',(0.,0.,1.));
#63121=DIRECTION('center_axis',(0.,1.,0.));
#63122=DIRECTION('ref_axis',(0.,0.,1.));
#63123=DIRECTION('',(0.,-1.,0.));
#63124=DIRECTION('center_axis',(0.,-1.,0.));
#63125=DIRECTION('ref_axis',(0.,0.,-1.));
#63126=DIRECTION('center_axis',(0.,1.,0.));
#63127=DIRECTION('ref_axis',(0.,0.,1.));
#63128=DIRECTION('center_axis',(0.,-1.,0.));
#63129=DIRECTION('ref_axis',(0.,0.,-1.));
#63130=DIRECTION('',(0.,1.,0.));
#63131=DIRECTION('center_axis',(0.,-1.,0.));
#63132=DIRECTION('ref_axis',(0.,0.,-1.));
#63133=DIRECTION('center_axis',(0.,1.,0.));
#63134=DIRECTION('ref_axis',(0.,0.,1.));
#63135=DIRECTION('center_axis',(0.,1.,0.));
#63136=DIRECTION('ref_axis',(0.,0.,1.));
#63137=DIRECTION('',(0.,-1.,0.));
#63138=DIRECTION('center_axis',(0.,-1.,0.));
#63139=DIRECTION('ref_axis',(0.,0.,-1.));
#63140=DIRECTION('center_axis',(0.,1.,0.));
#63141=DIRECTION('ref_axis',(0.,0.,1.));
#63142=DIRECTION('center_axis',(0.,-1.,0.));
#63143=DIRECTION('ref_axis',(0.,0.,-1.));
#63144=DIRECTION('',(0.,1.,0.));
#63145=DIRECTION('center_axis',(0.,-1.,0.));
#63146=DIRECTION('ref_axis',(0.,0.,-1.));
#63147=DIRECTION('center_axis',(0.,1.,0.));
#63148=DIRECTION('ref_axis',(0.,0.,1.));
#63149=DIRECTION('center_axis',(0.,1.,0.));
#63150=DIRECTION('ref_axis',(0.,0.,1.));
#63151=DIRECTION('',(0.,-1.,0.));
#63152=DIRECTION('center_axis',(0.,-1.,0.));
#63153=DIRECTION('ref_axis',(0.,0.,-1.));
#63154=DIRECTION('center_axis',(0.,1.,0.));
#63155=DIRECTION('ref_axis',(0.,0.,1.));
#63156=DIRECTION('center_axis',(0.,-1.,0.));
#63157=DIRECTION('ref_axis',(0.,0.,-1.));
#63158=DIRECTION('',(0.,1.,0.));
#63159=DIRECTION('center_axis',(0.,-1.,0.));
#63160=DIRECTION('ref_axis',(0.,0.,-1.));
#63161=DIRECTION('center_axis',(0.,1.,0.));
#63162=DIRECTION('ref_axis',(0.,0.,1.));
#63163=DIRECTION('center_axis',(0.,1.,0.));
#63164=DIRECTION('ref_axis',(0.,0.,1.));
#63165=DIRECTION('',(0.,-1.,0.));
#63166=DIRECTION('center_axis',(0.,-1.,0.));
#63167=DIRECTION('ref_axis',(0.,0.,-1.));
#63168=DIRECTION('center_axis',(0.,1.,0.));
#63169=DIRECTION('ref_axis',(0.,0.,1.));
#63170=DIRECTION('center_axis',(0.,-1.,0.));
#63171=DIRECTION('ref_axis',(0.,0.,-1.));
#63172=DIRECTION('',(0.,1.,0.));
#63173=DIRECTION('center_axis',(0.,-1.,0.));
#63174=DIRECTION('ref_axis',(0.,0.,-1.));
#63175=DIRECTION('center_axis',(0.,1.,0.));
#63176=DIRECTION('ref_axis',(0.,0.,1.));
#63177=DIRECTION('center_axis',(0.,1.,0.));
#63178=DIRECTION('ref_axis',(0.,0.,1.));
#63179=DIRECTION('',(0.,-1.,0.));
#63180=DIRECTION('center_axis',(0.,-1.,0.));
#63181=DIRECTION('ref_axis',(0.,0.,-1.));
#63182=DIRECTION('center_axis',(0.,1.,0.));
#63183=DIRECTION('ref_axis',(0.,0.,1.));
#63184=DIRECTION('center_axis',(0.,-1.,0.));
#63185=DIRECTION('ref_axis',(0.,0.,-1.));
#63186=DIRECTION('',(0.,1.,0.));
#63187=DIRECTION('center_axis',(0.,-1.,0.));
#63188=DIRECTION('ref_axis',(0.,0.,-1.));
#63189=DIRECTION('center_axis',(0.,1.,0.));
#63190=DIRECTION('ref_axis',(0.,0.,1.));
#63191=DIRECTION('center_axis',(0.,1.,0.));
#63192=DIRECTION('ref_axis',(0.,0.,1.));
#63193=DIRECTION('',(0.,-1.,0.));
#63194=DIRECTION('center_axis',(0.,-1.,0.));
#63195=DIRECTION('ref_axis',(0.,0.,-1.));
#63196=DIRECTION('center_axis',(0.,1.,0.));
#63197=DIRECTION('ref_axis',(0.,0.,1.));
#63198=DIRECTION('center_axis',(0.,-1.,0.));
#63199=DIRECTION('ref_axis',(0.,0.,-1.));
#63200=DIRECTION('',(0.,1.,0.));
#63201=DIRECTION('center_axis',(0.,-1.,0.));
#63202=DIRECTION('ref_axis',(0.,0.,-1.));
#63203=DIRECTION('center_axis',(0.,1.,0.));
#63204=DIRECTION('ref_axis',(0.,0.,1.));
#63205=DIRECTION('center_axis',(0.,1.,0.));
#63206=DIRECTION('ref_axis',(0.,0.,1.));
#63207=DIRECTION('',(0.,-1.,0.));
#63208=DIRECTION('center_axis',(0.,-1.,0.));
#63209=DIRECTION('ref_axis',(0.,0.,-1.));
#63210=DIRECTION('center_axis',(0.,1.,0.));
#63211=DIRECTION('ref_axis',(0.,0.,1.));
#63212=DIRECTION('center_axis',(0.,-1.,0.));
#63213=DIRECTION('ref_axis',(0.,0.,-1.));
#63214=DIRECTION('',(0.,1.,0.));
#63215=DIRECTION('center_axis',(0.,-1.,0.));
#63216=DIRECTION('ref_axis',(0.,0.,-1.));
#63217=DIRECTION('center_axis',(0.,1.,0.));
#63218=DIRECTION('ref_axis',(0.,0.,1.));
#63219=DIRECTION('center_axis',(0.,1.,0.));
#63220=DIRECTION('ref_axis',(0.,0.,1.));
#63221=DIRECTION('',(0.,-1.,0.));
#63222=DIRECTION('center_axis',(0.,-1.,0.));
#63223=DIRECTION('ref_axis',(0.,0.,-1.));
#63224=DIRECTION('center_axis',(0.,1.,0.));
#63225=DIRECTION('ref_axis',(0.,0.,1.));
#63226=DIRECTION('center_axis',(0.,-1.,0.));
#63227=DIRECTION('ref_axis',(0.,0.,-1.));
#63228=DIRECTION('',(0.,1.,0.));
#63229=DIRECTION('center_axis',(0.,-1.,0.));
#63230=DIRECTION('ref_axis',(0.,0.,-1.));
#63231=DIRECTION('center_axis',(0.,1.,0.));
#63232=DIRECTION('ref_axis',(0.,0.,1.));
#63233=DIRECTION('center_axis',(0.,1.,0.));
#63234=DIRECTION('ref_axis',(0.,0.,1.));
#63235=DIRECTION('',(0.,-1.,0.));
#63236=DIRECTION('center_axis',(0.,-1.,0.));
#63237=DIRECTION('ref_axis',(0.,0.,-1.));
#63238=DIRECTION('center_axis',(0.,1.,0.));
#63239=DIRECTION('ref_axis',(0.,0.,1.));
#63240=DIRECTION('center_axis',(0.,-1.,0.));
#63241=DIRECTION('ref_axis',(0.,0.,-1.));
#63242=DIRECTION('',(0.,1.,0.));
#63243=DIRECTION('center_axis',(0.,-1.,0.));
#63244=DIRECTION('ref_axis',(0.,0.,-1.));
#63245=DIRECTION('center_axis',(0.,1.,0.));
#63246=DIRECTION('ref_axis',(0.,0.,1.));
#63247=DIRECTION('center_axis',(0.,1.,0.));
#63248=DIRECTION('ref_axis',(0.,0.,1.));
#63249=DIRECTION('',(0.,-1.,0.));
#63250=DIRECTION('center_axis',(0.,-1.,0.));
#63251=DIRECTION('ref_axis',(0.,0.,-1.));
#63252=DIRECTION('center_axis',(0.,1.,0.));
#63253=DIRECTION('ref_axis',(0.,0.,1.));
#63254=DIRECTION('center_axis',(0.,-1.,0.));
#63255=DIRECTION('ref_axis',(0.,0.,-1.));
#63256=DIRECTION('',(0.,1.,0.));
#63257=DIRECTION('center_axis',(0.,-1.,0.));
#63258=DIRECTION('ref_axis',(0.,0.,-1.));
#63259=DIRECTION('center_axis',(0.,1.,0.));
#63260=DIRECTION('ref_axis',(0.,0.,1.));
#63261=DIRECTION('center_axis',(0.,1.,0.));
#63262=DIRECTION('ref_axis',(0.,0.,1.));
#63263=DIRECTION('',(0.,-1.,0.));
#63264=DIRECTION('center_axis',(0.,-1.,0.));
#63265=DIRECTION('ref_axis',(0.,0.,-1.));
#63266=DIRECTION('center_axis',(0.,1.,0.));
#63267=DIRECTION('ref_axis',(0.,0.,1.));
#63268=DIRECTION('center_axis',(0.,-1.,0.));
#63269=DIRECTION('ref_axis',(0.,0.,-1.));
#63270=DIRECTION('',(0.,1.,0.));
#63271=DIRECTION('center_axis',(0.,-1.,0.));
#63272=DIRECTION('ref_axis',(0.,0.,-1.));
#63273=DIRECTION('center_axis',(0.,1.,0.));
#63274=DIRECTION('ref_axis',(0.,0.,1.));
#63275=DIRECTION('center_axis',(0.,1.,0.));
#63276=DIRECTION('ref_axis',(0.,0.,1.));
#63277=DIRECTION('',(0.,-1.,0.));
#63278=DIRECTION('center_axis',(0.,-1.,0.));
#63279=DIRECTION('ref_axis',(0.,0.,-1.));
#63280=DIRECTION('center_axis',(0.,1.,0.));
#63281=DIRECTION('ref_axis',(0.,0.,1.));
#63282=DIRECTION('center_axis',(0.,-1.,0.));
#63283=DIRECTION('ref_axis',(0.,0.,-1.));
#63284=DIRECTION('',(0.,1.,0.));
#63285=DIRECTION('center_axis',(0.,-1.,0.));
#63286=DIRECTION('ref_axis',(0.,0.,-1.));
#63287=DIRECTION('center_axis',(0.,1.,0.));
#63288=DIRECTION('ref_axis',(0.,0.,1.));
#63289=DIRECTION('center_axis',(0.,1.,0.));
#63290=DIRECTION('ref_axis',(0.,0.,1.));
#63291=DIRECTION('',(0.,-1.,0.));
#63292=DIRECTION('center_axis',(0.,-1.,0.));
#63293=DIRECTION('ref_axis',(0.,0.,-1.));
#63294=DIRECTION('center_axis',(0.,1.,0.));
#63295=DIRECTION('ref_axis',(0.,0.,1.));
#63296=DIRECTION('center_axis',(0.,-1.,0.));
#63297=DIRECTION('ref_axis',(0.,0.,-1.));
#63298=DIRECTION('',(0.,1.,0.));
#63299=DIRECTION('center_axis',(0.,-1.,0.));
#63300=DIRECTION('ref_axis',(0.,0.,-1.));
#63301=DIRECTION('center_axis',(0.,1.,0.));
#63302=DIRECTION('ref_axis',(0.,0.,1.));
#63303=DIRECTION('center_axis',(0.,1.,0.));
#63304=DIRECTION('ref_axis',(0.,0.,1.));
#63305=DIRECTION('',(0.,-1.,0.));
#63306=DIRECTION('center_axis',(0.,-1.,0.));
#63307=DIRECTION('ref_axis',(0.,0.,-1.));
#63308=DIRECTION('center_axis',(0.,1.,0.));
#63309=DIRECTION('ref_axis',(0.,0.,1.));
#63310=DIRECTION('center_axis',(0.,-1.,0.));
#63311=DIRECTION('ref_axis',(0.,0.,-1.));
#63312=DIRECTION('',(0.,1.,0.));
#63313=DIRECTION('center_axis',(0.,-1.,0.));
#63314=DIRECTION('ref_axis',(0.,0.,-1.));
#63315=DIRECTION('center_axis',(0.,1.,0.));
#63316=DIRECTION('ref_axis',(0.,0.,1.));
#63317=DIRECTION('center_axis',(0.,1.,0.));
#63318=DIRECTION('ref_axis',(0.,0.,1.));
#63319=DIRECTION('',(0.,-1.,0.));
#63320=DIRECTION('center_axis',(0.,-1.,0.));
#63321=DIRECTION('ref_axis',(0.,0.,-1.));
#63322=DIRECTION('center_axis',(0.,1.,0.));
#63323=DIRECTION('ref_axis',(0.,0.,1.));
#63324=DIRECTION('center_axis',(0.,-1.,0.));
#63325=DIRECTION('ref_axis',(0.,0.,-1.));
#63326=DIRECTION('',(0.,1.,0.));
#63327=DIRECTION('center_axis',(0.,-1.,0.));
#63328=DIRECTION('ref_axis',(0.,0.,-1.));
#63329=DIRECTION('center_axis',(0.,1.,0.));
#63330=DIRECTION('ref_axis',(0.,0.,1.));
#63331=DIRECTION('center_axis',(0.,1.,0.));
#63332=DIRECTION('ref_axis',(0.,0.,1.));
#63333=DIRECTION('',(0.,-1.,0.));
#63334=DIRECTION('center_axis',(0.,-1.,0.));
#63335=DIRECTION('ref_axis',(0.,0.,-1.));
#63336=DIRECTION('center_axis',(0.,1.,0.));
#63337=DIRECTION('ref_axis',(0.,0.,1.));
#63338=DIRECTION('center_axis',(0.,-1.,0.));
#63339=DIRECTION('ref_axis',(0.,0.,-1.));
#63340=DIRECTION('',(0.,1.,0.));
#63341=DIRECTION('center_axis',(0.,-1.,0.));
#63342=DIRECTION('ref_axis',(0.,0.,-1.));
#63343=DIRECTION('center_axis',(0.,1.,0.));
#63344=DIRECTION('ref_axis',(0.,0.,1.));
#63345=DIRECTION('center_axis',(0.,1.,0.));
#63346=DIRECTION('ref_axis',(0.,0.,1.));
#63347=DIRECTION('',(0.,-1.,0.));
#63348=DIRECTION('center_axis',(0.,-1.,0.));
#63349=DIRECTION('ref_axis',(0.,0.,-1.));
#63350=DIRECTION('center_axis',(0.,1.,0.));
#63351=DIRECTION('ref_axis',(0.,0.,1.));
#63352=DIRECTION('center_axis',(0.,-1.,0.));
#63353=DIRECTION('ref_axis',(0.,0.,-1.));
#63354=DIRECTION('',(0.,1.,0.));
#63355=DIRECTION('center_axis',(0.,-1.,0.));
#63356=DIRECTION('ref_axis',(0.,0.,-1.));
#63357=DIRECTION('center_axis',(0.,1.,0.));
#63358=DIRECTION('ref_axis',(0.,0.,1.));
#63359=DIRECTION('center_axis',(0.,1.,0.));
#63360=DIRECTION('ref_axis',(0.,0.,1.));
#63361=DIRECTION('',(0.,-1.,0.));
#63362=DIRECTION('center_axis',(0.,-1.,0.));
#63363=DIRECTION('ref_axis',(0.,0.,-1.));
#63364=DIRECTION('center_axis',(0.,1.,0.));
#63365=DIRECTION('ref_axis',(0.,0.,1.));
#63366=DIRECTION('center_axis',(0.,-1.,0.));
#63367=DIRECTION('ref_axis',(0.,0.,-1.));
#63368=DIRECTION('',(0.,1.,0.));
#63369=DIRECTION('center_axis',(0.,-1.,0.));
#63370=DIRECTION('ref_axis',(0.,0.,-1.));
#63371=DIRECTION('center_axis',(0.,1.,0.));
#63372=DIRECTION('ref_axis',(0.,0.,1.));
#63373=DIRECTION('center_axis',(0.,1.,0.));
#63374=DIRECTION('ref_axis',(0.,0.,1.));
#63375=DIRECTION('',(0.,-1.,0.));
#63376=DIRECTION('center_axis',(0.,-1.,0.));
#63377=DIRECTION('ref_axis',(0.,0.,-1.));
#63378=DIRECTION('center_axis',(0.,1.,0.));
#63379=DIRECTION('ref_axis',(0.,0.,1.));
#63380=DIRECTION('center_axis',(0.,-1.,0.));
#63381=DIRECTION('ref_axis',(0.,0.,-1.));
#63382=DIRECTION('',(0.,1.,0.));
#63383=DIRECTION('center_axis',(0.,-1.,0.));
#63384=DIRECTION('ref_axis',(0.,0.,-1.));
#63385=DIRECTION('center_axis',(0.,1.,0.));
#63386=DIRECTION('ref_axis',(0.,0.,1.));
#63387=DIRECTION('center_axis',(0.,1.,0.));
#63388=DIRECTION('ref_axis',(0.,0.,1.));
#63389=DIRECTION('',(0.,-1.,0.));
#63390=DIRECTION('center_axis',(0.,-1.,0.));
#63391=DIRECTION('ref_axis',(0.,0.,-1.));
#63392=DIRECTION('center_axis',(0.,1.,0.));
#63393=DIRECTION('ref_axis',(0.,0.,1.));
#63394=DIRECTION('center_axis',(0.,-1.,0.));
#63395=DIRECTION('ref_axis',(0.,0.,-1.));
#63396=DIRECTION('',(0.,1.,0.));
#63397=DIRECTION('center_axis',(0.,-1.,0.));
#63398=DIRECTION('ref_axis',(0.,0.,-1.));
#63399=DIRECTION('center_axis',(0.,1.,0.));
#63400=DIRECTION('ref_axis',(0.,0.,1.));
#63401=DIRECTION('center_axis',(0.,1.,0.));
#63402=DIRECTION('ref_axis',(0.,0.,1.));
#63403=DIRECTION('',(0.,-1.,0.));
#63404=DIRECTION('center_axis',(0.,-1.,0.));
#63405=DIRECTION('ref_axis',(0.,0.,-1.));
#63406=DIRECTION('center_axis',(0.,1.,0.));
#63407=DIRECTION('ref_axis',(0.,0.,1.));
#63408=DIRECTION('center_axis',(0.,-1.,0.));
#63409=DIRECTION('ref_axis',(0.,0.,-1.));
#63410=DIRECTION('',(0.,1.,0.));
#63411=DIRECTION('center_axis',(0.,-1.,0.));
#63412=DIRECTION('ref_axis',(0.,0.,-1.));
#63413=DIRECTION('center_axis',(0.,1.,0.));
#63414=DIRECTION('ref_axis',(0.,0.,1.));
#63415=DIRECTION('center_axis',(0.,1.,0.));
#63416=DIRECTION('ref_axis',(0.,0.,1.));
#63417=DIRECTION('',(0.,-1.,0.));
#63418=DIRECTION('center_axis',(0.,-1.,0.));
#63419=DIRECTION('ref_axis',(0.,0.,-1.));
#63420=DIRECTION('center_axis',(0.,1.,0.));
#63421=DIRECTION('ref_axis',(0.,0.,1.));
#63422=DIRECTION('center_axis',(0.,-1.,0.));
#63423=DIRECTION('ref_axis',(0.,0.,-1.));
#63424=DIRECTION('',(0.,1.,0.));
#63425=DIRECTION('center_axis',(0.,-1.,0.));
#63426=DIRECTION('ref_axis',(0.,0.,-1.));
#63427=DIRECTION('center_axis',(0.,1.,0.));
#63428=DIRECTION('ref_axis',(0.,0.,1.));
#63429=DIRECTION('center_axis',(0.,1.,0.));
#63430=DIRECTION('ref_axis',(0.,0.,1.));
#63431=DIRECTION('',(0.,-1.,0.));
#63432=DIRECTION('center_axis',(0.,-1.,0.));
#63433=DIRECTION('ref_axis',(0.,0.,-1.));
#63434=DIRECTION('center_axis',(0.,1.,0.));
#63435=DIRECTION('ref_axis',(0.,0.,1.));
#63436=DIRECTION('center_axis',(0.,-1.,0.));
#63437=DIRECTION('ref_axis',(0.,0.,-1.));
#63438=DIRECTION('',(0.,1.,0.));
#63439=DIRECTION('center_axis',(0.,-1.,0.));
#63440=DIRECTION('ref_axis',(0.,0.,-1.));
#63441=DIRECTION('center_axis',(0.,1.,0.));
#63442=DIRECTION('ref_axis',(0.,0.,1.));
#63443=DIRECTION('center_axis',(0.,1.,0.));
#63444=DIRECTION('ref_axis',(0.,0.,1.));
#63445=DIRECTION('',(0.,-1.,0.));
#63446=DIRECTION('center_axis',(0.,-1.,0.));
#63447=DIRECTION('ref_axis',(0.,0.,-1.));
#63448=DIRECTION('center_axis',(0.,1.,0.));
#63449=DIRECTION('ref_axis',(0.,0.,1.));
#63450=DIRECTION('center_axis',(0.,-1.,0.));
#63451=DIRECTION('ref_axis',(0.,0.,-1.));
#63452=DIRECTION('',(0.,1.,0.));
#63453=DIRECTION('center_axis',(0.,-1.,0.));
#63454=DIRECTION('ref_axis',(0.,0.,-1.));
#63455=DIRECTION('center_axis',(0.,1.,0.));
#63456=DIRECTION('ref_axis',(0.,0.,1.));
#63457=DIRECTION('center_axis',(0.,1.,0.));
#63458=DIRECTION('ref_axis',(0.,0.,1.));
#63459=DIRECTION('',(0.,-1.,0.));
#63460=DIRECTION('center_axis',(0.,-1.,0.));
#63461=DIRECTION('ref_axis',(0.,0.,-1.));
#63462=DIRECTION('center_axis',(0.,1.,0.));
#63463=DIRECTION('ref_axis',(0.,0.,1.));
#63464=DIRECTION('center_axis',(0.,-1.,0.));
#63465=DIRECTION('ref_axis',(0.,0.,-1.));
#63466=DIRECTION('',(0.,1.,0.));
#63467=DIRECTION('center_axis',(0.,-1.,0.));
#63468=DIRECTION('ref_axis',(0.,0.,-1.));
#63469=DIRECTION('center_axis',(0.,1.,0.));
#63470=DIRECTION('ref_axis',(0.,0.,1.));
#63471=DIRECTION('center_axis',(0.,1.,0.));
#63472=DIRECTION('ref_axis',(0.,0.,1.));
#63473=DIRECTION('',(0.,-1.,0.));
#63474=DIRECTION('center_axis',(0.,-1.,0.));
#63475=DIRECTION('ref_axis',(0.,0.,-1.));
#63476=DIRECTION('center_axis',(0.,1.,0.));
#63477=DIRECTION('ref_axis',(0.,0.,1.));
#63478=DIRECTION('center_axis',(0.,-1.,0.));
#63479=DIRECTION('ref_axis',(0.,0.,-1.));
#63480=DIRECTION('',(0.,1.,0.));
#63481=DIRECTION('center_axis',(0.,-1.,0.));
#63482=DIRECTION('ref_axis',(0.,0.,-1.));
#63483=DIRECTION('center_axis',(0.,1.,0.));
#63484=DIRECTION('ref_axis',(0.,0.,1.));
#63485=DIRECTION('center_axis',(0.,1.,0.));
#63486=DIRECTION('ref_axis',(0.,0.,1.));
#63487=DIRECTION('',(0.,-1.,0.));
#63488=DIRECTION('center_axis',(0.,-1.,0.));
#63489=DIRECTION('ref_axis',(0.,0.,-1.));
#63490=DIRECTION('center_axis',(0.,1.,0.));
#63491=DIRECTION('ref_axis',(0.,0.,1.));
#63492=DIRECTION('center_axis',(0.,-1.,0.));
#63493=DIRECTION('ref_axis',(0.,0.,-1.));
#63494=DIRECTION('',(0.,1.,0.));
#63495=DIRECTION('center_axis',(0.,-1.,0.));
#63496=DIRECTION('ref_axis',(0.,0.,-1.));
#63497=DIRECTION('center_axis',(0.,1.,0.));
#63498=DIRECTION('ref_axis',(0.,0.,1.));
#63499=DIRECTION('center_axis',(0.,1.,0.));
#63500=DIRECTION('ref_axis',(0.,0.,1.));
#63501=DIRECTION('',(0.,-1.,0.));
#63502=DIRECTION('center_axis',(0.,-1.,0.));
#63503=DIRECTION('ref_axis',(0.,0.,-1.));
#63504=DIRECTION('center_axis',(0.,1.,0.));
#63505=DIRECTION('ref_axis',(0.,0.,1.));
#63506=DIRECTION('center_axis',(0.,-1.,0.));
#63507=DIRECTION('ref_axis',(0.,0.,-1.));
#63508=DIRECTION('',(0.,1.,0.));
#63509=DIRECTION('center_axis',(0.,-1.,0.));
#63510=DIRECTION('ref_axis',(0.,0.,-1.));
#63511=DIRECTION('center_axis',(0.,1.,0.));
#63512=DIRECTION('ref_axis',(0.,0.,1.));
#63513=DIRECTION('center_axis',(0.,1.,0.));
#63514=DIRECTION('ref_axis',(0.,0.,1.));
#63515=DIRECTION('',(0.,-1.,0.));
#63516=DIRECTION('center_axis',(0.,-1.,0.));
#63517=DIRECTION('ref_axis',(0.,0.,-1.));
#63518=DIRECTION('center_axis',(0.,1.,0.));
#63519=DIRECTION('ref_axis',(0.,0.,1.));
#63520=DIRECTION('center_axis',(0.,-1.,0.));
#63521=DIRECTION('ref_axis',(0.,0.,-1.));
#63522=DIRECTION('',(0.,1.,0.));
#63523=DIRECTION('center_axis',(0.,-1.,0.));
#63524=DIRECTION('ref_axis',(0.,0.,-1.));
#63525=DIRECTION('center_axis',(0.,1.,0.));
#63526=DIRECTION('ref_axis',(0.,0.,1.));
#63527=DIRECTION('center_axis',(0.,1.,0.));
#63528=DIRECTION('ref_axis',(0.,0.,1.));
#63529=DIRECTION('',(0.,-1.,0.));
#63530=DIRECTION('center_axis',(0.,-1.,0.));
#63531=DIRECTION('ref_axis',(0.,0.,-1.));
#63532=DIRECTION('center_axis',(0.,1.,0.));
#63533=DIRECTION('ref_axis',(0.,0.,1.));
#63534=DIRECTION('center_axis',(0.,-1.,0.));
#63535=DIRECTION('ref_axis',(0.,0.,-1.));
#63536=DIRECTION('',(0.,1.,0.));
#63537=DIRECTION('center_axis',(0.,-1.,0.));
#63538=DIRECTION('ref_axis',(0.,0.,-1.));
#63539=DIRECTION('center_axis',(0.,1.,0.));
#63540=DIRECTION('ref_axis',(0.,0.,1.));
#63541=DIRECTION('center_axis',(0.,1.,0.));
#63542=DIRECTION('ref_axis',(0.,0.,1.));
#63543=DIRECTION('',(0.,-1.,0.));
#63544=DIRECTION('center_axis',(0.,-1.,0.));
#63545=DIRECTION('ref_axis',(0.,0.,-1.));
#63546=DIRECTION('center_axis',(0.,1.,0.));
#63547=DIRECTION('ref_axis',(0.,0.,1.));
#63548=DIRECTION('center_axis',(0.,-1.,0.));
#63549=DIRECTION('ref_axis',(0.,0.,-1.));
#63550=DIRECTION('',(0.,1.,0.));
#63551=DIRECTION('center_axis',(0.,-1.,0.));
#63552=DIRECTION('ref_axis',(0.,0.,-1.));
#63553=DIRECTION('center_axis',(0.,1.,0.));
#63554=DIRECTION('ref_axis',(0.,0.,1.));
#63555=DIRECTION('center_axis',(0.,1.,0.));
#63556=DIRECTION('ref_axis',(0.,0.,1.));
#63557=DIRECTION('',(0.,-1.,0.));
#63558=DIRECTION('center_axis',(0.,-1.,0.));
#63559=DIRECTION('ref_axis',(0.,0.,-1.));
#63560=DIRECTION('center_axis',(0.,1.,0.));
#63561=DIRECTION('ref_axis',(0.,0.,1.));
#63562=DIRECTION('center_axis',(0.,-1.,0.));
#63563=DIRECTION('ref_axis',(0.,0.,-1.));
#63564=DIRECTION('',(0.,1.,0.));
#63565=DIRECTION('center_axis',(0.,-1.,0.));
#63566=DIRECTION('ref_axis',(0.,0.,-1.));
#63567=DIRECTION('center_axis',(0.,1.,0.));
#63568=DIRECTION('ref_axis',(0.,0.,1.));
#63569=DIRECTION('center_axis',(0.,1.,0.));
#63570=DIRECTION('ref_axis',(0.,0.,1.));
#63571=DIRECTION('',(0.,-1.,0.));
#63572=DIRECTION('center_axis',(0.,-1.,0.));
#63573=DIRECTION('ref_axis',(0.,0.,-1.));
#63574=DIRECTION('center_axis',(0.,1.,0.));
#63575=DIRECTION('ref_axis',(0.,0.,1.));
#63576=DIRECTION('center_axis',(0.,-1.,0.));
#63577=DIRECTION('ref_axis',(0.,0.,-1.));
#63578=DIRECTION('',(0.,1.,0.));
#63579=DIRECTION('center_axis',(0.,-1.,0.));
#63580=DIRECTION('ref_axis',(0.,0.,-1.));
#63581=DIRECTION('center_axis',(0.,1.,0.));
#63582=DIRECTION('ref_axis',(0.,0.,1.));
#63583=DIRECTION('center_axis',(0.,1.,0.));
#63584=DIRECTION('ref_axis',(0.,0.,1.));
#63585=DIRECTION('',(0.,-1.,0.));
#63586=DIRECTION('center_axis',(0.,-1.,0.));
#63587=DIRECTION('ref_axis',(0.,0.,-1.));
#63588=DIRECTION('center_axis',(0.,1.,0.));
#63589=DIRECTION('ref_axis',(0.,0.,1.));
#63590=DIRECTION('center_axis',(0.,-1.,0.));
#63591=DIRECTION('ref_axis',(0.,0.,-1.));
#63592=DIRECTION('',(0.,1.,0.));
#63593=DIRECTION('center_axis',(0.,-1.,0.));
#63594=DIRECTION('ref_axis',(0.,0.,-1.));
#63595=DIRECTION('center_axis',(0.,1.,0.));
#63596=DIRECTION('ref_axis',(0.,0.,1.));
#63597=DIRECTION('center_axis',(0.,1.,0.));
#63598=DIRECTION('ref_axis',(0.,0.,1.));
#63599=DIRECTION('',(0.,-1.,0.));
#63600=DIRECTION('center_axis',(0.,-1.,0.));
#63601=DIRECTION('ref_axis',(0.,0.,-1.));
#63602=DIRECTION('center_axis',(0.,1.,0.));
#63603=DIRECTION('ref_axis',(0.,0.,1.));
#63604=DIRECTION('center_axis',(0.,-1.,0.));
#63605=DIRECTION('ref_axis',(0.,0.,-1.));
#63606=DIRECTION('',(0.,1.,0.));
#63607=DIRECTION('center_axis',(0.,-1.,0.));
#63608=DIRECTION('ref_axis',(0.,0.,-1.));
#63609=DIRECTION('center_axis',(0.,1.,0.));
#63610=DIRECTION('ref_axis',(0.,0.,1.));
#63611=DIRECTION('center_axis',(0.,1.,0.));
#63612=DIRECTION('ref_axis',(0.,0.,1.));
#63613=DIRECTION('',(0.,-1.,0.));
#63614=DIRECTION('center_axis',(0.,-1.,0.));
#63615=DIRECTION('ref_axis',(0.,0.,-1.));
#63616=DIRECTION('center_axis',(0.,1.,0.));
#63617=DIRECTION('ref_axis',(0.,0.,1.));
#63618=DIRECTION('center_axis',(0.,-1.,0.));
#63619=DIRECTION('ref_axis',(0.,0.,-1.));
#63620=DIRECTION('',(0.,1.,0.));
#63621=DIRECTION('center_axis',(0.,-1.,0.));
#63622=DIRECTION('ref_axis',(0.,0.,-1.));
#63623=DIRECTION('center_axis',(0.,1.,0.));
#63624=DIRECTION('ref_axis',(0.,0.,1.));
#63625=DIRECTION('center_axis',(0.,1.,0.));
#63626=DIRECTION('ref_axis',(0.,0.,1.));
#63627=DIRECTION('',(0.,-1.,0.));
#63628=DIRECTION('center_axis',(0.,-1.,0.));
#63629=DIRECTION('ref_axis',(0.,0.,-1.));
#63630=DIRECTION('center_axis',(0.,1.,0.));
#63631=DIRECTION('ref_axis',(0.,0.,1.));
#63632=DIRECTION('center_axis',(0.,-1.,0.));
#63633=DIRECTION('ref_axis',(0.,0.,-1.));
#63634=DIRECTION('',(0.,1.,0.));
#63635=DIRECTION('center_axis',(0.,-1.,0.));
#63636=DIRECTION('ref_axis',(0.,0.,-1.));
#63637=DIRECTION('center_axis',(0.,1.,0.));
#63638=DIRECTION('ref_axis',(0.,0.,1.));
#63639=DIRECTION('center_axis',(0.,1.,0.));
#63640=DIRECTION('ref_axis',(0.,0.,1.));
#63641=DIRECTION('',(0.,-1.,0.));
#63642=DIRECTION('center_axis',(0.,-1.,0.));
#63643=DIRECTION('ref_axis',(0.,0.,-1.));
#63644=DIRECTION('center_axis',(0.,1.,0.));
#63645=DIRECTION('ref_axis',(0.,0.,1.));
#63646=DIRECTION('center_axis',(0.,-1.,0.));
#63647=DIRECTION('ref_axis',(0.,0.,-1.));
#63648=DIRECTION('',(0.,1.,0.));
#63649=DIRECTION('center_axis',(0.,-1.,0.));
#63650=DIRECTION('ref_axis',(0.,0.,-1.));
#63651=DIRECTION('center_axis',(0.,1.,0.));
#63652=DIRECTION('ref_axis',(0.,0.,1.));
#63653=DIRECTION('center_axis',(0.,1.,0.));
#63654=DIRECTION('ref_axis',(0.,0.,1.));
#63655=DIRECTION('',(0.,-1.,0.));
#63656=DIRECTION('center_axis',(0.,-1.,0.));
#63657=DIRECTION('ref_axis',(0.,0.,-1.));
#63658=DIRECTION('center_axis',(0.,1.,0.));
#63659=DIRECTION('ref_axis',(0.,0.,1.));
#63660=DIRECTION('center_axis',(0.,-1.,0.));
#63661=DIRECTION('ref_axis',(0.,0.,-1.));
#63662=DIRECTION('',(0.,1.,0.));
#63663=DIRECTION('center_axis',(0.,-1.,0.));
#63664=DIRECTION('ref_axis',(0.,0.,-1.));
#63665=DIRECTION('center_axis',(0.,1.,0.));
#63666=DIRECTION('ref_axis',(0.,0.,1.));
#63667=DIRECTION('center_axis',(0.,1.,0.));
#63668=DIRECTION('ref_axis',(0.,0.,1.));
#63669=DIRECTION('',(0.,-1.,0.));
#63670=DIRECTION('center_axis',(0.,-1.,0.));
#63671=DIRECTION('ref_axis',(0.,0.,-1.));
#63672=DIRECTION('center_axis',(0.,1.,0.));
#63673=DIRECTION('ref_axis',(0.,0.,1.));
#63674=DIRECTION('center_axis',(0.,-1.,0.));
#63675=DIRECTION('ref_axis',(0.,0.,-1.));
#63676=DIRECTION('',(0.,1.,0.));
#63677=DIRECTION('center_axis',(0.,-1.,0.));
#63678=DIRECTION('ref_axis',(0.,0.,-1.));
#63679=DIRECTION('center_axis',(0.,1.,0.));
#63680=DIRECTION('ref_axis',(0.,0.,1.));
#63681=DIRECTION('center_axis',(0.,1.,0.));
#63682=DIRECTION('ref_axis',(0.,0.,1.));
#63683=DIRECTION('',(0.,-1.,0.));
#63684=DIRECTION('center_axis',(0.,-1.,0.));
#63685=DIRECTION('ref_axis',(0.,0.,-1.));
#63686=DIRECTION('center_axis',(0.,1.,0.));
#63687=DIRECTION('ref_axis',(0.,0.,1.));
#63688=DIRECTION('center_axis',(0.,-1.,0.));
#63689=DIRECTION('ref_axis',(0.,0.,-1.));
#63690=DIRECTION('',(0.,1.,0.));
#63691=DIRECTION('center_axis',(0.,-1.,0.));
#63692=DIRECTION('ref_axis',(0.,0.,-1.));
#63693=DIRECTION('center_axis',(0.,1.,0.));
#63694=DIRECTION('ref_axis',(0.,0.,1.));
#63695=DIRECTION('center_axis',(0.,1.,0.));
#63696=DIRECTION('ref_axis',(0.,0.,1.));
#63697=DIRECTION('',(0.,-1.,0.));
#63698=DIRECTION('center_axis',(0.,-1.,0.));
#63699=DIRECTION('ref_axis',(0.,0.,-1.));
#63700=DIRECTION('center_axis',(0.,1.,0.));
#63701=DIRECTION('ref_axis',(0.,0.,1.));
#63702=DIRECTION('center_axis',(0.,-1.,0.));
#63703=DIRECTION('ref_axis',(0.,0.,-1.));
#63704=DIRECTION('',(0.,1.,0.));
#63705=DIRECTION('center_axis',(0.,-1.,0.));
#63706=DIRECTION('ref_axis',(0.,0.,-1.));
#63707=DIRECTION('center_axis',(0.,1.,0.));
#63708=DIRECTION('ref_axis',(0.,0.,1.));
#63709=DIRECTION('center_axis',(0.,1.,0.));
#63710=DIRECTION('ref_axis',(0.,0.,1.));
#63711=DIRECTION('',(0.,-1.,0.));
#63712=DIRECTION('center_axis',(0.,-1.,0.));
#63713=DIRECTION('ref_axis',(0.,0.,-1.));
#63714=DIRECTION('center_axis',(0.,1.,0.));
#63715=DIRECTION('ref_axis',(0.,0.,1.));
#63716=DIRECTION('center_axis',(0.,-1.,0.));
#63717=DIRECTION('ref_axis',(0.,0.,-1.));
#63718=DIRECTION('',(0.,1.,0.));
#63719=DIRECTION('center_axis',(0.,-1.,0.));
#63720=DIRECTION('ref_axis',(0.,0.,-1.));
#63721=DIRECTION('center_axis',(0.,1.,0.));
#63722=DIRECTION('ref_axis',(0.,0.,1.));
#63723=DIRECTION('center_axis',(0.,1.,0.));
#63724=DIRECTION('ref_axis',(0.,0.,1.));
#63725=DIRECTION('',(0.,-1.,0.));
#63726=DIRECTION('center_axis',(0.,-1.,0.));
#63727=DIRECTION('ref_axis',(0.,0.,-1.));
#63728=DIRECTION('center_axis',(0.,1.,0.));
#63729=DIRECTION('ref_axis',(0.,0.,1.));
#63730=DIRECTION('center_axis',(0.,-1.,0.));
#63731=DIRECTION('ref_axis',(0.,0.,-1.));
#63732=DIRECTION('',(0.,1.,0.));
#63733=DIRECTION('center_axis',(0.,-1.,0.));
#63734=DIRECTION('ref_axis',(0.,0.,-1.));
#63735=DIRECTION('center_axis',(0.,1.,0.));
#63736=DIRECTION('ref_axis',(0.,0.,1.));
#63737=DIRECTION('center_axis',(0.,1.,0.));
#63738=DIRECTION('ref_axis',(0.,0.,1.));
#63739=DIRECTION('',(0.,-1.,0.));
#63740=DIRECTION('center_axis',(0.,-1.,0.));
#63741=DIRECTION('ref_axis',(0.,0.,-1.));
#63742=DIRECTION('center_axis',(0.,1.,0.));
#63743=DIRECTION('ref_axis',(0.,0.,1.));
#63744=DIRECTION('center_axis',(0.,-1.,0.));
#63745=DIRECTION('ref_axis',(0.,0.,-1.));
#63746=DIRECTION('',(0.,1.,0.));
#63747=DIRECTION('center_axis',(0.,-1.,0.));
#63748=DIRECTION('ref_axis',(0.,0.,-1.));
#63749=DIRECTION('center_axis',(0.,1.,0.));
#63750=DIRECTION('ref_axis',(0.,0.,1.));
#63751=DIRECTION('center_axis',(0.,1.,0.));
#63752=DIRECTION('ref_axis',(0.,0.,1.));
#63753=DIRECTION('',(0.,-1.,0.));
#63754=DIRECTION('center_axis',(0.,-1.,0.));
#63755=DIRECTION('ref_axis',(0.,0.,-1.));
#63756=DIRECTION('center_axis',(0.,1.,0.));
#63757=DIRECTION('ref_axis',(0.,0.,1.));
#63758=DIRECTION('center_axis',(0.,-1.,0.));
#63759=DIRECTION('ref_axis',(0.,0.,-1.));
#63760=DIRECTION('',(0.,1.,0.));
#63761=DIRECTION('center_axis',(0.,-1.,0.));
#63762=DIRECTION('ref_axis',(0.,0.,-1.));
#63763=DIRECTION('center_axis',(0.,1.,0.));
#63764=DIRECTION('ref_axis',(0.,0.,1.));
#63765=DIRECTION('center_axis',(0.,1.,0.));
#63766=DIRECTION('ref_axis',(0.,0.,1.));
#63767=DIRECTION('',(0.,-1.,0.));
#63768=DIRECTION('center_axis',(0.,-1.,0.));
#63769=DIRECTION('ref_axis',(0.,0.,-1.));
#63770=DIRECTION('center_axis',(0.,1.,0.));
#63771=DIRECTION('ref_axis',(0.,0.,1.));
#63772=DIRECTION('center_axis',(0.,-1.,0.));
#63773=DIRECTION('ref_axis',(0.,0.,-1.));
#63774=DIRECTION('',(0.,1.,0.));
#63775=DIRECTION('center_axis',(0.,-1.,0.));
#63776=DIRECTION('ref_axis',(0.,0.,-1.));
#63777=DIRECTION('center_axis',(0.,1.,0.));
#63778=DIRECTION('ref_axis',(0.,0.,1.));
#63779=DIRECTION('center_axis',(0.,1.,0.));
#63780=DIRECTION('ref_axis',(0.,0.,1.));
#63781=DIRECTION('',(0.,-1.,0.));
#63782=DIRECTION('center_axis',(0.,-1.,0.));
#63783=DIRECTION('ref_axis',(0.,0.,-1.));
#63784=DIRECTION('center_axis',(0.,1.,0.));
#63785=DIRECTION('ref_axis',(0.,0.,1.));
#63786=DIRECTION('center_axis',(0.,-1.,0.));
#63787=DIRECTION('ref_axis',(0.,0.,-1.));
#63788=DIRECTION('',(0.,1.,0.));
#63789=DIRECTION('center_axis',(0.,-1.,0.));
#63790=DIRECTION('ref_axis',(0.,0.,-1.));
#63791=DIRECTION('center_axis',(0.,1.,0.));
#63792=DIRECTION('ref_axis',(0.,0.,1.));
#63793=DIRECTION('center_axis',(0.,1.,0.));
#63794=DIRECTION('ref_axis',(0.,0.,1.));
#63795=DIRECTION('',(0.,-1.,0.));
#63796=DIRECTION('center_axis',(0.,-1.,0.));
#63797=DIRECTION('ref_axis',(0.,0.,-1.));
#63798=DIRECTION('center_axis',(0.,1.,0.));
#63799=DIRECTION('ref_axis',(0.,0.,1.));
#63800=DIRECTION('center_axis',(0.,-1.,0.));
#63801=DIRECTION('ref_axis',(0.,0.,-1.));
#63802=DIRECTION('',(0.,1.,0.));
#63803=DIRECTION('center_axis',(0.,-1.,0.));
#63804=DIRECTION('ref_axis',(0.,0.,-1.));
#63805=DIRECTION('center_axis',(0.,1.,0.));
#63806=DIRECTION('ref_axis',(0.,0.,1.));
#63807=DIRECTION('center_axis',(0.,1.,0.));
#63808=DIRECTION('ref_axis',(0.,0.,1.));
#63809=DIRECTION('',(0.,-1.,0.));
#63810=DIRECTION('center_axis',(0.,-1.,0.));
#63811=DIRECTION('ref_axis',(0.,0.,-1.));
#63812=DIRECTION('center_axis',(0.,1.,0.));
#63813=DIRECTION('ref_axis',(0.,0.,1.));
#63814=DIRECTION('center_axis',(0.,-1.,0.));
#63815=DIRECTION('ref_axis',(0.,0.,-1.));
#63816=DIRECTION('',(0.,1.,0.));
#63817=DIRECTION('center_axis',(0.,-1.,0.));
#63818=DIRECTION('ref_axis',(0.,0.,-1.));
#63819=DIRECTION('center_axis',(0.,1.,0.));
#63820=DIRECTION('ref_axis',(0.,0.,1.));
#63821=DIRECTION('center_axis',(0.,1.,0.));
#63822=DIRECTION('ref_axis',(0.,0.,1.));
#63823=DIRECTION('',(0.,-1.,0.));
#63824=DIRECTION('center_axis',(0.,-1.,0.));
#63825=DIRECTION('ref_axis',(0.,0.,-1.));
#63826=DIRECTION('center_axis',(0.,1.,0.));
#63827=DIRECTION('ref_axis',(0.,0.,1.));
#63828=DIRECTION('center_axis',(0.,-1.,0.));
#63829=DIRECTION('ref_axis',(0.,0.,-1.));
#63830=DIRECTION('',(0.,1.,0.));
#63831=DIRECTION('center_axis',(0.,-1.,0.));
#63832=DIRECTION('ref_axis',(0.,0.,-1.));
#63833=DIRECTION('center_axis',(0.,1.,0.));
#63834=DIRECTION('ref_axis',(0.,0.,1.));
#63835=DIRECTION('center_axis',(0.,1.,0.));
#63836=DIRECTION('ref_axis',(0.,0.,1.));
#63837=DIRECTION('',(0.,-1.,0.));
#63838=DIRECTION('center_axis',(0.,-1.,0.));
#63839=DIRECTION('ref_axis',(0.,0.,-1.));
#63840=DIRECTION('center_axis',(0.,1.,0.));
#63841=DIRECTION('ref_axis',(0.,0.,1.));
#63842=DIRECTION('center_axis',(0.,-1.,0.));
#63843=DIRECTION('ref_axis',(0.,0.,-1.));
#63844=DIRECTION('',(0.,1.,0.));
#63845=DIRECTION('center_axis',(0.,-1.,0.));
#63846=DIRECTION('ref_axis',(0.,0.,-1.));
#63847=DIRECTION('center_axis',(0.,1.,0.));
#63848=DIRECTION('ref_axis',(0.,0.,1.));
#63849=DIRECTION('center_axis',(0.,1.,0.));
#63850=DIRECTION('ref_axis',(0.,0.,1.));
#63851=DIRECTION('',(0.,-1.,0.));
#63852=DIRECTION('center_axis',(0.,-1.,0.));
#63853=DIRECTION('ref_axis',(0.,0.,-1.));
#63854=DIRECTION('center_axis',(0.,1.,0.));
#63855=DIRECTION('ref_axis',(0.,0.,1.));
#63856=DIRECTION('center_axis',(0.,-1.,0.));
#63857=DIRECTION('ref_axis',(0.,0.,-1.));
#63858=DIRECTION('',(0.,1.,0.));
#63859=DIRECTION('center_axis',(0.,-1.,0.));
#63860=DIRECTION('ref_axis',(0.,0.,-1.));
#63861=DIRECTION('center_axis',(0.,1.,0.));
#63862=DIRECTION('ref_axis',(0.,0.,1.));
#63863=DIRECTION('center_axis',(0.,1.,0.));
#63864=DIRECTION('ref_axis',(0.,0.,1.));
#63865=DIRECTION('',(0.,-1.,0.));
#63866=DIRECTION('center_axis',(0.,-1.,0.));
#63867=DIRECTION('ref_axis',(0.,0.,-1.));
#63868=DIRECTION('center_axis',(0.,1.,0.));
#63869=DIRECTION('ref_axis',(0.,0.,1.));
#63870=DIRECTION('center_axis',(0.,-1.,0.));
#63871=DIRECTION('ref_axis',(0.,0.,-1.));
#63872=DIRECTION('',(0.,1.,0.));
#63873=DIRECTION('center_axis',(0.,-1.,0.));
#63874=DIRECTION('ref_axis',(0.,0.,-1.));
#63875=DIRECTION('center_axis',(0.,1.,0.));
#63876=DIRECTION('ref_axis',(0.,0.,1.));
#63877=DIRECTION('center_axis',(0.,1.,0.));
#63878=DIRECTION('ref_axis',(0.,0.,1.));
#63879=DIRECTION('',(0.,-1.,0.));
#63880=DIRECTION('center_axis',(0.,-1.,0.));
#63881=DIRECTION('ref_axis',(0.,0.,-1.));
#63882=DIRECTION('center_axis',(0.,1.,0.));
#63883=DIRECTION('ref_axis',(0.,0.,1.));
#63884=DIRECTION('center_axis',(0.,-1.,0.));
#63885=DIRECTION('ref_axis',(0.,0.,-1.));
#63886=DIRECTION('',(0.,1.,0.));
#63887=DIRECTION('center_axis',(0.,-1.,0.));
#63888=DIRECTION('ref_axis',(0.,0.,-1.));
#63889=DIRECTION('center_axis',(0.,1.,0.));
#63890=DIRECTION('ref_axis',(0.,0.,1.));
#63891=DIRECTION('center_axis',(0.,1.,0.));
#63892=DIRECTION('ref_axis',(0.,0.,1.));
#63893=DIRECTION('',(0.,-1.,0.));
#63894=DIRECTION('center_axis',(0.,-1.,0.));
#63895=DIRECTION('ref_axis',(0.,0.,-1.));
#63896=DIRECTION('center_axis',(0.,1.,0.));
#63897=DIRECTION('ref_axis',(0.,0.,1.));
#63898=DIRECTION('center_axis',(0.,-1.,0.));
#63899=DIRECTION('ref_axis',(0.,0.,-1.));
#63900=DIRECTION('',(0.,1.,0.));
#63901=DIRECTION('center_axis',(0.,-1.,0.));
#63902=DIRECTION('ref_axis',(0.,0.,-1.));
#63903=DIRECTION('center_axis',(0.,1.,0.));
#63904=DIRECTION('ref_axis',(0.,0.,1.));
#63905=DIRECTION('center_axis',(0.,1.,0.));
#63906=DIRECTION('ref_axis',(0.,0.,1.));
#63907=DIRECTION('',(0.,-1.,0.));
#63908=DIRECTION('center_axis',(0.,-1.,0.));
#63909=DIRECTION('ref_axis',(0.,0.,-1.));
#63910=DIRECTION('center_axis',(0.,1.,0.));
#63911=DIRECTION('ref_axis',(0.,0.,1.));
#63912=DIRECTION('center_axis',(0.,-1.,0.));
#63913=DIRECTION('ref_axis',(0.,0.,-1.));
#63914=DIRECTION('',(0.,1.,0.));
#63915=DIRECTION('center_axis',(0.,-1.,0.));
#63916=DIRECTION('ref_axis',(0.,0.,-1.));
#63917=DIRECTION('center_axis',(0.,1.,0.));
#63918=DIRECTION('ref_axis',(0.,0.,1.));
#63919=DIRECTION('center_axis',(0.,1.,0.));
#63920=DIRECTION('ref_axis',(0.,0.,1.));
#63921=DIRECTION('',(0.,-1.,0.));
#63922=DIRECTION('center_axis',(0.,-1.,0.));
#63923=DIRECTION('ref_axis',(0.,0.,-1.));
#63924=DIRECTION('center_axis',(0.,1.,0.));
#63925=DIRECTION('ref_axis',(0.,0.,1.));
#63926=DIRECTION('center_axis',(0.,-1.,0.));
#63927=DIRECTION('ref_axis',(0.,0.,-1.));
#63928=DIRECTION('',(0.,1.,0.));
#63929=DIRECTION('center_axis',(0.,-1.,0.));
#63930=DIRECTION('ref_axis',(0.,0.,-1.));
#63931=DIRECTION('center_axis',(0.,1.,0.));
#63932=DIRECTION('ref_axis',(0.,0.,1.));
#63933=DIRECTION('center_axis',(0.,1.,0.));
#63934=DIRECTION('ref_axis',(0.,0.,1.));
#63935=DIRECTION('',(0.,-1.,0.));
#63936=DIRECTION('center_axis',(0.,-1.,0.));
#63937=DIRECTION('ref_axis',(0.,0.,-1.));
#63938=DIRECTION('center_axis',(0.,1.,0.));
#63939=DIRECTION('ref_axis',(0.,0.,1.));
#63940=DIRECTION('center_axis',(0.,-1.,0.));
#63941=DIRECTION('ref_axis',(0.,0.,-1.));
#63942=DIRECTION('',(0.,1.,0.));
#63943=DIRECTION('center_axis',(0.,-1.,0.));
#63944=DIRECTION('ref_axis',(0.,0.,-1.));
#63945=DIRECTION('center_axis',(0.,1.,0.));
#63946=DIRECTION('ref_axis',(0.,0.,1.));
#63947=DIRECTION('center_axis',(0.,1.,0.));
#63948=DIRECTION('ref_axis',(0.,0.,1.));
#63949=DIRECTION('',(0.,-1.,0.));
#63950=DIRECTION('center_axis',(0.,-1.,0.));
#63951=DIRECTION('ref_axis',(0.,0.,-1.));
#63952=DIRECTION('center_axis',(0.,1.,0.));
#63953=DIRECTION('ref_axis',(0.,0.,1.));
#63954=DIRECTION('center_axis',(0.,-1.,0.));
#63955=DIRECTION('ref_axis',(0.,0.,-1.));
#63956=DIRECTION('',(0.,1.,0.));
#63957=DIRECTION('center_axis',(0.,-1.,0.));
#63958=DIRECTION('ref_axis',(0.,0.,-1.));
#63959=DIRECTION('center_axis',(0.,1.,0.));
#63960=DIRECTION('ref_axis',(0.,0.,1.));
#63961=DIRECTION('center_axis',(0.,1.,0.));
#63962=DIRECTION('ref_axis',(0.,0.,1.));
#63963=DIRECTION('',(0.,-1.,0.));
#63964=DIRECTION('center_axis',(0.,-1.,0.));
#63965=DIRECTION('ref_axis',(0.,0.,-1.));
#63966=DIRECTION('center_axis',(0.,1.,0.));
#63967=DIRECTION('ref_axis',(0.,0.,1.));
#63968=DIRECTION('center_axis',(0.,-1.,0.));
#63969=DIRECTION('ref_axis',(0.,0.,-1.));
#63970=DIRECTION('',(0.,1.,0.));
#63971=DIRECTION('center_axis',(0.,-1.,0.));
#63972=DIRECTION('ref_axis',(0.,0.,-1.));
#63973=DIRECTION('center_axis',(0.,1.,0.));
#63974=DIRECTION('ref_axis',(0.,0.,1.));
#63975=DIRECTION('center_axis',(0.,1.,0.));
#63976=DIRECTION('ref_axis',(0.,0.,1.));
#63977=DIRECTION('',(0.,-1.,0.));
#63978=DIRECTION('center_axis',(0.,-1.,0.));
#63979=DIRECTION('ref_axis',(0.,0.,-1.));
#63980=DIRECTION('center_axis',(0.,1.,0.));
#63981=DIRECTION('ref_axis',(0.,0.,1.));
#63982=DIRECTION('center_axis',(0.,-1.,0.));
#63983=DIRECTION('ref_axis',(0.,0.,-1.));
#63984=DIRECTION('',(0.,1.,0.));
#63985=DIRECTION('center_axis',(0.,-1.,0.));
#63986=DIRECTION('ref_axis',(0.,0.,-1.));
#63987=DIRECTION('center_axis',(0.,1.,0.));
#63988=DIRECTION('ref_axis',(0.,0.,1.));
#63989=DIRECTION('center_axis',(0.,1.,0.));
#63990=DIRECTION('ref_axis',(0.,0.,1.));
#63991=DIRECTION('',(0.,-1.,0.));
#63992=DIRECTION('center_axis',(0.,-1.,0.));
#63993=DIRECTION('ref_axis',(0.,0.,-1.));
#63994=DIRECTION('center_axis',(0.,1.,0.));
#63995=DIRECTION('ref_axis',(0.,0.,1.));
#63996=DIRECTION('center_axis',(0.,-1.,0.));
#63997=DIRECTION('ref_axis',(0.,0.,-1.));
#63998=DIRECTION('',(0.,1.,0.));
#63999=DIRECTION('center_axis',(0.,-1.,0.));
#64000=DIRECTION('ref_axis',(0.,0.,-1.));
#64001=DIRECTION('center_axis',(0.,1.,0.));
#64002=DIRECTION('ref_axis',(0.,0.,1.));
#64003=DIRECTION('center_axis',(0.,1.,0.));
#64004=DIRECTION('ref_axis',(0.,0.,1.));
#64005=DIRECTION('',(0.,-1.,0.));
#64006=DIRECTION('center_axis',(0.,-1.,0.));
#64007=DIRECTION('ref_axis',(0.,0.,-1.));
#64008=DIRECTION('center_axis',(0.,1.,0.));
#64009=DIRECTION('ref_axis',(0.,0.,1.));
#64010=DIRECTION('center_axis',(0.,-1.,0.));
#64011=DIRECTION('ref_axis',(0.,0.,-1.));
#64012=DIRECTION('',(0.,1.,0.));
#64013=DIRECTION('center_axis',(0.,-1.,0.));
#64014=DIRECTION('ref_axis',(0.,0.,-1.));
#64015=DIRECTION('center_axis',(0.,1.,0.));
#64016=DIRECTION('ref_axis',(0.,0.,1.));
#64017=DIRECTION('center_axis',(0.,1.,0.));
#64018=DIRECTION('ref_axis',(0.,0.,1.));
#64019=DIRECTION('',(0.,-1.,0.));
#64020=DIRECTION('center_axis',(0.,-1.,0.));
#64021=DIRECTION('ref_axis',(0.,0.,-1.));
#64022=DIRECTION('center_axis',(0.,1.,0.));
#64023=DIRECTION('ref_axis',(0.,0.,1.));
#64024=DIRECTION('center_axis',(0.,-1.,0.));
#64025=DIRECTION('ref_axis',(0.,0.,-1.));
#64026=DIRECTION('',(0.,1.,0.));
#64027=DIRECTION('center_axis',(0.,-1.,0.));
#64028=DIRECTION('ref_axis',(0.,0.,-1.));
#64029=DIRECTION('center_axis',(0.,1.,0.));
#64030=DIRECTION('ref_axis',(0.,0.,1.));
#64031=DIRECTION('center_axis',(0.,1.,0.));
#64032=DIRECTION('ref_axis',(0.,0.,1.));
#64033=DIRECTION('',(0.,-1.,0.));
#64034=DIRECTION('center_axis',(0.,-1.,0.));
#64035=DIRECTION('ref_axis',(0.,0.,-1.));
#64036=DIRECTION('center_axis',(0.,1.,0.));
#64037=DIRECTION('ref_axis',(0.,0.,1.));
#64038=DIRECTION('center_axis',(0.,-1.,0.));
#64039=DIRECTION('ref_axis',(0.,0.,-1.));
#64040=DIRECTION('',(0.,1.,0.));
#64041=DIRECTION('center_axis',(0.,-1.,0.));
#64042=DIRECTION('ref_axis',(0.,0.,-1.));
#64043=DIRECTION('center_axis',(0.,-1.,0.));
#64044=DIRECTION('ref_axis',(0.,0.,-1.));
#64045=DIRECTION('center_axis',(-1.,0.,-1.22464679914735E-16));
#64046=DIRECTION('ref_axis',(-1.22464679914735E-16,0.,1.));
#64047=DIRECTION('center_axis',(0.,1.,0.));
#64048=DIRECTION('ref_axis',(0.,0.,-1.));
#64049=DIRECTION('center_axis',(0.,-1.,0.));
#64050=DIRECTION('ref_axis',(0.,0.,1.));
#64051=DIRECTION('center_axis',(0.,-1.,0.));
#64052=DIRECTION('ref_axis',(0.,0.,-1.));
#64053=DIRECTION('',(0.,1.,0.));
#64054=DIRECTION('center_axis',(0.,-1.,0.));
#64055=DIRECTION('ref_axis',(0.,0.,-1.));
#64056=DIRECTION('center_axis',(0.,-1.,2.84598943930249E-15));
#64057=DIRECTION('ref_axis',(0.,0.,-1.));
#64058=DIRECTION('center_axis',(0.,-1.,2.84598943930249E-15));
#64059=DIRECTION('ref_axis',(0.,-2.84598943930249E-15,-1.));
#64060=DIRECTION('center_axis',(-1.,-3.48533185724897E-31,-1.22464679914735E-16));
#64061=DIRECTION('ref_axis',(-1.22464679914735E-16,0.,1.));
#64062=DIRECTION('center_axis',(0.,1.,-2.84598943930249E-15));
#64063=DIRECTION('ref_axis',(0.,-2.84598943930249E-15,-1.));
#64064=DIRECTION('center_axis',(0.,1.,-2.84598943930249E-15));
#64065=DIRECTION('ref_axis',(0.,-2.84598943930249E-15,-1.));
#64066=DIRECTION('center_axis',(0.,1.,-2.84598943930249E-15));
#64067=DIRECTION('ref_axis',(0.,0.,1.));
#64068=DIRECTION('center_axis',(0.,1.,-2.84598943930249E-15));
#64069=DIRECTION('ref_axis',(0.,2.84598943930249E-15,1.));
#64070=DIRECTION('center_axis',(-1.,3.48533185724897E-31,1.22464679914735E-16));
#64071=DIRECTION('ref_axis',(-1.22464679914735E-16,0.,-1.));
#64072=DIRECTION('center_axis',(0.,-1.,2.84598943930249E-15));
#64073=DIRECTION('ref_axis',(0.,2.84598943930249E-15,1.));
#64074=DIRECTION('center_axis',(0.,1.,-2.84598943930249E-15));
#64075=DIRECTION('ref_axis',(0.,2.84598943930249E-15,1.));
#64076=DIRECTION('',(0.,-1.,2.84598943930249E-15));
#64077=DIRECTION('center_axis',(1.,0.,0.));
#64078=DIRECTION('ref_axis',(0.,0.,1.));
#64079=DIRECTION('center_axis',(0.,-1.,0.));
#64080=DIRECTION('ref_axis',(0.,0.,-1.));
#64081=DIRECTION('center_axis',(0.,-1.,0.));
#64082=DIRECTION('ref_axis',(0.,0.,-1.));
#64083=DIRECTION('center_axis',(0.,-1.,0.));
#64084=DIRECTION('ref_axis',(0.,0.,1.));
#64085=DIRECTION('center_axis',(-1.,0.,-1.22464679914735E-16));
#64086=DIRECTION('ref_axis',(-1.22464679914735E-16,0.,1.));
#64087=DIRECTION('center_axis',(0.,1.,0.));
#64088=DIRECTION('ref_axis',(0.,0.,-1.));
#64089=DIRECTION('center_axis',(0.,1.,0.));
#64090=DIRECTION('ref_axis',(0.,0.,1.));
#64091=DIRECTION('center_axis',(0.,1.,0.));
#64092=DIRECTION('ref_axis',(0.,0.,1.));
#64093=DIRECTION('center_axis',(-1.,0.,1.22464679914735E-16));
#64094=DIRECTION('ref_axis',(-1.22464679914735E-16,0.,-1.));
#64095=DIRECTION('center_axis',(0.,-1.,0.));
#64096=DIRECTION('ref_axis',(0.,0.,1.));
#64097=DIRECTION('center_axis',(0.,-1.,0.));
#64098=DIRECTION('ref_axis',(0.,0.,-1.));
#64099=DIRECTION('center_axis',(-1.,0.,-1.22464679914735E-16));
#64100=DIRECTION('ref_axis',(-1.22464679914735E-16,0.,1.));
#64101=DIRECTION('center_axis',(0.,1.,0.));
#64102=DIRECTION('ref_axis',(0.,0.,1.));
#64103=DIRECTION('center_axis',(0.,-1.,0.));
#64104=DIRECTION('ref_axis',(0.,0.,-1.));
#64105=DIRECTION('center_axis',(0.,1.,0.));
#64106=DIRECTION('ref_axis',(0.,0.,1.));
#64107=DIRECTION('',(9.85939117684628E-18,0.996753959471403,-0.0805080385929296));
#64108=DIRECTION('center_axis',(0.,-1.,0.));
#64109=DIRECTION('ref_axis',(0.,0.,-1.));
#64110=DIRECTION('center_axis',(0.,-1.,0.));
#64111=DIRECTION('ref_axis',(0.,0.,-1.));
#64112=DIRECTION('center_axis',(0.,-1.,0.));
#64113=DIRECTION('ref_axis',(0.,0.,-1.));
#64114=DIRECTION('center_axis',(-1.,0.,-1.22464679914735E-16));
#64115=DIRECTION('ref_axis',(-1.22464679914735E-16,0.,1.));
#64116=DIRECTION('center_axis',(0.,1.,0.));
#64117=DIRECTION('ref_axis',(0.,0.,-1.));
#64118=DIRECTION('center_axis',(0.,1.,0.));
#64119=DIRECTION('ref_axis',(0.,0.,1.));
#64120=DIRECTION('',(0.,-1.,0.));
#64121=DIRECTION('center_axis',(0.,1.,0.));
#64122=DIRECTION('ref_axis',(0.,0.,1.));
#64123=DIRECTION('',(0.,1.,0.));
#64124=DIRECTION('center_axis',(0.,-1.,0.));
#64125=DIRECTION('ref_axis',(0.,0.,-1.));
#64126=DIRECTION('center_axis',(0.,1.,0.));
#64127=DIRECTION('ref_axis',(0.,0.,1.));
#64128=DIRECTION('',(0.,-1.,0.));
#64129=DIRECTION('center_axis',(0.,1.,0.));
#64130=DIRECTION('ref_axis',(0.,0.,1.));
#64131=DIRECTION('center_axis',(0.,1.,0.));
#64132=DIRECTION('ref_axis',(0.,0.,1.));
#64133=DIRECTION('center_axis',(0.,-1.,0.));
#64134=DIRECTION('ref_axis',(0.,0.,-1.));
#64135=DIRECTION('center_axis',(0.,-1.,0.));
#64136=DIRECTION('ref_axis',(0.,0.,-1.));
#64137=DIRECTION('center_axis',(0.,1.,-2.84598943930249E-15));
#64138=DIRECTION('ref_axis',(0.,2.84598943930249E-15,1.));
#64139=DIRECTION('center_axis',(0.,-1.,2.84598943930249E-15));
#64140=DIRECTION('ref_axis',(0.,-2.84598943930249E-15,-1.));
#64141=DIRECTION('center_axis',(0.,1.,0.));
#64142=DIRECTION('ref_axis',(0.,0.,1.));
#64143=DIRECTION('center_axis',(0.,1.,0.));
#64144=DIRECTION('ref_axis',(0.,0.,1.));
#64145=DIRECTION('center_axis',(0.,1.,0.));
#64146=DIRECTION('ref_axis',(0.,0.,1.));
#64147=DIRECTION('center_axis',(0.,-1.,0.));
#64148=DIRECTION('ref_axis',(0.,0.,-1.));
#64149=DIRECTION('center_axis',(0.,1.,0.));
#64150=DIRECTION('ref_axis',(0.,0.,1.));
#64151=DIRECTION('center_axis',(0.,-1.,0.));
#64152=DIRECTION('ref_axis',(0.,0.,-1.));
#64153=DIRECTION('center_axis',(0.,1.,0.));
#64154=DIRECTION('ref_axis',(0.,0.,1.));
#64155=DIRECTION('center_axis',(0.,-1.,0.));
#64156=DIRECTION('ref_axis',(0.,0.,-1.));
#64157=DIRECTION('center_axis',(0.,1.,0.));
#64158=DIRECTION('ref_axis',(0.,0.,1.));
#64159=DIRECTION('center_axis',(0.,-1.,0.));
#64160=DIRECTION('ref_axis',(0.,0.,-1.));
#64161=DIRECTION('center_axis',(0.,1.,0.));
#64162=DIRECTION('ref_axis',(0.,0.,1.));
#64163=DIRECTION('center_axis',(0.,-1.,0.));
#64164=DIRECTION('ref_axis',(0.,0.,-1.));
#64165=DIRECTION('center_axis',(0.,1.,0.));
#64166=DIRECTION('ref_axis',(0.,0.,1.));
#64167=DIRECTION('center_axis',(0.,-1.,0.));
#64168=DIRECTION('ref_axis',(0.,0.,-1.));
#64169=DIRECTION('center_axis',(0.,1.,0.));
#64170=DIRECTION('ref_axis',(0.,0.,1.));
#64171=DIRECTION('center_axis',(0.,-1.,0.));
#64172=DIRECTION('ref_axis',(0.,0.,-1.));
#64173=DIRECTION('center_axis',(0.,1.,0.));
#64174=DIRECTION('ref_axis',(0.,0.,1.));
#64175=DIRECTION('center_axis',(0.,-1.,0.));
#64176=DIRECTION('ref_axis',(0.,0.,-1.));
#64177=DIRECTION('center_axis',(0.,1.,0.));
#64178=DIRECTION('ref_axis',(0.,0.,1.));
#64179=DIRECTION('center_axis',(0.,-1.,0.));
#64180=DIRECTION('ref_axis',(0.,0.,-1.));
#64181=DIRECTION('center_axis',(0.,1.,0.));
#64182=DIRECTION('ref_axis',(0.,0.,1.));
#64183=DIRECTION('center_axis',(0.,-1.,0.));
#64184=DIRECTION('ref_axis',(0.,0.,-1.));
#64185=DIRECTION('center_axis',(0.,1.,0.));
#64186=DIRECTION('ref_axis',(0.,0.,1.));
#64187=DIRECTION('center_axis',(0.,-1.,0.));
#64188=DIRECTION('ref_axis',(0.,0.,-1.));
#64189=DIRECTION('center_axis',(0.,1.,0.));
#64190=DIRECTION('ref_axis',(0.,0.,1.));
#64191=DIRECTION('center_axis',(0.,-1.,0.));
#64192=DIRECTION('ref_axis',(0.,0.,-1.));
#64193=DIRECTION('center_axis',(0.,1.,0.));
#64194=DIRECTION('ref_axis',(0.,0.,1.));
#64195=DIRECTION('center_axis',(0.,-1.,0.));
#64196=DIRECTION('ref_axis',(0.,0.,-1.));
#64197=DIRECTION('center_axis',(0.,1.,0.));
#64198=DIRECTION('ref_axis',(0.,0.,1.));
#64199=DIRECTION('center_axis',(0.,-1.,0.));
#64200=DIRECTION('ref_axis',(0.,0.,-1.));
#64201=DIRECTION('center_axis',(0.,1.,0.));
#64202=DIRECTION('ref_axis',(0.,0.,1.));
#64203=DIRECTION('center_axis',(0.,-1.,0.));
#64204=DIRECTION('ref_axis',(0.,0.,-1.));
#64205=DIRECTION('center_axis',(0.,1.,0.));
#64206=DIRECTION('ref_axis',(0.,0.,1.));
#64207=DIRECTION('center_axis',(0.,-1.,0.));
#64208=DIRECTION('ref_axis',(0.,0.,-1.));
#64209=DIRECTION('center_axis',(0.,1.,0.));
#64210=DIRECTION('ref_axis',(0.,0.,1.));
#64211=DIRECTION('center_axis',(0.,-1.,0.));
#64212=DIRECTION('ref_axis',(0.,0.,-1.));
#64213=DIRECTION('center_axis',(0.,1.,0.));
#64214=DIRECTION('ref_axis',(0.,0.,1.));
#64215=DIRECTION('center_axis',(0.,-1.,0.));
#64216=DIRECTION('ref_axis',(0.,0.,-1.));
#64217=DIRECTION('center_axis',(0.,1.,0.));
#64218=DIRECTION('ref_axis',(0.,0.,1.));
#64219=DIRECTION('center_axis',(0.,-1.,0.));
#64220=DIRECTION('ref_axis',(0.,0.,-1.));
#64221=DIRECTION('center_axis',(0.,1.,0.));
#64222=DIRECTION('ref_axis',(0.,0.,1.));
#64223=DIRECTION('center_axis',(0.,-1.,0.));
#64224=DIRECTION('ref_axis',(0.,0.,-1.));
#64225=DIRECTION('center_axis',(0.,1.,0.));
#64226=DIRECTION('ref_axis',(0.,0.,1.));
#64227=DIRECTION('center_axis',(0.,-1.,0.));
#64228=DIRECTION('ref_axis',(0.,0.,-1.));
#64229=DIRECTION('center_axis',(0.,1.,0.));
#64230=DIRECTION('ref_axis',(0.,0.,1.));
#64231=DIRECTION('center_axis',(0.,-1.,0.));
#64232=DIRECTION('ref_axis',(0.,0.,-1.));
#64233=DIRECTION('center_axis',(0.,1.,0.));
#64234=DIRECTION('ref_axis',(0.,0.,1.));
#64235=DIRECTION('center_axis',(0.,-1.,0.));
#64236=DIRECTION('ref_axis',(0.,0.,-1.));
#64237=DIRECTION('center_axis',(0.,1.,0.));
#64238=DIRECTION('ref_axis',(0.,0.,1.));
#64239=DIRECTION('center_axis',(0.,-1.,0.));
#64240=DIRECTION('ref_axis',(0.,0.,-1.));
#64241=DIRECTION('center_axis',(0.,1.,0.));
#64242=DIRECTION('ref_axis',(0.,0.,1.));
#64243=DIRECTION('center_axis',(0.,-1.,0.));
#64244=DIRECTION('ref_axis',(0.,0.,-1.));
#64245=DIRECTION('center_axis',(0.,1.,0.));
#64246=DIRECTION('ref_axis',(0.,0.,1.));
#64247=DIRECTION('center_axis',(0.,-1.,0.));
#64248=DIRECTION('ref_axis',(0.,0.,-1.));
#64249=DIRECTION('center_axis',(0.,1.,0.));
#64250=DIRECTION('ref_axis',(0.,0.,1.));
#64251=DIRECTION('center_axis',(0.,-1.,0.));
#64252=DIRECTION('ref_axis',(0.,0.,-1.));
#64253=DIRECTION('center_axis',(0.,1.,0.));
#64254=DIRECTION('ref_axis',(0.,0.,1.));
#64255=DIRECTION('center_axis',(0.,-1.,0.));
#64256=DIRECTION('ref_axis',(0.,0.,-1.));
#64257=DIRECTION('center_axis',(0.,1.,0.));
#64258=DIRECTION('ref_axis',(0.,0.,1.));
#64259=DIRECTION('center_axis',(0.,-1.,0.));
#64260=DIRECTION('ref_axis',(0.,0.,-1.));
#64261=DIRECTION('center_axis',(0.,1.,0.));
#64262=DIRECTION('ref_axis',(0.,0.,1.));
#64263=DIRECTION('center_axis',(0.,-1.,0.));
#64264=DIRECTION('ref_axis',(0.,0.,-1.));
#64265=DIRECTION('center_axis',(0.,1.,0.));
#64266=DIRECTION('ref_axis',(0.,0.,1.));
#64267=DIRECTION('center_axis',(0.,-1.,0.));
#64268=DIRECTION('ref_axis',(0.,0.,-1.));
#64269=DIRECTION('center_axis',(0.,1.,0.));
#64270=DIRECTION('ref_axis',(0.,0.,1.));
#64271=DIRECTION('center_axis',(0.,-1.,0.));
#64272=DIRECTION('ref_axis',(0.,0.,-1.));
#64273=DIRECTION('center_axis',(0.,1.,0.));
#64274=DIRECTION('ref_axis',(0.,0.,1.));
#64275=DIRECTION('center_axis',(0.,-1.,0.));
#64276=DIRECTION('ref_axis',(0.,0.,-1.));
#64277=DIRECTION('center_axis',(0.,1.,0.));
#64278=DIRECTION('ref_axis',(0.,0.,1.));
#64279=DIRECTION('center_axis',(0.,-1.,0.));
#64280=DIRECTION('ref_axis',(0.,0.,-1.));
#64281=DIRECTION('center_axis',(0.,1.,0.));
#64282=DIRECTION('ref_axis',(0.,0.,1.));
#64283=DIRECTION('center_axis',(0.,-1.,0.));
#64284=DIRECTION('ref_axis',(0.,0.,-1.));
#64285=DIRECTION('center_axis',(0.,1.,0.));
#64286=DIRECTION('ref_axis',(0.,0.,1.));
#64287=DIRECTION('center_axis',(0.,-1.,0.));
#64288=DIRECTION('ref_axis',(0.,0.,-1.));
#64289=DIRECTION('center_axis',(0.,1.,0.));
#64290=DIRECTION('ref_axis',(0.,0.,1.));
#64291=DIRECTION('center_axis',(0.,-1.,0.));
#64292=DIRECTION('ref_axis',(0.,0.,-1.));
#64293=DIRECTION('center_axis',(0.,1.,0.));
#64294=DIRECTION('ref_axis',(0.,0.,1.));
#64295=DIRECTION('center_axis',(0.,-1.,0.));
#64296=DIRECTION('ref_axis',(0.,0.,-1.));
#64297=DIRECTION('center_axis',(0.,1.,0.));
#64298=DIRECTION('ref_axis',(0.,0.,1.));
#64299=DIRECTION('center_axis',(0.,-1.,0.));
#64300=DIRECTION('ref_axis',(0.,0.,-1.));
#64301=DIRECTION('center_axis',(0.,1.,0.));
#64302=DIRECTION('ref_axis',(0.,0.,1.));
#64303=DIRECTION('center_axis',(0.,-1.,0.));
#64304=DIRECTION('ref_axis',(0.,0.,-1.));
#64305=DIRECTION('center_axis',(0.,1.,0.));
#64306=DIRECTION('ref_axis',(0.,0.,1.));
#64307=DIRECTION('center_axis',(0.,-1.,0.));
#64308=DIRECTION('ref_axis',(0.,0.,-1.));
#64309=DIRECTION('center_axis',(0.,1.,0.));
#64310=DIRECTION('ref_axis',(0.,0.,1.));
#64311=DIRECTION('center_axis',(0.,-1.,0.));
#64312=DIRECTION('ref_axis',(0.,0.,-1.));
#64313=DIRECTION('center_axis',(0.,1.,0.));
#64314=DIRECTION('ref_axis',(0.,0.,1.));
#64315=DIRECTION('center_axis',(0.,-1.,0.));
#64316=DIRECTION('ref_axis',(0.,0.,-1.));
#64317=DIRECTION('center_axis',(0.,1.,0.));
#64318=DIRECTION('ref_axis',(0.,0.,1.));
#64319=DIRECTION('center_axis',(0.,-1.,0.));
#64320=DIRECTION('ref_axis',(0.,0.,-1.));
#64321=DIRECTION('center_axis',(0.,1.,0.));
#64322=DIRECTION('ref_axis',(0.,0.,1.));
#64323=DIRECTION('center_axis',(0.,-1.,0.));
#64324=DIRECTION('ref_axis',(0.,0.,-1.));
#64325=DIRECTION('center_axis',(0.,1.,0.));
#64326=DIRECTION('ref_axis',(0.,0.,1.));
#64327=DIRECTION('center_axis',(0.,-1.,0.));
#64328=DIRECTION('ref_axis',(0.,0.,-1.));
#64329=DIRECTION('center_axis',(0.,1.,0.));
#64330=DIRECTION('ref_axis',(0.,0.,1.));
#64331=DIRECTION('center_axis',(0.,-1.,0.));
#64332=DIRECTION('ref_axis',(0.,0.,-1.));
#64333=DIRECTION('center_axis',(0.,1.,0.));
#64334=DIRECTION('ref_axis',(0.,0.,1.));
#64335=DIRECTION('center_axis',(0.,-1.,0.));
#64336=DIRECTION('ref_axis',(0.,0.,-1.));
#64337=DIRECTION('center_axis',(0.,1.,0.));
#64338=DIRECTION('ref_axis',(0.,0.,1.));
#64339=DIRECTION('center_axis',(0.,-1.,0.));
#64340=DIRECTION('ref_axis',(0.,0.,-1.));
#64341=DIRECTION('center_axis',(0.,1.,0.));
#64342=DIRECTION('ref_axis',(0.,0.,1.));
#64343=DIRECTION('center_axis',(0.,-1.,0.));
#64344=DIRECTION('ref_axis',(0.,0.,-1.));
#64345=DIRECTION('center_axis',(0.,1.,0.));
#64346=DIRECTION('ref_axis',(0.,0.,1.));
#64347=DIRECTION('center_axis',(0.,-1.,0.));
#64348=DIRECTION('ref_axis',(0.,0.,-1.));
#64349=DIRECTION('center_axis',(0.,1.,0.));
#64350=DIRECTION('ref_axis',(0.,0.,1.));
#64351=DIRECTION('center_axis',(0.,-1.,0.));
#64352=DIRECTION('ref_axis',(0.,0.,-1.));
#64353=DIRECTION('center_axis',(0.,1.,0.));
#64354=DIRECTION('ref_axis',(0.,0.,1.));
#64355=DIRECTION('center_axis',(0.,-1.,0.));
#64356=DIRECTION('ref_axis',(0.,0.,-1.));
#64357=DIRECTION('center_axis',(0.,1.,0.));
#64358=DIRECTION('ref_axis',(0.,0.,1.));
#64359=DIRECTION('center_axis',(0.,-1.,0.));
#64360=DIRECTION('ref_axis',(0.,0.,-1.));
#64361=DIRECTION('center_axis',(0.,1.,0.));
#64362=DIRECTION('ref_axis',(0.,0.,1.));
#64363=DIRECTION('center_axis',(0.,-1.,0.));
#64364=DIRECTION('ref_axis',(0.,0.,-1.));
#64365=DIRECTION('center_axis',(0.,1.,0.));
#64366=DIRECTION('ref_axis',(0.,0.,1.));
#64367=DIRECTION('center_axis',(0.,-1.,0.));
#64368=DIRECTION('ref_axis',(0.,0.,-1.));
#64369=DIRECTION('center_axis',(0.,1.,0.));
#64370=DIRECTION('ref_axis',(0.,0.,1.));
#64371=DIRECTION('center_axis',(0.,-1.,0.));
#64372=DIRECTION('ref_axis',(0.,0.,-1.));
#64373=DIRECTION('center_axis',(0.,1.,0.));
#64374=DIRECTION('ref_axis',(0.,0.,1.));
#64375=DIRECTION('center_axis',(0.,-1.,0.));
#64376=DIRECTION('ref_axis',(0.,0.,-1.));
#64377=DIRECTION('center_axis',(0.,1.,0.));
#64378=DIRECTION('ref_axis',(0.,0.,1.));
#64379=DIRECTION('center_axis',(0.,-1.,0.));
#64380=DIRECTION('ref_axis',(0.,0.,-1.));
#64381=DIRECTION('center_axis',(0.,1.,0.));
#64382=DIRECTION('ref_axis',(0.,0.,1.));
#64383=DIRECTION('center_axis',(0.,-1.,0.));
#64384=DIRECTION('ref_axis',(0.,0.,-1.));
#64385=DIRECTION('center_axis',(0.,1.,0.));
#64386=DIRECTION('ref_axis',(0.,0.,1.));
#64387=DIRECTION('center_axis',(0.,-1.,0.));
#64388=DIRECTION('ref_axis',(0.,0.,-1.));
#64389=DIRECTION('center_axis',(0.,1.,0.));
#64390=DIRECTION('ref_axis',(0.,0.,1.));
#64391=DIRECTION('center_axis',(0.,-1.,0.));
#64392=DIRECTION('ref_axis',(0.,0.,-1.));
#64393=DIRECTION('center_axis',(0.,1.,0.));
#64394=DIRECTION('ref_axis',(0.,0.,1.));
#64395=DIRECTION('center_axis',(0.,-1.,0.));
#64396=DIRECTION('ref_axis',(0.,0.,-1.));
#64397=DIRECTION('center_axis',(0.,1.,0.));
#64398=DIRECTION('ref_axis',(0.,0.,1.));
#64399=DIRECTION('center_axis',(0.,-1.,0.));
#64400=DIRECTION('ref_axis',(0.,0.,-1.));
#64401=DIRECTION('center_axis',(0.,1.,0.));
#64402=DIRECTION('ref_axis',(0.,0.,1.));
#64403=DIRECTION('center_axis',(0.,-1.,0.));
#64404=DIRECTION('ref_axis',(0.,0.,-1.));
#64405=DIRECTION('center_axis',(0.,1.,0.));
#64406=DIRECTION('ref_axis',(0.,0.,1.));
#64407=DIRECTION('center_axis',(0.,-1.,0.));
#64408=DIRECTION('ref_axis',(0.,0.,-1.));
#64409=DIRECTION('center_axis',(0.,1.,0.));
#64410=DIRECTION('ref_axis',(0.,0.,1.));
#64411=DIRECTION('center_axis',(0.,-1.,0.));
#64412=DIRECTION('ref_axis',(0.,0.,-1.));
#64413=DIRECTION('center_axis',(0.,1.,0.));
#64414=DIRECTION('ref_axis',(0.,0.,1.));
#64415=DIRECTION('center_axis',(0.,-1.,0.));
#64416=DIRECTION('ref_axis',(0.,0.,-1.));
#64417=DIRECTION('center_axis',(0.,1.,0.));
#64418=DIRECTION('ref_axis',(0.,0.,1.));
#64419=DIRECTION('center_axis',(0.,-1.,0.));
#64420=DIRECTION('ref_axis',(0.,0.,-1.));
#64421=DIRECTION('center_axis',(0.,1.,0.));
#64422=DIRECTION('ref_axis',(0.,0.,1.));
#64423=DIRECTION('center_axis',(0.,-1.,0.));
#64424=DIRECTION('ref_axis',(0.,0.,-1.));
#64425=DIRECTION('center_axis',(0.,1.,0.));
#64426=DIRECTION('ref_axis',(0.,0.,1.));
#64427=DIRECTION('center_axis',(0.,-1.,0.));
#64428=DIRECTION('ref_axis',(0.,0.,-1.));
#64429=DIRECTION('center_axis',(0.,1.,0.));
#64430=DIRECTION('ref_axis',(0.,0.,1.));
#64431=DIRECTION('center_axis',(0.,-1.,0.));
#64432=DIRECTION('ref_axis',(0.,0.,-1.));
#64433=DIRECTION('center_axis',(0.,1.,0.));
#64434=DIRECTION('ref_axis',(0.,0.,1.));
#64435=DIRECTION('center_axis',(0.,-1.,0.));
#64436=DIRECTION('ref_axis',(0.,0.,-1.));
#64437=DIRECTION('center_axis',(0.,1.,0.));
#64438=DIRECTION('ref_axis',(0.,0.,1.));
#64439=DIRECTION('center_axis',(0.,-1.,0.));
#64440=DIRECTION('ref_axis',(0.,0.,-1.));
#64441=DIRECTION('center_axis',(0.,1.,0.));
#64442=DIRECTION('ref_axis',(0.,0.,1.));
#64443=DIRECTION('center_axis',(0.,-1.,0.));
#64444=DIRECTION('ref_axis',(0.,0.,-1.));
#64445=DIRECTION('center_axis',(0.,1.,0.));
#64446=DIRECTION('ref_axis',(0.,0.,1.));
#64447=DIRECTION('center_axis',(0.,-1.,0.));
#64448=DIRECTION('ref_axis',(0.,0.,-1.));
#64449=DIRECTION('center_axis',(0.,1.,0.));
#64450=DIRECTION('ref_axis',(0.,0.,1.));
#64451=DIRECTION('center_axis',(0.,-1.,0.));
#64452=DIRECTION('ref_axis',(0.,0.,-1.));
#64453=DIRECTION('center_axis',(0.,1.,0.));
#64454=DIRECTION('ref_axis',(0.,0.,1.));
#64455=DIRECTION('center_axis',(0.,-1.,0.));
#64456=DIRECTION('ref_axis',(0.,0.,-1.));
#64457=DIRECTION('center_axis',(0.,1.,0.));
#64458=DIRECTION('ref_axis',(0.,0.,1.));
#64459=DIRECTION('center_axis',(0.,-1.,0.));
#64460=DIRECTION('ref_axis',(0.,0.,-1.));
#64461=DIRECTION('center_axis',(0.,1.,0.));
#64462=DIRECTION('ref_axis',(0.,0.,1.));
#64463=DIRECTION('center_axis',(0.,-1.,0.));
#64464=DIRECTION('ref_axis',(0.,0.,-1.));
#64465=DIRECTION('center_axis',(0.,1.,0.));
#64466=DIRECTION('ref_axis',(0.,0.,1.));
#64467=DIRECTION('center_axis',(0.,-1.,0.));
#64468=DIRECTION('ref_axis',(0.,0.,-1.));
#64469=DIRECTION('center_axis',(0.,1.,0.));
#64470=DIRECTION('ref_axis',(0.,0.,1.));
#64471=DIRECTION('center_axis',(0.,-1.,0.));
#64472=DIRECTION('ref_axis',(0.,0.,-1.));
#64473=DIRECTION('center_axis',(0.,1.,0.));
#64474=DIRECTION('ref_axis',(0.,0.,1.));
#64475=DIRECTION('center_axis',(0.,-1.,0.));
#64476=DIRECTION('ref_axis',(0.,0.,-1.));
#64477=DIRECTION('center_axis',(0.,1.,0.));
#64478=DIRECTION('ref_axis',(0.,0.,1.));
#64479=DIRECTION('center_axis',(0.,-1.,0.));
#64480=DIRECTION('ref_axis',(0.,0.,-1.));
#64481=DIRECTION('center_axis',(0.,1.,0.));
#64482=DIRECTION('ref_axis',(0.,0.,1.));
#64483=DIRECTION('center_axis',(0.,-1.,0.));
#64484=DIRECTION('ref_axis',(0.,0.,-1.));
#64485=DIRECTION('center_axis',(0.,1.,0.));
#64486=DIRECTION('ref_axis',(0.,0.,1.));
#64487=DIRECTION('center_axis',(0.,-1.,0.));
#64488=DIRECTION('ref_axis',(0.,0.,-1.));
#64489=DIRECTION('center_axis',(0.,1.,0.));
#64490=DIRECTION('ref_axis',(0.,0.,1.));
#64491=DIRECTION('center_axis',(0.,-1.,0.));
#64492=DIRECTION('ref_axis',(0.,0.,-1.));
#64493=DIRECTION('center_axis',(0.,1.,0.));
#64494=DIRECTION('ref_axis',(0.,0.,1.));
#64495=DIRECTION('center_axis',(0.,-1.,0.));
#64496=DIRECTION('ref_axis',(0.,0.,-1.));
#64497=DIRECTION('center_axis',(0.,1.,0.));
#64498=DIRECTION('ref_axis',(0.,0.,1.));
#64499=DIRECTION('center_axis',(0.,-1.,0.));
#64500=DIRECTION('ref_axis',(0.,0.,-1.));
#64501=DIRECTION('center_axis',(0.,1.,0.));
#64502=DIRECTION('ref_axis',(0.,0.,1.));
#64503=DIRECTION('center_axis',(0.,-1.,0.));
#64504=DIRECTION('ref_axis',(0.,0.,-1.));
#64505=DIRECTION('center_axis',(0.,1.,0.));
#64506=DIRECTION('ref_axis',(0.,0.,1.));
#64507=DIRECTION('center_axis',(0.,-1.,0.));
#64508=DIRECTION('ref_axis',(0.,0.,-1.));
#64509=DIRECTION('center_axis',(0.,1.,0.));
#64510=DIRECTION('ref_axis',(0.,0.,1.));
#64511=DIRECTION('center_axis',(0.,-1.,0.));
#64512=DIRECTION('ref_axis',(0.,0.,-1.));
#64513=DIRECTION('center_axis',(0.,1.,0.));
#64514=DIRECTION('ref_axis',(0.,0.,1.));
#64515=DIRECTION('center_axis',(0.,-1.,0.));
#64516=DIRECTION('ref_axis',(0.,0.,-1.));
#64517=DIRECTION('center_axis',(0.,1.,0.));
#64518=DIRECTION('ref_axis',(0.,0.,1.));
#64519=DIRECTION('center_axis',(0.,-1.,0.));
#64520=DIRECTION('ref_axis',(0.,0.,-1.));
#64521=DIRECTION('center_axis',(0.,1.,0.));
#64522=DIRECTION('ref_axis',(0.,0.,1.));
#64523=DIRECTION('center_axis',(0.,-1.,0.));
#64524=DIRECTION('ref_axis',(0.,0.,-1.));
#64525=DIRECTION('center_axis',(0.,1.,0.));
#64526=DIRECTION('ref_axis',(0.,0.,1.));
#64527=DIRECTION('center_axis',(0.,-1.,0.));
#64528=DIRECTION('ref_axis',(0.,0.,-1.));
#64529=DIRECTION('center_axis',(0.,1.,0.));
#64530=DIRECTION('ref_axis',(0.,0.,1.));
#64531=DIRECTION('center_axis',(0.,-1.,0.));
#64532=DIRECTION('ref_axis',(0.,0.,-1.));
#64533=DIRECTION('center_axis',(0.,1.,0.));
#64534=DIRECTION('ref_axis',(0.,0.,1.));
#64535=DIRECTION('center_axis',(0.,-1.,0.));
#64536=DIRECTION('ref_axis',(0.,0.,-1.));
#64537=DIRECTION('center_axis',(0.,1.,0.));
#64538=DIRECTION('ref_axis',(0.,0.,1.));
#64539=DIRECTION('center_axis',(0.,-1.,0.));
#64540=DIRECTION('ref_axis',(0.,0.,-1.));
#64541=DIRECTION('center_axis',(0.,1.,0.));
#64542=DIRECTION('ref_axis',(0.,0.,1.));
#64543=DIRECTION('center_axis',(0.,-1.,0.));
#64544=DIRECTION('ref_axis',(0.,0.,-1.));
#64545=DIRECTION('center_axis',(0.,1.,0.));
#64546=DIRECTION('ref_axis',(0.,0.,1.));
#64547=DIRECTION('center_axis',(0.,-1.,0.));
#64548=DIRECTION('ref_axis',(0.,0.,-1.));
#64549=DIRECTION('center_axis',(0.,1.,0.));
#64550=DIRECTION('ref_axis',(0.,0.,1.));
#64551=DIRECTION('center_axis',(0.,-1.,0.));
#64552=DIRECTION('ref_axis',(0.,0.,-1.));
#64553=DIRECTION('center_axis',(0.,1.,0.));
#64554=DIRECTION('ref_axis',(0.,0.,1.));
#64555=DIRECTION('center_axis',(0.,-1.,0.));
#64556=DIRECTION('ref_axis',(0.,0.,-1.));
#64557=DIRECTION('center_axis',(0.,1.,0.));
#64558=DIRECTION('ref_axis',(0.,0.,1.));
#64559=DIRECTION('center_axis',(0.,-1.,0.));
#64560=DIRECTION('ref_axis',(0.,0.,-1.));
#64561=DIRECTION('center_axis',(0.,1.,0.));
#64562=DIRECTION('ref_axis',(0.,0.,1.));
#64563=DIRECTION('center_axis',(0.,-1.,0.));
#64564=DIRECTION('ref_axis',(0.,0.,-1.));
#64565=DIRECTION('center_axis',(0.,1.,0.));
#64566=DIRECTION('ref_axis',(0.,0.,1.));
#64567=DIRECTION('center_axis',(0.,-1.,0.));
#64568=DIRECTION('ref_axis',(0.,0.,-1.));
#64569=DIRECTION('center_axis',(0.,1.,0.));
#64570=DIRECTION('ref_axis',(0.,0.,1.));
#64571=DIRECTION('center_axis',(0.,-1.,0.));
#64572=DIRECTION('ref_axis',(0.,0.,-1.));
#64573=DIRECTION('center_axis',(0.,1.,0.));
#64574=DIRECTION('ref_axis',(0.,0.,1.));
#64575=DIRECTION('center_axis',(0.,-1.,0.));
#64576=DIRECTION('ref_axis',(0.,0.,-1.));
#64577=DIRECTION('center_axis',(0.,1.,0.));
#64578=DIRECTION('ref_axis',(0.,0.,1.));
#64579=DIRECTION('center_axis',(0.,-1.,0.));
#64580=DIRECTION('ref_axis',(0.,0.,-1.));
#64581=DIRECTION('center_axis',(0.,1.,0.));
#64582=DIRECTION('ref_axis',(0.,0.,1.));
#64583=DIRECTION('center_axis',(0.,-1.,0.));
#64584=DIRECTION('ref_axis',(0.,0.,-1.));
#64585=DIRECTION('center_axis',(0.,1.,0.));
#64586=DIRECTION('ref_axis',(0.,0.,1.));
#64587=DIRECTION('center_axis',(0.,-1.,0.));
#64588=DIRECTION('ref_axis',(0.,0.,-1.));
#64589=DIRECTION('center_axis',(0.,1.,0.));
#64590=DIRECTION('ref_axis',(0.,0.,1.));
#64591=DIRECTION('center_axis',(0.,-1.,0.));
#64592=DIRECTION('ref_axis',(0.,0.,-1.));
#64593=DIRECTION('center_axis',(0.,1.,0.));
#64594=DIRECTION('ref_axis',(0.,0.,1.));
#64595=DIRECTION('center_axis',(0.,-1.,0.));
#64596=DIRECTION('ref_axis',(0.,0.,-1.));
#64597=DIRECTION('center_axis',(0.,1.,0.));
#64598=DIRECTION('ref_axis',(0.,0.,1.));
#64599=DIRECTION('center_axis',(0.,-1.,0.));
#64600=DIRECTION('ref_axis',(0.,0.,-1.));
#64601=DIRECTION('center_axis',(0.,1.,0.));
#64602=DIRECTION('ref_axis',(0.,0.,1.));
#64603=DIRECTION('center_axis',(0.,-1.,0.));
#64604=DIRECTION('ref_axis',(0.,0.,-1.));
#64605=DIRECTION('center_axis',(0.,1.,0.));
#64606=DIRECTION('ref_axis',(0.,0.,1.));
#64607=DIRECTION('center_axis',(0.,-1.,0.));
#64608=DIRECTION('ref_axis',(0.,0.,-1.));
#64609=DIRECTION('center_axis',(0.,1.,0.));
#64610=DIRECTION('ref_axis',(0.,0.,1.));
#64611=DIRECTION('center_axis',(0.,-1.,0.));
#64612=DIRECTION('ref_axis',(0.,0.,-1.));
#64613=DIRECTION('center_axis',(0.,1.,0.));
#64614=DIRECTION('ref_axis',(0.,0.,1.));
#64615=DIRECTION('center_axis',(0.,-1.,0.));
#64616=DIRECTION('ref_axis',(0.,0.,-1.));
#64617=DIRECTION('center_axis',(0.,1.,0.));
#64618=DIRECTION('ref_axis',(0.,0.,1.));
#64619=DIRECTION('center_axis',(0.,-1.,0.));
#64620=DIRECTION('ref_axis',(0.,0.,-1.));
#64621=DIRECTION('center_axis',(0.,1.,0.));
#64622=DIRECTION('ref_axis',(0.,0.,1.));
#64623=DIRECTION('center_axis',(0.,-1.,0.));
#64624=DIRECTION('ref_axis',(0.,0.,-1.));
#64625=DIRECTION('center_axis',(0.,1.,0.));
#64626=DIRECTION('ref_axis',(0.,0.,1.));
#64627=DIRECTION('center_axis',(0.,-1.,0.));
#64628=DIRECTION('ref_axis',(0.,0.,-1.));
#64629=DIRECTION('center_axis',(0.,1.,0.));
#64630=DIRECTION('ref_axis',(0.,0.,1.));
#64631=DIRECTION('center_axis',(0.,-1.,0.));
#64632=DIRECTION('ref_axis',(0.,0.,-1.));
#64633=DIRECTION('center_axis',(0.,1.,0.));
#64634=DIRECTION('ref_axis',(0.,0.,1.));
#64635=DIRECTION('center_axis',(0.,-1.,0.));
#64636=DIRECTION('ref_axis',(0.,0.,-1.));
#64637=DIRECTION('center_axis',(0.,1.,0.));
#64638=DIRECTION('ref_axis',(0.,0.,1.));
#64639=DIRECTION('center_axis',(0.,-1.,0.));
#64640=DIRECTION('ref_axis',(0.,0.,-1.));
#64641=DIRECTION('center_axis',(0.,1.,0.));
#64642=DIRECTION('ref_axis',(0.,0.,1.));
#64643=DIRECTION('center_axis',(0.,-1.,0.));
#64644=DIRECTION('ref_axis',(0.,0.,-1.));
#64645=DIRECTION('center_axis',(0.,1.,0.));
#64646=DIRECTION('ref_axis',(0.,0.,1.));
#64647=DIRECTION('center_axis',(0.,-1.,0.));
#64648=DIRECTION('ref_axis',(0.,0.,-1.));
#64649=DIRECTION('center_axis',(0.,1.,0.));
#64650=DIRECTION('ref_axis',(0.,0.,1.));
#64651=DIRECTION('center_axis',(0.,-1.,0.));
#64652=DIRECTION('ref_axis',(0.,0.,-1.));
#64653=DIRECTION('center_axis',(0.,1.,0.));
#64654=DIRECTION('ref_axis',(0.,0.,1.));
#64655=DIRECTION('center_axis',(0.,-1.,0.));
#64656=DIRECTION('ref_axis',(0.,0.,-1.));
#64657=DIRECTION('center_axis',(0.,1.,0.));
#64658=DIRECTION('ref_axis',(0.,0.,1.));
#64659=DIRECTION('center_axis',(0.,-1.,0.));
#64660=DIRECTION('ref_axis',(0.,0.,-1.));
#64661=DIRECTION('center_axis',(0.,1.,0.));
#64662=DIRECTION('ref_axis',(0.,0.,1.));
#64663=DIRECTION('center_axis',(0.,-1.,0.));
#64664=DIRECTION('ref_axis',(0.,0.,-1.));
#64665=DIRECTION('center_axis',(0.,1.,0.));
#64666=DIRECTION('ref_axis',(0.,0.,1.));
#64667=DIRECTION('center_axis',(0.,-1.,0.));
#64668=DIRECTION('ref_axis',(0.,0.,-1.));
#64669=DIRECTION('center_axis',(0.,1.,0.));
#64670=DIRECTION('ref_axis',(0.,0.,1.));
#64671=DIRECTION('center_axis',(0.,-1.,0.));
#64672=DIRECTION('ref_axis',(0.,0.,-1.));
#64673=DIRECTION('center_axis',(0.,1.,0.));
#64674=DIRECTION('ref_axis',(0.,0.,1.));
#64675=DIRECTION('center_axis',(0.,-1.,0.));
#64676=DIRECTION('ref_axis',(0.,0.,-1.));
#64677=DIRECTION('center_axis',(0.,1.,0.));
#64678=DIRECTION('ref_axis',(0.,0.,1.));
#64679=DIRECTION('center_axis',(0.,-1.,0.));
#64680=DIRECTION('ref_axis',(0.,0.,-1.));
#64681=DIRECTION('center_axis',(0.,1.,0.));
#64682=DIRECTION('ref_axis',(0.,0.,1.));
#64683=DIRECTION('center_axis',(0.,-1.,0.));
#64684=DIRECTION('ref_axis',(0.,0.,-1.));
#64685=DIRECTION('center_axis',(0.,1.,0.));
#64686=DIRECTION('ref_axis',(0.,0.,1.));
#64687=DIRECTION('center_axis',(0.,-1.,0.));
#64688=DIRECTION('ref_axis',(0.,0.,-1.));
#64689=DIRECTION('center_axis',(0.,1.,0.));
#64690=DIRECTION('ref_axis',(0.,0.,1.));
#64691=DIRECTION('center_axis',(0.,-1.,0.));
#64692=DIRECTION('ref_axis',(0.,0.,-1.));
#64693=DIRECTION('center_axis',(0.,1.,0.));
#64694=DIRECTION('ref_axis',(0.,0.,1.));
#64695=DIRECTION('center_axis',(0.,-1.,0.));
#64696=DIRECTION('ref_axis',(0.,0.,-1.));
#64697=DIRECTION('center_axis',(0.,1.,0.));
#64698=DIRECTION('ref_axis',(0.,0.,1.));
#64699=DIRECTION('center_axis',(0.,-1.,0.));
#64700=DIRECTION('ref_axis',(0.,0.,-1.));
#64701=DIRECTION('center_axis',(0.,1.,0.));
#64702=DIRECTION('ref_axis',(0.,0.,1.));
#64703=DIRECTION('center_axis',(0.,-1.,0.));
#64704=DIRECTION('ref_axis',(0.,0.,-1.));
#64705=DIRECTION('center_axis',(0.,1.,0.));
#64706=DIRECTION('ref_axis',(0.,0.,1.));
#64707=DIRECTION('center_axis',(0.,-1.,0.));
#64708=DIRECTION('ref_axis',(0.,0.,-1.));
#64709=DIRECTION('center_axis',(0.,1.,0.));
#64710=DIRECTION('ref_axis',(0.,0.,1.));
#64711=DIRECTION('center_axis',(0.,-1.,0.));
#64712=DIRECTION('ref_axis',(0.,0.,-1.));
#64713=DIRECTION('center_axis',(0.,1.,0.));
#64714=DIRECTION('ref_axis',(0.,0.,1.));
#64715=DIRECTION('center_axis',(0.,-1.,0.));
#64716=DIRECTION('ref_axis',(0.,0.,-1.));
#64717=DIRECTION('center_axis',(0.,1.,0.));
#64718=DIRECTION('ref_axis',(0.,0.,1.));
#64719=DIRECTION('center_axis',(0.,-1.,0.));
#64720=DIRECTION('ref_axis',(0.,0.,-1.));
#64721=DIRECTION('center_axis',(0.,1.,0.));
#64722=DIRECTION('ref_axis',(0.,0.,1.));
#64723=DIRECTION('center_axis',(0.,-1.,0.));
#64724=DIRECTION('ref_axis',(0.,0.,-1.));
#64725=DIRECTION('center_axis',(0.,1.,0.));
#64726=DIRECTION('ref_axis',(0.,0.,1.));
#64727=DIRECTION('center_axis',(0.,-1.,0.));
#64728=DIRECTION('ref_axis',(0.,0.,-1.));
#64729=DIRECTION('center_axis',(0.,1.,0.));
#64730=DIRECTION('ref_axis',(0.,0.,1.));
#64731=DIRECTION('center_axis',(0.,-1.,0.));
#64732=DIRECTION('ref_axis',(0.,0.,-1.));
#64733=DIRECTION('center_axis',(0.,1.,0.));
#64734=DIRECTION('ref_axis',(0.,0.,1.));
#64735=DIRECTION('center_axis',(0.,-1.,0.));
#64736=DIRECTION('ref_axis',(0.,0.,-1.));
#64737=DIRECTION('center_axis',(0.,1.,0.));
#64738=DIRECTION('ref_axis',(0.,0.,1.));
#64739=DIRECTION('center_axis',(0.,-1.,0.));
#64740=DIRECTION('ref_axis',(0.,0.,-1.));
#64741=DIRECTION('center_axis',(0.,1.,0.));
#64742=DIRECTION('ref_axis',(0.,0.,1.));
#64743=DIRECTION('center_axis',(0.,-1.,0.));
#64744=DIRECTION('ref_axis',(0.,0.,-1.));
#64745=DIRECTION('center_axis',(0.,1.,0.));
#64746=DIRECTION('ref_axis',(0.,0.,1.));
#64747=DIRECTION('center_axis',(0.,-1.,0.));
#64748=DIRECTION('ref_axis',(0.,0.,-1.));
#64749=DIRECTION('center_axis',(0.,1.,0.));
#64750=DIRECTION('ref_axis',(0.,0.,1.));
#64751=DIRECTION('center_axis',(0.,-1.,0.));
#64752=DIRECTION('ref_axis',(0.,0.,-1.));
#64753=DIRECTION('center_axis',(0.,1.,0.));
#64754=DIRECTION('ref_axis',(0.,0.,1.));
#64755=DIRECTION('center_axis',(0.,-1.,0.));
#64756=DIRECTION('ref_axis',(0.,0.,-1.));
#64757=DIRECTION('center_axis',(0.,1.,0.));
#64758=DIRECTION('ref_axis',(0.,0.,1.));
#64759=DIRECTION('center_axis',(0.,-1.,0.));
#64760=DIRECTION('ref_axis',(0.,0.,-1.));
#64761=DIRECTION('center_axis',(0.,1.,0.));
#64762=DIRECTION('ref_axis',(0.,0.,1.));
#64763=DIRECTION('center_axis',(0.,-1.,0.));
#64764=DIRECTION('ref_axis',(0.,0.,-1.));
#64765=DIRECTION('center_axis',(0.,1.,0.));
#64766=DIRECTION('ref_axis',(0.,0.,1.));
#64767=DIRECTION('center_axis',(0.,-1.,0.));
#64768=DIRECTION('ref_axis',(0.,0.,-1.));
#64769=DIRECTION('center_axis',(0.,1.,0.));
#64770=DIRECTION('ref_axis',(0.,0.,1.));
#64771=DIRECTION('center_axis',(0.,-1.,0.));
#64772=DIRECTION('ref_axis',(0.,0.,-1.));
#64773=DIRECTION('center_axis',(0.,1.,0.));
#64774=DIRECTION('ref_axis',(0.,0.,1.));
#64775=DIRECTION('center_axis',(0.,-1.,0.));
#64776=DIRECTION('ref_axis',(0.,0.,-1.));
#64777=DIRECTION('center_axis',(0.,1.,0.));
#64778=DIRECTION('ref_axis',(0.,0.,1.));
#64779=DIRECTION('center_axis',(0.,-1.,0.));
#64780=DIRECTION('ref_axis',(0.,0.,-1.));
#64781=DIRECTION('center_axis',(0.,1.,0.));
#64782=DIRECTION('ref_axis',(0.,0.,1.));
#64783=DIRECTION('center_axis',(0.,-1.,0.));
#64784=DIRECTION('ref_axis',(0.,0.,-1.));
#64785=DIRECTION('center_axis',(0.,1.,0.));
#64786=DIRECTION('ref_axis',(0.,0.,1.));
#64787=DIRECTION('center_axis',(0.,-1.,0.));
#64788=DIRECTION('ref_axis',(0.,0.,-1.));
#64789=DIRECTION('center_axis',(0.,1.,0.));
#64790=DIRECTION('ref_axis',(0.,0.,1.));
#64791=DIRECTION('center_axis',(0.,-1.,0.));
#64792=DIRECTION('ref_axis',(0.,0.,-1.));
#64793=DIRECTION('center_axis',(0.,1.,0.));
#64794=DIRECTION('ref_axis',(0.,0.,1.));
#64795=DIRECTION('center_axis',(0.,-1.,0.));
#64796=DIRECTION('ref_axis',(0.,0.,-1.));
#64797=DIRECTION('center_axis',(0.,1.,0.));
#64798=DIRECTION('ref_axis',(0.,0.,1.));
#64799=DIRECTION('center_axis',(0.,-1.,0.));
#64800=DIRECTION('ref_axis',(0.,0.,-1.));
#64801=DIRECTION('center_axis',(0.,1.,0.));
#64802=DIRECTION('ref_axis',(0.,0.,1.));
#64803=DIRECTION('center_axis',(0.,-1.,0.));
#64804=DIRECTION('ref_axis',(0.,0.,-1.));
#64805=DIRECTION('center_axis',(0.,1.,0.));
#64806=DIRECTION('ref_axis',(0.,0.,1.));
#64807=DIRECTION('center_axis',(0.,-1.,0.));
#64808=DIRECTION('ref_axis',(0.,0.,-1.));
#64809=DIRECTION('center_axis',(0.,1.,0.));
#64810=DIRECTION('ref_axis',(0.,0.,1.));
#64811=DIRECTION('center_axis',(0.,-1.,0.));
#64812=DIRECTION('ref_axis',(0.,0.,-1.));
#64813=DIRECTION('center_axis',(0.,1.,0.));
#64814=DIRECTION('ref_axis',(0.,0.,1.));
#64815=DIRECTION('center_axis',(0.,-1.,0.));
#64816=DIRECTION('ref_axis',(0.,0.,-1.));
#64817=DIRECTION('center_axis',(0.,1.,0.));
#64818=DIRECTION('ref_axis',(0.,0.,1.));
#64819=DIRECTION('center_axis',(0.,-1.,0.));
#64820=DIRECTION('ref_axis',(0.,0.,-1.));
#64821=DIRECTION('center_axis',(0.,1.,0.));
#64822=DIRECTION('ref_axis',(0.,0.,1.));
#64823=DIRECTION('center_axis',(0.,-1.,0.));
#64824=DIRECTION('ref_axis',(0.,0.,-1.));
#64825=DIRECTION('center_axis',(0.,1.,0.));
#64826=DIRECTION('ref_axis',(0.,0.,1.));
#64827=DIRECTION('center_axis',(0.,-1.,0.));
#64828=DIRECTION('ref_axis',(0.,0.,-1.));
#64829=DIRECTION('center_axis',(0.,1.,0.));
#64830=DIRECTION('ref_axis',(0.,0.,1.));
#64831=DIRECTION('center_axis',(0.,-1.,0.));
#64832=DIRECTION('ref_axis',(0.,0.,-1.));
#64833=DIRECTION('center_axis',(0.,1.,0.));
#64834=DIRECTION('ref_axis',(0.,0.,1.));
#64835=DIRECTION('center_axis',(0.,-1.,0.));
#64836=DIRECTION('ref_axis',(0.,0.,-1.));
#64837=DIRECTION('center_axis',(0.,1.,0.));
#64838=DIRECTION('ref_axis',(0.,0.,1.));
#64839=DIRECTION('center_axis',(0.,-1.,0.));
#64840=DIRECTION('ref_axis',(0.,0.,-1.));
#64841=DIRECTION('center_axis',(0.,1.,0.));
#64842=DIRECTION('ref_axis',(0.,0.,1.));
#64843=DIRECTION('center_axis',(0.,-1.,0.));
#64844=DIRECTION('ref_axis',(0.,0.,-1.));
#64845=DIRECTION('center_axis',(0.,1.,0.));
#64846=DIRECTION('ref_axis',(0.,0.,1.));
#64847=DIRECTION('center_axis',(0.,-1.,0.));
#64848=DIRECTION('ref_axis',(0.,0.,-1.));
#64849=DIRECTION('center_axis',(0.,1.,0.));
#64850=DIRECTION('ref_axis',(0.,0.,1.));
#64851=DIRECTION('center_axis',(0.,-1.,0.));
#64852=DIRECTION('ref_axis',(0.,0.,-1.));
#64853=DIRECTION('center_axis',(0.,1.,0.));
#64854=DIRECTION('ref_axis',(0.,0.,1.));
#64855=DIRECTION('center_axis',(0.,-1.,0.));
#64856=DIRECTION('ref_axis',(0.,0.,-1.));
#64857=DIRECTION('center_axis',(0.,1.,0.));
#64858=DIRECTION('ref_axis',(0.,0.,1.));
#64859=DIRECTION('center_axis',(0.,-1.,0.));
#64860=DIRECTION('ref_axis',(0.,0.,-1.));
#64861=DIRECTION('center_axis',(0.,1.,0.));
#64862=DIRECTION('ref_axis',(0.,0.,1.));
#64863=DIRECTION('center_axis',(0.,-1.,0.));
#64864=DIRECTION('ref_axis',(0.,0.,-1.));
#64865=DIRECTION('center_axis',(0.,1.,0.));
#64866=DIRECTION('ref_axis',(0.,0.,1.));
#64867=DIRECTION('center_axis',(0.,-1.,0.));
#64868=DIRECTION('ref_axis',(0.,0.,-1.));
#64869=DIRECTION('center_axis',(0.,1.,0.));
#64870=DIRECTION('ref_axis',(0.,0.,1.));
#64871=DIRECTION('center_axis',(0.,-1.,0.));
#64872=DIRECTION('ref_axis',(0.,0.,-1.));
#64873=DIRECTION('center_axis',(0.,1.,0.));
#64874=DIRECTION('ref_axis',(0.,0.,1.));
#64875=DIRECTION('center_axis',(0.,-1.,0.));
#64876=DIRECTION('ref_axis',(0.,0.,-1.));
#64877=DIRECTION('center_axis',(0.,1.,0.));
#64878=DIRECTION('ref_axis',(0.,0.,1.));
#64879=DIRECTION('center_axis',(0.,-1.,0.));
#64880=DIRECTION('ref_axis',(0.,0.,-1.));
#64881=DIRECTION('center_axis',(0.,1.,0.));
#64882=DIRECTION('ref_axis',(0.,0.,1.));
#64883=DIRECTION('center_axis',(0.,-1.,0.));
#64884=DIRECTION('ref_axis',(0.,0.,-1.));
#64885=DIRECTION('center_axis',(0.,1.,0.));
#64886=DIRECTION('ref_axis',(0.,0.,1.));
#64887=DIRECTION('center_axis',(0.,-1.,0.));
#64888=DIRECTION('ref_axis',(0.,0.,-1.));
#64889=DIRECTION('center_axis',(0.,1.,0.));
#64890=DIRECTION('ref_axis',(0.,0.,1.));
#64891=DIRECTION('center_axis',(0.,-1.,0.));
#64892=DIRECTION('ref_axis',(0.,0.,-1.));
#64893=DIRECTION('center_axis',(0.,1.,0.));
#64894=DIRECTION('ref_axis',(0.,0.,1.));
#64895=DIRECTION('center_axis',(0.,-1.,0.));
#64896=DIRECTION('ref_axis',(0.,0.,-1.));
#64897=DIRECTION('center_axis',(0.,1.,0.));
#64898=DIRECTION('ref_axis',(0.,0.,1.));
#64899=DIRECTION('center_axis',(0.,-1.,0.));
#64900=DIRECTION('ref_axis',(0.,0.,-1.));
#64901=DIRECTION('center_axis',(0.,1.,0.));
#64902=DIRECTION('ref_axis',(0.,0.,1.));
#64903=DIRECTION('center_axis',(0.,-1.,0.));
#64904=DIRECTION('ref_axis',(0.,0.,-1.));
#64905=DIRECTION('center_axis',(0.,1.,0.));
#64906=DIRECTION('ref_axis',(0.,0.,1.));
#64907=DIRECTION('center_axis',(0.,-1.,0.));
#64908=DIRECTION('ref_axis',(0.,0.,-1.));
#64909=DIRECTION('center_axis',(0.,1.,0.));
#64910=DIRECTION('ref_axis',(0.,0.,1.));
#64911=DIRECTION('center_axis',(0.,-1.,0.));
#64912=DIRECTION('ref_axis',(0.,0.,-1.));
#64913=DIRECTION('center_axis',(0.,1.,0.));
#64914=DIRECTION('ref_axis',(0.,0.,1.));
#64915=DIRECTION('center_axis',(0.,-1.,0.));
#64916=DIRECTION('ref_axis',(0.,0.,-1.));
#64917=DIRECTION('center_axis',(0.,1.,0.));
#64918=DIRECTION('ref_axis',(0.,0.,1.));
#64919=DIRECTION('center_axis',(0.,-1.,0.));
#64920=DIRECTION('ref_axis',(0.,0.,-1.));
#64921=DIRECTION('center_axis',(0.,1.,0.));
#64922=DIRECTION('ref_axis',(0.,0.,1.));
#64923=DIRECTION('center_axis',(0.,-1.,0.));
#64924=DIRECTION('ref_axis',(0.,0.,-1.));
#64925=DIRECTION('center_axis',(0.,1.,0.));
#64926=DIRECTION('ref_axis',(0.,0.,1.));
#64927=DIRECTION('center_axis',(0.,-1.,0.));
#64928=DIRECTION('ref_axis',(0.,0.,-1.));
#64929=DIRECTION('center_axis',(0.,1.,0.));
#64930=DIRECTION('ref_axis',(0.,0.,1.));
#64931=DIRECTION('center_axis',(0.,-1.,0.));
#64932=DIRECTION('ref_axis',(0.,0.,-1.));
#64933=DIRECTION('center_axis',(0.,1.,0.));
#64934=DIRECTION('ref_axis',(0.,0.,1.));
#64935=DIRECTION('center_axis',(0.,-1.,0.));
#64936=DIRECTION('ref_axis',(0.,0.,-1.));
#64937=DIRECTION('center_axis',(0.,1.,0.));
#64938=DIRECTION('ref_axis',(0.,0.,1.));
#64939=DIRECTION('center_axis',(0.,-1.,0.));
#64940=DIRECTION('ref_axis',(0.,0.,-1.));
#64941=DIRECTION('center_axis',(0.,1.,0.));
#64942=DIRECTION('ref_axis',(0.,0.,1.));
#64943=DIRECTION('center_axis',(0.,-1.,0.));
#64944=DIRECTION('ref_axis',(0.,0.,-1.));
#64945=DIRECTION('center_axis',(0.,1.,0.));
#64946=DIRECTION('ref_axis',(0.,0.,1.));
#64947=DIRECTION('center_axis',(0.,-1.,0.));
#64948=DIRECTION('ref_axis',(0.,0.,-1.));
#64949=DIRECTION('center_axis',(0.,1.,0.));
#64950=DIRECTION('ref_axis',(0.,0.,1.));
#64951=DIRECTION('center_axis',(0.,-1.,0.));
#64952=DIRECTION('ref_axis',(0.,0.,-1.));
#64953=DIRECTION('center_axis',(0.,1.,0.));
#64954=DIRECTION('ref_axis',(0.,0.,1.));
#64955=DIRECTION('center_axis',(0.,-1.,0.));
#64956=DIRECTION('ref_axis',(0.,0.,-1.));
#64957=DIRECTION('center_axis',(0.,1.,0.));
#64958=DIRECTION('ref_axis',(0.,0.,1.));
#64959=DIRECTION('center_axis',(0.,-1.,0.));
#64960=DIRECTION('ref_axis',(0.,0.,-1.));
#64961=DIRECTION('center_axis',(0.,1.,0.));
#64962=DIRECTION('ref_axis',(0.,0.,1.));
#64963=DIRECTION('center_axis',(0.,-1.,0.));
#64964=DIRECTION('ref_axis',(0.,0.,-1.));
#64965=DIRECTION('center_axis',(0.,1.,0.));
#64966=DIRECTION('ref_axis',(0.,0.,1.));
#64967=DIRECTION('center_axis',(0.,-1.,0.));
#64968=DIRECTION('ref_axis',(0.,0.,-1.));
#64969=DIRECTION('center_axis',(0.,1.,0.));
#64970=DIRECTION('ref_axis',(0.,0.,1.));
#64971=DIRECTION('center_axis',(0.,-1.,0.));
#64972=DIRECTION('ref_axis',(0.,0.,-1.));
#64973=DIRECTION('center_axis',(0.,1.,0.));
#64974=DIRECTION('ref_axis',(0.,0.,1.));
#64975=DIRECTION('center_axis',(0.,-1.,0.));
#64976=DIRECTION('ref_axis',(0.,0.,-1.));
#64977=DIRECTION('center_axis',(0.,1.,0.));
#64978=DIRECTION('ref_axis',(0.,0.,1.));
#64979=DIRECTION('center_axis',(0.,-1.,0.));
#64980=DIRECTION('ref_axis',(0.,0.,-1.));
#64981=DIRECTION('center_axis',(0.,1.,0.));
#64982=DIRECTION('ref_axis',(0.,0.,1.));
#64983=DIRECTION('center_axis',(0.,-1.,0.));
#64984=DIRECTION('ref_axis',(0.,0.,-1.));
#64985=DIRECTION('center_axis',(0.,1.,0.));
#64986=DIRECTION('ref_axis',(0.,0.,1.));
#64987=DIRECTION('center_axis',(0.,-1.,0.));
#64988=DIRECTION('ref_axis',(0.,0.,-1.));
#64989=DIRECTION('center_axis',(0.,1.,0.));
#64990=DIRECTION('ref_axis',(0.,0.,1.));
#64991=DIRECTION('center_axis',(0.,-1.,0.));
#64992=DIRECTION('ref_axis',(0.,0.,-1.));
#64993=DIRECTION('center_axis',(0.,1.,0.));
#64994=DIRECTION('ref_axis',(0.,0.,1.));
#64995=DIRECTION('center_axis',(0.,-1.,0.));
#64996=DIRECTION('ref_axis',(0.,0.,-1.));
#64997=DIRECTION('center_axis',(0.,1.,0.));
#64998=DIRECTION('ref_axis',(0.,0.,1.));
#64999=DIRECTION('center_axis',(0.,-1.,0.));
#65000=DIRECTION('ref_axis',(0.,0.,-1.));
#65001=DIRECTION('center_axis',(0.,1.,0.));
#65002=DIRECTION('ref_axis',(0.,0.,1.));
#65003=DIRECTION('center_axis',(0.,-1.,0.));
#65004=DIRECTION('ref_axis',(0.,0.,-1.));
#65005=DIRECTION('center_axis',(0.,1.,0.));
#65006=DIRECTION('ref_axis',(0.,0.,1.));
#65007=DIRECTION('center_axis',(0.,-1.,0.));
#65008=DIRECTION('ref_axis',(0.,0.,-1.));
#65009=DIRECTION('center_axis',(0.,1.,0.));
#65010=DIRECTION('ref_axis',(0.,0.,1.));
#65011=DIRECTION('center_axis',(0.,-1.,0.));
#65012=DIRECTION('ref_axis',(0.,0.,-1.));
#65013=DIRECTION('center_axis',(0.,1.,0.));
#65014=DIRECTION('ref_axis',(0.,0.,1.));
#65015=DIRECTION('center_axis',(0.,-1.,0.));
#65016=DIRECTION('ref_axis',(0.,0.,-1.));
#65017=DIRECTION('center_axis',(0.,1.,0.));
#65018=DIRECTION('ref_axis',(0.,0.,1.));
#65019=DIRECTION('center_axis',(0.,-1.,0.));
#65020=DIRECTION('ref_axis',(0.,0.,-1.));
#65021=DIRECTION('center_axis',(0.,1.,0.));
#65022=DIRECTION('ref_axis',(0.,0.,1.));
#65023=DIRECTION('center_axis',(0.,-1.,0.));
#65024=DIRECTION('ref_axis',(0.,0.,-1.));
#65025=DIRECTION('center_axis',(0.,1.,0.));
#65026=DIRECTION('ref_axis',(0.,0.,1.));
#65027=DIRECTION('center_axis',(0.,-1.,0.));
#65028=DIRECTION('ref_axis',(0.,0.,-1.));
#65029=DIRECTION('center_axis',(0.,1.,0.));
#65030=DIRECTION('ref_axis',(0.,0.,1.));
#65031=DIRECTION('center_axis',(0.,-1.,0.));
#65032=DIRECTION('ref_axis',(0.,0.,-1.));
#65033=DIRECTION('center_axis',(0.,1.,0.));
#65034=DIRECTION('ref_axis',(0.,0.,1.));
#65035=DIRECTION('center_axis',(0.,-1.,0.));
#65036=DIRECTION('ref_axis',(0.,0.,-1.));
#65037=DIRECTION('center_axis',(0.,1.,0.));
#65038=DIRECTION('ref_axis',(0.,0.,1.));
#65039=DIRECTION('center_axis',(0.,-1.,0.));
#65040=DIRECTION('ref_axis',(0.,0.,-1.));
#65041=DIRECTION('center_axis',(0.,1.,0.));
#65042=DIRECTION('ref_axis',(0.,0.,1.));
#65043=DIRECTION('center_axis',(0.,-1.,0.));
#65044=DIRECTION('ref_axis',(0.,0.,-1.));
#65045=DIRECTION('center_axis',(0.,1.,0.));
#65046=DIRECTION('ref_axis',(0.,0.,1.));
#65047=DIRECTION('center_axis',(0.,-1.,0.));
#65048=DIRECTION('ref_axis',(0.,0.,-1.));
#65049=DIRECTION('center_axis',(0.,1.,0.));
#65050=DIRECTION('ref_axis',(0.,0.,1.));
#65051=DIRECTION('center_axis',(0.,-1.,0.));
#65052=DIRECTION('ref_axis',(0.,0.,-1.));
#65053=DIRECTION('center_axis',(0.,1.,0.));
#65054=DIRECTION('ref_axis',(0.,0.,1.));
#65055=DIRECTION('center_axis',(0.,-1.,0.));
#65056=DIRECTION('ref_axis',(0.,0.,-1.));
#65057=DIRECTION('center_axis',(0.,1.,0.));
#65058=DIRECTION('ref_axis',(0.,0.,1.));
#65059=DIRECTION('center_axis',(0.,-1.,0.));
#65060=DIRECTION('ref_axis',(0.,0.,-1.));
#65061=DIRECTION('center_axis',(0.,1.,0.));
#65062=DIRECTION('ref_axis',(0.,0.,1.));
#65063=DIRECTION('center_axis',(0.,-1.,0.));
#65064=DIRECTION('ref_axis',(0.,0.,-1.));
#65065=DIRECTION('center_axis',(0.,1.,0.));
#65066=DIRECTION('ref_axis',(0.,0.,1.));
#65067=DIRECTION('center_axis',(0.,-1.,0.));
#65068=DIRECTION('ref_axis',(0.,0.,-1.));
#65069=DIRECTION('center_axis',(0.,1.,0.));
#65070=DIRECTION('ref_axis',(0.,0.,1.));
#65071=DIRECTION('center_axis',(0.,-1.,0.));
#65072=DIRECTION('ref_axis',(0.,0.,-1.));
#65073=DIRECTION('center_axis',(0.,1.,0.));
#65074=DIRECTION('ref_axis',(0.,0.,1.));
#65075=DIRECTION('center_axis',(0.,-1.,0.));
#65076=DIRECTION('ref_axis',(0.,0.,-1.));
#65077=DIRECTION('center_axis',(0.,1.,0.));
#65078=DIRECTION('ref_axis',(0.,0.,1.));
#65079=DIRECTION('center_axis',(0.,-1.,0.));
#65080=DIRECTION('ref_axis',(0.,0.,-1.));
#65081=DIRECTION('center_axis',(0.,1.,0.));
#65082=DIRECTION('ref_axis',(0.,0.,1.));
#65083=DIRECTION('center_axis',(0.,-1.,0.));
#65084=DIRECTION('ref_axis',(0.,0.,-1.));
#65085=DIRECTION('center_axis',(0.,1.,0.));
#65086=DIRECTION('ref_axis',(0.,0.,1.));
#65087=DIRECTION('center_axis',(0.,-1.,0.));
#65088=DIRECTION('ref_axis',(0.,0.,-1.));
#65089=DIRECTION('center_axis',(0.,1.,0.));
#65090=DIRECTION('ref_axis',(0.,0.,1.));
#65091=DIRECTION('center_axis',(0.,-1.,0.));
#65092=DIRECTION('ref_axis',(0.,0.,-1.));
#65093=DIRECTION('center_axis',(0.,1.,0.));
#65094=DIRECTION('ref_axis',(0.,0.,1.));
#65095=DIRECTION('center_axis',(0.,-1.,0.));
#65096=DIRECTION('ref_axis',(0.,0.,-1.));
#65097=DIRECTION('center_axis',(0.,1.,0.));
#65098=DIRECTION('ref_axis',(0.,0.,1.));
#65099=DIRECTION('center_axis',(0.,-1.,0.));
#65100=DIRECTION('ref_axis',(0.,0.,-1.));
#65101=DIRECTION('center_axis',(0.,1.,0.));
#65102=DIRECTION('ref_axis',(0.,0.,1.));
#65103=DIRECTION('center_axis',(0.,-1.,0.));
#65104=DIRECTION('ref_axis',(0.,0.,-1.));
#65105=DIRECTION('center_axis',(0.,1.,0.));
#65106=DIRECTION('ref_axis',(0.,0.,1.));
#65107=DIRECTION('center_axis',(0.,-1.,0.));
#65108=DIRECTION('ref_axis',(0.,0.,-1.));
#65109=DIRECTION('center_axis',(0.,1.,0.));
#65110=DIRECTION('ref_axis',(0.,0.,1.));
#65111=DIRECTION('center_axis',(0.,-1.,0.));
#65112=DIRECTION('ref_axis',(0.,0.,-1.));
#65113=DIRECTION('center_axis',(0.,1.,0.));
#65114=DIRECTION('ref_axis',(0.,0.,1.));
#65115=DIRECTION('center_axis',(0.,-1.,0.));
#65116=DIRECTION('ref_axis',(0.,0.,-1.));
#65117=DIRECTION('center_axis',(0.,1.,0.));
#65118=DIRECTION('ref_axis',(0.,0.,1.));
#65119=DIRECTION('center_axis',(0.,-1.,0.));
#65120=DIRECTION('ref_axis',(0.,0.,-1.));
#65121=DIRECTION('center_axis',(0.,1.,0.));
#65122=DIRECTION('ref_axis',(0.,0.,1.));
#65123=DIRECTION('center_axis',(0.,-1.,0.));
#65124=DIRECTION('ref_axis',(0.,0.,-1.));
#65125=DIRECTION('center_axis',(0.,1.,0.));
#65126=DIRECTION('ref_axis',(0.,0.,1.));
#65127=DIRECTION('center_axis',(0.,-1.,0.));
#65128=DIRECTION('ref_axis',(0.,0.,-1.));
#65129=DIRECTION('center_axis',(0.,1.,0.));
#65130=DIRECTION('ref_axis',(0.,0.,1.));
#65131=DIRECTION('center_axis',(0.,-1.,0.));
#65132=DIRECTION('ref_axis',(0.,0.,-1.));
#65133=DIRECTION('center_axis',(0.,1.,0.));
#65134=DIRECTION('ref_axis',(0.,0.,1.));
#65135=DIRECTION('center_axis',(0.,-1.,0.));
#65136=DIRECTION('ref_axis',(0.,0.,-1.));
#65137=DIRECTION('center_axis',(0.,1.,0.));
#65138=DIRECTION('ref_axis',(0.,0.,1.));
#65139=DIRECTION('center_axis',(0.,-1.,0.));
#65140=DIRECTION('ref_axis',(0.,0.,-1.));
#65141=DIRECTION('center_axis',(0.,1.,0.));
#65142=DIRECTION('ref_axis',(0.,0.,1.));
#65143=DIRECTION('center_axis',(0.,-1.,0.));
#65144=DIRECTION('ref_axis',(0.,0.,-1.));
#65145=DIRECTION('center_axis',(0.,1.,0.));
#65146=DIRECTION('ref_axis',(0.,0.,1.));
#65147=DIRECTION('center_axis',(0.,-1.,0.));
#65148=DIRECTION('ref_axis',(0.,0.,-1.));
#65149=DIRECTION('center_axis',(0.,1.,0.));
#65150=DIRECTION('ref_axis',(0.,0.,1.));
#65151=DIRECTION('center_axis',(0.,-1.,0.));
#65152=DIRECTION('ref_axis',(0.,0.,-1.));
#65153=DIRECTION('center_axis',(0.,1.,0.));
#65154=DIRECTION('ref_axis',(0.,0.,1.));
#65155=DIRECTION('center_axis',(0.,-1.,0.));
#65156=DIRECTION('ref_axis',(0.,0.,-1.));
#65157=DIRECTION('center_axis',(0.,1.,0.));
#65158=DIRECTION('ref_axis',(0.,0.,1.));
#65159=DIRECTION('center_axis',(0.,-1.,0.));
#65160=DIRECTION('ref_axis',(0.,0.,-1.));
#65161=DIRECTION('center_axis',(0.,1.,0.));
#65162=DIRECTION('ref_axis',(0.,0.,1.));
#65163=DIRECTION('center_axis',(0.,-1.,0.));
#65164=DIRECTION('ref_axis',(0.,0.,-1.));
#65165=DIRECTION('center_axis',(0.,1.,0.));
#65166=DIRECTION('ref_axis',(0.,0.,1.));
#65167=DIRECTION('center_axis',(0.,-1.,0.));
#65168=DIRECTION('ref_axis',(0.,0.,-1.));
#65169=DIRECTION('center_axis',(0.,1.,0.));
#65170=DIRECTION('ref_axis',(0.,0.,1.));
#65171=DIRECTION('center_axis',(0.,-1.,0.));
#65172=DIRECTION('ref_axis',(0.,0.,-1.));
#65173=DIRECTION('center_axis',(0.,1.,0.));
#65174=DIRECTION('ref_axis',(0.,0.,1.));
#65175=DIRECTION('center_axis',(0.,-1.,0.));
#65176=DIRECTION('ref_axis',(0.,0.,-1.));
#65177=DIRECTION('center_axis',(0.,1.,0.));
#65178=DIRECTION('ref_axis',(0.,0.,1.));
#65179=DIRECTION('center_axis',(0.,-1.,0.));
#65180=DIRECTION('ref_axis',(0.,0.,-1.));
#65181=DIRECTION('center_axis',(0.,1.,0.));
#65182=DIRECTION('ref_axis',(0.,0.,1.));
#65183=DIRECTION('center_axis',(0.,-1.,0.));
#65184=DIRECTION('ref_axis',(0.,0.,-1.));
#65185=DIRECTION('center_axis',(0.,1.,0.));
#65186=DIRECTION('ref_axis',(0.,0.,1.));
#65187=DIRECTION('center_axis',(0.,-1.,0.));
#65188=DIRECTION('ref_axis',(0.,0.,-1.));
#65189=DIRECTION('center_axis',(0.,1.,0.));
#65190=DIRECTION('ref_axis',(0.,0.,1.));
#65191=DIRECTION('center_axis',(0.,-1.,0.));
#65192=DIRECTION('ref_axis',(0.,0.,-1.));
#65193=DIRECTION('center_axis',(0.,1.,0.));
#65194=DIRECTION('ref_axis',(0.,0.,1.));
#65195=DIRECTION('center_axis',(0.,-1.,0.));
#65196=DIRECTION('ref_axis',(0.,0.,-1.));
#65197=DIRECTION('center_axis',(0.,1.,0.));
#65198=DIRECTION('ref_axis',(0.,0.,1.));
#65199=DIRECTION('center_axis',(0.,-1.,0.));
#65200=DIRECTION('ref_axis',(0.,0.,-1.));
#65201=DIRECTION('center_axis',(0.,1.,0.));
#65202=DIRECTION('ref_axis',(0.,0.,1.));
#65203=DIRECTION('center_axis',(0.,-1.,0.));
#65204=DIRECTION('ref_axis',(0.,0.,-1.));
#65205=DIRECTION('center_axis',(0.,1.,0.));
#65206=DIRECTION('ref_axis',(0.,0.,1.));
#65207=DIRECTION('center_axis',(0.,-1.,0.));
#65208=DIRECTION('ref_axis',(0.,0.,-1.));
#65209=DIRECTION('center_axis',(0.,1.,0.));
#65210=DIRECTION('ref_axis',(0.,0.,1.));
#65211=DIRECTION('center_axis',(0.,-1.,0.));
#65212=DIRECTION('ref_axis',(0.,0.,-1.));
#65213=DIRECTION('center_axis',(0.,1.,0.));
#65214=DIRECTION('ref_axis',(0.,0.,1.));
#65215=DIRECTION('center_axis',(0.,-1.,0.));
#65216=DIRECTION('ref_axis',(0.,0.,-1.));
#65217=DIRECTION('center_axis',(0.,1.,0.));
#65218=DIRECTION('ref_axis',(0.,0.,1.));
#65219=DIRECTION('center_axis',(0.,-1.,0.));
#65220=DIRECTION('ref_axis',(0.,0.,-1.));
#65221=DIRECTION('center_axis',(0.,1.,0.));
#65222=DIRECTION('ref_axis',(0.,0.,1.));
#65223=DIRECTION('center_axis',(0.,-1.,0.));
#65224=DIRECTION('ref_axis',(0.,0.,-1.));
#65225=DIRECTION('center_axis',(0.,1.,0.));
#65226=DIRECTION('ref_axis',(0.,0.,1.));
#65227=DIRECTION('center_axis',(0.,1.,0.));
#65228=DIRECTION('ref_axis',(0.,0.,1.));
#65229=DIRECTION('center_axis',(0.,1.,0.));
#65230=DIRECTION('ref_axis',(0.,0.,1.));
#65231=DIRECTION('center_axis',(0.,1.,0.));
#65232=DIRECTION('ref_axis',(0.,0.,1.));
#65233=DIRECTION('center_axis',(0.,1.,0.));
#65234=DIRECTION('ref_axis',(0.,0.,1.));
#65235=DIRECTION('center_axis',(0.,1.,0.));
#65236=DIRECTION('ref_axis',(0.,0.,1.));
#65237=DIRECTION('center_axis',(0.,1.,0.));
#65238=DIRECTION('ref_axis',(0.,0.,1.));
#65239=DIRECTION('center_axis',(0.,1.,0.));
#65240=DIRECTION('ref_axis',(0.,0.,1.));
#65241=DIRECTION('center_axis',(0.,1.,0.));
#65242=DIRECTION('ref_axis',(0.,0.,1.));
#65243=DIRECTION('center_axis',(0.,1.,0.));
#65244=DIRECTION('ref_axis',(0.,0.,1.));
#65245=DIRECTION('center_axis',(0.,1.,0.));
#65246=DIRECTION('ref_axis',(0.,0.,1.));
#65247=DIRECTION('center_axis',(0.,1.,0.));
#65248=DIRECTION('ref_axis',(0.,0.,1.));
#65249=DIRECTION('center_axis',(0.,1.,0.));
#65250=DIRECTION('ref_axis',(0.,0.,1.));
#65251=DIRECTION('center_axis',(0.,1.,0.));
#65252=DIRECTION('ref_axis',(0.,0.,1.));
#65253=DIRECTION('center_axis',(0.,1.,0.));
#65254=DIRECTION('ref_axis',(0.,0.,1.));
#65255=DIRECTION('center_axis',(0.,1.,0.));
#65256=DIRECTION('ref_axis',(0.,0.,1.));
#65257=DIRECTION('center_axis',(0.,1.,0.));
#65258=DIRECTION('ref_axis',(0.,0.,1.));
#65259=DIRECTION('center_axis',(0.,1.,0.));
#65260=DIRECTION('ref_axis',(0.,0.,1.));
#65261=DIRECTION('center_axis',(0.,1.,0.));
#65262=DIRECTION('ref_axis',(0.,0.,1.));
#65263=DIRECTION('center_axis',(0.,1.,0.));
#65264=DIRECTION('ref_axis',(0.,0.,1.));
#65265=DIRECTION('center_axis',(0.,1.,0.));
#65266=DIRECTION('ref_axis',(0.,0.,1.));
#65267=DIRECTION('center_axis',(0.,1.,0.));
#65268=DIRECTION('ref_axis',(0.,0.,1.));
#65269=DIRECTION('center_axis',(0.,1.,0.));
#65270=DIRECTION('ref_axis',(0.,0.,1.));
#65271=DIRECTION('center_axis',(0.,1.,0.));
#65272=DIRECTION('ref_axis',(0.,0.,1.));
#65273=DIRECTION('center_axis',(0.,1.,0.));
#65274=DIRECTION('ref_axis',(0.,0.,1.));
#65275=DIRECTION('center_axis',(0.,1.,0.));
#65276=DIRECTION('ref_axis',(0.,0.,1.));
#65277=DIRECTION('center_axis',(0.,1.,0.));
#65278=DIRECTION('ref_axis',(0.,0.,1.));
#65279=DIRECTION('center_axis',(0.,1.,0.));
#65280=DIRECTION('ref_axis',(0.,0.,1.));
#65281=DIRECTION('center_axis',(0.,1.,0.));
#65282=DIRECTION('ref_axis',(0.,0.,1.));
#65283=DIRECTION('center_axis',(0.,1.,0.));
#65284=DIRECTION('ref_axis',(0.,0.,1.));
#65285=DIRECTION('center_axis',(0.,1.,0.));
#65286=DIRECTION('ref_axis',(0.,0.,1.));
#65287=DIRECTION('center_axis',(0.,1.,0.));
#65288=DIRECTION('ref_axis',(0.,0.,1.));
#65289=DIRECTION('center_axis',(0.,1.,0.));
#65290=DIRECTION('ref_axis',(0.,0.,1.));
#65291=DIRECTION('center_axis',(0.,1.,0.));
#65292=DIRECTION('ref_axis',(0.,0.,1.));
#65293=DIRECTION('center_axis',(0.,1.,0.));
#65294=DIRECTION('ref_axis',(0.,0.,1.));
#65295=DIRECTION('center_axis',(0.,1.,0.));
#65296=DIRECTION('ref_axis',(0.,0.,1.));
#65297=DIRECTION('center_axis',(0.,1.,0.));
#65298=DIRECTION('ref_axis',(0.,0.,1.));
#65299=DIRECTION('center_axis',(0.,1.,0.));
#65300=DIRECTION('ref_axis',(0.,0.,1.));
#65301=DIRECTION('center_axis',(0.,1.,0.));
#65302=DIRECTION('ref_axis',(0.,0.,1.));
#65303=DIRECTION('center_axis',(0.,1.,0.));
#65304=DIRECTION('ref_axis',(0.,0.,1.));
#65305=DIRECTION('center_axis',(0.,1.,0.));
#65306=DIRECTION('ref_axis',(0.,0.,1.));
#65307=DIRECTION('center_axis',(0.,1.,0.));
#65308=DIRECTION('ref_axis',(0.,0.,1.));
#65309=DIRECTION('center_axis',(0.,1.,0.));
#65310=DIRECTION('ref_axis',(0.,0.,1.));
#65311=DIRECTION('center_axis',(0.,1.,0.));
#65312=DIRECTION('ref_axis',(0.,0.,1.));
#65313=DIRECTION('center_axis',(0.,1.,0.));
#65314=DIRECTION('ref_axis',(0.,0.,1.));
#65315=DIRECTION('center_axis',(0.,1.,0.));
#65316=DIRECTION('ref_axis',(0.,0.,1.));
#65317=DIRECTION('center_axis',(0.,1.,0.));
#65318=DIRECTION('ref_axis',(0.,0.,1.));
#65319=DIRECTION('center_axis',(0.,1.,0.));
#65320=DIRECTION('ref_axis',(0.,0.,1.));
#65321=DIRECTION('center_axis',(0.,1.,0.));
#65322=DIRECTION('ref_axis',(0.,0.,1.));
#65323=DIRECTION('center_axis',(0.,1.,0.));
#65324=DIRECTION('ref_axis',(0.,0.,1.));
#65325=DIRECTION('center_axis',(0.,1.,0.));
#65326=DIRECTION('ref_axis',(0.,0.,1.));
#65327=DIRECTION('center_axis',(0.,1.,0.));
#65328=DIRECTION('ref_axis',(0.,0.,1.));
#65329=DIRECTION('center_axis',(0.,1.,0.));
#65330=DIRECTION('ref_axis',(0.,0.,1.));
#65331=DIRECTION('center_axis',(0.,1.,0.));
#65332=DIRECTION('ref_axis',(0.,0.,1.));
#65333=DIRECTION('center_axis',(0.,1.,0.));
#65334=DIRECTION('ref_axis',(0.,0.,1.));
#65335=DIRECTION('center_axis',(0.,1.,0.));
#65336=DIRECTION('ref_axis',(0.,0.,1.));
#65337=DIRECTION('center_axis',(0.,1.,0.));
#65338=DIRECTION('ref_axis',(0.,0.,1.));
#65339=DIRECTION('center_axis',(0.,1.,0.));
#65340=DIRECTION('ref_axis',(0.,0.,1.));
#65341=DIRECTION('center_axis',(0.,1.,0.));
#65342=DIRECTION('ref_axis',(0.,0.,1.));
#65343=DIRECTION('center_axis',(0.,1.,0.));
#65344=DIRECTION('ref_axis',(0.,0.,1.));
#65345=DIRECTION('center_axis',(0.,1.,0.));
#65346=DIRECTION('ref_axis',(0.,0.,1.));
#65347=DIRECTION('center_axis',(0.,1.,0.));
#65348=DIRECTION('ref_axis',(0.,0.,1.));
#65349=DIRECTION('center_axis',(0.,1.,0.));
#65350=DIRECTION('ref_axis',(0.,0.,1.));
#65351=DIRECTION('center_axis',(0.,1.,0.));
#65352=DIRECTION('ref_axis',(0.,0.,1.));
#65353=DIRECTION('center_axis',(0.,1.,0.));
#65354=DIRECTION('ref_axis',(0.,0.,1.));
#65355=DIRECTION('center_axis',(0.,1.,0.));
#65356=DIRECTION('ref_axis',(0.,0.,1.));
#65357=DIRECTION('center_axis',(0.,1.,0.));
#65358=DIRECTION('ref_axis',(0.,0.,1.));
#65359=DIRECTION('center_axis',(0.,1.,0.));
#65360=DIRECTION('ref_axis',(0.,0.,1.));
#65361=DIRECTION('center_axis',(0.,1.,0.));
#65362=DIRECTION('ref_axis',(0.,0.,1.));
#65363=DIRECTION('center_axis',(0.,1.,0.));
#65364=DIRECTION('ref_axis',(0.,0.,1.));
#65365=DIRECTION('center_axis',(0.,1.,0.));
#65366=DIRECTION('ref_axis',(0.,0.,1.));
#65367=DIRECTION('center_axis',(0.,1.,0.));
#65368=DIRECTION('ref_axis',(0.,0.,1.));
#65369=DIRECTION('center_axis',(0.,1.,0.));
#65370=DIRECTION('ref_axis',(0.,0.,1.));
#65371=DIRECTION('center_axis',(0.,1.,0.));
#65372=DIRECTION('ref_axis',(0.,0.,1.));
#65373=DIRECTION('center_axis',(0.,1.,0.));
#65374=DIRECTION('ref_axis',(0.,0.,1.));
#65375=DIRECTION('center_axis',(0.,1.,0.));
#65376=DIRECTION('ref_axis',(0.,0.,1.));
#65377=DIRECTION('center_axis',(0.,1.,0.));
#65378=DIRECTION('ref_axis',(0.,0.,1.));
#65379=DIRECTION('center_axis',(0.,1.,0.));
#65380=DIRECTION('ref_axis',(0.,0.,1.));
#65381=DIRECTION('center_axis',(0.,1.,0.));
#65382=DIRECTION('ref_axis',(0.,0.,1.));
#65383=DIRECTION('center_axis',(0.,1.,0.));
#65384=DIRECTION('ref_axis',(0.,0.,1.));
#65385=DIRECTION('center_axis',(0.,1.,0.));
#65386=DIRECTION('ref_axis',(0.,0.,1.));
#65387=DIRECTION('center_axis',(0.,1.,0.));
#65388=DIRECTION('ref_axis',(0.,0.,1.));
#65389=DIRECTION('center_axis',(0.,1.,0.));
#65390=DIRECTION('ref_axis',(0.,0.,1.));
#65391=DIRECTION('center_axis',(0.,1.,0.));
#65392=DIRECTION('ref_axis',(0.,0.,1.));
#65393=DIRECTION('center_axis',(0.,1.,0.));
#65394=DIRECTION('ref_axis',(0.,0.,1.));
#65395=DIRECTION('center_axis',(0.,1.,0.));
#65396=DIRECTION('ref_axis',(0.,0.,1.));
#65397=DIRECTION('center_axis',(0.,1.,0.));
#65398=DIRECTION('ref_axis',(0.,0.,1.));
#65399=DIRECTION('center_axis',(0.,1.,0.));
#65400=DIRECTION('ref_axis',(0.,0.,1.));
#65401=DIRECTION('center_axis',(0.,1.,0.));
#65402=DIRECTION('ref_axis',(0.,0.,1.));
#65403=DIRECTION('center_axis',(0.,1.,0.));
#65404=DIRECTION('ref_axis',(0.,0.,1.));
#65405=DIRECTION('center_axis',(0.,1.,0.));
#65406=DIRECTION('ref_axis',(0.,0.,1.));
#65407=DIRECTION('center_axis',(0.,1.,0.));
#65408=DIRECTION('ref_axis',(0.,0.,1.));
#65409=DIRECTION('center_axis',(0.,1.,0.));
#65410=DIRECTION('ref_axis',(0.,0.,1.));
#65411=DIRECTION('center_axis',(0.,1.,0.));
#65412=DIRECTION('ref_axis',(0.,0.,1.));
#65413=DIRECTION('center_axis',(0.,1.,0.));
#65414=DIRECTION('ref_axis',(0.,0.,1.));
#65415=DIRECTION('center_axis',(0.,1.,0.));
#65416=DIRECTION('ref_axis',(0.,0.,1.));
#65417=DIRECTION('center_axis',(0.,1.,0.));
#65418=DIRECTION('ref_axis',(0.,0.,1.));
#65419=DIRECTION('center_axis',(0.,1.,0.));
#65420=DIRECTION('ref_axis',(0.,0.,1.));
#65421=DIRECTION('center_axis',(0.,1.,0.));
#65422=DIRECTION('ref_axis',(0.,0.,1.));
#65423=DIRECTION('center_axis',(0.,1.,0.));
#65424=DIRECTION('ref_axis',(0.,0.,1.));
#65425=DIRECTION('center_axis',(0.,1.,0.));
#65426=DIRECTION('ref_axis',(0.,0.,1.));
#65427=DIRECTION('center_axis',(0.,1.,0.));
#65428=DIRECTION('ref_axis',(0.,0.,1.));
#65429=DIRECTION('center_axis',(0.,1.,0.));
#65430=DIRECTION('ref_axis',(0.,0.,1.));
#65431=DIRECTION('center_axis',(0.,1.,0.));
#65432=DIRECTION('ref_axis',(0.,0.,1.));
#65433=DIRECTION('center_axis',(0.,1.,0.));
#65434=DIRECTION('ref_axis',(0.,0.,1.));
#65435=DIRECTION('center_axis',(0.,1.,0.));
#65436=DIRECTION('ref_axis',(0.,0.,1.));
#65437=DIRECTION('center_axis',(0.,1.,0.));
#65438=DIRECTION('ref_axis',(0.,0.,1.));
#65439=DIRECTION('center_axis',(0.,1.,0.));
#65440=DIRECTION('ref_axis',(0.,0.,1.));
#65441=DIRECTION('center_axis',(0.,1.,0.));
#65442=DIRECTION('ref_axis',(0.,0.,1.));
#65443=DIRECTION('center_axis',(0.,1.,0.));
#65444=DIRECTION('ref_axis',(0.,0.,1.));
#65445=DIRECTION('center_axis',(0.,1.,0.));
#65446=DIRECTION('ref_axis',(0.,0.,1.));
#65447=DIRECTION('center_axis',(0.,1.,0.));
#65448=DIRECTION('ref_axis',(0.,0.,1.));
#65449=DIRECTION('center_axis',(0.,1.,0.));
#65450=DIRECTION('ref_axis',(0.,0.,1.));
#65451=DIRECTION('center_axis',(0.,1.,0.));
#65452=DIRECTION('ref_axis',(0.,0.,1.));
#65453=DIRECTION('center_axis',(0.,1.,0.));
#65454=DIRECTION('ref_axis',(0.,0.,1.));
#65455=DIRECTION('center_axis',(0.,1.,0.));
#65456=DIRECTION('ref_axis',(0.,0.,1.));
#65457=DIRECTION('center_axis',(0.,1.,0.));
#65458=DIRECTION('ref_axis',(0.,0.,1.));
#65459=DIRECTION('center_axis',(0.,1.,0.));
#65460=DIRECTION('ref_axis',(0.,0.,1.));
#65461=DIRECTION('center_axis',(0.,1.,0.));
#65462=DIRECTION('ref_axis',(0.,0.,1.));
#106591=CARTESIAN_POINT('',(0.,0.,0.));
#106592=CARTESIAN_POINT('Ctrl Pts',(0.,1078.73142393294,339.50750164799));
#106593=CARTESIAN_POINT('Ctrl Pts',(-170.225481863728,1078.73142393294,
339.50750164799));
#106594=CARTESIAN_POINT('Ctrl Pts',(-170.225481863728,1078.73142393294,
509.732983511718));
#106595=CARTESIAN_POINT('Ctrl Pts',(-1.04233045748865E-14,1078.73142393294,
509.732983511718));
#106596=CARTESIAN_POINT('Ctrl Pts',(0.,1078.73142393294,320.460533783102));
#106597=CARTESIAN_POINT('Ctrl Pts',(-208.319417593505,1078.73142393294,
320.460533783101));
#106598=CARTESIAN_POINT('Ctrl Pts',(-208.319417593505,1078.73142393294,
528.779951376607));
#106599=CARTESIAN_POINT('Ctrl Pts',(-1.27558853978063E-14,1078.73142393294,
528.779951376607));
#106600=CARTESIAN_POINT('Ctrl Pts',(0.,1074.39201604106,297.79821279751));
#106601=CARTESIAN_POINT('Ctrl Pts',(-253.644059564688,1074.39201604106,
297.79821279751));
#106602=CARTESIAN_POINT('Ctrl Pts',(-253.644059564688,1074.39201604106,
551.442272362198));
#106603=CARTESIAN_POINT('Ctrl Pts',(-1.55312192834318E-14,1074.39201604106,
551.442272362198));
#106604=CARTESIAN_POINT('',(0.,1078.73142393294,339.50750164799));
#106605=CARTESIAN_POINT('',(-1.29772619291592E-14,1078.73142393294,509.732983511718));
#106606=CARTESIAN_POINT('Origin',(0.,1078.73142393294,424.620242579854));
#106607=CARTESIAN_POINT('',(1.55675932686082E-14,1074.39201604106,551.442272362198));
#106608=CARTESIAN_POINT('Ctrl Pts',(-1.29772619291592E-14,1078.73142393294,
509.732983511718));
#106609=CARTESIAN_POINT('Ctrl Pts',(-1.27558853978063E-14,1078.73142393294,
528.779951376607));
#106610=CARTESIAN_POINT('Ctrl Pts',(1.55675932686082E-14,1074.39201604106,
551.442272362198));
#106611=CARTESIAN_POINT('',(0.,1074.39201604106,297.79821279751));
#106612=CARTESIAN_POINT('Origin',(0.,1074.39201604106,424.620242579854));
#106613=CARTESIAN_POINT('Ctrl Pts',(0.,1078.73142393294,339.50750164799));
#106614=CARTESIAN_POINT('Ctrl Pts',(0.,1078.73142393294,320.460533783102));
#106615=CARTESIAN_POINT('Ctrl Pts',(0.,1074.39201604106,297.79821279751));
#106616=CARTESIAN_POINT('',(-80.0774492048026,1076.71653899679,503.992543977749));
#106617=CARTESIAN_POINT('',(-80.0774492048019,1076.92126679813,501.811462480293));
#106618=CARTESIAN_POINT('Ctrl Pts',(-80.0774492048026,1076.71653899679,
503.99254397775));
#106619=CARTESIAN_POINT('Ctrl Pts',(-80.0744534615737,1076.71683147352,
503.99254397775));
#106620=CARTESIAN_POINT('Ctrl Pts',(-80.0714573718756,1076.71712514229,
503.992531633677));
#106621=CARTESIAN_POINT('Ctrl Pts',(-79.943955331041,1076.72967184833,503.991480731246));
#106622=CARTESIAN_POINT('Ctrl Pts',(-79.8207166503327,1076.74379814044,
503.969143227292));
#106623=CARTESIAN_POINT('Ctrl Pts',(-79.577533957504,1076.77578352609,503.88051966644));
#106624=CARTESIAN_POINT('Ctrl Pts',(-79.4607372426172,1076.79359323853,
503.81141461075));
#106625=CARTESIAN_POINT('Ctrl Pts',(-79.2503459058597,1076.83112034606,
503.627408466814));
#106626=CARTESIAN_POINT('Ctrl Pts',(-79.1612532432344,1076.85052705261,
503.511054337047));
#106627=CARTESIAN_POINT('Ctrl Pts',(-79.034986449722,1076.88662226974,503.252524728555));
#106628=CARTESIAN_POINT('Ctrl Pts',(-78.9980549007521,1076.90302340953,
503.113237675));
#106629=CARTESIAN_POINT('Ctrl Pts',(-78.981158028069,1076.92937865835,502.845054518431));
#106630=CARTESIAN_POINT('Ctrl Pts',(-78.9950123084823,1076.9396744246,502.718929500932));
#106631=CARTESIAN_POINT('Ctrl Pts',(-79.0631424379183,1076.95481257403,
502.48437207685));
#106632=CARTESIAN_POINT('Ctrl Pts',(-79.114335267768,1076.95985546338,502.376940166403));
#106633=CARTESIAN_POINT('Ctrl Pts',(-79.2009077894259,1076.96315646626,
502.252333982574));
#106634=CARTESIAN_POINT('Ctrl Pts',(-79.2212198095973,1076.96368450051,
502.225788297461));
#106635=CARTESIAN_POINT('Ctrl Pts',(-79.2551483758368,1076.96420163092,
502.18543262218));
#106636=CARTESIAN_POINT('Ctrl Pts',(-79.2679670347454,1076.96432402283,
502.17098288737));
#106637=CARTESIAN_POINT('Ctrl Pts',(-79.2912378146408,1076.96442142972,
502.146114217026));
#106638=CARTESIAN_POINT('Ctrl Pts',(-79.3015300358806,1076.96442444417,
502.135552973688));
#106639=CARTESIAN_POINT('Ctrl Pts',(-79.325475365329,1076.96434204115,502.11195855146));
#106640=CARTESIAN_POINT('Ctrl Pts',(-79.3392587639923,1076.9642316591,502.099064815849));
#106641=CARTESIAN_POINT('Ctrl Pts',(-79.3775703970506,1076.9637581534,502.0650467013));
#106642=CARTESIAN_POINT('Ctrl Pts',(-79.4027138542756,1076.96327099962,
502.044647745071));
#106643=CARTESIAN_POINT('Ctrl Pts',(-79.5260338693428,1076.96007640994,
501.953385719726));
#106644=CARTESIAN_POINT('Ctrl Pts',(-79.6345730508686,1076.95496834037,
501.898137388195));
#106645=CARTESIAN_POINT('Ctrl Pts',(-79.8559752282958,1076.9405751612,501.82840729055));
#106646=CARTESIAN_POINT('Ctrl Pts',(-79.966456771482,1076.93174117589,501.811462480293));
#106647=CARTESIAN_POINT('Ctrl Pts',(-80.0774492048019,1076.92126679813,
501.811462480293));
#106648=CARTESIAN_POINT('Ctrl Pts',(-80.0774492048018,1076.92126679813,
501.811462480293));
#106649=CARTESIAN_POINT('Ctrl Pts',(-80.0774629292238,1076.92126550295,
501.811462480293));
#106650=CARTESIAN_POINT('Ctrl Pts',(-80.0774766536537,1076.92126420775,
501.811462480552));
#106651=CARTESIAN_POINT('Ctrl Pts',(-80.0774903780913,1076.92126291252,
501.81146248107));
#106652=CARTESIAN_POINT('Ctrl Pts',(-80.2021265314636,1076.90950053199,
501.811467186699));
#106653=CARTESIAN_POINT('Ctrl Pts',(-80.3256648570161,1076.89583323305,
501.83283599449));
#106654=CARTESIAN_POINT('Ctrl Pts',(-80.5700028028231,1076.86453989815,
501.919709426156));
#106655=CARTESIAN_POINT('Ctrl Pts',(-80.6876152646318,1076.84693308657,
501.988137880998));
#106656=CARTESIAN_POINT('Ctrl Pts',(-80.9000017320625,1076.80939942596,
502.1713164524));
#106657=CARTESIAN_POINT('Ctrl Pts',(-80.9901753298772,1076.78975278149,
502.28762664943));
#106658=CARTESIAN_POINT('Ctrl Pts',(-81.1180209332028,1076.75293615633,
502.545939183293));
#106659=CARTESIAN_POINT('Ctrl Pts',(-81.1556746375667,1076.73605729288,
502.684941916594));
#106660=CARTESIAN_POINT('Ctrl Pts',(-81.1740308668573,1076.70871614022,
502.952856609623));
#106661=CARTESIAN_POINT('Ctrl Pts',(-81.1608916991995,1076.69793149323,
503.078985121758));
#106662=CARTESIAN_POINT('Ctrl Pts',(-81.0937095185396,1076.68187189764,
503.315280887528));
#106663=CARTESIAN_POINT('Ctrl Pts',(-81.0422687355384,1076.67645734701,
503.424266348347));
#106664=CARTESIAN_POINT('Ctrl Pts',(-80.9548714480136,1076.67291908737,
503.550498510701));
#106665=CARTESIAN_POINT('Ctrl Pts',(-80.9344015515705,1076.67235413421,
503.577317294338));
#106666=CARTESIAN_POINT('Ctrl Pts',(-80.9001937579785,1076.67180071199,
503.618068925671));
#106667=CARTESIAN_POINT('Ctrl Pts',(-80.8872700626789,1076.67166965064,
503.632652871637));
#106668=CARTESIAN_POINT('Ctrl Pts',(-80.8638039277403,1076.67156506224,
503.657745619015));
#106669=CARTESIAN_POINT('Ctrl Pts',(-80.8534244163316,1076.6715616049,503.668399199569));
#106670=CARTESIAN_POINT('Ctrl Pts',(-80.8292723903451,1076.67164906506,
503.692195150688));
#106671=CARTESIAN_POINT('Ctrl Pts',(-80.8153674388274,1076.67176663838,
503.705195625592));
#106672=CARTESIAN_POINT('Ctrl Pts',(-80.7767073202748,1076.6722714466,503.739489346514));
#106673=CARTESIAN_POINT('Ctrl Pts',(-80.7513267907336,1076.672791148,503.760043730673));
#106674=CARTESIAN_POINT('Ctrl Pts',(-80.6266644716121,1076.67620269702,
503.852055507836));
#106675=CARTESIAN_POINT('Ctrl Pts',(-80.5168403634148,1076.68166443625,
503.907546730497));
#106676=CARTESIAN_POINT('Ctrl Pts',(-80.2955490543128,1076.69678724743,
503.976117862873));
#106677=CARTESIAN_POINT('Ctrl Pts',(-80.1867296369359,1076.70586986388,
503.99254397775));
#106678=CARTESIAN_POINT('Ctrl Pts',(-80.0774492048026,1076.71653899679,
503.99254397775));
#106679=CARTESIAN_POINT('',(-94.6032580293202,1076.74090351967,485.632861828239));
#106680=CARTESIAN_POINT('',(-94.6032580293197,1076.89762188922,483.451780330783));
#106681=CARTESIAN_POINT('Ctrl Pts',(-94.6032580293202,1076.74090351967,
485.63286182824));
#106682=CARTESIAN_POINT('Ctrl Pts',(-94.4934032622873,1076.75352605296,
485.63286182824));
#106683=CARTESIAN_POINT('Ctrl Pts',(-94.3841704543758,1076.76724681555,
485.616262376579));
#106684=CARTESIAN_POINT('Ctrl Pts',(-94.1464351966987,1076.79973481212,
485.542293254238));
#106685=CARTESIAN_POINT('Ctrl Pts',(-94.0227520764538,1076.81856962477,
485.475933789659));
#106686=CARTESIAN_POINT('Ctrl Pts',(-93.8025697775747,1076.8563159382,485.296740373648));
#106687=CARTESIAN_POINT('Ctrl Pts',(-93.7094593202231,1076.87484627511,
485.183773120545));
#106688=CARTESIAN_POINT('Ctrl Pts',(-93.5758671374664,1076.90758888432,
484.933433266239));
#106689=CARTESIAN_POINT('Ctrl Pts',(-93.534411712552,1076.92166811443,484.79959274449));
#106690=CARTESIAN_POINT('Ctrl Pts',(-93.5055131017688,1076.94342992723,
484.536401468821));
#106691=CARTESIAN_POINT('Ctrl Pts',(-93.5134824327387,1076.95143233486,
484.409867704565));
#106692=CARTESIAN_POINT('Ctrl Pts',(-93.5600329759078,1076.95985956288,
484.216275065995));
#106693=CARTESIAN_POINT('Ctrl Pts',(-93.5842379368745,1076.96203239778,
484.147060908851));
#106694=CARTESIAN_POINT('Ctrl Pts',(-93.6263115269911,1076.96368945428,
484.056992980237));
#106695=CARTESIAN_POINT('Ctrl Pts',(-93.6382737929135,1076.96400366827,
484.033623314572));
#106696=CARTESIAN_POINT('Ctrl Pts',(-93.6591896714621,1076.96431490958,
483.996160281757));
#106697=CARTESIAN_POINT('Ctrl Pts',(-93.6676434573539,1076.96438582567,
483.981801614756));
#106698=CARTESIAN_POINT('Ctrl Pts',(-93.6845453285145,1076.96442611176,
483.954542490863));
#106699=CARTESIAN_POINT('Ctrl Pts',(-93.6929444419125,1076.96440268101,
483.941616604474));
#106700=CARTESIAN_POINT('Ctrl Pts',(-93.7129292816478,1076.96425007526,
483.912242966635));
#106701=CARTESIAN_POINT('Ctrl Pts',(-93.724701520582,1076.96409086024,483.895929460495));
#106702=CARTESIAN_POINT('Ctrl Pts',(-93.7624748523549,1076.963373952,483.846524192872));
#106703=CARTESIAN_POINT('Ctrl Pts',(-93.7899415522706,1076.96257163799,
483.81460892862));
#106704=CARTESIAN_POINT('Ctrl Pts',(-93.9196445930091,1076.95762210125,
483.680435726889));
#106705=CARTESIAN_POINT('Ctrl Pts',(-94.0396516800389,1076.95014256301,
483.597637961895));
#106706=CARTESIAN_POINT('Ctrl Pts',(-94.246520508683,1076.93342095431,483.508600621991));
#106707=CARTESIAN_POINT('Ctrl Pts',(-94.3241836294889,1076.92644211135,
483.484997789265));
#106708=CARTESIAN_POINT('Ctrl Pts',(-94.4695396532436,1076.91214081338,
483.457937088357));
#106709=CARTESIAN_POINT('Ctrl Pts',(-94.5363541198077,1076.9051120287,483.451780330783));
#106710=CARTESIAN_POINT('Ctrl Pts',(-94.6032580293197,1076.89762188922,
483.451780330783));
#106711=CARTESIAN_POINT('Ctrl Pts',(-94.6032580293197,1076.89762188922,
483.451780330783));
#106712=CARTESIAN_POINT('Ctrl Pts',(-94.6033088295668,1076.89761620195,
483.451780330783));
#106713=CARTESIAN_POINT('Ctrl Pts',(-94.6033596298654,1076.8976105144,483.451780334333));
#106714=CARTESIAN_POINT('Ctrl Pts',(-94.6034104302152,1076.8976048266,483.451780341432));
#106715=CARTESIAN_POINT('Ctrl Pts',(-94.7345782155871,1076.88291876555,
483.451798671868));
#106716=CARTESIAN_POINT('Ctrl Pts',(-94.8645199165171,1076.86663371627,
483.475479152504));
#106717=CARTESIAN_POINT('Ctrl Pts',(-95.1194516259798,1076.83100336629,
483.571323081755));
#106718=CARTESIAN_POINT('Ctrl Pts',(-95.24091267592,1076.81183445465,483.646396699055));
#106719=CARTESIAN_POINT('Ctrl Pts',(-95.4504511381765,1076.77393950236,
483.840637335467));
#106720=CARTESIAN_POINT('Ctrl Pts',(-95.5358689623058,1076.75558168784,
483.958862417053));
#106721=CARTESIAN_POINT('Ctrl Pts',(-95.6520833276736,1076.72364111572,
484.21413129241));
#106722=CARTESIAN_POINT('Ctrl Pts',(-95.6848687531977,1076.71011140889,
484.347438871334));
#106723=CARTESIAN_POINT('Ctrl Pts',(-95.6993860135574,1076.68872679539,
484.616451385736));
#106724=CARTESIAN_POINT('Ctrl Pts',(-95.6821786999132,1076.68093128049,
484.749708287279));
#106725=CARTESIAN_POINT('Ctrl Pts',(-95.6250071691597,1076.67452004241,
484.927186355404));
#106726=CARTESIAN_POINT('Ctrl Pts',(-95.6050779052817,1076.67321222476,
484.97643194779));
#106727=CARTESIAN_POINT('Ctrl Pts',(-95.5715286428288,1076.67209627377,
485.044570774938));
#106728=CARTESIAN_POINT('Ctrl Pts',(-95.5607766979455,1076.67185853078,
485.064777617924));
#106729=CARTESIAN_POINT('Ctrl Pts',(-95.5422279124747,1076.67163220854,
485.097138602302));
#106730=CARTESIAN_POINT('Ctrl Pts',(-95.5348120391529,1076.67158400241,
485.109501880515));
#106731=CARTESIAN_POINT('Ctrl Pts',(-95.518779683349,1076.67156534638,485.135066913996));
#106732=CARTESIAN_POINT('Ctrl Pts',(-95.5101177694239,1076.67160257376,
485.148236032317));
#106733=CARTESIAN_POINT('Ctrl Pts',(-95.4889316728475,1076.67180194277,
485.178973763344));
#106734=CARTESIAN_POINT('Ctrl Pts',(-95.476165970251,1076.672005032,485.19636702731));
#106735=CARTESIAN_POINT('Ctrl Pts',(-95.4326636719739,1076.67295772295,
485.252094906878));
#106736=CARTESIAN_POINT('Ctrl Pts',(-95.3998579760909,1076.67407291771,
485.288725236744));
#106737=CARTESIAN_POINT('Ctrl Pts',(-95.261000092873,1076.68023290497,485.424159775002));
#106738=CARTESIAN_POINT('Ctrl Pts',(-95.1383265104726,1076.68863623939,
485.503495528396));
#106739=CARTESIAN_POINT('Ctrl Pts',(-94.8940061951528,1076.70981789088,
485.600016013295));
#106740=CARTESIAN_POINT('Ctrl Pts',(-94.7778927388487,1076.72137705126,
485.625223525282));
#106741=CARTESIAN_POINT('Ctrl Pts',(-94.6411952947611,1076.7365793124,485.632367414648));
#106742=CARTESIAN_POINT('Ctrl Pts',(-94.6222173980957,1076.73872505013,
485.63286182824));
#106743=CARTESIAN_POINT('Ctrl Pts',(-94.6032580293201,1076.74090351967,
485.63286182824));
#106744=CARTESIAN_POINT('',(-93.6720377362212,1077.61442735558,472.874586465029));
#106745=CARTESIAN_POINT('',(-93.6720377362213,1077.7163862265,470.676924193044));
#106746=CARTESIAN_POINT('Ctrl Pts',(-93.6720377362213,1077.61442735558,
472.874586465029));
#106747=CARTESIAN_POINT('Ctrl Pts',(-93.5677573540383,1077.62420150145,
472.874586465029));
#106748=CARTESIAN_POINT('Ctrl Pts',(-93.4639081817383,1077.63458923107,
472.859741243044));
#106749=CARTESIAN_POINT('Ctrl Pts',(-93.2274100948857,1077.65976663472,
472.790586039158));
#106750=CARTESIAN_POINT('Ctrl Pts',(-93.1001671010855,1077.67454354204,
472.724726821711));
#106751=CARTESIAN_POINT('Ctrl Pts',(-92.8753830609211,1077.70331191389,
472.546338198103));
#106752=CARTESIAN_POINT('Ctrl Pts',(-92.7806725594652,1077.71700728856,
472.43453227919));
#106753=CARTESIAN_POINT('Ctrl Pts',(-92.6442782205473,1077.74049969227,
472.187843968462));
#106754=CARTESIAN_POINT('Ctrl Pts',(-92.6009800357877,1077.75027798954,
472.056842117196));
#106755=CARTESIAN_POINT('Ctrl Pts',(-92.5645514630971,1077.76578299318,
471.783922622182));
#106756=CARTESIAN_POINT('Ctrl Pts',(-92.5723175270602,1077.77132437777,
471.644386886577));
#106757=CARTESIAN_POINT('Ctrl Pts',(-92.6171461547586,1077.77537343022,
471.464608895946));
#106758=CARTESIAN_POINT('Ctrl Pts',(-92.6313139919142,1077.77610402404,
471.420082301668));
#106759=CARTESIAN_POINT('Ctrl Pts',(-92.6552158608447,1077.77672038478,
471.358779940149));
#106760=CARTESIAN_POINT('Ctrl Pts',(-92.6626228297686,1077.77685015463,
471.341155770395));
#106761=CARTESIAN_POINT('Ctrl Pts',(-92.6770340275328,1077.77699746164,
471.309224656014));
#106762=CARTESIAN_POINT('Ctrl Pts',(-92.6838967055807,1077.77703011986,
471.294859748602));
#106763=CARTESIAN_POINT('Ctrl Pts',(-92.6983844259794,1077.7770268126,471.266154808273));
#106764=CARTESIAN_POINT('Ctrl Pts',(-92.7060200917941,1077.77698946655,
471.251824640119));
#106765=CARTESIAN_POINT('Ctrl Pts',(-92.7254310449002,1077.77681123887,
471.217263273819));
#106766=CARTESIAN_POINT('Ctrl Pts',(-92.7375404027597,1077.77663197313,
471.197229366688));
#106767=CARTESIAN_POINT('Ctrl Pts',(-92.7822999176905,1077.77574284715,
471.128255162783));
#106768=CARTESIAN_POINT('Ctrl Pts',(-92.8182257847877,1077.77464215865,
471.081570174133));
#106769=CARTESIAN_POINT('Ctrl Pts',(-92.9554883524616,1077.76923248309,
470.930062508393));
#106770=CARTESIAN_POINT('Ctrl Pts',(-93.0736767060949,1077.76264360369,
470.842727633437));
#106771=CARTESIAN_POINT('Ctrl Pts',(-93.284470346795,1077.74825807343,470.743833021938));
#106772=CARTESIAN_POINT('Ctrl Pts',(-93.367713387491,1077.74204260413,470.71630235684));
#106773=CARTESIAN_POINT('Ctrl Pts',(-93.5253158985138,1077.72931495661,
470.684285821923));
#106774=CARTESIAN_POINT('Ctrl Pts',(-93.5986020744376,1077.72303707031,
470.676924193044));
#106775=CARTESIAN_POINT('Ctrl Pts',(-93.6720377362213,1077.7163862265,470.676924193044));
#106776=CARTESIAN_POINT('Ctrl Pts',(-93.6720377362213,1077.7163862265,470.676924193044));
#106777=CARTESIAN_POINT('Ctrl Pts',(-93.6720989375535,1077.71638068368,
470.676924193044));
#106778=CARTESIAN_POINT('Ctrl Pts',(-93.6721601389895,1077.71637514061,
470.676924198158));
#106779=CARTESIAN_POINT('Ctrl Pts',(-93.6722213405288,1077.71636959727,
470.676924208384));
#106780=CARTESIAN_POINT('Ctrl Pts',(-93.8069747497468,1077.70416429332,
470.676946724406));
#106781=CARTESIAN_POINT('Ctrl Pts',(-93.9405034286092,1077.69085743869,
470.701755567198));
#106782=CARTESIAN_POINT('Ctrl Pts',(-94.2016506327738,1077.66224222225,
470.802097597682));
#106783=CARTESIAN_POINT('Ctrl Pts',(-94.3255124721466,1077.64712899308,
470.880501190131));
#106784=CARTESIAN_POINT('Ctrl Pts',(-94.5347300985438,1077.61827007746,
471.08011089913));
#106785=CARTESIAN_POINT('Ctrl Pts',(-94.6184413026895,1077.60478566402,
471.199088474615));
#106786=CARTESIAN_POINT('Ctrl Pts',(-94.729661473487,1077.58235596944,471.450324393789));
#106787=CARTESIAN_POINT('Ctrl Pts',(-94.7608620275231,1077.57328087477,
471.578278060553));
#106788=CARTESIAN_POINT('Ctrl Pts',(-94.7768576812629,1077.55920485216,
471.840396296642));
#106789=CARTESIAN_POINT('Ctrl Pts',(-94.7611515141652,1077.55435498801,
471.972426858902));
#106790=CARTESIAN_POINT('Ctrl Pts',(-94.7132899750522,1077.55143783682,
472.128147618054));
#106791=CARTESIAN_POINT('Ctrl Pts',(-94.7029580846465,1077.55102179974,
472.15731793579));
#106792=CARTESIAN_POINT('Ctrl Pts',(-94.683983093621,1077.55056687217,472.204465013655));
#106793=CARTESIAN_POINT('Ctrl Pts',(-94.676058017025,1077.5504464427,472.222710256017));
#106794=CARTESIAN_POINT('Ctrl Pts',(-94.6609819777631,1077.55033416925,
472.25499103914));
#106795=CARTESIAN_POINT('Ctrl Pts',(-94.6540163463915,1077.55032075153,
472.269106716838));
#106796=CARTESIAN_POINT('Ctrl Pts',(-94.6386592725339,1077.55036888241,
472.298612639016));
#106797=CARTESIAN_POINT('Ctrl Pts',(-94.6301980232085,1077.55043909918,
472.313961437729));
#106798=CARTESIAN_POINT('Ctrl Pts',(-94.6069026241503,1077.5507426939,472.353927678301));
#106799=CARTESIAN_POINT('Ctrl Pts',(-94.5914641541615,1077.55105160265,
472.378175900708));
#106800=CARTESIAN_POINT('Ctrl Pts',(-94.5201589573807,1077.55291755194,
472.481033754357));
#106801=CARTESIAN_POINT('Ctrl Pts',(-94.4550534889925,1077.55569273445,
472.552672163626));
#106802=CARTESIAN_POINT('Ctrl Pts',(-94.2985309346692,1077.56426334619,
472.685004076036));
#106803=CARTESIAN_POINT('Ctrl Pts',(-94.2057085098637,1077.57034929027,
472.742393452037));
#106804=CARTESIAN_POINT('Ctrl Pts',(-93.9942646670983,1077.58605709614,
472.833304396527));
#106805=CARTESIAN_POINT('Ctrl Pts',(-93.8753492459016,1077.59590949919,
472.862427008106));
#106806=CARTESIAN_POINT('Ctrl Pts',(-93.7268170147061,1077.60933804293,
472.873563519947));
#106807=CARTESIAN_POINT('Ctrl Pts',(-93.6994125152431,1077.61186153181,
472.874586465029));
#106808=CARTESIAN_POINT('Ctrl Pts',(-93.6720377362213,1077.61442735558,
472.874586465029));
#106809=CARTESIAN_POINT('',(-90.2477595453604,1078.31906551735,460.717880652247));
#106810=CARTESIAN_POINT('',(-90.2477595453604,1078.37785269114,458.166992409975));
#106811=CARTESIAN_POINT('Ctrl Pts',(-90.2477595453603,1078.31906551735,
460.717880652247));
#106812=CARTESIAN_POINT('Ctrl Pts',(-90.2327982517213,1078.31998718321,
460.717880652247));
#106813=CARTESIAN_POINT('Ctrl Pts',(-90.2178282660456,1078.32091437956,
460.717617403605));
#106814=CARTESIAN_POINT('Ctrl Pts',(-90.043575120828,1078.33176482721,460.71147887043));
#106815=CARTESIAN_POINT('Ctrl Pts',(-89.886755391279,1078.34208576221,460.676061788484));
#106816=CARTESIAN_POINT('Ctrl Pts',(-89.5854872611562,1078.36301604073,
460.545481693515));
#106817=CARTESIAN_POINT('Ctrl Pts',(-89.4452959445034,1078.37340027169,
460.448116084544));
#106818=CARTESIAN_POINT('Ctrl Pts',(-89.2139758478804,1078.39203625929,
460.207419305018));
#106819=CARTESIAN_POINT('Ctrl Pts',(-89.1238577528026,1078.40016459373,
460.067568688696));
#106820=CARTESIAN_POINT('Ctrl Pts',(-89.0106452747436,1078.41260133485,
459.783327773387));
#106821=CARTESIAN_POINT('Ctrl Pts',(-88.980534811914,1078.41720851565,459.64447860233));
#106822=CARTESIAN_POINT('Ctrl Pts',(-88.9683367981648,1078.42325841417,
459.389970877563));
#106823=CARTESIAN_POINT('Ctrl Pts',(-88.9780938758569,1078.42511565521,
459.276212343589));
#106824=CARTESIAN_POINT('Ctrl Pts',(-89.0105033541495,1078.42640768501,
459.130649493654));
#106825=CARTESIAN_POINT('Ctrl Pts',(-89.0196454756031,1078.42662929176,
459.09638747785));
#106826=CARTESIAN_POINT('Ctrl Pts',(-89.036460872709,1078.42684554272,459.042493179283));
#106827=CARTESIAN_POINT('Ctrl Pts',(-89.0432135336209,1078.42689582627,
459.022593618969));
#106828=CARTESIAN_POINT('Ctrl Pts',(-89.0567634716925,1078.42693336289,
458.985685888084));
#106829=CARTESIAN_POINT('Ctrl Pts',(-89.063441455711,1078.42692789351,458.968639676382));
#106830=CARTESIAN_POINT('Ctrl Pts',(-89.0792381930181,1078.42686416129,
458.93074001787));
#106831=CARTESIAN_POINT('Ctrl Pts',(-89.0885528277506,1078.42679340298,
458.90997503149));
#106832=CARTESIAN_POINT('Ctrl Pts',(-89.117169212609,1078.42648547986,458.850495787964));
#106833=CARTESIAN_POINT('Ctrl Pts',(-89.1378904705034,1078.42615605814,
458.812500967417));
#106834=CARTESIAN_POINT('Ctrl Pts',(-89.2494795984902,1078.42390412161,
458.630548929456));
#106835=CARTESIAN_POINT('Ctrl Pts',(-89.3665830069868,1078.42017199183,
458.504765896987));
#106836=CARTESIAN_POINT('Ctrl Pts',(-89.6158695020872,1078.41020970943,
458.326138649693));
#106837=CARTESIAN_POINT('Ctrl Pts',(-89.7388956965627,1078.4046794168,458.264963799376));
#106838=CARTESIAN_POINT('Ctrl Pts',(-89.9918262523886,1078.39212139507,
458.18635595696));
#106839=CARTESIAN_POINT('Ctrl Pts',(-90.1194443891827,1078.38527238758,
458.166992409975));
#106840=CARTESIAN_POINT('Ctrl Pts',(-90.2477595453605,1078.37785269114,
458.166992409975));
#106841=CARTESIAN_POINT('Ctrl Pts',(-90.2477595453605,1078.37785269114,
458.166992409974));
#106842=CARTESIAN_POINT('Ctrl Pts',(-90.2478324244995,1078.37784847698,
458.166992409974));
#106843=CARTESIAN_POINT('Ctrl Pts',(-90.2479053038633,1078.37784426263,
458.166992416221));
#106844=CARTESIAN_POINT('Ctrl Pts',(-90.2479781834512,1078.3778400481,458.166992428714));
#106845=CARTESIAN_POINT('Ctrl Pts',(-90.4072919887955,1078.36862713961,
458.167019738469));
#106846=CARTESIAN_POINT('Ctrl Pts',(-90.5651677819751,1078.35867654221,
458.196895678002));
#106847=CARTESIAN_POINT('Ctrl Pts',(-90.8708241345389,1078.33764553449,
458.316767158458));
#106848=CARTESIAN_POINT('Ctrl Pts',(-91.0144005994746,1078.3267382461,458.409182948326));
#106849=CARTESIAN_POINT('Ctrl Pts',(-91.2543332497696,1078.30637298371,
458.641908303166));
#106850=CARTESIAN_POINT('Ctrl Pts',(-91.3494706778114,1078.29708088055,
458.778881164629));
#106851=CARTESIAN_POINT('Ctrl Pts',(-91.4710865323649,1078.28258952335,
459.056231867705));
#106852=CARTESIAN_POINT('Ctrl Pts',(-91.5056040365209,1078.27706244958,
459.190374667953));
#106853=CARTESIAN_POINT('Ctrl Pts',(-91.5295395049849,1078.26895951083,
459.454844678659));
#106854=CARTESIAN_POINT('Ctrl Pts',(-91.5218465515413,1078.26624929941,
459.583252359866));
#106855=CARTESIAN_POINT('Ctrl Pts',(-91.4874400031134,1078.26444461224,
459.744635337777));
#106856=CARTESIAN_POINT('Ctrl Pts',(-91.4781338890357,1078.26414997498,
459.780535424518));
#106857=CARTESIAN_POINT('Ctrl Pts',(-91.4609077268045,1078.26386000067,
459.836774160456));
#106858=CARTESIAN_POINT('Ctrl Pts',(-91.4540075142604,1078.26379133509,
459.857402221682));
#106859=CARTESIAN_POINT('Ctrl Pts',(-91.4402753088666,1078.2637358018,459.89521162881));
#106860=CARTESIAN_POINT('Ctrl Pts',(-91.4335907385148,1078.26373819291,
459.912440272066));
#106861=CARTESIAN_POINT('Ctrl Pts',(-91.4179825895442,1078.26380518905,
459.95021322715));
#106862=CARTESIAN_POINT('Ctrl Pts',(-91.4088874623377,1078.2638828574,459.970679935325));
#106863=CARTESIAN_POINT('Ctrl Pts',(-91.3816603578278,1078.26421798958,
460.027843598228));
#106864=CARTESIAN_POINT('Ctrl Pts',(-91.3622948627012,1078.26457087229,
460.06392130448));
#106865=CARTESIAN_POINT('Ctrl Pts',(-91.2535722720426,1078.26708713234,
460.244991450979));
#106866=CARTESIAN_POINT('Ctrl Pts',(-91.1375908418323,1078.27142677595,
460.371909259997));
#106867=CARTESIAN_POINT('Ctrl Pts',(-90.89063281603,1078.28278378677,460.552335975317));
#106868=CARTESIAN_POINT('Ctrl Pts',(-90.7690567174844,1078.28900377703,
460.614352732602));
#106869=CARTESIAN_POINT('Ctrl Pts',(-90.513202878717,1078.30310708823,460.697055991285));
#106870=CARTESIAN_POINT('Ctrl Pts',(-90.380825036293,1078.31086823689,460.717880652247));
#106871=CARTESIAN_POINT('Ctrl Pts',(-90.2477595453603,1078.31906551735,
460.717880652247));
#106872=CARTESIAN_POINT('',(-86.3230601853152,1078.66271960918,449.952384165744));
#106873=CARTESIAN_POINT('',(-86.3230601853153,1078.68303149632,446.995777901357));
#106874=CARTESIAN_POINT('Ctrl Pts',(-86.3230601853152,1078.66271960918,
449.952384165744));
#106875=CARTESIAN_POINT('Ctrl Pts',(-86.3219893136851,1078.66274837852,
449.952384165744));
#106876=CARTESIAN_POINT('Ctrl Pts',(-86.3209183914346,1078.66277714952,
449.952383002147));
#106877=CARTESIAN_POINT('Ctrl Pts',(-86.1332083697891,1078.66782014887,
449.951975054968));
#106878=CARTESIAN_POINT('Ctrl Pts',(-85.9483182623366,1078.6727868702,449.916227592599));
#106879=CARTESIAN_POINT('Ctrl Pts',(-85.5935530569033,1078.6822529705,449.774602911678));
#106880=CARTESIAN_POINT('Ctrl Pts',(-85.4282654883527,1078.68662678793,
449.666930277804));
#106881=CARTESIAN_POINT('Ctrl Pts',(-85.1536649443362,1078.69400200111,
449.397993711266));
#106882=CARTESIAN_POINT('Ctrl Pts',(-85.0452361752256,1078.69698175616,
449.241070641324));
#106883=CARTESIAN_POINT('Ctrl Pts',(-84.8998827329711,1078.70144206657,
448.909744723854));
#106884=CARTESIAN_POINT('Ctrl Pts',(-84.8587403413835,1078.70300008527,
448.74055367043));
#106885=CARTESIAN_POINT('Ctrl Pts',(-84.8414343770874,1078.70461263675,
448.46900283252));
#106886=CARTESIAN_POINT('Ctrl Pts',(-84.8451198713728,1078.70502007381,
448.369517451852));
#106887=CARTESIAN_POINT('Ctrl Pts',(-84.8638170256399,1078.70533761927,
448.234599199511));
#106888=CARTESIAN_POINT('Ctrl Pts',(-84.870250125856,1078.70539915702,448.198245783733));
#106889=CARTESIAN_POINT('Ctrl Pts',(-84.8830601167758,1078.70546027829,
448.138899337221));
#106890=CARTESIAN_POINT('Ctrl Pts',(-84.8886448447503,1078.7054740855,448.115752136688));
#106891=CARTESIAN_POINT('Ctrl Pts',(-84.9005336739799,1078.70548116606,
448.071222576539));
#106892=CARTESIAN_POINT('Ctrl Pts',(-84.9067671709716,1078.70547569801,
448.049827914266));
#106893=CARTESIAN_POINT('Ctrl Pts',(-84.9223509492737,1078.70544236374,
448.000520122945));
#106894=CARTESIAN_POINT('Ctrl Pts',(-84.9320560671682,1078.70540788418,
447.972729020238));
#106895=CARTESIAN_POINT('Ctrl Pts',(-84.9650283518623,1078.70525120061,
447.886657824034));
#106896=CARTESIAN_POINT('Ctrl Pts',(-84.9911794707813,1078.70507413603,
447.829557798599));
#106897=CARTESIAN_POINT('Ctrl Pts',(-85.1138785811796,1078.70404784773,
447.601236637608));
#106898=CARTESIAN_POINT('Ctrl Pts',(-85.2404477033097,1078.70258807734,
447.448447719624));
#106899=CARTESIAN_POINT('Ctrl Pts',(-85.5180168122914,1078.69859589733,
447.223849449712));
#106900=CARTESIAN_POINT('Ctrl Pts',(-85.6584950184123,1078.69632926921,
447.143846921644));
#106901=CARTESIAN_POINT('Ctrl Pts',(-85.973574281774,1078.69057592466,447.027006745919));
#106902=CARTESIAN_POINT('Ctrl Pts',(-86.1476258600309,1078.68703696195,
446.995777901357));
#106903=CARTESIAN_POINT('Ctrl Pts',(-86.3230601853154,1078.68303149632,
446.995777901357));
#106904=CARTESIAN_POINT('Ctrl Pts',(-86.3230601853153,1078.68303149632,
446.995777901357));
#106905=CARTESIAN_POINT('Ctrl Pts',(-86.3231037532579,1078.68303050158,
446.995777901357));
#106906=CARTESIAN_POINT('Ctrl Pts',(-86.3231473212856,1078.68302950683,
446.995777903283));
#106907=CARTESIAN_POINT('Ctrl Pts',(-86.3231908893986,1078.68302851204,
446.995777907135));
#106908=CARTESIAN_POINT('Ctrl Pts',(-86.5113795548305,1078.67873161425,
446.995794545825));
#106909=CARTESIAN_POINT('Ctrl Pts',(-86.6978364457682,1078.67397007578,
447.031745567121));
#106910=CARTESIAN_POINT('Ctrl Pts',(-87.0537013248571,1078.66381058891,
447.174223629047));
#106911=CARTESIAN_POINT('Ctrl Pts',(-87.2187323359064,1078.65849680364,
447.281924061899));
#106912=CARTESIAN_POINT('Ctrl Pts',(-87.4924716008461,1078.64859012056,
447.550346108494));
#106913=CARTESIAN_POINT('Ctrl Pts',(-87.6004774446379,1078.64407484309,
447.70660239725));
#106914=CARTESIAN_POINT('Ctrl Pts',(-87.7457840386515,1078.6368402648,448.036984561462));
#106915=CARTESIAN_POINT('Ctrl Pts',(-87.7870783246366,1078.63406305431,
448.20602200215));
#106916=CARTESIAN_POINT('Ctrl Pts',(-87.8046993616625,1078.63111784649,
448.477581050921));
#106917=CARTESIAN_POINT('Ctrl Pts',(-87.8011107850664,1078.6303496369,448.577203692244));
#106918=CARTESIAN_POINT('Ctrl Pts',(-87.7824753157512,1078.62974695066,
448.712557434865));
#106919=CARTESIAN_POINT('Ctrl Pts',(-87.7760135969678,1078.62962913423,
448.749199048912));
#106920=CARTESIAN_POINT('Ctrl Pts',(-87.7631010239068,1078.6295119873,448.809107730244));
#106921=CARTESIAN_POINT('Ctrl Pts',(-87.7574502758618,1078.62948555117,
448.832529878704));
#106922=CARTESIAN_POINT('Ctrl Pts',(-87.7453884064107,1078.62947240845,
448.877657941451));
#106923=CARTESIAN_POINT('Ctrl Pts',(-87.7390462559079,1078.62948337909,
448.899375444873));
#106924=CARTESIAN_POINT('Ctrl Pts',(-87.7231398310093,1078.62954918598,
448.949535715553));
#106925=CARTESIAN_POINT('Ctrl Pts',(-87.7132030298227,1078.62961715035,
448.977849862148));
#106926=CARTESIAN_POINT('Ctrl Pts',(-87.679228711486,1078.62992641947,449.065976923457));
#106927=CARTESIAN_POINT('Ctrl Pts',(-87.6521383269708,1078.63027691846,
449.124530815579));
#106928=CARTESIAN_POINT('Ctrl Pts',(-87.5272729774475,1078.63224471684,
449.35380373895));
#106929=CARTESIAN_POINT('Ctrl Pts',(-87.3997279375185,1078.6349729785,449.505980258295));
#106930=CARTESIAN_POINT('Ctrl Pts',(-87.1210580936803,1078.64166558737,
449.728767677051));
#106931=CARTESIAN_POINT('Ctrl Pts',(-86.9805207319876,1078.64525869543,
449.807789584479));
#106932=CARTESIAN_POINT('Ctrl Pts',(-86.6676033718544,1078.65346701037,
449.922039748485));
#106933=CARTESIAN_POINT('Ctrl Pts',(-86.4959918761742,1078.65807373949,
449.952384165744));
#106934=CARTESIAN_POINT('Ctrl Pts',(-86.3230601853152,1078.66271960918,
449.952384165744));
#106935=CARTESIAN_POINT('',(-69.1578093449745,1078.64674583663,483.000863198568));
#106936=CARTESIAN_POINT('',(-69.1578093449747,1078.69514019783,480.044256934181));
#106937=CARTESIAN_POINT('Ctrl Pts',(-69.1578093449745,1078.64674583663,
483.000863198568));
#106938=CARTESIAN_POINT('Ctrl Pts',(-69.1220937668084,1078.64759196713,
483.000863198568));
#106939=CARTESIAN_POINT('Ctrl Pts',(-69.0863498276105,1078.64845820303,
482.99956888825));
#106940=CARTESIAN_POINT('Ctrl Pts',(-68.8768662085712,1078.6536434673,482.984343449551));
#106941=CARTESIAN_POINT('Ctrl Pts',(-68.7066832936626,1078.65829077859,
482.941088098396));
#106942=CARTESIAN_POINT('Ctrl Pts',(-68.3777949600251,1078.66799062584,
482.792148860044));
#106943=CARTESIAN_POINT('Ctrl Pts',(-68.2237562448034,1078.67295694628,
482.683519495698));
#106944=CARTESIAN_POINT('Ctrl Pts',(-67.9583997108454,1078.68240848418,
482.408532395796));
#106945=CARTESIAN_POINT('Ctrl Pts',(-67.8519529437903,1078.68676874044,
482.242475741192));
#106946=CARTESIAN_POINT('Ctrl Pts',(-67.7121084334976,1078.69411350738,
481.884538077247));
#106947=CARTESIAN_POINT('Ctrl Pts',(-67.6777201905111,1078.69707705634,
481.696980993371));
#106948=CARTESIAN_POINT('Ctrl Pts',(-67.6813191949551,1078.70156116495,
481.330864883684));
#106949=CARTESIAN_POINT('Ctrl Pts',(-67.7148960065625,1078.70312947517,
481.155443117896));
#106950=CARTESIAN_POINT('Ctrl Pts',(-67.8118699942329,1078.70466121946,
480.904251222763));
#106951=CARTESIAN_POINT('Ctrl Pts',(-67.8529853071337,1078.70502962209,
480.821637090225));
#106952=CARTESIAN_POINT('Ctrl Pts',(-67.921526960054,1078.7053360895,480.711124816198));
#106953=CARTESIAN_POINT('Ctrl Pts',(-67.942771262791,1078.70539962805,480.679646211886));
#106954=CARTESIAN_POINT('Ctrl Pts',(-67.9788928060586,1078.70546039652,
480.63033104458));
#106955=CARTESIAN_POINT('Ctrl Pts',(-67.9930194307043,1078.70547380595,
480.611966145203));
#106956=CARTESIAN_POINT('Ctrl Pts',(-68.0230900753445,1078.70548165651,
480.574719032977));
#106957=CARTESIAN_POINT('Ctrl Pts',(-68.0390877603405,1078.70547477867,
480.555889253051));
#106958=CARTESIAN_POINT('Ctrl Pts',(-68.0773204176942,1078.70543340838,
480.51310912399));
#106959=CARTESIAN_POINT('Ctrl Pts',(-68.0998926254822,1078.70539074163,
480.489477427577));
#106960=CARTESIAN_POINT('Ctrl Pts',(-68.1729193002667,1078.70519722749,
480.417928429381));
#106961=CARTESIAN_POINT('Ctrl Pts',(-68.2259837965977,1078.7049790155,480.372812039255));
#106962=CARTESIAN_POINT('Ctrl Pts',(-68.4405702555798,1078.7038067604,480.215014037646));
#106963=CARTESIAN_POINT('Ctrl Pts',(-68.6208052854813,1078.70225534419,
480.131254604214));
#106964=CARTESIAN_POINT('Ctrl Pts',(-68.9253462279713,1078.69860635502,
480.05801257821));
#106965=CARTESIAN_POINT('Ctrl Pts',(-69.0413762084877,1078.69700068759,
480.044256934181));
#106966=CARTESIAN_POINT('Ctrl Pts',(-69.1578093449746,1078.69514019783,
480.044256934181));
#106967=CARTESIAN_POINT('Ctrl Pts',(-69.1578093449747,1078.69514019783,
480.044256934181));
#106968=CARTESIAN_POINT('Ctrl Pts',(-69.1578255873479,1078.69513993829,
480.044256934181));
#106969=CARTESIAN_POINT('Ctrl Pts',(-69.1578418297291,1078.69513967875,
480.044256934449));
#106970=CARTESIAN_POINT('Ctrl Pts',(-69.157858072118,1078.6951394192,480.044256934984));
#106971=CARTESIAN_POINT('Ctrl Pts',(-69.3304172925023,1078.69238198582,
480.044262622801));
#106972=CARTESIAN_POINT('Ctrl Pts',(-69.5016402651383,1078.68909651496,
480.074481766387));
#106973=CARTESIAN_POINT('Ctrl Pts',(-69.8382050392031,1078.68127504934,
480.197075232476));
#106974=CARTESIAN_POINT('Ctrl Pts',(-69.9991185706044,1078.67672836683,
480.292909581556));
#106975=CARTESIAN_POINT('Ctrl Pts',(-70.2844405337472,1078.66679166732,
480.545668199062));
#106976=CARTESIAN_POINT('Ctrl Pts',(-70.4036363608493,1078.66146765396,
480.70309082141));
#106977=CARTESIAN_POINT('Ctrl Pts',(-70.5717345936668,1078.65128240561,
481.050804271054));
#106978=CARTESIAN_POINT('Ctrl Pts',(-70.6207385150725,1078.64651419783,
481.236929995868));
#106979=CARTESIAN_POINT('Ctrl Pts',(-70.643809200598,1078.63883572837,481.593955476461));
#106980=CARTESIAN_POINT('Ctrl Pts',(-70.6262425150681,1078.6358277134,481.761316621795));
#106981=CARTESIAN_POINT('Ctrl Pts',(-70.5469147492507,1078.63195396571,
482.043838842373));
#106982=CARTESIAN_POINT('Ctrl Pts',(-70.4973005612334,1078.63076075498,
482.160612556531));
#106983=CARTESIAN_POINT('Ctrl Pts',(-70.4112452026124,1078.62986506717,
482.307548963095));
#106984=CARTESIAN_POINT('Ctrl Pts',(-70.3873719454327,1078.62969817139,
482.344438933343));
#106985=CARTESIAN_POINT('Ctrl Pts',(-70.3460392107666,1078.62953296329,
482.40246719796));
#106986=CARTESIAN_POINT('Ctrl Pts',(-70.3295726739802,1078.62949480491,
482.424279246017));
#106987=CARTESIAN_POINT('Ctrl Pts',(-70.2969879577151,1078.62947022325,
482.465040988458));
#106988=CARTESIAN_POINT('Ctrl Pts',(-70.2809774640063,1078.62947944854,
482.48406491604));
#106989=CARTESIAN_POINT('Ctrl Pts',(-70.2434089302868,1078.62954815663,
482.526484950677));
#106990=CARTESIAN_POINT('Ctrl Pts',(-70.2215602004611,1078.62962094107,
482.549607163961));
#106991=CARTESIAN_POINT('Ctrl Pts',(-70.1534914889801,1078.62994290845,
482.617139272593));
#106992=CARTESIAN_POINT('Ctrl Pts',(-70.1051142213755,1078.630295898,482.659265768164));
#106993=CARTESIAN_POINT('Ctrl Pts',(-69.8972925153034,1078.63228055406,
482.817726952498));
#106994=CARTESIAN_POINT('Ctrl Pts',(-69.7180755427923,1078.63503192318,
482.904726208679));
#106995=CARTESIAN_POINT('Ctrl Pts',(-69.4063231087205,1078.64109433978,
482.9851528028));
#106996=CARTESIAN_POINT('Ctrl Pts',(-69.2822383408889,1078.64379801457,
483.000863198568));
#106997=CARTESIAN_POINT('Ctrl Pts',(-69.1578093449745,1078.64674583663,
483.000863198568));
#106998=CARTESIAN_POINT('',(-68.281968522817,1078.28930526318,494.414414572902));
#106999=CARTESIAN_POINT('',(-68.2819685228173,1078.40494192759,491.86352633063));
#107000=CARTESIAN_POINT('Ctrl Pts',(-68.2819685228169,1078.28930526318,
494.414414572903));
#107001=CARTESIAN_POINT('Ctrl Pts',(-68.2268299973128,1078.29194915715,
494.414414572903));
#107002=CARTESIAN_POINT('Ctrl Pts',(-68.1716716781174,1078.2947564259,494.410839066877));
#107003=CARTESIAN_POINT('Ctrl Pts',(-67.9689152532529,1078.30566708968,
494.384366341749));
#107004=CARTESIAN_POINT('Ctrl Pts',(-67.8255576261282,1078.3145504416,494.339253502769));
#107005=CARTESIAN_POINT('Ctrl Pts',(-67.5511678987433,1078.33392330302,
494.196492245403));
#107006=CARTESIAN_POINT('Ctrl Pts',(-67.4242506988773,1078.34431070701,
494.096435629777));
#107007=CARTESIAN_POINT('Ctrl Pts',(-67.2084150268444,1078.36520475051,
493.848027835637));
#107008=CARTESIAN_POINT('Ctrl Pts',(-67.1240358591932,1078.37548319379,
493.699772664207));
#107009=CARTESIAN_POINT('Ctrl Pts',(-67.0194581552401,1078.393793904,493.383468981787));
#107010=CARTESIAN_POINT('Ctrl Pts',(-66.9984816421114,1078.40171502936,
493.219040849127));
#107011=CARTESIAN_POINT('Ctrl Pts',(-67.0189661114801,1078.41399807541,
492.908188050846));
#107012=CARTESIAN_POINT('Ctrl Pts',(-67.0540168145405,1078.41855449535,
492.764013049827));
#107013=CARTESIAN_POINT('Ctrl Pts',(-67.1516743758756,1078.42381114958,
492.540148623869));
#107014=CARTESIAN_POINT('Ctrl Pts',(-67.2004349724833,1078.42527980687,
492.45600542429));
#107015=CARTESIAN_POINT('Ctrl Pts',(-67.2795034245054,1078.42641946076,
492.349610104343));
#107016=CARTESIAN_POINT('Ctrl Pts',(-67.3019344077776,1078.42663933247,
492.321927465234));
#107017=CARTESIAN_POINT('Ctrl Pts',(-67.3405658070389,1078.42685775428,
492.278135013906));
#107018=CARTESIAN_POINT('Ctrl Pts',(-67.3560919764303,1078.42690746162,
492.261457287901));
#107019=CARTESIAN_POINT('Ctrl Pts',(-67.3868845947875,1078.42693479384,
492.23010840154));
#107020=CARTESIAN_POINT('Ctrl Pts',(-67.4020860214614,1078.42691729369,
492.215383830676));
#107021=CARTESIAN_POINT('Ctrl Pts',(-67.4380043830343,1078.4268061449,492.182284184333));
#107022=CARTESIAN_POINT('Ctrl Pts',(-67.4589673129964,1078.42669071656,
492.164191980125));
#107023=CARTESIAN_POINT('Ctrl Pts',(-67.5255311999959,1078.42617220555,
492.110422463409));
#107024=CARTESIAN_POINT('Ctrl Pts',(-67.572982585475,1078.42559337072,492.077157468938));
#107025=CARTESIAN_POINT('Ctrl Pts',(-67.6866117922098,1078.42374835658,
492.008522129749));
#107026=CARTESIAN_POINT('Ctrl Pts',(-67.7539752922965,1078.42233399342,
491.975534101653));
#107027=CARTESIAN_POINT('Ctrl Pts',(-67.9700643467163,1078.41683480429,
491.892365402126));
#107028=CARTESIAN_POINT('Ctrl Pts',(-68.1253745050975,1078.4115692788,491.86352633063));
#107029=CARTESIAN_POINT('Ctrl Pts',(-68.2819685228173,1078.40494192759,
491.86352633063));
#107030=CARTESIAN_POINT('Ctrl Pts',(-68.2819685228173,1078.40494192759,
491.86352633063));
#107031=CARTESIAN_POINT('Ctrl Pts',(-68.2819829283623,1078.40494131792,
491.86352633063));
#107032=CARTESIAN_POINT('Ctrl Pts',(-68.2819973339181,1078.40494070824,
491.863526330874));
#107033=CARTESIAN_POINT('Ctrl Pts',(-68.2820117394848,1078.40494009854,
491.863526331362));
#107034=CARTESIAN_POINT('Ctrl Pts',(-68.4272840304119,1078.39879168051,
491.863531253714));
#107035=CARTESIAN_POINT('Ctrl Pts',(-68.5714448488071,1078.39156228246,
491.888355050204));
#107036=CARTESIAN_POINT('Ctrl Pts',(-68.856114368212,1078.37478838096,491.989310049922));
#107037=CARTESIAN_POINT('Ctrl Pts',(-68.9929838731265,1078.36524384175,
492.06855112643));
#107038=CARTESIAN_POINT('Ctrl Pts',(-69.2401818060572,1078.34460579562,
492.280439104039));
#107039=CARTESIAN_POINT('Ctrl Pts',(-69.3452689297273,1078.33364938682,
492.414647381526));
#107040=CARTESIAN_POINT('Ctrl Pts',(-69.4961255434096,1078.31268815387,
492.714283929801));
#107041=CARTESIAN_POINT('Ctrl Pts',(-69.5411959190575,1078.30287512033,
492.876452206662));
#107042=CARTESIAN_POINT('Ctrl Pts',(-69.5651285669973,1078.28658287664,
493.192770983976));
#107043=CARTESIAN_POINT('Ctrl Pts',(-69.5498486225684,1078.28000195096,
493.343683187072));
#107044=CARTESIAN_POINT('Ctrl Pts',(-69.4699801429818,1078.27021897769,
493.62398246855));
#107045=CARTESIAN_POINT('Ctrl Pts',(-69.4091759352283,1078.26689649371,
493.752183733321));
#107046=CARTESIAN_POINT('Ctrl Pts',(-69.3047151517117,1078.26463987754,
493.902185344627));
#107047=CARTESIAN_POINT('Ctrl Pts',(-69.2791339195289,1078.26426398191,
493.935317753207));
#107048=CARTESIAN_POINT('Ctrl Pts',(-69.2359818467912,1078.2638929568,493.985860400982));
#107049=CARTESIAN_POINT('Ctrl Pts',(-69.2194546082755,1078.26380487283,
494.004120072329));
#107050=CARTESIAN_POINT('Ctrl Pts',(-69.1879156040516,1078.26373353815,
494.036999374624));
#107051=CARTESIAN_POINT('Ctrl Pts',(-69.1730522981399,1078.26373657664,
494.051749595717));
#107052=CARTESIAN_POINT('Ctrl Pts',(-69.1393976081116,1078.2638224945,494.083542423332));
#107053=CARTESIAN_POINT('Ctrl Pts',(-69.1204473950492,1078.26392208766,
494.100403760098));
#107054=CARTESIAN_POINT('Ctrl Pts',(-69.0655984514433,1078.26435079716,
494.146350951707));
#107055=CARTESIAN_POINT('Ctrl Pts',(-69.0286056692421,1078.26480095416,
494.174066583747));
#107056=CARTESIAN_POINT('Ctrl Pts',(-68.8491702885579,1078.26770143216,
494.293869834285));
#107057=CARTESIAN_POINT('Ctrl Pts',(-68.6908257250236,1078.27225785884,
494.358933903536));
#107058=CARTESIAN_POINT('Ctrl Pts',(-68.4444135365115,1078.2818687177,494.40665186068));
#107059=CARTESIAN_POINT('Ctrl Pts',(-68.3632125148549,1078.28540961131,
494.414414572903));
#107060=CARTESIAN_POINT('Ctrl Pts',(-68.2819685228169,1078.28930526318,
494.414414572903));
#107061=CARTESIAN_POINT('',(-66.3937896239303,1077.5767973048,506.897628369571));
#107062=CARTESIAN_POINT('',(-66.3937896239306,1077.7522985528,504.699966097586));
#107063=CARTESIAN_POINT('Ctrl Pts',(-66.3937896239303,1077.5767973048,506.897628369571));
#107064=CARTESIAN_POINT('Ctrl Pts',(-66.3853559678242,1077.57736420966,
506.897628369571));
#107065=CARTESIAN_POINT('Ctrl Pts',(-66.3769184655453,1077.57793920547,
506.8975312759));
#107066=CARTESIAN_POINT('Ctrl Pts',(-66.2463058532424,1077.586961466,506.894521901349));
#107067=CARTESIAN_POINT('Ctrl Pts',(-66.1255620075913,1077.59694399031,
506.871349468675));
#107068=CARTESIAN_POINT('Ctrl Pts',(-65.8870614803648,1077.62003119709,
506.782764275726));
#107069=CARTESIAN_POINT('Ctrl Pts',(-65.7723496933046,1077.63314310058,
506.714624527884));
#107070=CARTESIAN_POINT('Ctrl Pts',(-65.5651978050541,1077.66124918253,
506.534401986959));
#107071=CARTESIAN_POINT('Ctrl Pts',(-65.4769865219931,1077.67605382795,
506.421019613032));
#107072=CARTESIAN_POINT('Ctrl Pts',(-65.3475489881898,1077.70475069346,
506.164595790279));
#107073=CARTESIAN_POINT('Ctrl Pts',(-65.3084300766143,1077.71835008719,
506.023488598657));
#107074=CARTESIAN_POINT('Ctrl Pts',(-65.2879564868442,1077.74157487067,
505.742844215521));
#107075=CARTESIAN_POINT('Ctrl Pts',(-65.3033985549367,1077.75119462358,
505.606152551454));
#107076=CARTESIAN_POINT('Ctrl Pts',(-65.3860865330705,1077.7667390475,505.33738744492));
#107077=CARTESIAN_POINT('Ctrl Pts',(-65.4555593111009,1077.77225545012,
505.208761274875));
#107078=CARTESIAN_POINT('Ctrl Pts',(-65.5706518389485,1077.77568246524,
505.070012687636));
#107079=CARTESIAN_POINT('Ctrl Pts',(-65.5945547767765,1077.77618820348,
505.043875559786));
#107080=CARTESIAN_POINT('Ctrl Pts',(-65.6358852820681,1077.77674264264,
505.002849821875));
#107081=CARTESIAN_POINT('Ctrl Pts',(-65.6525891034229,1077.77688971025,
504.987272060215));
#107082=CARTESIAN_POINT('Ctrl Pts',(-65.6833669877132,1077.7770268665,504.96031262419));
#107083=CARTESIAN_POINT('Ctrl Pts',(-65.6972595005272,1077.77704324399,
504.948736909486));
#107084=CARTESIAN_POINT('Ctrl Pts',(-65.7271925313,1077.77698438522,504.925022366546));
#107085=CARTESIAN_POINT('Ctrl Pts',(-65.7432933581614,1077.77689868045,
504.912970617086));
#107086=CARTESIAN_POINT('Ctrl Pts',(-65.7865327726175,1077.77652918517,
504.882420045287));
#107087=CARTESIAN_POINT('Ctrl Pts',(-65.814184471588,1077.77615454949,504.864684984899));
#107088=CARTESIAN_POINT('Ctrl Pts',(-65.9355076578786,1077.77393708599,
504.794334767766));
#107089=CARTESIAN_POINT('Ctrl Pts',(-66.0357896988928,1077.77070569018,
504.754390776742));
#107090=CARTESIAN_POINT('Ctrl Pts',(-66.2233464398009,1077.76231141693,
504.709908902157));
#107091=CARTESIAN_POINT('Ctrl Pts',(-66.3084454335179,1077.75770593228,
504.699966097586));
#107092=CARTESIAN_POINT('Ctrl Pts',(-66.3937896239306,1077.7522985528,504.699966097586));
#107093=CARTESIAN_POINT('Ctrl Pts',(-66.3937896239306,1077.7522985528,504.699966097586));
#107094=CARTESIAN_POINT('Ctrl Pts',(-66.3938084673047,1077.75229735889,
504.699966097586));
#107095=CARTESIAN_POINT('Ctrl Pts',(-66.3938273106907,1077.75229616494,
504.699966098071));
#107096=CARTESIAN_POINT('Ctrl Pts',(-66.3938461540887,1077.75229497095,
504.69996609904));
#107097=CARTESIAN_POINT('Ctrl Pts',(-66.5156065443393,1077.74457977763,
504.699972363091));
#107098=CARTESIAN_POINT('Ctrl Pts',(-66.6364182768944,1077.73532348152,
504.720215429604));
#107099=CARTESIAN_POINT('Ctrl Pts',(-66.8764665702453,1077.71349650879,
504.802826892518));
#107100=CARTESIAN_POINT('Ctrl Pts',(-66.992684073827,1077.70087981196,504.86809095845));
#107101=CARTESIAN_POINT('Ctrl Pts',(-67.2041756848766,1077.67328580985,
505.043160212084));
#107102=CARTESIAN_POINT('Ctrl Pts',(-67.2951805003475,1077.65845238968,
505.154435897107));
#107103=CARTESIAN_POINT('Ctrl Pts',(-67.4308921457612,1077.62913719015,
505.40779887864));
#107104=CARTESIAN_POINT('Ctrl Pts',(-67.4734317282079,1077.61494517145,
505.548020848206));
#107105=CARTESIAN_POINT('Ctrl Pts',(-67.500710521595,1077.59022855711,505.828823720037));
#107106=CARTESIAN_POINT('Ctrl Pts',(-67.4883762012569,1077.57975598967,
505.966508905856));
#107107=CARTESIAN_POINT('Ctrl Pts',(-67.4125473874403,1077.56284062142,
506.234002406126));
#107108=CARTESIAN_POINT('Ctrl Pts',(-67.3484000506283,1077.55667530757,
506.360980143391));
#107109=CARTESIAN_POINT('Ctrl Pts',(-67.2363282566319,1077.55230743023,
506.505409444125));
#107110=CARTESIAN_POINT('Ctrl Pts',(-67.208878139826,1077.55155830391,506.536905377716));
#107111=CARTESIAN_POINT('Ctrl Pts',(-67.16403020963,1077.55079497178,506.582801028961));
#107112=CARTESIAN_POINT('Ctrl Pts',(-67.1478735815684,1077.55060126855,
506.59835333289));
#107113=CARTESIAN_POINT('Ctrl Pts',(-67.1174308896334,1077.55038077494,
506.625913165198));
#107114=CARTESIAN_POINT('Ctrl Pts',(-67.1032934568024,1077.55033139792,
506.638071783022));
#107115=CARTESIAN_POINT('Ctrl Pts',(-67.0741656131291,1077.55033423883,
506.661860383956));
#107116=CARTESIAN_POINT('Ctrl Pts',(-67.0591698389931,1077.55038821396,
506.673473544454));
#107117=CARTESIAN_POINT('Ctrl Pts',(-67.021952643986,1077.55064735473,506.700784421853));
#107118=CARTESIAN_POINT('Ctrl Pts',(-66.9994350087688,1077.5509079106,506.716055773345));
#107119=CARTESIAN_POINT('Ctrl Pts',(-66.9193343639818,1077.55218544493,
506.766143298981));
#107120=CARTESIAN_POINT('Ctrl Pts',(-66.8591513321462,1077.55374861682,
506.796489695749));
#107121=CARTESIAN_POINT('Ctrl Pts',(-66.6681341490792,1077.56044538203,
506.871749450635));
#107122=CARTESIAN_POINT('Ctrl Pts',(-66.5314743793487,1077.56754222529,
506.897628369571));
#107123=CARTESIAN_POINT('Ctrl Pts',(-66.3937896239304,1077.5767973048,506.897628369571));
#107124=CARTESIAN_POINT('',(-62.0518715958015,1076.69664647652,518.930937549326));
#107125=CARTESIAN_POINT('',(-62.0518715958009,1076.94043266168,516.749856051871));
#107126=CARTESIAN_POINT('Ctrl Pts',(-62.0518715958021,1076.69664647652,
518.930937549327));
#107127=CARTESIAN_POINT('Ctrl Pts',(-62.0309428736203,1076.69823468214,
518.930937549327));
#107128=CARTESIAN_POINT('Ctrl Pts',(-62.0099972381441,1076.69989227498,
518.93033508609));
#107129=CARTESIAN_POINT('Ctrl Pts',(-61.8702596372939,1076.71140673666,
518.922273344549));
#107130=CARTESIAN_POINT('Ctrl Pts',(-61.7535543466491,1076.72322347486,
518.896032706119));
#107131=CARTESIAN_POINT('Ctrl Pts',(-61.5232595973848,1076.75112850709,
518.803033990147));
#107132=CARTESIAN_POINT('Ctrl Pts',(-61.4127569856185,1076.76729365557,
518.733459504443));
#107133=CARTESIAN_POINT('Ctrl Pts',(-61.2139218145621,1076.80255979482,
518.552171175206));
#107134=CARTESIAN_POINT('Ctrl Pts',(-61.1297606841958,1076.82148425931,
518.439134765405));
#107135=CARTESIAN_POINT('Ctrl Pts',(-61.0064647608932,1076.85917061545,
518.182943057433));
#107136=CARTESIAN_POINT('Ctrl Pts',(-60.9702209374447,1076.87755055723,
518.041234693432));
#107137=CARTESIAN_POINT('Ctrl Pts',(-60.9556737561427,1076.90983262079,
517.75846838187));
#107138=CARTESIAN_POINT('Ctrl Pts',(-60.9748424773294,1076.92362217153,
517.62019281886));
#107139=CARTESIAN_POINT('Ctrl Pts',(-61.0621948369667,1076.94537645386,
517.363549963148));
#107140=CARTESIAN_POINT('Ctrl Pts',(-61.1274639683931,1076.95338497051,
517.246765259848));
#107141=CARTESIAN_POINT('Ctrl Pts',(-61.2509713977901,1076.96067484561,
517.097751600319));
#107142=CARTESIAN_POINT('Ctrl Pts',(-61.2935481798764,1076.96232004537,
517.054322467613));
#107143=CARTESIAN_POINT('Ctrl Pts',(-61.3597302000752,1076.96374168155,
516.997229572262));
#107144=CARTESIAN_POINT('Ctrl Pts',(-61.3805619022868,1076.96404818309,
516.980551382795));
#107145=CARTESIAN_POINT('Ctrl Pts',(-61.4155780365264,1076.96433999714,
516.954566038484));
#107146=CARTESIAN_POINT('Ctrl Pts',(-61.4294038456974,1076.96440171807,
516.944796696053));
#107147=CARTESIAN_POINT('Ctrl Pts',(-61.4588678731883,1076.96442293565,
516.924989363265));
#107148=CARTESIAN_POINT('Ctrl Pts',(-61.4745463073216,1076.96437188453,
516.91502136754));
#107149=CARTESIAN_POINT('Ctrl Pts',(-61.5123304531631,1076.96410341071,
516.892333209576));
#107150=CARTESIAN_POINT('Ctrl Pts',(-61.5346419319995,1076.96383117584,
516.879978886678));
#107151=CARTESIAN_POINT('Ctrl Pts',(-61.6090510508618,1076.96255842063,
516.842122262473));
#107152=CARTESIAN_POINT('Ctrl Pts',(-61.6627392432878,1076.96107413403,
516.819997545311));
#107153=CARTESIAN_POINT('Ctrl Pts',(-61.8259400467811,1076.95494888004,
516.76749847443));
#107154=CARTESIAN_POINT('Ctrl Pts',(-61.9386176641616,1076.9486863086,516.749856051871));
#107155=CARTESIAN_POINT('Ctrl Pts',(-62.0518715958011,1076.94043266168,
516.749856051871));
#107156=CARTESIAN_POINT('Ctrl Pts',(-62.0518715958011,1076.94043266168,
516.749856051871));
#107157=CARTESIAN_POINT('Ctrl Pts',(-62.0518860945413,1076.94043160505,
516.749856051871));
#107158=CARTESIAN_POINT('Ctrl Pts',(-62.0519005932904,1076.94043054838,
516.749856052221));
#107159=CARTESIAN_POINT('Ctrl Pts',(-62.0519150920495,1076.94042949168,
516.749856052799));
#107160=CARTESIAN_POINT('Ctrl Pts',(-62.1689455307399,1076.93190010702,
516.74986072057));
#107161=CARTESIAN_POINT('Ctrl Pts',(-62.285050312318,1076.92135637129,516.768701950391));
#107162=CARTESIAN_POINT('Ctrl Pts',(-62.5175394541443,1076.89581215433,
516.845968825757));
#107163=CARTESIAN_POINT('Ctrl Pts',(-62.6310190020822,1076.88066991008,
516.907530197521));
#107164=CARTESIAN_POINT('Ctrl Pts',(-62.8394594150589,1076.84686333787,
517.07348046616));
#107165=CARTESIAN_POINT('Ctrl Pts',(-62.9303300689801,1076.82830263051,
517.179540249254));
#107166=CARTESIAN_POINT('Ctrl Pts',(-63.0708671223406,1076.7902651475,517.425692916797));
#107167=CARTESIAN_POINT('Ctrl Pts',(-63.1169984188379,1076.77114306749,
517.564894100113));
#107168=CARTESIAN_POINT('Ctrl Pts',(-63.1513190562355,1076.7365705027,517.848010775854));
#107169=CARTESIAN_POINT('Ctrl Pts',(-63.1413083435132,1076.72131909065,
517.989032987736));
#107170=CARTESIAN_POINT('Ctrl Pts',(-63.0720823829983,1076.69736849267,
518.245588451812));
#107171=CARTESIAN_POINT('Ctrl Pts',(-63.0187168505342,1076.68832791401,
518.360306003776));
#107172=CARTESIAN_POINT('Ctrl Pts',(-62.899836155743,1076.67786005376,518.531054132045));
#107173=CARTESIAN_POINT('Ctrl Pts',(-62.8452960169199,1076.67491672067,
518.59308750105));
#107174=CARTESIAN_POINT('Ctrl Pts',(-62.7615126542785,1076.67260893543,
518.669028856576));
#107175=CARTESIAN_POINT('Ctrl Pts',(-62.7379049398262,1076.67215874285,
518.68867746773));
#107176=CARTESIAN_POINT('Ctrl Pts',(-62.6977606012892,1076.67171059659,
518.71931569315));
#107177=CARTESIAN_POINT('Ctrl Pts',(-62.6816992167771,1076.67160888965,
518.730895664975));
#107178=CARTESIAN_POINT('Ctrl Pts',(-62.6500338078085,1076.6715554871,518.75244034779));
#107179=CARTESIAN_POINT('Ctrl Pts',(-62.6344741045533,1076.67159442363,
518.762457412867));
#107180=CARTESIAN_POINT('Ctrl Pts',(-62.5978415909017,1076.67183458187,
518.784743194191));
#107181=CARTESIAN_POINT('Ctrl Pts',(-62.5765979847648,1076.67208333266,
518.796710272157));
#107182=CARTESIAN_POINT('Ctrl Pts',(-62.5091961101175,1076.67320687118,
518.831757187203));
#107183=CARTESIAN_POINT('Ctrl Pts',(-62.4617991714205,1076.67446907833,
518.852275281));
#107184=CARTESIAN_POINT('Ctrl Pts',(-62.2967790475951,1076.68040509685,
518.910213838104));
#107185=CARTESIAN_POINT('Ctrl Pts',(-62.174616158295,1076.68733183217,518.930937549327));
#107186=CARTESIAN_POINT('Ctrl Pts',(-62.0518715958021,1076.69664647652,
518.930937549327));
#107187=CARTESIAN_POINT('',(-79.4772023228642,1078.65448750233,467.378693963514));
#107188=CARTESIAN_POINT('',(-79.4772023228643,1078.68962000954,464.422087699128));
#107189=CARTESIAN_POINT('Ctrl Pts',(-79.4772023228642,1078.65448750233,
467.378693963514));
#107190=CARTESIAN_POINT('Ctrl Pts',(-79.4699089493478,1078.65467754156,
467.378693963514));
#107191=CARTESIAN_POINT('Ctrl Pts',(-79.4626135119311,1078.65486804194,
467.37863998956));
#107192=CARTESIAN_POINT('Ctrl Pts',(-79.2756436512785,1078.6597605043,467.375871667671));
#107193=CARTESIAN_POINT('Ctrl Pts',(-79.0979527863087,1078.66464638793,
467.340473831258));
#107194=CARTESIAN_POINT('Ctrl Pts',(-78.7518256378851,1078.67449916672,
467.202841918134));
#107195=CARTESIAN_POINT('Ctrl Pts',(-78.5883194849916,1078.67934854359,
467.097238535432));
#107196=CARTESIAN_POINT('Ctrl Pts',(-78.3103484198939,1078.68806921248,
466.828506201587));
#107197=CARTESIAN_POINT('Ctrl Pts',(-78.1988374302271,1078.69185430098,
466.667683721362));
#107198=CARTESIAN_POINT('Ctrl Pts',(-78.0504298588254,1078.69784732802,
466.326410125835));
#107199=CARTESIAN_POINT('Ctrl Pts',(-78.0094872349183,1078.7001144017,466.151368340374));
#107200=CARTESIAN_POINT('Ctrl Pts',(-77.9921230780727,1078.70345252511,
465.799565326274));
#107201=CARTESIAN_POINT('Ctrl Pts',(-78.0142689356406,1078.70453002986,
465.625701199463));
#107202=CARTESIAN_POINT('Ctrl Pts',(-78.0791044252518,1078.70520849538,
465.418104226389));
#107203=CARTESIAN_POINT('Ctrl Pts',(-78.0939238002015,1078.70531014839,
465.377113998268));
#107204=CARTESIAN_POINT('Ctrl Pts',(-78.1214134034484,1078.70542214597,
465.310449007007));
#107205=CARTESIAN_POINT('Ctrl Pts',(-78.1330571459278,1078.70545185736,
465.28438052663));
#107206=CARTESIAN_POINT('Ctrl Pts',(-78.1553956241902,1078.70547912026,
465.23802212617));
#107207=CARTESIAN_POINT('Ctrl Pts',(-78.1658215987045,1078.70548185375,
465.217612795024));
#107208=CARTESIAN_POINT('Ctrl Pts',(-78.1890012309822,1078.70546766202,
465.174728774328));
#107209=CARTESIAN_POINT('Ctrl Pts',(-78.2018782554098,1078.70544819281,
465.152329338921));
#107210=CARTESIAN_POINT('Ctrl Pts',(-78.2377454740045,1078.70536440738,
465.093559117774));
#107211=CARTESIAN_POINT('Ctrl Pts',(-78.2617474687001,1078.70527893133,
465.057835087687));
#107212=CARTESIAN_POINT('Ctrl Pts',(-78.3753394022478,1078.7047501631,464.903743500304));
#107213=CARTESIAN_POINT('Ctrl Pts',(-78.4808956004949,1078.70394945296,
464.798220491965));
#107214=CARTESIAN_POINT('Ctrl Pts',(-78.7219583311996,1078.70150402876,
464.620629726257));
#107215=CARTESIAN_POINT('Ctrl Pts',(-78.8565367240314,1078.6998573544,464.550222893131));
#107216=CARTESIAN_POINT('Ctrl Pts',(-79.1532470397934,1078.69553189093,
464.448890448833));
#107217=CARTESIAN_POINT('Ctrl Pts',(-79.314675118167,1078.69281018161,464.422087699128));
#107218=CARTESIAN_POINT('Ctrl Pts',(-79.4772023228643,1078.68962000954,
464.422087699128));
#107219=CARTESIAN_POINT('Ctrl Pts',(-79.4772023228643,1078.68962000954,
464.422087699128));
#107220=CARTESIAN_POINT('Ctrl Pts',(-79.4772374221895,1078.68961932059,
464.422087699128));
#107221=CARTESIAN_POINT('Ctrl Pts',(-79.4772725215661,1078.68961863162,
464.422087700378));
#107222=CARTESIAN_POINT('Ctrl Pts',(-79.4773076209938,1078.68961794263,
464.422087702878));
#107223=CARTESIAN_POINT('Ctrl Pts',(-79.6578351445778,1078.68607423721,
464.422100561682));
#107224=CARTESIAN_POINT('Ctrl Pts',(-79.8368317539902,1078.68200453645,
464.455181557539));
#107225=CARTESIAN_POINT('Ctrl Pts',(-80.1867070141573,1078.67273506018,
464.589033850225));
#107226=CARTESIAN_POINT('Ctrl Pts',(-80.3525644969555,1078.66756098388,
464.693414859106));
#107227=CARTESIAN_POINT('Ctrl Pts',(-80.6340883428405,1078.65714770488,
464.959929228747));
#107228=CARTESIAN_POINT('Ctrl Pts',(-80.747171545548,1078.65201361478,465.119342388313));
#107229=CARTESIAN_POINT('Ctrl Pts',(-80.8991659411406,1078.64310800614,
465.458632852703));
#107230=CARTESIAN_POINT('Ctrl Pts',(-80.9420213988041,1078.63933891585,
465.633099070356));
#107231=CARTESIAN_POINT('Ctrl Pts',(-80.9635642652209,1078.6334210861,465.98865397077));
#107232=CARTESIAN_POINT('Ctrl Pts',(-80.9421536870177,1078.63132275593,
466.16682496811));
#107233=CARTESIAN_POINT('Ctrl Pts',(-80.8765123219844,1078.63000398886,
466.379215479463));
#107234=CARTESIAN_POINT('Ctrl Pts',(-80.8615403073948,1078.62980609902,
466.420919326469));
#107235=CARTESIAN_POINT('Ctrl Pts',(-80.8337123344805,1078.62958784544,
466.488693830072));
#107236=CARTESIAN_POINT('Ctrl Pts',(-80.821920249749,1078.62952980067,466.515170087636));
#107237=CARTESIAN_POINT('Ctrl Pts',(-80.7992810929771,1078.62947641098,
466.562227751899));
#107238=CARTESIAN_POINT('Ctrl Pts',(-80.7887119724455,1078.62947093756,
466.582932275856));
#107239=CARTESIAN_POINT('Ctrl Pts',(-80.7652055309049,1078.6294982132,466.626416808503));
#107240=CARTESIAN_POINT('Ctrl Pts',(-80.7521420032339,1078.62953588985,
466.64911961512));
#107241=CARTESIAN_POINT('Ctrl Pts',(-80.7157427964114,1078.62969797923,
466.708659528841));
#107242=CARTESIAN_POINT('Ctrl Pts',(-80.6913690895156,1078.6298633371,466.744831364274));
#107243=CARTESIAN_POINT('Ctrl Pts',(-80.5758345934766,1078.63088139912,
466.900925063529));
#107244=CARTESIAN_POINT('Ctrl Pts',(-80.4682664607717,1078.63242197353,
467.007571660406));
#107245=CARTESIAN_POINT('Ctrl Pts',(-80.2243697756869,1078.63681484799,
467.184877133115));
#107246=CARTESIAN_POINT('Ctrl Pts',(-80.0894097608931,1078.6396428075,467.254407262539));
#107247=CARTESIAN_POINT('Ctrl Pts',(-79.795016720375,1078.646399601,467.352912073684));
#107248=CARTESIAN_POINT('Ctrl Pts',(-79.6366024626598,1078.6503341046,467.378693963515));
#107249=CARTESIAN_POINT('Ctrl Pts',(-79.4772023228642,1078.65448750233,
467.378693963515));
#107250=CARTESIAN_POINT('',(-81.0356882485059,1078.30327084026,478.72049644629));
#107251=CARTESIAN_POINT('',(-81.035688248506,1078.39243716831,476.169608204017));
#107252=CARTESIAN_POINT('Ctrl Pts',(-81.0356882485058,1078.30327084026,
478.72049644629));
#107253=CARTESIAN_POINT('Ctrl Pts',(-81.0246146286944,1078.30389283659,
478.72049644629));
#107254=CARTESIAN_POINT('Ctrl Pts',(-81.013536285703,1078.30451982721,478.720352232097));
#107255=CARTESIAN_POINT('Ctrl Pts',(-80.849922124026,1078.31384932016,478.716087747516));
#107256=CARTESIAN_POINT('Ctrl Pts',(-80.6993645438354,1078.32332388982,
478.684773255856));
#107257=CARTESIAN_POINT('Ctrl Pts',(-80.406120054577,1078.34352880323,478.566307789147));
#107258=CARTESIAN_POINT('Ctrl Pts',(-80.2675087598995,1078.35411307893,
478.476302582562));
#107259=CARTESIAN_POINT('Ctrl Pts',(-80.0287142245288,1078.37463495229,
478.245708296621));
#107260=CARTESIAN_POINT('Ctrl Pts',(-79.9319852644289,1078.38434954179,
478.106051722543));
#107261=CARTESIAN_POINT('Ctrl Pts',(-79.8016771481059,1078.40100347093,
477.804932762459));
#107262=CARTESIAN_POINT('Ctrl Pts',(-79.7663133135025,1078.40791484644,
477.647584775361));
#107263=CARTESIAN_POINT('Ctrl Pts',(-79.7555600297393,1078.41884496892,
477.326581155275));
#107264=CARTESIAN_POINT('Ctrl Pts',(-79.7807759131022,1078.42274366209,
477.165797839069));
#107265=CARTESIAN_POINT('Ctrl Pts',(-79.8544214029996,1078.42568001192,
476.960734248989));
#107266=CARTESIAN_POINT('Ctrl Pts',(-79.8770533837945,1078.42622650527,
476.908842398745));
#107267=CARTESIAN_POINT('Ctrl Pts',(-79.9149852322163,1078.42670603233,
476.835580661151));
#107268=CARTESIAN_POINT('Ctrl Pts',(-79.9276157778859,1078.4268108751,476.81290805346));
#107269=CARTESIAN_POINT('Ctrl Pts',(-79.9510641285986,1078.42691440006,
476.773681786644));
#107270=CARTESIAN_POINT('Ctrl Pts',(-79.9615916111564,1078.42693243605,
476.756964905051));
#107271=CARTESIAN_POINT('Ctrl Pts',(-79.9840377208164,1078.4269145742,476.723093261105));
#107272=CARTESIAN_POINT('Ctrl Pts',(-79.995998033311,1078.42687554031,476.705973185222));
#107273=CARTESIAN_POINT('Ctrl Pts',(-80.0272864672442,1078.42670142049,
476.663450137169));
#107274=CARTESIAN_POINT('Ctrl Pts',(-80.047157582036,1078.42652655107,476.638464941525));
#107275=CARTESIAN_POINT('Ctrl Pts',(-80.1267336508165,1078.42559146828,
476.5457721397));
#107276=CARTESIAN_POINT('Ctrl Pts',(-80.1926209575092,1078.42434875834,
476.483731250177));
#107277=CARTESIAN_POINT('Ctrl Pts',(-80.3621838379226,1078.42014554662,
476.355010072729));
#107278=CARTESIAN_POINT('Ctrl Pts',(-80.4700396685857,1078.41675072151,
476.2953437933));
#107279=CARTESIAN_POINT('Ctrl Pts',(-80.7288782737061,1078.40704842616,
476.197504052671));
#107280=CARTESIAN_POINT('Ctrl Pts',(-80.8816760726839,1078.4002949488,476.169608204017));
#107281=CARTESIAN_POINT('Ctrl Pts',(-81.035688248506,1078.39243716831,476.169608204017));
#107282=CARTESIAN_POINT('Ctrl Pts',(-81.035688248506,1078.39243716831,476.169608204017));
#107283=CARTESIAN_POINT('Ctrl Pts',(-81.0357370854227,1078.39243467663,
476.169608204017));
#107284=CARTESIAN_POINT('Ctrl Pts',(-81.0357859224614,1078.39243218483,
476.169608206822));
#107285=CARTESIAN_POINT('Ctrl Pts',(-81.0358347596221,1078.39242969293,
476.169608212432));
#107286=CARTESIAN_POINT('Ctrl Pts',(-81.1884097858379,1078.38464458215,
476.169625738827));
#107287=CARTESIAN_POINT('Ctrl Pts',(-81.339705315759,1078.37589900606,476.197020008355));
#107288=CARTESIAN_POINT('Ctrl Pts',(-81.6362043920957,1078.35649949467,
476.307925396765));
#107289=CARTESIAN_POINT('Ctrl Pts',(-81.7773384188491,1078.34592786177,
476.394517607236));
#107290=CARTESIAN_POINT('Ctrl Pts',(-82.0221363012155,1078.32463965672,
476.619227519744));
#107291=CARTESIAN_POINT('Ctrl Pts',(-82.1223813506698,1078.31413352335,
476.756439070523));
#107292=CARTESIAN_POINT('Ctrl Pts',(-82.260471498279,1078.29547961063,477.054697824724));
#107293=CARTESIAN_POINT('Ctrl Pts',(-82.2998260628927,1078.28741236139,
477.211674781804));
#107294=CARTESIAN_POINT('Ctrl Pts',(-82.3180260970581,1078.27452931816,
477.528409403417));
#107295=CARTESIAN_POINT('Ctrl Pts',(-82.2980854407609,1078.26975642285,
477.685309053818));
#107296=CARTESIAN_POINT('Ctrl Pts',(-82.2302887610955,1078.26569519593,
477.896624925614));
#107297=CARTESIAN_POINT('Ctrl Pts',(-82.2057090814756,1078.26483744237,
477.956951338812));
#107298=CARTESIAN_POINT('Ctrl Pts',(-82.1637895291425,1078.26409446277,
478.040846633512));
#107299=CARTESIAN_POINT('Ctrl Pts',(-82.1500809942766,1078.26393382971,
478.066109657378));
#107300=CARTESIAN_POINT('Ctrl Pts',(-82.1253253740612,1078.26377514787,
478.108267852636));
#107301=CARTESIAN_POINT('Ctrl Pts',(-82.1147094808373,1078.26374289417,
478.125403033569));
#107302=CARTESIAN_POINT('Ctrl Pts',(-82.092485377571,1078.26374479904,478.159445633166));
#107303=CARTESIAN_POINT('Ctrl Pts',(-82.080866558139,1078.26378010682,478.176339045595));
#107304=CARTESIAN_POINT('Ctrl Pts',(-82.0515873176963,1078.26394966612,
478.21678611052));
#107305=CARTESIAN_POINT('Ctrl Pts',(-82.0335091520795,1078.26412027579,
478.240022357411));
#107306=CARTESIAN_POINT('Ctrl Pts',(-81.9677280412465,1078.26496015125,
478.318789414217));
#107307=CARTESIAN_POINT('Ctrl Pts',(-81.9160676781231,1078.26599227478,
478.370819582238));
#107308=CARTESIAN_POINT('Ctrl Pts',(-81.730506780143,1078.27081218889,478.528056937085));
#107309=CARTESIAN_POINT('Ctrl Pts',(-81.5801458160651,1078.27639325169,
478.610898179553));
#107310=CARTESIAN_POINT('Ctrl Pts',(-81.2942153277187,1078.28939691917,
478.700746590495));
#107311=CARTESIAN_POINT('Ctrl Pts',(-81.1652752015319,1078.2959920452,478.72049644629));
#107312=CARTESIAN_POINT('Ctrl Pts',(-81.0356882485059,1078.30327084026,
478.72049644629));
#107313=CARTESIAN_POINT('',(-81.8208965804703,1077.59408165985,491.319637120915));
#107314=CARTESIAN_POINT('',(-81.8208965804704,1077.73591376921,489.12197484893));
#107315=CARTESIAN_POINT('Ctrl Pts',(-81.8208965804702,1077.59408165985,
491.319637120915));
#107316=CARTESIAN_POINT('Ctrl Pts',(-81.8118915361856,1077.59482365131,
491.319637120915));
#107317=CARTESIAN_POINT('Ctrl Pts',(-81.8028833073338,1077.59557296073,
491.319526425073));
#107318=CARTESIAN_POINT('Ctrl Pts',(-81.6650299504941,1077.60714761654,
491.316135283922));
#107319=CARTESIAN_POINT('Ctrl Pts',(-81.5378374876298,1077.61926824562,
491.29032572045));
#107320=CARTESIAN_POINT('Ctrl Pts',(-81.2890739137649,1077.64591676414,
491.192312092427));
#107321=CARTESIAN_POINT('Ctrl Pts',(-81.1708563653607,1077.66032580353,
491.117520350974));
#107322=CARTESIAN_POINT('Ctrl Pts',(-80.9632826475642,1077.68950111704,
490.923075558048));
#107323=CARTESIAN_POINT('Ctrl Pts',(-80.8777154171757,1077.70396840503,
490.803164881407));
#107324=CARTESIAN_POINT('Ctrl Pts',(-80.7603977399351,1077.7298560879,490.541226072427));
#107325=CARTESIAN_POINT('Ctrl Pts',(-80.7280107668011,1077.74112818323,
490.402466783174));
#107326=CARTESIAN_POINT('Ctrl Pts',(-80.7182084710857,1077.75856843853,
490.136304571665));
#107327=CARTESIAN_POINT('Ctrl Pts',(-80.7349615340522,1077.76504817312,
490.011397952834));
#107328=CARTESIAN_POINT('Ctrl Pts',(-80.7976636227379,1077.77261702441,
489.811502576923));
#107329=CARTESIAN_POINT('Ctrl Pts',(-80.832069735605,1077.77474978174,489.734221745625));
#107330=CARTESIAN_POINT('Ctrl Pts',(-80.8898798419136,1077.77634356121,
489.636431121329));
#107331=CARTESIAN_POINT('Ctrl Pts',(-80.9057720620957,1077.77663908756,
489.611845063301));
#107332=CARTESIAN_POINT('Ctrl Pts',(-80.9331333362566,1077.77693110706,
489.573010483975));
#107333=CARTESIAN_POINT('Ctrl Pts',(-80.9440090522601,1077.77699826122,
489.558362881511));
#107334=CARTESIAN_POINT('Ctrl Pts',(-80.9654901296214,1077.77704056502,
489.530888332557));
#107335=CARTESIAN_POINT('Ctrl Pts',(-80.976032040185,1077.77702329235,489.518018342442));
#107336=CARTESIAN_POINT('Ctrl Pts',(-81.0007633359159,1077.77689835396,
489.48918640079));
#107337=CARTESIAN_POINT('Ctrl Pts',(-81.0151338254733,1077.77676647083,
489.473389028346));
#107338=CARTESIAN_POINT('Ctrl Pts',(-81.0600520314457,1077.77618036466,
489.42681279229));
#107339=CARTESIAN_POINT('Ctrl Pts',(-81.0919670543924,1077.77553457296,
489.397416206979));
#107340=CARTESIAN_POINT('Ctrl Pts',(-81.1684314400932,1077.77349358948,
489.334922941254));
#107341=CARTESIAN_POINT('Ctrl Pts',(-81.2139127955276,1077.77194298042,
489.303163477479));
#107342=CARTESIAN_POINT('Ctrl Pts',(-81.3532708389864,1077.76625856801,
489.220754906984));
#107343=CARTESIAN_POINT('Ctrl Pts',(-81.4522991486972,1077.7610929863,489.180188351247));
#107344=CARTESIAN_POINT('Ctrl Pts',(-81.642393652247,1077.74922189726,489.132882805429));
#107345=CARTESIAN_POINT('Ctrl Pts',(-81.7315060347125,1077.74293575321,
489.12197484893));
#107346=CARTESIAN_POINT('Ctrl Pts',(-81.8208965804703,1077.73591376921,
489.12197484893));
#107347=CARTESIAN_POINT('Ctrl Pts',(-81.8208965804703,1077.73591376921,
489.12197484893));
#107348=CARTESIAN_POINT('Ctrl Pts',(-81.8209326256086,1077.73591093772,
489.12197484893));
#107349=CARTESIAN_POINT('Ctrl Pts',(-81.8209686707924,1077.73590810611,
489.121974850652));
#107350=CARTESIAN_POINT('Ctrl Pts',(-81.821004716021,1077.73590527439,489.121974854199));
#107351=CARTESIAN_POINT('Ctrl Pts',(-81.9496463542983,1077.72579913187,
489.121987513779));
#107352=CARTESIAN_POINT('Ctrl Pts',(-82.0771879486502,1077.71429939178,
489.144588824965));
#107353=CARTESIAN_POINT('Ctrl Pts',(-82.3281263519596,1077.68850371663,
489.236232017209));
#107354=CARTESIAN_POINT('Ctrl Pts',(-82.4481876460914,1077.67428167137,
489.308035833405));
#107355=CARTESIAN_POINT('Ctrl Pts',(-82.6606397964049,1077.64490782975,
489.497244059042));
#107356=CARTESIAN_POINT('Ctrl Pts',(-82.749220716077,1077.63002708413,489.61503396911));
#107357=CARTESIAN_POINT('Ctrl Pts',(-82.8731942416252,1077.60287597756,
489.874276442954));
#107358=CARTESIAN_POINT('Ctrl Pts',(-82.9090585203821,1077.59078683123,
490.012502904669));
#107359=CARTESIAN_POINT('Ctrl Pts',(-82.9251666420322,1077.57194715739,
490.276411796771));
#107360=CARTESIAN_POINT('Ctrl Pts',(-82.91206039424,1077.56483498601,490.399452575105));
#107361=CARTESIAN_POINT('Ctrl Pts',(-82.8537628365387,1077.55582790869,
490.607078570887));
#107362=CARTESIAN_POINT('Ctrl Pts',(-82.8175118277962,1077.55311660244,
490.692812219282));
#107363=CARTESIAN_POINT('Ctrl Pts',(-82.755506224016,1077.55115312648,490.799488581695));
#107364=CARTESIAN_POINT('Ctrl Pts',(-82.7390062251826,1077.55080121714,
490.825325305712));
#107365=CARTESIAN_POINT('Ctrl Pts',(-82.7107542610172,1077.5504550759,490.865733425717));
#107366=CARTESIAN_POINT('Ctrl Pts',(-82.699673504174,1077.55037484557,490.880752370421));
#107367=CARTESIAN_POINT('Ctrl Pts',(-82.6779419108619,1077.5503191592,490.908689071181));
#107368=CARTESIAN_POINT('Ctrl Pts',(-82.6673679989646,1077.55033373751,
490.921659732327));
#107369=CARTESIAN_POINT('Ctrl Pts',(-82.6428036944148,1077.55045913459,
490.950424732042));
#107370=CARTESIAN_POINT('Ctrl Pts',(-82.6286465420175,1077.550594023,490.966067540874));
#107371=CARTESIAN_POINT('Ctrl Pts',(-82.5852589271665,1077.55118740396,
491.011318758765));
#107372=CARTESIAN_POINT('Ctrl Pts',(-82.5547905059292,1077.55183252429,
491.039682847927));
#107373=CARTESIAN_POINT('Ctrl Pts',(-82.4106545990951,1077.55585409507,
491.159345734858));
#107374=CARTESIAN_POINT('Ctrl Pts',(-82.2812024659983,1077.56198577209,
491.229134551155));
#107375=CARTESIAN_POINT('Ctrl Pts',(-82.0378234752273,1077.57723552437,
491.303508793025));
#107376=CARTESIAN_POINT('Ctrl Pts',(-81.9295920155049,1077.58512544789,
491.319637120915));
#107377=CARTESIAN_POINT('Ctrl Pts',(-81.8208965804703,1077.59408165985,
491.319637120915));
#107378=CARTESIAN_POINT('',(-88.5622696992322,1078.67883079978,412.779359758956));
#107379=CARTESIAN_POINT('',(-88.5622696999027,1078.6674873026,409.822753494571));
#107380=CARTESIAN_POINT('Ctrl Pts',(-88.5622696992322,1078.67883079978,
412.779359758958));
#107381=CARTESIAN_POINT('Ctrl Pts',(-88.3720465431456,1078.68346300856,
412.779359758958));
#107382=CARTESIAN_POINT('Ctrl Pts',(-88.1835393752714,1078.68762476377,
412.742643006163));
#107383=CARTESIAN_POINT('Ctrl Pts',(-87.8330299621801,1078.69469627254,
412.600624952613));
#107384=CARTESIAN_POINT('Ctrl Pts',(-87.6739489247432,1078.69756238392,
412.497535482797));
#107385=CARTESIAN_POINT('Ctrl Pts',(-87.4110242733929,1078.70187707695,
412.245095658751));
#107386=CARTESIAN_POINT('Ctrl Pts',(-87.3065626456926,1078.70337092014,
412.100918382936));
#107387=CARTESIAN_POINT('Ctrl Pts',(-87.1922830720543,1078.70477103525,
411.863280437301));
#107388=CARTESIAN_POINT('Ctrl Pts',(-87.1615575513009,1078.70509473567,
411.781644408685));
#107389=CARTESIAN_POINT('Ctrl Pts',(-87.1288978711513,1078.70535802001,
411.664409618201));
#107390=CARTESIAN_POINT('Ctrl Pts',(-87.1207771437061,1078.70541138917,
411.630722228774));
#107391=CARTESIAN_POINT('Ctrl Pts',(-87.1092252263883,1078.70546453852,
411.574142281458));
#107392=CARTESIAN_POINT('Ctrl Pts',(-87.1051345194932,1078.70547623568,
411.551398557956));
#107393=CARTESIAN_POINT('Ctrl Pts',(-87.0981626334012,1078.7054804261,411.50663702773));
#107394=CARTESIAN_POINT('Ctrl Pts',(-87.0952410569726,1078.70547365665,
411.484631579642));
#107395=CARTESIAN_POINT('Ctrl Pts',(-87.0895162870177,1078.70543683694,
411.432547037356));
#107396=CARTESIAN_POINT('Ctrl Pts',(-87.0871373275958,1078.70539928134,
411.402431296504));
#107397=CARTESIAN_POINT('Ctrl Pts',(-87.082411904188,1078.70522408831,411.304442748419));
#107398=CARTESIAN_POINT('Ctrl Pts',(-87.0838178213005,1078.70502038877,
411.236476986767));
#107399=CARTESIAN_POINT('Ctrl Pts',(-87.1075152500637,1078.70389881578,
410.972560504793));
#107400=CARTESIAN_POINT('Ctrl Pts',(-87.1642153990549,1078.70237783114,
410.781768540865));
#107401=CARTESIAN_POINT('Ctrl Pts',(-87.3323601198773,1078.69825985756,
410.465134173314));
#107402=CARTESIAN_POINT('Ctrl Pts',(-87.4309231016497,1078.69592960438,
410.335917043225));
#107403=CARTESIAN_POINT('Ctrl Pts',(-87.6762789245318,1078.69004880737,
410.104698021033));
#107404=CARTESIAN_POINT('Ctrl Pts',(-87.8246111859352,1078.68645095964,
410.007957014957));
#107405=CARTESIAN_POINT('Ctrl Pts',(-88.1603822288219,1078.67803437732,
409.865946290356));
#107406=CARTESIAN_POINT('Ctrl Pts',(-88.3468328146265,1078.67321809151,
409.826391913944));
#107407=CARTESIAN_POINT('Ctrl Pts',(-88.5445356951068,1078.66795983999,
409.822833239939));
#107408=CARTESIAN_POINT('Ctrl Pts',(-88.5534044842976,1078.66772366684,
409.822753494563));
#107409=CARTESIAN_POINT('Ctrl Pts',(-88.5622697005729,1078.6674873026,409.822753494571));
#107410=CARTESIAN_POINT('Ctrl Pts',(-88.5622697005729,1078.6674873026,409.822753494571));
#107411=CARTESIAN_POINT('Ctrl Pts',(-88.7482632788002,1078.66252834504,
409.82275349474));
#107412=CARTESIAN_POINT('Ctrl Pts',(-88.9326839838793,1078.65747797831,
409.857856290321));
#107413=CARTESIAN_POINT('Ctrl Pts',(-89.2800864525725,1078.64789049099,
409.995207055741));
#107414=CARTESIAN_POINT('Ctrl Pts',(-89.4397013581415,1078.64345127623,
410.096636922239));
#107415=CARTESIAN_POINT('Ctrl Pts',(-89.7035541722497,1078.6363283406,410.345277781389));
#107416=CARTESIAN_POINT('Ctrl Pts',(-89.8086570987339,1078.63360899343,
410.487072400501));
#107417=CARTESIAN_POINT('Ctrl Pts',(-89.9270742879669,1078.63091347673,
410.725713827499));
#107418=CARTESIAN_POINT('Ctrl Pts',(-89.959986675958,1078.63025236458,410.811057805764));
#107419=CARTESIAN_POINT('Ctrl Pts',(-89.994507635958,1078.62971995358,410.933166340795));
#107420=CARTESIAN_POINT('Ctrl Pts',(-90.0029554151524,1078.62961297761,
410.967779783559));
#107421=CARTESIAN_POINT('Ctrl Pts',(-90.0148960647361,1078.62950648655,
411.025718890385));
#107422=CARTESIAN_POINT('Ctrl Pts',(-90.0190960092562,1078.62948284379,
411.048883412025));
#107423=CARTESIAN_POINT('Ctrl Pts',(-90.0262181507212,1078.62947332018,
411.094321821039));
#107424=CARTESIAN_POINT('Ctrl Pts',(-90.0291893723829,1078.62948575078,
411.116581643447));
#107425=CARTESIAN_POINT('Ctrl Pts',(-90.0349780532876,1078.62955506483,
411.169035941086));
#107426=CARTESIAN_POINT('Ctrl Pts',(-90.0373758374848,1078.62962597853,
411.199266507595));
#107427=CARTESIAN_POINT('Ctrl Pts',(-90.0396300006932,1078.62978247808,
411.245813272079));
#107428=CARTESIAN_POINT('Ctrl Pts',(-90.0401488707183,1078.6298460624,411.262089135427));
#107429=CARTESIAN_POINT('Ctrl Pts',(-90.040398755281,1078.62991850175,411.278370581859));
#107430=CARTESIAN_POINT('Ctrl Pts',(-90.0421089956495,1078.63041428546,
411.389802783379));
#107431=CARTESIAN_POINT('Ctrl Pts',(-90.0312128827685,1078.63132398269,
411.501068368572));
#107432=CARTESIAN_POINT('Ctrl Pts',(-89.9779962522632,1078.63427467906,
411.750050090782));
#107433=CARTESIAN_POINT('Ctrl Pts',(-89.9278941082664,1078.63654858306,
411.884958985214));
#107434=CARTESIAN_POINT('Ctrl Pts',(-89.7817738647771,1078.64242142456,
412.152062147659));
#107435=CARTESIAN_POINT('Ctrl Pts',(-89.6817174915438,1078.64611047156,
412.279949410848));
#107436=CARTESIAN_POINT('Ctrl Pts',(-89.4342242384996,1078.65449935178,
412.507575555964));
#107437=CARTESIAN_POINT('Ctrl Pts',(-89.2854378955564,1078.65918827646,
412.602216692662));
#107438=CARTESIAN_POINT('Ctrl Pts',(-88.9500209872393,1078.66892647233,
412.739885380551));
#107439=CARTESIAN_POINT('Ctrl Pts',(-88.7644669161036,1078.67388501125,
412.777437263733));
#107440=CARTESIAN_POINT('Ctrl Pts',(-88.5719892200386,1078.67859384164,
412.779335800596));
#107441=CARTESIAN_POINT('Ctrl Pts',(-88.5671288996929,1078.67871247122,
412.779359758958));
#107442=CARTESIAN_POINT('Ctrl Pts',(-88.5622696992322,1078.67883079978,
412.779359758958));
#107443=CARTESIAN_POINT('',(-96.6088930673541,1078.35304757369,421.000273047718));
#107444=CARTESIAN_POINT('',(-96.6088930673544,1078.34478217746,418.449384805446));
#107445=CARTESIAN_POINT('Ctrl Pts',(-96.608893067354,1078.35304757369,421.000273047718));
#107446=CARTESIAN_POINT('Ctrl Pts',(-96.4411564053785,1078.36372558668,
421.000273047718));
#107447=CARTESIAN_POINT('Ctrl Pts',(-96.2750044101523,1078.37400306029,
420.967183692732));
#107448=CARTESIAN_POINT('Ctrl Pts',(-95.9679692011027,1078.39248845416,
420.839756898053));
#107449=CARTESIAN_POINT('Ctrl Pts',(-95.8295373430025,1078.40056280147,
420.747810081579));
#107450=CARTESIAN_POINT('Ctrl Pts',(-95.6123829417737,1078.412878806,420.53321688905));
#107451=CARTESIAN_POINT('Ctrl Pts',(-95.5293799427867,1078.41742648329,
420.418511532374));
#107452=CARTESIAN_POINT('Ctrl Pts',(-95.4165609832057,1078.42336871561,
420.191545765542));
#107453=CARTESIAN_POINT('Ctrl Pts',(-95.3799678353809,1078.4251832957,420.084313466252));
#107454=CARTESIAN_POINT('Ctrl Pts',(-95.3512046396373,1078.42643124959,
419.939713717261));
#107455=CARTESIAN_POINT('Ctrl Pts',(-95.3458366620551,1078.42664268365,
419.90550609858));
#107456=CARTESIAN_POINT('Ctrl Pts',(-95.3395277148658,1078.42684860335,
419.850865132454));
#107457=CARTESIAN_POINT('Ctrl Pts',(-95.3376749296248,1078.4268965,419.830554869784));
#107458=CARTESIAN_POINT('Ctrl Pts',(-95.3351138846986,1078.42693294963,
419.792382646171));
#107459=CARTESIAN_POINT('Ctrl Pts',(-95.3342925845398,1078.42692811306,
419.774533252375));
#107460=CARTESIAN_POINT('Ctrl Pts',(-95.3332974444016,1078.4268685624,419.73468693578));
#107461=CARTESIAN_POINT('Ctrl Pts',(-95.3333171057799,1078.42680259814,
419.71269091993));
#107462=CARTESIAN_POINT('Ctrl Pts',(-95.3350236084832,1078.42651536784,
419.648927201414));
#107463=CARTESIAN_POINT('Ctrl Pts',(-95.3381946140514,1078.4262079424,419.607228903325));
#107464=CARTESIAN_POINT('Ctrl Pts',(-95.3646195983356,1078.4240482944,419.396999232236));
#107465=CARTESIAN_POINT('Ctrl Pts',(-95.419373153071,1078.42037839787,419.234211423141));
#107466=CARTESIAN_POINT('Ctrl Pts',(-95.5725099644199,1078.41053271886,
418.969039496746));
#107467=CARTESIAN_POINT('Ctrl Pts',(-95.6590553100129,1078.4050613179,418.862799618694));
#107468=CARTESIAN_POINT('Ctrl Pts',(-95.8721100587869,1078.39162143158,
418.673089397293));
#107469=CARTESIAN_POINT('Ctrl Pts',(-96.0000096685498,1078.38356507368,
418.594236415888));
#107470=CARTESIAN_POINT('Ctrl Pts',(-96.2882865967761,1078.36529676825,
418.479874465366));
#107471=CARTESIAN_POINT('Ctrl Pts',(-96.4478799282913,1078.35512374414,
418.449384805446));
#107472=CARTESIAN_POINT('Ctrl Pts',(-96.6088930673548,1078.34478217746,
418.449384805446));
#107473=CARTESIAN_POINT('Ctrl Pts',(-96.6088930673548,1078.34478217746,
418.449384805446));
#107474=CARTESIAN_POINT('Ctrl Pts',(-96.6090238328897,1078.34477377864,
418.449384805446));
#107475=CARTESIAN_POINT('Ctrl Pts',(-96.6091545993613,1078.34476537971,
418.449384825556));
#107476=CARTESIAN_POINT('Ctrl Pts',(-96.6092853667651,1078.34475698068,
418.449384865777));
#107477=CARTESIAN_POINT('Ctrl Pts',(-96.7781840641058,1078.33390881808,
418.449436815417));
#107478=CARTESIAN_POINT('Ctrl Pts',(-96.9454236811818,1078.32308238173,
418.483037464539));
#107479=CARTESIAN_POINT('Ctrl Pts',(-97.2526487103228,1078.30313265084,
418.611605927842));
#107480=CARTESIAN_POINT('Ctrl Pts',(-97.3904437732686,1078.29415721113,
418.703602447287));
#107481=CARTESIAN_POINT('Ctrl Pts',(-97.6069684432521,1078.28017173905,
418.918348363267));
#107482=CARTESIAN_POINT('Ctrl Pts',(-97.689839152874,1078.2748765614,419.033347266563));
#107483=CARTESIAN_POINT('Ctrl Pts',(-97.8017923212791,1078.26794721432,
419.259806506448));
#107484=CARTESIAN_POINT('Ctrl Pts',(-97.8379520527778,1078.26581376158,
419.366113891067));
#107485=CARTESIAN_POINT('Ctrl Pts',(-97.8665581381454,1078.26433496545,
419.50979672806));
#107486=CARTESIAN_POINT('Ctrl Pts',(-97.8719396195343,1078.26408207387,
419.54407002045));
#107487=CARTESIAN_POINT('Ctrl Pts',(-97.8782748555643,1078.26383537897,
419.598932935124));
#107488=CARTESIAN_POINT('Ctrl Pts',(-97.8801383359718,1078.26377802594,
419.619399329966));
#107489=CARTESIAN_POINT('Ctrl Pts',(-97.8826989434441,1078.26373525483,
419.657769482161));
#107490=CARTESIAN_POINT('Ctrl Pts',(-97.8835148994611,1078.26374154366,
419.675660201531));
#107491=CARTESIAN_POINT('Ctrl Pts',(-97.8844999904487,1078.26381444934,
419.715832257367));
#107492=CARTESIAN_POINT('Ctrl Pts',(-97.8844625442838,1078.2638954001,419.738112705142));
#107493=CARTESIAN_POINT('Ctrl Pts',(-97.8826586561125,1078.26424800808,
419.802803525369));
#107494=CARTESIAN_POINT('Ctrl Pts',(-97.8793590894313,1078.26462575466,
419.845139695908));
#107495=CARTESIAN_POINT('Ctrl Pts',(-97.8522819676114,1078.26724351246,
420.056062005821));
#107496=CARTESIAN_POINT('Ctrl Pts',(-97.7970373399257,1078.27164432092,
420.218802382153));
#107497=CARTESIAN_POINT('Ctrl Pts',(-97.643243576394,1078.28310383072,420.483340876153));
#107498=CARTESIAN_POINT('Ctrl Pts',(-97.5566384047077,1078.28937278886,
420.589106385314));
#107499=CARTESIAN_POINT('Ctrl Pts',(-97.3439211599217,1078.30435189313,
420.777701893593));
#107500=CARTESIAN_POINT('Ctrl Pts',(-97.2164873800139,1078.31311945353,
420.856028921133));
#107501=CARTESIAN_POINT('Ctrl Pts',(-96.9301325538843,1078.33231895252,
420.969428425943));
#107502=CARTESIAN_POINT('Ctrl Pts',(-96.7720542839807,1078.34265680146,
420.99981801351));
#107503=CARTESIAN_POINT('Ctrl Pts',(-96.6112907641862,1078.35289492281,
421.000271357194));
#107504=CARTESIAN_POINT('Ctrl Pts',(-96.6100918752876,1078.35297125831,
421.000273047718));
#107505=CARTESIAN_POINT('Ctrl Pts',(-96.608893067354,1078.35304757369,421.000273047718));
#107506=CARTESIAN_POINT('',(-104.753539540172,1077.66045630879,430.69792801177));
#107507=CARTESIAN_POINT('',(-104.753539540172,1077.67122217491,428.500265739785));
#107508=CARTESIAN_POINT('Ctrl Pts',(-104.753539540173,1077.66045630879,
430.69792801177));
#107509=CARTESIAN_POINT('Ctrl Pts',(-104.665620762378,1077.66953439425,
430.69792801177));
#107510=CARTESIAN_POINT('Ctrl Pts',(-104.577820809394,1077.67861004491,
430.687375893461));
#107511=CARTESIAN_POINT('Ctrl Pts',(-104.351123445455,1077.70207399203,
430.63183273988));
#107512=CARTESIAN_POINT('Ctrl Pts',(-104.218319609593,1077.71585004638,
430.569706428685));
#107513=CARTESIAN_POINT('Ctrl Pts',(-103.991013504431,1077.73957922168,
430.402083048091));
#107514=CARTESIAN_POINT('Ctrl Pts',(-103.896754594879,1077.74949975389,
430.300681307374));
#107515=CARTESIAN_POINT('Ctrl Pts',(-103.751674047223,1077.76506878071,
430.070177655793));
#107516=CARTESIAN_POINT('Ctrl Pts',(-103.701384955506,1077.77065556777,
429.943581637273));
#107517=CARTESIAN_POINT('Ctrl Pts',(-103.665470205862,1077.77507824458,
429.760799175423));
#107518=CARTESIAN_POINT('Ctrl Pts',(-103.659125711864,1077.77594593367,
429.710011696374));
#107519=CARTESIAN_POINT('Ctrl Pts',(-103.655144653883,1077.776683831,429.637047095014));
#107520=CARTESIAN_POINT('Ctrl Pts',(-103.654605759401,1077.77684051502,
429.615101075762));
#107521=CARTESIAN_POINT('Ctrl Pts',(-103.654799106998,1077.77698962827,
429.579356677061));
#107522=CARTESIAN_POINT('Ctrl Pts',(-103.655133568426,1077.77702143461,
429.565562705391));
#107523=CARTESIAN_POINT('Ctrl Pts',(-103.656376372779,1077.77703407627,
429.536728899218));
#107524=CARTESIAN_POINT('Ctrl Pts',(-103.657334452703,1077.77700996203,
429.521694130414));
#107525=CARTESIAN_POINT('Ctrl Pts',(-103.660332586206,1077.77688024178,
429.486171312399));
#107526=CARTESIAN_POINT('Ctrl Pts',(-103.662639901655,1077.77674803136,
429.465711801408));
#107527=CARTESIAN_POINT('Ctrl Pts',(-103.672067549693,1077.77612822872,
429.399004127164));
#107528=CARTESIAN_POINT('Ctrl Pts',(-103.68156597282,1077.77540318433,429.353148475303));
#107529=CARTESIAN_POINT('Ctrl Pts',(-103.732641877495,1077.77121575433,
429.16720675395));
#107530=CARTESIAN_POINT('Ctrl Pts',(-103.798990576823,1077.7652556671,429.035590811263));
#107531=CARTESIAN_POINT('Ctrl Pts',(-103.962445650476,1077.74993136629,
428.827247625019));
#107532=CARTESIAN_POINT('Ctrl Pts',(-104.050523213927,1077.74149890571,
428.746275707446));
#107533=CARTESIAN_POINT('Ctrl Pts',(-104.24332608149,1077.72268663222,428.619477357485));
#107534=CARTESIAN_POINT('Ctrl Pts',(-104.345692450359,1077.71255409562,
428.572646466051));
#107535=CARTESIAN_POINT('Ctrl Pts',(-104.550985544958,1077.6919361633,428.51433065816));
#107536=CARTESIAN_POINT('Ctrl Pts',(-104.652034278672,1077.6816652382,428.500265739785));
#107537=CARTESIAN_POINT('Ctrl Pts',(-104.753539540172,1077.67122217491,
428.500265739785));
#107538=CARTESIAN_POINT('Ctrl Pts',(-104.753539540172,1077.67122217491,
428.500265739785));
#107539=CARTESIAN_POINT('Ctrl Pts',(-104.753621771129,1077.67121371483,
428.500265739785));
#107540=CARTESIAN_POINT('Ctrl Pts',(-104.753704002386,1077.67120525463,
428.500265749015));
#107541=CARTESIAN_POINT('Ctrl Pts',(-104.75378623394,1077.67119679432,428.500265767477));
#107542=CARTESIAN_POINT('Ctrl Pts',(-104.900517796687,1077.65610046838,
428.500298709538));
#107543=CARTESIAN_POINT('Ctrl Pts',(-105.045800523816,1077.64088944,428.529721821319));
#107544=CARTESIAN_POINT('Ctrl Pts',(-105.312932914101,1077.61243730724,
428.642535747821));
#107545=CARTESIAN_POINT('Ctrl Pts',(-105.432794474776,1077.5994227841,428.723532962091));
#107546=CARTESIAN_POINT('Ctrl Pts',(-105.621654555545,1077.57850681184,
428.913983809731));
#107547=CARTESIAN_POINT('Ctrl Pts',(-105.693868838685,1077.57031405657,
429.016998651975));
#107548=CARTESIAN_POINT('Ctrl Pts',(-105.799176783322,1077.55797322637,
429.240096076958));
#107549=CARTESIAN_POINT('Ctrl Pts',(-105.832510274906,1077.55381211552,
429.358071980582));
#107550=CARTESIAN_POINT('Ctrl Pts',(-105.848955940181,1077.55129397634,
429.507852615428));
#107551=CARTESIAN_POINT('Ctrl Pts',(-105.850974463313,1077.55093190504,
429.5366519147));
#107552=CARTESIAN_POINT('Ctrl Pts',(-105.852428428032,1077.55053499933,
429.584181780693));
#107553=CARTESIAN_POINT('Ctrl Pts',(-105.852523154506,1077.55042988131,
429.602876669696));
#107554=CARTESIAN_POINT('Ctrl Pts',(-105.851836458914,1077.55033268639,
429.636453088896));
#107555=CARTESIAN_POINT('Ctrl Pts',(-105.851229370754,1077.55032197857,
429.651333327891));
#107556=CARTESIAN_POINT('Ctrl Pts',(-105.849300796291,1077.55036797892,
429.682856867601));
#107557=CARTESIAN_POINT('Ctrl Pts',(-105.847902079528,1077.55043298755,
429.699491547961));
#107558=CARTESIAN_POINT('Ctrl Pts',(-105.843181715915,1077.55071361145,
429.743575329433));
#107559=CARTESIAN_POINT('Ctrl Pts',(-105.839202285154,1077.55099996445,
429.770940923325));
#107560=CARTESIAN_POINT('Ctrl Pts',(-105.816884053324,1077.5527696387,429.892120706807));
#107561=CARTESIAN_POINT('Ctrl Pts',(-105.787389925437,1077.55545785379,
429.983420553608));
#107562=CARTESIAN_POINT('Ctrl Pts',(-105.700209827115,1077.56382072101,
430.167356278329));
#107563=CARTESIAN_POINT('Ctrl Pts',(-105.639821682493,1077.56979383656,
430.257560864994));
#107564=CARTESIAN_POINT('Ctrl Pts',(-105.485794488914,1077.58527230502,
430.427319683297));
#107565=CARTESIAN_POINT('Ctrl Pts',(-105.390018630039,1077.59501673188,
430.502974946802));
#107566=CARTESIAN_POINT('Ctrl Pts',(-105.168565812765,1077.6176822067,430.62502929099));
#107567=CARTESIAN_POINT('Ctrl Pts',(-105.042763154243,1077.63062515425,
430.667317225829));
#107568=CARTESIAN_POINT('Ctrl Pts',(-104.859791132155,1077.64948899038,
430.694078487688));
#107569=CARTESIAN_POINT('Ctrl Pts',(-104.806643653434,1077.65497302422,
430.69792801177));
#107570=CARTESIAN_POINT('Ctrl Pts',(-104.753539540173,1077.66045630879,
430.69792801177));
#107571=CARTESIAN_POINT('',(-110.796881705951,1076.79846644782,441.973714359567));
#107572=CARTESIAN_POINT('',(-110.796881705952,1076.84100217604,439.792632862112));
#107573=CARTESIAN_POINT('Ctrl Pts',(-110.796881705951,1076.79846644782,
441.973714359568));
#107574=CARTESIAN_POINT('Ctrl Pts',(-110.692273774677,1076.81241408223,
441.973714359568));
#107575=CARTESIAN_POINT('Ctrl Pts',(-110.588028811789,1076.82655918924,
441.958661837672));
#107576=CARTESIAN_POINT('Ctrl Pts',(-110.348684785172,1076.85962684279,
441.887824330035));
#107577=CARTESIAN_POINT('Ctrl Pts',(-110.219371784325,1076.877980297,441.819537372388));
#107578=CARTESIAN_POINT('Ctrl Pts',(-110.000351151244,1076.91015763524,
441.640675412221));
#107579=CARTESIAN_POINT('Ctrl Pts',(-109.910929629034,1076.923879414,441.533925201476));
#107580=CARTESIAN_POINT('Ctrl Pts',(-109.782461101245,1076.94503069519,
441.302864272028));
#107581=CARTESIAN_POINT('Ctrl Pts',(-109.74068377013,1076.9527437549,441.182689327982));
#107582=CARTESIAN_POINT('Ctrl Pts',(-109.709471388927,1076.96045410788,
440.990387616337));
#107583=CARTESIAN_POINT('Ctrl Pts',(-109.704885215509,1076.96234971779,
440.921979321037));
#107584=CARTESIAN_POINT('Ctrl Pts',(-109.70740490224,1076.96378815122,440.829188651065));
#107585=CARTESIAN_POINT('Ctrl Pts',(-109.708884892985,1076.96405957878,
440.804833727284));
#107586=CARTESIAN_POINT('Ctrl Pts',(-109.712635154749,1076.96432820452,
440.765158889882));
#107587=CARTESIAN_POINT('Ctrl Pts',(-109.71441682864,1076.96438940442,440.749802474235));
#107588=CARTESIAN_POINT('Ctrl Pts',(-109.718472879028,1076.96442436584,
440.72033081604));
#107589=CARTESIAN_POINT('Ctrl Pts',(-109.720699520378,1076.96440437256,
440.706212383326));
#107590=CARTESIAN_POINT('Ctrl Pts',(-109.726469843612,1076.96427351887,
440.673780747735));
#107591=CARTESIAN_POINT('Ctrl Pts',(-109.7302070774,1076.96413683291,440.655506898849));
#107592=CARTESIAN_POINT('Ctrl Pts',(-109.743219717341,1076.96352035238,
440.599267826861));
#107593=CARTESIAN_POINT('Ctrl Pts',(-109.754067283443,1076.96282921733,
440.561702889637));
#107594=CARTESIAN_POINT('Ctrl Pts',(-109.814439595316,1076.95830494407,
440.388188327854));
#107595=CARTESIAN_POINT('Ctrl Pts',(-109.888623562675,1076.95107882451,
440.262547084959));
#107596=CARTESIAN_POINT('Ctrl Pts',(-110.062839703741,1076.93211989836,
440.068274204388));
#107597=CARTESIAN_POINT('Ctrl Pts',(-110.154010601421,1076.9216439643,439.994622440335));
#107598=CARTESIAN_POINT('Ctrl Pts',(-110.341671486236,1076.89915372656,
439.887155452571));
#107599=CARTESIAN_POINT('Ctrl Pts',(-110.434726911207,1076.88766844724,
439.849698395017));
#107600=CARTESIAN_POINT('Ctrl Pts',(-110.618310048536,1076.86439463511,
439.803633080794));
#107601=CARTESIAN_POINT('Ctrl Pts',(-110.707453167309,1076.85284210735,
439.792632862112));
#107602=CARTESIAN_POINT('Ctrl Pts',(-110.796881705953,1076.84100217604,
439.792632862112));
#107603=CARTESIAN_POINT('Ctrl Pts',(-110.796881705953,1076.84100217604,
439.792632862112));
#107604=CARTESIAN_POINT('Ctrl Pts',(-110.797144710037,1076.8409673555,439.792632862112));
#107605=CARTESIAN_POINT('Ctrl Pts',(-110.797407716591,1076.84093253247,
439.792632957254));
#107606=CARTESIAN_POINT('Ctrl Pts',(-110.797670725563,1076.84089770697,
439.792633147545));
#107607=CARTESIAN_POINT('Ctrl Pts',(-110.940875143062,1076.82193574766,
439.792736757725));
#107608=CARTESIAN_POINT('Ctrl Pts',(-111.082679377719,1076.80251686205,
439.821046646856));
#107609=CARTESIAN_POINT('Ctrl Pts',(-111.347617338863,1076.76494997321,
439.931019391774));
#107610=CARTESIAN_POINT('Ctrl Pts',(-111.468259603526,1076.74715260503,
440.011817417049));
#107611=CARTESIAN_POINT('Ctrl Pts',(-111.663219862428,1076.7170028084,440.207700701182));
#107612=CARTESIAN_POINT('Ctrl Pts',(-111.73889487444,1076.70457505583,440.317907003865));
#107613=CARTESIAN_POINT('Ctrl Pts',(-111.850563178268,1076.68445565207,
440.568443064145));
#107614=CARTESIAN_POINT('Ctrl Pts',(-111.882534220777,1076.67732722463,
440.70781449107));
#107615=CARTESIAN_POINT('Ctrl Pts',(-111.887907283963,1076.67311846043,
440.882092345228));
#107616=CARTESIAN_POINT('Ctrl Pts',(-111.887453915195,1076.67253021244,
440.914649172624));
#107617=CARTESIAN_POINT('Ctrl Pts',(-111.884518469112,1076.67193211686,
440.96460803008));
#107618=CARTESIAN_POINT('Ctrl Pts',(-111.883071842286,1076.6717806839,440.982048878092));
#107619=CARTESIAN_POINT('Ctrl Pts',(-111.879649247935,1076.67160898888,
441.013966538923));
#107620=CARTESIAN_POINT('Ctrl Pts',(-111.877800927294,1076.67157118055,
441.028452600474));
#107621=CARTESIAN_POINT('Ctrl Pts',(-111.873474867749,1076.67157625955,
441.057670989545));
#107622=CARTESIAN_POINT('Ctrl Pts',(-111.870984243651,1076.67162100385,
441.072398091426));
#107623=CARTESIAN_POINT('Ctrl Pts',(-111.864148755149,1076.67183370564,
441.108313168006));
#107624=CARTESIAN_POINT('Ctrl Pts',(-111.859474700419,1076.67204783228,
441.12943126288));
#107625=CARTESIAN_POINT('Ctrl Pts',(-111.840686961053,1076.67311905997,
441.203767105688));
#107626=CARTESIAN_POINT('Ctrl Pts',(-111.823179257166,1076.67445681808,
441.256027453616));
#107627=CARTESIAN_POINT('Ctrl Pts',(-111.745741740518,1076.68131660462,
441.439754842337));
#107628=CARTESIAN_POINT('Ctrl Pts',(-111.663902326627,1076.6900350907,441.560138537338));
#107629=CARTESIAN_POINT('Ctrl Pts',(-111.476430942617,1076.71175599412,
441.744346762287));
#107630=CARTESIAN_POINT('Ctrl Pts',(-111.378726898161,1076.72359527886,
441.813110961287));
#107631=CARTESIAN_POINT('Ctrl Pts',(-111.155314698242,1076.75154113672,
441.921260149142));
#107632=CARTESIAN_POINT('Ctrl Pts',(-111.029570986107,1076.76772622122,
441.956431059971));
#107633=CARTESIAN_POINT('Ctrl Pts',(-110.866165924499,1076.78925564003,
441.972065634675));
#107634=CARTESIAN_POINT('Ctrl Pts',(-110.831503928816,1076.79385018115,
441.973714359568));
#107635=CARTESIAN_POINT('Ctrl Pts',(-110.796881705951,1076.79846644782,
441.973714359568));
#107636=CARTESIAN_POINT('',(-89.3961860936676,1078.67097321562,431.48354716413));
#107637=CARTESIAN_POINT('',(-89.3961860936676,1078.67555974723,428.526940899744));
#107638=CARTESIAN_POINT('Ctrl Pts',(-89.3961860936678,1078.67097321562,
431.48354716413));
#107639=CARTESIAN_POINT('Ctrl Pts',(-89.3503684205628,1078.6721747184,431.48354716413));
#107640=CARTESIAN_POINT('Ctrl Pts',(-89.3045016225727,1078.67336423892,
431.481417139091));
#107641=CARTESIAN_POINT('Ctrl Pts',(-89.0639230639002,1078.67953217154,
431.458950921387));
#107642=CARTESIAN_POINT('Ctrl Pts',(-88.8746373636803,1078.68412818373,
431.402261580626));
#107643=CARTESIAN_POINT('Ctrl Pts',(-88.5330027004404,1078.69204156997,
431.220516060359));
#107644=CARTESIAN_POINT('Ctrl Pts',(-88.3831469945233,1078.69531624797,
431.098739153579));
#107645=CARTESIAN_POINT('Ctrl Pts',(-88.1541705001929,1078.70019971376,
430.824044466892));
#107646=CARTESIAN_POINT('Ctrl Pts',(-88.0699999443497,1078.70194023454,
430.679240083613));
#107647=CARTESIAN_POINT('Ctrl Pts',(-87.9653316907437,1078.70416949295,
430.3996148194));
#107648=CARTESIAN_POINT('Ctrl Pts',(-87.9357979108968,1078.70483203888,
430.270083290523));
#107649=CARTESIAN_POINT('Ctrl Pts',(-87.9201609749338,1078.70529363399,
430.097132364434));
#107650=CARTESIAN_POINT('Ctrl Pts',(-87.9181668276158,1078.70537280154,
430.055768046747));
#107651=CARTESIAN_POINT('Ctrl Pts',(-87.9177594245223,1078.7054500744,429.989808453584));
#107652=CARTESIAN_POINT('Ctrl Pts',(-87.918220082033,1078.70546803225,429.965242250974));
#107653=CARTESIAN_POINT('Ctrl Pts',(-87.9202278753444,1078.7054814182,429.919300758652));
#107654=CARTESIAN_POINT('Ctrl Pts',(-87.9216279836036,1078.70547943631,
429.897925401036));
#107655=CARTESIAN_POINT('Ctrl Pts',(-87.9258105131604,1078.70545655004,
429.850048997176));
#107656=CARTESIAN_POINT('Ctrl Pts',(-87.9288459451285,1078.70543115622,
429.823577485973));
#107657=CARTESIAN_POINT('Ctrl Pts',(-87.9397257026432,1078.70532051322,
429.747037398998));
#107658=CARTESIAN_POINT('Ctrl Pts',(-87.9494308166955,1078.70520204839,
429.697272144726));
#107659=CARTESIAN_POINT('Ctrl Pts',(-88.009378559838,1078.7043948384,429.456481844696));
#107660=CARTESIAN_POINT('Ctrl Pts',(-88.0949993889729,1078.70306520414,
429.276351340573));
#107661=CARTESIAN_POINT('Ctrl Pts',(-88.3085838548858,1078.69933176898,
428.991517520783));
#107662=CARTESIAN_POINT('Ctrl Pts',(-88.4234937228195,1078.69721031364,
428.880794932558));
#107663=CARTESIAN_POINT('Ctrl Pts',(-88.6833406166949,1078.69203232056,
428.700602039454));
#107664=CARTESIAN_POINT('Ctrl Pts',(-88.8264409007805,1078.68901143704,
428.632063451516));
#107665=CARTESIAN_POINT('Ctrl Pts',(-89.1135426005729,1078.6825108496,428.547310221386));
#107666=CARTESIAN_POINT('Ctrl Pts',(-89.2545008260199,1078.67914164015,
428.526940899744));
#107667=CARTESIAN_POINT('Ctrl Pts',(-89.3961860936677,1078.67555974723,
428.526940899744));
#107668=CARTESIAN_POINT('Ctrl Pts',(-89.3961860936677,1078.67555974723,
428.526940899743));
#107669=CARTESIAN_POINT('Ctrl Pts',(-89.3962427801943,1078.67555831416,
428.526940899743));
#107670=CARTESIAN_POINT('Ctrl Pts',(-89.3962994668373,1078.67555688106,
428.526940902775));
#107671=CARTESIAN_POINT('Ctrl Pts',(-89.3963561535964,1078.67555544792,
428.526940909296));
#107672=CARTESIAN_POINT('Ctrl Pts',(-89.592592917535,1078.67059424695,428.526963483905));
#107673=CARTESIAN_POINT('Ctrl Pts',(-89.7868711403322,1078.66530455267,
428.566059828392));
#107674=CARTESIAN_POINT('Ctrl Pts',(-90.1455237677059,1078.65489299863,
428.716447037405));
#107675=CARTESIAN_POINT('Ctrl Pts',(-90.3069516447766,1078.64987461811,
428.824982534491));
#107676=CARTESIAN_POINT('Ctrl Pts',(-90.5639852988258,1078.64146856408,
429.082758398322));
#107677=CARTESIAN_POINT('Ctrl Pts',(-90.6629613753267,1078.63803012931,
429.224204035469));
#107678=CARTESIAN_POINT('Ctrl Pts',(-90.8046827979466,1078.6328410931,429.527513504186));
#107679=CARTESIAN_POINT('Ctrl Pts',(-90.8488395845207,1078.63105794091,
429.686037599397));
#107680=CARTESIAN_POINT('Ctrl Pts',(-90.8709485547003,1078.62990838013,
429.893463944237));
#107681=CARTESIAN_POINT('Ctrl Pts',(-90.8736746522949,1078.62972718908,
429.938560351527));
#107682=CARTESIAN_POINT('Ctrl Pts',(-90.8747098084299,1078.62955017559,
430.009618815121));
#107683=CARTESIAN_POINT('Ctrl Pts',(-90.874406017504,1078.62950828611,430.035532223773));
#107684=CARTESIAN_POINT('Ctrl Pts',(-90.8725898400971,1078.62947295051,
430.083287837502));
#107685=CARTESIAN_POINT('Ctrl Pts',(-90.8712730739436,1078.62947298496,
430.105130261123));
#107686=CARTESIAN_POINT('Ctrl Pts',(-90.8673373367039,1078.62950848658,
430.152779217494));
#107687=CARTESIAN_POINT('Ctrl Pts',(-90.8645230313847,1078.62955051016,
430.178562364891));
#107688=CARTESIAN_POINT('Ctrl Pts',(-90.8547741527985,1078.62973121606,
430.250319136657));
#107689=CARTESIAN_POINT('Ctrl Pts',(-90.8463472804366,1078.62992003172,
430.296059113835));
#107690=CARTESIAN_POINT('Ctrl Pts',(-90.7911388502875,1078.63128071601,
430.532542485652));
#107691=CARTESIAN_POINT('Ctrl Pts',(-90.7088479183431,1078.63365390632,
430.712948633658));
#107692=CARTESIAN_POINT('Ctrl Pts',(-90.5017020705458,1078.63976408734,
430.999152287797));
#107693=CARTESIAN_POINT('Ctrl Pts',(-90.3900075983879,1078.64308907709,
431.110835136399));
#107694=CARTESIAN_POINT('Ctrl Pts',(-90.1239594440925,1078.65087851801,
431.303367194158));
#107695=CARTESIAN_POINT('Ctrl Pts',(-89.9686290285824,1078.65535737901,
431.378955271829));
#107696=CARTESIAN_POINT('Ctrl Pts',(-89.6710761276956,1078.66364245453,
431.464315639791));
#107697=CARTESIAN_POINT('Ctrl Pts',(-89.5338528917158,1078.66736310127,
431.48354716413));
#107698=CARTESIAN_POINT('Ctrl Pts',(-89.3961860936678,1078.67097321562,
431.48354716413));
#107699=CARTESIAN_POINT('',(-104.994450521159,1076.76862933859,464.654297310259));
#107700=CARTESIAN_POINT('',(-104.994450521158,1076.8704842326,462.473215812804));
#107701=CARTESIAN_POINT('Ctrl Pts',(-104.994450521159,1076.76862933859,
464.65429731026));
#107702=CARTESIAN_POINT('Ctrl Pts',(-104.858658359836,1076.78586976643,
464.65429731026));
#107703=CARTESIAN_POINT('Ctrl Pts',(-104.724111967629,1076.8040722823,464.628935472442));
#107704=CARTESIAN_POINT('Ctrl Pts',(-104.462350706126,1076.84178842186,
464.526705426959));
#107705=CARTESIAN_POINT('Ctrl Pts',(-104.338796665719,1076.86094842948,
464.447262771309));
#107706=CARTESIAN_POINT('Ctrl Pts',(-104.133160632069,1076.89582341618,
464.24741888124));
#107707=CARTESIAN_POINT('Ctrl Pts',(-104.051818760982,1076.91130880812,
464.130132324092));
#107708=CARTESIAN_POINT('Ctrl Pts',(-103.949391403289,1076.93472987125,
463.895686030557));
#107709=CARTESIAN_POINT('Ctrl Pts',(-103.920333066717,1076.9434016353,463.78435057897));
#107710=CARTESIAN_POINT('Ctrl Pts',(-103.898342221727,1076.95632754564,
463.560541570395));
#107711=CARTESIAN_POINT('Ctrl Pts',(-103.904282010018,1076.96065179248,
463.449602661549));
#107712=CARTESIAN_POINT('Ctrl Pts',(-103.932945385877,1076.9634002689,463.311987610233));
#107713=CARTESIAN_POINT('Ctrl Pts',(-103.940280223014,1076.96382645952,
463.282854404866));
#107714=CARTESIAN_POINT('Ctrl Pts',(-103.953690373367,1076.96424190995,
463.237577294334));
#107715=CARTESIAN_POINT('Ctrl Pts',(-103.958961004619,1076.9643400147,463.221213010892));
#107716=CARTESIAN_POINT('Ctrl Pts',(-103.96891034016,1076.96441900298,463.192654396277));
#107717=CARTESIAN_POINT('Ctrl Pts',(-103.973425261387,1076.96442241245,
463.180406981277));
#107718=CARTESIAN_POINT('Ctrl Pts',(-103.984192399116,1076.96436037745,
463.152740253009));
#107719=CARTESIAN_POINT('Ctrl Pts',(-103.990579735707,1076.96427577895,
463.137377257781));
#107720=CARTESIAN_POINT('Ctrl Pts',(-104.008815295691,1076.96391201987,
463.096200351771));
#107721=CARTESIAN_POINT('Ctrl Pts',(-104.021323831314,1076.96353773417,
463.070694857799));
#107722=CARTESIAN_POINT('Ctrl Pts',(-104.085329266719,1076.96107805047,
462.952130525259));
#107723=CARTESIAN_POINT('Ctrl Pts',(-104.149228396746,1076.95713089861,
462.866506244061));
#107724=CARTESIAN_POINT('Ctrl Pts',(-104.301841385759,1076.94529522403,
462.714332647535));
#107725=CARTESIAN_POINT('Ctrl Pts',(-104.390321610185,1076.93736453761,
462.649315741908));
#107726=CARTESIAN_POINT('Ctrl Pts',(-104.571126005816,1076.91937744636,
462.554230757962));
#107727=CARTESIAN_POINT('Ctrl Pts',(-104.660748401951,1076.90979666082,
462.521188143708));
#107728=CARTESIAN_POINT('Ctrl Pts',(-104.83256621036,1076.89024834434,462.482248176407));
#107729=CARTESIAN_POINT('Ctrl Pts',(-104.913414836135,1076.88060035961,
462.473215812804));
#107730=CARTESIAN_POINT('Ctrl Pts',(-104.994450521158,1076.8704842326,462.473215812804));
#107731=CARTESIAN_POINT('Ctrl Pts',(-104.994450521158,1076.8704842326,462.473215812804));
#107732=CARTESIAN_POINT('Ctrl Pts',(-104.994528833149,1076.87047445649,
462.473215812804));
#107733=CARTESIAN_POINT('Ctrl Pts',(-104.994607145314,1076.87046467994,
462.473215821239));
#107734=CARTESIAN_POINT('Ctrl Pts',(-104.994685457652,1076.87045490295,
462.47321583811));
#107735=CARTESIAN_POINT('Ctrl Pts',(-105.131886787753,1076.85332585709,
462.473245395557));
#107736=CARTESIAN_POINT('Ctrl Pts',(-105.267772173138,1076.83508401853,
462.499165114115));
#107737=CARTESIAN_POINT('Ctrl Pts',(-105.530374457735,1076.79715501205,
462.602932847247));
#107738=CARTESIAN_POINT('Ctrl Pts',(-105.653583153228,1076.77780211827,
462.682850918198));
#107739=CARTESIAN_POINT('Ctrl Pts',(-105.858177340716,1076.74233967145,
462.883240741875));
#107740=CARTESIAN_POINT('Ctrl Pts',(-105.938927628521,1076.72646720446,
463.000542870787));
#107741=CARTESIAN_POINT('Ctrl Pts',(-106.043399555415,1076.70163199974,
463.241666955628));
#107742=CARTESIAN_POINT('Ctrl Pts',(-106.072798134984,1076.69218792766,
463.360574308658));
#107743=CARTESIAN_POINT('Ctrl Pts',(-106.089666298165,1076.67930832872,
463.58505686271));
#107744=CARTESIAN_POINT('Ctrl Pts',(-106.082735619161,1076.67524669101,
463.688724171103));
#107745=CARTESIAN_POINT('Ctrl Pts',(-106.055199289107,1076.67258694552,
463.818611382102));
#107746=CARTESIAN_POINT('Ctrl Pts',(-106.047963104158,1076.67216048016,
463.847041661286));
#107747=CARTESIAN_POINT('Ctrl Pts',(-106.034703928088,1076.67174195216,
463.891544105304));
#107748=CARTESIAN_POINT('Ctrl Pts',(-106.029433539461,1076.67164299098,
463.90782341647));
#107749=CARTESIAN_POINT('Ctrl Pts',(-106.018995802968,1076.6715624156,463.93764968879));
#107750=CARTESIAN_POINT('Ctrl Pts',(-106.01393724764,1076.67156516842,463.951230329643));
#107751=CARTESIAN_POINT('Ctrl Pts',(-106.002168856373,1076.67165894452,
463.980997215355));
#107752=CARTESIAN_POINT('Ctrl Pts',(-105.995336666991,1076.67176827397,
463.997130426362));
#107753=CARTESIAN_POINT('Ctrl Pts',(-105.974958748641,1076.6722404088,464.042194545623));
#107754=CARTESIAN_POINT('Ctrl Pts',(-105.960527522606,1076.67273755706,
464.070702461631));
#107755=CARTESIAN_POINT('Ctrl Pts',(-105.874190085076,1076.67652915516,
464.224143244695));
#107756=CARTESIAN_POINT('Ctrl Pts',(-105.779397311726,1076.68347705017,
464.334352387907));
#107757=CARTESIAN_POINT('Ctrl Pts',(-105.575552107716,1076.70206999252,
464.493708257795));
#107758=CARTESIAN_POINT('Ctrl Pts',(-105.474509528114,1076.7123695875,464.549637315668));
#107759=CARTESIAN_POINT('Ctrl Pts',(-105.24793524325,1076.73743542702,464.63193754997));
#107760=CARTESIAN_POINT('Ctrl Pts',(-105.122649946795,1076.75236364489,
464.654054595566));
#107761=CARTESIAN_POINT('Ctrl Pts',(-104.995838203487,1076.76845318515,
464.654296648121));
#107762=CARTESIAN_POINT('Ctrl Pts',(-104.995144346057,1076.76854124928,
464.65429731026));
#107763=CARTESIAN_POINT('Ctrl Pts',(-104.994450521159,1076.76862933859,
464.65429731026));
#107764=CARTESIAN_POINT('',(-101.429261354592,1077.63689261564,452.368613624749));
#107765=CARTESIAN_POINT('',(-101.429261354592,1077.69451627758,450.170951352764));
#107766=CARTESIAN_POINT('Ctrl Pts',(-101.429261354592,1077.63689261564,
452.368613624749));
#107767=CARTESIAN_POINT('Ctrl Pts',(-101.307605703774,1077.64915059475,
452.368613624749));
#107768=CARTESIAN_POINT('Ctrl Pts',(-101.18668444173,1077.66179391028,452.348409001666));
#107769=CARTESIAN_POINT('Ctrl Pts',(-100.933618173617,1077.6892560253,452.261258318599));
#107770=CARTESIAN_POINT('Ctrl Pts',(-100.80650567583,1077.7037342887,452.186793901045));
#107771=CARTESIAN_POINT('Ctrl Pts',(-100.592363567915,1077.72965390654,
451.995681680799));
#107772=CARTESIAN_POINT('Ctrl Pts',(-100.506087865567,1077.7409464009,451.882278538947));
#107773=CARTESIAN_POINT('Ctrl Pts',(-100.389540214887,1077.75825533559,
451.645782492565));
#107774=CARTESIAN_POINT('Ctrl Pts',(-100.354126513678,1077.76465606984,
451.52770444186));
#107775=CARTESIAN_POINT('Ctrl Pts',(-100.327844344213,1077.7724947649,451.317549332329));
#107776=CARTESIAN_POINT('Ctrl Pts',(-100.327600274001,1077.77477784652,
451.227910410291));
#107777=CARTESIAN_POINT('Ctrl Pts',(-100.341573462965,1077.77638028958,
451.111152839007));
#107778=CARTESIAN_POINT('Ctrl Pts',(-100.346012308605,1077.77665806041,
451.083235064126));
#107779=CARTESIAN_POINT('Ctrl Pts',(-100.354818929977,1077.77692965332,
451.038938135266));
#107780=CARTESIAN_POINT('Ctrl Pts',(-100.358497462294,1077.77699268214,
451.022435895688));
#107781=CARTESIAN_POINT('Ctrl Pts',(-100.365790889745,1077.77703645925,
450.992939322167));
#107782=CARTESIAN_POINT('Ctrl Pts',(-100.369267007333,1077.77703128793,
450.979914324867));
#107783=CARTESIAN_POINT('Ctrl Pts',(-100.377936166874,1077.7769618355,450.949675645639));
#107784=CARTESIAN_POINT('Ctrl Pts',(-100.383313741584,1077.77687842007,
450.932519062293));
#107785=CARTESIAN_POINT('Ctrl Pts',(-100.399756472976,1077.7765179199,450.884243895061));
#107786=CARTESIAN_POINT('Ctrl Pts',(-100.41180635154,1077.77613737507,450.853482828614));
#107787=CARTESIAN_POINT('Ctrl Pts',(-100.484498524452,1077.77328377933,
450.690009776044));
#107788=CARTESIAN_POINT('Ctrl Pts',(-100.569692629977,1077.76813739926,
450.569922918353));
#107789=CARTESIAN_POINT('Ctrl Pts',(-100.760536161183,1077.75427975263,
450.390119661033));
#107790=CARTESIAN_POINT('Ctrl Pts',(-100.857420541936,1077.7465783772,450.324289715235));
#107791=CARTESIAN_POINT('Ctrl Pts',(-101.039523498113,1077.73103967016,
450.238895285109));
#107792=CARTESIAN_POINT('Ctrl Pts',(-101.120185883533,1077.72385572255,
450.211916445114));
#107793=CARTESIAN_POINT('Ctrl Pts',(-101.277497005792,1077.7092800982,450.178829841757));
#107794=CARTESIAN_POINT('Ctrl Pts',(-101.353291460102,1077.70202396362,
450.170951352764));
#107795=CARTESIAN_POINT('Ctrl Pts',(-101.429261354593,1077.69451627758,
450.170951352764));
#107796=CARTESIAN_POINT('Ctrl Pts',(-101.429261354593,1077.69451627758,
450.170951352764));
#107797=CARTESIAN_POINT('Ctrl Pts',(-101.429339798802,1077.69450852537,
450.170951352764));
#107798=CARTESIAN_POINT('Ctrl Pts',(-101.429418243198,1077.69450077289,
450.170951361164));
#107799=CARTESIAN_POINT('Ctrl Pts',(-101.429496687781,1077.69449302015,
450.170951377965));
#107800=CARTESIAN_POINT('Ctrl Pts',(-101.570117366432,1077.6805953591,450.170981494251));
#107801=CARTESIAN_POINT('Ctrl Pts',(-101.709404414697,1077.66602412535,
450.198004259033));
#107802=CARTESIAN_POINT('Ctrl Pts',(-101.974748435885,1077.63660106094,
450.304877484262));
#107803=CARTESIAN_POINT('Ctrl Pts',(-102.097648397907,1077.6220376026,450.385530117599));
#107804=CARTESIAN_POINT('Ctrl Pts',(-102.300392047101,1077.59607630245,
450.585709210324));
#107805=CARTESIAN_POINT('Ctrl Pts',(-102.380088023211,1077.58480026738,
450.701603731434));
#107806=CARTESIAN_POINT('Ctrl Pts',(-102.486864493364,1077.56724237183,
450.945723512633));
#107807=CARTESIAN_POINT('Ctrl Pts',(-102.517236113633,1077.56073632167,
451.070034462404));
#107808=CARTESIAN_POINT('Ctrl Pts',(-102.530485864684,1077.55395826846,
451.269276335541));
#107809=CARTESIAN_POINT('Ctrl Pts',(-102.528117831316,1077.55222618741,
451.341998907716));
#107810=CARTESIAN_POINT('Ctrl Pts',(-102.515183211102,1077.5509077679,451.439717906269));
#107811=CARTESIAN_POINT('Ctrl Pts',(-102.510863569694,1077.55065819379,
451.465335737234));
#107812=CARTESIAN_POINT('Ctrl Pts',(-102.502325869235,1077.55041101153,
451.506919510223));
#107813=CARTESIAN_POINT('Ctrl Pts',(-102.498648933293,1077.5503546808,451.522985245446));
#107814=CARTESIAN_POINT('Ctrl Pts',(-102.490877143383,1077.55032261067,
451.553744166218));
#107815=CARTESIAN_POINT('Ctrl Pts',(-102.486835014044,1077.55034116096,
451.568446632));
#107816=CARTESIAN_POINT('Ctrl Pts',(-102.476813400386,1077.55046219859,
451.602138890561));
#107817=CARTESIAN_POINT('Ctrl Pts',(-102.470621270859,1077.55058857809,
451.621059535528));
#107818=CARTESIAN_POINT('Ctrl Pts',(-102.44987370328,1077.55115831956,451.679074506687));
#107819=CARTESIAN_POINT('Ctrl Pts',(-102.433605206687,1077.5517968029,451.717512673844));
#107820=CARTESIAN_POINT('Ctrl Pts',(-102.350769277051,1077.55579025146,
451.885854571335));
#107821=CARTESIAN_POINT('Ctrl Pts',(-102.260962116599,1077.561907593,452.00253898184));
#107822=CARTESIAN_POINT('Ctrl Pts',(-102.062285427086,1077.57766885212,
452.175646847466));
#107823=CARTESIAN_POINT('Ctrl Pts',(-101.961667307769,1077.58630783823,
452.23818708051));
#107824=CARTESIAN_POINT('Ctrl Pts',(-101.734338897954,1077.60696361097,
452.333240482375));
#107825=CARTESIAN_POINT('Ctrl Pts',(-101.607797366091,1077.61906373766,
452.361613190581));
#107826=CARTESIAN_POINT('Ctrl Pts',(-101.462631740008,1077.63353889845,
452.368233908657));
#107827=CARTESIAN_POINT('Ctrl Pts',(-101.445939644068,1077.63521211726,
452.368613624749));
#107828=CARTESIAN_POINT('Ctrl Pts',(-101.429261354592,1077.63689261564,
452.368613624749));
#107829=CARTESIAN_POINT('',(-95.5155706932853,1078.335920315,441.193367887108));
#107830=CARTESIAN_POINT('',(-95.5155706932855,1078.36174835417,438.642479644836));
#107831=CARTESIAN_POINT('Ctrl Pts',(-95.5155706932858,1078.335920315,441.193367887108));
#107832=CARTESIAN_POINT('Ctrl Pts',(-95.4111650117638,1078.34261218989,
441.193367887108));
#107833=CARTESIAN_POINT('Ctrl Pts',(-95.3069403455621,1078.34935333886,
441.180547621747));
#107834=CARTESIAN_POINT('Ctrl Pts',(-95.0415379989269,1078.36667274019,
441.113977418461));
#107835=CARTESIAN_POINT('Ctrl Pts',(-94.8875378294586,1078.37687478399,
441.040801713221));
#107836=CARTESIAN_POINT('Ctrl Pts',(-94.6211947967623,1078.39494797311,
440.841831258262));
#107837=CARTESIAN_POINT('Ctrl Pts',(-94.5101532264005,1078.40271926822,
440.719601144812));
#107838=CARTESIAN_POINT('Ctrl Pts',(-94.3502012312986,1078.41462450173,
440.45605199741));
#107839=CARTESIAN_POINT('Ctrl Pts',(-94.2967225248972,1078.41899296749,
440.32053829704));
#107840=CARTESIAN_POINT('Ctrl Pts',(-94.2472215401051,1078.4240533987,440.083756446023));
#107841=CARTESIAN_POINT('Ctrl Pts',(-94.2382709359166,1078.42546434301,
439.986617993523));
#107842=CARTESIAN_POINT('Ctrl Pts',(-94.2411740814405,1078.42649355455,
439.856831077137));
#107843=CARTESIAN_POINT('Ctrl Pts',(-94.243150250138,1078.42667954197,439.824300513367));
#107844=CARTESIAN_POINT('Ctrl Pts',(-94.2483461187777,1078.42686262727,
439.771980174333));
#107845=CARTESIAN_POINT('Ctrl Pts',(-94.2507902387295,1078.4269049037,439.752128525486));
#107846=CARTESIAN_POINT('Ctrl Pts',(-94.2563257391841,1078.42693323349,
439.714489567494));
#107847=CARTESIAN_POINT('Ctrl Pts',(-94.259329922922,1078.42692437279,439.696694349757));
#107848=CARTESIAN_POINT('Ctrl Pts',(-94.2670033721579,1078.42685365778,
439.656461826716));
#107849=CARTESIAN_POINT('Ctrl Pts',(-94.2719017829188,1078.42677816682,
439.634074627876));
#107850=CARTESIAN_POINT('Ctrl Pts',(-94.2883841190779,1078.42644433089,
439.567402091362));
#107851=CARTESIAN_POINT('Ctrl Pts',(-94.3017509040923,1078.42607897945,
439.523596933438));
#107852=CARTESIAN_POINT('Ctrl Pts',(-94.3755538628997,1078.42369309505,
439.321397383178));
#107853=CARTESIAN_POINT('Ctrl Pts',(-94.4648057222744,1078.41989727353,
439.175395008897));
#107854=CARTESIAN_POINT('Ctrl Pts',(-94.6729613332543,1078.40982820227,
438.95070920374));
#107855=CARTESIAN_POINT('Ctrl Pts',(-94.7815198966757,1078.40423331603,
438.865953113181));
#107856=CARTESIAN_POINT('Ctrl Pts',(-95.0000296449497,1078.39232693233,
438.745902276943));
#107857=CARTESIAN_POINT('Ctrl Pts',(-95.1053525005845,1078.38637056336,
438.705023934537));
#107858=CARTESIAN_POINT('Ctrl Pts',(-95.3131762615605,1078.37417675069,
438.654564547404));
#107859=CARTESIAN_POINT('Ctrl Pts',(-95.4142012927564,1078.36806750606,
438.642479644836));
#107860=CARTESIAN_POINT('Ctrl Pts',(-95.5155706932855,1078.36174835417,
438.642479644836));
#107861=CARTESIAN_POINT('Ctrl Pts',(-95.5155706932855,1078.36174835417,
438.642479644836));
#107862=CARTESIAN_POINT('Ctrl Pts',(-95.5156721781734,1078.36174202782,
438.642479644836));
#107863=CARTESIAN_POINT('Ctrl Pts',(-95.5157736634065,1078.36173570126,
438.642479656949));
#107864=CARTESIAN_POINT('Ctrl Pts',(-95.5158751489827,1078.36172937449,
438.642479681174));
#107865=CARTESIAN_POINT('Ctrl Pts',(-95.6819526409652,1078.3513758431,438.642519324808));
#107866=CARTESIAN_POINT('Ctrl Pts',(-95.8464280210779,1078.34061188616,
438.674996311814));
#107867=CARTESIAN_POINT('Ctrl Pts',(-96.1551547787413,1078.31939507363,
438.801767312496));
#107868=CARTESIAN_POINT('Ctrl Pts',(-96.2962316659722,1078.30915212528,
438.895441517433));
#107869=CARTESIAN_POINT('Ctrl Pts',(-96.526298600044,1078.2914383833,439.124345093502));
#107870=CARTESIAN_POINT('Ctrl Pts',(-96.6161466462865,1078.28398359501,
439.254517570002));
#107871=CARTESIAN_POINT('Ctrl Pts',(-96.7479248536023,1078.27185279146,
439.549557216462));
#107872=CARTESIAN_POINT('Ctrl Pts',(-96.7854148901343,1078.26748934377,
439.713181488898));
#107873=CARTESIAN_POINT('Ctrl Pts',(-96.7916602299975,1078.26479107824,
439.920054866255));
#107874=CARTESIAN_POINT('Ctrl Pts',(-96.790944607503,1078.26439360767,439.960709768068));
#107875=CARTESIAN_POINT('Ctrl Pts',(-96.7867037236683,1078.26397300568,
440.025475162709));
#107876=CARTESIAN_POINT('Ctrl Pts',(-96.7844275958912,1078.26386365463,
440.049638105698));
#107877=CARTESIAN_POINT('Ctrl Pts',(-96.7792072515004,1078.2637557252,440.092054590898));
#107878=CARTESIAN_POINT('Ctrl Pts',(-96.7765529539311,1078.26373694388,
440.110336439396));
#107879=CARTESIAN_POINT('Ctrl Pts',(-96.7702751038564,1078.26375567953,
440.147829154859));
#107880=CARTESIAN_POINT('Ctrl Pts',(-96.7666050904893,1078.26379652429,
440.167027316342));
#107881=CARTESIAN_POINT('Ctrl Pts',(-96.7561993855903,1078.2639788657,440.215404124046));
#107882=CARTESIAN_POINT('Ctrl Pts',(-96.7488747468521,1078.26416229516,
440.244443560783));
#107883=CARTESIAN_POINT('Ctrl Pts',(-96.7166902878999,1078.26515057891,
440.355413706194));
#107884=CARTESIAN_POINT('Ctrl Pts',(-96.6846313263266,1078.26647454538,
440.43501175105));
#107885=CARTESIAN_POINT('Ctrl Pts',(-96.588797529577,1078.27102595418,440.617553685033));
#107886=CARTESIAN_POINT('Ctrl Pts',(-96.5179040708547,1078.27478743375,
440.715802746704));
#107887=CARTESIAN_POINT('Ctrl Pts',(-96.3390656351305,1078.28487699519,
440.901522687317));
#107888=CARTESIAN_POINT('Ctrl Pts',(-96.2285097408588,1078.29142226283,
440.98436808755));
#107889=CARTESIAN_POINT('Ctrl Pts',(-95.974354769648,1078.30690338705,441.117367802158));
#107890=CARTESIAN_POINT('Ctrl Pts',(-95.8306287246488,1078.31588032969,
441.162859488262));
#107891=CARTESIAN_POINT('Ctrl Pts',(-95.6269453490775,1078.32879928642,
441.189724286364));
#107892=CARTESIAN_POINT('Ctrl Pts',(-95.571232289585,1078.33235268885,441.193367887108));
#107893=CARTESIAN_POINT('Ctrl Pts',(-95.5155706932857,1078.33592031499,
441.193367887108));
#107894=CARTESIAN_POINT('',(-5.99814689883682,1077.55052528867,530.41919439426));
#107895=CARTESIAN_POINT('',(-5.99814689883688,1077.77685018773,528.221532122276));
#107896=CARTESIAN_POINT('Ctrl Pts',(-5.99814689883686,1077.55052528867,
530.419194394261));
#107897=CARTESIAN_POINT('Ctrl Pts',(-5.99625157451302,1077.55053689014,
530.419194394261));
#107898=CARTESIAN_POINT('Ctrl Pts',(-5.99435621017774,1077.55054901575,
530.419189490521));
#107899=CARTESIAN_POINT('Ctrl Pts',(-5.95516251023783,1077.55081059178,
530.418986673861));
#107900=CARTESIAN_POINT('Ctrl Pts',(-5.91790066207507,1077.55126217839,
530.416894720419));
#107901=CARTESIAN_POINT('Ctrl Pts',(-5.80468871392544,1077.5532533346,530.404737083079));
#107902=CARTESIAN_POINT('Ctrl Pts',(-5.72964359113455,1077.55543236532,
530.388628980098));
#107903=CARTESIAN_POINT('Ctrl Pts',(-5.51807109371232,1077.56409236501,
530.319507345083));
#107904=CARTESIAN_POINT('Ctrl Pts',(-5.38980568816756,1077.57259502735,
530.246971516507));
#107905=CARTESIAN_POINT('Ctrl Pts',(-5.18501442972,1077.59256506602,530.069931278608));
#107906=CARTESIAN_POINT('Ctrl Pts',(-5.10520905667489,1077.60328642072,
529.972780228673));
#107907=CARTESIAN_POINT('Ctrl Pts',(-4.97682800013577,1077.62765370819,
529.747500600443));
#107908=CARTESIAN_POINT('Ctrl Pts',(-4.93227056529072,1077.6412613617,529.619387270914));
#107909=CARTESIAN_POINT('Ctrl Pts',(-4.89011014567468,1077.67001268881,
529.34370690663));
#107910=CARTESIAN_POINT('Ctrl Pts',(-4.89663170480415,1077.68492512121,
529.197982555071));
#107911=CARTESIAN_POINT('Ctrl Pts',(-4.96566336731164,1077.71307903982,
528.917606861634));
#107912=CARTESIAN_POINT('Ctrl Pts',(-5.0274178409016,1077.72605912643,528.785583485956));
#107913=CARTESIAN_POINT('Ctrl Pts',(-5.19233601030598,1077.74763244216,
528.561412409395));
#107914=CARTESIAN_POINT('Ctrl Pts',(-5.29073346742357,1077.75630078835,
528.468914039881));
#107915=CARTESIAN_POINT('Ctrl Pts',(-5.49533693715638,1077.7682395786,528.337229939953));
#107916=CARTESIAN_POINT('Ctrl Pts',(-5.5955710041969,1077.77214423415,528.292100479986));
#107917=CARTESIAN_POINT('Ctrl Pts',(-5.74421572185004,1077.7754395239,528.250327385468));
#107918=CARTESIAN_POINT('Ctrl Pts',(-5.78828107617766,1077.77613099263,
528.240819421478));
#107919=CARTESIAN_POINT('Ctrl Pts',(-5.86233038665581,1077.77682681411,
528.229549148356));
#107920=CARTESIAN_POINT('Ctrl Pts',(-5.89202299874192,1077.77698389145,
528.226261187363));
#107921=CARTESIAN_POINT('Ctrl Pts',(-5.94721628748892,1077.77705135184,
528.222417728899));
#107922=CARTESIAN_POINT('Ctrl Pts',(-5.97267302793693,1077.77699463516,
528.22153234558));
#107923=CARTESIAN_POINT('Ctrl Pts',(-5.99813726465766,1077.77685024236,
528.221532122318));
#107924=CARTESIAN_POINT('Ctrl Pts',(-5.99814689883633,1077.77685018773,
528.221532122276));
#107925=CARTESIAN_POINT('Ctrl Pts',(-6.03403752468953,1077.77664664181,
528.221532122276));
#107926=CARTESIAN_POINT('Ctrl Pts',(-6.06989519952883,1077.77626926427,
528.223289913179));
#107927=CARTESIAN_POINT('Ctrl Pts',(-6.17620342407288,1077.774631476,528.233736703841));
#107928=CARTESIAN_POINT('Ctrl Pts',(-6.24594319565952,1077.77287310659,
528.24749148978));
#107929=CARTESIAN_POINT('Ctrl Pts',(-6.45376854617888,1077.76550530709,
528.309830747198));
#107930=CARTESIAN_POINT('Ctrl Pts',(-6.58379450417654,1077.75786641588,
528.379239756435));
#107931=CARTESIAN_POINT('Ctrl Pts',(-6.79255995050972,1077.73947563506,
528.551046657383));
#107932=CARTESIAN_POINT('Ctrl Pts',(-6.8744895962233,1077.72947377155,528.645890896189));
#107933=CARTESIAN_POINT('Ctrl Pts',(-7.00828360006629,1077.70628653847,
528.867441368));
#107934=CARTESIAN_POINT('Ctrl Pts',(-7.0560413653166,1077.69309881595,528.994276264719));
#107935=CARTESIAN_POINT('Ctrl Pts',(-7.1052442529102,1077.6646610266,529.268780480461));
#107936=CARTESIAN_POINT('Ctrl Pts',(-7.10242420913194,1077.64959680605,
529.414720044921));
#107937=CARTESIAN_POINT('Ctrl Pts',(-7.0404778165884,1077.62059389268,529.696955104784));
#107938=CARTESIAN_POINT('Ctrl Pts',(-6.98200917043208,1077.6069278055,529.830611541411));
#107939=CARTESIAN_POINT('Ctrl Pts',(-6.82220676816419,1077.58375419136,
530.059609284421));
#107940=CARTESIAN_POINT('Ctrl Pts',(-6.72543730811032,1077.57422170571,
530.155034572304));
#107941=CARTESIAN_POINT('Ctrl Pts',(-6.51859958642837,1077.56060987426,
530.29490747696));
#107942=CARTESIAN_POINT('Ctrl Pts',(-6.41396045197862,1077.55601586345,
530.343953694494));
#107943=CARTESIAN_POINT('Ctrl Pts',(-6.25908219165767,1077.55217890304,
530.388767037483));
#107944=CARTESIAN_POINT('Ctrl Pts',(-6.21382930607271,1077.55138257418,
530.398813970393));
#107945=CARTESIAN_POINT('Ctrl Pts',(-6.1381096864318,1077.55057980532,530.41066599318));
#107946=CARTESIAN_POINT('Ctrl Pts',(-6.10796468216702,1077.55039594603,
530.414113590531));
#107947=CARTESIAN_POINT('Ctrl Pts',(-6.05123494798002,1077.55030312154,
530.418232290127));
#107948=CARTESIAN_POINT('Ctrl Pts',(-6.024694848476,1077.55036278595,530.419194394261));
#107949=CARTESIAN_POINT('Ctrl Pts',(-5.99814689883686,1077.55052528867,
530.419194394261));
#107950=CARTESIAN_POINT('',(-14.9669751953828,1078.26481065249,521.463636077531));
#107951=CARTESIAN_POINT('',(-14.9669751953831,1078.42603095152,518.912747835258));
#107952=CARTESIAN_POINT('Ctrl Pts',(-14.9669751953828,1078.26481065249,
521.463636077531));
#107953=CARTESIAN_POINT('Ctrl Pts',(-14.8840637748006,1078.26570128176,
521.463636077531));
#107954=CARTESIAN_POINT('Ctrl Pts',(-14.8013579449129,1078.26714355705,
521.455551522256));
#107955=CARTESIAN_POINT('Ctrl Pts',(-14.5537465604665,1078.27313268402,
521.406685807278));
#107956=CARTESIAN_POINT('Ctrl Pts',(-14.3957277923221,1078.27929036862,
521.34106585285));
#107957=CARTESIAN_POINT('Ctrl Pts',(-14.1357242669877,1078.29378715813,
521.166203806205));
#107958=CARTESIAN_POINT('Ctrl Pts',(-14.0307601869211,1078.30155359426,
521.066235321447));
#107959=CARTESIAN_POINT('Ctrl Pts',(-13.8520520489992,1078.31915918547,
520.826719033803));
#107960=CARTESIAN_POINT('Ctrl Pts',(-13.7828050194282,1078.32896433589,
520.686686188885));
#107961=CARTESIAN_POINT('Ctrl Pts',(-13.6948414272472,1078.34958104434,
520.377975725675));
#107962=CARTESIAN_POINT('Ctrl Pts',(-13.6809576326698,1078.36021810875,
520.210865778312));
#107963=CARTESIAN_POINT('Ctrl Pts',(-13.7182217730068,1078.38034555768,
519.879215693371));
#107964=CARTESIAN_POINT('Ctrl Pts',(-13.7695938782063,1078.38963277858,
519.717909230261));
#107965=CARTESIAN_POINT('Ctrl Pts',(-13.9268469953116,1078.40516638536,
519.433448029209));
#107966=CARTESIAN_POINT('Ctrl Pts',(-14.0277996544593,1078.41143642874,
519.310988082309));
#107967=CARTESIAN_POINT('Ctrl Pts',(-14.2531230341966,1078.42038035336,
519.122466835079));
#107968=CARTESIAN_POINT('Ctrl Pts',(-14.3710958524674,1078.42336647845,
519.052279763025));
#107969=CARTESIAN_POINT('Ctrl Pts',(-14.5470792565021,1078.42579035591,
518.982689924465));
#107970=CARTESIAN_POINT('Ctrl Pts',(-14.5973600212422,1078.42627852434,
518.96633568821));
#107971=CARTESIAN_POINT('Ctrl Pts',(-14.6812535315019,1078.42676739158,
518.944703244199));
#107972=CARTESIAN_POINT('Ctrl Pts',(-14.7143189158074,1078.42688008554,
518.937565758563));
#107973=CARTESIAN_POINT('Ctrl Pts',(-14.7783386230042,1078.42694625596,
518.926389366863));
#107974=CARTESIAN_POINT('Ctrl Pts',(-14.8092344514433,1078.42691145112,
518.922155866722));
#107975=CARTESIAN_POINT('Ctrl Pts',(-14.8801991700964,1078.42667968432,
518.915070148516));
#107976=CARTESIAN_POINT('Ctrl Pts',(-14.9203095720602,1078.42643908678,
518.912969845802));
#107977=CARTESIAN_POINT('Ctrl Pts',(-14.9626259596285,1078.42606986321,
518.912753396805));
#107978=CARTESIAN_POINT('Ctrl Pts',(-14.9648005775582,1078.42605056793,
518.912747835258));
#107979=CARTESIAN_POINT('Ctrl Pts',(-14.9669751953831,1078.42603095152,
518.912747835258));
#107980=CARTESIAN_POINT('Ctrl Pts',(-14.9669751953831,1078.42603095152,
518.912747835258));
#107981=CARTESIAN_POINT('Ctrl Pts',(-14.9669963294508,1078.42603076088,
518.912747835258));
#107982=CARTESIAN_POINT('Ctrl Pts',(-14.9670174635184,1078.42603057021,
518.912747835782));
#107983=CARTESIAN_POINT('Ctrl Pts',(-14.9670385975861,1078.42603037951,
518.912747836833));
#107984=CARTESIAN_POINT('Ctrl Pts',(-15.0508711366131,1078.42527391702,
518.91275200414));
#107985=CARTESIAN_POINT('Ctrl Pts',(-15.1344926621712,1078.42404252594,
518.921021396378));
#107986=CARTESIAN_POINT('Ctrl Pts',(-15.3828314393348,1078.41892080874,
518.970602243735));
#107987=CARTESIAN_POINT('Ctrl Pts',(-15.5406578597173,1078.41365282696,
519.036534404558));
#107988=CARTESIAN_POINT('Ctrl Pts',(-15.8007897652478,1078.40085990006,
519.212270378563));
#107989=CARTESIAN_POINT('Ctrl Pts',(-15.9059426375644,1078.39386650394,
519.312987051048));
#107990=CARTESIAN_POINT('Ctrl Pts',(-16.084764132545,1078.37752517669,519.554451961017));
#107991=CARTESIAN_POINT('Ctrl Pts',(-16.1537850219646,1078.36816898871,
519.695711086767));
#107992=CARTESIAN_POINT('Ctrl Pts',(-16.2405780395232,1078.34781501935,
520.007222418239));
#107993=CARTESIAN_POINT('Ctrl Pts',(-16.2533116890618,1078.33694060142,
520.175863473803));
#107994=CARTESIAN_POINT('Ctrl Pts',(-16.2128993166143,1078.31582637112,
520.508233024411));
#107995=CARTESIAN_POINT('Ctrl Pts',(-16.1602105279201,1078.30579044325,
520.66878949279));
#107996=CARTESIAN_POINT('Ctrl Pts',(-16.0013218645856,1078.28866975536,
520.950589724364));
#107997=CARTESIAN_POINT('Ctrl Pts',(-15.900313741323,1078.28157880434,521.071390335792));
#107998=CARTESIAN_POINT('Ctrl Pts',(-15.6764206193954,1078.27138154275,
521.256600438396));
#107999=CARTESIAN_POINT('Ctrl Pts',(-15.5599847466809,1078.26792207522,
521.32536687353));
#108000=CARTESIAN_POINT('Ctrl Pts',(-15.3859927535195,1078.26508682437,
521.393990512086));
#108001=CARTESIAN_POINT('Ctrl Pts',(-15.3358988461925,1078.26450957978,
521.410248306169));
#108002=CARTESIAN_POINT('Ctrl Pts',(-15.2520147660141,1078.26392919726,
521.431842308626));
#108003=CARTESIAN_POINT('Ctrl Pts',(-15.2187614326536,1078.2637954148,521.438998694873));
#108004=CARTESIAN_POINT('Ctrl Pts',(-15.1541290539122,1078.26371955013,
521.450225879352));
#108005=CARTESIAN_POINT('Ctrl Pts',(-15.1228063827288,1078.26376461504,
521.454475027578));
#108006=CARTESIAN_POINT('Ctrl Pts',(-15.0504852084235,1078.26405564199,
521.46156167709));
#108007=CARTESIAN_POINT('Ctrl Pts',(-15.0094433975959,1078.26435760333,
521.463590190717));
#108008=CARTESIAN_POINT('Ctrl Pts',(-14.9679093429678,1078.2648006355,521.46363582097));
#108009=CARTESIAN_POINT('Ctrl Pts',(-14.9674422659131,1078.26480563524,
521.463636077531));
#108010=CARTESIAN_POINT('Ctrl Pts',(-14.9669751953828,1078.26481065249,
521.463636077531));
#108011=CARTESIAN_POINT('',(-22.5035000139861,1078.63105472707,512.783427991792));
#108012=CARTESIAN_POINT('',(-22.5035000139863,1078.70463504016,509.826821727405));
#108013=CARTESIAN_POINT('Ctrl Pts',(-22.503500013986,1078.63105472707,512.783427991792));
#108014=CARTESIAN_POINT('Ctrl Pts',(-22.4866131393249,1078.63119537603,
512.783427991792));
#108015=CARTESIAN_POINT('Ctrl Pts',(-22.4697230374544,1078.63134520182,
512.783138640098));
#108016=CARTESIAN_POINT('Ctrl Pts',(-22.2564438309899,1078.63335213982,
512.775825059762));
#108017=CARTESIAN_POINT('Ctrl Pts',(-22.0633670060187,1078.63640805523,
512.729999251495));
#108018=CARTESIAN_POINT('Ctrl Pts',(-21.73593348499,1078.64364815094,512.579145630744));
#108019=CARTESIAN_POINT('Ctrl Pts',(-21.5994177766968,1078.64750787693,
512.486190611309));
#108020=CARTESIAN_POINT('Ctrl Pts',(-21.3532336058568,1078.65616653841,
512.250402802075));
#108021=CARTESIAN_POINT('Ctrl Pts',(-21.2484882435221,1078.66094147988,
512.106128332391));
#108022=CARTESIAN_POINT('Ctrl Pts',(-21.0895328385584,1078.6707535532,511.776217186613));
#108023=CARTESIAN_POINT('Ctrl Pts',(-21.0408755713378,1078.67569105934,
511.591422106885));
#108024=CARTESIAN_POINT('Ctrl Pts',(-21.0155711088123,1078.68487174283,
511.208000152065));
#108025=CARTESIAN_POINT('Ctrl Pts',(-21.041320678264,1078.68900204053,511.012881063472));
#108026=CARTESIAN_POINT('Ctrl Pts',(-21.1643993578183,1078.69582055692,
510.651631738279));
#108027=CARTESIAN_POINT('Ctrl Pts',(-21.2575622877129,1078.69850743778,
510.487879708474));
#108028=CARTESIAN_POINT('Ctrl Pts',(-21.4986248017531,1078.70259043296,
510.20524567757));
#108029=CARTESIAN_POINT('Ctrl Pts',(-21.6438032309659,1078.70397036822,
510.088394310602));
#108030=CARTESIAN_POINT('Ctrl Pts',(-21.8639162363545,1078.70501767972,
509.970765468915));
#108031=CARTESIAN_POINT('Ctrl Pts',(-21.9230371623637,1078.70521343827,
509.944005713321));
#108032=CARTESIAN_POINT('Ctrl Pts',(-22.0203370579845,1078.70540677582,
509.907461311816));
#108033=CARTESIAN_POINT('Ctrl Pts',(-22.0574823032989,1078.70545205536,
509.895168107777));
#108034=CARTESIAN_POINT('Ctrl Pts',(-22.1279356992911,1078.7054856114,509.874914760205));
#108035=CARTESIAN_POINT('Ctrl Pts',(-22.1611181117293,1078.70548032343,
509.866610307785));
#108036=CARTESIAN_POINT('Ctrl Pts',(-22.2359581713495,1078.70542160338,
509.850616793126));
#108037=CARTESIAN_POINT('Ctrl Pts',(-22.2777187020305,1078.70535704858,
509.843552027201));
#108038=CARTESIAN_POINT('Ctrl Pts',(-22.3806344301835,1078.70511991512,
509.830658027611));
#108039=CARTESIAN_POINT('Ctrl Pts',(-22.4419602626397,1078.70491208442,
509.826828139419));
#108040=CARTESIAN_POINT('Ctrl Pts',(-22.5033457918472,1078.70463573459,
509.82682173545));
#108041=CARTESIAN_POINT('Ctrl Pts',(-22.503397199361,1078.70463550316,509.826821730087));
#108042=CARTESIAN_POINT('Ctrl Pts',(-22.5034486067408,1078.70463527168,
509.826821727406));
#108043=CARTESIAN_POINT('Ctrl Pts',(-22.5035000139863,1078.70463504016,
509.826821727406));
#108044=CARTESIAN_POINT('Ctrl Pts',(-22.5035000139863,1078.70463504015,
509.826821727406));
#108045=CARTESIAN_POINT('Ctrl Pts',(-22.6999431535576,1078.70375031174,
509.826821727406));
#108046=CARTESIAN_POINT('Ctrl Pts',(-22.8944252605779,1078.70218239496,
509.86597802692));
#108047=CARTESIAN_POINT('Ctrl Pts',(-23.2260476523347,1078.69795920695,
510.005147255519));
#108048=CARTESIAN_POINT('Ctrl Pts',(-23.3650410264147,1078.69555650679,
510.092788524152));
#108049=CARTESIAN_POINT('Ctrl Pts',(-23.618871788352,1078.68952227114,510.318934274039));
#108050=CARTESIAN_POINT('Ctrl Pts',(-23.7286918856681,1078.68584927833,
510.459238343909));
#108051=CARTESIAN_POINT('Ctrl Pts',(-23.8996148619197,1078.67729450252,
510.78337132357));
#108052=CARTESIAN_POINT('Ctrl Pts',(-23.9549745129172,1078.67241982118,
510.966629185851));
#108053=CARTESIAN_POINT('Ctrl Pts',(-23.9939459883892,1078.66216114497,
511.349253265408));
#108054=CARTESIAN_POINT('Ctrl Pts',(-23.9751487448127,1078.65686949352,
511.545184600554));
#108055=CARTESIAN_POINT('Ctrl Pts',(-23.8647850039104,1078.64713354384,
511.91127044371));
#108056=CARTESIAN_POINT('Ctrl Pts',(-23.777045119279,1078.64275876997,512.078818369425));
#108057=CARTESIAN_POINT('Ctrl Pts',(-23.5377300378039,1078.63538886956,
512.379615425074));
#108058=CARTESIAN_POINT('Ctrl Pts',(-23.3855469346556,1078.6325554677,512.507691403558));
#108059=CARTESIAN_POINT('Ctrl Pts',(-23.1537877386577,1078.63041905963,
512.634417826553));
#108060=CARTESIAN_POINT('Ctrl Pts',(-23.0927105917142,1078.63002172931,
512.662594950278));
#108061=CARTESIAN_POINT('Ctrl Pts',(-22.992561123175,1078.62962914044,512.700760374292));
#108062=CARTESIAN_POINT('Ctrl Pts',(-22.9546311509793,1078.62953636008,
512.713478499856));
#108063=CARTESIAN_POINT('Ctrl Pts',(-22.8826389400606,1078.62946389858,
512.73441060299));
#108064=CARTESIAN_POINT('Ctrl Pts',(-22.8487095354434,1078.62947153576,
512.742982448831));
#108065=CARTESIAN_POINT('Ctrl Pts',(-22.7727869887952,1078.62958044117,
512.759320835298));
#108066=CARTESIAN_POINT('Ctrl Pts',(-22.7306968491649,1078.62970188294,
512.766488257087));
#108067=CARTESIAN_POINT('Ctrl Pts',(-22.6270231116153,1078.63014849078,
512.779554805226));
#108068=CARTESIAN_POINT('Ctrl Pts',(-22.5652831616516,1078.63054014191,
512.783427991792));
#108069=CARTESIAN_POINT('Ctrl Pts',(-22.503500013986,1078.63105472707,512.783427991792));
#108070=CARTESIAN_POINT('',(-3.9889441036734,1078.62952598896,515.567896071097));
#108071=CARTESIAN_POINT('',(-3.98894410367367,1078.70545282671,512.611289806711));
#108072=CARTESIAN_POINT('Ctrl Pts',(-3.98894410367339,1078.62952598896,
515.567896071097));
#108073=CARTESIAN_POINT('Ctrl Pts',(-3.97557954633002,1078.62954585557,
515.567896071097));
#108074=CARTESIAN_POINT('Ctrl Pts',(-3.96221426603179,1078.62957176346,
515.567714838267));
#108075=CARTESIAN_POINT('Ctrl Pts',(-3.8925818337087,1078.62973820289,515.565825684791));
#108076=CARTESIAN_POINT('Ctrl Pts',(-3.83644530112953,1078.62997953828,
515.561086337221));
#108077=CARTESIAN_POINT('Ctrl Pts',(-3.66587032856376,1078.63103846207,
515.536817915507));
#108078=CARTESIAN_POINT('Ctrl Pts',(-3.55334980457449,1078.63219293344,
515.507017548996));
#108079=CARTESIAN_POINT('Ctrl Pts',(-3.2618459890488,1078.63638717737,515.391782908239));
#108080=CARTESIAN_POINT('Ctrl Pts',(-3.09462218266161,1078.6401407127,515.283136431196));
#108081=CARTESIAN_POINT('Ctrl Pts',(-2.8322928991613,1078.64848047957,515.025786265432));
#108082=CARTESIAN_POINT('Ctrl Pts',(-2.73235785647567,1078.65281227588,
514.886641081079));
#108083=CARTESIAN_POINT('Ctrl Pts',(-2.57893237056587,1078.66214960547,
514.569620538358));
#108084=CARTESIAN_POINT('Ctrl Pts',(-2.53056467850437,1078.66709701536,
514.392396344916));
#108085=CARTESIAN_POINT('Ctrl Pts',(-2.49961058230914,1078.67693702634,
514.016309205842));
#108086=CARTESIAN_POINT('Ctrl Pts',(-2.52228850411433,1078.68170124812,
513.820494124643));
#108087=CARTESIAN_POINT('Ctrl Pts',(-2.64179113186497,1078.69007640222,
513.450943900934));
#108088=CARTESIAN_POINT('Ctrl Pts',(-2.73668149203204,1078.6936230876,513.280556001807));
#108089=CARTESIAN_POINT('Ctrl Pts',(-2.97657675542087,1078.6991469545,512.99778433898));
#108090=CARTESIAN_POINT('Ctrl Pts',(-3.11497587303917,1078.70118866009,
512.884139562166));
#108091=CARTESIAN_POINT('Ctrl Pts',(-3.38118250318559,1078.70371200763,
512.736030196637));
#108092=CARTESIAN_POINT('Ctrl Pts',(-3.49964810861994,1078.70446243519,
512.68884436575));
#108093=CARTESIAN_POINT('Ctrl Pts',(-3.68054142585995,1078.70514282573,
512.64258404416));
#108094=CARTESIAN_POINT('Ctrl Pts',(-3.7392458118229,1078.70529591639,512.631307042471));
#108095=CARTESIAN_POINT('Ctrl Pts',(-3.84050239514498,1078.70544857754,
512.618150902082));
#108096=CARTESIAN_POINT('Ctrl Pts',(-3.882749205525,1078.70547971775,512.614499973586));
#108097=CARTESIAN_POINT('Ctrl Pts',(-3.94635948868066,1078.70547820009,
512.611749999776));
#108098=CARTESIAN_POINT('Ctrl Pts',(-3.96764200581816,1078.70546957949,
512.611290052986));
#108099=CARTESIAN_POINT('Ctrl Pts',(-3.98892700603221,1078.70545284015,
512.61128980681));
#108100=CARTESIAN_POINT('Ctrl Pts',(-3.98893270524644,1078.70545283567,
512.611289806744));
#108101=CARTESIAN_POINT('Ctrl Pts',(-3.98893840446025,1078.70545283119,
512.611289806711));
#108102=CARTESIAN_POINT('Ctrl Pts',(-3.98894410367366,1078.70545282671,
512.611289806711));
#108103=CARTESIAN_POINT('Ctrl Pts',(-3.98894410367366,1078.70545282671,
512.611289806711));
#108104=CARTESIAN_POINT('Ctrl Pts',(-4.03787639450469,1078.7054143345,512.611289806711));
#108105=CARTESIAN_POINT('Ctrl Pts',(-4.08677847020839,1078.70533300906,
512.613719318494));
#108106=CARTESIAN_POINT('Ctrl Pts',(-4.22075193636127,1078.70499064457,
512.627064134004));
#108107=CARTESIAN_POINT('Ctrl Pts',(-4.30513368183501,1078.7046414018,512.642959141823));
#108108=CARTESIAN_POINT('Ctrl Pts',(-4.57794119745513,1078.70304202139,
512.719370449642));
#108109=CARTESIAN_POINT('Ctrl Pts',(-4.75561195822102,1078.70123179215,
512.810279607493));
#108110=CARTESIAN_POINT('Ctrl Pts',(-5.04059969034957,1078.69650907921,
513.037346969308));
#108111=CARTESIAN_POINT('Ctrl Pts',(-5.1525179032029,1078.69384088833,513.162612966679));
#108112=CARTESIAN_POINT('Ctrl Pts',(-5.3366551908863,1078.68725408687,513.456080988321));
#108113=CARTESIAN_POINT('Ctrl Pts',(-5.40360259185759,1078.68330499974,
513.624408312825));
#108114=CARTESIAN_POINT('Ctrl Pts',(-5.47638507738358,1078.67425140327,
513.989526988659));
#108115=CARTESIAN_POINT('Ctrl Pts',(-5.47675302990086,1078.6691679112,514.184005102085));
#108116=CARTESIAN_POINT('Ctrl Pts',(-5.40256299088101,1078.65877709986,
514.563722667025));
#108117=CARTESIAN_POINT('Ctrl Pts',(-5.32809344979178,1078.65357300242,
514.745184755656));
#108118=CARTESIAN_POINT('Ctrl Pts',(-5.11867735485001,1078.64429362908,
515.06072666782));
#108119=CARTESIAN_POINT('Ctrl Pts',(-4.98881577998556,1078.64026196557,
515.193977130005));
#108120=CARTESIAN_POINT('Ctrl Pts',(-4.70670876744872,1078.63429634077,
515.391832795471));
#108121=CARTESIAN_POINT('Ctrl Pts',(-4.56154984555295,1078.63219753844,
515.461869640279));
#108122=CARTESIAN_POINT('Ctrl Pts',(-4.34326753126651,1078.63038212659,
515.526391544756));
#108123=CARTESIAN_POINT('Ctrl Pts',(-4.27730879521058,1078.6299914462,515.541068519988));
#108124=CARTESIAN_POINT('Ctrl Pts',(-4.16613656476757,1078.6295950361,515.557926493658));
#108125=CARTESIAN_POINT('Ctrl Pts',(-4.12141087466975,1078.62950448441,
515.562635088888));
#108126=CARTESIAN_POINT('Ctrl Pts',(-4.04737063402253,1078.62946800522,
515.567030028428));
#108127=CARTESIAN_POINT('Ctrl Pts',(-4.0181590962076,1078.62948256043,515.567896071097));
#108128=CARTESIAN_POINT('Ctrl Pts',(-3.98894410367339,1078.62952598896,
515.567896071097));
#108129=CARTESIAN_POINT('',(-41.3143294401482,1076.68214102845,529.795163061528));
#108130=CARTESIAN_POINT('',(-41.3143294401472,1076.95433007119,527.614081564072));
#108131=CARTESIAN_POINT('Ctrl Pts',(-41.3143294401484,1076.68214102845,
529.795163061529));
#108132=CARTESIAN_POINT('Ctrl Pts',(-41.2773532062123,1076.68401340828,
529.795163061529));
#108133=CARTESIAN_POINT('Ctrl Pts',(-41.2403641585233,1076.68612555935,
529.793282476709));
#108134=CARTESIAN_POINT('Ctrl Pts',(-41.0916802738423,1076.69558300308,
529.778094241651));
#108135=CARTESIAN_POINT('Ctrl Pts',(-40.982442325362,1076.70474658777,529.74946695222));
#108136=CARTESIAN_POINT('Ctrl Pts',(-40.7657520329234,1076.72761663204,
529.655283541194));
#108137=CARTESIAN_POINT('Ctrl Pts',(-40.661332177464,1076.74153707759,529.586781886565));
#108138=CARTESIAN_POINT('Ctrl Pts',(-40.472571066346,1076.77317219352,529.410836213898));
#108139=CARTESIAN_POINT('Ctrl Pts',(-40.3921931906226,1076.79084766685,
529.302041545776));
#108140=CARTESIAN_POINT('Ctrl Pts',(-40.2704123107375,1076.82820945122,
529.051586041641));
#108141=CARTESIAN_POINT('Ctrl Pts',(-40.2336512592061,1076.84759879574,
528.910344328474));
#108142=CARTESIAN_POINT('Ctrl Pts',(-40.2174768337832,1076.88394278164,
528.623315243353));
#108143=CARTESIAN_POINT('Ctrl Pts',(-40.237542682625,1076.90058944192,528.480248851961));
#108144=CARTESIAN_POINT('Ctrl Pts',(-40.3273254919708,1076.92777386773,
528.223240517014));
#108145=CARTESIAN_POINT('Ctrl Pts',(-40.3911653338904,1076.93854435829,
528.109837635294));
#108146=CARTESIAN_POINT('Ctrl Pts',(-40.5462307588409,1076.95395240713,
527.92209964645));
#108147=CARTESIAN_POINT('Ctrl Pts',(-40.6323854102545,1076.95906150556,
527.84595306808));
#108148=CARTESIAN_POINT('Ctrl Pts',(-40.7612077031207,1076.96281651451,
527.763982304864));
#108149=CARTESIAN_POINT('Ctrl Pts',(-40.794600371696,1076.96349818409,527.745127807664));
#108150=CARTESIAN_POINT('Ctrl Pts',(-40.8496698516572,1076.96416939454,
527.717754792231));
#108151=CARTESIAN_POINT('Ctrl Pts',(-40.8707433593247,1076.96432584668,
527.708104629852));
#108152=CARTESIAN_POINT('Ctrl Pts',(-40.9091996231162,1076.9644334277,527.691956251063));
#108153=CARTESIAN_POINT('Ctrl Pts',(-40.9264705446296,1076.96441935555,
527.685216505806));
#108154=CARTESIAN_POINT('Ctrl Pts',(-40.9671508477464,1076.96424215317,
527.67052511976));
#108155=CARTESIAN_POINT('Ctrl Pts',(-40.990674735862,1076.96403095435,527.662922966839));
#108156=CARTESIAN_POINT('Ctrl Pts',(-41.0577495325793,1076.96312540197,
527.643738036847));
#108157=CARTESIAN_POINT('Ctrl Pts',(-41.1017823575711,1076.96217742873,
527.634047185999));
#108158=CARTESIAN_POINT('Ctrl Pts',(-41.2018975214531,1076.95923923163,
527.618433245831));
#108159=CARTESIAN_POINT('Ctrl Pts',(-41.258081909659,1076.95705246719,527.614081564072));
#108160=CARTESIAN_POINT('Ctrl Pts',(-41.3143294401472,1076.95433007119,
527.614081564072));
#108161=CARTESIAN_POINT('Ctrl Pts',(-41.3143294401472,1076.95433007119,
527.614081564072));
#108162=CARTESIAN_POINT('Ctrl Pts',(-41.3143342582443,1076.954329838,527.614081564072));
#108163=CARTESIAN_POINT('Ctrl Pts',(-41.3143390763419,1076.9543296048,527.614081564095));
#108164=CARTESIAN_POINT('Ctrl Pts',(-41.3143438944399,1076.95432937159,
527.614081564159));
#108165=CARTESIAN_POINT('Ctrl Pts',(-41.4218177571127,1076.94912743262,
527.61408298865));
#108166=CARTESIAN_POINT('Ctrl Pts',(-41.5285839269821,1076.94201581872,
527.629970842879));
#108167=CARTESIAN_POINT('Ctrl Pts',(-41.7465398764455,1076.92332522854,
527.696156819038));
#108168=CARTESIAN_POINT('Ctrl Pts',(-41.8551083744335,1076.91143242287,
527.750008868671));
#108169=CARTESIAN_POINT('Ctrl Pts',(-42.0589640033117,1076.8833436954,527.897149040317));
#108170=CARTESIAN_POINT('Ctrl Pts',(-42.1505015252907,1076.8670766189,527.992418056515));
#108171=CARTESIAN_POINT('Ctrl Pts',(-42.3011123191613,1076.83147634675,
528.219303416123));
#108172=CARTESIAN_POINT('Ctrl Pts',(-42.3556523794505,1076.81231881471,
528.351193817558));
#108173=CARTESIAN_POINT('Ctrl Pts',(-42.4119343242816,1076.7744051732,528.631303749692));
#108174=CARTESIAN_POINT('Ctrl Pts',(-42.4120238714279,1076.75601786499,
528.777213302029));
#108175=CARTESIAN_POINT('Ctrl Pts',(-42.3567499892214,1076.72393871357,
529.052853298823));
#108176=CARTESIAN_POINT('Ctrl Pts',(-42.3049903317031,1076.71031796148,
529.18066405343));
#108177=CARTESIAN_POINT('Ctrl Pts',(-42.1543372528411,1076.68820744054,
529.414238842814));
#108178=CARTESIAN_POINT('Ctrl Pts',(-42.0555282974927,1076.68010067045,
529.516961357787));
#108179=CARTESIAN_POINT('Ctrl Pts',(-41.9049993341205,1076.67427558416,
529.622326933881));
#108180=CARTESIAN_POINT('Ctrl Pts',(-41.8689120808022,1076.6732632532,529.644575584759));
#108181=CARTESIAN_POINT('Ctrl Pts',(-41.8079907982816,1076.67215898277,
529.677400659774));
#108182=CARTESIAN_POINT('Ctrl Pts',(-41.7839035379483,1076.67186607917,
529.689254012106));
#108183=CARTESIAN_POINT('Ctrl Pts',(-41.7403344899076,1076.67158708777,
529.708731399799));
#108184=CARTESIAN_POINT('Ctrl Pts',(-41.7210256829323,1076.67154742352,
529.716706077007));
#108185=CARTESIAN_POINT('Ctrl Pts',(-41.6801628030987,1076.67163705262,
529.732224372033));
#108186=CARTESIAN_POINT('Ctrl Pts',(-41.6585774119473,1076.67178233153,
529.739655319584));
#108187=CARTESIAN_POINT('Ctrl Pts',(-41.6020983112158,1076.67241315148,
529.757136396111));
#108188=CARTESIAN_POINT('Ctrl Pts',(-41.5669110503444,1076.67304855044,
529.766130080952));
#108189=CARTESIAN_POINT('Ctrl Pts',(-41.4597866241902,1076.67570131867,
529.787882716096));
#108190=CARTESIAN_POINT('Ctrl Pts',(-41.387082831868,1076.67845698686,529.795163061529));
#108191=CARTESIAN_POINT('Ctrl Pts',(-41.3143294401484,1076.68214102845,
529.795163061529));
#108192=CARTESIAN_POINT('',(-48.0649554680748,1077.56338652908,518.927727241935));
#108193=CARTESIAN_POINT('',(-48.064955468075,1077.76488388158,516.73006496995));
#108194=CARTESIAN_POINT('Ctrl Pts',(-48.0649554680755,1077.56338652908,
518.927727241935));
#108195=CARTESIAN_POINT('Ctrl Pts',(-48.0145010273267,1077.56585180285,
518.927727241935));
#108196=CARTESIAN_POINT('Ctrl Pts',(-47.9640080026722,1077.56864550973,
518.924252272737));
#108197=CARTESIAN_POINT('Ctrl Pts',(-47.796039599905,1077.57903610607,518.900930551175));
#108198=CARTESIAN_POINT('Ctrl Pts',(-47.6817794730932,1077.58792237194,
518.865574638573));
#108199=CARTESIAN_POINT('Ctrl Pts',(-47.4595039067031,1077.60903595514,
518.754983962953));
#108200=CARTESIAN_POINT('Ctrl Pts',(-47.3547210668178,1077.62132914573,
518.677266611072));
#108201=CARTESIAN_POINT('Ctrl Pts',(-47.170326116537,1077.64824277595,518.481934787316));
#108202=CARTESIAN_POINT('Ctrl Pts',(-47.0948596323801,1077.66273265577,
518.363431087428));
#108203=CARTESIAN_POINT('Ctrl Pts',(-46.9898154918473,1077.69187953984,
518.098582349962));
#108204=CARTESIAN_POINT('Ctrl Pts',(-46.9635362291813,1077.7062346296,517.953729404063));
#108205=CARTESIAN_POINT('Ctrl Pts',(-46.9690145884228,1077.73177117505,
517.667251220634));
#108206=CARTESIAN_POINT('Ctrl Pts',(-46.9986857143744,1077.74281759757,
517.528301087755));
#108207=CARTESIAN_POINT('Ctrl Pts',(-47.1056804118959,1077.76027751622,
517.276870741214));
#108208=CARTESIAN_POINT('Ctrl Pts',(-47.1791052670855,1077.76678989412,
517.165374239164));
#108209=CARTESIAN_POINT('Ctrl Pts',(-47.3189758623651,1077.77334205686,
517.019063429134));
#108210=CARTESIAN_POINT('Ctrl Pts',(-47.3719917744344,1077.77497057583,
516.973255993722));
#108211=CARTESIAN_POINT('Ctrl Pts',(-47.4536554849855,1077.776367297,516.915301368854));
#108212=CARTESIAN_POINT('Ctrl Pts',(-47.479010752856,1077.77666610845,516.898835917402));
#108213=CARTESIAN_POINT('Ctrl Pts',(-47.5213219030368,1077.77695163645,
516.873777440269));
#108214=CARTESIAN_POINT('Ctrl Pts',(-47.5378776790546,1077.7770131232,516.864542365627));
#108215=CARTESIAN_POINT('Ctrl Pts',(-47.5729058783718,1077.77703996874,
516.846174719934));
#108216=CARTESIAN_POINT('Ctrl Pts',(-47.5914128481066,1077.77699652695,
516.837124206612));
#108217=CARTESIAN_POINT('Ctrl Pts',(-47.6355330724613,1077.7767592945,516.817064621247));
#108218=CARTESIAN_POINT('Ctrl Pts',(-47.6613318700247,1077.77651793062,
516.806499685223));
#108219=CARTESIAN_POINT('Ctrl Pts',(-47.7452557410909,1077.77540887468,
516.775803766469));
#108220=CARTESIAN_POINT('Ctrl Pts',(-47.8046698637717,1077.7741389845,516.759569074191));
#108221=CARTESIAN_POINT('Ctrl Pts',(-47.9310529949326,1077.77044907064,
516.73619484361));
#108222=CARTESIAN_POINT('Ctrl Pts',(-47.9979446125574,1077.76794311597,
516.73006496995));
#108223=CARTESIAN_POINT('Ctrl Pts',(-48.0649554680748,1077.76488388158,
516.73006496995));
#108224=CARTESIAN_POINT('Ctrl Pts',(-48.0649554680748,1077.76488388158,
516.73006496995));
#108225=CARTESIAN_POINT('Ctrl Pts',(-48.0649598430732,1077.76488368185,
516.73006496995));
#108226=CARTESIAN_POINT('Ctrl Pts',(-48.0649642180723,1077.76488348212,
516.730064969925));
#108227=CARTESIAN_POINT('Ctrl Pts',(-48.0649685930717,1077.76488328238,
516.730064969977));
#108228=CARTESIAN_POINT('Ctrl Pts',(-48.1783489980554,1077.75970702632,
516.730066324253));
#108229=CARTESIAN_POINT('Ctrl Pts',(-48.2909640961249,1077.75299756761,
516.747615160064));
#108230=CARTESIAN_POINT('Ctrl Pts',(-48.518206698586,1077.73608207952,516.820088184502));
#108231=CARTESIAN_POINT('Ctrl Pts',(-48.630094046204,1077.72570265682,516.878265831029));
#108232=CARTESIAN_POINT('Ctrl Pts',(-48.8375422331832,1077.70184037015,
517.035875863945));
#108233=CARTESIAN_POINT('Ctrl Pts',(-48.9292511454738,1077.68837061489,
517.13699504206));
#108234=CARTESIAN_POINT('Ctrl Pts',(-49.076806488182,1077.65953151255,517.376286722553));
#108235=CARTESIAN_POINT('Ctrl Pts',(-49.1278911292269,1077.64437086784,
517.51444485906));
#108236=CARTESIAN_POINT('Ctrl Pts',(-49.1727820385911,1077.61567177391,
517.80054201422));
#108237=CARTESIAN_POINT('Ctrl Pts',(-49.1670092371341,1077.60238215247,
517.945636395291));
#108238=CARTESIAN_POINT('Ctrl Pts',(-49.1030894837639,1077.58048233853,
518.211675364131));
#108239=CARTESIAN_POINT('Ctrl Pts',(-49.0506933432679,1077.57171147817,
518.331513012622));
#108240=CARTESIAN_POINT('Ctrl Pts',(-48.9137484537884,1077.5589952769,518.536400788778));
#108241=CARTESIAN_POINT('Ctrl Pts',(-48.8339457995117,1077.55472998722,
518.622430126506));
#108242=CARTESIAN_POINT('Ctrl Pts',(-48.7118559167702,1077.55163430139,
518.717951772243));
#108243=CARTESIAN_POINT('Ctrl Pts',(-48.6804376729709,1077.55107969025,
518.739984630358));
#108244=CARTESIAN_POINT('Ctrl Pts',(-48.628410105786,1077.55053427899,518.772548047195));
#108245=CARTESIAN_POINT('Ctrl Pts',(-48.608511334067,1077.55040688114,518.784148521431));
#108246=CARTESIAN_POINT('Ctrl Pts',(-48.5721331343716,1077.55031714445,
518.803851051258));
#108247=CARTESIAN_POINT('Ctrl Pts',(-48.5557876574196,1077.55032651165,
518.812181462383));
#108248=CARTESIAN_POINT('Ctrl Pts',(-48.5172563691362,1077.55046276701,
518.830618504336));
#108249=CARTESIAN_POINT('Ctrl Pts',(-48.4949280004348,1077.55062723332,
518.840403612521));
#108250=CARTESIAN_POINT('Ctrl Pts',(-48.431225361482,1077.55133326594,518.865829806309));
#108251=CARTESIAN_POINT('Ctrl Pts',(-48.3892097524541,1077.55207220881,
518.879726004704));
#108252=CARTESIAN_POINT('Ctrl Pts',(-48.2543653682687,1077.55528433236,
518.915466015449));
#108253=CARTESIAN_POINT('Ctrl Pts',(-48.1597284755232,1077.55875578884,
518.927727241935));
#108254=CARTESIAN_POINT('Ctrl Pts',(-48.0649554680755,1077.56338652908,
518.927727241935));
#108255=CARTESIAN_POINT('',(-52.5439991194435,1078.27787179661,507.113735502178));
#108256=CARTESIAN_POINT('',(-52.5439991194437,1078.41491649088,504.562847259905));
#108257=CARTESIAN_POINT('Ctrl Pts',(-52.5439991194441,1078.27787179661,
507.113735502178));
#108258=CARTESIAN_POINT('Ctrl Pts',(-52.4986442771421,1078.27956269921,
507.113735502178));
#108259=CARTESIAN_POINT('Ctrl Pts',(-52.4532386218892,1078.28139109926,
507.111316334615));
#108260=CARTESIAN_POINT('Ctrl Pts',(-52.2679433665825,1078.28940503941,
507.091441651501));
#108261=CARTESIAN_POINT('Ctrl Pts',(-52.1314099928142,1078.29660548746,
507.05333718123));
#108262=CARTESIAN_POINT('Ctrl Pts',(-51.8658116666798,1078.31324672697,
506.929188792383));
#108263=CARTESIAN_POINT('Ctrl Pts',(-51.7404285211826,1078.32268861784,
506.840414518152));
#108264=CARTESIAN_POINT('Ctrl Pts',(-51.5191679411933,1078.34285032232,
506.614960460239));
#108265=CARTESIAN_POINT('Ctrl Pts',(-51.4281340532332,1078.35342681473,
506.477310289254));
#108266=CARTESIAN_POINT('Ctrl Pts',(-51.3012013249814,1078.37398778512,
506.170747028407));
#108267=CARTESIAN_POINT('Ctrl Pts',(-51.2682084167509,1078.38374779276,
506.004016022769));
#108268=CARTESIAN_POINT('Ctrl Pts',(-51.2688907632724,1078.40054457389,
505.675133975294));
#108269=CARTESIAN_POINT('Ctrl Pts',(-51.2995208059245,1078.40754151525,
505.516063695471));
#108270=CARTESIAN_POINT('Ctrl Pts',(-51.4200773886815,1078.41875122293,
505.213029763869));
#108271=CARTESIAN_POINT('Ctrl Pts',(-51.5106296082965,1078.42276998262,
505.072572155123));
#108272=CARTESIAN_POINT('Ctrl Pts',(-51.6633428479768,1078.4256964583,504.914076643506));
#108273=CARTESIAN_POINT('Ctrl Pts',(-51.7036385084434,1078.426220819,504.87729043587));
#108274=CARTESIAN_POINT('Ctrl Pts',(-51.7685152953052,1078.4267121243,504.825274505618));
#108275=CARTESIAN_POINT('Ctrl Pts',(-51.7914630822053,1078.42682534233,
504.808112808865));
#108276=CARTESIAN_POINT('Ctrl Pts',(-51.8339693610143,1078.42692852969,
504.778502901022));
#108277=CARTESIAN_POINT('Ctrl Pts',(-51.85332625225,1078.426937945,504.765787361048));
#108278=CARTESIAN_POINT('Ctrl Pts',(-51.8953202222838,1078.42687972818,
504.739810120037));
#108279=CARTESIAN_POINT('Ctrl Pts',(-51.9180419639268,1078.42680173631,
504.726705568707));
#108280=CARTESIAN_POINT('Ctrl Pts',(-51.9797576465656,1078.42646791388,
504.69360431753));
#108281=CARTESIAN_POINT('Ctrl Pts',(-52.01940431159,1078.42612814473,504.674901065275));
#108282=CARTESIAN_POINT('Ctrl Pts',(-52.1980810234138,1078.42405657482,
504.601604395505));
#108283=CARTESIAN_POINT('Ctrl Pts',(-52.3450857331372,1078.4209624869,504.569642288513));
#108284=CARTESIAN_POINT('Ctrl Pts',(-52.5108155057554,1078.41596659625,
504.563171036046));
#108285=CARTESIAN_POINT('Ctrl Pts',(-52.5274067847652,1078.4154498872,504.562847259905));
#108286=CARTESIAN_POINT('Ctrl Pts',(-52.5439991194437,1078.41491649088,
504.562847259905));
#108287=CARTESIAN_POINT('Ctrl Pts',(-52.5439991194437,1078.41491649088,
504.562847259905));
#108288=CARTESIAN_POINT('Ctrl Pts',(-52.544008079654,1078.41491620283,504.562847259905));
#108289=CARTESIAN_POINT('Ctrl Pts',(-52.5440170398646,1078.41491591478,
504.56284726));
#108290=CARTESIAN_POINT('Ctrl Pts',(-52.5440260000755,1078.41491562673,
504.562847260189));
#108291=CARTESIAN_POINT('Ctrl Pts',(-52.6807106207702,1078.41052145713,
504.562850140886));
#108292=CARTESIAN_POINT('Ctrl Pts',(-52.8164686631165,1078.40502727986,
504.584824495826));
#108293=CARTESIAN_POINT('Ctrl Pts',(-53.0878585470118,1078.39154213021,
504.674983409868));
#108294=CARTESIAN_POINT('Ctrl Pts',(-53.220195364015,1078.3834675677,504.74659532574));
#108295=CARTESIAN_POINT('Ctrl Pts',(-53.4629705438839,1078.36519532637,
504.939358940828));
#108296=CARTESIAN_POINT('Ctrl Pts',(-53.5688001439053,1078.35504191809,
505.062176281989));
#108297=CARTESIAN_POINT('Ctrl Pts',(-53.7333772667468,1078.33387359429,
505.347714228365));
#108298=CARTESIAN_POINT('Ctrl Pts',(-53.7878303959066,1078.32304757444,
505.509377161157));
#108299=CARTESIAN_POINT('Ctrl Pts',(-53.829975549002,1078.30309169221,505.839904830851));
#108300=CARTESIAN_POINT('Ctrl Pts',(-53.8190890232239,1078.29411126856,
506.005390567118));
#108301=CARTESIAN_POINT('Ctrl Pts',(-53.7391564514496,1078.27978192806,
506.307719020495));
#108302=CARTESIAN_POINT('Ctrl Pts',(-53.6764949059545,1078.2742763811,506.443474578826));
#108303=CARTESIAN_POINT('Ctrl Pts',(-53.5356430599943,1078.26778775998,
506.646453133765));
#108304=CARTESIAN_POINT('Ctrl Pts',(-53.470205072877,1078.26592891012,506.720692161054));
#108305=CARTESIAN_POINT('Ctrl Pts',(-53.3684007172843,1078.26443147481,
506.812244325751));
#108306=CARTESIAN_POINT('Ctrl Pts',(-53.3388064915731,1078.26413099571,
506.836541709559));
#108307=CARTESIAN_POINT('Ctrl Pts',(-53.2880420463172,1078.26383082245,
506.874529502126));
#108308=CARTESIAN_POINT('Ctrl Pts',(-53.2674794631115,1078.26376334058,
506.88898901963));
#108309=CARTESIAN_POINT('Ctrl Pts',(-53.2266443211653,1078.2637324558,506.915936658567));
#108310=CARTESIAN_POINT('Ctrl Pts',(-53.2064228488732,1078.26376370447,
506.928483388593));
#108311=CARTESIAN_POINT('Ctrl Pts',(-53.1584150395403,1078.26394458987,
506.956441477233));
#108312=CARTESIAN_POINT('Ctrl Pts',(-53.1303806368008,1078.26413031448,
506.971394737863));
#108313=CARTESIAN_POINT('Ctrl Pts',(-53.0401906655634,1078.26497503102,
507.015256899258));
#108314=CARTESIAN_POINT('Ctrl Pts',(-52.9762529287781,1078.26593173545,
507.040210314352));
#108315=CARTESIAN_POINT('Ctrl Pts',(-52.7914285797817,1078.2696604641,507.095679226291));
#108316=CARTESIAN_POINT('Ctrl Pts',(-52.667903440952,1078.27325244113,507.113735502178));
#108317=CARTESIAN_POINT('Ctrl Pts',(-52.5439991194441,1078.27787179661,
507.113735502178));
#108318=CARTESIAN_POINT('',(-55.8158882427213,1078.63997504936,496.136128111847));
#108319=CARTESIAN_POINT('',(-55.8158882427217,1078.69949549139,493.17952184746));
#108320=CARTESIAN_POINT('Ctrl Pts',(-55.8158882427213,1078.63997504936,
496.136128111847));
#108321=CARTESIAN_POINT('Ctrl Pts',(-55.7381761621697,1078.64151398949,
496.136128111847));
#108322=CARTESIAN_POINT('Ctrl Pts',(-55.6604683092864,1078.64318748345,
496.130000302946));
#108323=CARTESIAN_POINT('Ctrl Pts',(-55.416052423721,1078.64884766251,496.091093319474));
#108324=CARTESIAN_POINT('Ctrl Pts',(-55.2544465367711,1078.65318431832,
496.035832602985));
#108325=CARTESIAN_POINT('Ctrl Pts',(-54.94601132426,1078.66252338863,495.866901885036));
#108326=CARTESIAN_POINT('Ctrl Pts',(-54.803802738849,1078.66746722632,495.750636405023));
#108327=CARTESIAN_POINT('Ctrl Pts',(-54.5601086818315,1078.67729340092,
495.461982382799));
#108328=CARTESIAN_POINT('Ctrl Pts',(-54.4648213922992,1078.68204475838,
495.288917633588));
#108329=CARTESIAN_POINT('Ctrl Pts',(-54.3480562560232,1078.69035884261,
494.918549985383));
#108330=CARTESIAN_POINT('Ctrl Pts',(-54.3266007807071,1078.69386378003,
494.725202486329));
#108331=CARTESIAN_POINT('Ctrl Pts',(-54.3571894053235,1078.69920699931,
494.363710454937));
#108332=CARTESIAN_POINT('Ctrl Pts',(-54.4006686152582,1078.70115814677,
494.197973752867));
#108333=CARTESIAN_POINT('Ctrl Pts',(-54.5313053539874,1078.70379577326,
493.912164267285));
#108334=CARTESIAN_POINT('Ctrl Pts',(-54.6100947628516,1078.70461690227,
493.790515106427));
#108335=CARTESIAN_POINT('Ctrl Pts',(-54.7374721507079,1078.705221843,493.645508700875));
#108336=CARTESIAN_POINT('Ctrl Pts',(-54.7715034960503,1078.70533186944,
493.610434872485));
#108337=CARTESIAN_POINT('Ctrl Pts',(-54.8289920197998,1078.70544028254,
493.556778248848));
#108338=CARTESIAN_POINT('Ctrl Pts',(-54.8513854833553,1078.70546543502,
493.537109811828));
#108339=CARTESIAN_POINT('Ctrl Pts',(-54.8949247678817,1078.70548297794,
493.501140880741));
#108340=CARTESIAN_POINT('Ctrl Pts',(-54.9159476721064,1078.70547851921,
493.484709982686));
#108341=CARTESIAN_POINT('Ctrl Pts',(-54.9643394375763,1078.70543970664,
493.448955091846));
#108342=CARTESIAN_POINT('Ctrl Pts',(-54.9919437658391,1078.70539802359,
493.429974309028));
#108343=CARTESIAN_POINT('Ctrl Pts',(-55.0751380384177,1078.70521578472,
493.376839631339));
#108344=CARTESIAN_POINT('Ctrl Pts',(-55.132370378762,1078.70501927599,493.345408277861));
#108345=CARTESIAN_POINT('Ctrl Pts',(-55.2658228272856,1078.70440139534,
493.283222039045));
#108346=CARTESIAN_POINT('Ctrl Pts',(-55.3429080832118,1078.70393632846,
493.254830058092));
#108347=CARTESIAN_POINT('Ctrl Pts',(-55.5502578875137,1078.7023895069,493.197502204148));
#108348=CARTESIAN_POINT('Ctrl Pts',(-55.6827707839958,1078.70111160033,
493.17952184746));
#108349=CARTESIAN_POINT('Ctrl Pts',(-55.8158882427217,1078.69949549139,
493.17952184746));
#108350=CARTESIAN_POINT('Ctrl Pts',(-55.8158882427217,1078.69949549139,
493.17952184746));
#108351=CARTESIAN_POINT('Ctrl Pts',(-55.8159000830156,1078.69949534765,
493.17952184746));
#108352=CARTESIAN_POINT('Ctrl Pts',(-55.8159119233143,1078.6994952039,493.179521847602));
#108353=CARTESIAN_POINT('Ctrl Pts',(-55.8159237636178,1078.69949506015,
493.179521847887));
#108354=CARTESIAN_POINT('Ctrl Pts',(-55.9794669437012,1078.697509496,493.179525777528));
#108355=CARTESIAN_POINT('Ctrl Pts',(-56.1418739339458,1078.69503594291,
493.206668486392));
#108356=CARTESIAN_POINT('Ctrl Pts',(-56.4642283140259,1078.68885330115,
493.317494273381));
#108357=CARTESIAN_POINT('Ctrl Pts',(-56.620191844934,1078.68510311682,493.404860507457));
#108358=CARTESIAN_POINT('Ctrl Pts',(-56.9038669012547,1078.67640524987,
493.639014332784));
#108359=CARTESIAN_POINT('Ctrl Pts',(-57.0259632007142,1078.67146741882,
493.787545880715));
#108360=CARTESIAN_POINT('Ctrl Pts',(-57.2090528540562,1078.66116333372,
494.126432935689));
#108361=CARTESIAN_POINT('Ctrl Pts',(-57.2668540772811,1078.65589337403,
494.314333985789));
#108362=CARTESIAN_POINT('Ctrl Pts',(-57.3053909479616,1078.64630679125,
494.692693485502));
#108363=CARTESIAN_POINT('Ctrl Pts',(-57.2892537050925,1078.64204836896,
494.879269873133));
#108364=CARTESIAN_POINT('Ctrl Pts',(-57.1873539376165,1078.63501285798,
495.241664465276));
#108365=CARTESIAN_POINT('Ctrl Pts',(-57.1006254796562,1078.63235236716,
495.413633894357));
#108366=CARTESIAN_POINT('Ctrl Pts',(-56.9434526347171,1078.63034957464,
495.61608640209));
#108367=CARTESIAN_POINT('Ctrl Pts',(-56.8999128617944,1078.62997713082,
495.665077305353));
#108368=CARTESIAN_POINT('Ctrl Pts',(-56.8291832737198,1078.62963033988,
495.734744787117));
#108369=CARTESIAN_POINT('Ctrl Pts',(-56.8042908779995,1078.62955065203,
495.757635570108));
#108370=CARTESIAN_POINT('Ctrl Pts',(-56.7581163548514,1078.6294768266,495.797262327063));
#108371=CARTESIAN_POINT('Ctrl Pts',(-56.7371178441088,1078.62946876772,
495.814305548708));
#108372=CARTESIAN_POINT('Ctrl Pts',(-56.6915994559401,1078.62950421266,
495.849223269005));
#108373=CARTESIAN_POINT('Ctrl Pts',(-56.6669728114318,1078.62955410197,
495.866938317575));
#108374=CARTESIAN_POINT('Ctrl Pts',(-56.6003281284012,1078.62976846143,
495.911833311335));
#108375=CARTESIAN_POINT('Ctrl Pts',(-56.5574457528482,1078.6299861943,495.937659038498));
#108376=CARTESIAN_POINT('Ctrl Pts',(-56.3671092090801,1078.63128264162,
496.039505266986));
#108377=CARTESIAN_POINT('Ctrl Pts',(-56.2087602522833,1078.63318248535,
496.092583017586));
#108378=CARTESIAN_POINT('Ctrl Pts',(-55.9690462876418,1078.63707281428,
496.130178026875));
#108379=CARTESIAN_POINT('Ctrl Pts',(-55.8924652122921,1078.63845858794,
496.136128111847));
#108380=CARTESIAN_POINT('Ctrl Pts',(-55.8158882427213,1078.63997504936,
496.136128111847));
#108381=CARTESIAN_POINT('',(-40.0345449899137,1078.63462185218,506.210414596646));
#108382=CARTESIAN_POINT('',(-40.034544989914,1078.7026568498,503.25380833226));
#108383=CARTESIAN_POINT('Ctrl Pts',(-40.0345449899137,1078.63462185218,
506.210414596647));
#108384=CARTESIAN_POINT('Ctrl Pts',(-39.933258250339,1078.63609822354,506.210414596647));
#108385=CARTESIAN_POINT('Ctrl Pts',(-39.831992934802,1078.63786301688,506.200004964856));
#108386=CARTESIAN_POINT('Ctrl Pts',(-39.5729316752126,1078.64308303955,
506.145908031524));
#108387=CARTESIAN_POINT('Ctrl Pts',(-39.4201008036855,1078.64686749493,
506.08649678629));
#108388=CARTESIAN_POINT('Ctrl Pts',(-39.1286730549577,1078.65540843741,
505.913536323377));
#108389=CARTESIAN_POINT('Ctrl Pts',(-38.9945519874464,1078.66014658622,
505.797372361076));
#108390=CARTESIAN_POINT('Ctrl Pts',(-38.765611758857,1078.66992924473,505.513614639003));
#108391=CARTESIAN_POINT('Ctrl Pts',(-38.6763669008811,1078.67487807669,
505.34554104547));
#108392=CARTESIAN_POINT('Ctrl Pts',(-38.5639735921682,1078.68414476881,
504.978762411192));
#108393=CARTESIAN_POINT('Ctrl Pts',(-38.5442911297931,1078.68834555087,
504.782802219003));
#108394=CARTESIAN_POINT('Ctrl Pts',(-38.5813873444244,1078.69532057629,
504.402296862145));
#108395=CARTESIAN_POINT('Ctrl Pts',(-38.634805018151,1078.69808856571,504.22105406683));
#108396=CARTESIAN_POINT('Ctrl Pts',(-38.8090985689076,1078.70241361652,
503.883040137149));
#108397=CARTESIAN_POINT('Ctrl Pts',(-38.9303202102076,1078.70389690259,
503.730446529508));
#108398=CARTESIAN_POINT('Ctrl Pts',(-39.1226275039791,1078.70497374679,
503.567078410624));
#108399=CARTESIAN_POINT('Ctrl Pts',(-39.1700827343216,1078.70516294172,
503.531444743352));
#108400=CARTESIAN_POINT('Ctrl Pts',(-39.2513682316366,1078.70537039634,
503.477731603099));
#108401=CARTESIAN_POINT('Ctrl Pts',(-39.2839888419741,1078.70542545713,
503.457945012923));
#108402=CARTESIAN_POINT('Ctrl Pts',(-39.3435670224156,1078.70547731193,
503.424889471978));
#108403=CARTESIAN_POINT('Ctrl Pts',(-39.3702329000793,1078.70548401992,
503.4111385892));
#108404=CARTESIAN_POINT('Ctrl Pts',(-39.4271171972576,1078.70546425462,
503.383963214299));
#108405=CARTESIAN_POINT('Ctrl Pts',(-39.4574050806584,1078.70543434434,
503.37072182486));
#108406=CARTESIAN_POINT('Ctrl Pts',(-39.5373714213134,1078.70530541979,
503.338910410266));
#108407=CARTESIAN_POINT('Ctrl Pts',(-39.5876500715567,1078.70517570366,
503.321978264619));
#108408=CARTESIAN_POINT('Ctrl Pts',(-39.7676132958365,1078.70453972674,
503.271967097767));
#108409=CARTESIAN_POINT('Ctrl Pts',(-39.900762934436,1078.70376561848,503.253809917498));
#108410=CARTESIAN_POINT('Ctrl Pts',(-40.0345274717492,1078.70265699499,
503.253808332364));
#108411=CARTESIAN_POINT('Ctrl Pts',(-40.0345333111388,1078.70265694659,
503.253808332295));
#108412=CARTESIAN_POINT('Ctrl Pts',(-40.0345391505271,1078.7026568982,503.25380833226));
#108413=CARTESIAN_POINT('Ctrl Pts',(-40.034544989914,1078.7026568498,503.25380833226));
#108414=CARTESIAN_POINT('Ctrl Pts',(-40.034544989914,1078.7026568498,503.25380833226));
#108415=CARTESIAN_POINT('Ctrl Pts',(-40.1870861698988,1078.70139257487,
503.25380833226));
#108416=CARTESIAN_POINT('Ctrl Pts',(-40.3387075824845,1078.69970632408,
503.277418627439));
#108417=CARTESIAN_POINT('Ctrl Pts',(-40.644307575697,1078.69522353048,503.374952849358));
#108418=CARTESIAN_POINT('Ctrl Pts',(-40.7946844730414,1078.69235962397,
503.453099222605));
#108419=CARTESIAN_POINT('Ctrl Pts',(-41.0731515358608,1078.68537363958,
503.664592747099));
#108420=CARTESIAN_POINT('Ctrl Pts',(-41.1962022846745,1078.68122526846,
503.799992955703));
#108421=CARTESIAN_POINT('Ctrl Pts',(-41.3942613937534,1078.67182122879,
504.120086316256));
#108422=CARTESIAN_POINT('Ctrl Pts',(-41.4630451756302,1078.66659606366,
504.304575468052));
#108423=CARTESIAN_POINT('Ctrl Pts',(-41.5247800067169,1078.65617525521,
504.687939704521));
#108424=CARTESIAN_POINT('Ctrl Pts',(-41.5177819598931,1078.65108481618,
504.882993551684));
#108425=CARTESIAN_POINT('Ctrl Pts',(-41.4327461327301,1078.6423370141,505.243866559487));
#108426=CARTESIAN_POINT('Ctrl Pts',(-41.3612897767765,1078.63867254317,
505.407845986762));
#108427=CARTESIAN_POINT('Ctrl Pts',(-41.1751706699865,1078.63331759805,
505.685496222142));
#108428=CARTESIAN_POINT('Ctrl Pts',(-41.0676822154739,1078.63148297625,
505.801037120108));
#108429=CARTESIAN_POINT('Ctrl Pts',(-40.9008382405138,1078.63009065515,
505.931244722696));
#108430=CARTESIAN_POINT('Ctrl Pts',(-40.8557846356255,1078.62982884185,
505.962538266879));
#108431=CARTESIAN_POINT('Ctrl Pts',(-40.7803490443768,1078.62956909803,
506.008941776923));
#108432=CARTESIAN_POINT('Ctrl Pts',(-40.7510036608353,1078.62950848841,
506.025636229184));
#108433=CARTESIAN_POINT('Ctrl Pts',(-40.6942131746564,1078.62946662967,
506.05541815989));
#108434=CARTESIAN_POINT('Ctrl Pts',(-40.6668853893315,1078.62947805342,
506.068692304597));
#108435=CARTESIAN_POINT('Ctrl Pts',(-40.6042329065985,1078.62957444609,
506.096773133909));
#108436=CARTESIAN_POINT('Ctrl Pts',(-40.56870272132,1078.629677762,506.111068060059));
#108437=CARTESIAN_POINT('Ctrl Pts',(-40.4622717437087,1078.63012789064,
506.149157232906));
#108438=CARTESIAN_POINT('Ctrl Pts',(-40.3900772345219,1078.63061242184,
506.168971012288));
#108439=CARTESIAN_POINT('Ctrl Pts',(-40.2235011822194,1078.63211880381,
506.201359340723));
#108440=CARTESIAN_POINT('Ctrl Pts',(-40.1290137673779,1078.6332448605,506.210414596647));
#108441=CARTESIAN_POINT('Ctrl Pts',(-40.0345449899137,1078.63462185218,
506.210414596647));
#108442=CARTESIAN_POINT('',(-34.5096048204685,1078.26956110846,516.263437971404));
#108443=CARTESIAN_POINT('',(-34.5096048204688,1078.42202250585,513.712549729131));
#108444=CARTESIAN_POINT('Ctrl Pts',(-34.5096048204687,1078.26956110846,
516.263437971403));
#108445=CARTESIAN_POINT('Ctrl Pts',(-34.3781595851867,1078.27280332059,
516.263437971403));
#108446=CARTESIAN_POINT('Ctrl Pts',(-34.2473014668533,1078.27733135701,
516.243116621277));
#108447=CARTESIAN_POINT('Ctrl Pts',(-33.9875836940846,1078.28895388381,
516.160204287482));
#108448=CARTESIAN_POINT('Ctrl Pts',(-33.8615086191089,1078.29610910236,
516.095481226303));
#108449=CARTESIAN_POINT('Ctrl Pts',(-33.6263664264477,1078.31267233544,
515.920648540955));
#108450=CARTESIAN_POINT('Ctrl Pts',(-33.5214294590781,1078.322082882,515.808630798506));
#108451=CARTESIAN_POINT('Ctrl Pts',(-33.3500319054978,1078.34220282634,
515.543703624841));
#108452=CARTESIAN_POINT('Ctrl Pts',(-33.2884764078526,1078.35277147479,
515.390825895484));
#108453=CARTESIAN_POINT('Ctrl Pts',(-33.2254191302722,1078.37336835185,
515.065221580362));
#108454=CARTESIAN_POINT('Ctrl Pts',(-33.226437950399,1078.38317090214,514.895188092461));
#108455=CARTESIAN_POINT('Ctrl Pts',(-33.2930447262667,1078.40010065184,
514.572420400151));
#108456=CARTESIAN_POINT('Ctrl Pts',(-33.3552301369026,1078.4071775404,514.422154131845));
#108457=CARTESIAN_POINT('Ctrl Pts',(-33.5370928998336,1078.41866703871,
514.145480475725));
#108458=CARTESIAN_POINT('Ctrl Pts',(-33.657834487675,1078.42280636536,514.023564507335));
#108459=CARTESIAN_POINT('Ctrl Pts',(-33.842737444783,1078.42572190575,513.899496597316));
#108460=CARTESIAN_POINT('Ctrl Pts',(-33.8883070778172,1078.42622474724,
513.872858046193));
#108461=CARTESIAN_POINT('Ctrl Pts',(-33.9629561338825,1078.42672167601,
513.835220862287));
#108462=CARTESIAN_POINT('Ctrl Pts',(-33.9910117688328,1078.42684008775,
513.822330250798));
#108463=CARTESIAN_POINT('Ctrl Pts',(-34.0413321025789,1078.42693406492,
513.801386421076));
#108464=CARTESIAN_POINT('Ctrl Pts',(-34.0634049962602,1078.42693656199,
513.792911322874));
#108465=CARTESIAN_POINT('Ctrl Pts',(-34.1142066783052,1078.4268550657,513.775009300899));
#108466=CARTESIAN_POINT('Ctrl Pts',(-34.1430605880461,1078.42674681602,
513.765980549334));
#108467=CARTESIAN_POINT('Ctrl Pts',(-34.2217440415278,1078.42628615213,
513.744397306075));
#108468=CARTESIAN_POINT('Ctrl Pts',(-34.2720545294198,1078.42581637524,
513.733814548442));
#108469=CARTESIAN_POINT('Ctrl Pts',(-34.3846943410285,1078.42437988848,
513.717143026564));
#108470=CARTESIAN_POINT('Ctrl Pts',(-34.4471095633331,1078.42332948689,
513.712549729131));
#108471=CARTESIAN_POINT('Ctrl Pts',(-34.5096048204688,1078.42202250585,
513.712549729131));
#108472=CARTESIAN_POINT('Ctrl Pts',(-34.5096048204688,1078.42202250585,
513.712549729131));
#108473=CARTESIAN_POINT('Ctrl Pts',(-34.5096083249495,1078.42202243256,
513.712549729131));
#108474=CARTESIAN_POINT('Ctrl Pts',(-34.5096118294305,1078.42202235927,
513.712549729145));
#108475=CARTESIAN_POINT('Ctrl Pts',(-34.5096153339117,1078.42202228598,
513.712549729174));
#108476=CARTESIAN_POINT('Ctrl Pts',(-34.6788906624206,1078.41848210556,
513.712551124505));
#108477=CARTESIAN_POINT('Ctrl Pts',(-34.8464290549155,1078.41311075097,
513.746250451062));
#108478=CARTESIAN_POINT('Ctrl Pts',(-35.1359553121413,1078.40014343692,
513.867551311148));
#108479=CARTESIAN_POINT('Ctrl Pts',(-35.2589159630341,1078.39307230121,
513.945778393466));
#108480=CARTESIAN_POINT('Ctrl Pts',(-35.4818547242167,1078.37658781807,
514.14781922937));
#108481=CARTESIAN_POINT('Ctrl Pts',(-35.5773306722079,1078.36716819326,
514.273080049463));
#108482=CARTESIAN_POINT('Ctrl Pts',(-35.7235800354469,1078.34671685574,
514.562289401582));
#108483=CARTESIAN_POINT('Ctrl Pts',(-35.7690251798978,1078.33581292178,
514.72565620032));
#108484=CARTESIAN_POINT('Ctrl Pts',(-35.7939442369292,1078.31474727396,
515.059759364467));
#108485=CARTESIAN_POINT('Ctrl Pts',(-35.7735106256755,1078.30478586434,
515.227268355529));
#108486=CARTESIAN_POINT('Ctrl Pts',(-35.6732220271771,1078.2879504767,515.532513944678));
#108487=CARTESIAN_POINT('Ctrl Pts',(-35.5989618694391,1078.28103729642,
515.669054685904));
#108488=CARTESIAN_POINT('Ctrl Pts',(-35.4155787819824,1078.27094006414,
515.896258729525));
#108489=CARTESIAN_POINT('Ctrl Pts',(-35.3122410260585,1078.26750497277,
515.98875731029));
#108490=CARTESIAN_POINT('Ctrl Pts',(-35.1553933362622,1078.26489491808,
516.088923488741));
#108491=CARTESIAN_POINT('Ctrl Pts',(-35.1132567881329,1078.2644040275,516.112579795059));
#108492=CARTESIAN_POINT('Ctrl Pts',(-35.0431913200874,1078.26391702542,
516.146840553654));
#108493=CARTESIAN_POINT('Ctrl Pts',(-35.0160556257707,1078.26380335526,
516.158954075922));
#108494=CARTESIAN_POINT('Ctrl Pts',(-34.9637699410496,1078.26372442065,
516.180136855707));
#108495=CARTESIAN_POINT('Ctrl Pts',(-34.9387095644595,1078.26374533838,
516.189384717918));
#108496=CARTESIAN_POINT('Ctrl Pts',(-34.8814984340421,1078.26392412015,
516.208478307941));
#108497=CARTESIAN_POINT('Ctrl Pts',(-34.849211869092,1078.26411591235,516.217853254797));
#108498=CARTESIAN_POINT('Ctrl Pts',(-34.753114777645,1078.26495074676,516.241683577449));
#108499=CARTESIAN_POINT('Ctrl Pts',(-34.688523965642,1078.26584788725,516.252518175395));
#108500=CARTESIAN_POINT('Ctrl Pts',(-34.5854895384334,1078.26779742569,
516.261747118207));
#108501=CARTESIAN_POINT('Ctrl Pts',(-34.5475227526251,1078.26862582937,
516.263437971403));
#108502=CARTESIAN_POINT('Ctrl Pts',(-34.5096048204687,1078.26956110846,
516.263437971403));
#108503=CARTESIAN_POINT('',(-27.6354521170187,1077.55448697719,526.884160690467));
#108504=CARTESIAN_POINT('',(-27.6354521170191,1077.7731748795,524.686498418482));
#108505=CARTESIAN_POINT('Ctrl Pts',(-27.6354521170187,1077.55448697719,
526.884160690467));
#108506=CARTESIAN_POINT('Ctrl Pts',(-27.4944194254515,1077.55845967166,
526.884160690467));
#108507=CARTESIAN_POINT('Ctrl Pts',(-27.3547655994155,1077.5651885524,526.857010205863));
#108508=CARTESIAN_POINT('Ctrl Pts',(-27.1123084716077,1077.58201060038,
526.759129373448));
#108509=CARTESIAN_POINT('Ctrl Pts',(-27.0087974110687,1077.59135802978,
526.695944893038));
#108510=CARTESIAN_POINT('Ctrl Pts',(-26.8186154364285,1077.61331290848,
526.531868835868));
#108511=CARTESIAN_POINT('Ctrl Pts',(-26.7356817152725,1077.62595899111,
526.429467635875));
#108512=CARTESIAN_POINT('Ctrl Pts',(-26.6049852710548,1077.65340079863,
526.191905641563));
#108513=CARTESIAN_POINT('Ctrl Pts',(-26.5614978708921,1077.66804164051,
526.056967889487));
#108514=CARTESIAN_POINT('Ctrl Pts',(-26.5271042387479,1077.69706818465,
525.773116606164));
#108515=CARTESIAN_POINT('Ctrl Pts',(-26.5384377884101,1077.71115024743,
525.626583722595));
#108516=CARTESIAN_POINT('Ctrl Pts',(-26.6160007339918,1077.73585153354,
525.352188612712));
#108517=CARTESIAN_POINT('Ctrl Pts',(-26.6792045143013,1077.74637215479,
525.226263733483));
#108518=CARTESIAN_POINT('Ctrl Pts',(-26.8506200369833,1077.76335471662,
525.003364520485));
#108519=CARTESIAN_POINT('Ctrl Pts',(-26.9577338924268,1077.76960835039,
524.908867437982));
#108520=CARTESIAN_POINT('Ctrl Pts',(-27.126159928436,1077.77465432355,524.810176943307));
#108521=CARTESIAN_POINT('Ctrl Pts',(-27.1743180298784,1077.77566097145,
524.786501222173));
#108522=CARTESIAN_POINT('Ctrl Pts',(-27.2505560510525,1077.7766137893,524.755716031541));
#108523=CARTESIAN_POINT('Ctrl Pts',(-27.277503781822,1077.77683515238,524.746040336496));
#108524=CARTESIAN_POINT('Ctrl Pts',(-27.3270077544142,1077.77703575551,
524.730419954695));
#108525=CARTESIAN_POINT('Ctrl Pts',(-27.3494334710484,1077.77705237691,
524.724120088884));
#108526=CARTESIAN_POINT('Ctrl Pts',(-27.3977437097661,1077.77693106318,
524.712191442753));
#108527=CARTESIAN_POINT('Ctrl Pts',(-27.4236654094531,1077.77677172016,
524.706776344388));
#108528=CARTESIAN_POINT('Ctrl Pts',(-27.4933862554123,1077.77609332008,
524.694822034415));
#108529=CARTESIAN_POINT('Ctrl Pts',(-27.5374240335677,1077.77540513217,
524.6899852492));
#108530=CARTESIAN_POINT('Ctrl Pts',(-27.5995589824073,1077.77407182594,
524.686938093064));
#108531=CARTESIAN_POINT('Ctrl Pts',(-27.6175026981217,1077.77364454734,
524.686498418482));
#108532=CARTESIAN_POINT('Ctrl Pts',(-27.6354521170191,1077.7731748795,524.686498418482));
#108533=CARTESIAN_POINT('Ctrl Pts',(-27.6354561400331,1077.77317477423,
524.686498418489));
#108534=CARTESIAN_POINT('Ctrl Pts',(-27.7820956642943,1077.76933772555,
524.686498955362));
#108535=CARTESIAN_POINT('Ctrl Pts',(-27.9271441422489,1077.76272533786,
524.715850776585));
#108536=CARTESIAN_POINT('Ctrl Pts',(-28.1739877151007,1077.7461839246,524.81984742957));
#108537=CARTESIAN_POINT('Ctrl Pts',(-28.2772144729253,1077.73712729329,
524.885179807013));
#108538=CARTESIAN_POINT('Ctrl Pts',(-28.465932537063,1077.71567113954,525.053813521592));
#108539=CARTESIAN_POINT('Ctrl Pts',(-28.54756760258,1077.70321909422,525.158582208306));
#108540=CARTESIAN_POINT('Ctrl Pts',(-28.6745327676321,1077.67588233529,
525.400812310426));
#108541=CARTESIAN_POINT('Ctrl Pts',(-28.7154274784568,1077.66113102755,
525.537971543861));
#108542=CARTESIAN_POINT('Ctrl Pts',(-28.7431770550444,1077.63175362073,
525.823645092682));
#108543=CARTESIAN_POINT('Ctrl Pts',(-28.7284302767064,1077.61741865038,
525.969646916927));
#108544=CARTESIAN_POINT('Ctrl Pts',(-28.6449441352305,1077.59219522922,
526.240846925399));
#108545=CARTESIAN_POINT('Ctrl Pts',(-28.5795927763327,1077.58139702623,
526.364330327838));
#108546=CARTESIAN_POINT('Ctrl Pts',(-28.4015536566291,1077.56360198954,
526.586490696771));
#108547=CARTESIAN_POINT('Ctrl Pts',(-28.2883033202278,1077.55702438246,
526.681222253459));
#108548=CARTESIAN_POINT('Ctrl Pts',(-28.118571025877,1077.55230238546,526.773366796316));
#108549=CARTESIAN_POINT('Ctrl Pts',(-28.0760380383956,1077.55146969774,
526.793053012111));
#108550=CARTESIAN_POINT('Ctrl Pts',(-28.0069991874668,1077.5506558012,526.819797117005));
#108551=CARTESIAN_POINT('Ctrl Pts',(-27.9812673491887,1077.55046431516,
526.828681016945));
#108552=CARTESIAN_POINT('Ctrl Pts',(-27.9327825569301,1077.55030907861,
526.843429295737));
#108553=CARTESIAN_POINT('Ctrl Pts',(-27.9101205994786,1077.55031762927,
526.849537089353));
#108554=CARTESIAN_POINT('Ctrl Pts',(-27.8597731253211,1077.55051373359,
526.861391147864));
#108555=CARTESIAN_POINT('Ctrl Pts',(-27.8320269931328,1077.55073743459,
526.86680386544));
#108556=CARTESIAN_POINT('Ctrl Pts',(-27.7533535565146,1077.55169446046,
526.879023691287));
#108557=CARTESIAN_POINT('Ctrl Pts',(-27.7021200903622,1077.5526937158,526.883337529065));
#108558=CARTESIAN_POINT('Ctrl Pts',(-27.6456694783558,1077.55420283149,
526.884125076254));
#108559=CARTESIAN_POINT('Ctrl Pts',(-27.6405598934223,1077.55434309824,
526.884160690467));
#108560=CARTESIAN_POINT('Ctrl Pts',(-27.6354521170187,1077.55448697719,
526.884160690467));
#108561=CARTESIAN_POINT('',(-18.7711528398125,1076.67369445817,536.110401727133));
#108562=CARTESIAN_POINT('',(-18.7711528398114,1076.96239239593,533.929320229677));
#108563=CARTESIAN_POINT('Ctrl Pts',(-18.7711528398125,1076.67369445817,
536.110401727133));
#108564=CARTESIAN_POINT('Ctrl Pts',(-18.7378804569628,1076.67446093905,
536.110401727133));
#108565=CARTESIAN_POINT('Ctrl Pts',(-18.7046206626837,1076.67543331161,
536.108879017021));
#108566=CARTESIAN_POINT('Ctrl Pts',(-18.5272337525884,1076.68172279721,
536.092597788566));
#108567=CARTESIAN_POINT('Ctrl Pts',(-18.3872766379643,1076.69060559347,
536.050775989781));
#108568=CARTESIAN_POINT('Ctrl Pts',(-18.1537505337702,1076.7126886191,535.926769037891));
#108569=CARTESIAN_POINT('Ctrl Pts',(-18.0579697079482,1076.72474508379,
535.853501593805));
#108570=CARTESIAN_POINT('Ctrl Pts',(-17.886902156147,1076.75308894105,535.671291466018));
#108571=CARTESIAN_POINT('Ctrl Pts',(-17.8155522268604,1076.76943501427,
535.561171622241));
#108572=CARTESIAN_POINT('Ctrl Pts',(-17.7111553573034,1076.80497018818,
535.311966774057));
#108573=CARTESIAN_POINT('Ctrl Pts',(-17.6824284223714,1076.82396971125,
535.173473734423));
#108574=CARTESIAN_POINT('Ctrl Pts',(-17.6789074975495,1076.86159765628,
534.88876956391));
#108575=CARTESIAN_POINT('Ctrl Pts',(-17.7058880366738,1076.87984471399,
534.745107066));
#108576=CARTESIAN_POINT('Ctrl Pts',(-17.8120177685867,1076.91175883886,
534.482845643484));
#108577=CARTESIAN_POINT('Ctrl Pts',(-17.8876864205616,1076.92532263287,
534.365695713357));
#108578=CARTESIAN_POINT('Ctrl Pts',(-18.0817082999133,1076.94733838705,
534.163039433835));
#108579=CARTESIAN_POINT('Ctrl Pts',(-18.199238741333,1076.9554303907,534.080451454268));
#108580=CARTESIAN_POINT('Ctrl Pts',(-18.3746955392613,1076.9616169263,534.002735542328));
#108581=CARTESIAN_POINT('Ctrl Pts',(-18.4212096783747,1076.96278143829,
533.985808584999));
#108582=CARTESIAN_POINT('Ctrl Pts',(-18.4961774846045,1076.96392959738,
533.964169585458));
#108583=CARTESIAN_POINT('Ctrl Pts',(-18.523935830246,1076.96420372957,533.957326422666));
#108584=CARTESIAN_POINT('Ctrl Pts',(-18.5755035674115,1076.96443793394,
533.946744260779));
#108585=CARTESIAN_POINT('Ctrl Pts',(-18.5992285780617,1076.96444072849,
533.942688669616));
#108586=CARTESIAN_POINT('Ctrl Pts',(-18.6510674633464,1076.96422008411,
533.935583658997));
#108587=CARTESIAN_POINT('Ctrl Pts',(-18.6792039575024,1076.96395717902,
533.932836110281));
#108588=CARTESIAN_POINT('Ctrl Pts',(-18.7286390493162,1076.96324559583,
533.929941831058));
#108589=CARTESIAN_POINT('Ctrl Pts',(-18.7498944078045,1076.96285919691,
533.929320229677));
#108590=CARTESIAN_POINT('Ctrl Pts',(-18.7711528398114,1076.96239239593,
533.929320229677));
#108591=CARTESIAN_POINT('Ctrl Pts',(-18.7711528398114,1076.96239239593,
533.929320229677));
#108592=CARTESIAN_POINT('Ctrl Pts',(-18.7711593766065,1076.96239225239,
533.929320229677));
#108593=CARTESIAN_POINT('Ctrl Pts',(-18.7711659134019,1076.96239210885,
533.929320229734));
#108594=CARTESIAN_POINT('Ctrl Pts',(-18.7711724501977,1076.96239196529,
533.929320229852));
#108595=CARTESIAN_POINT('Ctrl Pts',(-18.8565470695821,1076.96051707751,
533.92932176508));
#108596=CARTESIAN_POINT('Ctrl Pts',(-18.9415806054822,1076.95735439006,
533.939348641314));
#108597=CARTESIAN_POINT('Ctrl Pts',(-19.1311778469061,1076.94732487712,
533.984639419983));
#108598=CARTESIAN_POINT('Ctrl Pts',(-19.2332505207632,1076.93971791319,
534.026023063032));
#108599=CARTESIAN_POINT('Ctrl Pts',(-19.4322264027534,1076.91999849037,
534.144003844772));
#108600=CARTESIAN_POINT('Ctrl Pts',(-19.5257787844361,1076.90761052154,
534.223242102698));
#108601=CARTESIAN_POINT('Ctrl Pts',(-19.6896244258647,1076.87861076925,
534.417202776863));
#108602=CARTESIAN_POINT('Ctrl Pts',(-19.7558130643799,1076.86195584331,
534.532870669917));
#108603=CARTESIAN_POINT('Ctrl Pts',(-19.8470606724238,1076.82577138095,
534.791809293444));
#108604=CARTESIAN_POINT('Ctrl Pts',(-19.8676232339308,1076.80644511075,
534.934197365998));
#108605=CARTESIAN_POINT('Ctrl Pts',(-19.8527423631478,1076.76870475962,
535.220301377621));
#108606=CARTESIAN_POINT('Ctrl Pts',(-19.8168486234442,1076.75065191003,
535.361373301155));
#108607=CARTESIAN_POINT('Ctrl Pts',(-19.6959630684685,1076.71958458469,
535.61339210574));
#108608=CARTESIAN_POINT('Ctrl Pts',(-19.6152485022439,1076.70658854724,
535.723545725683));
#108609=CARTESIAN_POINT('Ctrl Pts',(-19.4206961725884,1076.68647771366,
535.905572984115));
#108610=CARTESIAN_POINT('Ctrl Pts',(-19.3097538384437,1076.67934105716,
535.977138375156));
#108611=CARTESIAN_POINT('Ctrl Pts',(-19.1467569215491,1076.67394631301,
536.04468022157));
#108612=CARTESIAN_POINT('Ctrl Pts',(-19.1038417330316,1076.67293972572,
536.059405377297));
#108613=CARTESIAN_POINT('Ctrl Pts',(-19.033663976462,1076.67194329584,536.078690605452));
#108614=CARTESIAN_POINT('Ctrl Pts',(-19.0069350927697,1076.6717093418,536.084961511477));
#108615=CARTESIAN_POINT('Ctrl Pts',(-18.9584943858724,1076.67154464201,
536.094413085446));
#108616=CARTESIAN_POINT('Ctrl Pts',(-18.9368703335593,1076.67156227912,
536.09795967355));
#108617=CARTESIAN_POINT('Ctrl Pts',(-18.8863234875917,1076.67181449225,
536.104693134127));
#108618=CARTESIAN_POINT('Ctrl Pts',(-18.8573522663231,1076.6721181415,536.107378591539));
#108619=CARTESIAN_POINT('Ctrl Pts',(-18.8092665804636,1076.67288406952,
536.109902316604));
#108620=CARTESIAN_POINT('Ctrl Pts',(-18.7902076457917,1076.6732555012,536.110401727133));
#108621=CARTESIAN_POINT('Ctrl Pts',(-18.7711528398125,1076.67369445817,
536.110401727133));
#108622=CARTESIAN_POINT('',(-83.8577571500211,1078.68595559847,394.657284692478));
#108623=CARTESIAN_POINT('',(-83.8577571699087,1078.65918801557,391.700678428093));
#108624=CARTESIAN_POINT('Ctrl Pts',(-83.857757150021,1078.68595559847,394.657284692479));
#108625=CARTESIAN_POINT('Ctrl Pts',(-83.7830020049961,1078.68756601077,
394.657284692479));
#108626=CARTESIAN_POINT('Ctrl Pts',(-83.7081818716811,1078.68909176713,
394.65161448755));
#108627=CARTESIAN_POINT('Ctrl Pts',(-83.4473097045803,1078.69413214015,
394.611658438446));
#108628=CARTESIAN_POINT('Ctrl Pts',(-83.2678576875645,1078.69709119872,
394.5475779628));
#108629=CARTESIAN_POINT('Ctrl Pts',(-82.9555074237683,1078.70153146215,
394.362880050757));
#108630=CARTESIAN_POINT('Ctrl Pts',(-82.8225076238217,1078.70308077374,
394.248529135822));
#108631=CARTESIAN_POINT('Ctrl Pts',(-82.6516281007895,1078.70464604701,
394.039149515351));
#108632=CARTESIAN_POINT('Ctrl Pts',(-82.5982181108242,1078.70503348135,
393.958851975401));
#108633=CARTESIAN_POINT('Ctrl Pts',(-82.535740029746,1078.70534048075,393.841550260136));
#108634=CARTESIAN_POINT('Ctrl Pts',(-82.5197021499793,1078.70540102225,
393.808533282827));
#108635=CARTESIAN_POINT('Ctrl Pts',(-82.4952411485322,1078.7054612726,393.753007193096));
#108636=CARTESIAN_POINT('Ctrl Pts',(-82.4861084175877,1078.70547477707,
393.730828492865));
#108637=CARTESIAN_POINT('Ctrl Pts',(-82.4694008190376,1078.70548101321,
393.68727347696));
#108638=CARTESIAN_POINT('Ctrl Pts',(-82.4617702176421,1078.70547484159,
393.665925560053));
#108639=CARTESIAN_POINT('Ctrl Pts',(-82.445102997834,1078.70543892756,393.615679087994));
#108640=CARTESIAN_POINT('Ctrl Pts',(-82.4364572227992,1078.70540198493,
393.586661580845));
#108641=CARTESIAN_POINT('Ctrl Pts',(-82.4118776292392,1078.7052326084,393.493839697126));
#108642=CARTESIAN_POINT('Ctrl Pts',(-82.3993059989355,1078.70503931191,
393.429228270991));
#108643=CARTESIAN_POINT('Ctrl Pts',(-82.3664518067997,1078.70395439044,
393.168779889638));
#108644=CARTESIAN_POINT('Ctrl Pts',(-82.3810479627093,1078.70245681784,
392.970603162102));
#108645=CARTESIAN_POINT('Ctrl Pts',(-82.477378225941,1078.69838679515,392.62589133012));
#108646=CARTESIAN_POINT('Ctrl Pts',(-82.5458454370355,1078.69607986296,
392.478811472983));
#108647=CARTESIAN_POINT('Ctrl Pts',(-82.7355870232928,1078.69024848228,
392.200768214227));
#108648=CARTESIAN_POINT('Ctrl Pts',(-82.8595022990829,1078.68667601281,
392.074604992627));
#108649=CARTESIAN_POINT('Ctrl Pts',(-83.1564653130985,1078.67830698645,
391.864012121185));
#108650=CARTESIAN_POINT('Ctrl Pts',(-83.3297793584802,1078.67351179497,
391.785357451956));
#108651=CARTESIAN_POINT('Ctrl Pts',(-83.6263047866715,1078.66541325289,
391.714282887937));
#108652=CARTESIAN_POINT('Ctrl Pts',(-83.7419675128545,1078.66228048325,
391.700678426534));
#108653=CARTESIAN_POINT('Ctrl Pts',(-83.8577571699228,1078.6591880161,391.700678428093));
#108654=CARTESIAN_POINT('Ctrl Pts',(-83.8577571699228,1078.6591880161,391.700678428093));
#108655=CARTESIAN_POINT('Ctrl Pts',(-83.9361428063095,1078.65709452164,
391.700678429148));
#108656=CARTESIAN_POINT('Ctrl Pts',(-84.0145866217131,1078.65501982623,
391.706912780499));
#108657=CARTESIAN_POINT('Ctrl Pts',(-84.2777277500826,1078.64816109357,
391.749204980039));
#108658=CARTESIAN_POINT('Ctrl Pts',(-84.4557642993797,1078.64369124269,
391.814051899594));
#108659=CARTESIAN_POINT('Ctrl Pts',(-84.767012057516,1078.6365087334,392.000321846345));
#108660=CARTESIAN_POINT('Ctrl Pts',(-84.9000006834767,1078.63375775461,
392.116098628436));
#108661=CARTESIAN_POINT('Ctrl Pts',(-85.0681332592125,1078.63098308652,
392.32512370263));
#108662=CARTESIAN_POINT('Ctrl Pts',(-85.1195945401495,1078.63029128167,
392.403191166495));
#108663=CARTESIAN_POINT('Ctrl Pts',(-85.1804949501597,1078.6297326019,392.517861140866));
#108664=CARTESIAN_POINT('Ctrl Pts',(-85.1964325685189,1078.62962003544,
392.550758955335));
#108665=CARTESIAN_POINT('Ctrl Pts',(-85.2208593784637,1078.62950795544,
392.606341466739));
#108666=CARTESIAN_POINT('Ctrl Pts',(-85.2300397724008,1078.62948308274,
392.628704567858));
#108667=CARTESIAN_POINT('Ctrl Pts',(-85.2469014151216,1078.62947314879,
392.672829015174));
#108668=CARTESIAN_POINT('Ctrl Pts',(-85.2546296799325,1078.6294863213,392.694565083902));
#108669=CARTESIAN_POINT('Ctrl Pts',(-85.2715916654432,1078.62955959754,
392.74605848812));
#108670=CARTESIAN_POINT('Ctrl Pts',(-85.2803995957563,1078.62963451504,
392.775944483141));
#108671=CARTESIAN_POINT('Ctrl Pts',(-85.3056802704074,1078.62998047341,
392.872926123062));
#108672=CARTESIAN_POINT('Ctrl Pts',(-85.3183974782786,1078.63037894675,
392.940904097667));
#108673=CARTESIAN_POINT('Ctrl Pts',(-85.3319452307445,1078.6313252237,393.058309575461));
#108674=CARTESIAN_POINT('Ctrl Pts',(-85.3351402243465,1078.63179597117,
393.107348224157));
#108675=CARTESIAN_POINT('Ctrl Pts',(-85.3358886250479,1078.63234098491,
393.156453950822));
#108676=CARTESIAN_POINT('Ctrl Pts',(-85.3380512724778,1078.63391590668,
393.298354370417));
#108677=CARTESIAN_POINT('Ctrl Pts',(-85.319769042644,1078.63610153108,393.439820960922));
#108678=CARTESIAN_POINT('Ctrl Pts',(-85.2384769594119,1078.64180196812,
393.73100120205));
#108679=CARTESIAN_POINT('Ctrl Pts',(-85.1704821986696,1078.6454133185,393.877450934156));
#108680=CARTESIAN_POINT('Ctrl Pts',(-84.9823652816383,1078.65367758615,
394.154166395819));
#108681=CARTESIAN_POINT('Ctrl Pts',(-84.8597262402881,1078.65832495621,
394.279792018397));
#108682=CARTESIAN_POINT('Ctrl Pts',(-84.566136971883,1078.66802426645,394.489889677009));
#108683=CARTESIAN_POINT('Ctrl Pts',(-84.3949648404668,1078.67298987461,
394.568835447));
#108684=CARTESIAN_POINT('Ctrl Pts',(-84.0969449776526,1078.68058133679,
394.642751299174));
#108685=CARTESIAN_POINT('Ctrl Pts',(-83.9774343555987,1078.68337745292,
394.657284692479));
#108686=CARTESIAN_POINT('Ctrl Pts',(-83.857757150021,1078.68595559847,394.657284692479));
#108687=CARTESIAN_POINT('',(-93.479943233477,1078.36968470723,401.021131275777));
#108688=CARTESIAN_POINT('',(-93.4799432334773,1078.32768892479,398.470243033506));
#108689=CARTESIAN_POINT('Ctrl Pts',(-93.4799432334771,1078.36968470723,
401.021131275778));
#108690=CARTESIAN_POINT('Ctrl Pts',(-93.3443468026236,1078.37788346231,
401.021131275778));
#108691=CARTESIAN_POINT('Ctrl Pts',(-93.2093682722063,1078.38557917959,
400.999506151711));
#108692=CARTESIAN_POINT('Ctrl Pts',(-92.928228749206,1078.40067097742,400.906706245128));
#108693=CARTESIAN_POINT('Ctrl Pts',(-92.7870338447336,1078.40763059762,
400.828399373262));
#108694=CARTESIAN_POINT('Ctrl Pts',(-92.5426108389938,1078.41853931467,
400.624950294691));
#108695=CARTESIAN_POINT('Ctrl Pts',(-92.4410200677746,1078.42243681255,
400.502230414303));
#108696=CARTESIAN_POINT('Ctrl Pts',(-92.3353783834339,1078.42553732989,
400.311653448111));
#108697=CARTESIAN_POINT('Ctrl Pts',(-92.3100605755805,1078.42614825743,
400.257274590558));
#108698=CARTESIAN_POINT('Ctrl Pts',(-92.2791932132023,1078.42667705383,
400.176568920504));
#108699=CARTESIAN_POINT('Ctrl Pts',(-92.2705015924285,1078.42679127773,
400.151532750479));
#108700=CARTESIAN_POINT('Ctrl Pts',(-92.2570434538043,1078.42690397468,
400.108482066834));
#108701=CARTESIAN_POINT('Ctrl Pts',(-92.2518802888594,1078.42692676604,
400.090600805307));
#108702=CARTESIAN_POINT('Ctrl Pts',(-92.2422505638834,1078.42692490132,
400.054287235839));
#108703=CARTESIAN_POINT('Ctrl Pts',(-92.2378001219983,1078.42689934626,
400.035855456433));
#108704=CARTESIAN_POINT('Ctrl Pts',(-92.2279503806879,1078.42677699572,
399.99066928959));
#108705=CARTESIAN_POINT('Ctrl Pts',(-92.2229957402848,1078.42665386976,
399.963827764946));
#108706=CARTESIAN_POINT('Ctrl Pts',(-92.2086630231361,1078.42604428688,
399.869278765671));
#108707=CARTESIAN_POINT('Ctrl Pts',(-92.2038680061345,1078.4252910569,399.80099849208));
#108708=CARTESIAN_POINT('Ctrl Pts',(-92.2063023970707,1078.42156961972,
399.562532434339));
#108709=CARTESIAN_POINT('Ctrl Pts',(-92.2420643603704,1078.41701476496,
399.394500946095));
#108710=CARTESIAN_POINT('Ctrl Pts',(-92.3655777692062,1078.40555107239,
399.109529049789));
#108711=CARTESIAN_POINT('Ctrl Pts',(-92.4423752417591,1078.39926392785,
398.990746016807));
#108712=CARTESIAN_POINT('Ctrl Pts',(-92.6397786825266,1078.38424410647,
398.773983516468));
#108713=CARTESIAN_POINT('Ctrl Pts',(-92.7620361835586,1078.37546399791,
398.680479090426));
#108714=CARTESIAN_POINT('Ctrl Pts',(-92.9872004074533,1078.35992808373,
398.564990802216));
#108715=CARTESIAN_POINT('Ctrl Pts',(-93.0816331847033,1078.3535622419,398.529880805453));
#108716=CARTESIAN_POINT('Ctrl Pts',(-93.2776558908996,1078.34062563531,
398.482317337839));
#108717=CARTESIAN_POINT('Ctrl Pts',(-93.3786182744213,1078.33409880642,
398.470243033506));
#108718=CARTESIAN_POINT('Ctrl Pts',(-93.4799432334774,1078.32768892479,
398.470243033506));
#108719=CARTESIAN_POINT('Ctrl Pts',(-93.4799432334774,1078.32768892479,
398.470243033506));
#108720=CARTESIAN_POINT('Ctrl Pts',(-93.4800221521823,1078.32768393234,
398.470243033506));
#108721=CARTESIAN_POINT('Ctrl Pts',(-93.4801010711071,1078.32767893996,
398.47024304083));
#108722=CARTESIAN_POINT('Ctrl Pts',(-93.4801799902509,1078.32767394766,
398.47024305548));
#108723=CARTESIAN_POINT('Ctrl Pts',(-93.6475450953458,1078.31708668642,
398.470274122951));
#108724=CARTESIAN_POINT('Ctrl Pts',(-93.813324821803,1078.30697958876,398.503247682793));
#108725=CARTESIAN_POINT('Ctrl Pts',(-94.1110507908088,1078.2897294135,398.626569583309));
#108726=CARTESIAN_POINT('Ctrl Pts',(-94.2421493192321,1078.28256603449,
398.711376395216));
#108727=CARTESIAN_POINT('Ctrl Pts',(-94.4731405686298,1078.27107926861,
398.929147344998));
#108728=CARTESIAN_POINT('Ctrl Pts',(-94.569046186137,1078.26702254175,399.06226731877));
#108729=CARTESIAN_POINT('Ctrl Pts',(-94.6529473653915,1078.26462949997,
399.243498387251));
#108730=CARTESIAN_POINT('Ctrl Pts',(-94.667049114324,1078.26429572699,399.277806795964));
#108731=CARTESIAN_POINT('Ctrl Pts',(-94.6876349454864,1078.26393260091,
399.334842287549));
#108732=CARTESIAN_POINT('Ctrl Pts',(-94.695017900571,1078.26383669524,399.35722049196));
#108733=CARTESIAN_POINT('Ctrl Pts',(-94.7070735842507,1078.26374648541,
399.397477868595));
#108734=CARTESIAN_POINT('Ctrl Pts',(-94.7119856526584,1078.2637347001,399.415278189755));
#108735=CARTESIAN_POINT('Ctrl Pts',(-94.7215007570535,1078.26376851016,
399.452928577923));
#108736=CARTESIAN_POINT('Ctrl Pts',(-94.7260180708382,1078.26382015356,
399.472794937436));
#108737=CARTESIAN_POINT('Ctrl Pts',(-94.7365988302227,1078.26404408383,
399.52509143752));
#108738=CARTESIAN_POINT('Ctrl Pts',(-94.7418832482197,1078.26427119764,
399.55766300504));
#108739=CARTESIAN_POINT('Ctrl Pts',(-94.7589552501901,1078.26561079107,
399.696841893122));
#108740=CARTESIAN_POINT('Ctrl Pts',(-94.7585335945485,1078.26756087739,
399.804488076565));
#108741=CARTESIAN_POINT('Ctrl Pts',(-94.7284222724645,1078.2736692602,400.035142288318));
#108742=CARTESIAN_POINT('Ctrl Pts',(-94.6939426921799,1078.278112298,400.156383552612));
#108743=CARTESIAN_POINT('Ctrl Pts',(-94.5844842414275,1078.28959199805,
400.39877399275));
#108744=CARTESIAN_POINT('Ctrl Pts',(-94.5058292701608,1078.29679870896,
400.516443260722));
#108745=CARTESIAN_POINT('Ctrl Pts',(-94.3052864300364,1078.31345013503,
400.729958641151));
#108746=CARTESIAN_POINT('Ctrl Pts',(-94.1819085725339,1078.32289706299,
400.821423045078));
#108747=CARTESIAN_POINT('Ctrl Pts',(-93.8987493745196,1078.34306541874,
400.961463479716));
#108748=CARTESIAN_POINT('Ctrl Pts',(-93.7395389413744,1078.35364300685,
401.00510255998));
#108749=CARTESIAN_POINT('Ctrl Pts',(-93.5442751715031,1078.36576886695,
401.019915801626));
#108750=CARTESIAN_POINT('Ctrl Pts',(-93.5120918319992,1078.36774086193,
401.021131275778));
#108751=CARTESIAN_POINT('Ctrl Pts',(-93.4799432334771,1078.36968470723,
401.021131275778));
#108752=CARTESIAN_POINT('',(-103.499585384594,1077.68406953396,408.809642574865));
#108753=CARTESIAN_POINT('',(-103.499585384594,1077.64750623718,406.61198030288));
#108754=CARTESIAN_POINT('Ctrl Pts',(-103.499585384593,1077.68406953396,
408.809642574865));
#108755=CARTESIAN_POINT('Ctrl Pts',(-103.387195904803,1077.69544404394,
408.809642574865));
#108756=CARTESIAN_POINT('Ctrl Pts',(-103.275219790437,1077.70642353688,
408.79239857909));
#108757=CARTESIAN_POINT('Ctrl Pts',(-103.033088326383,1077.72939676398,
408.715662964053));
#108758=CARTESIAN_POINT('Ctrl Pts',(-102.907898540638,1077.74071996647,
408.647468219755));
#108759=CARTESIAN_POINT('Ctrl Pts',(-102.705108256707,1077.75805576399,
408.479631245935));
#108760=CARTESIAN_POINT('Ctrl Pts',(-102.624742911153,1077.76446604495,
408.386807518368));
#108761=CARTESIAN_POINT('Ctrl Pts',(-102.51405891374,1077.77241716349,408.205169765255));
#108762=CARTESIAN_POINT('Ctrl Pts',(-102.476624646068,1077.77475445129,
408.122167372458));
#108763=CARTESIAN_POINT('Ctrl Pts',(-102.441461890835,1077.77637828966,
408.00847543288));
#108764=CARTESIAN_POINT('Ctrl Pts',(-102.434153463183,1077.77665665802,
407.981152193012));
#108765=CARTESIAN_POINT('Ctrl Pts',(-102.424194390188,1077.77692835504,
407.937188192762));
#108766=CARTESIAN_POINT('Ctrl Pts',(-102.42085834713,1077.77699146811,407.920716689828));
#108767=CARTESIAN_POINT('Ctrl Pts',(-102.415318214654,1077.77703812476,
407.889724956683));
#108768=CARTESIAN_POINT('Ctrl Pts',(-102.413024910849,1077.7770307153,407.875224574348));
#108769=CARTESIAN_POINT('Ctrl Pts',(-102.408525549262,1077.77694853326,
407.842544264892));
#108770=CARTESIAN_POINT('Ctrl Pts',(-102.406482064689,1077.77685756785,
407.824346534452));
#108771=CARTESIAN_POINT('Ctrl Pts',(-102.401855056095,1077.7764605486,407.771194294265));
#108772=CARTESIAN_POINT('Ctrl Pts',(-102.400487934671,1077.77603414094,
407.736158649954));
#108773=CARTESIAN_POINT('Ctrl Pts',(-102.402087814159,1077.77297595205,
407.554773456108));
#108774=CARTESIAN_POINT('Ctrl Pts',(-102.432600529893,1077.76767653332,
407.410246970002));
#108775=CARTESIAN_POINT('Ctrl Pts',(-102.536710677082,1077.75353423174,
407.168615955267));
#108776=CARTESIAN_POINT('Ctrl Pts',(-102.599789875725,1077.74570258254,
407.069383771022));
#108777=CARTESIAN_POINT('Ctrl Pts',(-102.762352772215,1077.72657605154,
406.885953758826));
#108778=CARTESIAN_POINT('Ctrl Pts',(-102.86358111237,1077.71515978003,406.805631539784));
#108779=CARTESIAN_POINT('Ctrl Pts',(-103.057064140004,1077.6939836464,406.700836816488));
#108780=CARTESIAN_POINT('Ctrl Pts',(-103.143010528088,1077.68475060885,
406.667394956358));
#108781=CARTESIAN_POINT('Ctrl Pts',(-103.319555893004,1077.66609486489,
406.623083169243));
#108782=CARTESIAN_POINT('Ctrl Pts',(-103.409399714469,1077.65674657888,
406.61198030288));
#108783=CARTESIAN_POINT('Ctrl Pts',(-103.499585384594,1077.64750623718,
406.61198030288));
#108784=CARTESIAN_POINT('Ctrl Pts',(-103.499585384594,1077.64750623718,
406.61198030288));
#108785=CARTESIAN_POINT('Ctrl Pts',(-103.499677903439,1077.64749675779,
406.61198030288));
#108786=CARTESIAN_POINT('Ctrl Pts',(-103.499770422644,1077.6474872785,406.611980314598));
#108787=CARTESIAN_POINT('Ctrl Pts',(-103.499862942206,1077.64747779934,
406.611980337968));
#108788=CARTESIAN_POINT('Ctrl Pts',(-103.645113351412,1077.63259604917,
406.612017027284));
#108789=CARTESIAN_POINT('Ctrl Pts',(-103.78901276622,1077.61822198197,406.640853589671));
#108790=CARTESIAN_POINT('Ctrl Pts',(-104.050499855146,1077.5929165144,406.750104219455));
#108791=CARTESIAN_POINT('Ctrl Pts',(-104.166776622412,1077.58206955235,
406.826846821377));
#108792=CARTESIAN_POINT('Ctrl Pts',(-104.359585229407,1077.56505932727,
407.014439894671));
#108793=CARTESIAN_POINT('Ctrl Pts',(-104.436360211142,1077.55881456015,
407.121712524817));
#108794=CARTESIAN_POINT('Ctrl Pts',(-104.518664583071,1077.55312449566,
407.295305133208));
#108795=CARTESIAN_POINT('Ctrl Pts',(-104.540205719576,1077.55183917524,
407.352649557091));
#108796=CARTESIAN_POINT('Ctrl Pts',(-104.563392490146,1077.55080367557,
407.434553513139));
#108797=CARTESIAN_POINT('Ctrl Pts',(-104.569163649531,1077.55059554773,
407.457816567282));
#108798=CARTESIAN_POINT('Ctrl Pts',(-104.577163530036,1077.55039678801,
407.495264322674));
#108799=CARTESIAN_POINT('Ctrl Pts',(-104.57988289321,1077.55035237737,407.509335590598));
#108800=CARTESIAN_POINT('Ctrl Pts',(-104.584899660064,1077.55032279116,
407.538327872764));
#108801=CARTESIAN_POINT('Ctrl Pts',(-104.587166359717,1077.55034089609,
407.553251045044));
#108802=CARTESIAN_POINT('Ctrl Pts',(-104.591680568707,1077.55045930185,
407.587743127609));
#108803=CARTESIAN_POINT('Ctrl Pts',(-104.593710738872,1077.55058295483,
407.607334956696));
#108804=CARTESIAN_POINT('Ctrl Pts',(-104.59835973683,1077.55114023486,407.668087676534));
#108805=CARTESIAN_POINT('Ctrl Pts',(-104.599188787289,1077.55176454043,
407.709345782444));
#108806=CARTESIAN_POINT('Ctrl Pts',(-104.592420320313,1077.55570454201,
407.896386519467));
#108807=CARTESIAN_POINT('Ctrl Pts',(-104.558149962599,1077.56179066911,
408.03960335307));
#108808=CARTESIAN_POINT('Ctrl Pts',(-104.447617840476,1077.5774967984,408.278720181223));
#108809=CARTESIAN_POINT('Ctrl Pts',(-104.381421926256,1077.58610752184,
408.376847563264));
#108810=CARTESIAN_POINT('Ctrl Pts',(-104.212973558089,1077.60671077601,
408.55643095952));
#108811=CARTESIAN_POINT('Ctrl Pts',(-104.109175869781,1077.61878832806,
408.63403867532));
#108812=CARTESIAN_POINT('Ctrl Pts',(-103.870733798094,1077.64537003777,
408.754299904278));
#108813=CARTESIAN_POINT('Ctrl Pts',(-103.736380651267,1077.65975831344,
408.792724592087));
#108814=CARTESIAN_POINT('Ctrl Pts',(-103.565530808957,1077.67736519591,
408.808160083521));
#108815=CARTESIAN_POINT('Ctrl Pts',(-103.532540320879,1077.68073429073,
408.809642574865));
#108816=CARTESIAN_POINT('Ctrl Pts',(-103.499585384593,1077.68406953396,
408.809642574865));
#108817=CARTESIAN_POINT('',(-111.756957497768,1076.82908683399,418.58236328462));
#108818=CARTESIAN_POINT('',(-111.75695749777,1076.81044237657,416.401281787164));
#108819=CARTESIAN_POINT('Ctrl Pts',(-111.756957497768,1076.82908683399,
418.582363284621));
#108820=CARTESIAN_POINT('Ctrl Pts',(-111.628259262186,1076.8463078706,418.582363284621));
#108821=CARTESIAN_POINT('Ctrl Pts',(-111.500348586371,1076.86315267952,
418.559579819116));
#108822=CARTESIAN_POINT('Ctrl Pts',(-111.246798174954,1076.89600265962,
418.465958371192));
#108823=CARTESIAN_POINT('Ctrl Pts',(-111.124924534418,1076.911467731,418.391744289392));
#108824=CARTESIAN_POINT('Ctrl Pts',(-110.930262576408,1076.93559468084,
418.21350468216));
#108825=CARTESIAN_POINT('Ctrl Pts',(-110.854450678783,1076.94472378238,
418.11616918541));
#108826=CARTESIAN_POINT('Ctrl Pts',(-110.747079300555,1076.95711960265,
417.916401071468));
#108827=CARTESIAN_POINT('Ctrl Pts',(-110.711140439506,1076.96099751614,
417.818036534783));
#108828=CARTESIAN_POINT('Ctrl Pts',(-110.683801095832,1076.96348609575,
417.687884112442));
#108829=CARTESIAN_POINT('Ctrl Pts',(-110.679007433349,1076.96387630448,
417.659538662239));
#108830=CARTESIAN_POINT('Ctrl Pts',(-110.673222765968,1076.96425764857,
417.614594389605));
#108831=CARTESIAN_POINT('Ctrl Pts',(-110.671481815592,1076.96434773263,
417.598107341844));
#108832=CARTESIAN_POINT('Ctrl Pts',(-110.669075432751,1076.96441934202,
417.568971525337));
#108833=CARTESIAN_POINT('Ctrl Pts',(-110.668253236375,1076.96442148999,
417.556339095609));
#108834=CARTESIAN_POINT('Ctrl Pts',(-110.666879590667,1076.96436055169,
417.527493054449));
#108835=CARTESIAN_POINT('Ctrl Pts',(-110.666469633752,1076.96427894538,
417.511275920127));
#108836=CARTESIAN_POINT('Ctrl Pts',(-110.666338713738,1076.9639279657,417.467119864967));
#108837=CARTESIAN_POINT('Ctrl Pts',(-110.66732936936,1076.96356568417,417.439192707383));
#108838=CARTESIAN_POINT('Ctrl Pts',(-110.677327174604,1076.96113241606,
417.304097911965));
#108839=CARTESIAN_POINT('Ctrl Pts',(-110.701075157017,1076.95714930044,
417.198694067498));
#108840=CARTESIAN_POINT('Ctrl Pts',(-110.779225135746,1076.94522297492,
416.996578366205));
#108841=CARTESIAN_POINT('Ctrl Pts',(-110.833702655736,1076.93728064874,
416.901252350489));
#108842=CARTESIAN_POINT('Ctrl Pts',(-110.977153046549,1076.91688585791,
416.719718413115));
#108843=CARTESIAN_POINT('Ctrl Pts',(-111.068482638917,1076.90414816897,
416.637328507757));
#108844=CARTESIAN_POINT('Ctrl Pts',(-111.26119942533,1076.8775905672,416.514664442732));
#108845=CARTESIAN_POINT('Ctrl Pts',(-111.358823174717,1076.8642527306,416.471006946803));
#108846=CARTESIAN_POINT('Ctrl Pts',(-111.557414731369,1076.83729812384,
416.415035320248));
#108847=CARTESIAN_POINT('Ctrl Pts',(-111.656961589264,1076.82386419738,
416.401281787164));
#108848=CARTESIAN_POINT('Ctrl Pts',(-111.756957497771,1076.81044237657,
416.401281787164));
#108849=CARTESIAN_POINT('Ctrl Pts',(-111.756957497771,1076.81044237657,
416.401281787165));
#108850=CARTESIAN_POINT('Ctrl Pts',(-111.757267709608,1076.81040073879,
416.401281787165));
#108851=CARTESIAN_POINT('Ctrl Pts',(-111.757577925767,1076.81035910114,
416.401281919527));
#108852=CARTESIAN_POINT('Ctrl Pts',(-111.757888146164,1076.81031746362,
416.401282184264));
#108853=CARTESIAN_POINT('Ctrl Pts',(-111.902996520501,1076.79084114005,
416.401406017257));
#108854=CARTESIAN_POINT('Ctrl Pts',(-112.046743521567,1076.77169855101,
416.430491124244));
#108855=CARTESIAN_POINT('Ctrl Pts',(-112.309506872607,1076.73706338498,
416.54128472119));
#108856=CARTESIAN_POINT('Ctrl Pts',(-112.426914414638,1076.72177026875,
416.619978092971));
#108857=CARTESIAN_POINT('Ctrl Pts',(-112.610593742355,1076.69830509568,
416.802822001851));
#108858=CARTESIAN_POINT('Ctrl Pts',(-112.680687760257,1076.68956305877,
416.90003483103));
#108859=CARTESIAN_POINT('Ctrl Pts',(-112.775652343149,1076.67822796178,
417.091279122111));
#108860=CARTESIAN_POINT('Ctrl Pts',(-112.806488667435,1076.67478243055,
417.180888335835));
#108861=CARTESIAN_POINT('Ctrl Pts',(-112.830946879632,1076.67247436043,
417.300530613086));
#108862=CARTESIAN_POINT('Ctrl Pts',(-112.835457774785,1076.67209468439,
417.327861662961));
#108863=CARTESIAN_POINT('Ctrl Pts',(-112.840977616086,1076.67172032577,
417.371619185811));
#108864=CARTESIAN_POINT('Ctrl Pts',(-112.842663810689,1076.67163186579,
417.387946243501));
#108865=CARTESIAN_POINT('Ctrl Pts',(-112.84512027116,1076.67156185247,417.418457189968));
#108866=CARTESIAN_POINT('Ctrl Pts',(-112.845983174103,1076.6715674915,417.432629866402));
#108867=CARTESIAN_POINT('Ctrl Pts',(-112.847281541207,1076.6716644326,417.464062975881));
#108868=CARTESIAN_POINT('Ctrl Pts',(-112.847584329845,1076.67177394905,
417.481324757331));
#108869=CARTESIAN_POINT('Ctrl Pts',(-112.847277345293,1076.67224918448,
417.530821221527));
#108870=CARTESIAN_POINT('Ctrl Pts',(-112.8456482608,1076.67275449419,417.563028604543));
#108871=CARTESIAN_POINT('Ctrl Pts',(-112.828942160006,1076.67658199652,
417.73861788006));
#108872=CARTESIAN_POINT('Ctrl Pts',(-112.786990441977,1076.68355429553,
417.877825079406));
#108873=CARTESIAN_POINT('Ctrl Pts',(-112.665274248443,1076.7021883218,418.106195316027));
#108874=CARTESIAN_POINT('Ctrl Pts',(-112.595585198562,1076.71250485626,
418.198310352126));
#108875=CARTESIAN_POINT('Ctrl Pts',(-112.421820259228,1076.7376028886,418.365452664304));
#108876=CARTESIAN_POINT('Ctrl Pts',(-112.316242023973,1076.75254589309,
418.436487945748));
#108877=CARTESIAN_POINT('Ctrl Pts',(-112.076327646254,1076.78589013309,
418.543451279366));
#108878=CARTESIAN_POINT('Ctrl Pts',(-111.942348722303,1076.8041941881,418.575112552085));
#108879=CARTESIAN_POINT('Ctrl Pts',(-111.789698540157,1076.82470143,418.581994958318));
#108880=CARTESIAN_POINT('Ctrl Pts',(-111.773321650249,1076.82689715619,
418.582363284621));
#108881=CARTESIAN_POINT('Ctrl Pts',(-111.756957497768,1076.82908683399,
418.582363284621));
#108882=CARTESIAN_POINT('',(-4.59241321360755,1076.96429318502,313.820919344588));
#108883=CARTESIAN_POINT('',(-4.59241321360898,1076.67169969354,311.639837847132));
#108884=CARTESIAN_POINT('Ctrl Pts',(-4.59241321360756,1076.96429318502,
313.820919344589));
#108885=CARTESIAN_POINT('Ctrl Pts',(-4.58729141192633,1076.96432069071,
313.820919344589));
#108886=CARTESIAN_POINT('Ctrl Pts',(-4.58216931622271,1076.96434347666,
313.820883262235));
#108887=CARTESIAN_POINT('Ctrl Pts',(-4.55268786777427,1076.96444744273,
313.820467822336));
#108888=CARTESIAN_POINT('Ctrl Pts',(-4.52834681763773,1076.9644264611,313.819308398949));
#108889=CARTESIAN_POINT('Ctrl Pts',(-4.47186306088004,1076.96412909633,
313.81471738548));
#108890=CARTESIAN_POINT('Ctrl Pts',(-4.43979518576418,1076.96377179711,
313.81067042068));
#108891=CARTESIAN_POINT('Ctrl Pts',(-4.35106200456937,1076.96225555879,
313.795442454999));
#108892=CARTESIAN_POINT('Ctrl Pts',(-4.29504813396338,1076.96068964902,
313.781179160654));
#108893=CARTESIAN_POINT('Ctrl Pts',(-4.10334820036271,1076.95315811824,
313.715809651604));
#108894=CARTESIAN_POINT('Ctrl Pts',(-3.97712765537905,1076.94420059741,
313.64228441493));
#108895=CARTESIAN_POINT('Ctrl Pts',(-3.77807475162618,1076.92205481482,
313.465839559047));
#108896=CARTESIAN_POINT('Ctrl Pts',(-3.70137252335428,1076.90992091133,
313.370702534953));
#108897=CARTESIAN_POINT('Ctrl Pts',(-3.57730558465704,1076.88138648815,
313.150162388361));
#108898=CARTESIAN_POINT('Ctrl Pts',(-3.53410540296603,1076.86493319215,
313.024610501353));
#108899=CARTESIAN_POINT('Ctrl Pts',(-3.49293822453981,1076.829053337,312.754261159156));
#108900=CARTESIAN_POINT('Ctrl Pts',(-3.49916309745467,1076.80981604943,
312.61115533408));
#108901=CARTESIAN_POINT('Ctrl Pts',(-3.56661826077018,1076.771958454,312.333104019716));
#108902=CARTESIAN_POINT('Ctrl Pts',(-3.62813357417901,1076.75370491763,
312.200906315366));
#108903=CARTESIAN_POINT('Ctrl Pts',(-3.79463761831558,1076.72197916882,
311.974416325197));
#108904=CARTESIAN_POINT('Ctrl Pts',(-3.89559692218598,1076.7085736548,311.880383538161));
#108905=CARTESIAN_POINT('Ctrl Pts',(-4.12289809990298,1076.68772609551,
311.737328147627));
#108906=CARTESIAN_POINT('Ctrl Pts',(-4.24616683617815,1076.68024738659,
311.687886528618));
#108907=CARTESIAN_POINT('Ctrl Pts',(-4.42333628054291,1076.6743115547,311.651915824879));
#108908=CARTESIAN_POINT('Ctrl Pts',(-4.47185491688664,1076.67314588412,
311.6454192786));
#108909=CARTESIAN_POINT('Ctrl Pts',(-4.54453812250696,1076.6720779021,311.640626358958));
#108910=CARTESIAN_POINT('Ctrl Pts',(-4.56846673687735,1076.6718347264,311.639838072435));
#108911=CARTESIAN_POINT('Ctrl Pts',(-4.59240295092762,1076.6716997514,311.63983784718));
#108912=CARTESIAN_POINT('Ctrl Pts',(-4.59240637182156,1076.67169973211,
311.639837847148));
#108913=CARTESIAN_POINT('Ctrl Pts',(-4.59240979271534,1076.67169971282,
311.639837847132));
#108914=CARTESIAN_POINT('Ctrl Pts',(-4.59241321360898,1076.67169969354,
311.639837847132));
#108915=CARTESIAN_POINT('Ctrl Pts',(-4.59241321360898,1076.67169969354,
311.639837847132));
#108916=CARTESIAN_POINT('Ctrl Pts',(-4.61963976148801,1076.67154619972,
311.639837847132));
#108917=CARTESIAN_POINT('Ctrl Pts',(-4.64685685878174,1076.67153280805,
311.640857457555));
#108918=CARTESIAN_POINT('Ctrl Pts',(-4.70549373046377,1076.67180653836,
311.645256991049));
#108919=CARTESIAN_POINT('Ctrl Pts',(-4.73686073894702,1076.67214185729,
311.648985620302));
#108920=CARTESIAN_POINT('Ctrl Pts',(-4.82129447019147,1076.67355784612,
311.662761510641));
#108921=CARTESIAN_POINT('Ctrl Pts',(-4.87383616757046,1076.67499655887,
311.675394736954));
#108922=CARTESIAN_POINT('Ctrl Pts',(-5.06278685633759,1076.68224252415,
311.735945191482));
#108923=CARTESIAN_POINT('Ctrl Pts',(-5.19003318628404,1076.6912545598,311.806860980777));
#108924=CARTESIAN_POINT('Ctrl Pts',(-5.39141937328519,1076.71358036343,
311.978453906474));
#108925=CARTESIAN_POINT('Ctrl Pts',(-5.46942446138266,1076.72579093342,
312.071158674187));
#108926=CARTESIAN_POINT('Ctrl Pts',(-5.59728194242799,1076.75441450228,
312.286985756856));
#108927=CARTESIAN_POINT('Ctrl Pts',(-5.64306900721297,1076.77087528038,
312.410362266729));
#108928=CARTESIAN_POINT('Ctrl Pts',(-5.69066760956401,1076.80657872611,
312.67702863095));
#108929=CARTESIAN_POINT('Ctrl Pts',(-5.68840316010873,1076.82562354149,
312.818780749043));
#108930=CARTESIAN_POINT('Ctrl Pts',(-5.62939171111655,1076.86320394024,
313.097584341478));
#108931=CARTESIAN_POINT('Ctrl Pts',(-5.57162369771359,1076.88135917392,
313.231783869726));
#108932=CARTESIAN_POINT('Ctrl Pts',(-5.41074762692253,1076.91301948294,
313.464285973936));
#108933=CARTESIAN_POINT('Ctrl Pts',(-5.31137024183056,1076.92642847705,
313.561950175355));
#108934=CARTESIAN_POINT('Ctrl Pts',(-5.08104710013323,1076.94780601059,
313.715078109525));
#108935=CARTESIAN_POINT('Ctrl Pts',(-4.95225472506798,1076.95557912384,
313.769128268537));
#108936=CARTESIAN_POINT('Ctrl Pts',(-4.76774811052037,1076.96164639615,
313.807890106027));
#108937=CARTESIAN_POINT('Ctrl Pts',(-4.71821465098195,1076.96281554133,
313.814790621794));
#108938=CARTESIAN_POINT('Ctrl Pts',(-4.64309093629956,1076.96390544454,
313.820035965356));
#108939=CARTESIAN_POINT('Ctrl Pts',(-4.61775567411502,1076.96415708804,
313.820919344589));
#108940=CARTESIAN_POINT('Ctrl Pts',(-4.59241321360756,1076.96429318502,
313.820919344589));
#108941=CARTESIAN_POINT('',(-27.7552687727498,1076.95995571924,317.220797722382));
#108942=CARTESIAN_POINT('',(-27.7552687727512,1076.67624971362,315.039716224926));
#108943=CARTESIAN_POINT('Ctrl Pts',(-27.7552687727499,1076.95995571924,
317.220797722383));
#108944=CARTESIAN_POINT('Ctrl Pts',(-27.7283065932649,1076.9608315155,317.220797722383));
#108945=CARTESIAN_POINT('Ctrl Pts',(-27.7013269466995,1076.96158071917,
317.219797825468));
#108946=CARTESIAN_POINT('Ctrl Pts',(-27.6380375280953,1076.96303827534,
317.215090801021));
#108947=CARTESIAN_POINT('Ctrl Pts',(-27.6018441062499,1076.96363908436,
317.210566671319));
#108948=CARTESIAN_POINT('Ctrl Pts',(-27.5421598760239,1076.96424144341,
317.200045209562));
#108949=CARTESIAN_POINT('Ctrl Pts',(-27.5185233406895,1076.96437664644,
317.195063966051));
#108950=CARTESIAN_POINT('Ctrl Pts',(-27.4727725357422,1076.96443551049,
317.183823413574));
#108951=CARTESIAN_POINT('Ctrl Pts',(-27.4506527530679,1076.96436923397,
317.177642015045));
#108952=CARTESIAN_POINT('Ctrl Pts',(-27.3994333479822,1076.96399247892,
317.1615687837));
#108953=CARTESIAN_POINT('Ctrl Pts',(-27.370525558967,1076.96360722564,317.151136644694));
#108954=CARTESIAN_POINT('Ctrl Pts',(-27.2809741631887,1076.96186228721,
317.114475514941));
#108955=CARTESIAN_POINT('Ctrl Pts',(-27.2222700454178,1076.95989543648,
317.083959217189));
#108956=CARTESIAN_POINT('Ctrl Pts',(-27.0445564264891,1076.9511983321,316.970030246813));
#108957=CARTESIAN_POINT('Ctrl Pts',(-26.9394359176285,1076.94167740887,
316.868248954268));
#108958=CARTESIAN_POINT('Ctrl Pts',(-26.7879377872872,1076.91856026459,
316.648428107375));
#108959=CARTESIAN_POINT('Ctrl Pts',(-26.7360743008871,1076.90598960822,
316.536939532749));
#108960=CARTESIAN_POINT('Ctrl Pts',(-26.6685714347086,1076.87665653534,
316.291422777216));
#108961=CARTESIAN_POINT('Ctrl Pts',(-26.6570743801922,1076.85985904197,
316.15826683924));
#108962=CARTESIAN_POINT('Ctrl Pts',(-26.683286842315,1076.82346318484,315.884160849458));
#108963=CARTESIAN_POINT('Ctrl Pts',(-26.7247343598561,1076.80407850786,
315.74592401004));
#108964=CARTESIAN_POINT('Ctrl Pts',(-26.8590086649868,1076.76643261199,
315.492542911362));
#108965=CARTESIAN_POINT('Ctrl Pts',(-26.9509072428477,1076.74852722254,
315.379880588055));
#108966=CARTESIAN_POINT('Ctrl Pts',(-27.165830693425,1076.71793190902,315.202974765251));
#108967=CARTESIAN_POINT('Ctrl Pts',(-27.2844707606106,1076.70522514792,
315.137406121238));
#108968=CARTESIAN_POINT('Ctrl Pts',(-27.5227910213039,1076.68665485675,
315.058440623339));
#108969=CARTESIAN_POINT('Ctrl Pts',(-27.6385873640558,1076.68022264015,
315.039716557163));
#108970=CARTESIAN_POINT('Ctrl Pts',(-27.755265667519,1076.67624981935,315.03971622493));
#108971=CARTESIAN_POINT('Ctrl Pts',(-27.7552687727511,1076.67624971362,
315.039716224926));
#108972=CARTESIAN_POINT('Ctrl Pts',(-27.8007518713627,1076.67470106072,
315.039716224926));
#108973=CARTESIAN_POINT('Ctrl Pts',(-27.8461971406638,1076.67353185038,
315.042561401899));
#108974=CARTESIAN_POINT('Ctrl Pts',(-27.9202855407047,1076.67224860099,
315.051878823282));
#108975=CARTESIAN_POINT('Ctrl Pts',(-27.9490710048065,1076.67190703763,
315.056678431789));
#108976=CARTESIAN_POINT('Ctrl Pts',(-28.0000313111751,1076.67158427596,
315.067292271787));
#108977=CARTESIAN_POINT('Ctrl Pts',(-28.0222792846111,1076.67154132652,
315.072661557919));
#108978=CARTESIAN_POINT('Ctrl Pts',(-28.0685876243102,1076.67165897077,
315.085392056044));
#108979=CARTESIAN_POINT('Ctrl Pts',(-28.0925946139439,1076.67184008542,
315.092893685262));
#108980=CARTESIAN_POINT('Ctrl Pts',(-28.1542559773114,1076.67262044032,
315.11452835087));
#108981=CARTESIAN_POINT('Ctrl Pts',(-28.191421324654,1076.67340451482,315.129924308094));
#108982=CARTESIAN_POINT('Ctrl Pts',(-28.33763630249,1076.67777933126,315.200192997297));
#108983=CARTESIAN_POINT('Ctrl Pts',(-28.4378615576082,1076.68380215683,
315.271083493085));
#108984=CARTESIAN_POINT('Ctrl Pts',(-28.6057533053263,1076.70026477736,
315.438032105936));
#108985=CARTESIAN_POINT('Ctrl Pts',(-28.6738365810709,1076.71033062527,
315.531373911654));
#108986=CARTESIAN_POINT('Ctrl Pts',(-28.7835382230844,1076.7349519754,315.745741443132));
#108987=CARTESIAN_POINT('Ctrl Pts',(-28.8210098270542,1076.74967060233,
315.866999484348));
#108988=CARTESIAN_POINT('Ctrl Pts',(-28.854256696121,1076.78264601847,316.126738212153));
#108989=CARTESIAN_POINT('Ctrl Pts',(-28.8461190155926,1076.80081702579,
316.263653738805));
#108990=CARTESIAN_POINT('Ctrl Pts',(-28.7774318909521,1076.83874830462,
316.537604021781));
#108991=CARTESIAN_POINT('Ctrl Pts',(-28.7134896140636,1076.85815994421,
316.671203027659));
#108992=CARTESIAN_POINT('Ctrl Pts',(-28.5394420059432,1076.89354415798,
316.901257682134));
#108993=CARTESIAN_POINT('Ctrl Pts',(-28.4325714020263,1076.90928919192,
316.996716669842));
#108994=CARTESIAN_POINT('Ctrl Pts',(-28.1982878041784,1076.93465221454,
317.135199002589));
#108995=CARTESIAN_POINT('Ctrl Pts',(-28.0753080562897,1076.94447665053,
317.18089597302));
#108996=CARTESIAN_POINT('Ctrl Pts',(-27.8836893492438,1076.95506208686,
317.215117900989));
#108997=CARTESIAN_POINT('Ctrl Pts',(-27.8195286686761,1076.95786840369,
317.220797722383));
#108998=CARTESIAN_POINT('Ctrl Pts',(-27.7552687727499,1076.95995571924,
317.220797722383));
#108999=CARTESIAN_POINT('',(-15.901306121126,1077.7757685569,322.059817014206));
#109000=CARTESIAN_POINT('',(-15.9013061211259,1077.55169226467,319.862154742221));
#109001=CARTESIAN_POINT('Ctrl Pts',(-15.901306121126,1077.7757685569,322.059817014206));
#109002=CARTESIAN_POINT('Ctrl Pts',(-15.8763153185509,1077.77614444359,
322.059817014206));
#109003=CARTESIAN_POINT('Ctrl Pts',(-15.8513260666884,1077.77643663632,
322.058964462218));
#109004=CARTESIAN_POINT('Ctrl Pts',(-15.7992118709224,1077.77687111121,
322.055402752679));
#109005=CARTESIAN_POINT('Ctrl Pts',(-15.7721196426239,1077.77699748596,
322.052536352266));
#109006=CARTESIAN_POINT('Ctrl Pts',(-15.7193773953242,1077.77704836048,
322.044964810555));
#109007=CARTESIAN_POINT('Ctrl Pts',(-15.693733258665,1077.77698139505,322.040347667022));
#109008=CARTESIAN_POINT('Ctrl Pts',(-15.6340889654077,1077.77660956875,
322.027404544378));
#109009=CARTESIAN_POINT('Ctrl Pts',(-15.6002757202476,1077.7762312001,322.018357257053));
#109010=CARTESIAN_POINT('Ctrl Pts',(-15.4954092673977,1077.77452401565,
321.984860110433));
#109011=CARTESIAN_POINT('Ctrl Pts',(-15.4264140583218,1077.77260769411,
321.954737703618));
#109012=CARTESIAN_POINT('Ctrl Pts',(-15.2338516749138,1077.76482613741,
321.846011556185));
#109013=CARTESIAN_POINT('Ctrl Pts',(-15.1223597126749,1077.75702121677,
321.749615662955));
#109014=CARTESIAN_POINT('Ctrl Pts',(-14.9565068695404,1077.73834570816,
321.535756964948));
#109015=CARTESIAN_POINT('Ctrl Pts',(-14.8974444185682,1077.72821424148,
321.424902304248));
#109016=CARTESIAN_POINT('Ctrl Pts',(-14.815846395992,1077.70479394902,321.178655454585));
#109017=CARTESIAN_POINT('Ctrl Pts',(-14.7973751725187,1077.69150802529,
321.044049350579));
#109018=CARTESIAN_POINT('Ctrl Pts',(-14.8104680840599,1077.66292909833,
320.764718967026));
#109019=CARTESIAN_POINT('Ctrl Pts',(-14.8458506578202,1077.64782959948,
320.622650324851));
#109020=CARTESIAN_POINT('Ctrl Pts',(-14.9693979142027,1077.61891985513,
320.361181895259));
#109021=CARTESIAN_POINT('Ctrl Pts',(-15.0561021188595,1077.60537548996,
320.244108958898));
#109022=CARTESIAN_POINT('Ctrl Pts',(-15.261793050972,1077.58260156969,320.057536280435));
#109023=CARTESIAN_POINT('Ctrl Pts',(-15.3760943816234,1077.57330979647,
319.986605614853));
#109024=CARTESIAN_POINT('Ctrl Pts',(-15.6070919418772,1077.56004935432,
319.896096315778));
#109025=CARTESIAN_POINT('Ctrl Pts',(-15.719690296169,1077.55559535068,319.871216440949));
#109026=CARTESIAN_POINT('Ctrl Pts',(-15.8565128661309,1077.55249125783,
319.862839684625));
#109027=CARTESIAN_POINT('Ctrl Pts',(-15.8789061743036,1077.55205562809,
319.862154742221));
#109028=CARTESIAN_POINT('Ctrl Pts',(-15.901306121126,1077.55169226467,319.862154742221));
#109029=CARTESIAN_POINT('Ctrl Pts',(-15.901306121126,1077.55169226467,319.862154742221));
#109030=CARTESIAN_POINT('Ctrl Pts',(-15.9013154729183,1077.55169211297,
319.862154742221));
#109031=CARTESIAN_POINT('Ctrl Pts',(-15.9013248247117,1077.55169196128,
319.862154742341));
#109032=CARTESIAN_POINT('Ctrl Pts',(-15.9013341765063,1077.5516918096,319.86215474258));
#109033=CARTESIAN_POINT('Ctrl Pts',(-15.9354270010144,1077.55113886074,
319.862155613039));
#109034=CARTESIAN_POINT('Ctrl Pts',(-15.969503221363,1077.55075384282,319.863743150515));
#109035=CARTESIAN_POINT('Ctrl Pts',(-16.0295162085435,1077.55037270648,
319.869346152583));
#109036=CARTESIAN_POINT('Ctrl Pts',(-16.05548515086,1077.55030715598,319.872710190745));
#109037=CARTESIAN_POINT('Ctrl Pts',(-16.1086477485862,1077.55037833879,
319.881538190335));
#109038=CARTESIAN_POINT('Ctrl Pts',(-16.1358040189333,1077.55052713191,
319.887110404563));
#109039=CARTESIAN_POINT('Ctrl Pts',(-16.2035721971005,1077.55118327113,
319.903709135491));
#109040=CARTESIAN_POINT('Ctrl Pts',(-16.2438123836615,1077.55183582535,
319.916051576552));
#109041=CARTESIAN_POINT('Ctrl Pts',(-16.3891197145259,1077.55517374827,
319.96991664901));
#109042=CARTESIAN_POINT('Ctrl Pts',(-16.4882562820175,1077.55941189024,
320.025228405409));
#109043=CARTESIAN_POINT('Ctrl Pts',(-16.6682470308535,1077.57129210572,
320.165643791508));
#109044=CARTESIAN_POINT('Ctrl Pts',(-16.7474617131533,1077.57893653912,
320.250531662784));
#109045=CARTESIAN_POINT('Ctrl Pts',(-16.8827297744749,1077.59771946772,
320.450867575481));
#109046=CARTESIAN_POINT('Ctrl Pts',(-16.9348080994281,1077.60898296415,
320.566984549141));
#109047=CARTESIAN_POINT('Ctrl Pts',(-16.999661876788,1077.63425790322,320.821134373471));
#109048=CARTESIAN_POINT('Ctrl Pts',(-17.0085147851678,1077.64820141357,
320.958038324616));
#109049=CARTESIAN_POINT('Ctrl Pts',(-16.9745994864718,1077.67734414832,
321.238225219221));
#109050=CARTESIAN_POINT('Ctrl Pts',(-16.928204810578,1077.69227788608,321.378517652842));
#109051=CARTESIAN_POINT('Ctrl Pts',(-16.7845999240235,1077.71980366842,
321.630143207751));
#109052=CARTESIAN_POINT('Ctrl Pts',(-16.6898009891721,1077.73218168076,
321.739656395799));
#109053=CARTESIAN_POINT('Ctrl Pts',(-16.4752118164617,1077.75204183279,
321.906790796576));
#109054=CARTESIAN_POINT('Ctrl Pts',(-16.3607870364596,1077.7597522867,321.967387962371));
#109055=CARTESIAN_POINT('Ctrl Pts',(-16.1444952563454,1077.76988030395,
322.037099431661));
#109056=CARTESIAN_POINT('Ctrl Pts',(-16.0469166395223,1077.77306540288,
322.054591994785));
#109057=CARTESIAN_POINT('Ctrl Pts',(-15.9326289447255,1077.77526457008,
322.059482198915));
#109058=CARTESIAN_POINT('Ctrl Pts',(-15.9169672284338,1077.77553299816,
322.059817014206));
#109059=CARTESIAN_POINT('Ctrl Pts',(-15.901306121126,1077.7757685569,322.059817014206));
#109060=CARTESIAN_POINT('',(-5.22978306525612,1078.42681724135,329.304317191978));
#109061=CARTESIAN_POINT('',(-5.22978306525612,1078.26387343671,326.753428949706));
#109062=CARTESIAN_POINT('Ctrl Pts',(-5.22978306525612,1078.42681724135,
329.304317191978));
#109063=CARTESIAN_POINT('Ctrl Pts',(-5.21817028911033,1078.42685380516,
329.304317191978));
#109064=CARTESIAN_POINT('Ctrl Pts',(-5.20655679442347,1078.42688114565,
329.304158592439));
#109065=CARTESIAN_POINT('Ctrl Pts',(-5.16100430481912,1078.42695218218,
329.302913916183));
#109066=CARTESIAN_POINT('Ctrl Pts',(-5.12711338286783,1078.42692617242,
329.300631508059));
#109067=CARTESIAN_POINT('Ctrl Pts',(-5.05124102899184,1078.42669038787,
329.292468925888));
#109068=CARTESIAN_POINT('Ctrl Pts',(-5.00938046874832,1078.42643689142,
329.285843363698));
#109069=CARTESIAN_POINT('Ctrl Pts',(-4.88956556139944,1078.42535139762,
329.260709366201));
#109070=CARTESIAN_POINT('Ctrl Pts',(-4.81293064865789,1078.42420795463,
329.236929669119));
#109071=CARTESIAN_POINT('Ctrl Pts',(-4.58266992306639,1078.41932324785,
329.140944099275));
#109072=CARTESIAN_POINT('Ctrl Pts',(-4.44089376022422,1078.41415833089,
329.045277202033));
#109073=CARTESIAN_POINT('Ctrl Pts',(-4.22049158176406,1078.40154118619,
328.821942320666));
#109074=CARTESIAN_POINT('Ctrl Pts',(-4.13725339237452,1078.39462432085,
328.702654126653));
#109075=CARTESIAN_POINT('Ctrl Pts',(-4.00946950365154,1078.37842387353,
328.431156616306));
#109076=CARTESIAN_POINT('Ctrl Pts',(-3.96953530824098,1078.36912992539,
328.279370354261));
#109077=CARTESIAN_POINT('Ctrl Pts',(-3.94541827194013,1078.34887201492,
327.957567159541));
#109078=CARTESIAN_POINT('Ctrl Pts',(-3.96579539791426,1078.33802728437,
327.790103478902));
#109079=CARTESIAN_POINT('Ctrl Pts',(-4.07008338707345,1078.31687148192,
327.472173835751));
#109080=CARTESIAN_POINT('Ctrl Pts',(-4.1531559897116,1078.30676709278,327.324797726721));
#109081=CARTESIAN_POINT('Ctrl Pts',(-4.36504731564363,1078.2893987037,327.078184844938));
#109082=CARTESIAN_POINT('Ctrl Pts',(-4.4890086736669,1078.28215286931,326.978698259012));
#109083=CARTESIAN_POINT('Ctrl Pts',(-4.74619433616403,1078.27175416546,
326.841074725353));
#109084=CARTESIAN_POINT('Ctrl Pts',(-4.87363484038006,1078.2682171669,326.796842524499));
#109085=CARTESIAN_POINT('Ctrl Pts',(-5.06037098935054,1078.26520873547,
326.763508636248));
#109086=CARTESIAN_POINT('Ctrl Pts',(-5.11567564599099,1078.26457242965,
326.75732766106));
#109087=CARTESIAN_POINT('Ctrl Pts',(-5.19071540936995,1078.26405133643,
326.753877890726));
#109088=CARTESIAN_POINT('Ctrl Pts',(-5.21023951006827,1078.26394686982,
326.753429205568));
#109089=CARTESIAN_POINT('Ctrl Pts',(-5.22976636012611,1078.26387349947,
326.753428949815));
#109090=CARTESIAN_POINT('Ctrl Pts',(-5.22977192850314,1078.26387347855,
326.753428949742));
#109091=CARTESIAN_POINT('Ctrl Pts',(-5.22977749687982,1078.26387345763,
326.753428949706));
#109092=CARTESIAN_POINT('Ctrl Pts',(-5.22978306525612,1078.26387343671,
326.753428949706));
#109093=CARTESIAN_POINT('Ctrl Pts',(-5.22978306525612,1078.26387343671,
326.753428949706));
#109094=CARTESIAN_POINT('Ctrl Pts',(-5.26413051380193,1078.26374441052,
326.753428949706));
#109095=CARTESIAN_POINT('Ctrl Pts',(-5.29846403555081,1078.2637116895,326.754816403494));
#109096=CARTESIAN_POINT('Ctrl Pts',(-5.37080486946607,1078.26384626869,
326.76067274049));
#109097=CARTESIAN_POINT('Ctrl Pts',(-5.40875149683686,1078.26403652857,
326.765469161249));
#109098=CARTESIAN_POINT('Ctrl Pts',(-5.50662085947742,1078.26483892336,
326.782337964163));
#109099=CARTESIAN_POINT('Ctrl Pts',(-5.56599011321287,1078.26563428291,
326.797023720027));
#109100=CARTESIAN_POINT('Ctrl Pts',(-5.78523386914472,1078.26974517431,
326.868291820281));
#109101=CARTESIAN_POINT('Ctrl Pts',(-5.9342881382041,1078.27499041673,326.952254384132));
#109102=CARTESIAN_POINT('Ctrl Pts',(-6.16926264670932,1078.28795185216,
327.154811053109));
#109103=CARTESIAN_POINT('Ctrl Pts',(-6.2599594072838,1078.29501218834,327.263813377943));
#109104=CARTESIAN_POINT('Ctrl Pts',(-6.40771546101825,1078.31141118208,
327.516664664636));
#109105=CARTESIAN_POINT('Ctrl Pts',(-6.4603254996497,1078.32075416327,327.660596885459));
#109106=CARTESIAN_POINT('Ctrl Pts',(-6.51426724469931,1078.34078303726,
327.970781555767));
#109107=CARTESIAN_POINT('Ctrl Pts',(-6.51118729517371,1078.35133351777,
328.135087825742));
#109108=CARTESIAN_POINT('Ctrl Pts',(-6.44221485146335,1078.37200493712,
328.459169753573));
#109109=CARTESIAN_POINT('Ctrl Pts',(-6.37482210851326,1078.38189816543,
328.615442749315));
#109110=CARTESIAN_POINT('Ctrl Pts',(-6.18661499244605,1078.39911311341,
328.887712488775));
#109111=CARTESIAN_POINT('Ctrl Pts',(-6.06956520407042,1078.40636287919,
329.00249266118));
#109112=CARTESIAN_POINT('Ctrl Pts',(-5.79905642962203,1078.41785859816,
329.18165742599));
#109113=CARTESIAN_POINT('Ctrl Pts',(-5.64820140192462,1078.42201395796,
329.24457695622));
#109114=CARTESIAN_POINT('Ctrl Pts',(-5.42983885156224,1078.42535425019,
329.29000668505));
#109115=CARTESIAN_POINT('Ctrl Pts',(-5.36928719555942,1078.42601802146,
329.298132529575));
#109116=CARTESIAN_POINT('Ctrl Pts',(-5.28221266556542,1078.42660514664,
329.303508871083));
#109117=CARTESIAN_POINT('Ctrl Pts',(-5.25599969646798,1078.42673469605,
329.304317191978));
#109118=CARTESIAN_POINT('Ctrl Pts',(-5.22978306525612,1078.42681724135,
329.304317191978));
#109119=CARTESIAN_POINT('',(-63.8195601713291,1078.69713855509,363.267501886));
#109120=CARTESIAN_POINT('',(-63.8195601713292,1078.64371919106,360.310895621613));
#109121=CARTESIAN_POINT('Ctrl Pts',(-63.8195601713295,1078.69713855509,
363.267501886));
#109122=CARTESIAN_POINT('Ctrl Pts',(-63.7654276633616,1078.69791571789,
363.267501886));
#109123=CARTESIAN_POINT('Ctrl Pts',(-63.7112348515189,1078.69863923751,
363.264528627404));
#109124=CARTESIAN_POINT('Ctrl Pts',(-63.4806174827022,1078.70150018512,
363.239050330233));
#109125=CARTESIAN_POINT('Ctrl Pts',(-63.3089585971147,1078.70308592287,
363.187855743175));
#109126=CARTESIAN_POINT('Ctrl Pts',(-63.0679262643324,1078.70464054456,
363.065522553551));
#109127=CARTESIAN_POINT('Ctrl Pts',(-62.9894676807408,1078.70501590417,
363.015943494998));
#109128=CARTESIAN_POINT('Ctrl Pts',(-62.8854962694621,1078.70533108872,
362.93567418569));
#109129=CARTESIAN_POINT('Ctrl Pts',(-62.8557706289723,1078.70539704784,
362.910800739169));
#109130=CARTESIAN_POINT('Ctrl Pts',(-62.8093656128901,1078.70546021498,
362.868762052048));
#109131=CARTESIAN_POINT('Ctrl Pts',(-62.7920654939823,1078.70547408166,
362.852309589674));
#109132=CARTESIAN_POINT('Ctrl Pts',(-62.75703720122,1078.70548167737,362.817343499119));
#109133=CARTESIAN_POINT('Ctrl Pts',(-62.7393767376307,1078.7054738528,362.798773133657));
#109134=CARTESIAN_POINT('Ctrl Pts',(-62.6993218465886,1078.70542815254,
362.754399674498));
#109135=CARTESIAN_POINT('Ctrl Pts',(-62.6773213699519,1078.70538115641,
362.728260646393));
#109136=CARTESIAN_POINT('Ctrl Pts',(-62.6108179918521,1078.70516671703,
362.643448501102));
#109137=CARTESIAN_POINT('Ctrl Pts',(-62.5697813447945,1078.7049233308,362.582201324117));
#109138=CARTESIAN_POINT('Ctrl Pts',(-62.4364456959654,1078.7036670757,362.346959598677));
#109139=CARTESIAN_POINT('Ctrl Pts',(-62.3745670561911,1078.70206695397,
362.15810698534));
#109140=CARTESIAN_POINT('Ctrl Pts',(-62.3323635444361,1078.69778702226,
361.800995099826));
#109141=CARTESIAN_POINT('Ctrl Pts',(-62.3401009842014,1078.69536514556,
361.637248430636));
#109142=CARTESIAN_POINT('Ctrl Pts',(-62.4115686960024,1078.68929087543,
361.305268495352));
#109143=CARTESIAN_POINT('Ctrl Pts',(-62.4794658479006,1078.68559525106,
361.140531861869));
#109144=CARTESIAN_POINT('Ctrl Pts',(-62.6772734345405,1078.67699749055,
360.831790216029));
#109145=CARTESIAN_POINT('Ctrl Pts',(-62.8095880196696,1078.67210256283,
360.693114562129));
#109146=CARTESIAN_POINT('Ctrl Pts',(-63.0788830265797,1078.66328791611,
360.502172178049));
#109147=CARTESIAN_POINT('Ctrl Pts',(-63.2042216726988,1078.65949595976,
360.437755469273));
#109148=CARTESIAN_POINT('Ctrl Pts',(-63.4920519938876,1078.65148884259,
360.338296316964));
#109149=CARTESIAN_POINT('Ctrl Pts',(-63.655229864875,1078.64736986489,360.310895621613));
#109150=CARTESIAN_POINT('Ctrl Pts',(-63.8195601713292,1078.64371919106,
360.310895621613));
#109151=CARTESIAN_POINT('Ctrl Pts',(-63.8195601713292,1078.64371919106,
360.310895621613));
#109152=CARTESIAN_POINT('Ctrl Pts',(-63.8195692561662,1078.64371898923,
360.310895621613));
#109153=CARTESIAN_POINT('Ctrl Pts',(-63.8195783410068,1078.64371878741,
360.310895621697));
#109154=CARTESIAN_POINT('Ctrl Pts',(-63.8195874258508,1078.64371858559,
360.310895621865));
#109155=CARTESIAN_POINT('Ctrl Pts',(-63.9840880711053,1078.64006418243,
360.310898654657));
#109156=CARTESIAN_POINT('Ctrl Pts',(-64.1474517009238,1078.63693314233,
360.338359260013));
#109157=CARTESIAN_POINT('Ctrl Pts',(-64.4375133454174,1078.63248761909,
360.438719377146));
#109158=CARTESIAN_POINT('Ctrl Pts',(-64.5646686302155,1078.63100970962,
360.504489606167));
#109159=CARTESIAN_POINT('Ctrl Pts',(-64.7189171915552,1078.629931692,360.61498571193));
#109160=CARTESIAN_POINT('Ctrl Pts',(-64.7560402577428,1078.62973704016,
360.644373691614));
#109161=CARTESIAN_POINT('Ctrl Pts',(-64.8133214071306,1078.62954551884,
360.694373110903));
#109162=CARTESIAN_POINT('Ctrl Pts',(-64.834398153059,1078.62950100695,360.713880913424));
#109163=CARTESIAN_POINT('Ctrl Pts',(-64.8731921848538,1078.62946960111,
360.751944240303));
#109164=CARTESIAN_POINT('Ctrl Pts',(-64.8910208318981,1078.62947704798,
360.77037129156));
#109165=CARTESIAN_POINT('Ctrl Pts',(-64.9300915095018,1078.6295439517,360.812913778697));
#109166=CARTESIAN_POINT('Ctrl Pts',(-64.95104463411,1078.62961608288,360.83727695762));
#109167=CARTESIAN_POINT('Ctrl Pts',(-65.0104012958941,1078.62993090917,
360.911025018266));
#109168=CARTESIAN_POINT('Ctrl Pts',(-65.046483463865,1078.63027019649,360.962185601849));
#109169=CARTESIAN_POINT('Ctrl Pts',(-65.1824629782876,1078.63220921242,
361.183566658344));
#109170=CARTESIAN_POINT('Ctrl Pts',(-65.251019535922,1078.63493719135,361.370621080719));
#109171=CARTESIAN_POINT('Ctrl Pts',(-65.3051133582954,1078.64163702058,
361.724127004683));
#109172=CARTESIAN_POINT('Ctrl Pts',(-65.3034107922253,1078.64523224278,
361.885549877209));
#109173=CARTESIAN_POINT('Ctrl Pts',(-65.2458716339885,1078.65347084342,
362.215021809456));
#109174=CARTESIAN_POINT('Ctrl Pts',(-65.1858599118924,1078.65810944785,
362.379885969386));
#109175=CARTESIAN_POINT('Ctrl Pts',(-65.0049667573119,1078.6678008815,362.691988432195));
#109176=CARTESIAN_POINT('Ctrl Pts',(-64.8816256635728,1078.67276841009,
362.834300953678));
#109177=CARTESIAN_POINT('Ctrl Pts',(-64.581690312079,1078.68223685099,363.070876817612));
#109178=CARTESIAN_POINT('Ctrl Pts',(-64.4058332189708,1078.68661220443,
363.16026913069));
#109179=CARTESIAN_POINT('Ctrl Pts',(-64.0878422058905,1078.69295053254,
363.249192272456));
#109180=CARTESIAN_POINT('Ctrl Pts',(-63.9538868561519,1078.69521007057,
363.267501886));
#109181=CARTESIAN_POINT('Ctrl Pts',(-63.8195601713295,1078.69713855509,
363.267501886));
#109182=CARTESIAN_POINT('',(-75.2807843499775,1078.39877300636,365.149931275707));
#109183=CARTESIAN_POINT('',(-75.2807843499774,1078.29624496504,362.599043033435));
#109184=CARTESIAN_POINT('Ctrl Pts',(-75.2807843499775,1078.39877300636,
365.149931275707));
#109185=CARTESIAN_POINT('Ctrl Pts',(-75.2161334842683,1078.40181327285,
365.149931275707));
#109186=CARTESIAN_POINT('Ctrl Pts',(-75.1514247503078,1078.4046523139,365.145015809985));
#109187=CARTESIAN_POINT('Ctrl Pts',(-74.9448585872546,1078.41307129843,
365.113299692974));
#109188=CARTESIAN_POINT('Ctrl Pts',(-74.8071834118907,1078.41769218236,
365.067477827383));
#109189=CARTESIAN_POINT('Ctrl Pts',(-74.5863101850922,1078.42343536425,
364.949549063762));
#109190=CARTESIAN_POINT('Ctrl Pts',(-74.499171623296,1078.42513500621,364.887965809381));
#109191=CARTESIAN_POINT('Ctrl Pts',(-74.3939533568889,1078.42639080928,
364.791873924468));
#109192=CARTESIAN_POINT('Ctrl Pts',(-74.3682783039198,1078.42662066959,
364.766339436608));
#109193=CARTESIAN_POINT('Ctrl Pts',(-74.3285856758789,1078.4268475706,364.723353057851));
#109194=CARTESIAN_POINT('Ctrl Pts',(-74.3138804217284,1078.42690004791,
364.706564336766));
#109195=CARTESIAN_POINT('Ctrl Pts',(-74.2867342554265,1078.42693505528,
364.67388008605));
#109196=CARTESIAN_POINT('Ctrl Pts',(-74.2742153451122,1078.42692380994,
364.658058138182));
#109197=CARTESIAN_POINT('Ctrl Pts',(-74.2466507018341,1078.42683500453,
364.621469458007));
#109198=CARTESIAN_POINT('Ctrl Pts',(-74.2318453978593,1078.42674032876,
364.600532622343));
#109199=CARTESIAN_POINT('Ctrl Pts',(-74.1894275609345,1078.42632234112,
364.536539413027));
#109200=CARTESIAN_POINT('Ctrl Pts',(-74.1637638132263,1078.42586570789,
364.492255420951));
#109201=CARTESIAN_POINT('Ctrl Pts',(-74.0648826593169,1078.4231351608,364.295214661423));
#109202=CARTESIAN_POINT('Ctrl Pts',(-74.0198471130781,1078.41913258796,
364.130296520653));
#109203=CARTESIAN_POINT('Ctrl Pts',(-73.99889279747,1078.40868075344,363.823672373705));
#109204=CARTESIAN_POINT('Ctrl Pts',(-74.0119178471483,1078.40288387041,
363.685322336896));
#109205=CARTESIAN_POINT('Ctrl Pts',(-74.0849456862005,1078.38880697799,
363.40606661576));
#109206=CARTESIAN_POINT('Ctrl Pts',(-74.148560344525,1078.38045633396,363.268277557071));
#109207=CARTESIAN_POINT('Ctrl Pts',(-74.3273946189254,1078.36171230716,
363.011895031162));
#109208=CARTESIAN_POINT('Ctrl Pts',(-74.4445747218407,1078.3513780663,362.897882325637));
#109209=CARTESIAN_POINT('Ctrl Pts',(-74.6771585021235,1078.33348783158,
362.744913697328));
#109210=CARTESIAN_POINT('Ctrl Pts',(-74.7826914890141,1078.32605355494,
362.694568377246));
#109211=CARTESIAN_POINT('Ctrl Pts',(-75.0187524433123,1078.31080177787,
362.619356602734));
#109212=CARTESIAN_POINT('Ctrl Pts',(-75.1493582059871,1078.3031483309,362.599043033435));
#109213=CARTESIAN_POINT('Ctrl Pts',(-75.2807843499774,1078.29624496504,
362.599043033435));
#109214=CARTESIAN_POINT('Ctrl Pts',(-75.2807843499774,1078.29624496504,
362.599043033435));
#109215=CARTESIAN_POINT('Ctrl Pts',(-75.2808246059088,1078.29624285053,
362.599043033435));
#109216=CARTESIAN_POINT('Ctrl Pts',(-75.2808648619172,1078.29624073609,
362.599043035341));
#109217=CARTESIAN_POINT('Ctrl Pts',(-75.2809051180025,1078.29623862173,
362.599043039152));
#109218=CARTESIAN_POINT('Ctrl Pts',(-75.4339110658859,1078.28820230906,
362.599057526832));
#109219=CARTESIAN_POINT('Ctrl Pts',(-75.585730203367,1078.28130554178,362.626604428352));
#109220=CARTESIAN_POINT('Ctrl Pts',(-75.8700236650462,1078.2707025985,362.733338630975));
#109221=CARTESIAN_POINT('Ctrl Pts',(-76.0005275537089,1078.26703110392,
362.810806746118));
#109222=CARTESIAN_POINT('Ctrl Pts',(-76.1462977818729,1078.26464543997,
362.936719743162));
#109223=CARTESIAN_POINT('Ctrl Pts',(-76.1767035716881,1078.26426694338,
362.965724159803));
#109224=CARTESIAN_POINT('Ctrl Pts',(-76.2221910149657,1078.26389723162,
363.013621316875));
#109225=CARTESIAN_POINT('Ctrl Pts',(-76.2382614055876,1078.26380971888,
363.031531518975));
#109226=CARTESIAN_POINT('Ctrl Pts',(-76.266922221215,1078.26373558589,363.06535133532));
#109227=CARTESIAN_POINT('Ctrl Pts',(-76.279658143114,1078.2637352656,363.081127324293));
#109228=CARTESIAN_POINT('Ctrl Pts',(-76.3066136828094,1078.26380783499,
363.116195714162));
#109229=CARTESIAN_POINT('Ctrl Pts',(-76.3206765016514,1078.26389403413,
363.13559878332));
#109230=CARTESIAN_POINT('Ctrl Pts',(-76.3582619672818,1078.26426397588,
363.190657162071));
#109231=CARTESIAN_POINT('Ctrl Pts',(-76.3805521556505,1078.264649296,363.227113984603));
#109232=CARTESIAN_POINT('Ctrl Pts',(-76.4819965114546,1078.26729100623,
363.413443730654));
#109233=CARTESIAN_POINT('Ctrl Pts',(-76.5325310959413,1078.27168449831,
363.576884398006));
#109234=CARTESIAN_POINT('Ctrl Pts',(-76.5634527382886,1078.28312828969,
363.880752998088));
#109235=CARTESIAN_POINT('Ctrl Pts',(-76.5554686847615,1078.28941049513,
364.017429732933));
#109236=CARTESIAN_POINT('Ctrl Pts',(-76.4939475753043,1078.30441417504,
364.295285570309));
#109237=CARTESIAN_POINT('Ctrl Pts',(-76.4367295223015,1078.31319122092,
364.433596763608));
#109238=CARTESIAN_POINT('Ctrl Pts',(-76.2713754352099,1078.33240509299,
364.693614326351));
#109239=CARTESIAN_POINT('Ctrl Pts',(-76.1611860349923,1078.34274708112,
364.811038803311));
#109240=CARTESIAN_POINT('Ctrl Pts',(-75.8956883837525,1078.36366889432,
365.004618549399));
#109241=CARTESIAN_POINT('Ctrl Pts',(-75.7407077768385,1078.37402253982,
365.076069801023));
#109242=CARTESIAN_POINT('Ctrl Pts',(-75.4792733932657,1078.38895729896,
365.138331357763));
#109243=CARTESIAN_POINT('Ctrl Pts',(-75.3800971557428,1078.39410273021,
365.149931275707));
#109244=CARTESIAN_POINT('Ctrl Pts',(-75.2807843499775,1078.39877300636,
365.149931275707));
#109245=CARTESIAN_POINT('',(-87.6738908373843,1077.72740193357,368.174465786616));
#109246=CARTESIAN_POINT('',(-87.6738908373841,1077.60298376124,365.976803514632));
#109247=CARTESIAN_POINT('Ctrl Pts',(-87.6738908373845,1077.72740193357,
368.174465786616));
#109248=CARTESIAN_POINT('Ctrl Pts',(-87.5573652041762,1077.73724060115,
368.174465786616));
#109249=CARTESIAN_POINT('Ctrl Pts',(-87.4413379559943,1077.74595717174,
368.155929576178));
#109250=CARTESIAN_POINT('Ctrl Pts',(-87.2081865583119,1077.76124290941,
368.079155469716));
#109251=CARTESIAN_POINT('Ctrl Pts',(-87.0940626911965,1077.76738850911,
368.017855331126));
#109252=CARTESIAN_POINT('Ctrl Pts',(-86.937335696392,1077.77366264064,367.894145559585));
#109253=CARTESIAN_POINT('Ctrl Pts',(-86.8859755761865,1077.77523785621,
367.844833744352));
#109254=CARTESIAN_POINT('Ctrl Pts',(-86.8223756947841,1077.77647476621,
367.770661603692));
#109255=CARTESIAN_POINT('Ctrl Pts',(-86.8057648978473,1077.77671665045,
367.749799280664));
#109256=CARTESIAN_POINT('Ctrl Pts',(-86.7796558363558,1077.77695715498,
367.714440349409));
#109257=CARTESIAN_POINT('Ctrl Pts',(-86.7697126380652,1077.7770113458,367.700287154191));
#109258=CARTESIAN_POINT('Ctrl Pts',(-86.7510769658923,1077.77703794975,
367.672383188798));
#109259=CARTESIAN_POINT('Ctrl Pts',(-86.7423476385495,1077.77701505646,
367.658662543958));
#109260=CARTESIAN_POINT('Ctrl Pts',(-86.7227413944098,1077.7768784821,367.626280580748));
#109261=CARTESIAN_POINT('Ctrl Pts',(-86.7121039478821,1077.77673751051,
367.607482510928));
#109262=CARTESIAN_POINT('Ctrl Pts',(-86.6803229937885,1077.77609450137,
367.54724495784));
#109263=CARTESIAN_POINT('Ctrl Pts',(-86.6612545546933,1077.77536423692,
367.504773625786));
#109264=CARTESIAN_POINT('Ctrl Pts',(-86.5937762745918,1077.77115672216,
367.324707375812));
#109265=CARTESIAN_POINT('Ctrl Pts',(-86.5703302700837,1077.76518941578,
367.179463664682));
#109266=CARTESIAN_POINT('Ctrl Pts',(-86.5803643398938,1077.74985083539,
366.914971971357));
#109267=CARTESIAN_POINT('Ctrl Pts',(-86.6041910643592,1077.74139850213,
366.797588014984));
#109268=CARTESIAN_POINT('Ctrl Pts',(-86.6923877389255,1077.7210800103,366.564750883201));
#109269=CARTESIAN_POINT('Ctrl Pts',(-86.7596651934525,1077.70912548192,
366.452342304681));
#109270=CARTESIAN_POINT('Ctrl Pts',(-86.9369203232877,1077.68257914247,
366.24862501908));
#109271=CARTESIAN_POINT('Ctrl Pts',(-87.0482725867131,1077.66808828252,
366.161493284213));
#109272=CARTESIAN_POINT('Ctrl Pts',(-87.2468460860523,1077.64510635443,
366.05978237616));
#109273=CARTESIAN_POINT('Ctrl Pts',(-87.3248097970308,1077.63664740925,
366.030421117856));
#109274=CARTESIAN_POINT('Ctrl Pts',(-87.4931076423008,1077.61951793621,
365.988005314607));
#109275=CARTESIAN_POINT('Ctrl Pts',(-87.5833033350967,1077.61095961518,
365.976803514632));
#109276=CARTESIAN_POINT('Ctrl Pts',(-87.6738908373841,1077.60298376124,
365.976803514632));
#109277=CARTESIAN_POINT('Ctrl Pts',(-87.6738908373841,1077.60298376124,
365.976803514632));
#109278=CARTESIAN_POINT('Ctrl Pts',(-87.6739295858868,1077.60298034959,
365.976803514632));
#109279=CARTESIAN_POINT('Ctrl Pts',(-87.6739683344612,1077.60297693806,
365.976803516681));
#109280=CARTESIAN_POINT('Ctrl Pts',(-87.674007083107,1077.60297352662,365.97680352078));
#109281=CARTESIAN_POINT('Ctrl Pts',(-87.8110948853574,1077.59090431333,
365.976818023346));
#109282=CARTESIAN_POINT('Ctrl Pts',(-87.9471081365583,1077.58034330989,
366.00248659144));
#109283=CARTESIAN_POINT('Ctrl Pts',(-88.2018405975823,1077.56352565653,
366.102358515398));
#109284=CARTESIAN_POINT('Ctrl Pts',(-88.3184445103972,1077.55738583551,
366.175299484557));
#109285=CARTESIAN_POINT('Ctrl Pts',(-88.4570236364598,1077.55249567817,
366.303080205187));
#109286=CARTESIAN_POINT('Ctrl Pts',(-88.4927285909642,1077.55152990991,
366.341030288748));
#109287=CARTESIAN_POINT('Ctrl Pts',(-88.5385533914332,1077.55073137724,
366.397248335192));
#109288=CARTESIAN_POINT('Ctrl Pts',(-88.5510474224014,1077.55056685126,
366.413482333986));
#109289=CARTESIAN_POINT('Ctrl Pts',(-88.5720144121306,1077.55038680279,
366.442361303932));
#109290=CARTESIAN_POINT('Ctrl Pts',(-88.580691801958,1077.55034383564,366.454850385869));
#109291=CARTESIAN_POINT('Ctrl Pts',(-88.5982445402759,1077.55032467677,
366.481267177206));
#109292=CARTESIAN_POINT('Ctrl Pts',(-88.607070691021,1077.55035453155,366.495222885357));
#109293=CARTESIAN_POINT('Ctrl Pts',(-88.6271147213411,1077.5505186285,366.528555878046));
#109294=CARTESIAN_POINT('Ctrl Pts',(-88.638061263345,1077.550686195,366.548087215086));
#109295=CARTESIAN_POINT('Ctrl Pts',(-88.671527076778,1077.55146414451,366.612324198192));
#109296=CARTESIAN_POINT('Ctrl Pts',(-88.691588364216,1077.55236494906,366.658231848467));
#109297=CARTESIAN_POINT('Ctrl Pts',(-88.7575613918226,1077.55728181453,
366.842552617564));
#109298=CARTESIAN_POINT('Ctrl Pts',(-88.7788484232324,1077.56391245768,
366.98805397235));
#109299=CARTESIAN_POINT('Ctrl Pts',(-88.7649366627409,1077.58057374157,
367.252513441476));
#109300=CARTESIAN_POINT('Ctrl Pts',(-88.7393088371827,1077.58966347007,
367.369749958813));
#109301=CARTESIAN_POINT('Ctrl Pts',(-88.6475228088464,1077.61114894308,
367.601344363622));
#109302=CARTESIAN_POINT('Ctrl Pts',(-88.5785904850142,1077.62360235186,
367.712662757938));
#109303=CARTESIAN_POINT('Ctrl Pts',(-88.3985567348636,1077.65075882583,
367.913390194743));
#109304=CARTESIAN_POINT('Ctrl Pts',(-88.2862066369907,1077.66532082558,
367.998694712242));
#109305=CARTESIAN_POINT('Ctrl Pts',(-88.0304113322889,1077.6944116005,368.125164019262));
#109306=CARTESIAN_POINT('Ctrl Pts',(-87.8883136821735,1077.70863675563,
368.163152580909));
#109307=CARTESIAN_POINT('Ctrl Pts',(-87.7198685969776,1077.72347788553,
368.173744969849));
#109308=CARTESIAN_POINT('Ctrl Pts',(-87.6968700256675,1077.72546172017,
368.174465786616));
#109309=CARTESIAN_POINT('Ctrl Pts',(-87.6738908373845,1077.72740193357,
368.174465786616));
#109310=CARTESIAN_POINT('',(-99.195671242928,1076.88734730071,373.742997844246));
#109311=CARTESIAN_POINT('',(-99.1956712429287,1076.75143050179,371.56191634679));
#109312=CARTESIAN_POINT('Ctrl Pts',(-99.1956712429275,1076.88734730071,
373.742997844247));
#109313=CARTESIAN_POINT('Ctrl Pts',(-99.0736283223645,1076.90169935678,
373.742997844247));
#109314=CARTESIAN_POINT('Ctrl Pts',(-98.9521493125783,1076.91466858142,
373.722510530752));
#109315=CARTESIAN_POINT('Ctrl Pts',(-98.722881029104,1076.93655311003,373.642505437814));
#109316=CARTESIAN_POINT('Ctrl Pts',(-98.6165758032035,1076.94538160664,
373.584362543656));
#109317=CARTESIAN_POINT('Ctrl Pts',(-98.4429100659212,1076.9572595498,373.447884683702));
#109318=CARTESIAN_POINT('Ctrl Pts',(-98.3728788279871,1076.96096862298,
373.375223966441));
#109319=CARTESIAN_POINT('Ctrl Pts',(-98.2965085693078,1076.9634476614,373.270232018967));
#109320=CARTESIAN_POINT('Ctrl Pts',(-98.2802183338221,1076.96385410401,
373.245825099279));
#109321=CARTESIAN_POINT('Ctrl Pts',(-98.2559131695869,1076.96425457554,
373.20602127878));
#109322=CARTESIAN_POINT('Ctrl Pts',(-98.2472480318087,1076.96434931847,
373.191040397767));
#109323=CARTESIAN_POINT('Ctrl Pts',(-98.231787152459,1076.96442531798,373.162779421882));
#109324=CARTESIAN_POINT('Ctrl Pts',(-98.2249003947043,1076.96442045692,
373.149554043209));
#109325=CARTESIAN_POINT('Ctrl Pts',(-98.2102834705255,1076.96432123289,
373.120020590978));
#109326=CARTESIAN_POINT('Ctrl Pts',(-98.2026826917412,1076.96420828855,
373.103653720111));
#109327=CARTESIAN_POINT('Ctrl Pts',(-98.1821750046192,1076.9637193216,373.056463076137));
#109328=CARTESIAN_POINT('Ctrl Pts',(-98.1702749096861,1076.96320143812,
373.025227000313));
#109329=CARTESIAN_POINT('Ctrl Pts',(-98.1147448066343,1076.95939190168,
372.856565076093));
#109330=CARTESIAN_POINT('Ctrl Pts',(-98.0973062481845,1076.95263957393,
372.712199361141));
#109331=CARTESIAN_POINT('Ctrl Pts',(-98.1172160193176,1076.93453988868,
372.453536329503));
#109332=CARTESIAN_POINT('Ctrl Pts',(-98.1443316171273,1076.9244749459,372.340607577463));
#109333=CARTESIAN_POINT('Ctrl Pts',(-98.2373238720896,1076.89985498333,
372.116712072768));
#109334=CARTESIAN_POINT('Ctrl Pts',(-98.3062049072568,1076.88513007261,
372.008858521594));
#109335=CARTESIAN_POINT('Ctrl Pts',(-98.4848473774606,1076.85201772236,
371.814063640996));
#109336=CARTESIAN_POINT('Ctrl Pts',(-98.5960196878507,1076.83370852677,
371.7312893177));
#109337=CARTESIAN_POINT('Ctrl Pts',(-98.7912365215574,1076.80456118302,
371.6365529696));
#109338=CARTESIAN_POINT('Ctrl Pts',(-98.8665380857841,1076.79389477705,
371.609717639631));
#109339=CARTESIAN_POINT('Ctrl Pts',(-99.0264816047437,1076.77237825944,
371.571799441588));
#109340=CARTESIAN_POINT('Ctrl Pts',(-99.1109041596281,1076.76162623678,
371.56191634679));
#109341=CARTESIAN_POINT('Ctrl Pts',(-99.1956712429287,1076.75143050179,
371.56191634679));
#109342=CARTESIAN_POINT('Ctrl Pts',(-99.1956712429287,1076.75143050179,
371.56191634679));
#109343=CARTESIAN_POINT('Ctrl Pts',(-99.1957283200062,1076.75142363659,
371.56191634679));
#109344=CARTESIAN_POINT('Ctrl Pts',(-99.19578539724,1076.75141677165,371.561916351271));
#109345=CARTESIAN_POINT('Ctrl Pts',(-99.1958424746294,1076.75140990695,
371.561916360233));
#109346=CARTESIAN_POINT('Ctrl Pts',(-99.3351577757383,1076.73465446801,
371.561938234883));
#109347=CARTESIAN_POINT('Ctrl Pts',(-99.4734071019285,1076.71964185485,
371.588656038097));
#109348=CARTESIAN_POINT('Ctrl Pts',(-99.7161381234471,1076.6964459697,371.686404254856));
#109349=CARTESIAN_POINT('Ctrl Pts',(-99.82094661711,1076.68780253686,371.750652243197));
#109350=CARTESIAN_POINT('Ctrl Pts',(-99.9771424816468,1076.6775001339,371.887061624022));
#109351=CARTESIAN_POINT('Ctrl Pts',(-100.034523423316,1076.67455483639,
371.950410338995));
#109352=CARTESIAN_POINT('Ctrl Pts',(-100.1000822094,1076.67244457439,372.042463658499));
#109353=CARTESIAN_POINT('Ctrl Pts',(-100.115331214849,1076.67207043337,
372.065705922058));
#109354=CARTESIAN_POINT('Ctrl Pts',(-100.138383581076,1076.67170327283,
372.103952707521));
#109355=CARTESIAN_POINT('Ctrl Pts',(-100.146754284508,1076.67161830542,
372.118598798295));
#109356=CARTESIAN_POINT('Ctrl Pts',(-100.161250809849,1076.6715620031,372.145387118025));
#109357=CARTESIAN_POINT('Ctrl Pts',(-100.167495537484,1076.6715718107,372.157460731202));
#109358=CARTESIAN_POINT('Ctrl Pts',(-100.181620096997,1076.67167681144,
372.186067440803));
#109359=CARTESIAN_POINT('Ctrl Pts',(-100.189312206167,1076.67180045741,
372.202688202966));
#109360=CARTESIAN_POINT('Ctrl Pts',(-100.210170193117,1076.67233665881,
372.250907092201));
#109361=CARTESIAN_POINT('Ctrl Pts',(-100.222270579505,1076.67290660126,
372.282938726163));
#109362=CARTESIAN_POINT('Ctrl Pts',(-100.27746691294,1076.67702211819,372.452827331005));
#109363=CARTESIAN_POINT('Ctrl Pts',(-100.294314900092,1076.68419817679,
372.597502874207));
#109364=CARTESIAN_POINT('Ctrl Pts',(-100.273215784234,1076.70320477396,
372.856203967397));
#109365=CARTESIAN_POINT('Ctrl Pts',(-100.245620991406,1076.71370265287,
372.968918041803));
#109366=CARTESIAN_POINT('Ctrl Pts',(-100.151825362005,1076.73914601096,
373.192033923503));
#109367=CARTESIAN_POINT('Ctrl Pts',(-100.082694943572,1076.75424225081,
373.299359770525));
#109368=CARTESIAN_POINT('Ctrl Pts',(-99.9039546807303,1076.78783535912,
373.492907388989));
#109369=CARTESIAN_POINT('Ctrl Pts',(-99.7929994064649,1076.80622551015,
373.575057070781));
#109370=CARTESIAN_POINT('Ctrl Pts',(-99.5389909591353,1076.84405296943,
373.697690927404));
#109371=CARTESIAN_POINT('Ctrl Pts',(-99.3967539688833,1076.8631299079,373.734129799356));
#109372=CARTESIAN_POINT('Ctrl Pts',(-99.2328506581823,1076.88294455326,
373.742522852492));
#109373=CARTESIAN_POINT('Ctrl Pts',(-99.2142544122992,1076.88516194913,
373.742997844247));
#109374=CARTESIAN_POINT('Ctrl Pts',(-99.1956712429275,1076.88734730071,
373.742997844247));
#109375=CARTESIAN_POINT('',(-75.4882582191906,1078.69210669589,377.909343604465));
#109376=CARTESIAN_POINT('',(-75.4882582209909,1078.65110559495,374.952737340079));
#109377=CARTESIAN_POINT('Ctrl Pts',(-75.4882582191907,1078.69210669589,
377.909343604465));
#109378=CARTESIAN_POINT('Ctrl Pts',(-75.3723553642364,1078.69420613881,
377.909343604465));
#109379=CARTESIAN_POINT('Ctrl Pts',(-75.256587670448,1078.69606590151,377.895712558815));
#109380=CARTESIAN_POINT('Ctrl Pts',(-74.9775322007986,1078.70004877863,
377.828761931101));
#109381=CARTESIAN_POINT('Ctrl Pts',(-74.8198153044357,1078.70185771599,
377.760572053417));
#109382=CARTESIAN_POINT('Ctrl Pts',(-74.5678748243461,1078.70412727041,
377.595247777887));
#109383=CARTESIAN_POINT('Ctrl Pts',(-74.4685339332241,1078.70479436216,
377.509301780905));
#109384=CARTESIAN_POINT('Ctrl Pts',(-74.3531109587763,1078.70527726789,
377.379034307612));
#109385=CARTESIAN_POINT('Ctrl Pts',(-74.3258568093545,1078.70536357389,
377.345411616369));
#109386=CARTESIAN_POINT('Ctrl Pts',(-74.2844809867876,1078.70544845401,
377.289522297816));
#109387=CARTESIAN_POINT('Ctrl Pts',(-74.269411432456,1078.7054681463,377.267989205266));
#109388=CARTESIAN_POINT('Ctrl Pts',(-74.2419697761637,1078.70548202747,
377.226463216105));
#109389=CARTESIAN_POINT('Ctrl Pts',(-74.2294848941881,1078.70547869262,
377.206554457254));
#109390=CARTESIAN_POINT('Ctrl Pts',(-74.2024030982817,1078.7054488587,377.160990807056));
#109391=CARTESIAN_POINT('Ctrl Pts',(-74.1880892206401,1078.70541666008,
377.135179277233));
#109392=CARTESIAN_POINT('Ctrl Pts',(-74.1480880766633,1078.70527527731,
377.057663016202));
#109393=CARTESIAN_POINT('Ctrl Pts',(-74.1246456264381,1078.70512211053,
377.004863166626));
#109394=CARTESIAN_POINT('Ctrl Pts',(-74.0349484347774,1078.70417865361,
376.766049210628));
#109395=CARTESIAN_POINT('Ctrl Pts',(-74.0032534078389,1078.70276108278,
376.569232269852));
#109396=CARTESIAN_POINT('Ctrl Pts',(-74.0175242273733,1078.69884917058,
376.212092296399));
#109397=CARTESIAN_POINT('Ctrl Pts',(-74.0498438928602,1078.69662979895,
376.054268760415));
#109398=CARTESIAN_POINT('Ctrl Pts',(-74.1689539178824,1078.69098482109,
375.741642429826));
#109399=CARTESIAN_POINT('Ctrl Pts',(-74.259468349416,1078.68750830159,375.590860557683));
#109400=CARTESIAN_POINT('Ctrl Pts',(-74.497478193385,1078.67932032412,375.31796608691));
#109401=CARTESIAN_POINT('Ctrl Pts',(-74.6465874232387,1078.67460612919,
375.201339900436));
#109402=CARTESIAN_POINT('Ctrl Pts',(-74.9872371740712,1078.66449165679,
375.026588823309));
#109403=CARTESIAN_POINT('Ctrl Pts',(-75.1769197320241,1078.65917180238,
374.972762191345));
#109404=CARTESIAN_POINT('Ctrl Pts',(-75.4104491222578,1078.65308609293,
374.954271430745));
#109405=CARTESIAN_POINT('Ctrl Pts',(-75.4493746762025,1078.65208707672,
374.952737339984));
#109406=CARTESIAN_POINT('Ctrl Pts',(-75.4882582227912,1078.65110559495,
374.952737340079));
#109407=CARTESIAN_POINT('Ctrl Pts',(-75.4882582227911,1078.65110559495,
374.952737340079));
#109408=CARTESIAN_POINT('Ctrl Pts',(-75.6377283020281,1078.64733273544,
374.952737340443));
#109409=CARTESIAN_POINT('Ctrl Pts',(-75.7865776407321,1078.64381852535,
374.975408230683));
#109410=CARTESIAN_POINT('Ctrl Pts',(-76.0944769116894,1078.63724511373,
375.071739479389));
#109411=CARTESIAN_POINT('Ctrl Pts',(-76.2489933327613,1078.63439627033,
375.151786494705));
#109412=CARTESIAN_POINT('Ctrl Pts',(-76.4684122859027,1078.63127796722,
375.319559165766));
#109413=CARTESIAN_POINT('Ctrl Pts',(-76.543805534904,1078.63044039654,375.390889675293));
#109414=CARTESIAN_POINT('Ctrl Pts',(-76.6366811080338,1078.62977669572,
375.499349378235));
#109415=CARTESIAN_POINT('Ctrl Pts',(-76.6610334217237,1078.62964561687,
375.530195436815));
#109416=CARTESIAN_POINT('Ctrl Pts',(-76.6991779067036,1078.62951517723,
375.582683817286));
#109417=CARTESIAN_POINT('Ctrl Pts',(-76.7136871158323,1078.62948585624,
375.603780219566));
#109418=CARTESIAN_POINT('Ctrl Pts',(-76.7407966396375,1078.62947201969,
375.645476889364));
#109419=CARTESIAN_POINT('Ctrl Pts',(-76.753454593751,1078.6294850376,375.666030164883));
#109420=CARTESIAN_POINT('Ctrl Pts',(-76.7817762502066,1078.62956133302,
375.714644326584));
#109421=CARTESIAN_POINT('Ctrl Pts',(-76.7970395231866,1078.62963981064,
375.742924332503));
#109422=CARTESIAN_POINT('Ctrl Pts',(-76.8422978146681,1078.62999718961,
375.833742113927));
#109423=CARTESIAN_POINT('Ctrl Pts',(-76.8688209305646,1078.63040263772,
375.897903621101));
#109424=CARTESIAN_POINT('Ctrl Pts',(-76.9385947214267,1078.63218843821,
376.107288762677));
#109425=CARTESIAN_POINT('Ctrl Pts',(-76.9641067637324,1078.63414625799,
376.257382120507));
#109426=CARTESIAN_POINT('Ctrl Pts',(-76.9663927178114,1078.63671295251,
376.408712135129));
#109427=CARTESIAN_POINT('Ctrl Pts',(-76.9687550474511,1078.63936540235,
376.565098207013));
#109428=CARTESIAN_POINT('Ctrl Pts',(-76.9462840670978,1078.64263324409,
376.720862236921));
#109429=CARTESIAN_POINT('Ctrl Pts',(-76.849045006429,1078.65032555411,377.033422833942));
#109430=CARTESIAN_POINT('Ctrl Pts',(-76.7703310052505,1078.65476804806,
377.186613134866));
#109431=CARTESIAN_POINT('Ctrl Pts',(-76.556457741345,1078.66423994707,377.469318337356));
#109432=CARTESIAN_POINT('Ctrl Pts',(-76.4194148317565,1078.66920200388,
377.59380461101));
#109433=CARTESIAN_POINT('Ctrl Pts',(-76.09490818475,1078.67898216859,377.793521966059));
#109434=CARTESIAN_POINT('Ctrl Pts',(-75.9076663876631,1078.6836606122,377.862293621273));
#109435=CARTESIAN_POINT('Ctrl Pts',(-75.638094200845,1078.68929363306,377.903652929645));
#109436=CARTESIAN_POINT('Ctrl Pts',(-75.563147994354,1078.69075015633,377.909343604465));
#109437=CARTESIAN_POINT('Ctrl Pts',(-75.4882582191907,1078.69210669589,
377.909343604465));
#109438=CARTESIAN_POINT('',(-86.2654713137622,1078.38513071259,382.129126937278));
#109439=CARTESIAN_POINT('',(-86.2654713137623,1078.31124838463,379.578238695006));
#109440=CARTESIAN_POINT('Ctrl Pts',(-86.2654713137622,1078.38513071259,
382.129126937278));
#109441=CARTESIAN_POINT('Ctrl Pts',(-86.2621547182598,1078.38531245274,
382.129126937278));
#109442=CARTESIAN_POINT('Ctrl Pts',(-86.2588374878412,1078.38549380858,
382.129114000842));
#109443=CARTESIAN_POINT('Ctrl Pts',(-86.0917677461627,1078.39460656414,
382.127810404116));
#109444=CARTESIAN_POINT('Ctrl Pts',(-85.9297263566369,1078.40242275905,
382.095007511258));
#109445=CARTESIAN_POINT('Ctrl Pts',(-85.6438360470429,1078.41444363147,
381.97684376163));
#109446=CARTESIAN_POINT('Ctrl Pts',(-85.5198491960599,1078.41886952219,
381.898666233538));
#109447=CARTESIAN_POINT('Ctrl Pts',(-85.3396895129841,1078.42398312223,
381.736340881773));
#109448=CARTESIAN_POINT('Ctrl Pts',(-85.2752894839162,1078.42540855029,
381.663436266356));
#109449=CARTESIAN_POINT('Ctrl Pts',(-85.2005866677153,1078.42647054059,
381.556463735536));
#109450=CARTESIAN_POINT('Ctrl Pts',(-85.1824928029337,1078.42666681157,
381.52824781302));
#109451=CARTESIAN_POINT('Ctrl Pts',(-85.1549758939361,1078.42686075099,
381.481370915634));
#109452=CARTESIAN_POINT('Ctrl Pts',(-85.14486345472,1078.42690540145,381.463133765222));
#109453=CARTESIAN_POINT('Ctrl Pts',(-85.1264023958257,1078.42693384648,
381.427826028171));
#109454=CARTESIAN_POINT('Ctrl Pts',(-85.1179792315186,1078.4269227042,381.410800710198));
#109455=CARTESIAN_POINT('Ctrl Pts',(-85.0996305820789,1078.42684091163,
381.371530432162));
#109456=CARTESIAN_POINT('Ctrl Pts',(-85.0899558203568,1078.42675437259,
381.349176585955));
#109457=CARTESIAN_POINT('Ctrl Pts',(-85.0626207109228,1078.42636969245,
381.280702840654));
#109458=CARTESIAN_POINT('Ctrl Pts',(-85.04699321582,1078.42594586249,381.233822948609));
#109459=CARTESIAN_POINT('Ctrl Pts',(-84.9899689914733,1078.42333734463,
381.022628530569));
#109460=CARTESIAN_POINT('Ctrl Pts',(-84.9788404704694,1078.41940782916,
380.851971940393));
#109461=CARTESIAN_POINT('Ctrl Pts',(-85.0196343822102,1078.40909248357,
380.547756161376));
#109462=CARTESIAN_POINT('Ctrl Pts',(-85.0598810465616,1078.4033688104,380.41524168594));
#109463=CARTESIAN_POINT('Ctrl Pts',(-85.1866963815276,1078.38943448825,
380.156840420775));
#109464=CARTESIAN_POINT('Ctrl Pts',(-85.2762164577842,1078.38114900333,
380.034724433226));
#109465=CARTESIAN_POINT('Ctrl Pts',(-85.5018643349163,1078.36251506329,
379.819363290741));
#109466=CARTESIAN_POINT('Ctrl Pts',(-85.6390156033082,1078.35222191958,
379.730984498714));
#109467=CARTESIAN_POINT('Ctrl Pts',(-85.940418487836,1078.33133882896,379.609597495995));
#109468=CARTESIAN_POINT('Ctrl Pts',(-86.1021781226936,1078.32093787104,
379.578238695006));
#109469=CARTESIAN_POINT('Ctrl Pts',(-86.2654713137625,1078.31124838463,
379.578238695006));
#109470=CARTESIAN_POINT('Ctrl Pts',(-86.2654713137625,1078.31124838463,
379.578238695006));
#109471=CARTESIAN_POINT('Ctrl Pts',(-86.265575958347,1078.31124217524,379.578238695006));
#109472=CARTESIAN_POINT('Ctrl Pts',(-86.2656806035614,1078.31123596613,
379.578238707884));
#109473=CARTESIAN_POINT('Ctrl Pts',(-86.2657852494035,1078.31122975733,
379.578238733642));
#109474=CARTESIAN_POINT('Ctrl Pts',(-86.4293026049154,1078.30152800581,
379.578278981526));
#109475=CARTESIAN_POINT('Ctrl Pts',(-86.5913564860174,1078.29272124311,
379.609764341875));
#109476=CARTESIAN_POINT('Ctrl Pts',(-86.8771103923418,1078.27890818754,
379.725167162856));
#109477=CARTESIAN_POINT('Ctrl Pts',(-87.0010080157548,1078.27368093378,
379.801702207554));
#109478=CARTESIAN_POINT('Ctrl Pts',(-87.1845084879564,1078.26743513804,
379.963654487604));
#109479=CARTESIAN_POINT('Ctrl Pts',(-87.2515171654767,1078.26563813562,
380.038514857939));
#109480=CARTESIAN_POINT('Ctrl Pts',(-87.3287326688149,1078.26430944615,
380.148416128401));
#109481=CARTESIAN_POINT('Ctrl Pts',(-87.3472491551574,1078.2640657592,380.177160382035));
#109482=CARTESIAN_POINT('Ctrl Pts',(-87.3753205099728,1078.26382535787,
380.224842683963));
#109483=CARTESIAN_POINT('Ctrl Pts',(-87.3855968713634,1078.26376994913,
380.243335461318));
#109484=CARTESIAN_POINT('Ctrl Pts',(-87.4043122307246,1078.2637340015,380.279080752547));
#109485=CARTESIAN_POINT('Ctrl Pts',(-87.4128308211753,1078.26374701227,
380.2962850005));
#109486=CARTESIAN_POINT('Ctrl Pts',(-87.4313377721645,1078.26384518278,
380.335885408117));
#109487=CARTESIAN_POINT('Ctrl Pts',(-87.4410750434965,1078.26394932319,
380.358390372272));
#109488=CARTESIAN_POINT('Ctrl Pts',(-87.4684632283201,1078.26441083775,
380.427056954226));
#109489=CARTESIAN_POINT('Ctrl Pts',(-87.4840856639928,1078.26491761527,
380.473975241045));
#109490=CARTESIAN_POINT('Ctrl Pts',(-87.5410400556552,1078.26802511368,
380.685231750097));
#109491=CARTESIAN_POINT('Ctrl Pts',(-87.5520988849694,1078.27269527575,
380.855884335518));
#109492=CARTESIAN_POINT('Ctrl Pts',(-87.5112581275218,1078.28461173595,
381.159604267135));
#109493=CARTESIAN_POINT('Ctrl Pts',(-87.4711738678357,1078.29112017793,
381.291665561591));
#109494=CARTESIAN_POINT('Ctrl Pts',(-87.3451063310103,1078.30653492256,
381.549021443521));
#109495=CARTESIAN_POINT('Ctrl Pts',(-87.2562627295294,1078.31548411379,
381.670638991274));
#109496=CARTESIAN_POINT('Ctrl Pts',(-87.0325714922947,1078.33495405235,
381.885231964823));
#109497=CARTESIAN_POINT('Ctrl Pts',(-86.8967577762174,1078.3453682177,381.973509683456));
#109498=CARTESIAN_POINT('Ctrl Pts',(-86.5949453282657,1078.36602661873,
382.096903707261));
#109499=CARTESIAN_POINT('Ctrl Pts',(-86.4309992401525,1078.37606024535,
382.129126937278));
#109500=CARTESIAN_POINT('Ctrl Pts',(-86.2654713137622,1078.38513071259,
382.129126937278));
#109501=CARTESIAN_POINT('',(-97.7222027015963,1077.70670509264,387.660380419275));
#109502=CARTESIAN_POINT('',(-97.7222027015963,1077.62441341004,385.46271814729));
#109503=CARTESIAN_POINT('Ctrl Pts',(-97.7222027015964,1077.70670509264,
387.660380419275));
#109504=CARTESIAN_POINT('Ctrl Pts',(-97.7124019766386,1077.70763427451,
387.660380419275));
#109505=CARTESIAN_POINT('Ctrl Pts',(-97.7025952568283,1077.70855872694,
387.660249297581));
#109506=CARTESIAN_POINT('Ctrl Pts',(-97.5502098697314,1077.72284132834,
387.656168217868));
#109507=CARTESIAN_POINT('Ctrl Pts',(-97.4096043505871,1077.73489851245,
387.624623763402));
#109508=CARTESIAN_POINT('Ctrl Pts',(-97.169800320246,1077.75347129077,387.518884174392));
#109509=CARTESIAN_POINT('Ctrl Pts',(-97.0691998068531,1077.76045188173,
387.453327295383));
#109510=CARTESIAN_POINT('Ctrl Pts',(-96.8984417573925,1077.77065894042,
387.29732888491));
#109511=CARTESIAN_POINT('Ctrl Pts',(-96.8277980615754,1077.77403230899,
387.209634913951));
#109512=CARTESIAN_POINT('Ctrl Pts',(-96.7560163049699,1077.77621092385,
387.085839992693));
#109513=CARTESIAN_POINT('Ctrl Pts',(-96.7415657066971,1077.77655464824,
387.058286804692));
#109514=CARTESIAN_POINT('Ctrl Pts',(-96.7206548707728,1077.77689079151,
387.013935641314));
#109515=CARTESIAN_POINT('Ctrl Pts',(-96.7134051313894,1077.77697027794,
386.997529731309));
#109516=CARTESIAN_POINT('Ctrl Pts',(-96.7013379606228,1077.77703368949,
386.968307491944));
#109517=CARTESIAN_POINT('Ctrl Pts',(-96.6963524665975,1077.77703579725,
386.955564962614));
#109518=CARTESIAN_POINT('Ctrl Pts',(-96.6855323263409,1077.77698284554,
386.926310805474));
#109519=CARTESIAN_POINT('Ctrl Pts',(-96.6798518570805,1077.7769116381,386.909746268716));
#109520=CARTESIAN_POINT('Ctrl Pts',(-96.6655000873494,1077.77660560169,
386.864391191729));
#109521=CARTESIAN_POINT('Ctrl Pts',(-96.6576109506054,1077.77629020174,
386.8353701896));
#109522=CARTESIAN_POINT('Ctrl Pts',(-96.6255902928541,1077.77419968886,
386.695079361964));
#109523=CARTESIAN_POINT('Ctrl Pts',(-96.6176693844983,1077.77082064868,
386.580878045216));
#109524=CARTESIAN_POINT('Ctrl Pts',(-96.6369579713206,1077.76091279066,
386.356221646851));
#109525=CARTESIAN_POINT('Ctrl Pts',(-96.6634347193482,1077.75449907891,
386.247079266533));
#109526=CARTESIAN_POINT('Ctrl Pts',(-96.7530886076295,1077.73818158454,
386.028921411652));
#109527=CARTESIAN_POINT('Ctrl Pts',(-96.8194458346927,1077.728081044,385.922914334021));
#109528=CARTESIAN_POINT('Ctrl Pts',(-96.9915923964205,1077.70471525454,
385.729829840551));
#109529=CARTESIAN_POINT('Ctrl Pts',(-97.0988197627813,1077.69144658987,
385.646725366817));
#109530=CARTESIAN_POINT('Ctrl Pts',(-97.294594857691,1077.66893024175,385.545699458093));
#109531=CARTESIAN_POINT('Ctrl Pts',(-97.3752307887054,1077.66003850054,
385.515409278508));
#109532=CARTESIAN_POINT('Ctrl Pts',(-97.5448000331111,1077.64207747447,
385.473500987036));
#109533=CARTESIAN_POINT('Ctrl Pts',(-97.6333258257655,1077.63307625427,
385.46271814729));
#109534=CARTESIAN_POINT('Ctrl Pts',(-97.7222027015963,1077.62441341004,
385.46271814729));
#109535=CARTESIAN_POINT('Ctrl Pts',(-97.7222027015963,1077.62441341004,
385.46271814729));
#109536=CARTESIAN_POINT('Ctrl Pts',(-97.722261074218,1077.62440772045,385.46271814729));
#109537=CARTESIAN_POINT('Ctrl Pts',(-97.7223194469913,1077.624402031,385.462718151941));
#109538=CARTESIAN_POINT('Ctrl Pts',(-97.7223778199155,1077.62439634171,
385.462718161244));
#109539=CARTESIAN_POINT('Ctrl Pts',(-97.8652491765215,1077.61047143409,
385.46274093034));
#109540=CARTESIAN_POINT('Ctrl Pts',(-98.0068781946763,1077.59763002745,
385.490628024508));
#109541=CARTESIAN_POINT('Ctrl Pts',(-98.2526251510877,1077.57726326324,
385.591451297604));
#109542=CARTESIAN_POINT('Ctrl Pts',(-98.3574907158762,1077.56938264513,
385.656619489785));
#109543=CARTESIAN_POINT('Ctrl Pts',(-98.5370654765183,1077.5576776994,385.815171509941));
#109544=CARTESIAN_POINT('Ctrl Pts',(-98.6118031717629,1077.55375460098,
385.906018887543));
#109545=CARTESIAN_POINT('Ctrl Pts',(-98.6868907005084,1077.55125604196,
386.03446325289));
#109546=CARTESIAN_POINT('Ctrl Pts',(-98.7017513784915,1077.55086778311,
386.062623199424));
#109547=CARTESIAN_POINT('Ctrl Pts',(-98.723157013672,1077.55048929991,386.107840569333));
#109548=CARTESIAN_POINT('Ctrl Pts',(-98.7305347775942,1077.55039988931,
386.124482269751));
#109549=CARTESIAN_POINT('Ctrl Pts',(-98.743363360559,1077.55032428065,386.155475219288));
#109550=CARTESIAN_POINT('Ctrl Pts',(-98.7489333442791,1077.55032408311,
386.169772019185));
#109551=CARTESIAN_POINT('Ctrl Pts',(-98.7604385844994,1077.55039873531,
386.201235696041));
#109552=CARTESIAN_POINT('Ctrl Pts',(-98.7662512061097,1077.55048736267,
386.218442399869));
#109553=CARTESIAN_POINT('Ctrl Pts',(-98.7812747190916,1077.55086882648,
386.266839833452));
#109554=CARTESIAN_POINT('Ctrl Pts',(-98.7895309779033,1077.5512675288,386.298305466541));
#109555=CARTESIAN_POINT('Ctrl Pts',(-98.8256759340566,1077.55417681907,
386.466049416065));
#109556=CARTESIAN_POINT('Ctrl Pts',(-98.8288759317787,1077.55930119417,
386.60624802771));
#109557=CARTESIAN_POINT('Ctrl Pts',(-98.7868430036914,1077.57316200743,
386.856958875455));
#109558=CARTESIAN_POINT('Ctrl Pts',(-98.7500125751257,1077.58104749303,
386.96687578604));
#109559=CARTESIAN_POINT('Ctrl Pts',(-98.6383089138675,1077.60028660184,
387.1814278163));
#109560=CARTESIAN_POINT('Ctrl Pts',(-98.5607974191268,1077.61176563041,
387.282805400229));
#109561=CARTESIAN_POINT('Ctrl Pts',(-98.3674509235807,1077.63739387053,
387.46141342537));
#109562=CARTESIAN_POINT('Ctrl Pts',(-98.2506919031589,1077.65146471467,
387.534575124751));
#109563=CARTESIAN_POINT('Ctrl Pts',(-97.9956721116306,1077.67973475138,
387.63463744473));
#109564=CARTESIAN_POINT('Ctrl Pts',(-97.8595260274799,1077.69368581638,
387.660380419275));
#109565=CARTESIAN_POINT('Ctrl Pts',(-97.7222027015963,1077.70670509264,
387.660380419275));
#109566=CARTESIAN_POINT('',(-107.832717977552,1076.85914687694,395.502558371549));
#109567=CARTESIAN_POINT('',(-107.832717977553,1076.78013798525,393.321476874093));
#109568=CARTESIAN_POINT('Ctrl Pts',(-107.832717977554,1076.85914687694,
395.502558371549));
#109569=CARTESIAN_POINT('Ctrl Pts',(-107.743834231058,1076.87056475884,
395.502558371549));
#109570=CARTESIAN_POINT('Ctrl Pts',(-107.655018492996,1076.88154915174,
395.491691901226));
#109571=CARTESIAN_POINT('Ctrl Pts',(-107.43387654173,1076.90781939257,395.436417944525));
#109572=CARTESIAN_POINT('Ctrl Pts',(-107.306890784662,1076.92186348896,
395.377469040284));
#109573=CARTESIAN_POINT('Ctrl Pts',(-107.093476636667,1076.94345094462,
395.223342404524));
#109574=CARTESIAN_POINT('Ctrl Pts',(-107.005777038169,1076.95136409676,
395.133798552405));
#109575=CARTESIAN_POINT('Ctrl Pts',(-106.89253177196,1076.95985669707,394.969631173146));
#109576=CARTESIAN_POINT('Ctrl Pts',(-106.856466274116,1076.96207863835,
394.903773857406));
#109577=CARTESIAN_POINT('Ctrl Pts',(-106.817521811368,1076.96371792518,
394.811153097107));
#109578=CARTESIAN_POINT('Ctrl Pts',(-106.80844590849,1076.96401800765,394.787249893623));
#109579=CARTESIAN_POINT('Ctrl Pts',(-106.795113727036,1076.96431392295,
394.748035464688));
#109580=CARTESIAN_POINT('Ctrl Pts',(-106.790337528235,1076.96438197428,
394.732912596409));
#109581=CARTESIAN_POINT('Ctrl Pts',(-106.781848225682,1076.96442545441,
394.703839658075));
#109582=CARTESIAN_POINT('Ctrl Pts',(-106.778079011649,1076.96440866751,
394.689909663929));
#109583=CARTESIAN_POINT('Ctrl Pts',(-106.770110157312,1076.96428478801,
394.657956786525));
#109584=CARTESIAN_POINT('Ctrl Pts',(-106.766090668207,1076.96415356652,
394.639893917074));
#109585=CARTESIAN_POINT('Ctrl Pts',(-106.755297954521,1076.96356896599,
394.584819605243));
#109586=CARTESIAN_POINT('Ctrl Pts',(-106.749979223518,1076.96292323385,
394.547555752335));
#109587=CARTESIAN_POINT('Ctrl Pts',(-106.733593452344,1076.95857768857,
394.366099626876));
#109588=CARTESIAN_POINT('Ctrl Pts',(-106.749367551661,1076.95146361364,
394.221115678595));
#109589=CARTESIAN_POINT('Ctrl Pts',(-106.827870156943,1076.93270635441,
393.972584113405));
#109590=CARTESIAN_POINT('Ctrl Pts',(-106.880405833519,1076.92232831509,
393.868095912839));
#109591=CARTESIAN_POINT('Ctrl Pts',(-107.023109630229,1076.89710299884,
393.670291014135));
#109592=CARTESIAN_POINT('Ctrl Pts',(-107.115459687654,1076.88210154595,
393.580703815282));
#109593=CARTESIAN_POINT('Ctrl Pts',(-107.311016879167,1076.85224750454,
393.448212750265));
#109594=CARTESIAN_POINT('Ctrl Pts',(-107.409560626406,1076.83785959358,
393.401074093128));
#109595=CARTESIAN_POINT('Ctrl Pts',(-107.616839334652,1076.80877365399,
393.337595562981));
#109596=CARTESIAN_POINT('Ctrl Pts',(-107.72446400748,1076.79422752107,393.321476874092));
#109597=CARTESIAN_POINT('Ctrl Pts',(-107.832717977553,1076.78013798525,
393.321476874092));
#109598=CARTESIAN_POINT('Ctrl Pts',(-107.832717977553,1076.78013798525,
393.321476874092));
#109599=CARTESIAN_POINT('Ctrl Pts',(-107.832801593366,1076.78012710243,
393.321476874092));
#109600=CARTESIAN_POINT('Ctrl Pts',(-107.832885209555,1076.78011621989,
393.321476883709));
#109601=CARTESIAN_POINT('Ctrl Pts',(-107.832968826119,1076.78010533762,
393.321476902943));
#109602=CARTESIAN_POINT('Ctrl Pts',(-107.976290564888,1076.76145274409,
393.321509870123));
#109603=CARTESIAN_POINT('Ctrl Pts',(-108.118396783563,1076.74390205806,
393.349796213408));
#109604=CARTESIAN_POINT('Ctrl Pts',(-108.371790543568,1076.71452021206,
393.455063317854));
#109605=CARTESIAN_POINT('Ctrl Pts',(-108.48268278115,1076.70255142369,393.526573111447));
#109606=CARTESIAN_POINT('Ctrl Pts',(-108.679563846868,1076.68339274454,
393.711040992627));
#109607=CARTESIAN_POINT('Ctrl Pts',(-108.761872786949,1076.67670331073,
393.824419531492));
#109608=CARTESIAN_POINT('Ctrl Pts',(-108.833425645152,1076.67291107488,
393.977547250601));
#109609=CARTESIAN_POINT('Ctrl Pts',(-108.845007144768,1076.67240572431,
394.005260532755));
#109610=CARTESIAN_POINT('Ctrl Pts',(-108.861958279561,1076.67185991099,
394.051050854009));
#109611=CARTESIAN_POINT('Ctrl Pts',(-108.868028528609,1076.67171637715,
394.068848988473));
#109612=CARTESIAN_POINT('Ctrl Pts',(-108.877981436976,1076.67158017808,
394.100704645584));
#109613=CARTESIAN_POINT('Ctrl Pts',(-108.882047932659,1076.67156084976,
394.114699410081));
#109614=CARTESIAN_POINT('Ctrl Pts',(-108.889968783515,1076.67160443275,
394.144149296745));
#109615=CARTESIAN_POINT('Ctrl Pts',(-108.893767425531,1076.67167513526,
394.159615633152));
#109616=CARTESIAN_POINT('Ctrl Pts',(-108.902759865924,1076.67198347169,
394.200030212478));
#109617=CARTESIAN_POINT('Ctrl Pts',(-108.907420116095,1076.67229571535,
394.225085892644));
#109618=CARTESIAN_POINT('Ctrl Pts',(-108.92319796496,1076.67410833811,394.330294146571));
#109619=CARTESIAN_POINT('Ctrl Pts',(-108.926250240401,1076.67670988062,
394.41135717249));
#109620=CARTESIAN_POINT('Ctrl Pts',(-108.912699057437,1076.68532792927,
394.595688063361));
#109621=CARTESIAN_POINT('Ctrl Pts',(-108.890287560378,1076.69206260374,
394.697665693222));
#109622=CARTESIAN_POINT('Ctrl Pts',(-108.812358953408,1076.71000823363,
394.905534729815));
#109623=CARTESIAN_POINT('Ctrl Pts',(-108.7531963639,1076.72158961181,395.008588695904));
#109624=CARTESIAN_POINT('Ctrl Pts',(-108.597337520389,1076.74906138808,
395.200252715122));
#109625=CARTESIAN_POINT('Ctrl Pts',(-108.498801915667,1076.76504418789,
395.285067420751));
#109626=CARTESIAN_POINT('Ctrl Pts',(-108.268111950518,1076.80003416511,
395.421511062668));
#109627=CARTESIAN_POINT('Ctrl Pts',(-108.135891714292,1076.81887756447,
395.468767126857));
#109628=CARTESIAN_POINT('Ctrl Pts',(-107.943459073455,1076.84475656851,
395.498343392934));
#109629=CARTESIAN_POINT('Ctrl Pts',(-107.888075329727,1076.85203574881,
395.502558371549));
#109630=CARTESIAN_POINT('Ctrl Pts',(-107.832717977554,1076.85914687694,
395.502558371549));
#109631=CARTESIAN_POINT('',(-69.482552265803,1076.93351373127,337.889334626622));
#109632=CARTESIAN_POINT('',(-69.4825522658041,1076.7038426352,335.708253129166));
#109633=CARTESIAN_POINT('Ctrl Pts',(-69.482552265803,1076.93351373127,337.889334626623));
#109634=CARTESIAN_POINT('Ctrl Pts',(-69.4806455417213,1076.93366952156,
337.889334626623));
#109635=CARTESIAN_POINT('Ctrl Pts',(-69.4787385413302,1076.93382481149,
337.88932962599));
#109636=CARTESIAN_POINT('Ctrl Pts',(-69.346539373702,1076.94455372551,337.888636098955));
#109637=CARTESIAN_POINT('Ctrl Pts',(-69.2172598274196,1076.95260563072,
337.864606939716));
#109638=CARTESIAN_POINT('Ctrl Pts',(-69.0345323697271,1076.96033080558,
337.795169885668));
#109639=CARTESIAN_POINT('Ctrl Pts',(-68.9760522862653,1076.96216490022,
337.766755690126));
#109640=CARTESIAN_POINT('Ctrl Pts',(-68.8973961547121,1076.96369723422,
337.719442570328));
#109641=CARTESIAN_POINT('Ctrl Pts',(-68.8748805788767,1076.96401668702,
337.704739224455));
#109642=CARTESIAN_POINT('Ctrl Pts',(-68.8394767011401,1076.9643223835,337.679705018433));
#109643=CARTESIAN_POINT('Ctrl Pts',(-68.8262403690781,1076.96438970002,
337.669888204085));
#109644=CARTESIAN_POINT('Ctrl Pts',(-68.7993083603979,1076.96442783121,
337.64895144849));
#109645=CARTESIAN_POINT('Ctrl Pts',(-68.7856499918525,1076.96439152641,
337.637791696533));
#109646=CARTESIAN_POINT('Ctrl Pts',(-68.7544788172581,1076.96417654368,
337.611036330553));
#109647=CARTESIAN_POINT('Ctrl Pts',(-68.7371870016368,1076.96395496774,
337.595197846194));
#109648=CARTESIAN_POINT('Ctrl Pts',(-68.6843380719293,1076.96294595699,
337.543560937507));
#109649=CARTESIAN_POINT('Ctrl Pts',(-68.6507533009033,1076.96180204728,
337.505852781911));
#109650=CARTESIAN_POINT('Ctrl Pts',(-68.5315759500406,1076.95565567046,
337.351757260213));
#109651=CARTESIAN_POINT('Ctrl Pts',(-68.466915680369,1076.94750167682,337.221291751667));
#109652=CARTESIAN_POINT('Ctrl Pts',(-68.3985533178926,1076.92686613888,
336.967288790625));
#109653=CARTESIAN_POINT('Ctrl Pts',(-68.3866862445795,1076.91552301861,
336.848236154612));
#109654=CARTESIAN_POINT('Ctrl Pts',(-68.4024228070353,1076.88846032279,
336.600061187796));
#109655=CARTESIAN_POINT('Ctrl Pts',(-68.4337617413244,1076.87263894941,
336.473011315067));
#109656=CARTESIAN_POINT('Ctrl Pts',(-68.54369542598,1076.83773329672,336.22653119835));
#109657=CARTESIAN_POINT('Ctrl Pts',(-68.6249506262102,1076.81879473621,
336.110727338302));
#109658=CARTESIAN_POINT('Ctrl Pts',(-68.8156040935837,1076.78344761007,
335.927019151369));
#109659=CARTESIAN_POINT('Ctrl Pts',(-68.9195814222719,1076.76723515419,
335.856497108887));
#109660=CARTESIAN_POINT('Ctrl Pts',(-69.0976118141404,1076.74366830961,
335.776014237312));
#109661=CARTESIAN_POINT('Ctrl Pts',(-69.1646226245242,1076.73558050823,
335.753234972091));
#109662=CARTESIAN_POINT('Ctrl Pts',(-69.3149948320073,1076.71909341971,
335.717949458206));
#109663=CARTESIAN_POINT('Ctrl Pts',(-69.3985893007012,1076.71096940083,
335.708253129166));
#109664=CARTESIAN_POINT('Ctrl Pts',(-69.4825522658041,1076.7038426352,335.708253129166));
#109665=CARTESIAN_POINT('Ctrl Pts',(-69.4825522658041,1076.7038426352,335.708253129166));
#109666=CARTESIAN_POINT('Ctrl Pts',(-69.4825705531623,1076.70384108297,
335.708253129166));
#109667=CARTESIAN_POINT('Ctrl Pts',(-69.4825888405381,1076.70383953079,
335.708253129627));
#109668=CARTESIAN_POINT('Ctrl Pts',(-69.4826071279312,1076.70383797866,
335.708253130547));
#109669=CARTESIAN_POINT('Ctrl Pts',(-69.6122661348406,1076.6928332308,335.708259653337));
#109670=CARTESIAN_POINT('Ctrl Pts',(-69.7410600097854,1076.68435586556,
335.731389570645));
#109671=CARTESIAN_POINT('Ctrl Pts',(-69.9252515962546,1076.67604353777,
335.799932842917));
#109672=CARTESIAN_POINT('Ctrl Pts',(-69.9853773394517,1076.6740281655,335.828804479751));
#109673=CARTESIAN_POINT('Ctrl Pts',(-70.065966362588,1076.67235332251,335.877027030626));
#109674=CARTESIAN_POINT('Ctrl Pts',(-70.0888852300184,1076.67200602789,
335.891938511393));
#109675=CARTESIAN_POINT('Ctrl Pts',(-70.1248349067323,1076.67167395913,
335.917300983904));
#109676=CARTESIAN_POINT('Ctrl Pts',(-70.1382271237482,1076.67160062707,
335.927216453134));
#109677=CARTESIAN_POINT('Ctrl Pts',(-70.1654173135824,1076.67155755917,
335.948329307373));
#109678=CARTESIAN_POINT('Ctrl Pts',(-70.1791791775886,1076.67159500239,
335.959564711252));
#109679=CARTESIAN_POINT('Ctrl Pts',(-70.2104970271546,1076.67182050406,
335.986434420972));
#109680=CARTESIAN_POINT('Ctrl Pts',(-70.2278335388946,1076.67205325274,
336.002309611403));
#109681=CARTESIAN_POINT('Ctrl Pts',(-70.2805374697881,1076.673108753,336.053799314351));
#109682=CARTESIAN_POINT('Ctrl Pts',(-70.3139607991339,1076.67430003511,
336.091294821934));
#109683=CARTESIAN_POINT('Ctrl Pts',(-70.4330963815764,1076.6807143756,336.24508761985));
#109684=CARTESIAN_POINT('Ctrl Pts',(-70.49784937384,1076.68924147617,336.375489895875));
#109685=CARTESIAN_POINT('Ctrl Pts',(-70.5663202198497,1076.7106436688,336.629068129207));
#109686=CARTESIAN_POINT('Ctrl Pts',(-70.5783051280181,1076.72234154244,
336.747740675396));
#109687=CARTESIAN_POINT('Ctrl Pts',(-70.5630714656046,1076.75002812789,
336.995035830317));
#109688=CARTESIAN_POINT('Ctrl Pts',(-70.5321877705488,1076.76610070584,
337.121631978629));
#109689=CARTESIAN_POINT('Ctrl Pts',(-70.423597839457,1076.80122695084,337.367252835835));
#109690=CARTESIAN_POINT('Ctrl Pts',(-70.3433102000216,1076.82011050786,
337.482752026317));
#109691=CARTESIAN_POINT('Ctrl Pts',(-70.1397833686064,1076.8578278015,337.680994956384));
#109692=CARTESIAN_POINT('Ctrl Pts',(-70.0169048613728,1076.87627974686,
337.760452494493));
#109693=CARTESIAN_POINT('Ctrl Pts',(-69.7549067552893,1076.90856542224,
337.863563967587));
#109694=CARTESIAN_POINT('Ctrl Pts',(-69.619441594183,1076.92232908849,337.889334626623));
#109695=CARTESIAN_POINT('Ctrl Pts',(-69.482552265803,1076.93351373127,337.889334626623));
#109696=CARTESIAN_POINT('',(-56.6885840720973,1077.75968243012,337.489274485682));
#109697=CARTESIAN_POINT('',(-56.6885840720974,1077.56894342885,335.291612213697));
#109698=CARTESIAN_POINT('Ctrl Pts',(-56.6885840720972,1077.75968243012,
337.489274485682));
#109699=CARTESIAN_POINT('Ctrl Pts',(-56.613442812984,1077.76373623307,337.489274485682));
#109700=CARTESIAN_POINT('Ctrl Pts',(-56.5383276565235,1077.7671323857,337.481566998586));
#109701=CARTESIAN_POINT('Ctrl Pts',(-56.3865521884614,1077.77264390424,
337.449940841078));
#109702=CARTESIAN_POINT('Ctrl Pts',(-56.3106458623279,1077.77465802433,
337.425299584034));
#109703=CARTESIAN_POINT('Ctrl Pts',(-56.2097428198071,1077.77628305086,
337.379940323458));
#109704=CARTESIAN_POINT('Ctrl Pts',(-56.1819845595998,1077.77660965807,
337.366020258967));
#109705=CARTESIAN_POINT('Ctrl Pts',(-56.1369653440164,1077.77693575642,
337.341003898954));
#109706=CARTESIAN_POINT('Ctrl Pts',(-56.1193598203174,1077.77700872447,
337.330566929611));
#109707=CARTESIAN_POINT('Ctrl Pts',(-56.0856173841726,1077.7770405101,337.309268104186));
#109708=CARTESIAN_POINT('Ctrl Pts',(-56.0694572267866,1077.77700484843,
337.298457500082));
#109709=CARTESIAN_POINT('Ctrl Pts',(-56.0323218691688,1077.77680172933,
337.272162730304));
#109710=CARTESIAN_POINT('Ctrl Pts',(-56.0115944661511,1077.77659357258,
337.256349892332));
#109711=CARTESIAN_POINT('Ctrl Pts',(-55.9476021541347,1077.77564178804,
337.203827277157));
#109712=CARTESIAN_POINT('Ctrl Pts',(-55.9066136065438,1077.77455785302,
337.164502756248));
#109713=CARTESIAN_POINT('Ctrl Pts',(-55.7718866054966,1077.76918085393,
337.01357711742));
#109714=CARTESIAN_POINT('Ctrl Pts',(-55.6975501542133,1077.76257803684,
336.886849074861));
#109715=CARTESIAN_POINT('Ctrl Pts',(-55.6104673649987,1077.74608591605,
336.634930365164));
#109716=CARTESIAN_POINT('Ctrl Pts',(-55.5901268619979,1077.73704060687,
336.514756146664));
#109717=CARTESIAN_POINT('Ctrl Pts',(-55.589356343351,1077.71560543996,336.26204679572));
#109718=CARTESIAN_POINT('Ctrl Pts',(-55.6126508740519,1077.70315950819,
336.131390238009));
#109719=CARTESIAN_POINT('Ctrl Pts',(-55.7077875383169,1077.67583059169,
335.875101844607));
#109720=CARTESIAN_POINT('Ctrl Pts',(-55.7824013406094,1077.66108014764,
335.752977937319));
#109721=CARTESIAN_POINT('Ctrl Pts',(-55.9672709205554,1077.63306107873,
335.551063375541));
#109722=CARTESIAN_POINT('Ctrl Pts',(-56.0732663837531,1077.61998074431,
335.470512491792));
#109723=CARTESIAN_POINT('Ctrl Pts',(-56.2594731817596,1077.60103232,335.375959466957));
#109724=CARTESIAN_POINT('Ctrl Pts',(-56.3313515194324,1077.59449180072,
335.348468860971));
#109725=CARTESIAN_POINT('Ctrl Pts',(-56.4978156201092,1077.58102251536,
335.304093553933));
#109726=CARTESIAN_POINT('Ctrl Pts',(-56.5929620084085,1077.57444466517,
335.291612213697));
#109727=CARTESIAN_POINT('Ctrl Pts',(-56.6885840720975,1077.56894342885,
335.291612213697));
#109728=CARTESIAN_POINT('Ctrl Pts',(-56.6885840720975,1077.56894342885,
335.291612213697));
#109729=CARTESIAN_POINT('Ctrl Pts',(-56.6886054837368,1077.56894219702,
335.291612213697));
#109730=CARTESIAN_POINT('Ctrl Pts',(-56.6886268953997,1077.56894096524,
335.291612214276));
#109731=CARTESIAN_POINT('Ctrl Pts',(-56.6886483070866,1077.56893973351,
335.291612215528));
#109732=CARTESIAN_POINT('Ctrl Pts',(-56.8261524989056,1077.56102968588,
335.291620253694));
#109733=CARTESIAN_POINT('Ctrl Pts',(-56.9625358482213,1077.55546902066,
335.317438268971));
#109734=CARTESIAN_POINT('Ctrl Pts',(-57.1275010395179,1077.55176827106,
335.382302884576));
#109735=CARTESIAN_POINT('Ctrl Pts',(-57.1635167452176,1077.55116664873,
335.398760540504));
#109736=CARTESIAN_POINT('Ctrl Pts',(-57.2187492407822,1077.55057716798,
335.427700492683));
#109737=CARTESIAN_POINT('Ctrl Pts',(-57.2385961998946,1077.55043734646,
335.438899543604));
#109738=CARTESIAN_POINT('Ctrl Pts',(-57.274532934087,1077.55031926313,335.460677859578));
#109739=CARTESIAN_POINT('Ctrl Pts',(-57.2907201865981,1077.55031926237,
335.471078332917));
#109740=CARTESIAN_POINT('Ctrl Pts',(-57.3254407128916,1077.55043726238,
335.49469713275));
#109741=CARTESIAN_POINT('Ctrl Pts',(-57.3438528839117,1077.55057681396,
335.508076981979));
#109742=CARTESIAN_POINT('Ctrl Pts',(-57.3938617433937,1077.55117448315,
335.546846668709));
#109743=CARTESIAN_POINT('Ctrl Pts',(-57.4244866662291,1077.55179580614,
335.573425151543));
#109744=CARTESIAN_POINT('Ctrl Pts',(-57.5580740842792,1077.55572990302,
335.702977760875));
#109745=CARTESIAN_POINT('Ctrl Pts',(-57.6413195462532,1077.56180608728,
335.824003580477));
#109746=CARTESIAN_POINT('Ctrl Pts',(-57.7450845616833,1077.57750963289,
336.066133436293));
#109747=CARTESIAN_POINT('Ctrl Pts',(-57.7737586136471,1077.58615022061,
336.181350369018));
#109748=CARTESIAN_POINT('Ctrl Pts',(-57.7943339688813,1077.606809626,336.427227303112));
#109749=CARTESIAN_POINT('Ctrl Pts',(-57.7824003765923,1077.61890859438,
336.556442315922));
#109750=CARTESIAN_POINT('Ctrl Pts',(-57.7118296547517,1077.64552330391,
336.814246723941));
#109751=CARTESIAN_POINT('Ctrl Pts',(-57.6502753482028,1077.65992134601,
336.939788007474));
#109752=CARTESIAN_POINT('Ctrl Pts',(-57.4794403334006,1077.68910347425,
337.167126248791));
#109753=CARTESIAN_POINT('Ctrl Pts',(-57.36946577095,1077.70358920761,337.2651649272));
#109754=CARTESIAN_POINT('Ctrl Pts',(-57.1215703856538,1077.72954462121,
337.410197946034));
#109755=CARTESIAN_POINT('Ctrl Pts',(-56.9869411183763,1077.74086153681,
337.457417069255));
#109756=CARTESIAN_POINT('Ctrl Pts',(-56.7944096421122,1077.75364784999,
337.485453510447));
#109757=CARTESIAN_POINT('Ctrl Pts',(-56.7414903885327,1077.75682818221,
337.489274485682));
#109758=CARTESIAN_POINT('Ctrl Pts',(-56.6885840720972,1077.75968243012,
337.489274485682));
#109759=CARTESIAN_POINT('',(-44.0648939479108,1078.41872688014,339.782224246531));
#109760=CARTESIAN_POINT('',(-44.0648939479107,1078.2734328653,337.231336004259));
#109761=CARTESIAN_POINT('Ctrl Pts',(-44.0648939479108,1078.41872688014,
339.782224246531));
#109762=CARTESIAN_POINT('Ctrl Pts',(-43.9698585685592,1078.42127600878,
339.782224246531));
#109763=CARTESIAN_POINT('Ctrl Pts',(-43.8748911966279,1078.42325397626,
339.771602237811));
#109764=CARTESIAN_POINT('Ctrl Pts',(-43.7242121194281,1078.42547969287,
339.737300270294));
#109765=CARTESIAN_POINT('Ctrl Pts',(-43.667617845379,1078.42609562414,339.720211708276));
#109766=CARTESIAN_POINT('Ctrl Pts',(-43.5837314112947,1078.42667110235,
339.688381229543));
#109767=CARTESIAN_POINT('Ctrl Pts',(-43.5554548940477,1078.4268036277,339.676468305807));
#109768=CARTESIAN_POINT('Ctrl Pts',(-43.5053435987973,1078.42692639709,
339.653194195071));
#109769=CARTESIAN_POINT('Ctrl Pts',(-43.4833559077857,1078.42693965325,
339.642198692177));
#109770=CARTESIAN_POINT('Ctrl Pts',(-43.4373976527315,1078.42687999769,
339.617530701329));
#109771=CARTESIAN_POINT('Ctrl Pts',(-43.4135252695797,1078.42679637772,
339.603701849644));
#109772=CARTESIAN_POINT('Ctrl Pts',(-43.3515726057863,1078.42643740777,
339.565077738407));
#109773=CARTESIAN_POINT('Ctrl Pts',(-43.31433734979,1078.4260732985,339.539003823256));
#109774=CARTESIAN_POINT('Ctrl Pts',(-43.1618656252936,1078.42392496087,
339.419615998369));
#109775=CARTESIAN_POINT('Ctrl Pts',(-43.0620000515213,1078.42081136629,
339.308600827055));
#109776=CARTESIAN_POINT('Ctrl Pts',(-42.9117761736833,1078.41221921664,
339.068342403409));
#109777=CARTESIAN_POINT('Ctrl Pts',(-42.8588046707743,1078.40702463369,
338.943083927874));
#109778=CARTESIAN_POINT('Ctrl Pts',(-42.7910566805472,1078.39413187769,
338.668107998734));
#109779=CARTESIAN_POINT('Ctrl Pts',(-42.7809529005184,1078.38633677174,
338.519289117061));
#109780=CARTESIAN_POINT('Ctrl Pts',(-42.8134108370878,1078.36855139611,
338.213583100402));
#109781=CARTESIAN_POINT('Ctrl Pts',(-42.8598155164218,1078.35859085684,
338.059631555308));
#109782=CARTESIAN_POINT('Ctrl Pts',(-43.0113674875638,1078.33755056151,
337.768252159249));
#109783=CARTESIAN_POINT('Ctrl Pts',(-43.1184390201791,1078.32664465516,
337.635244041802));
#109784=CARTESIAN_POINT('Ctrl Pts',(-43.3444784264674,1078.30872444725,
337.446864562296));
#109785=CARTESIAN_POINT('Ctrl Pts',(-43.4519113159758,1078.30153381717,
337.381308044457));
#109786=CARTESIAN_POINT('Ctrl Pts',(-43.6363565982265,1078.29115440135,
337.303137310967));
#109787=CARTESIAN_POINT('Ctrl Pts',(-43.7079861960549,1078.28753594555,
337.279986987218));
#109788=CARTESIAN_POINT('Ctrl Pts',(-43.874283065922,1078.28006182476,337.242054582449));
#109789=CARTESIAN_POINT('Ctrl Pts',(-43.9694259521163,1078.2764294892,337.231336100891));
#109790=CARTESIAN_POINT('Ctrl Pts',(-44.0648926569059,1078.27343290582,
337.23133600426));
#109791=CARTESIAN_POINT('Ctrl Pts',(-44.0648939479107,1078.2734328653,337.231336004259));
#109792=CARTESIAN_POINT('Ctrl Pts',(-44.1880047205763,1078.26956857586,
337.231336004259));
#109793=CARTESIAN_POINT('Ctrl Pts',(-44.3104925612769,1078.26679899349,
337.249160351226));
#109794=CARTESIAN_POINT('Ctrl Pts',(-44.4706067741549,1078.26467963642,
337.296788011882));
#109795=CARTESIAN_POINT('Ctrl Pts',(-44.5120000439969,1078.26427737102,
337.311464184729));
#109796=CARTESIAN_POINT('Ctrl Pts',(-44.5778875498776,1078.26387835467,
337.338727532798));
#109797=CARTESIAN_POINT('Ctrl Pts',(-44.6028752707143,1078.2637861645,337.350023706425));
#109798=CARTESIAN_POINT('Ctrl Pts',(-44.6498772982532,1078.26372736808,
337.373124526043));
#109799=CARTESIAN_POINT('Ctrl Pts',(-44.6719469510812,1078.263750252,337.384787619108));
#109800=CARTESIAN_POINT('Ctrl Pts',(-44.7213912479415,1078.26391818437,
337.412803476177));
#109801=CARTESIAN_POINT('Ctrl Pts',(-44.7485231994662,1078.26409527662,
337.429550065953));
#109802=CARTESIAN_POINT('Ctrl Pts',(-44.8279209712877,1078.26487350374,
337.482765306169));
#109803=CARTESIAN_POINT('Ctrl Pts',(-44.8781074114896,1078.26572049452,
337.522148538001));
#109804=CARTESIAN_POINT('Ctrl Pts',(-45.0507228634677,1078.26999963111,
337.679838407417));
#109805=CARTESIAN_POINT('Ctrl Pts',(-45.1520505367577,1078.27534679267,
337.818491183739));
#109806=CARTESIAN_POINT('Ctrl Pts',(-45.2819458029642,1078.28844897224,
338.100293223211));
#109807=CARTESIAN_POINT('Ctrl Pts',(-45.3192348827645,1078.29552830067,
338.236503697566));
#109808=CARTESIAN_POINT('Ctrl Pts',(-45.3491963327816,1078.31195866523,
338.527139642762));
#109809=CARTESIAN_POINT('Ctrl Pts',(-45.3376392626775,1078.32131730675,
338.679831390756));
#109810=CARTESIAN_POINT('Ctrl Pts',(-45.2586250696309,1078.34136719712,
338.984611036105));
#109811=CARTESIAN_POINT('Ctrl Pts',(-45.1878669986355,1078.35192173704,
339.133080819982));
#109812=CARTESIAN_POINT('Ctrl Pts',(-44.9910710420895,1078.37255856159,
339.399704198003));
#109813=CARTESIAN_POINT('Ctrl Pts',(-44.8651833819723,1078.38241385252,
339.514096763639));
#109814=CARTESIAN_POINT('Ctrl Pts',(-44.5822473190854,1078.39948632042,
339.683702256633));
#109815=CARTESIAN_POINT('Ctrl Pts',(-44.4292884205347,1078.40664767814,
339.739684338288));
#109816=CARTESIAN_POINT('Ctrl Pts',(-44.201977036801,1078.41475375434,339.776702094143));
#109817=CARTESIAN_POINT('Ctrl Pts',(-44.1334178162447,1078.41688886827,
339.782224246531));
#109818=CARTESIAN_POINT('Ctrl Pts',(-44.0648939479108,1078.41872688014,
339.782224246531));
#109819=CARTESIAN_POINT('',(-14.6999478050468,1078.7051236444,337.754967205958));
#109820=CARTESIAN_POINT('',(-14.6999478050467,1078.63014532468,334.798360941572));
#109821=CARTESIAN_POINT('Ctrl Pts',(-14.6999478050468,1078.7051236444,337.754967205958));
#109822=CARTESIAN_POINT('Ctrl Pts',(-14.6589123536955,1078.7052433175,337.754967205958));
#109823=CARTESIAN_POINT('Ctrl Pts',(-14.6178921577028,1078.7053326354,337.753258582307));
#109824=CARTESIAN_POINT('Ctrl Pts',(-14.5422341208689,1078.70544207271,
337.74694404751));
#109825=CARTESIAN_POINT('Ctrl Pts',(-14.5075879085124,1078.70547052478,
337.742813616038));
#109826=CARTESIAN_POINT('Ctrl Pts',(-14.4357656202781,1078.70548443118,
337.731661304056));
#109827=CARTESIAN_POINT('Ctrl Pts',(-14.3986471606966,1078.70546608187,
337.72443031423));
#109828=CARTESIAN_POINT('Ctrl Pts',(-14.3125881117328,1078.70536326053,
337.704211958564));
#109829=CARTESIAN_POINT('Ctrl Pts',(-14.2639561299985,1078.70525859826,
337.690117906049));
#109830=CARTESIAN_POINT('Ctrl Pts',(-14.1147826631352,1078.70478798948,
337.638452680117));
#109831=CARTESIAN_POINT('Ctrl Pts',(-14.0175446031057,1078.70426283054,
337.592419327622));
#109832=CARTESIAN_POINT('Ctrl Pts',(-13.758249841205,1078.70216932428,337.433129884863));
#109833=CARTESIAN_POINT('Ctrl Pts',(-13.6126630540636,1078.70011869856,
337.29745514565));
#109834=CARTESIAN_POINT('Ctrl Pts',(-13.399413227183,1078.69491773742,336.999607363213));
#109835=CARTESIAN_POINT('Ctrl Pts',(-13.325241670197,1078.69199617544,336.846062448113));
#109836=CARTESIAN_POINT('Ctrl Pts',(-13.2285735283737,1078.6848939826,336.508210561569));
#109837=CARTESIAN_POINT('Ctrl Pts',(-13.2112641298419,1078.68069073918,
336.325344224527));
#109838=CARTESIAN_POINT('Ctrl Pts',(-13.2451714983133,1078.67119546056,
335.949155420977));
#109839=CARTESIAN_POINT('Ctrl Pts',(-13.3012165217026,1078.66593770448,
335.75976615305));
#109840=CARTESIAN_POINT('Ctrl Pts',(-13.4826519806559,1078.65551499784,
335.415908764833));
#109841=CARTESIAN_POINT('Ctrl Pts',(-13.605449867651,1078.65045491218,335.264345333663));
#109842=CARTESIAN_POINT('Ctrl Pts',(-13.8908387664958,1078.64178807057,
335.026676995523));
#109843=CARTESIAN_POINT('Ctrl Pts',(-14.0472523841235,1078.6381751293,334.938335581696));
#109844=CARTESIAN_POINT('Ctrl Pts',(-14.3495679685873,1078.63320356144,
334.833502505654));
#109845=CARTESIAN_POINT('Ctrl Pts',(-14.4895158833743,1078.6315618089,334.806560824859));
#109846=CARTESIAN_POINT('Ctrl Pts',(-14.6540516932643,1078.6304135091,334.798895782795));
#109847=CARTESIAN_POINT('Ctrl Pts',(-14.6769708122268,1078.63027087472,
334.798361789893));
#109848=CARTESIAN_POINT('Ctrl Pts',(-14.6998931606234,1078.63014562323,
334.798360942585));
#109849=CARTESIAN_POINT('Ctrl Pts',(-14.6999113754354,1078.6301455237,334.798360941911));
#109850=CARTESIAN_POINT('Ctrl Pts',(-14.6999295902432,1078.63014542419,
334.798360941572));
#109851=CARTESIAN_POINT('Ctrl Pts',(-14.6999478050467,1078.63014532468,
334.798360941572));
#109852=CARTESIAN_POINT('Ctrl Pts',(-14.6999478050467,1078.63014532468,
334.798360941572));
#109853=CARTESIAN_POINT('Ctrl Pts',(-14.7496366904929,1078.62987387635,
334.798360941572));
#109854=CARTESIAN_POINT('Ctrl Pts',(-14.7992942996238,1078.62968439931,
334.800866162424));
#109855=CARTESIAN_POINT('Ctrl Pts',(-14.8867403145353,1078.62949663331,
334.809712077419));
#109856=CARTESIAN_POINT('Ctrl Pts',(-14.9245858035539,1078.62946433312,
334.815028901272));
#109857=CARTESIAN_POINT('Ctrl Pts',(-15.0019471554124,1078.62949962106,
334.828973111974));
#109858=CARTESIAN_POINT('Ctrl Pts',(-15.0414008598778,1078.6295730621,334.837767787017));
#109859=CARTESIAN_POINT('Ctrl Pts',(-15.1394814709311,1078.62989560303,
334.863892701655));
#109860=CARTESIAN_POINT('Ctrl Pts',(-15.1974861911861,1078.63021513983,
334.883262411773));
#109861=CARTESIAN_POINT('Ctrl Pts',(-15.4035650497694,1078.63182149038,
334.966592792844));
#109862=CARTESIAN_POINT('Ctrl Pts',(-15.5421111064959,1078.63382773723,
335.051054370372));
#109863=CARTESIAN_POINT('Ctrl Pts',(-15.7838671273692,1078.63917763711,
335.259120231833));
#109864=CARTESIAN_POINT('Ctrl Pts',(-15.88620544731,1078.64245551688,335.380526314563));
#109865=CARTESIAN_POINT('Ctrl Pts',(-16.0556344970397,1078.65016819128,
335.662760107197));
#109866=CARTESIAN_POINT('Ctrl Pts',(-16.1176273394778,1078.65461665645,
335.823955988844));
#109867=CARTESIAN_POINT('Ctrl Pts',(-16.185959543564,1078.66409952728,336.172373481196));
#109868=CARTESIAN_POINT('Ctrl Pts',(-16.1874143971128,1078.66906641868,
336.35761110391));
#109869=CARTESIAN_POINT('Ctrl Pts',(-16.1199834112205,1078.67885370572,
336.73250043513));
#109870=CARTESIAN_POINT('Ctrl Pts',(-16.0465580177525,1078.68353601572,
336.917708199298));
#109871=CARTESIAN_POINT('Ctrl Pts',(-15.8341720149533,1078.69160169471,
337.244037831854));
#109872=CARTESIAN_POINT('Ctrl Pts',(-15.6990081640736,1078.69494485142,
337.383083186043));
#109873=CARTESIAN_POINT('Ctrl Pts',(-15.3933037326129,1078.70012415692,
337.594580624634));
#109874=CARTESIAN_POINT('Ctrl Pts',(-15.2281790413487,1078.7020071838,337.669008364265));
#109875=CARTESIAN_POINT('Ctrl Pts',(-14.9434874709919,1078.70413372867,
337.73918496718));
#109876=CARTESIAN_POINT('Ctrl Pts',(-14.8304481116973,1078.70471821139,
337.753569334503));
#109877=CARTESIAN_POINT('Ctrl Pts',(-14.711236065491,1078.70509015022,337.754934883857));
#109878=CARTESIAN_POINT('Ctrl Pts',(-14.7055917909763,1078.70510718465,
337.754967205958));
#109879=CARTESIAN_POINT('Ctrl Pts',(-14.6999478050468,1078.7051236444,337.754967205958));
#109880=CARTESIAN_POINT('',(-25.1979747106604,1078.42435733551,332.502403403865));
#109881=CARTESIAN_POINT('',(-25.1979747106603,1078.26679962567,329.951515161593));
#109882=CARTESIAN_POINT('Ctrl Pts',(-25.1979747106604,1078.42435733551,
332.502403403865));
#109883=CARTESIAN_POINT('Ctrl Pts',(-25.152160999578,1078.42505470245,332.502403403865));
#109884=CARTESIAN_POINT('Ctrl Pts',(-25.1063479654105,1078.42561183531,
332.499934973706));
#109885=CARTESIAN_POINT('Ctrl Pts',(-25.0252461736709,1078.42634944539,
332.491157371042));
#109886=CARTESIAN_POINT('Ctrl Pts',(-24.9899331133854,1078.42658556673,
332.485828112392));
#109887=CARTESIAN_POINT('Ctrl Pts',(-24.9287492539622,1078.42684587456,
332.473949434464));
#109888=CARTESIAN_POINT('Ctrl Pts',(-24.9027740417738,1078.42690859574,
332.468056927039));
#109889=CARTESIAN_POINT('Ctrl Pts',(-24.849042837633,1078.426938142,332.45408553475));
#109890=CARTESIAN_POINT('Ctrl Pts',(-24.8213385508615,1078.42689636731,
332.445867599421));
#109891=CARTESIAN_POINT('Ctrl Pts',(-24.7570850203332,1078.42666450101,
332.424408058209));
#109892=CARTESIAN_POINT('Ctrl Pts',(-24.7208148879577,1078.42642835409,
332.410422715425));
#109893=CARTESIAN_POINT('Ctrl Pts',(-24.6084599785012,1078.42535813259,
332.361094055936));
#109894=CARTESIAN_POINT('Ctrl Pts',(-24.5351968034651,1078.42415126337,
332.319896847511));
#109895=CARTESIAN_POINT('Ctrl Pts',(-24.3276760062992,1078.4191009773,332.174619777398));
#109896=CARTESIAN_POINT('Ctrl Pts',(-24.2096372996228,1078.4138765529,332.050752574564));
#109897=CARTESIAN_POINT('Ctrl Pts',(-24.0422923077211,1078.40116943319,
331.785497718849));
#109898=CARTESIAN_POINT('Ctrl Pts',(-23.9866003231676,1078.39422554416,
331.651356599257));
#109899=CARTESIAN_POINT('Ctrl Pts',(-23.9198638252662,1078.37797500119,
331.359003512358));
#109900=CARTESIAN_POINT('Ctrl Pts',(-23.9133094359033,1078.36865673574,
331.20216901896));
#109901=CARTESIAN_POINT('Ctrl Pts',(-23.9585998767981,1078.34835887168,
330.882441906846));
#109902=CARTESIAN_POINT('Ctrl Pts',(-24.0144206331024,1078.33749981153,
330.723033929454));
#109903=CARTESIAN_POINT('Ctrl Pts',(-24.1844442927444,1078.31636709739,
330.434794148616));
#109904=CARTESIAN_POINT('Ctrl Pts',(-24.2970507612122,1078.30629851345,
330.308734657781));
#109905=CARTESIAN_POINT('Ctrl Pts',(-24.5554661786938,1078.28909552609,
330.114179678535));
#109906=CARTESIAN_POINT('Ctrl Pts',(-24.6963108177312,1078.28195547514,
330.043969101914));
#109907=CARTESIAN_POINT('Ctrl Pts',(-24.9606785236178,1078.2721924645,329.968156166984));
#109908=CARTESIAN_POINT('Ctrl Pts',(-25.0790207575768,1078.26894718679,
329.951515180457));
#109909=CARTESIAN_POINT('Ctrl Pts',(-25.1979745084014,1078.26679962932,
329.951515161593));
#109910=CARTESIAN_POINT('Ctrl Pts',(-25.1979747106603,1078.26679962567,
329.951515161593));
#109911=CARTESIAN_POINT('Ctrl Pts',(-25.2538390162154,1078.26579106784,
329.951515161593));
#109912=CARTESIAN_POINT('Ctrl Pts',(-25.3096461383107,1078.2650278866,329.955185413986));
#109913=CARTESIAN_POINT('Ctrl Pts',(-25.4010408522882,1078.26418420401,
329.967260573507));
#109914=CARTESIAN_POINT('Ctrl Pts',(-25.4368269000737,1078.26395863441,
329.973553353014));
#109915=CARTESIAN_POINT('Ctrl Pts',(-25.5003875254845,1078.26374726159,
329.987551522511));
#109916=CARTESIAN_POINT('Ctrl Pts',(-25.528261637163,1078.26372140329,329.994686723473));
#109917=CARTESIAN_POINT('Ctrl Pts',(-25.5864441219895,1078.26380940912,
330.01169641011));
#109918=CARTESIAN_POINT('Ctrl Pts',(-25.6166716843358,1078.26393854366,
330.0217766678));
#109919=CARTESIAN_POINT('Ctrl Pts',(-25.6945523141232,1078.26449138128,
330.05103226143));
#109920=CARTESIAN_POINT('Ctrl Pts',(-25.7414786658446,1078.26504649419,
330.07197155084));
#109921=CARTESIAN_POINT('Ctrl Pts',(-25.9260906165669,1078.26814828127,
330.168095987952));
#109922=CARTESIAN_POINT('Ctrl Pts',(-26.0505853878352,1078.2724199097,330.265517330287));
#109923=CARTESIAN_POINT('Ctrl Pts',(-26.2451111638944,1078.28354380179,
330.485941438791));
#109924=CARTESIAN_POINT('Ctrl Pts',(-26.3187027191012,1078.28993492838,
330.602823386777));
#109925=CARTESIAN_POINT('Ctrl Pts',(-26.430495652749,1078.30513901016,330.866516436001));
#109926=CARTESIAN_POINT('Ctrl Pts',(-26.4641653372882,1078.31399636629,
331.013031980771));
#109927=CARTESIAN_POINT('Ctrl Pts',(-26.47991708103,1078.33333093322,331.321855554161));
#109928=CARTESIAN_POINT('Ctrl Pts',(-26.4579025795552,1078.34370740875,
331.481832355953));
#109929=CARTESIAN_POINT('Ctrl Pts',(-26.353027678289,1078.36461949114,331.793655948564));
#109930=CARTESIAN_POINT('Ctrl Pts',(-26.2678904931126,1078.37492771218,
331.941522037978));
#109931=CARTESIAN_POINT('Ctrl Pts',(-26.0477585667338,1078.39334303653,
332.192218928031));
#109932=CARTESIAN_POINT('Ctrl Pts',(-25.9161694794889,1078.40133180787,
332.293773788076));
#109933=CARTESIAN_POINT('Ctrl Pts',(-25.6296807223542,1078.41405867805,
332.437169584067));
#109934=CARTESIAN_POINT('Ctrl Pts',(-25.4788877391697,1078.41884847287,
332.480790853491));
#109935=CARTESIAN_POINT('Ctrl Pts',(-25.2820480479779,1078.42295952733,
332.500325235152));
#109936=CARTESIAN_POINT('Ctrl Pts',(-25.2400110944244,1078.42371746628,
332.502403403865));
#109937=CARTESIAN_POINT('Ctrl Pts',(-25.1979747106604,1078.42435733551,
332.502403403865));
#109938=CARTESIAN_POINT('',(-37.1057957606637,1077.76997147869,327.631087921141));
#109939=CARTESIAN_POINT('',(-37.1057957606635,1077.5579316459,325.433425649156));
#109940=CARTESIAN_POINT('Ctrl Pts',(-37.1057957606639,1077.76997147869,
327.631087921141));
#109941=CARTESIAN_POINT('Ctrl Pts',(-37.0507987318168,1077.77190604638,
327.631087921141));
#109942=CARTESIAN_POINT('Ctrl Pts',(-36.9957541821996,1077.77345630688,
327.626959114939));
#109943=CARTESIAN_POINT('Ctrl Pts',(-36.8986799269302,1077.77549923108,
327.61224576858));
#109944=CARTESIAN_POINT('Ctrl Pts',(-36.8566408676037,1077.77614728382,
327.603328977249));
#109945=CARTESIAN_POINT('Ctrl Pts',(-36.7910552112728,1077.77678054052,
327.585345823688));
#109946=CARTESIAN_POINT('Ctrl Pts',(-36.7671154963525,1077.77692917547,
327.577892411466));
#109947=CARTESIAN_POINT('Ctrl Pts',(-36.7229587698778,1077.77704792786,
327.562468841074));
#109948=CARTESIAN_POINT('Ctrl Pts',(-36.7026829298606,1077.77703927445,
327.554705357602));
#109949=CARTESIAN_POINT('Ctrl Pts',(-36.6583938295681,1077.77687919098,
327.536225013625));
#109950=CARTESIAN_POINT('Ctrl Pts',(-36.6345088005065,1077.77669809455,
327.525236756178));
#109951=CARTESIAN_POINT('Ctrl Pts',(-36.5679569453334,1077.77592045116,
327.491677211778));
#109952=CARTESIAN_POINT('Ctrl Pts',(-36.5263549901042,1077.77510407512,
327.467139411149));
#109953=CARTESIAN_POINT('Ctrl Pts',(-36.3656673256076,1077.77056904092,
327.357507276023));
#109954=CARTESIAN_POINT('Ctrl Pts',(-36.2625920360524,1077.76437350324,
327.251822883907));
#109955=CARTESIAN_POINT('Ctrl Pts',(-36.1179450963914,1077.74858962957,
327.028268383998));
#109956=CARTESIAN_POINT('Ctrl Pts',(-36.0697037120012,1077.73990347443,
326.917410247792));
#109957=CARTESIAN_POINT('Ctrl Pts',(-36.0083464949823,1077.71914166221,
326.674206792521));
#109958=CARTESIAN_POINT('Ctrl Pts',(-35.999275836045,1077.70699389374,326.542752524337));
#109959=CARTESIAN_POINT('Ctrl Pts',(-36.0287616005446,1077.68013760776,
326.272935955355));
#109960=CARTESIAN_POINT('Ctrl Pts',(-36.0708062327943,1077.66554285194,
326.13724840386));
#109961=CARTESIAN_POINT('Ctrl Pts',(-36.2060056656884,1077.63611503389,
325.884974465073));
#109962=CARTESIAN_POINT('Ctrl Pts',(-36.2995550386854,1077.62157098013,
325.77158691681));
#109963=CARTESIAN_POINT('Ctrl Pts',(-36.4915776751045,1077.59907323847,
325.615447952087));
#109964=CARTESIAN_POINT('Ctrl Pts',(-36.5792024850074,1077.59056064311,
325.562447192936));
#109965=CARTESIAN_POINT('Ctrl Pts',(-36.7310998545457,1077.57841283068,
325.49734794043));
#109966=CARTESIAN_POINT('Ctrl Pts',(-36.7913278422833,1077.57417553721,
325.477481637902));
#109967=CARTESIAN_POINT('Ctrl Pts',(-36.935768174724,1077.56534061361,325.443330204206));
#109968=CARTESIAN_POINT('Ctrl Pts',(-37.0206145131777,1077.56115002462,
325.43342572128));
#109969=CARTESIAN_POINT('Ctrl Pts',(-37.1057948302677,1077.55793168106,
325.433425649157));
#109970=CARTESIAN_POINT('Ctrl Pts',(-37.1057957606634,1077.5579316459,325.433425649156));
#109971=CARTESIAN_POINT('Ctrl Pts',(-37.1819018986778,1077.55505615586,
325.433425649156));
#109972=CARTESIAN_POINT('Ctrl Pts',(-37.2578231472279,1077.55297389363,
325.441332273578));
#109973=CARTESIAN_POINT('Ctrl Pts',(-37.3645574303048,1077.55118391002,
325.463820301091));
#109974=CARTESIAN_POINT('Ctrl Pts',(-37.3964584062127,1077.55080015102,
325.472054170212));
#109975=CARTESIAN_POINT('Ctrl Pts',(-37.4476616454257,1077.55043295362,
325.487755483657));
#109976=CARTESIAN_POINT('Ctrl Pts',(-37.4672063328431,1077.55035358104,
325.494356178952));
#109977=CARTESIAN_POINT('Ctrl Pts',(-37.5075396586184,1077.55031767442,
325.509255218331));
#109978=CARTESIAN_POINT('Ctrl Pts',(-37.5282836445334,1077.55037212035,
325.517646349847));
#109979=CARTESIAN_POINT('Ctrl Pts',(-37.5763639693276,1077.55067151027,
325.538825625678));
#109980=CARTESIAN_POINT('Ctrl Pts',(-37.6034573646397,1077.55097609398,
325.552117676913));
#109981=CARTESIAN_POINT('Ctrl Pts',(-37.6879494814917,1077.55236674982,
325.597976802609));
#109982=CARTESIAN_POINT('Ctrl Pts',(-37.7429657864938,1077.553948481,325.63459730327));
#109983=CARTESIAN_POINT('Ctrl Pts',(-37.9084491018374,1077.56098962291,
325.767658168065));
#109984=CARTESIAN_POINT('Ctrl Pts',(-38.0029572944813,1077.56875408708,
325.881189615137));
#109985=CARTESIAN_POINT('Ctrl Pts',(-38.1307558457615,1077.58742051731,
326.117621726534));
#109986=CARTESIAN_POINT('Ctrl Pts',(-38.1705470485416,1077.59748227609,
326.234397852002));
#109987=CARTESIAN_POINT('Ctrl Pts',(-38.2116478433377,1077.62070890731,
326.48615956015));
#109988=CARTESIAN_POINT('Ctrl Pts',(-38.2091217001448,1077.63387487959,
326.619827418889));
#109989=CARTESIAN_POINT('Ctrl Pts',(-38.1546825940271,1077.662054189,326.889432100301));
#109990=CARTESIAN_POINT('Ctrl Pts',(-38.0995667696273,1077.67687374602,
327.022325921047));
#109991=CARTESIAN_POINT('Ctrl Pts',(-37.9403437576909,1077.70553168252,
327.261603277977));
#109992=CARTESIAN_POINT('Ctrl Pts',(-37.8369629836312,1077.71907910922,
327.365248436876));
#109993=CARTESIAN_POINT('Ctrl Pts',(-37.602967274512,1077.74218215927,327.521620702492));
#109994=CARTESIAN_POINT('Ctrl Pts',(-37.4763845891422,1077.75173219943,
327.575689200392));
#109995=CARTESIAN_POINT('Ctrl Pts',(-37.2649855750143,1077.76356243156,
327.62242852211));
#109996=CARTESIAN_POINT('Ctrl Pts',(-37.185440496621,1077.76716990674,327.631087921141));
#109997=CARTESIAN_POINT('Ctrl Pts',(-37.1057957606639,1077.76997147869,
327.631087921141));
#109998=CARTESIAN_POINT('',(-49.7050859019669,1076.94955520377,325.362209063876));
#109999=CARTESIAN_POINT('',(-49.7050859019678,1076.68713253746,323.18112756642));
#110000=CARTESIAN_POINT('Ctrl Pts',(-49.7050859019669,1076.94955520377,
325.362209063877));
#110001=CARTESIAN_POINT('Ctrl Pts',(-49.6460399786472,1076.95299643431,
325.362209063877));
#110002=CARTESIAN_POINT('Ctrl Pts',(-49.58693856471,1076.95587354174,325.357413855934));
#110003=CARTESIAN_POINT('Ctrl Pts',(-49.4669163176567,1076.96054214956,
325.337704192653));
#110004=CARTESIAN_POINT('Ctrl Pts',(-49.4064236017617,1076.96225869733,
325.322364600977));
#110005=CARTESIAN_POINT('Ctrl Pts',(-49.3242057966663,1076.96368973578,
325.2938328615));
#110006=CARTESIAN_POINT('Ctrl Pts',(-49.3011366422712,1076.96398683401,
325.284937843907));
#110007=CARTESIAN_POINT('Ctrl Pts',(-49.2615021139303,1076.96431313749,
325.268086523608));
#110008=CARTESIAN_POINT('Ctrl Pts',(-49.2447993283327,1076.96439158963,
325.260481801689));
#110009=CARTESIAN_POINT('Ctrl Pts',(-49.2104143436567,1076.96442869618,
325.24376630412));
#110010=CARTESIAN_POINT('Ctrl Pts',(-49.1927737557973,1076.96437678777,
325.234586120349));
#110011=CARTESIAN_POINT('Ctrl Pts',(-49.1519567431063,1076.96408777922,
325.211905614821));
#110012=CARTESIAN_POINT('Ctrl Pts',(-49.1290088083054,1076.96379254135,
325.198023038725));
#110013=CARTESIAN_POINT('Ctrl Pts',(-49.0573709533917,1076.9624374318,325.150993082848));
#110014=CARTESIAN_POINT('Ctrl Pts',(-49.0108565895208,1076.9608877905,325.114751116459));
#110015=CARTESIAN_POINT('Ctrl Pts',(-48.861222714599,1076.95345472606,324.977355147536));
#110016=CARTESIAN_POINT('Ctrl Pts',(-48.7755054433334,1076.94462512839,
324.859775958759));
#110017=CARTESIAN_POINT('Ctrl Pts',(-48.6645186776712,1076.92276836248,
324.61960299161));
#110018=CARTESIAN_POINT('Ctrl Pts',(-48.6325024177503,1076.91080296668,
324.502586298824));
#110019=CARTESIAN_POINT('Ctrl Pts',(-48.6068359393774,1076.8825796473,324.252221412734));
#110020=CARTESIAN_POINT('Ctrl Pts',(-48.6171694112931,1076.86625340712,
324.120360301));
#110021=CARTESIAN_POINT('Ctrl Pts',(-48.6866796476855,1076.83056196565,
323.856732994555));
#110022=CARTESIAN_POINT('Ctrl Pts',(-48.7490856498951,1076.81137638158,
323.728181714423));
#110023=CARTESIAN_POINT('Ctrl Pts',(-48.9188284544825,1076.77399917669,
323.50303606543));
#110024=CARTESIAN_POINT('Ctrl Pts',(-49.0243157812746,1076.75612934328,
323.408168544092));
#110025=CARTESIAN_POINT('Ctrl Pts',(-49.2171405867449,1076.73041995546,
323.292768333095));
#110026=CARTESIAN_POINT('Ctrl Pts',(-49.2940375705273,1076.7215242049,323.258059331199));
#110027=CARTESIAN_POINT('Ctrl Pts',(-49.4810832272676,1076.70289454892,
323.19850750249));
#110028=CARTESIAN_POINT('Ctrl Pts',(-49.5926721239983,1076.6939757664,323.18112756642));
#110029=CARTESIAN_POINT('Ctrl Pts',(-49.7050859019677,1076.68713253746,
323.18112756642));
#110030=CARTESIAN_POINT('Ctrl Pts',(-49.7050859019677,1076.68713253746,
323.18112756642));
#110031=CARTESIAN_POINT('Ctrl Pts',(-49.7050914492263,1076.68713219976,
323.18112756642));
#110032=CARTESIAN_POINT('Ctrl Pts',(-49.7050969964872,1076.68713186208,
323.1811275665));
#110033=CARTESIAN_POINT('Ctrl Pts',(-49.7051025437499,1076.6871315244,323.181127566585));
#110034=CARTESIAN_POINT('Ctrl Pts',(-49.8088206851785,1076.68081783899,
323.181129149337));
#110035=CARTESIAN_POINT('Ctrl Pts',(-49.9120892726801,1076.67634161631,
323.195927130838));
#110036=CARTESIAN_POINT('Ctrl Pts',(-50.0459484580094,1076.67300727247,
323.235154900677));
#110037=CARTESIAN_POINT('Ctrl Pts',(-50.0796160366933,1076.67239233504,
323.246839014162));
#110038=CARTESIAN_POINT('Ctrl Pts',(-50.1329751701086,1076.67178502818,
323.268338935774));
#110039=CARTESIAN_POINT('Ctrl Pts',(-50.153044503504,1076.67164427003,323.27713716433));
#110040=CARTESIAN_POINT('Ctrl Pts',(-50.19066912511,1076.67154917843,323.295001643121));
#110041=CARTESIAN_POINT('Ctrl Pts',(-50.2082692535228,1076.67157780006,
323.303951745155));
#110042=CARTESIAN_POINT('Ctrl Pts',(-50.2475561875321,1076.67180943091,
323.325291815224));
#110043=CARTESIAN_POINT('Ctrl Pts',(-50.2690789873096,1076.67205652613,
323.33795841797));
#110044=CARTESIAN_POINT('Ctrl Pts',(-50.3317134774138,1076.67313965593,
323.377776251054));
#110045=CARTESIAN_POINT('Ctrl Pts',(-50.3714327852864,1076.67431348698,
323.406980586524));
#110046=CARTESIAN_POINT('Ctrl Pts',(-50.5193156694129,1076.68068270556,
323.53196688866));
#110047=CARTESIAN_POINT('Ctrl Pts',(-50.6098383556455,1076.68920039534,
323.646015709891));
#110048=CARTESIAN_POINT('Ctrl Pts',(-50.7297360052905,1076.71060001064,
323.879894089432));
#110049=CARTESIAN_POINT('Ctrl Pts',(-50.766217518536,1076.72230878929,323.993612070658));
#110050=CARTESIAN_POINT('Ctrl Pts',(-50.8027981187008,1076.75001568232,
324.238868941098));
#110051=CARTESIAN_POINT('Ctrl Pts',(-50.7989166745544,1076.7660952531,324.36918024798));
#110052=CARTESIAN_POINT('Ctrl Pts',(-50.7437470917788,1076.80123169195,
324.632085196037));
#110053=CARTESIAN_POINT('Ctrl Pts',(-50.6892150515513,1076.82011778402,
324.761768185158));
#110054=CARTESIAN_POINT('Ctrl Pts',(-50.5313241389388,1076.85783783144,
324.998003904691));
#110055=CARTESIAN_POINT('Ctrl Pts',(-50.4276394566757,1076.8762899973,325.101269412309));
#110056=CARTESIAN_POINT('Ctrl Pts',(-50.1911036244038,1076.90880622727,
325.257697883359));
#110057=CARTESIAN_POINT('Ctrl Pts',(-50.0618732563135,1076.92274398555,
325.311519480018));
#110058=CARTESIAN_POINT('Ctrl Pts',(-49.8530821577486,1076.94003770994,
325.354668307415));
#110059=CARTESIAN_POINT('Ctrl Pts',(-49.779127659166,1076.94524000737,325.362209063877));
#110060=CARTESIAN_POINT('Ctrl Pts',(-49.7050859019669,1076.94955520377,
325.362209063877));
#110061=CARTESIAN_POINT('',(-86.2232976813461,1076.9124877279,354.254678911709));
#110062=CARTESIAN_POINT('',(-86.223297681347,1076.72560793676,352.073597414254));
#110063=CARTESIAN_POINT('Ctrl Pts',(-86.2232976813464,1076.9124877279,354.254678911711));
#110064=CARTESIAN_POINT('Ctrl Pts',(-86.1106700087104,1076.92394995339,
354.254678911711));
#110065=CARTESIAN_POINT('Ctrl Pts',(-85.9984479843176,1076.93386455963,
354.237230908178));
#110066=CARTESIAN_POINT('Ctrl Pts',(-85.7548899619962,1076.95197767004,
354.159227193133));
#110067=CARTESIAN_POINT('Ctrl Pts',(-85.6287945239059,1076.95886673878,
354.08948200948));
#110068=CARTESIAN_POINT('Ctrl Pts',(-85.4948783902631,1076.96291995683,
353.976378537235));
#110069=CARTESIAN_POINT('Ctrl Pts',(-85.4710647283615,1076.96348255733,
353.954375533283));
#110070=CARTESIAN_POINT('Ctrl Pts',(-85.4338411076001,1076.96409366365,
353.916772045896));
#110071=CARTESIAN_POINT('Ctrl Pts',(-85.4198313036292,1076.96425497713,
353.90179748482));
#110072=CARTESIAN_POINT('Ctrl Pts',(-85.3956531693964,1076.96440748106,
353.8744477722));
#110073=CARTESIAN_POINT('Ctrl Pts',(-85.3853198471695,1076.96442822542,
353.862227221899));
#110074=CARTESIAN_POINT('Ctrl Pts',(-85.3642048128736,1076.96437496735,
353.836111156062));
#110075=CARTESIAN_POINT('Ctrl Pts',(-85.3534829036369,1076.9642914137,353.822173493486));
#110076=CARTESIAN_POINT('Ctrl Pts',(-85.3263966080289,1076.96392829675,
353.785144040836));
#110077=CARTESIAN_POINT('Ctrl Pts',(-85.3105867383334,1076.96356046082,
353.761665037151));
#110078=CARTESIAN_POINT('Ctrl Pts',(-85.2481878537172,1076.96141770149,
353.66073317949));
#110079=CARTESIAN_POINT('Ctrl Pts',(-85.2104303172905,1076.95833556205,
353.578298258425));
#110080=CARTESIAN_POINT('Ctrl Pts',(-85.1510914289845,1076.94858128102,
353.39018380428));
#110081=CARTESIAN_POINT('Ctrl Pts',(-85.134130936169,1076.94140600827,353.284095820838));
#110082=CARTESIAN_POINT('Ctrl Pts',(-85.1313765667379,1076.92258949993,
353.056874669399));
#110083=CARTESIAN_POINT('Ctrl Pts',(-85.1498936083631,1076.91062347989,
352.937155489594));
#110084=CARTESIAN_POINT('Ctrl Pts',(-85.2285473991811,1076.88239895222,
352.698316308956));
#110085=CARTESIAN_POINT('Ctrl Pts',(-85.2917524177404,1076.86606956431,
352.582186930196));
#110086=CARTESIAN_POINT('Ctrl Pts',(-85.4627331970511,1076.8303715638,352.36986520423));
#110087=CARTESIAN_POINT('Ctrl Pts',(-85.5721656192275,1076.81118246124,
352.277940107348));
#110088=CARTESIAN_POINT('Ctrl Pts',(-85.7716420283623,1076.78098194181,
352.167777036374));
#110089=CARTESIAN_POINT('Ctrl Pts',(-85.8519240535133,1076.76980246967,
352.135145175158));
#110090=CARTESIAN_POINT('Ctrl Pts',(-86.0290190547706,1076.74711303435,
352.086648114149));
#110091=CARTESIAN_POINT('Ctrl Pts',(-86.1258876281242,1076.73583360847,
352.073597414254));
#110092=CARTESIAN_POINT('Ctrl Pts',(-86.2232976813471,1076.72560793676,
352.073597414254));
#110093=CARTESIAN_POINT('Ctrl Pts',(-86.2232976813471,1076.72560793676,
352.073597414254));
#110094=CARTESIAN_POINT('Ctrl Pts',(-86.2233382977044,1076.72560367304,
352.073597414254));
#110095=CARTESIAN_POINT('Ctrl Pts',(-86.2233789141559,1076.7255994095,352.073597416523));
#110096=CARTESIAN_POINT('Ctrl Pts',(-86.2234195307013,1076.72559514614,
352.073597421061));
#110097=CARTESIAN_POINT('Ctrl Pts',(-86.352409189064,1076.71205561553,352.073611833463));
#110098=CARTESIAN_POINT('Ctrl Pts',(-86.480575631451,1076.70055082089,352.096511565282));
#110099=CARTESIAN_POINT('Ctrl Pts',(-86.7226974278544,1076.68283928162,
352.186146101408));
#110100=CARTESIAN_POINT('Ctrl Pts',(-86.8347358248615,1076.67675513596,
352.251954646566));
#110101=CARTESIAN_POINT('Ctrl Pts',(-86.9563727615988,1076.6730211201,352.35614840662));
#110102=CARTESIAN_POINT('Ctrl Pts',(-86.9791202646848,1076.67247634619,
352.377385887761));
#110103=CARTESIAN_POINT('Ctrl Pts',(-87.015077807269,1076.67187843216,352.413957831622));
#110104=CARTESIAN_POINT('Ctrl Pts',(-87.0288231641388,1076.67171992704,
352.428736881043));
#110105=CARTESIAN_POINT('Ctrl Pts',(-87.0527719437454,1076.67157337991,
352.455964324506));
#110106=CARTESIAN_POINT('Ctrl Pts',(-87.0631246088755,1076.67155727495,
352.468272892784));
#110107=CARTESIAN_POINT('Ctrl Pts',(-87.0844920994205,1076.67162681896,
352.494848997105));
#110108=CARTESIAN_POINT('Ctrl Pts',(-87.0954328916507,1076.67172494973,
352.509169487017));
#110109=CARTESIAN_POINT('Ctrl Pts',(-87.1235095361551,1076.67214795035,
352.547870804807));
#110110=CARTESIAN_POINT('Ctrl Pts',(-87.1400083324327,1076.67257890375,
352.572692356219));
#110111=CARTESIAN_POINT('Ctrl Pts',(-87.2083307388048,1076.67521734954,
352.685219225984));
#110112=CARTESIAN_POINT('Ctrl Pts',(-87.2486979470708,1076.67918720723,
352.779197400646));
#110113=CARTESIAN_POINT('Ctrl Pts',(-87.3041124358866,1076.69113007012,
352.982485843146));
#110114=CARTESIAN_POINT('Ctrl Pts',(-87.3168160143593,1076.69929810105,
353.091211016504));
#110115=CARTESIAN_POINT('Ctrl Pts',(-87.3092618540888,1076.72018562122,
353.321578436446));
#110116=CARTESIAN_POINT('Ctrl Pts',(-87.2849250164885,1076.73318438117,
353.44157419653));
#110117=CARTESIAN_POINT('Ctrl Pts',(-87.1940484156991,1076.76321716278,
353.678327874337));
#110118=CARTESIAN_POINT('Ctrl Pts',(-87.1246917993476,1076.78026540416,
353.791971853215));
#110119=CARTESIAN_POINT('Ctrl Pts',(-86.9420713038994,1076.81680851671,
353.99653735009));
#110120=CARTESIAN_POINT('Ctrl Pts',(-86.8274306336196,1076.83606112735,
354.08314068069));
#110121=CARTESIAN_POINT('Ctrl Pts',(-86.5699763667257,1076.87316862321,
354.208060979568));
#110122=CARTESIAN_POINT('Ctrl Pts',(-86.429273298908,1076.89066372331,354.244713132033));
#110123=CARTESIAN_POINT('Ctrl Pts',(-86.2646505302865,1076.90822847593,
354.254091272874));
#110124=CARTESIAN_POINT('Ctrl Pts',(-86.2439672746539,1076.9103841637,354.254678911711));
#110125=CARTESIAN_POINT('Ctrl Pts',(-86.2232976813464,1076.9124877279,354.254678911711));
#110126=CARTESIAN_POINT('',(-73.7938092375735,1077.74530255756,351.20352665013));
#110127=CARTESIAN_POINT('',(-73.7938092375734,1077.58420144585,349.005864378145));
#110128=CARTESIAN_POINT('Ctrl Pts',(-73.7938092375746,1077.74530255756,
351.20352665013));
#110129=CARTESIAN_POINT('Ctrl Pts',(-73.769883441808,1077.74699181584,351.20352665013));
#110130=CARTESIAN_POINT('Ctrl Pts',(-73.7459292397079,1077.74862579125,
351.202745233119));
#110131=CARTESIAN_POINT('Ctrl Pts',(-73.5963574879468,1077.75846980289,
351.192947562019));
#110132=CARTESIAN_POINT('Ctrl Pts',(-73.4729823801501,1077.76500962047,
351.163183030474));
#110133=CARTESIAN_POINT('Ctrl Pts',(-73.2807897034584,1077.77257859337,
351.079984154165));
#110134=CARTESIAN_POINT('Ctrl Pts',(-73.2082940154623,1077.77469879822,
351.038267379108));
#110135=CARTESIAN_POINT('Ctrl Pts',(-73.1171602315749,1077.77631811397,
350.970991583833));
#110136=CARTESIAN_POINT('Ctrl Pts',(-73.0938527327019,1077.77662537864,
350.952270758455));
#110137=CARTESIAN_POINT('Ctrl Pts',(-73.0570920529911,1077.77693018526,
350.920192336047));
#110138=CARTESIAN_POINT('Ctrl Pts',(-73.0431706502578,1077.77699998685,
350.907396579794));
#110139=CARTESIAN_POINT('Ctrl Pts',(-73.0170663687754,1077.77704117237,
350.882129741572));
#110140=CARTESIAN_POINT('Ctrl Pts',(-73.0048365783284,1077.77701983436,
350.869715514687));
#110141=CARTESIAN_POINT('Ctrl Pts',(-72.9774240804161,1077.77687641546,
350.84053283029));
#110142=CARTESIAN_POINT('Ctrl Pts',(-72.9624538003779,1077.77672625347,
350.823576154841));
#110143=CARTESIAN_POINT('Ctrl Pts',(-72.9181926212019,1077.77605439756,
350.770208957175));
#110144=CARTESIAN_POINT('Ctrl Pts',(-72.8906943116465,1077.77530803227,
350.732385855732));
#110145=CARTESIAN_POINT('Ctrl Pts',(-72.7876613244233,1077.77103915678,
350.569820296116));
#110146=CARTESIAN_POINT('Ctrl Pts',(-72.7349599947952,1077.76503247187,
350.432497846024));
#110147=CARTESIAN_POINT('Ctrl Pts',(-72.6905343650455,1077.74961804802,
350.171390094682));
#110148=CARTESIAN_POINT('Ctrl Pts',(-72.6898266910601,1077.7411215929,350.051397067388));
#110149=CARTESIAN_POINT('Ctrl Pts',(-72.7286199156512,1077.72071917826,
349.805097050745));
#110150=CARTESIAN_POINT('Ctrl Pts',(-72.7715697705636,1077.7087279905,349.681179983827));
#110151=CARTESIAN_POINT('Ctrl Pts',(-72.9036577589566,1077.68212249008,
349.44535140389));
#110152=CARTESIAN_POINT('Ctrl Pts',(-72.9949871466016,1077.66761155408,
349.337251524034));
#110153=CARTESIAN_POINT('Ctrl Pts',(-73.1930475153763,1077.64141300526,
349.177571599089));
#110154=CARTESIAN_POINT('Ctrl Pts',(-73.2926249391797,1077.62985505809,
349.120162029067));
#110155=CARTESIAN_POINT('Ctrl Pts',(-73.5249284601887,1077.60607322753,
349.030799462205));
#110156=CARTESIAN_POINT('Ctrl Pts',(-73.6584887580826,1077.59429279595,
349.005923538466));
#110157=CARTESIAN_POINT('Ctrl Pts',(-73.7933279877136,1077.58423732673,
349.005864483564));
#110158=CARTESIAN_POINT('Ctrl Pts',(-73.7934884055767,1077.58422536376,
349.005864413307));
#110159=CARTESIAN_POINT('Ctrl Pts',(-73.7936488222002,1077.58421340347,
349.005864378145));
#110160=CARTESIAN_POINT('Ctrl Pts',(-73.7938092375731,1077.58420144585,
349.005864378145));
#110161=CARTESIAN_POINT('Ctrl Pts',(-73.7938092375731,1077.58420144585,
349.005864378145));
#110162=CARTESIAN_POINT('Ctrl Pts',(-73.9127579711805,1077.57533481387,
349.005864378145));
#110163=CARTESIAN_POINT('Ctrl Pts',(-74.0310190634156,1077.56793745143,
349.025178687888));
#110164=CARTESIAN_POINT('Ctrl Pts',(-74.2455312164974,1077.55730474254,
349.097292143534));
#110165=CARTESIAN_POINT('Ctrl Pts',(-74.3416174673074,1077.55378482318,
349.146133172946));
#110166=CARTESIAN_POINT('Ctrl Pts',(-74.4565104103741,1077.55132490339,
349.227550874274));
#110167=CARTESIAN_POINT('Ctrl Pts',(-74.4829840495733,1077.55090110641,
349.248194541628));
#110168=CARTESIAN_POINT('Ctrl Pts',(-74.5235557610025,1077.5504874011,349.282932687793));
#110169=CARTESIAN_POINT('Ctrl Pts',(-74.5382859532575,1077.55039106719,
349.296253449057));
#110170=CARTESIAN_POINT('Ctrl Pts',(-74.5651350068478,1077.55031863291,
349.321889955745));
#110171=CARTESIAN_POINT('Ctrl Pts',(-74.5773399300205,1077.55032849654,
349.334106365208));
#110172=CARTESIAN_POINT('Ctrl Pts',(-74.6040201376241,1077.55044811707,
349.362101151894));
#110173=CARTESIAN_POINT('Ctrl Pts',(-74.6183321234707,1077.55058123348,
349.378024980907));
#110174=CARTESIAN_POINT('Ctrl Pts',(-74.6583278629841,1077.55115878459,
349.425228967539));
#110175=CARTESIAN_POINT('Ctrl Pts',(-74.6827584932905,1077.55177443679,
349.457520204184));
#110176=CARTESIAN_POINT('Ctrl Pts',(-74.7871426080836,1077.5557028426,349.612585944698));
#110177=CARTESIAN_POINT('Ctrl Pts',(-74.8437562329453,1077.56181743687,
349.74912510091));
#110178=CARTESIAN_POINT('Ctrl Pts',(-74.8947463291063,1077.57759525021,
350.008361242852));
#110179=CARTESIAN_POINT('Ctrl Pts',(-74.8987087697233,1077.58623671196,
350.126908186342));
#110180=CARTESIAN_POINT('Ctrl Pts',(-74.8675109748959,1077.60689739488,
350.371513308744));
#110181=CARTESIAN_POINT('Ctrl Pts',(-74.8288765795316,1077.6189981894,350.495357450571));
#110182=CARTESIAN_POINT('Ctrl Pts',(-74.7060680826829,1077.64561586336,
350.732728466384));
#110183=CARTESIAN_POINT('Ctrl Pts',(-74.619665487082,1077.66001512009,350.842660302186));
#110184=CARTESIAN_POINT('Ctrl Pts',(-74.4051459038507,1077.68919424678,
351.029333606172));
#110185=CARTESIAN_POINT('Ctrl Pts',(-74.2771371650477,1077.70367560779,
351.10225761206));
#110186=CARTESIAN_POINT('Ctrl Pts',(-74.0272615767765,1077.72744772394,
351.184818012273));
#110187=CARTESIAN_POINT('Ctrl Pts',(-73.9108754585647,1077.73703720726,
351.20352665013));
#110188=CARTESIAN_POINT('Ctrl Pts',(-73.7938092375746,1077.74530255756,
351.20352665013));
#110189=CARTESIAN_POINT('',(-61.0059658728168,1078.41010379242,350.825616616696));
#110190=CARTESIAN_POINT('',(-61.0059658728168,1078.28342170814,348.274728374424));
#110191=CARTESIAN_POINT('Ctrl Pts',(-61.0059658728173,1078.41010379242,
350.825616616696));
#110192=CARTESIAN_POINT('Ctrl Pts',(-60.9835823540215,1078.4109445386,350.825616616696));
#110193=CARTESIAN_POINT('Ctrl Pts',(-60.9611778050674,1078.41175745992,
350.82502739226));
#110194=CARTESIAN_POINT('Ctrl Pts',(-60.7774291209768,1078.4181906595,350.815334014705));
#110195=CARTESIAN_POINT('Ctrl Pts',(-60.6191200404424,1078.42225757925,
350.776238705868));
#110196=CARTESIAN_POINT('Ctrl Pts',(-60.417522270934,1078.42547434699,350.683366845324));
#110197=CARTESIAN_POINT('Ctrl Pts',(-60.3645995731918,1078.42610381919,
350.654276292849));
#110198=CARTESIAN_POINT('Ctrl Pts',(-60.2898907365497,1078.42666702699,
350.606019679417));
#110199=CARTESIAN_POINT('Ctrl Pts',(-60.2663782038122,1078.42679236091,
350.589685355149));
#110200=CARTESIAN_POINT('Ctrl Pts',(-60.2256708122253,1078.42691530777,
350.559324824838));
#110201=CARTESIAN_POINT('Ctrl Pts',(-60.2082549415685,1078.42693534259,
350.54561515021));
#110202=CARTESIAN_POINT('Ctrl Pts',(-60.1729253108439,1078.42690717166,
350.516280999461));
#110203=CARTESIAN_POINT('Ctrl Pts',(-60.1550732490697,1078.42685394484,
350.500595535313));
#110204=CARTESIAN_POINT('Ctrl Pts',(-60.1106345171936,1078.42661943572,
350.4592939022));
#110205=CARTESIAN_POINT('Ctrl Pts',(-60.0847030480664,1078.42638370712,
350.433005826605));
#110206=CARTESIAN_POINT('Ctrl Pts',(-59.9880853087506,1078.42510201004,
350.326160112222));
#110207=CARTESIAN_POINT('Ctrl Pts',(-59.9265296506684,1078.42337392092,
350.237958763876));
#110208=CARTESIAN_POINT('Ctrl Pts',(-59.8175059324121,1078.4179504817,350.030328345937));
#110209=CARTESIAN_POINT('Ctrl Pts',(-59.7755270796808,1078.41397518225,
349.909327053499));
#110210=CARTESIAN_POINT('Ctrl Pts',(-59.7260766921979,1078.40357100613,
349.644345582651));
#110211=CARTESIAN_POINT('Ctrl Pts',(-59.7235613141722,1078.39698103055,
349.501198818696));
#110212=CARTESIAN_POINT('Ctrl Pts',(-59.767580262996,1078.38138883551,349.208261623922));
#110213=CARTESIAN_POINT('Ctrl Pts',(-59.8178971668436,1078.37235536533,
349.061327112453));
#110214=CARTESIAN_POINT('Ctrl Pts',(-59.9740915904031,1078.35249506362,
348.782427503392));
#110215=CARTESIAN_POINT('Ctrl Pts',(-60.0824132468098,1078.34176895436,
348.655051228122));
#110216=CARTESIAN_POINT('Ctrl Pts',(-60.3125778170563,1078.32303443442,
348.471993008598));
#110217=CARTESIAN_POINT('Ctrl Pts',(-60.4246332309683,1078.31506405064,
348.407665841913));
#110218=CARTESIAN_POINT('Ctrl Pts',(-60.6915389098853,1078.29845566072,
348.304059259342));
#110219=CARTESIAN_POINT('Ctrl Pts',(-60.8480392077451,1078.29022370571,
348.274728374424));
#110220=CARTESIAN_POINT('Ctrl Pts',(-61.0059658728168,1078.28342170814,
348.274728374424));
#110221=CARTESIAN_POINT('Ctrl Pts',(-61.0059658728168,1078.28342170814,
348.274728374424));
#110222=CARTESIAN_POINT('Ctrl Pts',(-61.0059827805808,1078.28342097991,
348.274728374424));
#110223=CARTESIAN_POINT('Ctrl Pts',(-61.005999688361,1078.2834202517,348.27472837476));
#110224=CARTESIAN_POINT('Ctrl Pts',(-61.0060165961576,1078.2834195235,348.274728375433));
#110225=CARTESIAN_POINT('Ctrl Pts',(-61.1593590601562,1078.27681528043,
348.274734473733));
#110226=CARTESIAN_POINT('Ctrl Pts',(-61.3115017102687,1078.27167170399,
348.3023941924));
#110227=CARTESIAN_POINT('Ctrl Pts',(-61.5294609256413,1078.26656243912,
348.384402300238));
#110228=CARTESIAN_POINT('Ctrl Pts',(-61.6010368702449,1078.26530680575,
348.419261274088));
#110229=CARTESIAN_POINT('Ctrl Pts',(-61.6976455193526,1078.26424351022,
348.478039852353));
#110230=CARTESIAN_POINT('Ctrl Pts',(-61.7256791657564,1078.26401878458,
348.496653631182));
#110231=CARTESIAN_POINT('Ctrl Pts',(-61.7698763406202,1078.26380403625,
348.528588013559));
#110232=CARTESIAN_POINT('Ctrl Pts',(-61.786505005854,1078.26375737109,348.541236062661));
#110233=CARTESIAN_POINT('Ctrl Pts',(-61.8204282979527,1078.26373448169,
348.568379505588));
#110234=CARTESIAN_POINT('Ctrl Pts',(-61.837664018575,1078.26376418286,348.582936894935));
#110235=CARTESIAN_POINT('Ctrl Pts',(-61.8771322488985,1078.26393115545,
348.618107348569));
#110236=CARTESIAN_POINT('Ctrl Pts',(-61.8990337049147,1078.2641018342,348.63907091478));
#110237=CARTESIAN_POINT('Ctrl Pts',(-61.9663995201969,1078.26488343763,
348.708316966918));
#110238=CARTESIAN_POINT('Ctrl Pts',(-62.0088525833007,1078.26577538336,
348.75936876583));
#110239=CARTESIAN_POINT('Ctrl Pts',(-62.1453593331114,1078.27018473839,
348.952296518979));
#110240=CARTESIAN_POINT('Ctrl Pts',(-62.2147952713521,1078.27558502052,
349.109304819584));
#110241=CARTESIAN_POINT('Ctrl Pts',(-62.2816741097721,1078.28876876373,
349.412265919201));
#110242=CARTESIAN_POINT('Ctrl Pts',(-62.289092421718,1078.29588005414,349.553304160252));
#110243=CARTESIAN_POINT('Ctrl Pts',(-62.2564400197717,1078.31236588406,
349.843752420324));
#110244=CARTESIAN_POINT('Ctrl Pts',(-62.2125777372731,1078.32174712249,
349.990562260382));
#110245=CARTESIAN_POINT('Ctrl Pts',(-62.0702790979688,1078.34182755987,
350.271701058825));
#110246=CARTESIAN_POINT('Ctrl Pts',(-61.9693691942809,1078.35238824387,
350.401774119559));
#110247=CARTESIAN_POINT('Ctrl Pts',(-61.7200869783476,1078.37300097648,
350.620281009542));
#110248=CARTESIAN_POINT('Ctrl Pts',(-61.572718682285,1078.38282673004,350.705129347727));
#110249=CARTESIAN_POINT('Ctrl Pts',(-61.2817936853834,1078.39865035328,
350.803115988936));
#110250=CARTESIAN_POINT('Ctrl Pts',(-61.1442812981844,1078.40490853391,
350.825616616696));
#110251=CARTESIAN_POINT('Ctrl Pts',(-61.0059658728173,1078.41010379242,
350.825616616696));
#110252=CARTESIAN_POINT('',(-49.361641103754,1078.70098643656,351.371678279531));
#110253=CARTESIAN_POINT('',(-49.3616411037539,1078.63750051791,348.415072015145));
#110254=CARTESIAN_POINT('Ctrl Pts',(-49.361641103754,1078.70098643656,351.371678279532));
#110255=CARTESIAN_POINT('Ctrl Pts',(-49.2474022975557,1078.70218551221,
351.371678279532));
#110256=CARTESIAN_POINT('Ctrl Pts',(-49.1333327929675,1078.70313956229,
351.358435789987));
#110257=CARTESIAN_POINT('Ctrl Pts',(-48.9242447656558,1078.70448454113,
351.309037947563));
#110258=CARTESIAN_POINT('Ctrl Pts',(-48.8293388095697,1078.70492697835,
351.276151812854));
#110259=CARTESIAN_POINT('Ctrl Pts',(-48.6999965585767,1078.70530180718,
351.216027256903));
#110260=CARTESIAN_POINT('Ctrl Pts',(-48.6622913268644,1078.7053809091,351.196483740757));
#110261=CARTESIAN_POINT('Ctrl Pts',(-48.6026699313023,1078.70545678433,
351.162246594364));
#110262=CARTESIAN_POINT('Ctrl Pts',(-48.5802140089712,1078.70547340844,
351.148541943398));
#110263=CARTESIAN_POINT('Ctrl Pts',(-48.534367693116,1078.70548220577,351.118854907875));
#110264=CARTESIAN_POINT('Ctrl Pts',(-48.5110467815598,1078.7054724093,351.10278460562));
#110265=CARTESIAN_POINT('Ctrl Pts',(-48.4576823902483,1078.70541596183,
351.063704064073));
#110266=CARTESIAN_POINT('Ctrl Pts',(-48.4280320949426,1078.70535806403,
351.040190451367));
#110267=CARTESIAN_POINT('Ctrl Pts',(-48.3374601039413,1078.7050942927,350.962521228007));
#110268=CARTESIAN_POINT('Ctrl Pts',(-48.2800956207935,1078.70479548163,
350.904453426482));
#110269=CARTESIAN_POINT('Ctrl Pts',(-48.1016976331506,1078.70336224855,
350.69121564366));
#110270=CARTESIAN_POINT('Ctrl Pts',(-48.0069076523202,1078.70166332956,
350.516832914347));
#110271=CARTESIAN_POINT('Ctrl Pts',(-47.900552771282,1078.69718193973,350.171972083686));
#110272=CARTESIAN_POINT('Ctrl Pts',(-47.8786484309515,1078.69464832435,
350.007931932167));
#110273=CARTESIAN_POINT('Ctrl Pts',(-47.8901581205458,1078.68834019769,
349.665765819091));
#110274=CARTESIAN_POINT('Ctrl Pts',(-47.9282280257163,1078.68452704653,
349.490401141928));
#110275=CARTESIAN_POINT('Ctrl Pts',(-48.0699098465574,1078.67571466901,
349.149491228314));
#110276=CARTESIAN_POINT('Ctrl Pts',(-48.1768371093475,1078.67072843342,
348.988849273787));
#110277=CARTESIAN_POINT('Ctrl Pts',(-48.4308943937773,1078.66105421524,
348.732369328139));
#110278=CARTESIAN_POINT('Ctrl Pts',(-48.5703201797615,1078.6564704628,348.633201775985));
#110279=CARTESIAN_POINT('Ctrl Pts',(-48.8124860674955,1078.64961844272,
348.517317059492));
#110280=CARTESIAN_POINT('Ctrl Pts',(-48.9054902156945,1078.64720357858,
348.483752957437));
#110281=CARTESIAN_POINT('Ctrl Pts',(-49.1189409154863,1078.642172311,348.430080862271));
#110282=CARTESIAN_POINT('Ctrl Pts',(-49.2399464028628,1078.63965826912,
348.415090001983));
#110283=CARTESIAN_POINT('Ctrl Pts',(-49.3614224096618,1078.63750439515,
348.415072031322));
#110284=CARTESIAN_POINT('Ctrl Pts',(-49.3614953079448,1078.6375031026,348.415072020537));
#110285=CARTESIAN_POINT('Ctrl Pts',(-49.3615682059758,1078.63750181019,
348.415072015145));
#110286=CARTESIAN_POINT('Ctrl Pts',(-49.3616411037539,1078.63750051791,
348.415072015145));
#110287=CARTESIAN_POINT('Ctrl Pts',(-49.3616411037539,1078.63750051791,
348.415072015145));
#110288=CARTESIAN_POINT('Ctrl Pts',(-49.5473794481685,1078.63420789306,
348.415072015145));
#110289=CARTESIAN_POINT('Ctrl Pts',(-49.7314770144804,1078.63181126302,
348.450076940995));
#110290=CARTESIAN_POINT('Ctrl Pts',(-49.9566522384781,1078.63015111076,
348.53893333064));
#110291=CARTESIAN_POINT('Ctrl Pts',(-50.0078076303818,1078.62986890781,
348.562578460187));
#110292=CARTESIAN_POINT('Ctrl Pts',(-50.086610561338,1078.62959029906,348.604620384083));
#110293=CARTESIAN_POINT('Ctrl Pts',(-50.1152030772046,1078.62952401153,
348.621127562959));
#110294=CARTESIAN_POINT('Ctrl Pts',(-50.1647507719704,1078.62947200173,
348.651989432685));
#110295=CARTESIAN_POINT('Ctrl Pts',(-50.1859336821702,1078.62947119004,
348.665952898537));
#110296=CARTESIAN_POINT('Ctrl Pts',(-50.233484907002,1078.62951912204,348.69908434006));
#110297=CARTESIAN_POINT('Ctrl Pts',(-50.2595996327525,1078.62958202898,
348.718593201347));
#110298=CARTESIAN_POINT('Ctrl Pts',(-50.3287621158506,1078.62985018255,
348.773915172431));
#110299=CARTESIAN_POINT('Ctrl Pts',(-50.3704543160287,1078.630125015,348.811335648915));
#110300=CARTESIAN_POINT('Ctrl Pts',(-50.5483957383052,1078.63182779745,
348.990290557874));
#110301=CARTESIAN_POINT('Ctrl Pts',(-50.6577288698742,1078.63440940937,
349.155747720034));
#110302=CARTESIAN_POINT('Ctrl Pts',(-50.7914599112017,1078.64087156722,
349.485437812721));
#110303=CARTESIAN_POINT('Ctrl Pts',(-50.8270896083253,1078.64436959382,
349.641881746109));
#110304=CARTESIAN_POINT('Ctrl Pts',(-50.847880572619,1078.65244966803,349.973843595793));
#110305=CARTESIAN_POINT('Ctrl Pts',(-50.8282401499088,1078.6570331927,350.147277574448));
#110306=CARTESIAN_POINT('Ctrl Pts',(-50.7262824892511,1078.66666845342,
350.491384812048));
#110307=CARTESIAN_POINT('Ctrl Pts',(-50.6404515340994,1078.67164038373,
350.657906846764));
#110308=CARTESIAN_POINT('Ctrl Pts',(-50.4055947837767,1078.68120425931,
350.958155708281));
#110309=CARTESIAN_POINT('Ctrl Pts',(-50.2557877467823,1078.68566765131,
351.086734958728));
#110310=CARTESIAN_POINT('Ctrl Pts',(-49.9194397133287,1078.69326155037,
351.275554836402));
#110311=CARTESIAN_POINT('Ctrl Pts',(-49.7371470374138,1078.69636009907,
351.335790823846));
#110312=CARTESIAN_POINT('Ctrl Pts',(-49.4863747495536,1078.69960458914,
351.367734830859));
#110313=CARTESIAN_POINT('Ctrl Pts',(-49.4239827183277,1078.70033208525,
351.371678279532));
#110314=CARTESIAN_POINT('Ctrl Pts',(-49.361641103754,1078.70098643656,351.371678279532));
#110315=CARTESIAN_POINT('',(-32.7463814565112,1078.70364178837,342.741777359158));
#110316=CARTESIAN_POINT('',(-32.7463814565112,1078.63286818763,339.785171094771));
#110317=CARTESIAN_POINT('Ctrl Pts',(-32.7463814565111,1078.70364178837,
342.741777359158));
#110318=CARTESIAN_POINT('Ctrl Pts',(-32.6713741841051,1078.70414194159,
342.741777359158));
#110319=CARTESIAN_POINT('Ctrl Pts',(-32.5963229919856,1078.70453928808,
342.736068777415));
#110320=CARTESIAN_POINT('Ctrl Pts',(-32.4619676045483,1078.70507352558,
342.715425854039));
#110321=CARTESIAN_POINT('Ctrl Pts',(-32.4026747646749,1078.70524517308,
342.702543552129));
#110322=CARTESIAN_POINT('Ctrl Pts',(-32.3096229810331,1078.70541410201,
342.676245888326));
#110323=CARTESIAN_POINT('Ctrl Pts',(-32.2752761282601,1078.70545376002,
342.665166599314));
#110324=CARTESIAN_POINT('Ctrl Pts',(-32.2116579431705,1078.70548445708,
342.642042431627));
#110325=CARTESIAN_POINT('Ctrl Pts',(-32.182300878416,1078.70548089485,342.630292661137));
#110326=CARTESIAN_POINT('Ctrl Pts',(-32.1179106121875,1078.70543316383,
342.60209321987));
#110327=CARTESIAN_POINT('Ctrl Pts',(-32.0831007842742,1078.70538011837,
342.585190972261));
#110328=CARTESIAN_POINT('Ctrl Pts',(-31.9856063501934,1078.70515161973,
342.533029089356));
#110329=CARTESIAN_POINT('Ctrl Pts',(-31.924777075105,1078.70491063053,342.494536557997));
#110330=CARTESIAN_POINT('Ctrl Pts',(-31.7089434112895,1078.70365917325,
342.334810492918));
#110331=CARTESIAN_POINT('Ctrl Pts',(-31.5758117086972,1078.70205794374,
342.187487834967));
#110332=CARTESIAN_POINT('Ctrl Pts',(-31.391956447934,1078.69776982643,341.877974582164));
#110333=CARTESIAN_POINT('Ctrl Pts',(-31.3323784881597,1078.69533634405,
341.724634479672));
#110334=CARTESIAN_POINT('Ctrl Pts',(-31.2630177903554,1078.6892374063,341.391358707963));
#110335=CARTESIAN_POINT('Ctrl Pts',(-31.2583746289087,1078.68553075741,
341.21296768739));
#110336=CARTESIAN_POINT('Ctrl Pts',(-31.3143545559451,1078.67691354353,
340.850199183331));
#110337=CARTESIAN_POINT('Ctrl Pts',(-31.3792849734701,1078.67201134558,
340.669724489054));
#110338=CARTESIAN_POINT('Ctrl Pts',(-31.5763580872497,1078.66173191616,
340.339144076358));
#110339=CARTESIAN_POINT('Ctrl Pts',(-31.7082342479793,1078.65644880894,
340.193150117647));
#110340=CARTESIAN_POINT('Ctrl Pts',(-31.9687313552379,1078.64821972667,
339.999565526789));
#110341=CARTESIAN_POINT('Ctrl Pts',(-32.0825776364142,1078.64512142403,
339.936231817622));
#110342=CARTESIAN_POINT('Ctrl Pts',(-32.3761475540104,1078.63836207686,
339.820257205896));
#110343=CARTESIAN_POINT('Ctrl Pts',(-32.5604271771752,1078.63510338789,
339.785171133029));
#110344=CARTESIAN_POINT('Ctrl Pts',(-32.7463811523675,1078.63286819129,
339.785171094771));
#110345=CARTESIAN_POINT('Ctrl Pts',(-32.7463814565112,1078.63286818763,
339.785171094771));
#110346=CARTESIAN_POINT('Ctrl Pts',(-32.8530886027707,1078.63158555127,
339.785171094771));
#110347=CARTESIAN_POINT('Ctrl Pts',(-32.9594854136948,1078.63064964381,
339.796724557869));
#110348=CARTESIAN_POINT('Ctrl Pts',(-33.1088409688472,1078.6298487241,339.829550125131));
#110349=CARTESIAN_POINT('Ctrl Pts',(-33.1534811476541,1078.62967771178,
339.841579322797));
#110350=CARTESIAN_POINT('Ctrl Pts',(-33.2287139910778,1078.62950852057,
339.865686373331));
#110351=CARTESIAN_POINT('Ctrl Pts',(-33.2596017028888,1078.62947461875,
339.876729642869));
#110352=CARTESIAN_POINT('Ctrl Pts',(-33.3212695504499,1078.62947974259,
339.901120527232));
#110353=CARTESIAN_POINT('Ctrl Pts',(-33.3520140885504,1078.62952040567,
339.914506831955));
#110354=CARTESIAN_POINT('Ctrl Pts',(-33.4257326566979,1078.6297118798,339.949632817897));
#110355=CARTESIAN_POINT('Ctrl Pts',(-33.4681508808316,1078.62990288704,
339.972448998294));
#110356=CARTESIAN_POINT('Ctrl Pts',(-33.6098470881348,1078.63082348223,
340.057834916935));
#110357=CARTESIAN_POINT('Ctrl Pts',(-33.7027488075639,1078.63193031958,
340.130116966911));
#110358=CARTESIAN_POINT('Ctrl Pts',(-33.8919236819845,1078.63537423128,
340.317290290093));
#110359=CARTESIAN_POINT('Ctrl Pts',(-33.9813026029615,1078.63794233502,
340.437341501565));
#110360=CARTESIAN_POINT('Ctrl Pts',(-34.1286422639572,1078.64438118988,
340.714059363595));
#110361=CARTESIAN_POINT('Ctrl Pts',(-34.1812054568531,1078.64831415834,
340.871331955417));
#110362=CARTESIAN_POINT('Ctrl Pts',(-34.2343278454567,1078.65708324425,
341.209410210286));
#110363=CARTESIAN_POINT('Ctrl Pts',(-34.2300629536692,1078.66189057828,
341.388353896305));
#110364=CARTESIAN_POINT('Ctrl Pts',(-34.1557398972309,1078.67172127567,
341.748512799217));
#110365=CARTESIAN_POINT('Ctrl Pts',(-34.0817114907015,1078.67664045421,
341.92563206815));
#110366=CARTESIAN_POINT('Ctrl Pts',(-33.8681204439433,1078.68571166209,
342.245807905333));
#110367=CARTESIAN_POINT('Ctrl Pts',(-33.7291470577312,1078.68975641055,
342.384838922209));
#110368=CARTESIAN_POINT('Ctrl Pts',(-33.4132957289521,1078.69637206328,
342.595712884842));
#110369=CARTESIAN_POINT('Ctrl Pts',(-33.2414233519641,1078.69895403983,
342.668669691896));
#110370=CARTESIAN_POINT('Ctrl Pts',(-32.9571302673294,1078.70203309239,
342.730501098562));
#110371=CARTESIAN_POINT('Ctrl Pts',(-32.8517992372279,1078.70293885596,
342.741777359158));
#110372=CARTESIAN_POINT('Ctrl Pts',(-32.7463814565111,1078.70364178837,
342.741777359158));
#110373=CARTESIAN_POINT('Origin',(0.,1121.00270384563,424.620242579854));
#110374=CARTESIAN_POINT('',(0.,1120.6032985308,433.13766592946));
#110375=CARTESIAN_POINT('Origin',(0.,1120.6032985308,424.620242579854));
#110376=CARTESIAN_POINT('',(-1.07991983210742E-15,1121.50270384563,433.438457210059));
#110377=CARTESIAN_POINT('Origin',(-1.07991983210742E-15,1121.00270384563,
433.438457210059));
#110378=CARTESIAN_POINT('Origin',(0.,1121.50270384563,424.620242579854));
#110379=CARTESIAN_POINT('Origin',(-96.6088930673541,1067.7251047501,419.724828926582));
#110380=CARTESIAN_POINT('',(-96.6088930673714,1076.34045666952,418.449384805446));
#110381=CARTESIAN_POINT('',(-96.6088930673541,1067.7251047501,418.449384805446));
#110382=CARTESIAN_POINT('Ctrl Pts',(-96.6091111714779,1076.34879426825,
421.00027302907));
#110383=CARTESIAN_POINT('Ctrl Pts',(-96.6934658979017,1076.34336808336,
421.000258604201));
#110384=CARTESIAN_POINT('Ctrl Pts',(-96.7776101869679,1076.33788022423,
420.991875696778));
#110385=CARTESIAN_POINT('Ctrl Pts',(-97.0246046251495,1076.32155185089,
420.942214030049));
#110386=CARTESIAN_POINT('Ctrl Pts',(-97.1808249622019,1076.31092564066,
420.877113178739));
#110387=CARTESIAN_POINT('Ctrl Pts',(-97.4590385965904,1076.29151215733,
420.690261995754));
#110388=CARTESIAN_POINT('Ctrl Pts',(-97.578386193813,1076.28291423195,420.570367896947));
#110389=CARTESIAN_POINT('Ctrl Pts',(-97.7636848388148,1076.2691425121,420.291538056674));
#110390=CARTESIAN_POINT('Ctrl Pts',(-97.8279726351012,1076.26409798675,
420.135421129003));
#110391=CARTESIAN_POINT('Ctrl Pts',(-97.8925180619294,1076.25842139181,
419.807694921063));
#110392=CARTESIAN_POINT('Ctrl Pts',(-97.8923486646185,1076.25783277121,
419.639350332658));
#110393=CARTESIAN_POINT('Ctrl Pts',(-97.8272870029328,1076.26123041105,
419.312532654493));
#110394=CARTESIAN_POINT('Ctrl Pts',(-97.7631404829371,1076.26517449256,
419.157242625782));
#110395=CARTESIAN_POINT('Ctrl Pts',(-97.5788022868022,1076.27698529881,
418.879974273196));
#110396=CARTESIAN_POINT('Ctrl Pts',(-97.4603375294596,1076.28473799535,
418.760722871916));
#110397=CARTESIAN_POINT('Ctrl Pts',(-97.184031603033,1076.30287163333,418.574250135011));
#110398=CARTESIAN_POINT('Ctrl Pts',(-97.0287317697544,1076.31308155743,
418.50896656265));
#110399=CARTESIAN_POINT('Ctrl Pts',(-96.7835295820195,1076.32910110253,
418.458641213602));
#110400=CARTESIAN_POINT('Ctrl Pts',(-96.7002900684221,1076.33452396562,
418.449926958333));
#110401=CARTESIAN_POINT('Ctrl Pts',(-96.5334138301987,1076.34535623463,
418.448892315101));
#110402=CARTESIAN_POINT('Ctrl Pts',(-96.450172515565,1076.35073999321,418.456554280965));
#110403=CARTESIAN_POINT('Ctrl Pts',(-96.202237145488,1076.36671788244,418.504184046656));
#110404=CARTESIAN_POINT('Ctrl Pts',(-96.0441417310531,1076.3768219841,418.568787674226));
#110405=CARTESIAN_POINT('Ctrl Pts',(-95.7628312524325,1076.39475610547,
418.755631963734));
#110406=CARTESIAN_POINT('Ctrl Pts',(-95.6422513989531,1076.40242267967,
418.875824267539));
#110407=CARTESIAN_POINT('Ctrl Pts',(-95.4545203116411,1076.41453184978,
419.15667837884));
#110408=CARTESIAN_POINT('Ctrl Pts',(-95.389402564051,1076.41884917017,419.314653376189));
#110409=CARTESIAN_POINT('Ctrl Pts',(-95.3245375004729,1076.4236669704,419.647371493635));
#110410=CARTESIAN_POINT('Ctrl Pts',(-95.3256387503052,1076.42411022557,
419.81879984222));
#110411=CARTESIAN_POINT('Ctrl Pts',(-95.394816262567,1076.42102943628,420.150827440191));
#110412=CARTESIAN_POINT('Ctrl Pts',(-95.4620611281913,1076.41754260207,
420.308103464037));
#110413=CARTESIAN_POINT('Ctrl Pts',(-95.653643033737,1076.40695423484,420.586643512474));
#110414=CARTESIAN_POINT('Ctrl Pts',(-95.7758659371814,1076.39996626672,
420.705263612867));
#110415=CARTESIAN_POINT('Ctrl Pts',(-96.0595238157265,1076.3831610753,420.888225198292));
#110416=CARTESIAN_POINT('Ctrl Pts',(-96.2182291908095,1076.37349975092,
420.950652212279));
#110417=CARTESIAN_POINT('Ctrl Pts',(-96.4585900798052,1076.35841675149,
420.993624920888));
#110418=CARTESIAN_POINT('Ctrl Pts',(-96.5337802450701,1076.35363999001,
421.000285910846));
#110419=CARTESIAN_POINT('Ctrl Pts',(-96.6091111714779,1076.34879426825,
421.00027302907));
#110420=CARTESIAN_POINT('Origin',(-96.6088930673541,1067.7251047501,419.724828926582));
#110421=CARTESIAN_POINT('',(-96.6088930673541,1076.34724098047,420.400273047718));
#110422=CARTESIAN_POINT('',(-96.6088930673541,1076.34281999372,419.049384805446));
#110423=CARTESIAN_POINT('Ctrl Pts',(-96.6088930673539,1076.34724098048,
420.400273047718));
#110424=CARTESIAN_POINT('Ctrl Pts',(-96.6630013691699,1076.34375464799,
420.400273047718));
#110425=CARTESIAN_POINT('Ctrl Pts',(-96.7170432733172,1076.34023157328,
420.393771073853));
#110426=CARTESIAN_POINT('Ctrl Pts',(-96.8568536895203,1076.3310097968,420.359468532486));
#110427=CARTESIAN_POINT('Ctrl Pts',(-96.9387782122827,1076.32549269668,
420.321013241726));
#110428=CARTESIAN_POINT('Ctrl Pts',(-97.0820158891483,1076.31565002899,
420.21495872601));
#110429=CARTESIAN_POINT('Ctrl Pts',(-97.1421790804019,1076.31140735321,
420.148728473975));
#110430=CARTESIAN_POINT('Ctrl Pts',(-97.2333937131289,1076.30477649208,
419.996938823552));
#110431=CARTESIAN_POINT('Ctrl Pts',(-97.263630432367,1076.30244937286,419.912906040649));
#110432=CARTESIAN_POINT('Ctrl Pts',(-97.2899522751061,1076.30007551188,
419.738113677132));
#110433=CARTESIAN_POINT('Ctrl Pts',(-97.2858573195978,1076.30004731371,
419.64908162663));
#110434=CARTESIAN_POINT('Ctrl Pts',(-97.243660907243,1076.3023088206,419.47768620825));
#110435=CARTESIAN_POINT('Ctrl Pts',(-97.2059913611933,1076.30457463278,
419.396995971581));
#110436=CARTESIAN_POINT('Ctrl Pts',(-97.1017281190888,1076.31108244457,
419.254573937871));
#110437=CARTESIAN_POINT('Ctrl Pts',(-97.0361007336843,1076.31526324838,
419.194256128484));
#110438=CARTESIAN_POINT('Ctrl Pts',(-96.8852372927702,1076.32495029318,
419.10218282481));
#110439=CARTESIAN_POINT('Ctrl Pts',(-96.8014020866585,1076.33036553896,
419.071386849031));
#110440=CARTESIAN_POINT('Ctrl Pts',(-96.6792674609004,1076.33826497715,
419.052139225811));
#110441=CARTESIAN_POINT('Ctrl Pts',(-96.6441196379992,1076.34053956284,
419.049386150044));
#110442=CARTESIAN_POINT('Ctrl Pts',(-96.6089188583591,1076.34281832411,
419.049384805945));
#110443=CARTESIAN_POINT('Ctrl Pts',(-96.6089102613534,1076.34281888064,
419.049384805617));
#110444=CARTESIAN_POINT('Ctrl Pts',(-96.6089016643518,1076.34281943718,
419.049384805446));
#110445=CARTESIAN_POINT('Ctrl Pts',(-96.6088930673541,1076.34281999372,
419.049384805446));
#110446=CARTESIAN_POINT('',(-96.6088930673541,1082.7251047501,419.049384805446));
#110447=CARTESIAN_POINT('',(-96.6088930673541,1067.7251047501,419.049384805446));
#110448=CARTESIAN_POINT('Origin',(-96.6088930673541,1082.7251047501,419.724828926582));
#110449=CARTESIAN_POINT('Ctrl Pts',(-96.6088930673541,1076.34281999372,
419.049384805446));
#110450=CARTESIAN_POINT('Ctrl Pts',(-96.5647749711265,1076.34567602779,
419.049384805446));
#110451=CARTESIAN_POINT('Ctrl Pts',(-96.5207611365838,1076.3485264382,419.053707309114));
#110452=CARTESIAN_POINT('Ctrl Pts',(-96.3893344285309,1076.35704212704,
419.079774994987));
#110453=CARTESIAN_POINT('Ctrl Pts',(-96.3055315220453,1076.36247676985,
419.114680582747));
#110454=CARTESIAN_POINT('Ctrl Pts',(-96.1566135189695,1076.3721827834,419.215198003661));
#110455=CARTESIAN_POINT('Ctrl Pts',(-96.0929422216552,1076.37636121942,
419.279758926146));
#110456=CARTESIAN_POINT('Ctrl Pts',(-95.9944757732211,1076.38295249723,
419.430191596767));
#110457=CARTESIAN_POINT('Ctrl Pts',(-95.9607219633189,1076.38529735789,
419.51458425605));
#110458=CARTESIAN_POINT('Ctrl Pts',(-95.9282585263141,1076.3878511197,419.691815258127));
#110459=CARTESIAN_POINT('Ctrl Pts',(-95.9299334347195,1076.38803143259,
419.782862020509));
#110460=CARTESIAN_POINT('Ctrl Pts',(-95.9689054643075,1076.38618059823,
419.958818508899));
#110461=CARTESIAN_POINT('Ctrl Pts',(-96.0057648545025,1076.38417032814,
420.041946979932));
#110462=CARTESIAN_POINT('Ctrl Pts',(-96.1097622097469,1076.37818175468,
420.188687195005));
#110463=CARTESIAN_POINT('Ctrl Pts',(-96.1757946134576,1076.37426617928,
420.250861067473));
#110464=CARTESIAN_POINT('Ctrl Pts',(-96.3283172821437,1076.36498138409,
420.345778970902));
#110465=CARTESIAN_POINT('Ctrl Pts',(-96.4133104738226,1076.35970172009,
420.37754595798));
#110466=CARTESIAN_POINT('Ctrl Pts',(-96.5374317443997,1076.35182760772,
420.397440208269));
#110467=CARTESIAN_POINT('Ctrl Pts',(-96.5731768688769,1076.34954226399,
420.400273047718));
#110468=CARTESIAN_POINT('Ctrl Pts',(-96.6088930673539,1076.34724098048,
420.400273047718));
#110469=CARTESIAN_POINT('Origin',(-103.499585384594,1067.7251047501,407.710811438872));
#110470=CARTESIAN_POINT('',(-103.499585384625,1075.63641735374,406.61198030288));
#110471=CARTESIAN_POINT('',(-103.499585384594,1067.7251047501,406.61198030288));
#110472=CARTESIAN_POINT('Ctrl Pts',(-103.499237229524,1075.67335103125,
408.80964251971));
#110473=CARTESIAN_POINT('Ctrl Pts',(-103.570842938863,1075.66603801704,
408.809665207356));
#110474=CARTESIAN_POINT('Ctrl Pts',(-103.642272130286,1075.65859878446,
408.80268854293));
#110475=CARTESIAN_POINT('Ctrl Pts',(-103.857312099209,1075.63575788223,
408.760215201832));
#110476=CARTESIAN_POINT('Ctrl Pts',(-103.994938595762,1075.62050843749,
408.702716643784));
#110477=CARTESIAN_POINT('Ctrl Pts',(-104.236668660875,1075.59247150676,
408.538474848238));
#110478=CARTESIAN_POINT('Ctrl Pts',(-104.339136961286,1075.57990651222,
408.434379507201));
#110479=CARTESIAN_POINT('Ctrl Pts',(-104.497456465949,1075.55902288678,
408.192895957227));
#110480=CARTESIAN_POINT('Ctrl Pts',(-104.55203586182,1075.55088577264,408.058053343401));
#110481=CARTESIAN_POINT('Ctrl Pts',(-104.605830509118,1075.54025643221,
407.775581124673));
#110482=CARTESIAN_POINT('Ctrl Pts',(-104.604847733568,1075.53783727971,
407.630841402448));
#110483=CARTESIAN_POINT('Ctrl Pts',(-104.547371063327,1075.53907653389,
407.350209343589));
#110484=CARTESIAN_POINT('Ctrl Pts',(-104.491602637381,1075.5427058224,407.217099347191));
#110485=CARTESIAN_POINT('Ctrl Pts',(-104.332126057741,1075.55552449156,
406.979489664524));
#110486=CARTESIAN_POINT('Ctrl Pts',(-104.229872213046,1075.56459934331,
406.877410552782));
#110487=CARTESIAN_POINT('Ctrl Pts',(-103.991532047764,1075.58696970732,
406.71777712761));
#110488=CARTESIAN_POINT('Ctrl Pts',(-103.857541658741,1075.60007222497,
406.662038734679));
#110489=CARTESIAN_POINT('Ctrl Pts',(-103.646058401863,1075.62136958147,
406.619401133722));
#110490=CARTESIAN_POINT('Ctrl Pts',(-103.574148099986,1075.6287101144,406.612145678));
#110491=CARTESIAN_POINT('Ctrl Pts',(-103.430023932663,1075.64360756256,
406.61182061805));
#110492=CARTESIAN_POINT('Ctrl Pts',(-103.358144535959,1075.65112975667,
406.618742976178));
#110493=CARTESIAN_POINT('Ctrl Pts',(-103.144009500649,1075.6738153511,406.660872723149));
#110494=CARTESIAN_POINT('Ctrl Pts',(-103.007547154574,1075.68865114894,
406.717459821904));
#110495=CARTESIAN_POINT('Ctrl Pts',(-102.765411353305,1075.71582812797,
406.880396711323));
#110496=CARTESIAN_POINT('Ctrl Pts',(-102.661909954341,1075.72792217764,
406.984877355043));
#110497=CARTESIAN_POINT('Ctrl Pts',(-102.501633689167,1075.74789608371,
407.228361262746));
#110498=CARTESIAN_POINT('Ctrl Pts',(-102.446449642118,1075.75558042025,
407.364917638641));
#110499=CARTESIAN_POINT('Ctrl Pts',(-102.392620475075,1075.76555576074,
407.652125573174));
#110500=CARTESIAN_POINT('Ctrl Pts',(-102.394636540744,1075.76773602572,
407.799843881201));
#110501=CARTESIAN_POINT('Ctrl Pts',(-102.455810470833,1075.76626291771,
408.082988733887));
#110502=CARTESIAN_POINT('Ctrl Pts',(-102.513202388073,1075.76274081205,
408.215781884077));
#110503=CARTESIAN_POINT('Ctrl Pts',(-102.677110990787,1075.75034653712,
408.453944106876));
#110504=CARTESIAN_POINT('Ctrl Pts',(-102.782837580232,1075.74150132232,
408.556332158873));
#110505=CARTESIAN_POINT('Ctrl Pts',(-103.027985011516,1075.71953762433,
408.713951888631));
#110506=CARTESIAN_POINT('Ctrl Pts',(-103.165014956945,1075.70662837047,
408.767544630906));
#110507=CARTESIAN_POINT('Ctrl Pts',(-103.371398898217,1075.68629194353,
408.804015321739));
#110508=CARTESIAN_POINT('Ctrl Pts',(-103.435264134528,1075.67988453476,
408.809622250391));
#110509=CARTESIAN_POINT('Ctrl Pts',(-103.499237229524,1075.67335103125,
408.80964251971));
#110510=CARTESIAN_POINT('Origin',(-103.499585384594,1067.7251047501,407.710811438872));
#110511=CARTESIAN_POINT('',(-103.499585384594,1075.66376111901,408.209642574865));
#110512=CARTESIAN_POINT('',(-103.499585384594,1075.64701319545,407.21198030288));
#110513=CARTESIAN_POINT('Ctrl Pts',(-103.499585384594,1075.66376111901,
408.209642574865));
#110514=CARTESIAN_POINT('Ctrl Pts',(-103.502071362693,1075.66350639334,
408.209642574865));
#110515=CARTESIAN_POINT('Ctrl Pts',(-103.504557676489,1075.66325128953,
408.209623991148));
#110516=CARTESIAN_POINT('Ctrl Pts',(-103.539600239299,1075.65965095847,
408.209099961378));
#110517=CARTESIAN_POINT('Ctrl Pts',(-103.572028400505,1075.6562601718,408.205426810701));
#110518=CARTESIAN_POINT('Ctrl Pts',(-103.669219505184,1075.64591619944,
408.184650261159));
#110519=CARTESIAN_POINT('Ctrl Pts',(-103.731134995342,1075.63907092801,
408.157680344789));
#110520=CARTESIAN_POINT('Ctrl Pts',(-103.840052189201,1075.6265048167,408.081333398875));
#110521=CARTESIAN_POINT('Ctrl Pts',(-103.886164608578,1075.62089391449,
408.032956602154));
#110522=CARTESIAN_POINT('Ctrl Pts',(-103.956328176386,1075.61170073141,
407.921713108968));
#110523=CARTESIAN_POINT('Ctrl Pts',(-103.980008644332,1075.60818007301,
407.86015016588));
#110524=CARTESIAN_POINT('Ctrl Pts',(-104.002208409432,1075.60366971968,
407.731620100496));
#110525=CARTESIAN_POINT('Ctrl Pts',(-104.000640174725,1075.60271181179,
407.665959140142));
#110526=CARTESIAN_POINT('Ctrl Pts',(-103.972385499019,1075.6034971417,407.539015070644));
#110527=CARTESIAN_POINT('Ctrl Pts',(-103.946022142635,1075.6052280724,407.478992720413));
#110528=CARTESIAN_POINT('Ctrl Pts',(-103.871712953719,1075.61116235175,
407.37229473525));
#110529=CARTESIAN_POINT('Ctrl Pts',(-103.824434517262,1075.61531430681,
407.326716025527));
#110530=CARTESIAN_POINT('Ctrl Pts',(-103.714848323074,1075.62550452348,
407.25609274143));
#110531=CARTESIAN_POINT('Ctrl Pts',(-103.653511860268,1075.63145482351,
407.2318550433));
#110532=CARTESIAN_POINT('Ctrl Pts',(-103.559699774815,1075.64086023512,
407.214701920339));
#110533=CARTESIAN_POINT('Ctrl Pts',(-103.529670011463,1075.64391337157,
407.21198030288));
#110534=CARTESIAN_POINT('Ctrl Pts',(-103.499585384594,1075.64701319545,
407.21198030288));
#110535=CARTESIAN_POINT('',(-103.499585384594,1082.7251047501,407.21198030288));
#110536=CARTESIAN_POINT('',(-103.499585384594,1067.7251047501,407.21198030288));
#110537=CARTESIAN_POINT('Origin',(-103.499585384594,1082.7251047501,407.710811438872));
#110538=CARTESIAN_POINT('Ctrl Pts',(-103.499585384594,1075.64701319545,
407.21198030288));
#110539=CARTESIAN_POINT('Ctrl Pts',(-103.499513271807,1075.64702062572,
407.21198030288));
#110540=CARTESIAN_POINT('Ctrl Pts',(-103.499441158706,1075.64702805626,
407.211980318517));
#110541=CARTESIAN_POINT('Ctrl Pts',(-103.499369045294,1075.64703548707,
407.211980349792));
#110542=CARTESIAN_POINT('Ctrl Pts',(-103.466724572183,1075.65039928297,
407.211994507455));
#110543=CARTESIAN_POINT('Ctrl Pts',(-103.434161726441,1075.65380296785,
407.21521310209));
#110544=CARTESIAN_POINT('Ctrl Pts',(-103.33689583746,1075.664116205,407.23458513421));
#110545=CARTESIAN_POINT('Ctrl Pts',(-103.274865982197,1075.67089625435,
407.260512561931));
#110546=CARTESIAN_POINT('Ctrl Pts',(-103.164782694419,1075.68336832813,
407.335116923966));
#110547=CARTESIAN_POINT('Ctrl Pts',(-103.117760449514,1075.68894240784,
407.382991737611));
#110548=CARTESIAN_POINT('Ctrl Pts',(-103.045243081654,1075.69814449495,
407.494430475869));
#110549=CARTESIAN_POINT('Ctrl Pts',(-103.020460482078,1075.70168204059,
407.556856021544));
#110550=CARTESIAN_POINT('Ctrl Pts',(-102.997130157182,1075.70617793649,
407.686349243561));
#110551=CARTESIAN_POINT('Ctrl Pts',(-102.998218997141,1075.70715000442,
407.751994498134));
#110552=CARTESIAN_POINT('Ctrl Pts',(-103.025545812247,1075.70648900357,
407.879183199904));
#110553=CARTESIAN_POINT('Ctrl Pts',(-103.051505854999,1075.70486302484,
407.939459087447));
#110554=CARTESIAN_POINT('Ctrl Pts',(-103.125173240855,1075.69918689037,
408.046820779613));
#110555=CARTESIAN_POINT('Ctrl Pts',(-103.172230360576,1075.69518359488,
408.092792831827));
#110556=CARTESIAN_POINT('Ctrl Pts',(-103.282414929773,1075.68518922301,
408.164786984131));
#110557=CARTESIAN_POINT('Ctrl Pts',(-103.344761955394,1075.6792567197,408.189633794588));
#110558=CARTESIAN_POINT('Ctrl Pts',(-103.43962405692,1075.66985494325,408.206935319653));
#110559=CARTESIAN_POINT('Ctrl Pts',(-103.469580270733,1075.66683559205,
408.209642574865));
#110560=CARTESIAN_POINT('Ctrl Pts',(-103.499585384594,1075.66376111901,
408.209642574865));
#110561=CARTESIAN_POINT('Origin',(-107.832717977552,1067.7251047501,394.412017622821));
#110562=CARTESIAN_POINT('',(-107.832717977578,1074.76154318277,393.321476874093));
#110563=CARTESIAN_POINT('',(-107.832717977552,1067.7251047501,393.321476874093));
#110564=CARTESIAN_POINT('Ctrl Pts',(-107.832910139828,1074.84118131354,
395.502558354619));
#110565=CARTESIAN_POINT('Ctrl Pts',(-107.903854913976,1074.8319916062,395.502545853564));
#110566=CARTESIAN_POINT('Ctrl Pts',(-107.974605324901,1074.82255439571,
395.49561052102));
#110567=CARTESIAN_POINT('Ctrl Pts',(-108.113974483817,1074.80341334749,
395.468066248453));
#110568=CARTESIAN_POINT('Ctrl Pts',(-108.18227296561,1074.79375135477,395.447466853533));
#110569=CARTESIAN_POINT('Ctrl Pts',(-108.383552042772,1074.76439718822,
395.364555872695));
#110570=CARTESIAN_POINT('Ctrl Pts',(-108.506532479351,1074.7451943403,395.281961889542));
#110571=CARTESIAN_POINT('Ctrl Pts',(-108.710269160931,1074.71067322688,
395.075172153568));
#110572=CARTESIAN_POINT('Ctrl Pts',(-108.789989509366,1074.69560519737,
394.953902490361));
#110573=CARTESIAN_POINT('Ctrl Pts',(-108.897265991725,1074.67147159055,
394.688279698583));
#110574=CARTESIAN_POINT('Ctrl Pts',(-108.924291576163,1074.66258573781,
394.546786497073));
#110575=CARTESIAN_POINT('Ctrl Pts',(-108.922174602421,1074.65223823734,
394.262243588738));
#110576=CARTESIAN_POINT('Ctrl Pts',(-108.893527587802,1074.65082028394,
394.122102134176));
#110577=CARTESIAN_POINT('Ctrl Pts',(-108.784263529771,1074.65563152539,
393.86077721138));
#110578=CARTESIAN_POINT('Ctrl Pts',(-108.704843923112,1074.66179882768,
393.742226857959));
#110579=CARTESIAN_POINT('Ctrl Pts',(-108.504816332335,1074.68093510674,
393.541519893516));
#110580=CARTESIAN_POINT('Ctrl Pts',(-108.38594290611,1074.69375465292,393.461601719654));
#110581=CARTESIAN_POINT('Ctrl Pts',(-108.123388677827,1074.72440253584,
393.351225217733));
#110582=CARTESIAN_POINT('Ctrl Pts',(-107.981978401088,1074.74198570064,
393.322346248265));
#110583=CARTESIAN_POINT('Ctrl Pts',(-107.767590175171,1074.7700758924,393.321069769749));
#110584=CARTESIAN_POINT('Ctrl Pts',(-107.696120910827,1074.77967830712,
393.327700062632));
#110585=CARTESIAN_POINT('Ctrl Pts',(-107.555795427375,1074.79900268354,
393.354812807297));
#110586=CARTESIAN_POINT('Ctrl Pts',(-107.48724521197,1074.80868084317,393.375186810816));
#110587=CARTESIAN_POINT('Ctrl Pts',(-107.287030355667,1074.83768519115,
393.456775942496));
#110588=CARTESIAN_POINT('Ctrl Pts',(-107.164973574096,1074.85640529594,
393.537680045991));
#110589=CARTESIAN_POINT('Ctrl Pts',(-106.960070173757,1074.89018328405,
393.742234430188));
#110590=CARTESIAN_POINT('Ctrl Pts',(-106.878990434508,1074.90493716678,
393.863688363703));
#110591=CARTESIAN_POINT('Ctrl Pts',(-106.768955434767,1074.92860023213,
394.13158258457));
#110592=CARTESIAN_POINT('Ctrl Pts',(-106.741091560602,1074.93727445006,
394.275284544965));
#110593=CARTESIAN_POINT('Ctrl Pts',(-106.743300631791,1074.94721750422,
394.562049905487));
#110594=CARTESIAN_POINT('Ctrl Pts',(-106.771973979401,1074.9485604562,394.702155806973));
#110595=CARTESIAN_POINT('Ctrl Pts',(-106.881415658133,1074.94396263451,
394.963773820071));
#110596=CARTESIAN_POINT('Ctrl Pts',(-106.961137569745,1074.93805868516,
395.082601658698));
#110597=CARTESIAN_POINT('Ctrl Pts',(-107.163657499755,1074.91946644001,
395.285309568277));
#110598=CARTESIAN_POINT('Ctrl Pts',(-107.28531438269,1074.90681428368,395.366215762831));
#110599=CARTESIAN_POINT('Ctrl Pts',(-107.550499991754,1074.8766722165,395.474958483077));
#110600=CARTESIAN_POINT('Ctrl Pts',(-107.691128263104,1074.85954678119,
395.502583337756));
#110601=CARTESIAN_POINT('Ctrl Pts',(-107.832910139828,1074.84118131354,
395.502558354619));
#110602=CARTESIAN_POINT('Origin',(-107.832717977552,1067.7251047501,394.412017622821));
#110603=CARTESIAN_POINT('',(-107.832717977552,1074.8199670159,394.902558371549));
#110604=CARTESIAN_POINT('',(-107.832717977552,1074.78413642061,393.921476874093));
#110605=CARTESIAN_POINT('Ctrl Pts',(-107.832717977552,1074.8199670159,394.902558371549));
#110606=CARTESIAN_POINT('Ctrl Pts',(-107.83392382367,1074.81981027287,394.902558371549));
#110607=CARTESIAN_POINT('Ctrl Pts',(-107.835129853334,1074.81965333798,
394.902553925238));
#110608=CARTESIAN_POINT('Ctrl Pts',(-107.86832801063,1074.81532879109,394.90230906005));
#110609=CARTESIAN_POINT('Ctrl Pts',(-107.900210461572,1074.81105729803,
394.898944004619));
#110610=CARTESIAN_POINT('Ctrl Pts',(-107.962902415974,1074.80241994308,
394.886051563901));
#110611=CARTESIAN_POINT('Ctrl Pts',(-107.993569896714,1074.79807321681,
394.876542057167));
#110612=CARTESIAN_POINT('Ctrl Pts',(-108.0836376156,1074.7849281648,394.838615112471));
#110613=CARTESIAN_POINT('Ctrl Pts',(-108.138510467907,1074.77637628905,
394.801188906155));
#110614=CARTESIAN_POINT('Ctrl Pts',(-108.229681180665,1074.76098307302,
394.707430962913));
#110615=CARTESIAN_POINT('Ctrl Pts',(-108.265341803572,1074.75426851599,
394.652254555808));
#110616=CARTESIAN_POINT('Ctrl Pts',(-108.312644906129,1074.74361978502,
394.532021316516));
#110617=CARTESIAN_POINT('Ctrl Pts',(-108.324227019244,1074.7397446815,394.468334043055));
#110618=CARTESIAN_POINT('Ctrl Pts',(-108.322171678761,1074.73529550747,
394.340428915001));
#110619=CARTESIAN_POINT('Ctrl Pts',(-108.308745384814,1074.73474192927,
394.277513882568));
#110620=CARTESIAN_POINT('Ctrl Pts',(-108.258576734306,1074.73702777487,
394.160357857072));
#110621=CARTESIAN_POINT('Ctrl Pts',(-108.222360722634,1074.73984155129,
394.107304158825));
#110622=CARTESIAN_POINT('Ctrl Pts',(-108.131503147455,1074.74849574992,
394.017740314956));
#110623=CARTESIAN_POINT('Ctrl Pts',(-108.07764587156,1074.75426967849,393.982238014158));
#110624=CARTESIAN_POINT('Ctrl Pts',(-107.95954634089,1074.76799050231,393.933877526661));
#110625=CARTESIAN_POINT('Ctrl Pts',(-107.896413195801,1074.77580841974,
393.921482136063));
#110626=CARTESIAN_POINT('Ctrl Pts',(-107.832758514871,1074.78413112039,
393.921476875766));
#110627=CARTESIAN_POINT('Ctrl Pts',(-107.832745002416,1074.78413288711,
393.921476874649));
#110628=CARTESIAN_POINT('Ctrl Pts',(-107.832731489977,1074.78413465385,
393.921476874093));
#110629=CARTESIAN_POINT('Ctrl Pts',(-107.832717977552,1074.78413642061,
393.921476874093));
#110630=CARTESIAN_POINT('',(-107.832717977552,1082.7251047501,393.921476874092));
#110631=CARTESIAN_POINT('',(-107.832717977552,1067.7251047501,393.921476874092));
#110632=CARTESIAN_POINT('Origin',(-107.832717977552,1082.7251047501,394.412017622821));
#110633=CARTESIAN_POINT('Ctrl Pts',(-107.832717977552,1074.78413642061,
393.921476874093));
#110634=CARTESIAN_POINT('Ctrl Pts',(-107.800604272338,1074.78833530606,
393.921476874093));
#110635=CARTESIAN_POINT('Ctrl Pts',(-107.768577169475,1074.79263405602,
393.924630379442));
#110636=CARTESIAN_POINT('Ctrl Pts',(-107.705650853594,1074.80130169454,
393.937136487566));
#110637=CARTESIAN_POINT('Ctrl Pts',(-107.674891200817,1074.80565111403,
393.946454427611));
#110638=CARTESIAN_POINT('Ctrl Pts',(-107.584867137173,1074.81873019232,
393.983682233695));
#110639=CARTESIAN_POINT('Ctrl Pts',(-107.530007475898,1074.82719627437,
394.020501214459));
#110640=CARTESIAN_POINT('Ctrl Pts',(-107.438068603545,1074.84249388482,
394.113454207606));
#110641=CARTESIAN_POINT('Ctrl Pts',(-107.401819425782,1074.84918310533,
394.168618631387));
#110642=CARTESIAN_POINT('Ctrl Pts',(-107.353409780512,1074.85980829449,
394.289294474671));
#110643=CARTESIAN_POINT('Ctrl Pts',(-107.341405020451,1074.86367556168,
394.353444839142));
#110644=CARTESIAN_POINT('Ctrl Pts',(-107.343013754148,1074.86810855196,
394.481869409797));
#110645=CARTESIAN_POINT('Ctrl Pts',(-107.356216144261,1074.86868008251,
394.544829605904));
#110646=CARTESIAN_POINT('Ctrl Pts',(-107.405996004093,1074.86650196661,
394.662230000609));
#110647=CARTESIAN_POINT('Ctrl Pts',(-107.442079945846,1074.86377251483,
394.715471003849));
#110648=CARTESIAN_POINT('Ctrl Pts',(-107.532789046877,1074.85531420137,
394.805441835666));
#110649=CARTESIAN_POINT('Ctrl Pts',(-107.586634462912,1074.84964866483,
394.841152004075));
#110650=CARTESIAN_POINT('Ctrl Pts',(-107.705111949593,1074.83607933483,
394.890009008638));
#110651=CARTESIAN_POINT('Ctrl Pts',(-107.768655973974,1074.82829417471,
394.902558371549));
#110652=CARTESIAN_POINT('Ctrl Pts',(-107.832717977552,1074.8199670159,394.902558371549));
#110653=CARTESIAN_POINT('Origin',(-86.3230601853152,1067.7251047501,448.47408103355));
#110654=CARTESIAN_POINT('',(-86.3230601853431,1076.68243856932,446.995777901357));
#110655=CARTESIAN_POINT('',(-86.3230601853152,1067.7251047501,446.995777901357));
#110656=CARTESIAN_POINT('Ctrl Pts',(-86.323166507663,1076.66188309602,449.95238416192));
#110657=CARTESIAN_POINT('Ctrl Pts',(-86.5172614368491,1076.65660731882,
449.952370202247));
#110658=CARTESIAN_POINT('Ctrl Pts',(-86.7094736205971,1076.65138668446,
449.914130614729));
#110659=CARTESIAN_POINT('Ctrl Pts',(-87.0682048713522,1076.64193094744,
449.765532290042));
#110660=CARTESIAN_POINT('Ctrl Pts',(-87.2312315510664,1076.63779524223,
449.656588436172));
#110661=CARTESIAN_POINT('Ctrl Pts',(-87.5056709311274,1076.63151683903,
449.382064201945));
#110662=CARTESIAN_POINT('Ctrl Pts',(-87.6144815374425,1076.62943854855,
449.219226268801));
#110663=CARTESIAN_POINT('Ctrl Pts',(-87.762812829159,1076.6278327369,448.86128268278));
#110664=CARTESIAN_POINT('Ctrl Pts',(-87.8010755829468,1076.62831568124,
448.669736455142));
#110665=CARTESIAN_POINT('Ctrl Pts',(-87.8016472192217,1076.63174641416,
448.28320356723));
#110666=CARTESIAN_POINT('Ctrl Pts',(-87.7641097372451,1076.63465248883,
448.091956916499));
#110667=CARTESIAN_POINT('Ctrl Pts',(-87.6176832980475,1076.64226268814,
447.734770499957));
#110668=CARTESIAN_POINT('Ctrl Pts',(-87.5102148846989,1076.64688667322,
447.572259245402));
#110669=CARTESIAN_POINT('Ctrl Pts',(-87.2387777836349,1076.65692796677,
447.297574466114));
#110670=CARTESIAN_POINT('Ctrl Pts',(-87.0773491930349,1076.66224324643,
447.188097761844));
#110671=CARTESIAN_POINT('Ctrl Pts',(-86.8104892082658,1076.67004015432,
447.075108429827));
#110672=CARTESIAN_POINT('Ctrl Pts',(-86.7180562722278,1076.67259256297,
447.046253957327));
#110673=CARTESIAN_POINT('Ctrl Pts',(-86.431201397442,1076.6800734711,446.986719209002));
#110674=CARTESIAN_POINT('Ctrl Pts',(-86.2328838610349,1076.68465096512,
446.985518930173));
#110675=CARTESIAN_POINT('Ctrl Pts',(-85.8487964974497,1076.69253439563,
447.060414648582));
#110676=CARTESIAN_POINT('Ctrl Pts',(-85.6667126046689,1076.69577849607,
447.135202738786));
#110677=CARTESIAN_POINT('Ctrl Pts',(-85.341832830451,1076.70087449289,447.351279210184));
#110678=CARTESIAN_POINT('Ctrl Pts',(-85.2022904039396,1076.7026828969,447.490530755828));
#110679=CARTESIAN_POINT('Ctrl Pts',(-84.9849845958677,1076.7049304295,447.815802891922));
#110680=CARTESIAN_POINT('Ctrl Pts',(-84.9096054342876,1076.70534782308,
447.998767235241));
#110681=CARTESIAN_POINT('Ctrl Pts',(-84.8346263006418,1076.7048087597,448.383212003071));
#110682=CARTESIAN_POINT('Ctrl Pts',(-84.835684426703,1076.70385768645,448.580867548382));
#110683=CARTESIAN_POINT('Ctrl Pts',(-84.9145712714694,1076.70051169125,
448.963523477952));
#110684=CARTESIAN_POINT('Ctrl Pts',(-84.9913286135803,1076.69814784631,
449.144811578407));
#110685=CARTESIAN_POINT('Ctrl Pts',(-85.2109345071113,1076.69194406988,
449.467406514347));
#110686=CARTESIAN_POINT('Ctrl Pts',(-85.3517320431411,1076.68815444462,
449.605465730436));
#110687=CARTESIAN_POINT('Ctrl Pts',(-85.5955775481193,1076.68158862809,
449.764563096708));
#110688=CARTESIAN_POINT('Ctrl Pts',(-85.680790816734,1076.67929497928,449.809020704177));
#110689=CARTESIAN_POINT('Ctrl Pts',(-85.8569752279724,1076.6745385003,449.88014016367));
#110690=CARTESIAN_POINT('Ctrl Pts',(-85.9474096947825,1076.67209040593,
449.906953479439));
#110691=CARTESIAN_POINT('Ctrl Pts',(-86.133137971659,1076.66705026916,449.943216367105));
#110692=CARTESIAN_POINT('Ctrl Pts',(-86.2280420848667,1076.66446871359,
449.952391003448));
#110693=CARTESIAN_POINT('Ctrl Pts',(-86.323166507663,1076.66188309602,449.95238416192));
#110694=CARTESIAN_POINT('Origin',(-86.3230601853152,1067.7251047501,448.47408103355));
#110695=CARTESIAN_POINT('',(-86.3230601853152,1076.66654097421,449.352384165744));
#110696=CARTESIAN_POINT('',(-86.3230601853154,1076.67873408293,447.595777901357));
#110697=CARTESIAN_POINT('Ctrl Pts',(-86.3230601853151,1076.66654097421,
449.352384165744));
#110698=CARTESIAN_POINT('Ctrl Pts',(-86.3901181015092,1076.66477558714,
449.352384165744));
#110699=CARTESIAN_POINT('Ctrl Pts',(-86.4571142523758,1076.66303405489,
449.344704219338));
#110700=CARTESIAN_POINT('Ctrl Pts',(-86.6349456175339,1076.65849642279,
449.303191689395));
#110701=CARTESIAN_POINT('Ctrl Pts',(-86.7409318553903,1076.65588594487,
449.255159581536));
#110702=CARTESIAN_POINT('Ctrl Pts',(-86.9282672280694,1076.65158872148,
449.120929485844));
#110703=CARTESIAN_POINT('Ctrl Pts',(-87.0078094645969,1076.64994579721,
449.036051140019));
#110704=CARTESIAN_POINT('Ctrl Pts',(-87.1294979961342,1076.6479566119,448.840564835501));
#110705=CARTESIAN_POINT('Ctrl Pts',(-87.1705189077138,1076.64762908125,
448.731892701794));
#110706=CARTESIAN_POINT('Ctrl Pts',(-87.2082992243034,1076.64836457455,
448.505101618138));
#110707=CARTESIAN_POINT('Ctrl Pts',(-87.2047642788882,1076.64941770649,
448.389193820259));
#110708=CARTESIAN_POINT('Ctrl Pts',(-87.1533029894093,1076.65270906129,
448.165390564633));
#110709=CARTESIAN_POINT('Ctrl Pts',(-87.1058985607682,1076.65491274874,
448.059649853931));
#110710=CARTESIAN_POINT('Ctrl Pts',(-86.9730765281975,1076.66007334864,
447.872346414937));
#110711=CARTESIAN_POINT('Ctrl Pts',(-86.8889138097755,1076.66297848812,
447.792602368897));
#110712=CARTESIAN_POINT('Ctrl Pts',(-86.7432564855229,1076.66749935026,
447.700681787845));
#110713=CARTESIAN_POINT('Ctrl Pts',(-86.6918267176327,1076.66902275366,
447.674879842137));
#110714=CARTESIAN_POINT('Ctrl Pts',(-86.5882581317525,1076.67195158694,
447.635060818344));
#110715=CARTESIAN_POINT('Ctrl Pts',(-86.5366134513795,1076.67335198428,
447.620453481324));
#110716=CARTESIAN_POINT('Ctrl Pts',(-86.4308998346368,1076.67610124917,
447.600753944207));
#110717=CARTESIAN_POINT('Ctrl Pts',(-86.3770394159166,1076.67744380712,
447.595778081493));
#110718=CARTESIAN_POINT('Ctrl Pts',(-86.3230631164002,1076.67873401287,
447.595777901362));
#110719=CARTESIAN_POINT('',(-86.3230601853152,1082.7251047501,447.595777901357));
#110720=CARTESIAN_POINT('',(-86.3230601853152,1067.7251047501,447.595777901357));
#110721=CARTESIAN_POINT('Origin',(-86.3230601853152,1082.7251047501,448.47408103355));
#110722=CARTESIAN_POINT('Ctrl Pts',(-86.3230601853156,1076.67873408293,
447.595777901357));
#110723=CARTESIAN_POINT('Ctrl Pts',(-86.2063772042534,1076.68152317411,
447.595777901357));
#110724=CARTESIAN_POINT('Ctrl Pts',(-86.0908516781534,1076.68402501507,
447.619029177307));
#110725=CARTESIAN_POINT('Ctrl Pts',(-85.8758342807902,1076.68825831458,
447.709245703915));
#110726=CARTESIAN_POINT('Ctrl Pts',(-85.7784499291699,1076.68995199795,
447.775234437677));
#110727=CARTESIAN_POINT('Ctrl Pts',(-85.61494962158,1076.69242874122,447.94152348628));
#110728=CARTESIAN_POINT('Ctrl Pts',(-85.5505234694667,1076.69318803405,
448.040230224465));
#110729=CARTESIAN_POINT('Ctrl Pts',(-85.4639913045317,1076.69373323332,
448.257140974017));
#110730=CARTESIAN_POINT('Ctrl Pts',(-85.4427853611372,1076.69351357969,
448.373194189322));
#110731=CARTESIAN_POINT('Ctrl Pts',(-85.4470130157523,1076.69209332713,
448.606569592611));
#110732=CARTESIAN_POINT('Ctrl Pts',(-85.4723188227951,1076.69090693583,
448.72156616507));
#110733=CARTESIAN_POINT('Ctrl Pts',(-85.5663144925847,1076.68761288142,
448.934869113926));
#110734=CARTESIAN_POINT('Ctrl Pts',(-85.6340383967117,1076.68553563327,
449.031068942445));
#110735=CARTESIAN_POINT('Ctrl Pts',(-85.8034210616211,1076.68062678245,
449.191771366874));
#110736=CARTESIAN_POINT('Ctrl Pts',(-85.9035306249559,1076.67783864142,
449.254527326388));
#110737=CARTESIAN_POINT('Ctrl Pts',(-86.0672423860777,1076.67337214142,
449.316302607773));
#110738=CARTESIAN_POINT('Ctrl Pts',(-86.12339803899,1076.6718547263,449.331352751992));
#110739=CARTESIAN_POINT('Ctrl Pts',(-86.2278178847014,1076.66905962772,
449.348513775272));
#110740=CARTESIAN_POINT('Ctrl Pts',(-86.275454598382,1076.66779425334,449.352384165744));
#110741=CARTESIAN_POINT('Ctrl Pts',(-86.3230601853151,1076.66654097421,
449.352384165744));
#110742=CARTESIAN_POINT('Origin',(-95.5155706932854,1067.7251047501,439.917923765972));
#110743=CARTESIAN_POINT('',(-95.5155706933052,1076.35760005837,438.642479644836));
#110744=CARTESIAN_POINT('',(-95.5155706932854,1067.7251047501,438.642479644836));
#110745=CARTESIAN_POINT('Ctrl Pts',(-95.5152422626988,1076.33152383034,
441.193367844822));
#110746=CARTESIAN_POINT('Ctrl Pts',(-95.6828139562135,1076.32067145058,
441.193410995024));
#110747=CARTESIAN_POINT('Ctrl Pts',(-95.8487982401502,1076.31007821196,
441.160429595892));
#110748=CARTESIAN_POINT('Ctrl Pts',(-96.1583840432205,1076.29077894953,
441.032190098894));
#110749=CARTESIAN_POINT('Ctrl Pts',(-96.2990284046096,1076.28226094656,
440.938236132061));
#110750=CARTESIAN_POINT('Ctrl Pts',(-96.5356946515849,1076.26868427456,
440.701530519116));
#110751=CARTESIAN_POINT('Ctrl Pts',(-96.6295306238772,1076.26375277916,
440.561214321463));
#110752=CARTESIAN_POINT('Ctrl Pts',(-96.7575246336427,1076.25831659374,
440.252744110367));
#110753=CARTESIAN_POINT('Ctrl Pts',(-96.7906131552752,1076.25785331984,
440.08770265456));
#110754=CARTESIAN_POINT('Ctrl Pts',(-96.7914086114346,1076.26149407278,
439.754483068864));
#110755=CARTESIAN_POINT('Ctrl Pts',(-96.7592059937086,1076.26555428597,
439.589571774213));
#110756=CARTESIAN_POINT('Ctrl Pts',(-96.6332654975541,1076.27757075149,
439.281314097811));
#110757=CARTESIAN_POINT('Ctrl Pts',(-96.5406732396144,1076.28541145008,
439.140985420101));
#110758=CARTESIAN_POINT('Ctrl Pts',(-96.3065934397241,1076.30367981313,
438.903572082332));
#110759=CARTESIAN_POINT('Ctrl Pts',(-96.1672147526564,1076.31393506852,
438.808889499782));
#110760=CARTESIAN_POINT('Ctrl Pts',(-95.9367383909986,1076.32998643442,
438.71113138861));
#110761=CARTESIAN_POINT('Ctrl Pts',(-95.8568522290869,1076.33541341161,
438.686154180861));
#110762=CARTESIAN_POINT('Ctrl Pts',(-95.693549633131,1076.34623590983,438.652214737871));
#110763=CARTESIAN_POINT('Ctrl Pts',(-95.6105276802408,1076.35160590179,
438.643294187491));
#110764=CARTESIAN_POINT('Ctrl Pts',(-95.3582991611468,1076.3675300373,438.640989092166));
#110765=CARTESIAN_POINT('Ctrl Pts',(-95.1906877056548,1076.37757908158,
438.673021968305));
#110766=CARTESIAN_POINT('Ctrl Pts',(-94.8780934410209,1076.39538146742,
438.800434011967));
#110767=CARTESIAN_POINT('Ctrl Pts',(-94.7361152043874,1076.40297107354,
438.894375362848));
#110768=CARTESIAN_POINT('Ctrl Pts',(-94.4964315895821,1076.41491058555,
439.132580605632));
#110769=CARTESIAN_POINT('Ctrl Pts',(-94.401286817847,1076.41913438666,439.274643977476));
#110770=CARTESIAN_POINT('Ctrl Pts',(-94.2718273939629,1076.42375173698,
439.588198443855));
#110771=CARTESIAN_POINT('Ctrl Pts',(-94.2390147023854,1076.42408915898,
439.756605778015));
#110772=CARTESIAN_POINT('Ctrl Pts',(-94.2412932871994,1076.42079372705,
440.095973795517));
#110773=CARTESIAN_POINT('Ctrl Pts',(-94.2762030297749,1076.41720145592,
440.263506279824));
#110774=CARTESIAN_POINT('Ctrl Pts',(-94.409120985165,1076.40641719041,440.574425162885));
#110775=CARTESIAN_POINT('Ctrl Pts',(-94.5055462696883,1076.39934239347,
440.714814519768));
#110776=CARTESIAN_POINT('Ctrl Pts',(-94.7474950406095,1076.38239560869,
440.950074021745));
#110777=CARTESIAN_POINT('Ctrl Pts',(-94.8907053021309,1076.37268187305,
441.042548865023));
#110778=CARTESIAN_POINT('Ctrl Pts',(-95.1966006470039,1076.35230137259,
441.163168135794));
#110779=CARTESIAN_POINT('Ctrl Pts',(-95.3552144545814,1076.34188764842,
441.193326637193));
#110780=CARTESIAN_POINT('Ctrl Pts',(-95.5152422626988,1076.33152383034,
441.193367844822));
#110781=CARTESIAN_POINT('Origin',(-95.5155706932854,1067.7251047501,439.917923765972));
#110782=CARTESIAN_POINT('',(-95.5155706932854,1076.33810018128,440.593367887109));
#110783=CARTESIAN_POINT('',(-95.5155706932854,1076.35191524971,439.242479644836));
#110784=CARTESIAN_POINT('Ctrl Pts',(-95.5155706932854,1076.33810018128,
440.593367887109));
#110785=CARTESIAN_POINT('Ctrl Pts',(-95.5230299670075,1076.33762039049,
440.593367887109));
#110786=CARTESIAN_POINT('Ctrl Pts',(-95.5304943432052,1076.33714118425,
440.593244323034));
#110787=CARTESIAN_POINT('Ctrl Pts',(-95.627504268366,1076.33092522636,440.590026799769));
#110788=CARTESIAN_POINT('Ctrl Pts',(-95.7155911655218,1076.32541224372,
440.569269688472));
#110789=CARTESIAN_POINT('Ctrl Pts',(-95.8775875839268,1076.31558272049,
440.494997225786));
#110790=CARTESIAN_POINT('Ctrl Pts',(-95.950092136511,1076.31134871855,440.442588892107));
#110791=CARTESIAN_POINT('Ctrl Pts',(-96.0706049845411,1076.30473754511,
440.312866459206));
#110792=CARTESIAN_POINT('Ctrl Pts',(-96.1175013592039,1076.30242126744,
440.236877363948));
#110793=CARTESIAN_POINT('Ctrl Pts',(-96.1792732406646,1076.30006955532,
440.071274783904));
#110794=CARTESIAN_POINT('Ctrl Pts',(-96.1936134077525,1076.30005266803,
439.983313047932));
#110795=CARTESIAN_POINT('Ctrl Pts',(-96.1876450931037,1076.30233602738,
439.80689653668));
#110796=CARTESIAN_POINT('Ctrl Pts',(-96.1674102694078,1076.30461244013,
439.720168206024));
#110797=CARTESIAN_POINT('Ctrl Pts',(-96.0947228253676,1076.31113950101,
439.559299527691));
#110798=CARTESIAN_POINT('Ctrl Pts',(-96.0429223630463,1076.31532888567,
439.486743418212));
#110799=CARTESIAN_POINT('Ctrl Pts',(-95.9142430055404,1076.3250295308,439.36555000779));
#110800=CARTESIAN_POINT('Ctrl Pts',(-95.8385381801963,1076.330449611,439.31814014607));
#110801=CARTESIAN_POINT('Ctrl Pts',(-95.7177361820896,1076.33871064195,
439.272153569839));
#110802=CARTESIAN_POINT('Ctrl Pts',(-95.6783620139873,1076.34135172418,
439.261121781354));
#110803=CARTESIAN_POINT('Ctrl Pts',(-95.5977925667714,1076.34665438765,
439.246242525049));
#110804=CARTESIAN_POINT('Ctrl Pts',(-95.5567507615488,1076.34930508029,
439.242482714328));
#110805=CARTESIAN_POINT('Ctrl Pts',(-95.5156210705524,1076.35191205661,
439.242479646715));
#110806=CARTESIAN_POINT('Ctrl Pts',(-95.5156042780997,1076.35191312098,
439.242479645462));
#110807=CARTESIAN_POINT('Ctrl Pts',(-95.5155874856773,1076.35191418535,
439.242479644836));
#110808=CARTESIAN_POINT('Ctrl Pts',(-95.5155706932854,1076.35191524971,
439.242479644836));
#110809=CARTESIAN_POINT('',(-95.5155706932854,1082.7251047501,439.242479644836));
#110810=CARTESIAN_POINT('',(-95.5155706932854,1067.7251047501,439.242479644836));
#110811=CARTESIAN_POINT('Origin',(-95.5155706932854,1082.7251047501,439.917923765972));
#110812=CARTESIAN_POINT('Ctrl Pts',(-95.5155706932854,1076.35191524971,
439.242479644836));
#110813=CARTESIAN_POINT('Ctrl Pts',(-95.4257877829596,1076.35760598816,
439.242479644836));
#110814=CARTESIAN_POINT('Ctrl Pts',(-95.3368745387622,1076.36300547989,
439.260381116648));
#110815=CARTESIAN_POINT('Ctrl Pts',(-95.1712970043486,1076.37262315823,
439.329913689638));
#110816=CARTESIAN_POINT('Ctrl Pts',(-95.0962644496087,1076.37674825756,
439.380825446226));
#110817=CARTESIAN_POINT('Ctrl Pts',(-94.9703261473707,1076.3832185644,439.509220382696));
#110818=CARTESIAN_POINT('Ctrl Pts',(-94.9207483488372,1076.38549570174,
439.585470636753));
#110819=CARTESIAN_POINT('Ctrl Pts',(-94.8546980200677,1076.38789194751,
439.752250744966));
#110820=CARTESIAN_POINT('Ctrl Pts',(-94.8386058514874,1076.388006019,439.840986744035));
#110821=CARTESIAN_POINT('Ctrl Pts',(-94.8418568845122,1076.38607531259,
440.018673303983));
#110822=CARTESIAN_POINT('Ctrl Pts',(-94.8608123091726,1076.38407067916,
440.105872600748));
#110823=CARTESIAN_POINT('Ctrl Pts',(-94.9317859374777,1076.37811315774,
440.269337621984));
#110824=CARTESIAN_POINT('Ctrl Pts',(-94.9836365508097,1076.37418693194,
440.343752813501));
#110825=CARTESIAN_POINT('Ctrl Pts',(-95.1133703141433,1076.36488745776,
440.467949083075));
#110826=CARTESIAN_POINT('Ctrl Pts',(-95.1899764453381,1076.35960461803,
440.516481846211));
#110827=CARTESIAN_POINT('Ctrl Pts',(-95.3510319527794,1076.34879392822,
440.578221706843));
#110828=CARTESIAN_POINT('Ctrl Pts',(-95.4329886699305,1076.34341197116,
440.593367887109));
#110829=CARTESIAN_POINT('Ctrl Pts',(-95.5155706932854,1076.33810018128,
440.593367887109));
#110830=CARTESIAN_POINT('Origin',(-104.753539540172,1067.7251047501,429.599096875777));
#110831=CARTESIAN_POINT('',(-104.753539540193,1075.66035026279,428.500265739785));
#110832=CARTESIAN_POINT('',(-104.753539540172,1067.7251047501,428.500265739785));
#110833=CARTESIAN_POINT('Ctrl Pts',(-104.753203728027,1075.6495208014,430.697927960456));
#110834=CARTESIAN_POINT('Ctrl Pts',(-104.900480042956,1075.63417453868,
430.697972969353));
#110835=CARTESIAN_POINT('Ctrl Pts',(-105.046335055649,1075.61900230498,
430.668408371385));
#110836=CARTESIAN_POINT('Ctrl Pts',(-105.315072036072,1075.59116670263,
430.554594465636));
#110837=CARTESIAN_POINT('Ctrl Pts',(-105.435805338195,1075.57872574262,
430.472531235281));
#110838=CARTESIAN_POINT('Ctrl Pts',(-105.638083926395,1075.55814657647,
430.26670957947));
#110839=CARTESIAN_POINT('Ctrl Pts',(-105.717889540202,1075.55018619578,
430.145201466243));
#110840=CARTESIAN_POINT('Ctrl Pts',(-105.825786489787,1075.53993329877,
429.878820981651));
#110841=CARTESIAN_POINT('Ctrl Pts',(-105.853102821232,1075.53771168743,
429.736734886952));
#110842=CARTESIAN_POINT('Ctrl Pts',(-105.851610307087,1075.53934106797,
429.450316660049));
#110843=CARTESIAN_POINT('Ctrl Pts',(-105.822938025717,1075.5431623155,429.308853765669));
#110844=CARTESIAN_POINT('Ctrl Pts',(-105.712951594158,1075.55633717576,
429.044563420142));
#110845=CARTESIAN_POINT('Ctrl Pts',(-105.632566779557,1075.56557513932,
428.924404614211));
#110846=CARTESIAN_POINT('Ctrl Pts',(-105.429866042245,1075.58821951279,
428.721180042264));
#110847=CARTESIAN_POINT('Ctrl Pts',(-105.309248312879,1075.60143030756,
428.640309884849));
#110848=CARTESIAN_POINT('Ctrl Pts',(-105.110033232513,1075.62283344418,
428.557201513108));
#110849=CARTESIAN_POINT('Ctrl Pts',(-105.04089791964,1075.63019795806,428.536056719325));
#110850=CARTESIAN_POINT('Ctrl Pts',(-104.899789171971,1075.64509975411,
428.507675700065));
#110851=CARTESIAN_POINT('Ctrl Pts',(-104.828152980214,1075.65260188103,
428.500451494514));
#110852=CARTESIAN_POINT('Ctrl Pts',(-104.610523619321,1075.67520212854,
428.499899378922));
#110853=CARTESIAN_POINT('Ctrl Pts',(-104.466016769097,1075.68994652228,
428.528552975495));
#110854=CARTESIAN_POINT('Ctrl Pts',(-104.197056730414,1075.7169178972,428.640509340355));
#110855=CARTESIAN_POINT('Ctrl Pts',(-104.075129543157,1075.72889582137,
428.722510568931));
#110856=CARTESIAN_POINT('Ctrl Pts',(-103.869985002791,1075.74862465936,
428.929725118191));
#110857=CARTESIAN_POINT('Ctrl Pts',(-103.788907408865,1075.75617197411,
429.052943954296));
#110858=CARTESIAN_POINT('Ctrl Pts',(-103.68080558744,1075.76572489395,429.321315274353));
#110859=CARTESIAN_POINT('Ctrl Pts',(-103.653765135895,1075.76774947395,
429.463310635218));
#110860=CARTESIAN_POINT('Ctrl Pts',(-103.655703044621,1075.76619401393,
429.749910518335));
#110861=CARTESIAN_POINT('Ctrl Pts',(-103.684727106134,1075.76262263895,
429.89166100879));
#110862=CARTESIAN_POINT('Ctrl Pts',(-103.796520628938,1075.75013016158,
430.158433119729));
#110863=CARTESIAN_POINT('Ctrl Pts',(-103.879155940594,1075.74123414344,
430.280358639091));
#110864=CARTESIAN_POINT('Ctrl Pts',(-104.086884357666,1075.71920019498,
430.484653206964));
#110865=CARTESIAN_POINT('Ctrl Pts',(-104.209888346711,1075.7062805828,430.565020155921));
#110866=CARTESIAN_POINT('Ctrl Pts',(-104.409299093131,1075.68540947004,
430.644922448304));
#110867=CARTESIAN_POINT('Ctrl Pts',(-104.476049332423,1075.67843389929,
430.664576481816));
#110868=CARTESIAN_POINT('Ctrl Pts',(-104.613063503368,1075.66413004391,
430.691167789154));
#110869=CARTESIAN_POINT('Ctrl Pts',(-104.683055196913,1075.65683031202,
430.697906522467));
#110870=CARTESIAN_POINT('Ctrl Pts',(-104.753203728027,1075.6495208014,430.697927960456));
#110871=CARTESIAN_POINT('Origin',(-104.753539540172,1067.7251047501,429.599096875777));
#110872=CARTESIAN_POINT('',(-104.753539540172,1075.6529321444,430.09792801177));
#110873=CARTESIAN_POINT('',(-104.753539540172,1075.65786345153,429.100265739785));
#110874=CARTESIAN_POINT('Ctrl Pts',(-104.753539540172,1075.6529321444,430.09792801177));
#110875=CARTESIAN_POINT('Ctrl Pts',(-104.75491854207,1075.65278861588,430.09792801177));
#110876=CARTESIAN_POINT('Ctrl Pts',(-104.756297668151,1075.65264509248,
430.097922293444));
#110877=CARTESIAN_POINT('Ctrl Pts',(-104.824346678404,1075.64556423468,
430.097357870435));
#110878=CARTESIAN_POINT('Ctrl Pts',(-104.890265025792,1075.63874646745,
430.083443905758));
#110879=CARTESIAN_POINT('Ctrl Pts',(-105.012201501236,1075.62623228538,
430.030718819393));
#110880=CARTESIAN_POINT('Ctrl Pts',(-105.067126415725,1075.62064759498,
429.992649514473));
#110881=CARTESIAN_POINT('Ctrl Pts',(-105.158275187127,1075.61152075326,
429.897890801476));
#110882=CARTESIAN_POINT('Ctrl Pts',(-105.193882096471,1075.60803841156,
429.842411760024));
#110883=CARTESIAN_POINT('Ctrl Pts',(-105.241579526787,1075.60360730913,
429.721070879668));
#110884=CARTESIAN_POINT('Ctrl Pts',(-105.253313431322,1075.60269027868,
429.656466455001));
#110885=CARTESIAN_POINT('Ctrl Pts',(-105.2513107664,1075.6035557548,429.526438301903));
#110886=CARTESIAN_POINT('Ctrl Pts',(-105.237623854927,1075.60532639985,
429.46231451433));
#110887=CARTESIAN_POINT('Ctrl Pts',(-105.186398834638,1075.61133551359,
429.342757781232));
#110888=CARTESIAN_POINT('Ctrl Pts',(-105.14928447161,1075.61552267919,429.288538457274));
#110889=CARTESIAN_POINT('Ctrl Pts',(-105.056167703792,1075.62577355843,
429.197191130533));
#110890=CARTESIAN_POINT('Ctrl Pts',(-105.000953634881,1075.63174869342,
429.161051507176));
#110891=CARTESIAN_POINT('Ctrl Pts',(-104.910877121333,1075.64135040035,
429.124658888835));
#110892=CARTESIAN_POINT('Ctrl Pts',(-104.88028424772,1075.6445902119,429.115587402101));
#110893=CARTESIAN_POINT('Ctrl Pts',(-104.817578083212,1075.65118828267,
429.103355711211));
#110894=CARTESIAN_POINT('Ctrl Pts',(-104.785595469618,1075.65453248655,
429.100265739785));
#110895=CARTESIAN_POINT('Ctrl Pts',(-104.753539540172,1075.65786345153,
429.100265739785));
#110896=CARTESIAN_POINT('',(-104.753539540172,1082.7251047501,429.100265739785));
#110897=CARTESIAN_POINT('',(-104.753539540172,1067.7251047501,429.100265739785));
#110898=CARTESIAN_POINT('Origin',(-104.753539540172,1082.7251047501,429.599096875777));
#110899=CARTESIAN_POINT('Ctrl Pts',(-104.753539540172,1075.65786345153,
429.100265739785));
#110900=CARTESIAN_POINT('Ctrl Pts',(-104.75346795341,1075.65787089019,429.100265739785));
#110901=CARTESIAN_POINT('Ctrl Pts',(-104.753396366282,1075.65787832878,
429.100265755192));
#110902=CARTESIAN_POINT('Ctrl Pts',(-104.753324778794,1075.6578857673,429.100265786012));
#110903=CARTESIAN_POINT('Ctrl Pts',(-104.686962910483,1075.66478130571,
429.100294356738));
#110904=CARTESIAN_POINT('Ctrl Pts',(-104.621235645922,1075.67152088023,
429.113565303564));
#110905=CARTESIAN_POINT('Ctrl Pts',(-104.498876025575,1075.68389797613,
429.16507081349));
#110906=CARTESIAN_POINT('Ctrl Pts',(-104.443425001876,1075.68941674587,
429.202766209488));
#110907=CARTESIAN_POINT('Ctrl Pts',(-104.350901439487,1075.69845229737,
429.297348716436));
#110908=CARTESIAN_POINT('Ctrl Pts',(-104.314585719611,1075.70189765785,
429.353121936495));
#110909=CARTESIAN_POINT('Ctrl Pts',(-104.266094122455,1075.70626601641,
429.474780855182));
#110910=CARTESIAN_POINT('Ctrl Pts',(-104.254053192325,1075.70718226731,
429.539303262049));
#110911=CARTESIAN_POINT('Ctrl Pts',(-104.255418784207,1075.70641096511,
429.669382186887));
#110912=CARTESIAN_POINT('Ctrl Pts',(-104.268818673046,1075.70473032009,
429.733641276545));
#110913=CARTESIAN_POINT('Ctrl Pts',(-104.319579146063,1075.69895077073,
429.853595944209));
#110914=CARTESIAN_POINT('Ctrl Pts',(-104.356533450706,1075.69489891119,
429.908065835912));
#110915=CARTESIAN_POINT('Ctrl Pts',(-104.450100574957,1075.68482951885,
430.000556228394));
#110916=CARTESIAN_POINT('Ctrl Pts',(-104.506150165916,1075.67887495066,
430.037306690302));
#110917=CARTESIAN_POINT('Ctrl Pts',(-104.597798222821,1075.66921721702,
430.074102295117));
#110918=CARTESIAN_POINT('Ctrl Pts',(-104.629012220032,1075.66593954012,
430.083222283081));
#110919=CARTESIAN_POINT('Ctrl Pts',(-104.691434319411,1075.65940527056,
430.095022538473));
#110920=CARTESIAN_POINT('Ctrl Pts',(-104.722455383358,1075.65616742862,
430.09792801177));
#110921=CARTESIAN_POINT('Ctrl Pts',(-104.753539540172,1075.6529321444,430.09792801177));
#110922=CARTESIAN_POINT('Origin',(-111.756957497768,1067.7251047501,417.491822535893));
#110923=CARTESIAN_POINT('',(-111.756957497784,1074.79209786668,416.401281787164));
#110924=CARTESIAN_POINT('',(-111.756957497768,1067.7251047501,416.401281787164));
#110925=CARTESIAN_POINT('Ctrl Pts',(-111.757173944974,1074.8108674823,418.582363263141));
#110926=CARTESIAN_POINT('Ctrl Pts',(-111.828369018416,1074.80126179765,
418.58234913256));
#110927=CARTESIAN_POINT('Ctrl Pts',(-111.8993932438,1074.79159616308,418.575363169141));
#110928=CARTESIAN_POINT('Ctrl Pts',(-112.112986052677,1074.76227600642,
418.532977014325));
#110929=CARTESIAN_POINT('Ctrl Pts',(-112.249671521804,1074.74315514854,
418.475731697485));
#110930=CARTESIAN_POINT('Ctrl Pts',(-112.489587534351,1074.70891584145,
418.312258102391));
#110931=CARTESIAN_POINT('Ctrl Pts',(-112.591248920725,1074.69404104959,
418.208730976483));
#110932=CARTESIAN_POINT('Ctrl Pts',(-112.747877742657,1074.67036863216,
417.968949724906));
#110933=CARTESIAN_POINT('Ctrl Pts',(-112.801771032909,1074.66174547335,
417.835403348587));
#110934=CARTESIAN_POINT('Ctrl Pts',(-112.854790240717,1074.65195312084,
417.555899494077));
#110935=CARTESIAN_POINT('Ctrl Pts',(-112.853829509201,1074.65082295652,
417.41288999358));
#110936=CARTESIAN_POINT('Ctrl Pts',(-112.797269999421,1074.65619647349,
417.135371467911));
#110937=CARTESIAN_POINT('Ctrl Pts',(-112.742319431075,1074.66263476029,
417.003678538191));
#110938=CARTESIAN_POINT('Ctrl Pts',(-112.584948650193,1074.68226237821,
416.767997893567));
#110939=CARTESIAN_POINT('Ctrl Pts',(-112.483783333288,1074.69529886287,
416.666546296024));
#110940=CARTESIAN_POINT('Ctrl Pts',(-112.247521232048,1074.72629641018,
416.507380196275));
#110941=CARTESIAN_POINT('Ctrl Pts',(-112.114342126929,1074.74400864694,
416.451653992195));
#110942=CARTESIAN_POINT('Ctrl Pts',(-111.904225205491,1074.77220838194,
416.408900838912));
#110943=CARTESIAN_POINT('Ctrl Pts',(-111.832834138731,1074.781830748,416.401572610849));
#110944=CARTESIAN_POINT('Ctrl Pts',(-111.68993678724,1074.80116657414,416.401008927996));
#110945=CARTESIAN_POINT('Ctrl Pts',(-111.618751538001,1074.81083631535,
416.407725139025));
#110946=CARTESIAN_POINT('Ctrl Pts',(-111.406558891734,1074.83977480743,
416.449001080662));
#110947=CARTESIAN_POINT('Ctrl Pts',(-111.271160348732,1074.85839618931,
416.504732318284));
#110948=CARTESIAN_POINT('Ctrl Pts',(-111.030528495974,1074.89188335811,
416.665731890742));
#110949=CARTESIAN_POINT('Ctrl Pts',(-110.927461150854,1074.90644753492,
416.769189489503));
#110950=CARTESIAN_POINT('Ctrl Pts',(-110.767625296664,1074.92966250548,
417.010720055326));
#110951=CARTESIAN_POINT('Ctrl Pts',(-110.712462791914,1074.93808223461,
417.146314622044));
#110952=CARTESIAN_POINT('Ctrl Pts',(-110.659106724347,1074.94748972575,
417.428081571844));
#110953=CARTESIAN_POINT('Ctrl Pts',(-110.660111085797,1074.9485578929,417.571079281942));
#110954=CARTESIAN_POINT('Ctrl Pts',(-110.716821982437,1074.94341878076,
417.848942680033));
#110955=CARTESIAN_POINT('Ctrl Pts',(-110.772035119322,1074.93725198434,
417.980970676675));
#110956=CARTESIAN_POINT('Ctrl Pts',(-110.931477108568,1074.91817490145,
418.219049774777));
#110957=CARTESIAN_POINT('Ctrl Pts',(-111.035157534774,1074.90530748675,
418.321970429161));
#110958=CARTESIAN_POINT('Ctrl Pts',(-111.276600097951,1074.87451979485,
418.481546744203));
#110959=CARTESIAN_POINT('Ctrl Pts',(-111.412102704599,1074.85688261778,
418.536456478853));
#110960=CARTESIAN_POINT('Ctrl Pts',(-111.621114619278,1074.82914878572,
418.57601257562));
#110961=CARTESIAN_POINT('Ctrl Pts',(-111.689080214018,1074.82005473184,
418.582376778178));
#110962=CARTESIAN_POINT('Ctrl Pts',(-111.757173944974,1074.8108674823,418.582363263141));
#110963=CARTESIAN_POINT('Origin',(-111.756957497768,1067.7251047501,417.491822535893));
#110964=CARTESIAN_POINT('',(-111.756957497768,1074.80630411877,417.982363284621));
#110965=CARTESIAN_POINT('',(-111.756957497768,1074.79784893105,417.001281787164));
#110966=CARTESIAN_POINT('Ctrl Pts',(-111.756957497768,1074.80630411877,
417.982363284621));
#110967=CARTESIAN_POINT('Ctrl Pts',(-111.758122579226,1074.80614680927,
417.982363284621));
#110968=CARTESIAN_POINT('Ctrl Pts',(-111.759287742904,1074.80598944682,
417.982359133837));
#110969=CARTESIAN_POINT('Ctrl Pts',(-111.792489563395,1074.80150414604,
417.982122540079));
#110970=CARTESIAN_POINT('Ctrl Pts',(-111.824428613561,1074.79715774821,
417.978756301525));
#110971=CARTESIAN_POINT('Ctrl Pts',(-111.920169596025,1074.7840323223,417.959058285948));
#110972=CARTESIAN_POINT('Ctrl Pts',(-111.98128266174,1074.77551819495,417.933006813256));
#110973=CARTESIAN_POINT('Ctrl Pts',(-112.088934161954,1074.76024863573,
417.858753351402));
#110974=CARTESIAN_POINT('Ctrl Pts',(-112.134628157483,1074.75361762822,
417.811572467289));
#110975=CARTESIAN_POINT('Ctrl Pts',(-112.204388627454,1074.74316509674,
417.702854312296));
#110976=CARTESIAN_POINT('Ctrl Pts',(-112.228128074018,1074.73940039555,
417.642649452916));
#110977=CARTESIAN_POINT('Ctrl Pts',(-112.250986578072,1074.73518380817,
417.516810173952));
#110978=CARTESIAN_POINT('Ctrl Pts',(-112.250054978383,1074.73475053742,
417.452494232804));
#110979=CARTESIAN_POINT('Ctrl Pts',(-112.223640476455,1074.73727160334,
417.32782259427));
#110980=CARTESIAN_POINT('Ctrl Pts',(-112.19843628193,1074.74019878948,417.268734382283));
#110981=CARTESIAN_POINT('Ctrl Pts',(-112.126731015357,1074.7490590343,417.163194451443));
#110982=CARTESIAN_POINT('Ctrl Pts',(-112.080798213839,1074.75492408497,
417.117885404554));
#110983=CARTESIAN_POINT('Ctrl Pts',(-111.973815063771,1074.76885940437,
417.047122570625));
#110984=CARTESIAN_POINT('Ctrl Pts',(-111.913642204305,1074.77681732983,
417.02255301957));
#110985=CARTESIAN_POINT('Ctrl Pts',(-111.819690596518,1074.78938851283,
417.004296465626));
#110986=CARTESIAN_POINT('Ctrl Pts',(-111.788356249039,1074.79360359439,
417.001281787164));
#110987=CARTESIAN_POINT('Ctrl Pts',(-111.756957497768,1074.79784893105,
417.001281787164));
#110988=CARTESIAN_POINT('',(-111.756957497768,1082.7251047501,417.001281787164));
#110989=CARTESIAN_POINT('',(-111.756957497768,1067.7251047501,417.001281787164));
#110990=CARTESIAN_POINT('Origin',(-111.756957497768,1082.7251047501,417.491822535893));
#110991=CARTESIAN_POINT('Ctrl Pts',(-111.756957497768,1074.79784893105,
417.001281787164));
#110992=CARTESIAN_POINT('Ctrl Pts',(-111.75689461651,1074.79785743305,417.001281787164));
#110993=CARTESIAN_POINT('Ctrl Pts',(-111.756831734994,1074.79786593517,
417.001281799255));
#110994=CARTESIAN_POINT('Ctrl Pts',(-111.756768853224,1074.79787443741,
417.001281823437));
#110995=CARTESIAN_POINT('Ctrl Pts',(-111.724708510328,1074.80220931429,
417.001294152707));
#110996=CARTESIAN_POINT('Ctrl Pts',(-111.692723880739,1074.80655641454,
417.004449512646));
#110997=CARTESIAN_POINT('Ctrl Pts',(-111.597177519773,1074.81961098445,
417.023451445351));
#110998=CARTESIAN_POINT('Ctrl Pts',(-111.536201424335,1074.82803720812,
417.048893667185));
#110999=CARTESIAN_POINT('Ctrl Pts',(-111.42793105659,1074.84321316049,417.122187470758));
#111000=CARTESIAN_POINT('Ctrl Pts',(-111.381641165088,1074.84982169605,
417.16924757614));
#111001=CARTESIAN_POINT('Ctrl Pts',(-111.310685003306,1074.86025526917,
417.278194578269));
#111002=CARTESIAN_POINT('Ctrl Pts',(-111.286433231381,1074.8640143001,417.33877238344));
#111003=CARTESIAN_POINT('Ctrl Pts',(-111.263022506741,1074.86822032095,
417.465038755468));
#111004=CARTESIAN_POINT('Ctrl Pts',(-111.263720260096,1074.86867504262,
417.529358895175));
#111005=CARTESIAN_POINT('Ctrl Pts',(-111.289697643028,1074.86626754205,
417.654201766278));
#111006=CARTESIAN_POINT('Ctrl Pts',(-111.314732530891,1074.86342703873,
417.713451591914));
#111007=CARTESIAN_POINT('Ctrl Pts',(-111.386207212044,1074.85476542394,
417.819367731334));
#111008=CARTESIAN_POINT('Ctrl Pts',(-111.432084671134,1074.84900924268,
417.864880964565));
#111009=CARTESIAN_POINT('Ctrl Pts',(-111.539816795936,1074.83516303436,
417.936532211971));
#111010=CARTESIAN_POINT('Ctrl Pts',(-111.600963410419,1074.82715661552,
417.961460574622));
#111011=CARTESIAN_POINT('Ctrl Pts',(-111.695393552302,1074.81458719603,
417.979460462524));
#111012=CARTESIAN_POINT('Ctrl Pts',(-111.726146777071,1074.81046418773,
417.982363284621));
#111013=CARTESIAN_POINT('Ctrl Pts',(-111.756957497768,1074.80630411877,
417.982363284621));
#111014=CARTESIAN_POINT('Origin',(-79.4772023228643,1067.7251047501,465.900390831321));
#111015=CARTESIAN_POINT('',(-79.4772023228921,1076.68910595681,464.422087699128));
#111016=CARTESIAN_POINT('',(-79.4772023228643,1067.7251047501,464.422087699128));
#111017=CARTESIAN_POINT('Ctrl Pts',(-79.4773207736094,1076.6535541543,467.378693958769));
#111018=CARTESIAN_POINT('Ctrl Pts',(-79.6713773118498,1076.64843867231,
467.378678409765));
#111019=CARTESIAN_POINT('Ctrl Pts',(-79.86355791831,1076.64366238044,467.340452351834));
#111020=CARTESIAN_POINT('Ctrl Pts',(-80.2221051063023,1076.63566604264,
467.191954301431));
#111021=CARTESIAN_POINT('Ctrl Pts',(-80.385001689945,1076.63252997765,467.08315387701));
#111022=CARTESIAN_POINT('Ctrl Pts',(-80.6592225868108,1076.62861881595,
466.8090805442));
#111023=CARTESIAN_POINT('Ctrl Pts',(-80.7679781329324,1076.62788120595,
466.646574536193));
#111024=CARTESIAN_POINT('Ctrl Pts',(-80.9164782089922,1076.62899174161,
466.289257129839));
#111025=CARTESIAN_POINT('Ctrl Pts',(-80.9549317568238,1076.63082244591,
466.09797586385));
#111026=CARTESIAN_POINT('Ctrl Pts',(-80.9560659558716,1076.63665533535,
465.711641132296));
#111027=CARTESIAN_POINT('Ctrl Pts',(-80.9187967152726,1076.6405940468,465.520314950613));
#111028=CARTESIAN_POINT('Ctrl Pts',(-80.7727863600171,1076.64975813045,
465.162712325768));
#111029=CARTESIAN_POINT('Ctrl Pts',(-80.6653957651852,1076.65488926548,
464.999892180117));
#111030=CARTESIAN_POINT('Ctrl Pts',(-80.4619123520525,1076.6627531713,464.793567716721));
#111031=CARTESIAN_POINT('Ctrl Pts',(-80.3875042400959,1076.66538434143,
464.731604357531));
#111032=CARTESIAN_POINT('Ctrl Pts',(-80.2276586167916,1076.67057108426,
464.623077804526));
#111033=CARTESIAN_POINT('Ctrl Pts',(-80.142603097741,1076.67311413955,464.576776185806));
#111034=CARTESIAN_POINT('Ctrl Pts',(-79.8734027534427,1076.68054042448,
464.46278330814));
#111035=CARTESIAN_POINT('Ctrl Pts',(-79.6797801662227,1076.68506645828,
464.423007479017));
#111036=CARTESIAN_POINT('Ctrl Pts',(-79.2892719337877,1076.69285388908,
464.421204035365));
#111037=CARTESIAN_POINT('Ctrl Pts',(-79.0962322658128,1076.69605170485,
464.458800853409));
#111038=CARTESIAN_POINT('Ctrl Pts',(-78.7350849451112,1076.70106353305,
464.60698613581));
#111039=CARTESIAN_POINT('Ctrl Pts',(-78.5706534717544,1076.70283087364,
464.716411105573));
#111040=CARTESIAN_POINT('Ctrl Pts',(-78.2932219028221,1076.70499407301,
464.993626917563));
#111041=CARTESIAN_POINT('Ctrl Pts',(-78.1832587368082,1076.70536681328,
465.15894531095));
#111042=CARTESIAN_POINT('Ctrl Pts',(-78.0345830847091,1076.70472822829,
465.52257559874));
#111043=CARTESIAN_POINT('Ctrl Pts',(-77.997223574233,1076.70372393956,465.717211250815));
#111044=CARTESIAN_POINT('Ctrl Pts',(-78.0006798152531,1076.70026427114,
466.108516119396));
#111045=CARTESIAN_POINT('Ctrl Pts',(-78.0409973261513,1076.69784400125,
466.301319033678));
#111046=CARTESIAN_POINT('Ctrl Pts',(-78.194107701336,1076.69153551541,466.660035848239));
#111047=CARTESIAN_POINT('Ctrl Pts',(-78.3053623993841,1076.68770177684,
466.822439755124));
#111048=CARTESIAN_POINT('Ctrl Pts',(-78.5133820383168,1076.68108741469,
467.025371971186));
#111049=CARTESIAN_POINT('Ctrl Pts',(-78.5881813312674,1076.67878159535,
467.085368776092));
#111050=CARTESIAN_POINT('Ctrl Pts',(-78.7499337728941,1076.67391472848,
467.191121363255));
#111051=CARTESIAN_POINT('Ctrl Pts',(-78.8367059389319,1076.67136132967,
467.236305672403));
#111052=CARTESIAN_POINT('Ctrl Pts',(-79.1021950212922,1076.66371040272,
467.342699065507));
#111053=CARTESIAN_POINT('Ctrl Pts',(-79.2888959287506,1076.65852118045,
467.378709056527));
#111054=CARTESIAN_POINT('Ctrl Pts',(-79.4773207736094,1076.6535541543,467.378693958769));
#111055=CARTESIAN_POINT('Origin',(-79.4772023228643,1067.7251047501,465.900390831321));
#111056=CARTESIAN_POINT('',(-79.4772023228642,1076.66179580959,466.778693963515));
#111057=CARTESIAN_POINT('',(-79.4772023228643,1076.68289265596,465.022087699128));
#111058=CARTESIAN_POINT('Ctrl Pts',(-79.4772023228642,1076.66179580959,
466.778693963515));
#111059=CARTESIAN_POINT('Ctrl Pts',(-79.4857706943264,1076.661581251,466.778693963515));
#111060=CARTESIAN_POINT('Ctrl Pts',(-79.4943443628444,1076.66136773358,
466.778568579773));
#111061=CARTESIAN_POINT('Ctrl Pts',(-79.6180460225395,1076.65830438857,
466.774944817879));
#111062=CARTESIAN_POINT('Ctrl Pts',(-79.7313993347598,1076.65571272977,
466.74895960446));
#111063=CARTESIAN_POINT('Ctrl Pts',(-79.9415719837507,1076.6514631756,466.654734254006));
#111064=CARTESIAN_POINT('Ctrl Pts',(-80.0363613716195,1076.64984857097,
466.587426342055));
#111065=CARTESIAN_POINT('Ctrl Pts',(-80.1944790720495,1076.64791978271,
466.42015987799));
#111066=CARTESIAN_POINT('Ctrl Pts',(-80.2563099089907,1076.64762411971,
466.32186195923));
#111067=CARTESIAN_POINT('Ctrl Pts',(-80.3385198977434,1076.64842148663,
466.107148066569));
#111068=CARTESIAN_POINT('Ctrl Pts',(-80.3581498408944,1076.64950465016,
465.99283240926));
#111069=CARTESIAN_POINT('Ctrl Pts',(-80.3522902572622,1076.65284946089,
465.763171373147));
#111070=CARTESIAN_POINT('Ctrl Pts',(-80.3268675305151,1076.65507640488,
465.650044443106));
#111071=CARTESIAN_POINT('Ctrl Pts',(-80.2339095005646,1076.66027249429,
465.439939545758));
#111072=CARTESIAN_POINT('Ctrl Pts',(-80.1672433907226,1076.66318946683,
465.344997078396));
#111073=CARTESIAN_POINT('Ctrl Pts',(-80.042700892681,1076.66771807545,465.225910284604));
#111074=CARTESIAN_POINT('Ctrl Pts',(-79.9974144236322,1076.66924207577,
465.190396467831));
#111075=CARTESIAN_POINT('Ctrl Pts',(-79.900589286229,1076.67226968345,465.12873531195));
#111076=CARTESIAN_POINT('Ctrl Pts',(-79.8492862372823,1076.67376602991,
465.10273019738));
#111077=CARTESIAN_POINT('Ctrl Pts',(-79.6942576590158,1076.67799255003,
465.042381510243));
#111078=CARTESIAN_POINT('Ctrl Pts',(-79.5862197918597,1076.68058364682,
465.022091072706));
#111079=CARTESIAN_POINT('Ctrl Pts',(-79.4772294980396,1076.68289208039,
465.022087699549));
#111080=CARTESIAN_POINT('Ctrl Pts',(-79.4772204396409,1076.68289227225,
465.022087699268));
#111081=CARTESIAN_POINT('Ctrl Pts',(-79.4772113812491,1076.68289246411,
465.022087699128));
#111082=CARTESIAN_POINT('Ctrl Pts',(-79.4772023228643,1076.68289265596,
465.022087699128));
#111083=CARTESIAN_POINT('',(-79.4772023228643,1082.7251047501,465.022087699128));
#111084=CARTESIAN_POINT('',(-79.4772023228643,1067.7251047501,465.022087699128));
#111085=CARTESIAN_POINT('Origin',(-79.4772023228643,1082.7251047501,465.900390831321));
#111086=CARTESIAN_POINT('Ctrl Pts',(-79.4772023228643,1076.68289265596,
465.022087699128));
#111087=CARTESIAN_POINT('Ctrl Pts',(-79.3608033170153,1076.68535795407,
465.022087699128));
#111088=CARTESIAN_POINT('Ctrl Pts',(-79.2455503107277,1076.68745541836,
465.04522672191));
#111089=CARTESIAN_POINT('Ctrl Pts',(-79.0304199919175,1076.69079932101,
465.135248625558));
#111090=CARTESIAN_POINT('Ctrl Pts',(-78.9327419473629,1076.69201259101,
465.201375736584));
#111091=CARTESIAN_POINT('Ctrl Pts',(-78.768703890884,1076.69348580652,465.368243895008));
#111092=CARTESIAN_POINT('Ctrl Pts',(-78.7040989728584,1076.69372956816,
465.467421941505));
#111093=CARTESIAN_POINT('Ctrl Pts',(-78.6176794381873,1076.69322646309,
465.685133549991));
#111094=CARTESIAN_POINT('Ctrl Pts',(-78.596676188045,1076.69248526583,465.801458285212));
#111095=CARTESIAN_POINT('Ctrl Pts',(-78.6014845360777,1076.69004089533,
466.035003685674));
#111096=CARTESIAN_POINT('Ctrl Pts',(-78.6270572558308,1076.68836333028,
466.149896022123));
#111097=CARTESIAN_POINT('Ctrl Pts',(-78.7215121176519,1076.68416339597,
466.362895931512));
#111098=CARTESIAN_POINT('Ctrl Pts',(-78.789423853008,1076.68168045485,466.458903395041));
#111099=CARTESIAN_POINT('Ctrl Pts',(-78.9155353807194,1076.67754967797,
466.5780338605));
#111100=CARTESIAN_POINT('Ctrl Pts',(-78.9607154788485,1076.67613226927,
466.613069501702));
#111101=CARTESIAN_POINT('Ctrl Pts',(-79.0573836203829,1076.67320938354,
466.673981829001));
#111102=CARTESIAN_POINT('Ctrl Pts',(-79.1086612891547,1076.67171059189,
466.699683105052));
#111103=CARTESIAN_POINT('Ctrl Pts',(-79.2627029750366,1076.66735002856,
466.75889487307));
#111104=CARTESIAN_POINT('Ctrl Pts',(-79.3695344822519,1076.66449189475,
466.778693963515));
#111105=CARTESIAN_POINT('Ctrl Pts',(-79.4772023228642,1076.66179580959,
466.778693963515));
#111106=CARTESIAN_POINT('Origin',(-90.2477595453604,1067.7251047501,459.442436531111));
#111107=CARTESIAN_POINT('',(-90.2477595453866,1076.37387335857,458.166992409975));
#111108=CARTESIAN_POINT('',(-90.2477595453604,1067.7251047501,458.166992409975));
#111109=CARTESIAN_POINT('Ctrl Pts',(-90.2473951380049,1076.31449558095,
460.717880600189));
#111110=CARTESIAN_POINT('Ctrl Pts',(-90.4149925201918,1076.30406321819,
460.717928484468));
#111111=CARTESIAN_POINT('Ctrl Pts',(-90.5810244388579,1076.29435900911,
460.684941623415));
#111112=CARTESIAN_POINT('Ctrl Pts',(-90.8906028854361,1076.27773119679,
460.556675727967));
#111113=CARTESIAN_POINT('Ctrl Pts',(-91.0311902148397,1076.27096807621,
460.462758836199));
#111114=CARTESIAN_POINT('Ctrl Pts',(-91.2677010387952,1076.26151736905,
460.226242819948));
#111115=CARTESIAN_POINT('Ctrl Pts',(-91.3614573749476,1076.25891190801,
460.086122300387));
#111116=CARTESIAN_POINT('Ctrl Pts',(-91.4894636636373,1076.25831245208,
459.77809376442));
#111117=CARTESIAN_POINT('Ctrl Pts',(-91.5226275761762,1076.26031136127,
459.613287069429));
#111118=CARTESIAN_POINT('Ctrl Pts',(-91.5237646897207,1076.2686084767,459.28035364862));
#111119=CARTESIAN_POINT('Ctrl Pts',(-91.4917496119433,1076.27482153916,
459.115471286924));
#111120=CARTESIAN_POINT('Ctrl Pts',(-91.3661653991122,1076.29050641563,
458.807052313795));
#111121=CARTESIAN_POINT('Ctrl Pts',(-91.273666100747,1076.29983013518,458.666536713084));
#111122=CARTESIAN_POINT('Ctrl Pts',(-91.0396594316448,1076.32019392865,
458.428752379496));
#111123=CARTESIAN_POINT('Ctrl Pts',(-90.9002504266469,1076.33104061181,
458.333877082239));
#111124=CARTESIAN_POINT('Ctrl Pts',(-90.6697075900341,1076.34728440329,
458.235917758385));
#111125=CARTESIAN_POINT('Ctrl Pts',(-90.5898448415355,1076.35265663299,
458.210889928147));
#111126=CARTESIAN_POINT('Ctrl Pts',(-90.3424368776555,1076.36856070555,
458.159302263942));
#111127=CARTESIAN_POINT('Ctrl Pts',(-90.1714882801023,1076.37856592741,
458.158063609476));
#111128=CARTESIAN_POINT('Ctrl Pts',(-89.8397465957344,1076.39621679187,
458.222313455795));
#111129=CARTESIAN_POINT('Ctrl Pts',(-89.6821722332112,1076.40370379496,
458.286872878131));
#111130=CARTESIAN_POINT('Ctrl Pts',(-89.4009393614874,1076.4153989733,458.473821287724));
#111131=CARTESIAN_POINT('Ctrl Pts',(-89.2801489336416,1076.41948958617,
458.594452002963));
#111132=CARTESIAN_POINT('Ctrl Pts',(-89.0924232299604,1076.42383922101,
458.876162491902));
#111133=CARTESIAN_POINT('Ctrl Pts',(-89.0274934847933,1076.42404876803,
459.034489783154));
#111134=CARTESIAN_POINT('Ctrl Pts',(-88.9633643405313,1076.42052079141,
459.366955042704));
#111135=CARTESIAN_POINT('Ctrl Pts',(-88.9646919349542,1076.41682369359,
459.537726478374));
#111136=CARTESIAN_POINT('Ctrl Pts',(-89.0337562040218,1076.40585083862,
459.868364025985));
#111137=CARTESIAN_POINT('Ctrl Pts',(-89.100659739176,1076.39868710692,460.024964939687));
#111138=CARTESIAN_POINT('Ctrl Pts',(-89.2917513009851,1076.3815753021,460.303503544349));
#111139=CARTESIAN_POINT('Ctrl Pts',(-89.4142549940543,1076.3717819452,460.422550099397));
#111140=CARTESIAN_POINT('Ctrl Pts',(-89.6998581839638,1076.35063884563,
460.606792905232));
#111141=CARTESIAN_POINT('Ctrl Pts',(-89.8604942758898,1076.33948408229,
460.669603518788));
#111142=CARTESIAN_POINT('Ctrl Pts',(-90.1009177432434,1076.32373433747,
460.711518116806));
#111143=CARTESIAN_POINT('Ctrl Pts',(-90.1740847277611,1076.31905890279,
460.717859654659));
#111144=CARTESIAN_POINT('Ctrl Pts',(-90.2473951380049,1076.31449558095,
460.717880600189));
#111145=CARTESIAN_POINT('Origin',(-90.2477595453604,1067.7251047501,459.442436531111));
#111146=CARTESIAN_POINT('',(-90.2477595453604,1076.32917837425,460.117880652247));
#111147=CARTESIAN_POINT('',(-90.2477595453606,1076.3606248843,458.766992409975));
#111148=CARTESIAN_POINT('Ctrl Pts',(-90.2477595453603,1076.32917837425,
460.117880652247));
#111149=CARTESIAN_POINT('Ctrl Pts',(-90.2572965053981,1076.32859342499,
460.117880652247));
#111150=CARTESIAN_POINT('Ctrl Pts',(-90.266841445427,1076.32801224415,460.117678667997));
#111151=CARTESIAN_POINT('Ctrl Pts',(-90.3649713709435,1076.32208148596,
460.113515719287));
#111152=CARTESIAN_POINT('Ctrl Pts',(-90.4519859111912,1076.31719251032,
460.092350909843));
#111153=CARTESIAN_POINT('Ctrl Pts',(-90.6127328843783,1076.3089705214,460.01763878999));
#111154=CARTESIAN_POINT('Ctrl Pts',(-90.6849346217564,1076.30571522265,
459.964885283311));
#111155=CARTESIAN_POINT('Ctrl Pts',(-90.8047232882335,1076.30134150474,
459.834639139193));
#111156=CARTESIAN_POINT('Ctrl Pts',(-90.8512057910747,1076.30026087909,
459.758488254488));
#111157=CARTESIAN_POINT('Ctrl Pts',(-90.9121552741609,1076.3004507403,459.592727808095));
#111158=CARTESIAN_POINT('Ctrl Pts',(-90.9260802207466,1076.30171526864,
459.504765666679));
#111159=CARTESIAN_POINT('Ctrl Pts',(-90.9193391352392,1076.30641611299,
459.328451622158));
#111160=CARTESIAN_POINT('Ctrl Pts',(-90.8987220164565,1076.309806762,459.24181781014));
#111161=CARTESIAN_POINT('Ctrl Pts',(-90.8253166579501,1076.31823580457,
459.081237916383));
#111162=CARTESIAN_POINT('Ctrl Pts',(-90.7731619803815,1076.32319538349,
459.008872035341));
#111163=CARTESIAN_POINT('Ctrl Pts',(-90.6438585005819,1076.33398835859,
458.888208399147));
#111164=CARTESIAN_POINT('Ctrl Pts',(-90.5678881490822,1076.33971955767,
458.841123369004));
#111165=CARTESIAN_POINT('Ctrl Pts',(-90.409162252535,1076.35067725464,458.781575796335));
#111166=CARTESIAN_POINT('Ctrl Pts',(-90.3287961942446,1076.35581800331,
458.766992409975));
#111167=CARTESIAN_POINT('Ctrl Pts',(-90.2477595453608,1076.3606248843,458.766992409975));
#111168=CARTESIAN_POINT('',(-90.2477595453604,1082.7251047501,458.766992409975));
#111169=CARTESIAN_POINT('',(-90.2477595453604,1067.7251047501,458.766992409975));
#111170=CARTESIAN_POINT('Origin',(-90.2477595453604,1082.7251047501,459.442436531111));
#111171=CARTESIAN_POINT('Ctrl Pts',(-90.2477595453608,1076.3606248843,458.766992409975));
#111172=CARTESIAN_POINT('Ctrl Pts',(-90.2476740819054,1076.36062995377,
458.766992409975));
#111173=CARTESIAN_POINT('Ctrl Pts',(-90.2475886177041,1076.36063502286,
458.766992426301));
#111174=CARTESIAN_POINT('Ctrl Pts',(-90.2475031527616,1076.36064009159,
458.766992458742));
#111175=CARTESIAN_POINT('Ctrl Pts',(-90.1576841753495,1076.36596704673,
458.767026553234));
#111176=CARTESIAN_POINT('Ctrl Pts',(-90.0687357095448,1076.37078390744,
458.784976170086));
#111177=CARTESIAN_POINT('Ctrl Pts',(-89.9031079874359,1076.37888217561,
458.854640640584));
#111178=CARTESIAN_POINT('Ctrl Pts',(-89.8280721524695,1076.38208554669,
458.905629095858));
#111179=CARTESIAN_POINT('Ctrl Pts',(-89.7022535079224,1076.38648665427,
459.034098107516));
#111180=CARTESIAN_POINT('Ctrl Pts',(-89.6527700077903,1076.38763878941,
459.110308275996));
#111181=CARTESIAN_POINT('Ctrl Pts',(-89.5865703611777,1076.38773229927,
459.277660306333));
#111182=CARTESIAN_POINT('Ctrl Pts',(-89.5705276812917,1076.38667266553,
459.367103428081));
#111183=CARTESIAN_POINT('Ctrl Pts',(-89.5744170575338,1076.38244544676,
459.546889603371));
#111184=CARTESIAN_POINT('Ctrl Pts',(-89.594270106551,1076.37932178872,459.635416429416));
#111185=CARTESIAN_POINT('Ctrl Pts',(-89.6674262014148,1076.37136061123,
459.799529708689));
#111186=CARTESIAN_POINT('Ctrl Pts',(-89.7200223908945,1076.36660000202,
459.873463499818));
#111187=CARTESIAN_POINT('Ctrl Pts',(-89.8512791660716,1076.35600260715,
459.99666138276));
#111188=CARTESIAN_POINT('Ctrl Pts',(-89.9287443458786,1076.35026587117,
460.044587310458));
#111189=CARTESIAN_POINT('Ctrl Pts',(-90.0884175699086,1076.33924971808,
460.103684060641));
#111190=CARTESIAN_POINT('Ctrl Pts',(-90.1678081753738,1076.33408218995,
460.117880652247));
#111191=CARTESIAN_POINT('Ctrl Pts',(-90.2477595453603,1076.32917837425,
460.117880652247));
#111192=CARTESIAN_POINT('Origin',(-101.429261354592,1067.7251047501,451.269782488757));
#111193=CARTESIAN_POINT('',(-101.429261354619,1075.68385821193,450.170951352764));
#111194=CARTESIAN_POINT('',(-101.429261354592,1067.7251047501,450.170951352764));
#111195=CARTESIAN_POINT('Ctrl Pts',(-101.428824831104,1075.62575125877,
452.368613538042));
#111196=CARTESIAN_POINT('Ctrl Pts',(-101.573543970317,1075.61103511209,
452.368671029413));
#111197=CARTESIAN_POINT('Ctrl Pts',(-101.716968304491,1075.59710718154,
452.340138063898));
#111198=CARTESIAN_POINT('Ctrl Pts',(-101.98404922685,1075.57260139272,452.229186104905));
#111199=CARTESIAN_POINT('Ctrl Pts',(-102.105224112842,1075.56224700518,
452.148078505666));
#111200=CARTESIAN_POINT('Ctrl Pts',(-102.308724606694,1075.54666616046,
451.944023198637));
#111201=CARTESIAN_POINT('Ctrl Pts',(-102.389291852746,1075.54156266542,
451.823362835185));
#111202=CARTESIAN_POINT('Ctrl Pts',(-102.499149199234,1075.53736334671,
451.558313457678));
#111203=CARTESIAN_POINT('Ctrl Pts',(-102.527586606201,1075.53828136185,
451.416689367917));
#111204=CARTESIAN_POINT('Ctrl Pts',(-102.528585005851,1075.54602103374,
451.130541210698));
#111205=CARTESIAN_POINT('Ctrl Pts',(-102.501137546036,1075.55276429535,
450.988863241077));
#111206=CARTESIAN_POINT('Ctrl Pts',(-102.393426157324,1075.57116695209,
450.723503440223));
#111207=CARTESIAN_POINT('Ctrl Pts',(-102.313957484765,1075.58266800443,
450.602500278067));
#111208=CARTESIAN_POINT('Ctrl Pts',(-102.112659620965,1075.60886453958,
450.397324375233));
#111209=CARTESIAN_POINT('Ctrl Pts',(-101.992478980741,1075.62332820295,
450.315343042515));
#111210=CARTESIAN_POINT('Ctrl Pts',(-101.793664510477,1075.64571534432,
450.23062965139));
#111211=CARTESIAN_POINT('Ctrl Pts',(-101.724714463618,1075.65324654696,
450.208964154126));
#111212=CARTESIAN_POINT('Ctrl Pts',(-101.51092097434,1075.67591701036,450.164264299751));
#111213=CARTESIAN_POINT('Ctrl Pts',(-101.363073605718,1075.69068622292,
450.163209338025));
#111214=CARTESIAN_POINT('Ctrl Pts',(-101.076433525723,1075.71762090883,
450.219008594389));
#111215=CARTESIAN_POINT('Ctrl Pts',(-100.94037211969,1075.72954308128,450.274955108786));
#111216=CARTESIAN_POINT('Ctrl Pts',(-100.697957721304,1075.74909097304,
450.436810959434));
#111217=CARTESIAN_POINT('Ctrl Pts',(-100.594000675888,1075.75652868986,
450.541046538769));
#111218=CARTESIAN_POINT('Ctrl Pts',(-100.432679844794,1075.76597495695,
450.784404075123));
#111219=CARTESIAN_POINT('Ctrl Pts',(-100.377033325883,1075.76788171489,
450.921065603358));
#111220=CARTESIAN_POINT('Ctrl Pts',(-100.322475883854,1075.76586122839,
451.208157841083));
#111221=CARTESIAN_POINT('Ctrl Pts',(-100.324107852411,1075.76195662614,
451.355612832337));
#111222=CARTESIAN_POINT('Ctrl Pts',(-100.384802397907,1075.74876668641,
451.640992358975));
#111223=CARTESIAN_POINT('Ctrl Pts',(-100.443189323568,1075.73961841438,
451.776017968428));
#111224=CARTESIAN_POINT('Ctrl Pts',(-100.609221178158,1075.71713607322,
452.015616628179));
#111225=CARTESIAN_POINT('Ctrl Pts',(-100.715352191986,1075.70401092934,
452.117717880423));
#111226=CARTESIAN_POINT('Ctrl Pts',(-100.898457705771,1075.68273065259,
452.2345567985));
#111227=CARTESIAN_POINT('Ctrl Pts',(-100.962326366096,1075.67549874985,
452.267033044876));
#111228=CARTESIAN_POINT('Ctrl Pts',(-101.092160019658,1075.66114233945,
452.317833223314));
#111229=CARTESIAN_POINT('Ctrl Pts',(-101.157599505607,1075.65405970112,
452.33666879454));
#111230=CARTESIAN_POINT('Ctrl Pts',(-101.291751240266,1075.63983794698,
452.362131740878));
#111231=CARTESIAN_POINT('Ctrl Pts',(-101.360207120892,1075.63272883129,
452.368586278854));
#111232=CARTESIAN_POINT('Ctrl Pts',(-101.428824831104,1075.62575125877,
452.368613538042));
#111233=CARTESIAN_POINT('Origin',(-101.429261354592,1067.7251047501,451.269782488757));
#111234=CARTESIAN_POINT('',(-101.429261354592,1075.64217240143,451.768613624749));
#111235=CARTESIAN_POINT('',(-101.429261354593,1075.66856733728,450.770951352764));
#111236=CARTESIAN_POINT('Ctrl Pts',(-101.429261354592,1075.64217240143,
451.768613624749));
#111237=CARTESIAN_POINT('Ctrl Pts',(-101.466625322109,1075.63839354457,
451.768613624749));
#111238=CARTESIAN_POINT('Ctrl Pts',(-101.503974500602,1075.63472064406,
451.76441563379));
#111239=CARTESIAN_POINT('Ctrl Pts',(-101.604479016645,1075.6251333703,451.741403281128));
#111240=CARTESIAN_POINT('Ctrl Pts',(-101.664919483172,1075.61970292959,
451.71431521238));
#111241=CARTESIAN_POINT('Ctrl Pts',(-101.771609546742,1075.61085297973,
451.638415711296));
#111242=CARTESIAN_POINT('Ctrl Pts',(-101.816900766962,1075.6075086123,451.590473884824));
#111243=CARTESIAN_POINT('Ctrl Pts',(-101.886268944348,1075.60337917568,
451.480035129975));
#111244=CARTESIAN_POINT('Ctrl Pts',(-101.909766742443,1075.60262211248,
451.418713403683));
#111245=CARTESIAN_POINT('Ctrl Pts',(-101.931875986063,1075.60380581233,
451.29057206556));
#111246=CARTESIAN_POINT('Ctrl Pts',(-101.930302916489,1075.60573073487,
451.22503969026));
#111247=CARTESIAN_POINT('Ctrl Pts',(-101.902126735514,1075.61202024156,
451.098110585345));
#111248=CARTESIAN_POINT('Ctrl Pts',(-101.875718903519,1075.61633035449,
451.037980671676));
#111249=CARTESIAN_POINT('Ctrl Pts',(-101.801195055009,1075.62677977734,
450.931000457423));
#111250=CARTESIAN_POINT('Ctrl Pts',(-101.753667768507,1075.63282862234,
450.885264232718));
#111251=CARTESIAN_POINT('Ctrl Pts',(-101.671194895238,1075.64258551325,
450.832322134364));
#111252=CARTESIAN_POINT('Ctrl Pts',(-101.641988912993,1075.64593367939,
450.817400432505));
#111253=CARTESIAN_POINT('Ctrl Pts',(-101.582652265061,1075.65253818379,
450.794107385504));
#111254=CARTESIAN_POINT('Ctrl Pts',(-101.552769804416,1075.65577663001,
450.785487935513));
#111255=CARTESIAN_POINT('Ctrl Pts',(-101.491621722104,1075.66223332618,
450.773881744183));
#111256=CARTESIAN_POINT('Ctrl Pts',(-101.460478627276,1075.66543770614,
450.770951352764));
#111257=CARTESIAN_POINT('Ctrl Pts',(-101.429261354593,1075.66856733728,
450.770951352764));
#111258=CARTESIAN_POINT('',(-101.429261354592,1082.7251047501,450.770951352764));
#111259=CARTESIAN_POINT('',(-101.429261354592,1067.7251047501,450.770951352764));
#111260=CARTESIAN_POINT('Origin',(-101.429261354592,1082.7251047501,451.269782488757));
#111261=CARTESIAN_POINT('Ctrl Pts',(-101.429261354593,1075.66856733728,
450.770951352764));
#111262=CARTESIAN_POINT('Ctrl Pts',(-101.429175761062,1075.6685759183,450.770951352764));
#111263=CARTESIAN_POINT('Ctrl Pts',(-101.429090166973,1075.66858449877,
450.770951374888));
#111264=CARTESIAN_POINT('Ctrl Pts',(-101.429004572336,1075.66859307867,
450.770951418949));
#111265=CARTESIAN_POINT('Ctrl Pts',(-101.362529805005,1075.67525642691,
450.770985638031));
#111266=CARTESIAN_POINT('Ctrl Pts',(-101.296673859189,1075.68148464945,
450.784307273578));
#111267=CARTESIAN_POINT('Ctrl Pts',(-101.17416604199,1075.69233675057,450.836001435219));
#111268=CARTESIAN_POINT('Ctrl Pts',(-101.118705158814,1075.69685802441,
450.873787915152));
#111269=CARTESIAN_POINT('Ctrl Pts',(-101.026316089801,1075.70355338138,
450.968463479552));
#111270=CARTESIAN_POINT('Ctrl Pts',(-100.990115036859,1075.70568647433,
451.024184226064));
#111271=CARTESIAN_POINT('Ctrl Pts',(-100.941739472419,1075.70731242583,
451.14576370675));
#111272=CARTESIAN_POINT('Ctrl Pts',(-100.929746901932,1075.70682245188,
451.210274363339));
#111273=CARTESIAN_POINT('Ctrl Pts',(-100.931175069105,1075.70329699079,
451.340371816795));
#111274=CARTESIAN_POINT('Ctrl Pts',(-100.944631276456,1075.70029130348,
451.404665834681));
#111275=CARTESIAN_POINT('Ctrl Pts',(-100.995984741017,1075.69203156629,
451.525769431355));
#111276=CARTESIAN_POINT('Ctrl Pts',(-101.033917198477,1075.68681056514,
451.581140146956));
#111277=CARTESIAN_POINT('Ctrl Pts',(-101.12929508331,1075.67485578366,451.673878168055));
#111278=CARTESIAN_POINT('Ctrl Pts',(-101.185866774295,1075.66823437907,
451.710261001859));
#111279=CARTESIAN_POINT('Ctrl Pts',(-101.278243710066,1075.6579987126,451.746321634162));
#111280=CARTESIAN_POINT('Ctrl Pts',(-101.309709438091,1075.65459710411,
451.755172100283));
#111281=CARTESIAN_POINT('Ctrl Pts',(-101.37074274857,1075.64815481417,451.766040101891));
#111282=CARTESIAN_POINT('Ctrl Pts',(-101.400006584011,1075.64513112337,
451.768613624749));
#111283=CARTESIAN_POINT('Ctrl Pts',(-101.429261354592,1075.64217240143,
451.768613624749));
#111284=CARTESIAN_POINT('Origin',(-110.796881705951,1067.7251047501,440.88317361084));
#111285=CARTESIAN_POINT('',(-110.796881705974,1074.82291082631,439.792632862112));
#111286=CARTESIAN_POINT('',(-110.796881705951,1067.7251047501,439.792632862112));
#111287=CARTESIAN_POINT('Ctrl Pts',(-110.797105361067,1074.77999286998,
441.973714336634));
#111288=CARTESIAN_POINT('Ctrl Pts',(-110.94348355177,1074.76031515429,441.973684316452));
#111289=CARTESIAN_POINT('Ctrl Pts',(-111.088520200642,1074.74130263312,
441.944183028484));
#111290=CARTESIAN_POINT('Ctrl Pts',(-111.355468495658,1074.70735540124,
441.830707025445));
#111291=CARTESIAN_POINT('Ctrl Pts',(-111.47530196927,1074.69266196889,441.749039437982));
#111292=CARTESIAN_POINT('Ctrl Pts',(-111.675601131087,1074.66941281543,
441.544538841122));
#111293=CARTESIAN_POINT('Ctrl Pts',(-111.754483912226,1074.66102693366,
441.424151601835));
#111294=CARTESIAN_POINT('Ctrl Pts',(-111.86103748437,1074.65172829746,441.160494132515));
#111295=CARTESIAN_POINT('Ctrl Pts',(-111.888028253745,1074.65085210625,
441.020088872214));
#111296=CARTESIAN_POINT('Ctrl Pts',(-111.886796482441,1074.6567199401,440.736877025722));
#111297=CARTESIAN_POINT('Ctrl Pts',(-111.858630045261,1074.66339754126,
440.596957194216));
#111298=CARTESIAN_POINT('Ctrl Pts',(-111.750295413962,1074.6834619519,440.334980400228));
#111299=CARTESIAN_POINT('Ctrl Pts',(-111.670842497709,1074.69669386072,
440.21566274908));
#111300=CARTESIAN_POINT('Ctrl Pts',(-111.470078312828,1074.72800902203,
440.01334173779));
#111301=CARTESIAN_POINT('Ctrl Pts',(-111.350259188695,1074.74583983454,
439.932662373144));
#111302=CARTESIAN_POINT('Ctrl Pts',(-111.152549809805,1074.77412359308,
439.849786511264));
#111303=CARTESIAN_POINT('Ctrl Pts',(-111.084083513385,1074.78374592789,
439.828707263087));
#111304=CARTESIAN_POINT('Ctrl Pts',(-110.944321453409,1074.80305320118,
439.800304398657));
#111305=CARTESIAN_POINT('Ctrl Pts',(-110.873349194707,1074.81269472288,
439.792990457562));
#111306=CARTESIAN_POINT('Ctrl Pts',(-110.657571261627,1074.8415236111,439.791945286038));
#111307=CARTESIAN_POINT('Ctrl Pts',(-110.514112629573,1074.86003078403,
439.820008247311));
#111308=CARTESIAN_POINT('Ctrl Pts',(-110.246794346848,1074.89324742946,
439.930534675914));
#111309=CARTESIAN_POINT('Ctrl Pts',(-110.125441587613,1074.90765269428,
440.011724697301));
#111310=CARTESIAN_POINT('Ctrl Pts',(-109.922203971637,1074.93039849742,
440.216234446847));
#111311=CARTESIAN_POINT('Ctrl Pts',(-109.842005480321,1074.93856779183,
440.337112198895));
#111312=CARTESIAN_POINT('Ctrl Pts',(-109.733915731825,1074.94762980625,
440.601325409095));
#111313=CARTESIAN_POINT('Ctrl Pts',(-109.706326683477,1074.94854259667,
440.741620931826));
#111314=CARTESIAN_POINT('Ctrl Pts',(-109.706355270303,1074.94309864505,
441.025226449537));
#111315=CARTESIAN_POINT('Ctrl Pts',(-109.734079176414,1074.93678250172,
441.165657709974));
#111316=CARTESIAN_POINT('Ctrl Pts',(-109.842760866284,1074.9174281049,441.430838479501));
#111317=CARTESIAN_POINT('Ctrl Pts',(-109.923803895461,1074.90443647703,
441.552413102722));
#111318=CARTESIAN_POINT('Ctrl Pts',(-110.128406458997,1074.87346552783,
441.756895815543));
#111319=CARTESIAN_POINT('Ctrl Pts',(-110.250054594975,1074.85577660562,
441.837699186511));
#111320=CARTESIAN_POINT('Ctrl Pts',(-110.448836749423,1074.82771140611,
441.919076633296));
#111321=CARTESIAN_POINT('Ctrl Pts',(-110.516364905335,1074.81829981499,
441.939362542594));
#111322=CARTESIAN_POINT('Ctrl Pts',(-110.655091245718,1074.79919877588,
441.966791599466));
#111323=CARTESIAN_POINT('Ctrl Pts',(-110.726012464015,1074.78954993452,
441.973728916823));
#111324=CARTESIAN_POINT('Ctrl Pts',(-110.797105361067,1074.77999286998,
441.973714336634));
#111325=CARTESIAN_POINT('Origin',(-110.796881705951,1067.7251047501,440.88317361084));
#111326=CARTESIAN_POINT('',(-110.796881705951,1074.79242545665,441.373714359568));
#111327=CARTESIAN_POINT('',(-110.796881705951,1074.81171529132,440.392632862112));
#111328=CARTESIAN_POINT('Ctrl Pts',(-110.796881705951,1074.79242545665,
441.373714359568));
#111329=CARTESIAN_POINT('Ctrl Pts',(-110.797786191687,1074.79230410707,
441.373714359568));
#111330=CARTESIAN_POINT('Ctrl Pts',(-110.798690737079,1074.79218279516,
441.373711857939));
#111331=CARTESIAN_POINT('Ctrl Pts',(-110.865211266256,1074.78326484229,
441.37334386692));
#111332=CARTESIAN_POINT('Ctrl Pts',(-110.930162714815,1074.77479705536,
441.359818516996));
#111333=CARTESIAN_POINT('Ctrl Pts',(-111.050222236907,1074.75964388772,
441.308218999479));
#111334=CARTESIAN_POINT('Ctrl Pts',(-111.10429124951,1074.75308331224,441.270952994277));
#111335=CARTESIAN_POINT('Ctrl Pts',(-111.194042578868,1074.74279701432,
441.17811141175));
#111336=CARTESIAN_POINT('Ctrl Pts',(-111.229146768844,1074.73912533272,
441.123783231449));
#111337=CARTESIAN_POINT('Ctrl Pts',(-111.276317327878,1074.73510149318,
441.004949108279));
#111338=CARTESIAN_POINT('Ctrl Pts',(-111.288065990577,1074.73476714158,
440.941721814427));
#111339=CARTESIAN_POINT('Ctrl Pts',(-111.286724467102,1074.73748093841,
440.814289054747));
#111340=CARTESIAN_POINT('Ctrl Pts',(-111.27364581082,1074.7405016105,440.751380682394));
#111341=CARTESIAN_POINT('Ctrl Pts',(-111.224104855968,1074.74953313192,
440.633747223378));
#111342=CARTESIAN_POINT('Ctrl Pts',(-111.187966971081,1074.75547515032,
440.580257315185));
#111343=CARTESIAN_POINT('Ctrl Pts',(-111.096945747979,1074.76953619832,
440.489789711359));
#111344=CARTESIAN_POINT('Ctrl Pts',(-111.042749008856,1074.7775414189,440.453851251935));
#111345=CARTESIAN_POINT('Ctrl Pts',(-110.953841827618,1074.79020181952,
440.417336716221));
#111346=CARTESIAN_POINT('Ctrl Pts',(-110.923343030664,1074.79447471961,
440.408150353881));
#111347=CARTESIAN_POINT('Ctrl Pts',(-110.860796572288,1074.80310121376,
440.395763566507));
#111348=CARTESIAN_POINT('Ctrl Pts',(-110.828879020003,1074.80743593212,
440.392632862112));
#111349=CARTESIAN_POINT('Ctrl Pts',(-110.796881705951,1074.81171529132,
440.392632862112));
#111350=CARTESIAN_POINT('',(-110.796881705951,1082.7251047501,440.392632862112));
#111351=CARTESIAN_POINT('',(-110.796881705951,1067.7251047501,440.392632862112));
#111352=CARTESIAN_POINT('Origin',(-110.796881705951,1082.7251047501,440.88317361084));
#111353=CARTESIAN_POINT('Ctrl Pts',(-110.796881705951,1074.81171529132,
440.392632862112));
#111354=CARTESIAN_POINT('Ctrl Pts',(-110.796800433509,1074.8117261608,440.392632862112));
#111355=CARTESIAN_POINT('Ctrl Pts',(-110.796719160552,1074.81173702992,
440.392632882309));
#111356=CARTESIAN_POINT('Ctrl Pts',(-110.796637887089,1074.81174789867,
440.392632922706));
#111357=CARTESIAN_POINT('Ctrl Pts',(-110.731386270444,1074.82047404469,
440.392665355438));
#111358=CARTESIAN_POINT('Ctrl Pts',(-110.666720623711,1074.8288468084,440.405717121953));
#111359=CARTESIAN_POINT('Ctrl Pts',(-110.546326109029,1074.84389122311,
440.456431152121));
#111360=CARTESIAN_POINT('Ctrl Pts',(-110.491749163602,1074.8504206601,440.493545729109));
#111361=CARTESIAN_POINT('Ctrl Pts',(-110.400901860152,1074.86066985068,
440.586533917516));
#111362=CARTESIAN_POINT('Ctrl Pts',(-110.365295313079,1074.86432560277,
440.641204083187));
#111363=CARTESIAN_POINT('Ctrl Pts',(-110.317687268505,1074.86831513604,
440.760451244923));
#111364=CARTESIAN_POINT('Ctrl Pts',(-110.305813334118,1074.86865888794,
440.823658359471));
#111365=CARTESIAN_POINT('Ctrl Pts',(-110.30690528324,1074.86603420645,440.951175505274));
#111366=CARTESIAN_POINT('Ctrl Pts',(-110.31989222242,1074.86308803514,441.014189692276));
#111367=CARTESIAN_POINT('Ctrl Pts',(-110.369332767942,1074.85423162507,
441.132067233784));
#111368=CARTESIAN_POINT('Ctrl Pts',(-110.405467601649,1074.84838740974,
441.185686945772));
#111369=CARTESIAN_POINT('Ctrl Pts',(-110.497127501705,1074.83440666427,
441.276942815033));
#111370=CARTESIAN_POINT('Ctrl Pts',(-110.552165749063,1074.82635909903,
441.313288309164));
#111371=CARTESIAN_POINT('Ctrl Pts',(-110.642223161231,1074.81361095413,
441.349790887485));
#111372=CARTESIAN_POINT('Ctrl Pts',(-110.672926082968,1074.8093264257,441.358867733615));
#111373=CARTESIAN_POINT('Ctrl Pts',(-110.734800811584,1074.80080836035,
441.370761405948));
#111374=CARTESIAN_POINT('Ctrl Pts',(-110.76580605255,1074.79659469598,441.373714359568));
#111375=CARTESIAN_POINT('Ctrl Pts',(-110.796881705951,1074.79242545665,
441.373714359568));
#111376=CARTESIAN_POINT('Origin',(-69.1578093449747,1067.7251047501,481.522560066374));
#111377=CARTESIAN_POINT('',(-69.1578093449979,1076.6946925711,480.044256934181));
#111378=CARTESIAN_POINT('',(-69.1578093449747,1067.7251047501,480.044256934181));
#111379=CARTESIAN_POINT('Ctrl Pts',(-69.1578534910652,1076.64572415765,
483.000863197909));
#111380=CARTESIAN_POINT('Ctrl Pts',(-69.3520466123464,1076.64107006247,
483.000857398782));
#111381=CARTESIAN_POINT('Ctrl Pts',(-69.5443646856791,1076.63704453658,
482.96258724071));
#111382=CARTESIAN_POINT('Ctrl Pts',(-69.9029585790611,1076.63104156109,
482.813973068201));
#111383=CARTESIAN_POINT('Ctrl Pts',(-70.06578441007,1076.62912526241,482.705177728005));
#111384=CARTESIAN_POINT('Ctrl Pts',(-70.3397664037465,1076.62785868295,
482.43128278759));
#111385=CARTESIAN_POINT('Ctrl Pts',(-70.4484034651645,1076.6285149798,482.26899375864));
#111386=CARTESIAN_POINT('Ctrl Pts',(-70.5968530602563,1076.63226388891,
481.912171287804));
#111387=CARTESIAN_POINT('Ctrl Pts',(-70.635373255508,1076.63531162612,481.7211479596));
#111388=CARTESIAN_POINT('Ctrl Pts',(-70.6368305743748,1076.64314502678,
481.335148627493));
#111389=CARTESIAN_POINT('Ctrl Pts',(-70.5997593297441,1076.64784852514,
481.143881781424));
#111390=CARTESIAN_POINT('Ctrl Pts',(-70.4541500357107,1076.65797750975,
480.786211519797));
#111391=CARTESIAN_POINT('Ctrl Pts',(-70.3469225550915,1076.66330023062,
480.623272986609));
#111392=CARTESIAN_POINT('Ctrl Pts',(-70.1436357428308,1076.67106272851,
480.41673104042));
#111393=CARTESIAN_POINT('Ctrl Pts',(-70.069288050044,1076.67359620194,480.354690715285));
#111394=CARTESIAN_POINT('Ctrl Pts',(-69.8271376497734,1076.68099936237,
480.189928182539));
#111395=CARTESIAN_POINT('Ctrl Pts',(-69.644467384676,1076.68550062963,480.112921324492));
#111396=CARTESIAN_POINT('Ctrl Pts',(-69.2610670673237,1076.69321259593,
480.035041249039));
#111397=CARTESIAN_POINT('Ctrl Pts',(-69.0642350746438,1076.69636314841,
480.034397912974));
#111398=CARTESIAN_POINT('Ctrl Pts',(-68.6813723762028,1076.70127064601,
480.109583154842));
#111399=CARTESIAN_POINT('Ctrl Pts',(-68.4991289955559,1076.70298574406,
480.184785473457));
#111400=CARTESIAN_POINT('Ctrl Pts',(-68.1738614375616,1076.70504878505,
480.402023564848));
#111401=CARTESIAN_POINT('Ctrl Pts',(-68.0341946314356,1076.705376912,480.542128323284));
#111402=CARTESIAN_POINT('Ctrl Pts',(-67.8177661864602,1076.70465733861,
480.868393826114));
#111403=CARTESIAN_POINT('Ctrl Pts',(-67.7430559236265,1076.7036167256,481.051265004334));
#111404=CARTESIAN_POINT('Ctrl Pts',(-67.6692951014785,1076.70008714064,
481.434786315442));
#111405=CARTESIAN_POINT('Ctrl Pts',(-67.6707044431848,1076.69763031507,
481.631606673994));
#111406=CARTESIAN_POINT('Ctrl Pts',(-67.7498936363522,1076.69124335579,
482.013827147402));
#111407=CARTESIAN_POINT('Ctrl Pts',(-67.8270903594424,1076.68736423883,
482.195425233566));
#111408=CARTESIAN_POINT('Ctrl Pts',(-67.9915155812525,1076.68068561915,
482.435989318868));
#111409=CARTESIAN_POINT('Ctrl Pts',(-68.0532692814349,1076.67835803169,
482.50977044806));
#111410=CARTESIAN_POINT('Ctrl Pts',(-68.1913390059092,1076.67345969519,
482.645430029059));
#111411=CARTESIAN_POINT('Ctrl Pts',(-68.2675419814773,1076.6708974976,482.706758169247));
#111412=CARTESIAN_POINT('Ctrl Pts',(-68.5116665156276,1076.66307951883,
482.866260119487));
#111413=CARTESIAN_POINT('Ctrl Pts',(-68.6934238718275,1076.65773437225,
482.939379589634));
#111414=CARTESIAN_POINT('Ctrl Pts',(-68.9743622230062,1076.65025167938,
482.992309082317));
#111415=CARTESIAN_POINT('Ctrl Pts',(-69.066006941971,1076.64792538177,483.000865940693));
#111416=CARTESIAN_POINT('Ctrl Pts',(-69.1578534910652,1076.64572415765,
483.000863197909));
#111417=CARTESIAN_POINT('Origin',(-69.1578093449747,1067.7251047501,481.522560066374));
#111418=CARTESIAN_POINT('',(-69.1578093449746,1076.65741108281,482.400863198568));
#111419=CARTESIAN_POINT('',(-69.1578093449744,1076.68648464657,480.644256934181));
#111420=CARTESIAN_POINT('Ctrl Pts',(-69.1578093449746,1076.65741108281,
482.400863198568));
#111421=CARTESIAN_POINT('Ctrl Pts',(-69.2234418991496,1076.6559402335,482.400863198568));
#111422=CARTESIAN_POINT('Ctrl Pts',(-69.2890259697938,1076.65458596451,
482.393506311697));
#111423=CARTESIAN_POINT('Ctrl Pts',(-69.4656324118671,1076.65129261893,
482.353182614794));
#111424=CARTESIAN_POINT('Ctrl Pts',(-69.571819936465,1076.6497153178,482.305686807597));
#111425=CARTESIAN_POINT('Ctrl Pts',(-69.7596569569364,1076.64787071332,
482.172506146584));
#111426=CARTESIAN_POINT('Ctrl Pts',(-69.8395218595992,1076.64762051612,
482.088174007604));
#111427=CARTESIAN_POINT('Ctrl Pts',(-69.9620961476268,1076.64850686382,
481.893680683398));
#111428=CARTESIAN_POINT('Ctrl Pts',(-70.0036798545837,1076.64963192794,
481.785444498049));
#111429=CARTESIAN_POINT('Ctrl Pts',(-70.0428234626304,1076.65304808726,
481.55918185984));
#111430=CARTESIAN_POINT('Ctrl Pts',(-70.0400292849277,1076.65530344979,
481.443343021985));
#111431=CARTESIAN_POINT('Ctrl Pts',(-69.9900378964925,1076.66053930322,
481.219243524958));
#111432=CARTESIAN_POINT('Ctrl Pts',(-69.9432918137948,1076.66346733952,
481.113145343748));
#111433=CARTESIAN_POINT('Ctrl Pts',(-69.8445544662576,1076.66800051871,
480.972021712607));
#111434=CARTESIAN_POINT('Ctrl Pts',(-69.8071161421933,1076.66952437174,
480.928327771717));
#111435=CARTESIAN_POINT('Ctrl Pts',(-69.7242446613695,1076.67254902727,
480.848866227006));
#111436=CARTESIAN_POINT('Ctrl Pts',(-69.6790090045838,1076.67404255437,
480.813290409741));
#111437=CARTESIAN_POINT('Ctrl Pts',(-69.5320560412162,1076.67845657641,
480.719418444827));
#111438=CARTESIAN_POINT('Ctrl Pts',(-69.4218891224324,1076.68120355579,
480.676769441779));
#111439=CARTESIAN_POINT('Ctrl Pts',(-69.2574551311642,1076.68463859819,
480.648503983826));
#111440=CARTESIAN_POINT('Ctrl Pts',(-69.2076810999441,1076.68559798675,
480.644256934181));
#111441=CARTESIAN_POINT('Ctrl Pts',(-69.157809344974,1076.68648464657,480.644256934181));
#111442=CARTESIAN_POINT('',(-69.1578093449747,1082.7251047501,480.644256934181));
#111443=CARTESIAN_POINT('',(-69.1578093449747,1067.7251047501,480.644256934181));
#111444=CARTESIAN_POINT('Origin',(-69.1578093449747,1082.7251047501,481.522560066374));
#111445=CARTESIAN_POINT('Ctrl Pts',(-69.1578034448267,1076.68648475146,
480.644256934201));
#111446=CARTESIAN_POINT('Ctrl Pts',(-69.0413256637295,1076.68855557259,
480.64425771666));
#111447=CARTESIAN_POINT('Ctrl Pts',(-68.9259972394792,1076.69020053972,
480.667428872737));
#111448=CARTESIAN_POINT('Ctrl Pts',(-68.7109178618377,1076.6925746641,480.757497738844));
#111449=CARTESIAN_POINT('Ctrl Pts',(-68.613337610142,1076.69328117763,480.823572092937));
#111450=CARTESIAN_POINT('Ctrl Pts',(-68.4496593311885,1076.69371963535,
480.990043135918));
#111451=CARTESIAN_POINT('Ctrl Pts',(-68.3852149705645,1076.69344715755,
481.088799595298));
#111452=CARTESIAN_POINT('Ctrl Pts',(-68.2987971436756,1076.6919231308,481.305532099511));
#111453=CARTESIAN_POINT('Ctrl Pts',(-68.2776098766221,1076.69068659907,
481.421318711384));
#111454=CARTESIAN_POINT('Ctrl Pts',(-68.2816683989113,1076.68729786405,
481.654361485375));
#111455=CARTESIAN_POINT('Ctrl Pts',(-68.3068627986114,1076.6851765445,481.769301587661));
#111456=CARTESIAN_POINT('Ctrl Pts',(-68.4008529499654,1076.68019194474,
481.983147336794));
#111457=CARTESIAN_POINT('Ctrl Pts',(-68.4689181916272,1076.67737269356,
482.079830109188));
#111458=CARTESIAN_POINT('Ctrl Pts',(-68.5960343334076,1076.67287855751,
482.200194577173));
#111459=CARTESIAN_POINT('Ctrl Pts',(-68.641990916816,1076.67135580326,482.235799792611));
#111460=CARTESIAN_POINT('Ctrl Pts',(-68.7887122087969,1076.66677549102,
482.327827110654));
#111461=CARTESIAN_POINT('Ctrl Pts',(-68.8974035657164,1076.66372781536,
482.369246363832));
#111462=CARTESIAN_POINT('Ctrl Pts',(-69.0596088337739,1076.65967636945,
482.396748218617));
#111463=CARTESIAN_POINT('Ctrl Pts',(-69.1087226494482,1076.65851113343,
482.400863198568));
#111464=CARTESIAN_POINT('Ctrl Pts',(-69.1578093449746,1076.65741108281,
482.400863198568));
#111465=CARTESIAN_POINT('Origin',(-81.035688248506,1067.7251047501,477.445052325154));
#111466=CARTESIAN_POINT('',(-81.035688248534,1076.38861150411,476.169608204017));
#111467=CARTESIAN_POINT('',(-81.035688248506,1067.7251047501,476.169608204017));
#111468=CARTESIAN_POINT('Ctrl Pts',(-81.0350577987155,1076.29855081768,
478.720496290475));
#111469=CARTESIAN_POINT('Ctrl Pts',(-81.2025872754575,1076.28904104832,
478.720579100011));
#111470=CARTESIAN_POINT('Ctrl Pts',(-81.3685713429343,1076.28071251082,
478.687653651935));
#111471=CARTESIAN_POINT('Ctrl Pts',(-81.6779649861134,1076.26760505678,
478.55958789631));
#111472=CARTESIAN_POINT('Ctrl Pts',(-81.8184203241435,1076.26294804639,
478.46587303349));
#111473=CARTESIAN_POINT('Ctrl Pts',(-82.0547972518833,1076.25810168175,
478.229889358828));
#111474=CARTESIAN_POINT('Ctrl Pts',(-82.1485512834177,1076.25794630665,
478.090102318924));
#111475=CARTESIAN_POINT('Ctrl Pts',(-82.2768528229317,1076.26218228058,
477.782644138906));
#111476=CARTESIAN_POINT('Ctrl Pts',(-82.3102484857368,1076.26652278209,
477.618028368156));
#111477=CARTESIAN_POINT('Ctrl Pts',(-82.3119826647834,1076.2790267047,477.285168278088));
#111478=CARTESIAN_POINT('Ctrl Pts',(-82.2802282147205,1076.28706960511,
477.120143535699));
#111479=CARTESIAN_POINT('Ctrl Pts',(-82.1550323352381,1076.30563793529,
476.811272820305));
#111480=CARTESIAN_POINT('Ctrl Pts',(-82.0626112673567,1076.31598830964,
476.670449657923));
#111481=CARTESIAN_POINT('Ctrl Pts',(-81.8872474634401,1076.33209795959,
476.491859992467));
#111482=CARTESIAN_POINT('Ctrl Pts',(-81.8230420025745,1076.33753081149,
476.438174772569));
#111483=CARTESIAN_POINT('Ctrl Pts',(-81.6850684766686,1076.34835045727,
476.344128585188));
#111484=CARTESIAN_POINT('Ctrl Pts',(-81.6116280997105,1076.35371156829,
476.303990155284));
#111485=CARTESIAN_POINT('Ctrl Pts',(-81.3790489997821,1076.36956256003,
476.205092004347));
#111486=CARTESIAN_POINT('Ctrl Pts',(-81.2116281892164,1076.37950643801,
476.170502300506));
#111487=CARTESIAN_POINT('Ctrl Pts',(-80.8737184860208,1076.3969948398,476.168752249334));
#111488=CARTESIAN_POINT('Ctrl Pts',(-80.7065692166189,1076.4043825128,476.201308734276));
#111489=CARTESIAN_POINT('Ctrl Pts',(-80.394267683289,1076.41585345873,476.329752933126));
#111490=CARTESIAN_POINT('Ctrl Pts',(-80.252268303724,1076.41982178174,476.42446734997));
#111491=CARTESIAN_POINT('Ctrl Pts',(-80.0132049540281,1076.42391724823,
476.664042335541));
#111492=CARTESIAN_POINT('Ctrl Pts',(-79.9186337580982,1076.42399815458,
476.806586549861));
#111493=CARTESIAN_POINT('Ctrl Pts',(-79.7908232378988,1076.42021996792,
477.119999971423));
#111494=CARTESIAN_POINT('Ctrl Pts',(-79.7587569641805,1076.4164036502,477.287674129747));
#111495=CARTESIAN_POINT('Ctrl Pts',(-79.7618344059718,1076.4052118501,477.62536860419));
#111496=CARTESIAN_POINT('Ctrl Pts',(-79.7968236670402,1076.39794918094,
477.792026290804));
#111497=CARTESIAN_POINT('Ctrl Pts',(-79.9297897299973,1076.38066932286,
478.102626681248));
#111498=CARTESIAN_POINT('Ctrl Pts',(-80.0267102412019,1076.37080744361,
478.243390457155));
#111499=CARTESIAN_POINT('Ctrl Pts',(-80.2709610251275,1076.34957324633,
478.48001817901));
#111500=CARTESIAN_POINT('Ctrl Pts',(-80.4163480458686,1076.33839736225,
478.573047215329));
#111501=CARTESIAN_POINT('Ctrl Pts',(-80.7222066175661,1076.31726838241,
478.69130787995));
#111502=CARTESIAN_POINT('Ctrl Pts',(-80.8779342293022,1076.30746989828,
478.720418624561));
#111503=CARTESIAN_POINT('Ctrl Pts',(-81.0350577987155,1076.29855081768,
478.720496290475));
#111504=CARTESIAN_POINT('Origin',(-81.035688248506,1067.7251047501,477.445052325154));
#111505=CARTESIAN_POINT('',(-81.035688248506,1076.32087957987,478.12049644629));
#111506=CARTESIAN_POINT('',(-81.0356882485063,1076.36858155369,476.769608204017));
#111507=CARTESIAN_POINT('Ctrl Pts',(-81.0356882485058,1076.32087957987,
478.12049644629));
#111508=CARTESIAN_POINT('Ctrl Pts',(-81.0876899683255,1076.31799162062,
478.12049644629));
#111509=CARTESIAN_POINT('Ctrl Pts',(-81.1396509250425,1076.31531083151,
478.114491043542));
#111510=CARTESIAN_POINT('Ctrl Pts',(-81.2767049632162,1076.30881714018,
478.082213763299));
#111511=CARTESIAN_POINT('Ctrl Pts',(-81.3580914012869,1076.30558998787,
478.045161876903));
#111512=CARTESIAN_POINT('Ctrl Pts',(-81.5017615346713,1076.30127879455,
477.941849337013));
#111513=CARTESIAN_POINT('Ctrl Pts',(-81.5626924302093,1076.30023185449,
477.876680169358));
#111514=CARTESIAN_POINT('Ctrl Pts',(-81.6559233030925,1076.30048940395,
477.726685444176));
#111515=CARTESIAN_POINT('Ctrl Pts',(-81.687359818685,1076.30178720242,477.643363879025));
#111516=CARTESIAN_POINT('Ctrl Pts',(-81.7164386739801,1076.30654910395,
477.469340570339));
#111517=CARTESIAN_POINT('Ctrl Pts',(-81.7137814951616,1076.30996693042,
477.380330855999));
#111518=CARTESIAN_POINT('Ctrl Pts',(-81.6743968578101,1076.3184404379,477.208224530291));
#111519=CARTESIAN_POINT('Ctrl Pts',(-81.6379696361283,1076.32341688763,
477.126803176128));
#111520=CARTESIAN_POINT('Ctrl Pts',(-81.5357678564573,1076.33423131285,
476.982469018654));
#111521=CARTESIAN_POINT('Ctrl Pts',(-81.4709012897918,1076.33996689521,
476.920982383539));
#111522=CARTESIAN_POINT('Ctrl Pts',(-81.3197704532662,1076.35151253806,
476.82565555341));
#111523=CARTESIAN_POINT('Ctrl Pts',(-81.2346252268159,1076.35720761268,
476.793296719234));
#111524=CARTESIAN_POINT('Ctrl Pts',(-81.1093088234223,1076.36458502301,
476.77262422383));
#111525=CARTESIAN_POINT('Ctrl Pts',(-81.0725580361971,1076.36663518759,
476.769611028284));
#111526=CARTESIAN_POINT('Ctrl Pts',(-81.0357400173349,1076.36857882086,
476.76960820633));
#111527=CARTESIAN_POINT('Ctrl Pts',(-81.0357227610269,1076.36857973182,
476.769608205008));
#111528=CARTESIAN_POINT('Ctrl Pts',(-81.0357055047511,1076.36858064277,
476.769608204017));
#111529=CARTESIAN_POINT('Ctrl Pts',(-81.0356882485066,1076.36858155369,
476.769608204017));
#111530=CARTESIAN_POINT('',(-81.035688248506,1082.7251047501,476.769608204017));
#111531=CARTESIAN_POINT('',(-81.035688248506,1067.7251047501,476.769608204017));
#111532=CARTESIAN_POINT('Origin',(-81.035688248506,1082.7251047501,477.445052325154));
#111533=CARTESIAN_POINT('Ctrl Pts',(-81.0356882485066,1076.36858155369,
476.769608204017));
#111534=CARTESIAN_POINT('Ctrl Pts',(-80.9459376043467,1076.37331926323,
476.769608204017));
#111535=CARTESIAN_POINT('Ctrl Pts',(-80.8570465935824,1076.37735746331,
476.787496825715));
#111536=CARTESIAN_POINT('Ctrl Pts',(-80.6913756260759,1076.3836223215,476.857048565197));
#111537=CARTESIAN_POINT('Ctrl Pts',(-80.6162677526475,1076.38578648672,
476.908028783951));
#111538=CARTESIAN_POINT('Ctrl Pts',(-80.490354059149,1076.38796575458,477.036482166989));
#111539=CARTESIAN_POINT('Ctrl Pts',(-80.4408421981638,1076.38795784533,
477.112671384822));
#111540=CARTESIAN_POINT('Ctrl Pts',(-80.3746031318373,1076.38574772309,
477.2799034164));
#111541=CARTESIAN_POINT('Ctrl Pts',(-80.3585233940397,1076.38356883935,
477.369242298903));
#111542=CARTESIAN_POINT('Ctrl Pts',(-80.3622558168713,1076.37727679008,
477.548898300214));
#111543=CARTESIAN_POINT('Ctrl Pts',(-80.382020323534,1076.37322599853,477.63740972814));
#111544=CARTESIAN_POINT('Ctrl Pts',(-80.4550618199596,1076.36371555603,
477.801709096096));
#111545=CARTESIAN_POINT('Ctrl Pts',(-80.507708273909,1076.35834542562,477.875817963691));
#111546=CARTESIAN_POINT('Ctrl Pts',(-80.605452720709,1076.34987842304,477.967610853476));
#111547=CARTESIAN_POINT('Ctrl Pts',(-80.6404817164721,1076.34703887773,
477.994580700113));
#111548=CARTESIAN_POINT('Ctrl Pts',(-80.7539130304431,1076.33838431086,
478.065424897086));
#111549=CARTESIAN_POINT('Ctrl Pts',(-80.8386464989045,1076.33260746561,
478.097308551931));
#111550=CARTESIAN_POINT('Ctrl Pts',(-80.9631062455084,1076.32501022693,
478.117573261705));
#111551=CARTESIAN_POINT('Ctrl Pts',(-80.9994071681082,1076.32289448018,
478.12049644629));
#111552=CARTESIAN_POINT('Ctrl Pts',(-81.0356882485058,1076.32087957987,
478.12049644629));
#111553=CARTESIAN_POINT('Origin',(-93.6720377362213,1067.7251047501,471.775755329037));
#111554=CARTESIAN_POINT('',(-93.6720377362212,1075.70592960701,470.676924193044));
#111555=CARTESIAN_POINT('',(-93.6720377362213,1067.7251047501,470.676924193044));
#111556=CARTESIAN_POINT('Ctrl Pts',(-93.6724912621575,1075.60299418635,
472.874586371436));
#111557=CARTESIAN_POINT('Ctrl Pts',(-93.8169302540145,1075.58933558814,
472.874526756422));
#111558=CARTESIAN_POINT('Ctrl Pts',(-93.9600910334365,1075.57706485313,
472.845988318381));
#111559=CARTESIAN_POINT('Ctrl Pts',(-94.2265607311415,1075.55691151587,
472.735247792837));
#111560=CARTESIAN_POINT('Ctrl Pts',(-94.3473884187733,1075.54920204289,
472.654445900629));
#111561=CARTESIAN_POINT('Ctrl Pts',(-94.5505303134195,1075.53949431675,
472.451185501296));
#111562=CARTESIAN_POINT('Ctrl Pts',(-94.6310424305107,1075.53756147911,
472.330990881764));
#111563=CARTESIAN_POINT('Ctrl Pts',(-94.7412746804731,1075.53976384039,
472.066661254209));
#111564=CARTESIAN_POINT('Ctrl Pts',(-94.7699955975805,1075.54386435273,
471.925217352867));
#111565=CARTESIAN_POINT('Ctrl Pts',(-94.7717056673004,1075.55754939313,
471.638964047272));
#111566=CARTESIAN_POINT('Ctrl Pts',(-94.7445019646648,1075.56701403193,
471.496970713478));
#111567=CARTESIAN_POINT('Ctrl Pts',(-94.637016943371,1075.59002791232,471.230801805686));
#111568=CARTESIAN_POINT('Ctrl Pts',(-94.5574400275378,1075.60337795513,
471.109307337067));
#111569=CARTESIAN_POINT('Ctrl Pts',(-94.4063394473801,1075.62491014947,
470.955124244313));
#111570=CARTESIAN_POINT('Ctrl Pts',(-94.3509033093937,1075.63230386669,
470.908707578224));
#111571=CARTESIAN_POINT('Ctrl Pts',(-94.2319879551823,1075.64723723404,
470.827574452807));
#111572=CARTESIAN_POINT('Ctrl Pts',(-94.1688138660993,1075.65474178336,
470.79300164833));
#111573=CARTESIAN_POINT('Ctrl Pts',(-93.9685431431715,1075.67730907353,
470.707679880593));
#111574=CARTESIAN_POINT('Ctrl Pts',(-93.824244517943,1075.69197607329,470.677765702776));
#111575=CARTESIAN_POINT('Ctrl Pts',(-93.5328349810482,1075.71869264892,
470.676121075161));
#111576=CARTESIAN_POINT('Ctrl Pts',(-93.3885638460807,1075.73049592361,
470.704169315622));
#111577=CARTESIAN_POINT('Ctrl Pts',(-93.118898028987,1075.74979914152,470.815151093479));
#111578=CARTESIAN_POINT('Ctrl Pts',(-92.9962482006577,1075.75710075947,
470.897062055314));
#111579=CARTESIAN_POINT('Ctrl Pts',(-92.7921704384465,1075.76613296183,
471.102140540071));
#111580=CARTESIAN_POINT('Ctrl Pts',(-92.7119651934467,1075.76788731263,
471.222399927589));
#111581=CARTESIAN_POINT('Ctrl Pts',(-92.602133018938,1075.76579171759,471.487141717504));
#111582=CARTESIAN_POINT('Ctrl Pts',(-92.5736649139426,1075.76195513217,
471.629015406361));
#111583=CARTESIAN_POINT('Ctrl Pts',(-92.5727508400567,1075.7489670063,471.91821427215));
#111584=CARTESIAN_POINT('Ctrl Pts',(-92.6013627896465,1075.73984827547,
472.062639524665));
#111585=CARTESIAN_POINT('Ctrl Pts',(-92.7130987407103,1075.7174364238,472.33171554884));
#111586=CARTESIAN_POINT('Ctrl Pts',(-92.7951223488863,1075.70436191303,
472.453694586321));
#111587=CARTESIAN_POINT('Ctrl Pts',(-92.9490408166069,1075.68315553206,
472.606290889229));
#111588=CARTESIAN_POINT('Ctrl Pts',(-93.0044293445341,1075.67595097932,
472.65143098531));
#111589=CARTESIAN_POINT('Ctrl Pts',(-93.1233387940823,1075.66125814001,
472.730466514943));
#111590=CARTESIAN_POINT('Ctrl Pts',(-93.1866147717712,1075.65380259906,
472.764141522232));
#111591=CARTESIAN_POINT('Ctrl Pts',(-93.385771493417,1075.63136578552,472.846365209264));
#111592=CARTESIAN_POINT('Ctrl Pts',(-93.5284035649352,1075.61661956506,
472.87464584146));
#111593=CARTESIAN_POINT('Ctrl Pts',(-93.6724912621575,1075.60299418635,
472.874586371436));
#111594=CARTESIAN_POINT('Origin',(-93.6720377362213,1067.7251047501,471.775755329037));
#111595=CARTESIAN_POINT('',(-93.6720377362213,1075.63195590694,472.274586465029));
#111596=CARTESIAN_POINT('',(-93.6720377362213,1075.67866049267,471.276924193045));
#111597=CARTESIAN_POINT('Ctrl Pts',(-93.6720377362214,1075.63195590694,
472.274586465029));
#111598=CARTESIAN_POINT('Ctrl Pts',(-93.6737691348478,1075.63179365252,
472.274586465029));
#111599=CARTESIAN_POINT('Ctrl Pts',(-93.675500986709,1075.63163176809,472.274577450741));
#111600=CARTESIAN_POINT('Ctrl Pts',(-93.743328560288,1075.6253077827,472.273870966368));
#111601=CARTESIAN_POINT('Ctrl Pts',(-93.8086976309984,1075.61981426241,
472.260051449589));
#111602=CARTESIAN_POINT('Ctrl Pts',(-93.9294189604092,1075.61090887706,
472.208008495179));
#111603=CARTESIAN_POINT('Ctrl Pts',(-93.9837309733091,1075.60755437524,
472.170660119206));
#111604=CARTESIAN_POINT('Ctrl Pts',(-94.0747040602113,1075.60339910519,
472.077284693635));
#111605=CARTESIAN_POINT('Ctrl Pts',(-94.110547226867,1075.60262743349,472.022277883647));
#111606=CARTESIAN_POINT('Ctrl Pts',(-94.1590787287541,1075.60378121623,
471.901638891653));
#111607=CARTESIAN_POINT('Ctrl Pts',(-94.1713055789272,1075.60569234708,
471.837222228766));
#111608=CARTESIAN_POINT('Ctrl Pts',(-94.1704066890215,1075.61195888507,
471.707154680144));
#111609=CARTESIAN_POINT('Ctrl Pts',(-94.1571976209969,1075.6162607745,471.642785171551));
#111610=CARTESIAN_POINT('Ctrl Pts',(-94.1067412339385,1075.62669969183,
471.522485245883));
#111611=CARTESIAN_POINT('Ctrl Pts',(-94.0698363103155,1075.63274628175,
471.467769964241));
#111612=CARTESIAN_POINT('Ctrl Pts',(-94.0003209811604,1075.64249340348,
471.398756760698));
#111613=CARTESIAN_POINT('Ctrl Pts',(-93.9749618585148,1075.64583148274,
471.378094761762));
#111614=CARTESIAN_POINT('Ctrl Pts',(-93.9206384928281,1075.65258399093,
471.342061386539));
#111615=CARTESIAN_POINT('Ctrl Pts',(-93.8918063336955,1075.65598272677,
471.326762543099));
#111616=CARTESIAN_POINT('Ctrl Pts',(-93.8015629462923,1075.66609816722,
471.289667018385));
#111617=CARTESIAN_POINT('Ctrl Pts',(-93.7371481923161,1075.67265257079,
471.276928469069));
#111618=CARTESIAN_POINT('Ctrl Pts',(-93.6720705043938,1075.67865746911,
471.276924194121));
#111619=CARTESIAN_POINT('Ctrl Pts',(-93.6720595816534,1075.67865847699,
471.276924193404));
#111620=CARTESIAN_POINT('Ctrl Pts',(-93.6720486589293,1075.67865948484,
471.276924193045));
#111621=CARTESIAN_POINT('Ctrl Pts',(-93.6720377362213,1075.67866049267,
471.276924193045));
#111622=CARTESIAN_POINT('',(-93.6720377362213,1082.7251047501,471.276924193044));
#111623=CARTESIAN_POINT('',(-93.6720377362213,1067.7251047501,471.276924193044));
#111624=CARTESIAN_POINT('Origin',(-93.6720377362213,1082.7251047501,471.775755329037));
#111625=CARTESIAN_POINT('Ctrl Pts',(-93.6720377362213,1075.67866049267,
471.276924193045));
#111626=CARTESIAN_POINT('Ctrl Pts',(-93.6057021697443,1075.68478125021,
471.276924193045));
#111627=CARTESIAN_POINT('Ctrl Pts',(-93.5399634596612,1075.69021285038,
471.290156336786));
#111628=CARTESIAN_POINT('Ctrl Pts',(-93.4179970438533,1075.69903597252,
471.341438225336));
#111629=CARTESIAN_POINT('Ctrl Pts',(-93.3628981850123,1075.70235892845,
471.378747617469));
#111630=CARTESIAN_POINT('Ctrl Pts',(-93.2710109458655,1075.7064665635,471.472052912521));
#111631=CARTESIAN_POINT('Ctrl Pts',(-93.2348802972019,1075.70724676277,
471.526848205431));
#111632=CARTESIAN_POINT('Ctrl Pts',(-93.1856677095831,1075.70620435935,
471.647267394553));
#111633=CARTESIAN_POINT('Ctrl Pts',(-93.1730860586743,1075.70439100265,
471.711694413156));
#111634=CARTESIAN_POINT('Ctrl Pts',(-93.1733293925817,1075.69836557453,
471.841952972592));
#111635=CARTESIAN_POINT('Ctrl Pts',(-93.1862574974906,1075.69420280903,
471.906498430089));
#111636=CARTESIAN_POINT('Ctrl Pts',(-93.2366226107059,1075.68394572461,
472.0280667968));
#111637=CARTESIAN_POINT('Ctrl Pts',(-93.2740394554466,1075.67791644558,
472.0836995133));
#111638=CARTESIAN_POINT('Ctrl Pts',(-93.3442711117432,1075.66818445032,
472.153188397825));
#111639=CARTESIAN_POINT('Ctrl Pts',(-93.3695203473757,1075.66488807269,
472.173711286108));
#111640=CARTESIAN_POINT('Ctrl Pts',(-93.4236710698175,1075.6581869491,472.209578650767));
#111641=CARTESIAN_POINT('Ctrl Pts',(-93.452453444199,1075.65479742239,472.224833554217));
#111642=CARTESIAN_POINT('Ctrl Pts',(-93.5426317880684,1075.64466393579,
472.261873245006));
#111643=CARTESIAN_POINT('Ctrl Pts',(-93.6070151801627,1075.63804936053,
472.274586465029));
#111644=CARTESIAN_POINT('Ctrl Pts',(-93.6720377362214,1075.63195590694,
472.274586465029));
#111645=CARTESIAN_POINT('Origin',(-104.994450521158,1067.7251047501,463.563756561532));
#111646=CARTESIAN_POINT('',(-104.994450521158,1074.8526378468,462.473215812804));
#111647=CARTESIAN_POINT('',(-104.994450521158,1067.7251047501,462.473215812804));
#111648=CARTESIAN_POINT('Ctrl Pts',(-104.993489577313,1074.75006270401,
464.654296886886));
#111649=CARTESIAN_POINT('Ctrl Pts',(-105.137367767514,1074.73163951737,
464.654423667032));
#111650=CARTESIAN_POINT('Ctrl Pts',(-105.280072879011,1074.71463613285,
464.626075909733));
#111651=CARTESIAN_POINT('Ctrl Pts',(-105.545324057093,1074.68569695547,
464.515734326609));
#111652=CARTESIAN_POINT('Ctrl Pts',(-105.665476382385,1074.67399870599,
464.435296075217));
#111653=CARTESIAN_POINT('Ctrl Pts',(-105.867001838481,1074.65758776391,
464.233154467582));
#111654=CARTESIAN_POINT('Ctrl Pts',(-105.946730719867,1074.6529721013,464.113906624031));
#111655=CARTESIAN_POINT('Ctrl Pts',(-106.055683810394,1074.65143823157,
463.851986175433));
#111656=CARTESIAN_POINT('Ctrl Pts',(-106.084056288577,1074.65449593288,
463.712112038072));
#111657=CARTESIAN_POINT('Ctrl Pts',(-106.085883608058,1074.66788353223,
463.429046701911));
#111658=CARTESIAN_POINT('Ctrl Pts',(-106.059155506872,1074.67809875985,
463.288701813979));
#111659=CARTESIAN_POINT('Ctrl Pts',(-105.953374507423,1074.70439182409,
463.025150401418));
#111660=CARTESIAN_POINT('Ctrl Pts',(-105.874863628056,1074.72026544387,
462.904684537913));
#111661=CARTESIAN_POINT('Ctrl Pts',(-105.675433656561,1074.75558205367,
462.699949665295));
#111662=CARTESIAN_POINT('Ctrl Pts',(-105.555975816372,1074.77472591118,
462.617960354975));
#111663=CARTESIAN_POINT('Ctrl Pts',(-105.358517822884,1074.8038144677,462.533300937462));
#111664=CARTESIAN_POINT('Ctrl Pts',(-105.290235479964,1074.81349026178,
462.511664545201));
#111665=CARTESIAN_POINT('Ctrl Pts',(-105.078437171931,1074.84238669272,
462.466825187557));
#111666=CARTESIAN_POINT('Ctrl Pts',(-104.931817723056,1074.86090661222,
462.465356096695));
#111667=CARTESIAN_POINT('Ctrl Pts',(-104.647237696593,1074.8940390347,462.519928292812));
#111668=CARTESIAN_POINT('Ctrl Pts',(-104.511978138741,1074.90835773384,
462.57507423291));
#111669=CARTESIAN_POINT('Ctrl Pts',(-104.270797373955,1074.93097649917,
462.735194331009));
#111670=CARTESIAN_POINT('Ctrl Pts',(-104.167278755511,1074.93905994392,
462.838443218777));
#111671=CARTESIAN_POINT('Ctrl Pts',(-104.008363161499,1074.94778814809,
463.076956530643));
#111672=CARTESIAN_POINT('Ctrl Pts',(-103.953527163956,1074.94851122642,
463.209030175445));
#111673=CARTESIAN_POINT('Ctrl Pts',(-103.897397084343,1074.94269359972,
463.487006669484));
#111674=CARTESIAN_POINT('Ctrl Pts',(-103.89675656806,1074.93619993154,463.630106351421));
#111675=CARTESIAN_POINT('Ctrl Pts',(-103.950724284045,1074.91652422059,
463.911467977091));
#111676=CARTESIAN_POINT('Ctrl Pts',(-104.006041448505,1074.90339307649,
464.046641489684));
#111677=CARTESIAN_POINT('Ctrl Pts',(-104.166220633862,1074.87215504748,
464.287909340975));
#111678=CARTESIAN_POINT('Ctrl Pts',(-104.269769523854,1074.85432750344,
464.391457913392));
#111679=CARTESIAN_POINT('Ctrl Pts',(-104.449555246214,1074.82602986511,
464.511082923885));
#111680=CARTESIAN_POINT('Ctrl Pts',(-104.512467851101,1074.81649698506,
464.54458547443));
#111681=CARTESIAN_POINT('Ctrl Pts',(-104.643520285306,1074.79732832783,
464.598708574211));
#111682=CARTESIAN_POINT('Ctrl Pts',(-104.711341338543,1074.78773558188,
464.619279248892));
#111683=CARTESIAN_POINT('Ctrl Pts',(-104.850723767376,1074.76865710029,
464.647142030681));
#111684=CARTESIAN_POINT('Ctrl Pts',(-104.922002764286,1074.75921638392,
464.654233895348));
#111685=CARTESIAN_POINT('Ctrl Pts',(-104.993489577313,1074.75006270401,
464.654296886886));
#111686=CARTESIAN_POINT('Origin',(-104.994450521158,1067.7251047501,463.563756561532));
#111687=CARTESIAN_POINT('',(-104.994450521158,1074.77893852154,464.05429731026));
#111688=CARTESIAN_POINT('',(-104.994450521158,1074.82513013623,463.073215812804));
#111689=CARTESIAN_POINT('Ctrl Pts',(-104.994450521158,1074.77893852154,
464.05429731026));
#111690=CARTESIAN_POINT('Ctrl Pts',(-105.030095890685,1074.77439673021,
464.05429731026));
#111691=CARTESIAN_POINT('Ctrl Pts',(-105.065745517352,1074.77003297191,
464.050412186953));
#111692=CARTESIAN_POINT('Ctrl Pts',(-105.163681512993,1074.75855790272,
464.028670857344));
#111693=CARTESIAN_POINT('Ctrl Pts',(-105.223343682509,1074.75217048114,
464.002413949173));
#111694=CARTESIAN_POINT('Ctrl Pts',(-105.328667510103,1074.74219393818,
463.928484696109));
#111695=CARTESIAN_POINT('Ctrl Pts',(-105.373423586705,1074.73867624248,
463.881761777249));
#111696=CARTESIAN_POINT('Ctrl Pts',(-105.442219218817,1074.73497992791,
463.773974006962));
#111697=CARTESIAN_POINT('Ctrl Pts',(-105.465707864338,1074.73481509992,
463.714108546454));
#111698=CARTESIAN_POINT('Ctrl Pts',(-105.488479889226,1074.73785905108,
463.588739883212));
#111699=CARTESIAN_POINT('Ctrl Pts',(-105.487533259021,1074.74103652407,
463.524511433594));
#111700=CARTESIAN_POINT('Ctrl Pts',(-105.461148520179,1074.7503474454,463.399674225694));
#111701=CARTESIAN_POINT('Ctrl Pts',(-105.435795894582,1074.75640913827,
463.340335266017));
#111702=CARTESIAN_POINT('Ctrl Pts',(-105.363573412933,1074.77065743129,
463.234310312591));
#111703=CARTESIAN_POINT('Ctrl Pts',(-105.317177481959,1074.77872845181,
463.188771704626));
#111704=CARTESIAN_POINT('Ctrl Pts',(-105.236483829072,1074.79149302069,
463.135871837016));
#111705=CARTESIAN_POINT('Ctrl Pts',(-105.207910629415,1074.79582979228,
463.120925430747));
#111706=CARTESIAN_POINT('Ctrl Pts',(-105.149116860948,1074.80441314705,
463.097189721489));
#111707=CARTESIAN_POINT('Ctrl Pts',(-105.119091577843,1074.80864054609,
463.088286888806));
#111708=CARTESIAN_POINT('Ctrl Pts',(-105.057488876431,1074.81701159186,
463.076263403711));
#111709=CARTESIAN_POINT('Ctrl Pts',(-105.026034191749,1074.8211360572,463.073218466764));
#111710=CARTESIAN_POINT('Ctrl Pts',(-104.994491767958,1074.82512492024,
463.073215814539));
#111711=CARTESIAN_POINT('Ctrl Pts',(-104.994478019,1074.82512665893,463.073215813383));
#111712=CARTESIAN_POINT('Ctrl Pts',(-104.994464270067,1074.8251283976,463.073215812804));
#111713=CARTESIAN_POINT('Ctrl Pts',(-104.994450521158,1074.82513013623,
463.073215812804));
#111714=CARTESIAN_POINT('',(-104.994450521158,1082.7251047501,463.073215812804));
#111715=CARTESIAN_POINT('',(-104.994450521158,1067.7251047501,463.073215812804));
#111716=CARTESIAN_POINT('Origin',(-104.994450521158,1082.7251047501,463.563756561532));
#111717=CARTESIAN_POINT('Ctrl Pts',(-104.994450521158,1074.82513013623,
463.073215812804));
#111718=CARTESIAN_POINT('Ctrl Pts',(-104.929134780518,1074.83338971686,
463.073215812804));
#111719=CARTESIAN_POINT('Ctrl Pts',(-104.864372632066,1074.84095001567,
463.08626102952));
#111720=CARTESIAN_POINT('Ctrl Pts',(-104.743862011825,1074.85376020283,
463.137031952008));
#111721=CARTESIAN_POINT('Ctrl Pts',(-104.689285712492,1074.85889120532,
463.174154416784));
#111722=CARTESIAN_POINT('Ctrl Pts',(-104.598966777381,1074.86593142847,
463.266616183336));
#111723=CARTESIAN_POINT('Ctrl Pts',(-104.563685271589,1074.86784902223,
463.320543505307));
#111724=CARTESIAN_POINT('Ctrl Pts',(-104.515827292603,1074.86834965407,
463.438820828996));
#111725=CARTESIAN_POINT('Ctrl Pts',(-104.50367647131,1074.86693664149,463.501938919774));
#111726=CARTESIAN_POINT('Ctrl Pts',(-104.504150930195,1074.86093236406,
463.6295110763));
#111727=CARTESIAN_POINT('Ctrl Pts',(-104.516881728838,1074.85638733246,
463.692681254243));
#111728=CARTESIAN_POINT('Ctrl Pts',(-104.5663688629,1074.84457922523,463.812086803098));
#111729=CARTESIAN_POINT('Ctrl Pts',(-104.603275539818,1074.83736414877,
463.866868200142));
#111730=CARTESIAN_POINT('Ctrl Pts',(-104.696435940095,1074.82127878478,
463.958884685947));
#111731=CARTESIAN_POINT('Ctrl Pts',(-104.751884373655,1074.81255586224,
463.995135213247));
#111732=CARTESIAN_POINT('Ctrl Pts',(-104.842594637019,1074.79934181929,
464.0313047854));
#111733=CARTESIAN_POINT('Ctrl Pts',(-104.873524270356,1074.79499132664,
464.040242492033));
#111734=CARTESIAN_POINT('Ctrl Pts',(-104.934634235345,1074.78668581557,
464.05156178044));
#111735=CARTESIAN_POINT('Ctrl Pts',(-104.964540878907,1074.7827494893,464.05429731026));
#111736=CARTESIAN_POINT('Ctrl Pts',(-104.994450521158,1074.77893852154,
464.05429731026));
#111737=CARTESIAN_POINT('Origin',(-55.8158882427217,1067.7251047501,494.657824979653));
#111738=CARTESIAN_POINT('',(-55.8158882427496,1076.69910051006,493.17952184746));
#111739=CARTESIAN_POINT('',(-55.8158882427217,1067.7251047501,493.17952184746));
#111740=CARTESIAN_POINT('Ctrl Pts',(-57.2940029153359,1076.64571253121,
494.681429327873));
#111741=CARTESIAN_POINT('Ctrl Pts',(-57.2970861273448,1076.65033938597,
494.488357235108));
#111742=CARTESIAN_POINT('Ctrl Pts',(-57.2623109437452,1076.65549195305,
494.296546507661));
#111743=CARTESIAN_POINT('Ctrl Pts',(-57.1563128506684,1076.66335905769,
494.026976710274));
#111744=CARTESIAN_POINT('Ctrl Pts',(-57.1122476020844,1076.66598700711,
493.940775273864));
#111745=CARTESIAN_POINT('Ctrl Pts',(-57.0079236857122,1076.67115904959,
493.778186891722));
#111746=CARTESIAN_POINT('Ctrl Pts',(-56.9479117161991,1076.67369065833,
493.702191547212));
#111747=CARTESIAN_POINT('Ctrl Pts',(-56.7448274654058,1076.68108498756,
493.491224108044));
#111748=CARTESIAN_POINT('Ctrl Pts',(-56.581935758937,1076.68557793453,493.378346098784));
#111749=CARTESIAN_POINT('Ctrl Pts',(-56.2228054111147,1076.69327299039,
493.223325920551));
#111750=CARTESIAN_POINT('Ctrl Pts',(-56.0303254656401,1076.69641487917,
493.182225388176));
#111751=CARTESIAN_POINT('Ctrl Pts',(-55.640164985733,1076.70130569293,493.177071759869));
#111752=CARTESIAN_POINT('Ctrl Pts',(-55.4463199432541,1076.70301258711,
493.213202969801));
#111753=CARTESIAN_POINT('Ctrl Pts',(-55.0832621058866,1076.70505910468,
493.358965902032));
#111754=CARTESIAN_POINT('Ctrl Pts',(-54.9177371508854,1076.70537890105,
493.467404272984));
#111755=CARTESIAN_POINT('Ctrl Pts',(-54.6388244198768,1076.70464167866,
493.742300828558));
#111756=CARTESIAN_POINT('Ctrl Pts',(-54.5281179015418,1076.70359198019,
493.905955049508));
#111757=CARTESIAN_POINT('Ctrl Pts',(-54.3771381331761,1076.70004341043,
494.266188308545));
#111758=CARTESIAN_POINT('Ctrl Pts',(-54.3380906066545,1076.69757708303,
494.45910768757));
#111759=CARTESIAN_POINT('Ctrl Pts',(-54.3370881340296,1076.69117204073,
494.849428321895));
#111760=CARTESIAN_POINT('Ctrl Pts',(-54.3753325767836,1076.68728473173,
495.042989296045));
#111761=CARTESIAN_POINT('Ctrl Pts',(-54.48681820115,1076.68059650085,495.312167589186));
#111762=CARTESIAN_POINT('Ctrl Pts',(-54.5320900300352,1076.67826624934,
495.397049254801));
#111763=CARTESIAN_POINT('Ctrl Pts',(-54.6393344195377,1076.67336333136,
495.558171091746));
#111764=CARTESIAN_POINT('Ctrl Pts',(-54.7013118826123,1076.6707992158,495.633847942096));
#111765=CARTESIAN_POINT('Ctrl Pts',(-54.9074558971707,1076.6629777965,495.840102357091));
#111766=CARTESIAN_POINT('Ctrl Pts',(-55.0703097504237,1076.65763333709,
495.949003880213));
#111767=CARTESIAN_POINT('Ctrl Pts',(-55.4289045490332,1076.64748045596,
496.097730756909));
#111768=CARTESIAN_POINT('Ctrl Pts',(-55.6211913806661,1076.64277749116,
496.136063240489));
#111769=CARTESIAN_POINT('Ctrl Pts',(-56.0094935863397,1076.63499579872,
496.136192783591));
#111770=CARTESIAN_POINT('Ctrl Pts',(-56.2017324936643,1076.63199875157,
496.098029869471));
#111771=CARTESIAN_POINT('Ctrl Pts',(-56.5600799978547,1076.62840406014,
495.949751020717));
#111772=CARTESIAN_POINT('Ctrl Pts',(-56.7227652434645,1076.62783944081,
495.841239952424));
#111773=CARTESIAN_POINT('Ctrl Pts',(-56.9966772267137,1076.62928815504,
495.568012544925));
#111774=CARTESIAN_POINT('Ctrl Pts',(-57.1053849872915,1076.63127933247,
495.406085393848));
#111775=CARTESIAN_POINT('Ctrl Pts',(-57.2522748438085,1076.63730171277,
495.05460157633));
#111776=CARTESIAN_POINT('Ctrl Pts',(-57.2910052075554,1076.64121398928,
494.869147108234));
#111777=CARTESIAN_POINT('Ctrl Pts',(-57.2940029153359,1076.64571253121,
494.681429327873));
#111778=CARTESIAN_POINT('Origin',(-55.8158882427217,1067.7251047501,494.657824979653));
#111779=CARTESIAN_POINT('',(-55.8158882427216,1076.65362934538,495.536128111846));
#111780=CARTESIAN_POINT('',(-55.8158882427215,1076.68940454296,493.77952184746));
#111781=CARTESIAN_POINT('Ctrl Pts',(-55.8158882427216,1076.65362934538,
495.536128111847));
#111782=CARTESIAN_POINT('Ctrl Pts',(-55.9318099253898,1076.6514841644,495.536128111847));
#111783=CARTESIAN_POINT('Ctrl Pts',(-56.0465906650825,1076.64985449637,
495.513181130269));
#111784=CARTESIAN_POINT('Ctrl Pts',(-56.2597332812426,1076.64792005606,
495.424397387823));
#111785=CARTESIAN_POINT('Ctrl Pts',(-56.356150285274,1076.64762439934,495.359786049275));
#111786=CARTESIAN_POINT('Ctrl Pts',(-56.5187548885584,1076.64842144831,
495.196950801317));
#111787=CARTESIAN_POINT('Ctrl Pts',(-56.5833076956239,1076.64950824845,
495.100253495072));
#111788=CARTESIAN_POINT('Ctrl Pts',(-56.6714627049711,1076.65286727937,
494.887375877515));
#111789=CARTESIAN_POINT('Ctrl Pts',(-56.6941678581457,1076.65510581828,
494.773247505017));
#111790=CARTESIAN_POINT('Ctrl Pts',(-56.6942147740036,1076.66031704546,
494.543158682441));
#111791=CARTESIAN_POINT('Ctrl Pts',(-56.6717125907137,1076.66323443647,
494.4294211434));
#111792=CARTESIAN_POINT('Ctrl Pts',(-56.606100422734,1076.66776210203,494.270170403875));
#111793=CARTESIAN_POINT('Ctrl Pts',(-56.5790833909399,1076.6692858448,494.219368012302));
#111794=CARTESIAN_POINT('Ctrl Pts',(-56.5155193997886,1076.67231347924,
494.123757001964));
#111795=CARTESIAN_POINT('Ctrl Pts',(-56.4791234046984,1076.67381008737,
494.079178587676));
#111796=CARTESIAN_POINT('Ctrl Pts',(-56.3561618958448,1076.67823756045,
493.955542808976));
#111797=CARTESIAN_POINT('Ctrl Pts',(-56.2579414138775,1076.68099912889,
493.889913730455));
#111798=CARTESIAN_POINT('Ctrl Pts',(-56.0438306225788,1076.68580135196,
493.801920488004));
#111799=CARTESIAN_POINT('Ctrl Pts',(-55.9304168842139,1076.6878121255,493.77952184746));
#111800=CARTESIAN_POINT('Ctrl Pts',(-55.8158882427215,1076.68940454296,
493.77952184746));
#111801=CARTESIAN_POINT('',(-55.8158882427217,1082.7251047501,493.77952184746));
#111802=CARTESIAN_POINT('',(-55.8158882427217,1067.7251047501,493.77952184746));
#111803=CARTESIAN_POINT('Origin',(-55.8158882427217,1082.7251047501,494.657824979653));
#111804=CARTESIAN_POINT('Ctrl Pts',(-55.8158882427215,1076.68940454296,
493.77952184746));
#111805=CARTESIAN_POINT('Ctrl Pts',(-55.7821001946735,1076.68987433529,
493.77952184746));
#111806=CARTESIAN_POINT('Ctrl Pts',(-55.7482262561783,1076.6903067822,493.781475913434));
#111807=CARTESIAN_POINT('Ctrl Pts',(-55.7145493171291,1076.69070046539,
493.785387695844));
#111808=CARTESIAN_POINT('Ctrl Pts',(-55.6808922225021,1076.6910939166,493.789297173203));
#111809=CARTESIAN_POINT('Ctrl Pts',(-55.6474325946985,1076.69144864976,
493.795162012409));
#111810=CARTESIAN_POINT('Ctrl Pts',(-55.6144491808781,1076.69176324906,
493.802933936079));
#111811=CARTESIAN_POINT('Ctrl Pts',(-55.581442507272,1076.69207807021,493.810711340481));
#111812=CARTESIAN_POINT('Ctrl Pts',(-55.5489133962765,1076.69235270089,
493.820398332048));
#111813=CARTESIAN_POINT('Ctrl Pts',(-55.5171271742132,1076.69258572228,
493.831896280573));
#111814=CARTESIAN_POINT('Ctrl Pts',(-55.5046378310411,1076.69267728032,
493.836414018624));
#111815=CARTESIAN_POINT('Ctrl Pts',(-55.492262970637,1076.69276241456,493.841210808931));
#111816=CARTESIAN_POINT('Ctrl Pts',(-55.4800177556225,1076.69284103895,
493.846278672955));
#111817=CARTESIAN_POINT('Ctrl Pts',(-55.4493021409524,1076.69303825855,
493.858990786084));
#111818=CARTESIAN_POINT('Ctrl Pts',(-55.4192090869223,1076.69319580211,
493.87349241555));
#111819=CARTESIAN_POINT('Ctrl Pts',(-55.3899988367886,1076.69331340156,
493.889687878652));
#111820=CARTESIAN_POINT('Ctrl Pts',(-55.3608116220149,1076.69343090827,
493.905870569925));
#111821=CARTESIAN_POINT('Ctrl Pts',(-55.3325064623312,1076.69350853384,
493.923744129845));
#111822=CARTESIAN_POINT('Ctrl Pts',(-55.3053211225215,1076.69354601083,
493.943165894641));
#111823=CARTESIAN_POINT('Ctrl Pts',(-55.2781218566449,1076.69358350702,
493.962597608505));
#111824=CARTESIAN_POINT('Ctrl Pts',(-55.2520441293685,1076.69358081348,
493.983578693448));
#111825=CARTESIAN_POINT('Ctrl Pts',(-55.2272950298924,1076.69353766235,
494.005924356988));
#111826=CARTESIAN_POINT('Ctrl Pts',(-55.216333613823,1076.69351855065,494.015821287405));
#111827=CARTESIAN_POINT('Ctrl Pts',(-55.2056323644168,1076.69349150272,
494.025985384072));
#111828=CARTESIAN_POINT('Ctrl Pts',(-55.1952069125942,1076.69345649528,
494.036398331969));
#111829=CARTESIAN_POINT('Ctrl Pts',(-55.1691826970598,1076.69336910902,
494.062391334963));
#111830=CARTESIAN_POINT('Ctrl Pts',(-55.1447437569286,1076.69323205413,
494.090072711985));
#111831=CARTESIAN_POINT('Ctrl Pts',(-55.122118922625,1076.69304601473,494.119215174216));
#111832=CARTESIAN_POINT('Ctrl Pts',(-55.0995148656774,1076.69286014618,
494.148330873674));
#111833=CARTESIAN_POINT('Ctrl Pts',(-55.0787220094823,1076.69262538305,
494.178904513048));
#111834=CARTESIAN_POINT('Ctrl Pts',(-55.0599299770165,1076.69234240759,
494.210674565886));
#111835=CARTESIAN_POINT('Ctrl Pts',(-55.0411416141871,1076.69205948739,
494.242438414789));
#111836=CARTESIAN_POINT('Ctrl Pts',(-55.0243536261026,1076.69172837369,
494.275397675653));
#111837=CARTESIAN_POINT('Ctrl Pts',(-55.0097112425333,1076.69134974834,
494.309263598563));
#111838=CARTESIAN_POINT('Ctrl Pts',(-55.00801180533,1076.69130580399,494.313194175101));
#111839=CARTESIAN_POINT('Ctrl Pts',(-55.0063412185899,1076.69126121963,
494.317136939995));
#111840=CARTESIAN_POINT('Ctrl Pts',(-55.0046996678512,1076.69121599633,
494.321091423232));
#111841=CARTESIAN_POINT('Ctrl Pts',(-54.9799734517168,1076.69053481046,
494.380656689733));
#111842=CARTESIAN_POINT('Ctrl Pts',(-54.9619045291505,1076.68971277992,
494.44270380246));
#111843=CARTESIAN_POINT('Ctrl Pts',(-54.9507810139883,1076.68875358168,
494.506148103322));
#111844=CARTESIAN_POINT('Ctrl Pts',(-54.94206944209,1076.68800236911,494.555835596927));
#111845=CARTESIAN_POINT('Ctrl Pts',(-54.9376183128041,1076.68716702462,
494.606383269385));
#111846=CARTESIAN_POINT('Ctrl Pts',(-54.9375852955171,1076.68624931446,
494.657254933818));
#111847=CARTESIAN_POINT('Ctrl Pts',(-54.9375535676497,1076.68536744351,
494.70613991419));
#111848=CARTESIAN_POINT('Ctrl Pts',(-54.9415996313463,1076.6844205659,494.754701443179));
#111849=CARTESIAN_POINT('Ctrl Pts',(-54.9495839293193,1076.68341457731,
494.802508180478));
#111850=CARTESIAN_POINT('Ctrl Pts',(-54.9579461006785,1076.68236097824,
494.852577470324));
#111851=CARTESIAN_POINT('Ctrl Pts',(-54.9706280948863,1076.6812425407,494.901822277584));
#111852=CARTESIAN_POINT('Ctrl Pts',(-54.9875207779439,1076.68006603769,
494.949756025139));
#111853=CARTESIAN_POINT('Ctrl Pts',(-54.9927155722863,1076.67970424252,
494.964496487607));
#111854=CARTESIAN_POINT('Ctrl Pts',(-54.9983088980644,1076.67933695628,
494.979112820609));
#111855=CARTESIAN_POINT('Ctrl Pts',(-55.0042983918879,1076.67896437592,
494.993590234026));
#111856=CARTESIAN_POINT('Ctrl Pts',(-55.0200636920399,1076.67798368518,
495.031697088241));
#111857=CARTESIAN_POINT('Ctrl Pts',(-55.0384962901014,1076.67697084568,
495.068642297839));
#111858=CARTESIAN_POINT('Ctrl Pts',(-55.0594003527511,1076.67593566601,
495.104078791232));
#111859=CARTESIAN_POINT('Ctrl Pts',(-55.0803703395622,1076.67489722175,
495.139627039031));
#111860=CARTESIAN_POINT('Ctrl Pts',(-55.1038271479132,1076.6738362962,495.173656708332));
#111861=CARTESIAN_POINT('Ctrl Pts',(-55.1295307205056,1076.67276279107,
495.205848467944));
#111862=CARTESIAN_POINT('Ctrl Pts',(-55.1498187127608,1076.67191546668,
495.231257627209));
#111863=CARTESIAN_POINT('Ctrl Pts',(-55.1715055634551,1076.67106030516,
495.255522324595));
#111864=CARTESIAN_POINT('Ctrl Pts',(-55.1944563571628,1076.67020217557,
495.278501065572));
#111865=CARTESIAN_POINT('Ctrl Pts',(-55.2244257789509,1076.66908161966,
495.308506981239));
#111866=CARTESIAN_POINT('Ctrl Pts',(-55.2565645231671,1076.66795552721,
495.336332204534));
#111867=CARTESIAN_POINT('Ctrl Pts',(-55.2905527314867,1076.66683710651,
495.361699252983));
#111868=CARTESIAN_POINT('Ctrl Pts',(-55.3245065779363,1076.66571981652,
495.387040655502));
#111869=CARTESIAN_POINT('Ctrl Pts',(-55.3603058985636,1076.66461018279,
495.409928645985));
#111870=CARTESIAN_POINT('Ctrl Pts',(-55.3975995587667,1076.66352137361,
495.430127361429));
#111871=CARTESIAN_POINT('Ctrl Pts',(-55.4347481129749,1076.66243680088,
495.450247485641));
#111872=CARTESIAN_POINT('Ctrl Pts',(-55.4733791295403,1076.66137289095,
495.467699041941));
#111873=CARTESIAN_POINT('Ctrl Pts',(-55.5131174748948,1076.66034265901,
495.482292234412));
#111874=CARTESIAN_POINT('Ctrl Pts',(-55.5527151677933,1076.65931607353,
495.4968337748));
#111875=CARTESIAN_POINT('Ctrl Pts',(-55.5934120861939,1076.65832292806,
495.508536971963));
#111876=CARTESIAN_POINT('Ctrl Pts',(-55.6348132231612,1076.65737610005,
495.517259810988));
#111877=CARTESIAN_POINT('Ctrl Pts',(-55.6759343182162,1076.65643567649,
495.525923647756));
#111878=CARTESIAN_POINT('Ctrl Pts',(-55.7177498362673,1076.65554094593,
495.53164716325));
#111879=CARTESIAN_POINT('Ctrl Pts',(-55.759853498463,1076.65470452627,495.534338812662));
#111880=CARTESIAN_POINT('Ctrl Pts',(-55.7784875977145,1076.65433434643,
495.535530073937));
#111881=CARTESIAN_POINT('Ctrl Pts',(-55.79717791048,1076.65397558818,495.536128111847));
#111882=CARTESIAN_POINT('Ctrl Pts',(-55.8158882427216,1076.65362934538,
495.536128111847));
#111883=CARTESIAN_POINT('Origin',(-68.2819685228173,1067.7251047501,493.138970451766));
#111884=CARTESIAN_POINT('',(-68.2819685228347,1076.40124852519,491.86352633063));
#111885=CARTESIAN_POINT('',(-68.2819685228173,1067.7251047501,491.86352633063));
#111886=CARTESIAN_POINT('Ctrl Pts',(-68.28346036406,1076.28433347533,494.414413700426));
#111887=CARTESIAN_POINT('Ctrl Pts',(-68.4507247165836,1076.27623971056,
494.414218057178));
#111888=CARTESIAN_POINT('Ctrl Pts',(-68.6163941082646,1076.26973623853,
494.381121241454));
#111889=CARTESIAN_POINT('Ctrl Pts',(-68.9251148339525,1076.26086237681,
494.252957240118));
#111890=CARTESIAN_POINT('Ctrl Pts',(-69.0652141470784,1076.25856900424,
494.15933750728));
#111891=CARTESIAN_POINT('Ctrl Pts',(-69.3011533784143,1076.25859589523,
493.92367273988));
#111892=CARTESIAN_POINT('Ctrl Pts',(-69.3947797701972,1076.26090533003,
493.784050058676));
#111893=CARTESIAN_POINT('Ctrl Pts',(-69.5230973071309,1076.26977603473,
493.476742386807));
#111894=CARTESIAN_POINT('Ctrl Pts',(-69.5565242665948,1076.27624887419,
493.31204540069));
#111895=CARTESIAN_POINT('Ctrl Pts',(-69.5582682694181,1076.29236389343,
492.978828645352));
#111896=CARTESIAN_POINT('Ctrl Pts',(-69.5264060108366,1076.30185418939,
492.813512226457));
#111897=CARTESIAN_POINT('Ctrl Pts',(-69.4007987743507,1076.3224317955,492.504222142674));
#111898=CARTESIAN_POINT('Ctrl Pts',(-69.30810009183,1076.3333229227,492.363257618105));
#111899=CARTESIAN_POINT('Ctrl Pts',(-69.0720632380055,1076.35510063472,
492.123494272292));
#111900=CARTESIAN_POINT('Ctrl Pts',(-68.9303646132984,1076.36577121848,
492.027643532448));
#111901=CARTESIAN_POINT('Ctrl Pts',(-68.618627538777,1076.38529820527,491.897278417455));
#111902=CARTESIAN_POINT('Ctrl Pts',(-68.4518005764208,1076.3939771793,491.863691508352));
#111903=CARTESIAN_POINT('Ctrl Pts',(-68.1142574840619,1076.40842911541,
491.863362007998));
#111904=CARTESIAN_POINT('Ctrl Pts',(-67.9468862164521,1076.4140573458,491.896770805172));
#111905=CARTESIAN_POINT('Ctrl Pts',(-67.6341061620142,1076.42166822459,
492.027268821322));
#111906=CARTESIAN_POINT('Ctrl Pts',(-67.4919651124891,1076.42356086842,
492.123335356597));
#111907=CARTESIAN_POINT('Ctrl Pts',(-67.253679533919,1076.42336420323,492.365515393761));
#111908=CARTESIAN_POINT('Ctrl Pts',(-67.1599417634095,1076.42127739741,
492.509167522619));
#111909=CARTESIAN_POINT('Ctrl Pts',(-67.0345376360758,1076.41329897268,
492.823944335523));
#111910=CARTESIAN_POINT('Ctrl Pts',(-67.0038350587453,1076.40750105159,
492.991786039058));
#111911=CARTESIAN_POINT('Ctrl Pts',(-67.0095776549753,1076.3927512793,493.329242637938));
#111912=CARTESIAN_POINT('Ctrl Pts',(-67.0458392912545,1076.38394597266,
493.495517830332));
#111913=CARTESIAN_POINT('Ctrl Pts',(-67.146396932864,1076.3693004159,493.725528588682));
#111914=CARTESIAN_POINT('Ctrl Pts',(-67.1867291668689,1076.36427303905,
493.797772779109));
#111915=CARTESIAN_POINT('Ctrl Pts',(-67.2809487626751,1076.35390579143,
493.933690962128));
#111916=CARTESIAN_POINT('Ctrl Pts',(-67.3346658747061,1076.3485890675,493.997013071455));
#111917=CARTESIAN_POINT('Ctrl Pts',(-67.5156666153374,1076.3322570061,494.172504309097));
#111918=CARTESIAN_POINT('Ctrl Pts',(-67.6594579543074,1076.3212390108,494.264982563189));
#111919=CARTESIAN_POINT('Ctrl Pts',(-67.9656582728335,1076.30108565678,
494.384823070276));
#111920=CARTESIAN_POINT('Ctrl Pts',(-68.1238430822138,1076.29205720553,
494.414600399163));
#111921=CARTESIAN_POINT('Ctrl Pts',(-68.28346036406,1076.28433347533,494.414413700426));
#111922=CARTESIAN_POINT('Origin',(-68.2819685228173,1067.7251047501,493.138970451766));
#111923=CARTESIAN_POINT('',(-68.2819685228173,1076.31358867648,493.814414572903));
#111924=CARTESIAN_POINT('',(-68.2819685228168,1076.37545952532,492.46352633063));
#111925=CARTESIAN_POINT('Ctrl Pts',(-68.2819685228173,1076.31358867648,
493.814414572903));
#111926=CARTESIAN_POINT('Ctrl Pts',(-68.2864411550903,1076.31337786948,
493.814414572903));
#111927=CARTESIAN_POINT('Ctrl Pts',(-68.2909158340225,1076.31316900213,
493.814370147943));
#111928=CARTESIAN_POINT('Ctrl Pts',(-68.3838552239154,1076.3088732745,493.812522758853));
#111929=CARTESIAN_POINT('Ctrl Pts',(-68.4711496327909,1076.30563774319,
493.793398173427));
#111930=CARTESIAN_POINT('Ctrl Pts',(-68.6332391257118,1076.30130401655,
493.722610190779));
#111931=CARTESIAN_POINT('Ctrl Pts',(-68.7064803386932,1076.30024379268,
493.6717186001));
#111932=CARTESIAN_POINT('Ctrl Pts',(-68.8291498753305,1076.300473154,493.544684578535));
#111933=CARTESIAN_POINT('Ctrl Pts',(-68.8774057128442,1076.30175750292,
493.469818716931));
#111934=CARTESIAN_POINT('Ctrl Pts',(-68.9424310720892,1076.30649637888,
493.305731364767));
#111935=CARTESIAN_POINT('Ctrl Pts',(-68.9585386094659,1076.30990566649,
493.218098001518));
#111936=CARTESIAN_POINT('Ctrl Pts',(-68.9561614864957,1076.31836794158,
493.041450750661));
#111937=CARTESIAN_POINT('Ctrl Pts',(-68.9376160109658,1076.32334182643,
492.954141112806));
#111938=CARTESIAN_POINT('Ctrl Pts',(-68.867916727381,1076.33415469827,492.791503619692));
#111939=CARTESIAN_POINT('Ctrl Pts',(-68.8173619963439,1076.33989098519,
492.717759030771));
#111940=CARTESIAN_POINT('Ctrl Pts',(-68.6897538986778,1076.35142054282,
492.593065306653));
#111941=CARTESIAN_POINT('Ctrl Pts',(-68.6135705877628,1076.35709993303,
492.543699464199));
#111942=CARTESIAN_POINT('Ctrl Pts',(-68.4512493750913,1076.36725084899,
492.479632558453));
#111943=CARTESIAN_POINT('Ctrl Pts',(-68.3673872694444,1076.37168574005,
492.463621698737));
#111944=CARTESIAN_POINT('Ctrl Pts',(-68.2827260003963,1076.37542607939,
492.463526755188));
#111945=CARTESIAN_POINT('Ctrl Pts',(-68.2824735011445,1076.37543723482,
492.463526472023));
#111946=CARTESIAN_POINT('Ctrl Pts',(-68.2822210085788,1076.37544838346,
492.46352633063));
#111947=CARTESIAN_POINT('Ctrl Pts',(-68.2819685228162,1076.37545952532,
492.46352633063));
#111948=CARTESIAN_POINT('',(-68.2819685228173,1082.7251047501,492.46352633063));
#111949=CARTESIAN_POINT('',(-68.2819685228173,1067.7251047501,492.46352633063));
#111950=CARTESIAN_POINT('Origin',(-68.2819685228173,1082.7251047501,493.138970451766));
#111951=CARTESIAN_POINT('Ctrl Pts',(-68.2819685228162,1076.37545952532,
492.46352633063));
#111952=CARTESIAN_POINT('Ctrl Pts',(-68.1923058793769,1076.37941621885,
492.46352633063));
#111953=CARTESIAN_POINT('Ctrl Pts',(-68.1035011486521,1076.3825178246,492.481379977689));
#111954=CARTESIAN_POINT('Ctrl Pts',(-67.9383966698456,1076.38669236412,
492.550617802864));
#111955=CARTESIAN_POINT('Ctrl Pts',(-67.8636891351381,1076.38773405336,
492.601153607532));
#111956=CARTESIAN_POINT('Ctrl Pts',(-67.7389491901221,1076.38763727639,
492.727679936259));
#111957=CARTESIAN_POINT('Ctrl Pts',(-67.689875002397,1076.38652356686,492.802145822773));
#111958=CARTESIAN_POINT('Ctrl Pts',(-67.6225539748602,1076.38222927618,
492.967238976585));
#111959=CARTESIAN_POINT('Ctrl Pts',(-67.6055794948339,1076.37905299928,
493.056471144438));
#111960=CARTESIAN_POINT('Ctrl Pts',(-67.6075487900604,1076.37100669699,
493.236124391691));
#111961=CARTESIAN_POINT('Ctrl Pts',(-67.6264112580172,1076.36621842504,
493.3247501305));
#111962=CARTESIAN_POINT('Ctrl Pts',(-67.6794323987065,1076.35831982768,
493.447354940598));
#111963=CARTESIAN_POINT('Ctrl Pts',(-67.7007344862452,1076.35562021979,
493.485837650045));
#111964=CARTESIAN_POINT('Ctrl Pts',(-67.7505366092786,1076.35007996947,
493.558179967727));
#111965=CARTESIAN_POINT('Ctrl Pts',(-67.778931956496,1076.347252097,493.591861516285));
#111966=CARTESIAN_POINT('Ctrl Pts',(-67.8751166977207,1076.33855925955,
493.685659388942));
#111967=CARTESIAN_POINT('Ctrl Pts',(-67.9518640126957,1076.33272861279,
493.735152037157));
#111968=CARTESIAN_POINT('Ctrl Pts',(-68.1144526174297,1076.32220392407,
493.798699872179));
#111969=CARTESIAN_POINT('Ctrl Pts',(-68.1978485987653,1076.31755347115,
493.814414572903));
#111970=CARTESIAN_POINT('Ctrl Pts',(-68.2819685228173,1076.31358867648,
493.814414572903));
#111971=CARTESIAN_POINT('Origin',(-81.8208965804705,1067.7251047501,490.220805984922));
#111972=CARTESIAN_POINT('',(-81.8208965804703,1075.72563758024,489.12197484893));
#111973=CARTESIAN_POINT('',(-81.8208965804705,1067.7251047501,489.12197484893));
#111974=CARTESIAN_POINT('Ctrl Pts',(-81.8203373471217,1075.58255321203,
491.319636978608));
#111975=CARTESIAN_POINT('Ctrl Pts',(-81.9646166296934,1075.57055250947,
491.319710407358));
#111976=CARTESIAN_POINT('Ctrl Pts',(-82.1076543015382,1075.56048347303,
491.291366883468));
#111977=CARTESIAN_POINT('Ctrl Pts',(-82.3739159099637,1075.54556110887,
491.181130335127));
#111978=CARTESIAN_POINT('Ctrl Pts',(-82.494635113198,1075.54082336383,491.100680853538));
#111979=CARTESIAN_POINT('Ctrl Pts',(-82.6978507957194,1075.53738048746,
490.898195365247));
#111980=CARTESIAN_POINT('Ctrl Pts',(-82.7784964943414,1075.53868154857,
490.778383852575));
#111981=CARTESIAN_POINT('Ctrl Pts',(-82.8893387983906,1075.54714880989,
490.514622704056));
#111982=CARTESIAN_POINT('Ctrl Pts',(-82.9184286424565,1075.55423018492,
490.37329056519));
#111983=CARTESIAN_POINT('Ctrl Pts',(-82.9209480543768,1075.57321784832,
490.086938074674));
#111984=CARTESIAN_POINT('Ctrl Pts',(-82.8940753521044,1075.58496062669,
489.944689724177));
#111985=CARTESIAN_POINT('Ctrl Pts',(-82.7870675930831,1075.6115118452,489.677915064077));
#111986=CARTESIAN_POINT('Ctrl Pts',(-82.7076098244324,1075.62608482105,
489.556041063862));
#111987=CARTESIAN_POINT('Ctrl Pts',(-82.5565427608021,1075.64853464767,
489.401376995566));
#111988=CARTESIAN_POINT('Ctrl Pts',(-82.5011454202698,1075.65607337828,
489.354837736317));
#111989=CARTESIAN_POINT('Ctrl Pts',(-82.3207397628291,1075.67870862611,
489.231344855946));
#111990=CARTESIAN_POINT('Ctrl Pts',(-82.1844971094241,1075.69337870064,
489.173561564481));
#111991=CARTESIAN_POINT('Ctrl Pts',(-81.8982106477311,1075.71997194167,
489.11507227108));
#111992=CARTESIAN_POINT('Ctrl Pts',(-81.7510559619819,1075.73165729849,
489.114538175976));
#111993=CARTESIAN_POINT('Ctrl Pts',(-81.4651538278172,1075.75062697051,
489.17101295363));
#111994=CARTESIAN_POINT('Ctrl Pts',(-81.3292540072322,1075.7577332212,489.227340633631));
#111995=CARTESIAN_POINT('Ctrl Pts',(-81.0871420691125,1075.76647355093,
489.389957368954));
#111996=CARTESIAN_POINT('Ctrl Pts',(-80.9834303138446,1075.76801710112,
489.494602294134));
#111997=CARTESIAN_POINT('Ctrl Pts',(-80.8229474671619,1075.76529117916,
489.738303819777));
#111998=CARTESIAN_POINT('Ctrl Pts',(-80.7678188203122,1075.76105076667,
489.874837375416));
#111999=CARTESIAN_POINT('Ctrl Pts',(-80.7140371765568,1075.74724912962,
490.161323105469));
#112000=CARTESIAN_POINT('Ctrl Pts',(-80.7159396644293,1075.737824714,490.308363349736));
#112001=CARTESIAN_POINT('Ctrl Pts',(-80.7769326337171,1075.71486884397,
490.593530058177));
#112002=CARTESIAN_POINT('Ctrl Pts',(-80.8356659658541,1075.70154513099,
490.728774888186));
#112003=CARTESIAN_POINT('Ctrl Pts',(-80.9599158685222,1075.68005764875,
490.907298409197));
#112004=CARTESIAN_POINT('Ctrl Pts',(-81.0064703572462,1075.6727703422,490.961930090968));
#112005=CARTESIAN_POINT('Ctrl Pts',(-81.109749956188,1075.65794178802,491.061562738272));
#112006=CARTESIAN_POINT('Ctrl Pts',(-81.1662810764314,1075.65043384449,
491.106288507833));
#112007=CARTESIAN_POINT('Ctrl Pts',(-81.3497181808003,1075.62776190875,
491.224190695909));
#112008=CARTESIAN_POINT('Ctrl Pts',(-81.487266511086,1075.61291106123,491.277936473259));
#112009=CARTESIAN_POINT('Ctrl Pts',(-81.693743883515,1075.59343542508,491.314090566497));
#112010=CARTESIAN_POINT('Ctrl Pts',(-81.7569663426371,1075.58782421534,
491.319604726898));
#112011=CARTESIAN_POINT('Ctrl Pts',(-81.8203373471217,1075.58255321203,
491.319636978608));
#112012=CARTESIAN_POINT('Origin',(-81.8208965804705,1067.7251047501,490.220805984922));
#112013=CARTESIAN_POINT('',(-81.8208965804705,1075.62273721903,490.719637120915));
#112014=CARTESIAN_POINT('',(-81.820896580471,1075.68770968364,489.72197484893));
#112015=CARTESIAN_POINT('Ctrl Pts',(-81.8208965804704,1075.62273721903,
490.719637120915));
#112016=CARTESIAN_POINT('Ctrl Pts',(-81.8588780724229,1075.61961893,490.719637120915));
#112017=CARTESIAN_POINT('Ctrl Pts',(-81.8968463527419,1075.61678257443,
490.715299293843));
#112018=CARTESIAN_POINT('Ctrl Pts',(-81.9976197562922,1075.61003590419,
490.691827487908));
#112019=CARTESIAN_POINT('Ctrl Pts',(-82.0577185983606,1075.60687226465,
490.664677186573));
#112020=CARTESIAN_POINT('Ctrl Pts',(-82.1638192327644,1075.60313082568,
490.588862270848));
#112021=CARTESIAN_POINT('Ctrl Pts',(-82.2088376321711,1075.60257710667,
490.54106500921));
#112022=CARTESIAN_POINT('Ctrl Pts',(-82.2779498742101,1075.6041617528,490.430937922303));
#112023=CARTESIAN_POINT('Ctrl Pts',(-82.3013818132731,1075.60628063025,
490.369725899407));
#112024=CARTESIAN_POINT('Ctrl Pts',(-82.3235293872305,1075.61292268631,
490.241618157459));
#112025=CARTESIAN_POINT('Ctrl Pts',(-82.3219409959161,1075.61738828803,
490.175965021238));
#112026=CARTESIAN_POINT('Ctrl Pts',(-82.2936394865667,1075.62808942795,
490.048694371556));
#112027=CARTESIAN_POINT('Ctrl Pts',(-82.2670455329507,1075.63423207163,
489.988328440433));
#112028=CARTESIAN_POINT('Ctrl Pts',(-82.2108403700009,1075.64407656532,
489.907997267171));
#112029=CARTESIAN_POINT('Ctrl Pts',(-82.1894673926781,1075.64744644861,
489.883077890287));
#112030=CARTESIAN_POINT('Ctrl Pts',(-82.1421791932408,1075.65424552923,
489.837817587488));
#112031=CARTESIAN_POINT('Ctrl Pts',(-82.1163780874431,1075.65765889112,
489.817577227677));
#112032=CARTESIAN_POINT('Ctrl Pts',(-82.0325593384745,1075.66792326837,
489.764217231675));
#112033=CARTESIAN_POINT('Ctrl Pts',(-81.9696965176828,1075.67456753992,
489.740031918538));
#112034=CARTESIAN_POINT('Ctrl Pts',(-81.8764847473424,1075.68309081853,
489.724302826255));
#112035=CARTESIAN_POINT('Ctrl Pts',(-81.848720763783,1075.68547411165,489.72197484893));
#112036=CARTESIAN_POINT('Ctrl Pts',(-81.8208965804714,1075.68770968364,
489.72197484893));
#112037=CARTESIAN_POINT('',(-81.8208965804705,1082.7251047501,489.72197484893));
#112038=CARTESIAN_POINT('',(-81.8208965804705,1067.7251047501,489.72197484893));
#112039=CARTESIAN_POINT('Origin',(-81.8208965804705,1082.7251047501,490.220805984922));
#112040=CARTESIAN_POINT('Ctrl Pts',(-81.8208965804714,1075.68770968364,
489.72197484893));
#112041=CARTESIAN_POINT('Ctrl Pts',(-81.8207984790147,1075.68771756574,
489.72197484893));
#112042=CARTESIAN_POINT('Ctrl Pts',(-81.8207003768087,1075.68772544599,
489.721974878031));
#112043=CARTESIAN_POINT('Ctrl Pts',(-81.820602273868,1075.68773332441,489.721974935911));
#112044=CARTESIAN_POINT('Ctrl Pts',(-81.7542336351232,1075.69306323746,
489.722014092904));
#112045=CARTESIAN_POINT('Ctrl Pts',(-81.6884706566742,1075.69747669195,
489.73529825801));
#112046=CARTESIAN_POINT('Ctrl Pts',(-81.5660255278227,1075.70396160132,
489.786894832373));
#112047=CARTESIAN_POINT('Ctrl Pts',(-81.5105806699821,1075.70597139481,
489.824634589899));
#112048=CARTESIAN_POINT('Ctrl Pts',(-81.4187028763101,1075.70728846299,
489.918649282645));
#112049=CARTESIAN_POINT('Ctrl Pts',(-81.3827992951993,1075.70664027812,
489.973569025033));
#112050=CARTESIAN_POINT('Ctrl Pts',(-81.3335242572579,1075.70277203779,
490.095432948114));
#112051=CARTESIAN_POINT('Ctrl Pts',(-81.3211946552715,1075.6995335249,490.16135988493));
#112052=CARTESIAN_POINT('Ctrl Pts',(-81.3230344980214,1075.69084730567,
490.2942555415));
#112053=CARTESIAN_POINT('Ctrl Pts',(-81.3372608131545,1075.68548091103,
490.35987688527));
#112054=CARTESIAN_POINT('Ctrl Pts',(-81.390631021944,1075.67329905375,490.481878157933));
#112055=CARTESIAN_POINT('Ctrl Pts',(-81.4293656593663,1075.66659692712,
490.537003193671));
#112056=CARTESIAN_POINT('Ctrl Pts',(-81.5014678562907,1075.65630439878,
490.605338489547));
#112057=CARTESIAN_POINT('Ctrl Pts',(-81.527332271515,1075.65289408786,490.625429196208));
#112058=CARTESIAN_POINT('Ctrl Pts',(-81.6110935566909,1075.64263303744,
490.678206100116));
#112059=CARTESIAN_POINT('Ctrl Pts',(-81.6737373478057,1075.63595515846,
490.702039981009));
#112060=CARTESIAN_POINT('Ctrl Pts',(-81.7662844050241,1075.62736601428,
490.717395580663));
#112061=CARTESIAN_POINT('Ctrl Pts',(-81.793593906212,1075.62497877472,490.719637120915));
#112062=CARTESIAN_POINT('Ctrl Pts',(-81.8208965804704,1075.62273721903,
490.719637120915));
#112063=CARTESIAN_POINT('Origin',(-94.6032580293197,1067.7251047501,484.542321079512));
#112064=CARTESIAN_POINT('',(-94.6032580293197,1074.88000163213,483.451780330783));
#112065=CARTESIAN_POINT('',(-94.6032580293197,1067.7251047501,483.451780330783));
#112066=CARTESIAN_POINT('Ctrl Pts',(-94.6024687290833,1074.72207722087,
485.632861542604));
#112067=CARTESIAN_POINT('Ctrl Pts',(-94.745896664052,1074.7054542846,485.63296535141));
#112068=CARTESIAN_POINT('Ctrl Pts',(-94.8881904781405,1074.69097422865,
485.604772829182));
#112069=CARTESIAN_POINT('Ctrl Pts',(-95.15266120531,1074.66823897832,485.495062329079));
#112070=CARTESIAN_POINT('Ctrl Pts',(-95.2724181595792,1074.66014758065,
485.415183548233));
#112071=CARTESIAN_POINT('Ctrl Pts',(-95.4737463182846,1074.65147622274,
485.21432125542));
#112072=CARTESIAN_POINT('Ctrl Pts',(-95.5535724265119,1074.65092522316,
485.095714625435));
#112073=CARTESIAN_POINT('Ctrl Pts',(-95.66336567463,1074.65742595818,484.83469329457));
#112074=CARTESIAN_POINT('Ctrl Pts',(-95.6922583981725,1074.66440433594,
484.694954729699));
#112075=CARTESIAN_POINT('Ctrl Pts',(-95.6952297931477,1074.68500431369,
484.411552000752));
#112076=CARTESIAN_POINT('Ctrl Pts',(-95.6688934506936,1074.69846571525,
484.270680473507));
#112077=CARTESIAN_POINT('Ctrl Pts',(-95.5635056872982,1074.7301393527,484.005929220394));
#112078=CARTESIAN_POINT('Ctrl Pts',(-95.4849113886009,1074.74809568166,
483.884765536165));
#112079=CARTESIAN_POINT('Ctrl Pts',(-95.3354082583345,1074.77650113298,
483.730922002435));
#112080=CARTESIAN_POINT('Ctrl Pts',(-95.2805439144007,1074.78616535173,
483.684596042482));
#112081=CARTESIAN_POINT('Ctrl Pts',(-95.162760948298,1074.80552929484,483.603530038944));
#112082=CARTESIAN_POINT('Ctrl Pts',(-95.1001353917849,1074.81518538595,
483.568931131701));
#112083=CARTESIAN_POINT('Ctrl Pts',(-94.9014833492655,1074.8439957061,483.483389043402));
#112084=CARTESIAN_POINT('Ctrl Pts',(-94.7581467770505,1074.8624183042,483.453109785185));
#112085=CARTESIAN_POINT('Ctrl Pts',(-94.468525646668,1074.89530267907,483.450543856115));
#112086=CARTESIAN_POINT('Ctrl Pts',(-94.3250650326983,1074.90947031478,
483.477954009334));
#112087=CARTESIAN_POINT('Ctrl Pts',(-94.0569836323811,1074.93174628175,
483.587438277236));
#112088=CARTESIAN_POINT('Ctrl Pts',(-93.9350801038396,1074.9396364655,483.668332137648));
#112089=CARTESIAN_POINT('Ctrl Pts',(-93.7322722672411,1074.94794831263,
483.870961103211));
#112090=CARTESIAN_POINT('Ctrl Pts',(-93.6525214656037,1074.94845783271,
483.989648223678));
#112091=CARTESIAN_POINT('Ctrl Pts',(-93.5427663055076,1074.94222195788,
484.251147178559));
#112092=CARTESIAN_POINT('Ctrl Pts',(-93.5139706064368,1074.93552546865,
484.391347020229));
#112093=CARTESIAN_POINT('Ctrl Pts',(-93.5115161919005,1074.91547687092,
484.677855297207));
#112094=CARTESIAN_POINT('Ctrl Pts',(-93.5391549381978,1074.90218075921,
484.821277616227));
#112095=CARTESIAN_POINT('Ctrl Pts',(-93.6487067240138,1074.87068512212,
485.089289147712));
#112096=CARTESIAN_POINT('Ctrl Pts',(-93.7298082798916,1074.85276960261,
485.211140951457));
#112097=CARTESIAN_POINT('Ctrl Pts',(-93.9353946458708,1074.8145642406,485.416703002735));
#112098=CARTESIAN_POINT('Ctrl Pts',(-94.0582756150637,1074.79461906541,
485.498127843746));
#112099=CARTESIAN_POINT('Ctrl Pts',(-94.3232856728116,1074.75635740111,
485.605573678612));
#112100=CARTESIAN_POINT('Ctrl Pts',(-94.4621322209791,1074.73834186855,
485.63275997128));
#112101=CARTESIAN_POINT('Ctrl Pts',(-94.6024687290833,1074.72207722087,
485.632861542604));
#112102=CARTESIAN_POINT('Origin',(-94.6032580293197,1067.7251047501,484.542321079512));
#112103=CARTESIAN_POINT('',(-94.6032580293198,1074.76643751182,485.03286182824));
#112104=CARTESIAN_POINT('',(-94.60325802932,1074.83751173097,484.051780330783));
#112105=CARTESIAN_POINT('Ctrl Pts',(-94.6032580293198,1074.76643751182,
485.03286182824));
#112106=CARTESIAN_POINT('Ctrl Pts',(-94.6064097860182,1074.76607494461,
485.03286182824));
#112107=CARTESIAN_POINT('Ctrl Pts',(-94.6095631087125,1074.765714379,485.032831452973));
#112108=CARTESIAN_POINT('Ctrl Pts',(-94.6771372393172,1074.75803452305,
485.031528117375));
#112109=CARTESIAN_POINT('Ctrl Pts',(-94.7407944245279,1074.75171223875,
485.017603492421));
#112110=CARTESIAN_POINT('Ctrl Pts',(-94.8586327401454,1074.7418854872,484.966005962437));
#112111=CARTESIAN_POINT('Ctrl Pts',(-94.9117375447669,1074.73845089191,
484.929083822759));
#112112=CARTESIAN_POINT('Ctrl Pts',(-95.0005030181127,1074.73492674128,
484.837081653654));
#112113=CARTESIAN_POINT('Ctrl Pts',(-95.0353817940901,1074.7348499967,484.783063505805));
#112114=CARTESIAN_POINT('Ctrl Pts',(-95.0825445278263,1074.7380647946,484.664693286736));
#112115=CARTESIAN_POINT('Ctrl Pts',(-95.0943431949663,1074.74132438622,
484.601541527186));
#112116=CARTESIAN_POINT('Ctrl Pts',(-95.0932115512552,1074.75078405641,
484.473923114327));
#112117=CARTESIAN_POINT('Ctrl Pts',(-95.0801080805805,1074.7569114572,484.410717421114));
#112118=CARTESIAN_POINT('Ctrl Pts',(-95.0302899119064,1074.77126494828,
484.292455501764));
#112119=CARTESIAN_POINT('Ctrl Pts',(-94.9938128842482,1074.77937423418,
484.238617070232));
#112120=CARTESIAN_POINT('Ctrl Pts',(-94.9251845633391,1074.7921660622,484.170801255045));
#112121=CARTESIAN_POINT('Ctrl Pts',(-94.9001564002189,1074.79650407244,
484.150512099338));
#112122=CARTESIAN_POINT('Ctrl Pts',(-94.8465456064098,1074.80519900672,
484.115155060813));
#112123=CARTESIAN_POINT('Ctrl Pts',(-94.8180886671918,1074.80953642642,
484.100158106668));
#112124=CARTESIAN_POINT('Ctrl Pts',(-94.7296563935429,1074.82223691641,
484.064123506368));
#112125=CARTESIAN_POINT('Ctrl Pts',(-94.6667958248473,1074.83028711391,
484.051780330783));
#112126=CARTESIAN_POINT('Ctrl Pts',(-94.6032580293202,1074.83751173097,
484.051780330783));
#112127=CARTESIAN_POINT('',(-94.6032580293197,1082.7251047501,484.051780330783));
#112128=CARTESIAN_POINT('',(-94.6032580293197,1067.7251047501,484.051780330783));
#112129=CARTESIAN_POINT('Origin',(-94.6032580293197,1082.7251047501,484.542321079512));
#112130=CARTESIAN_POINT('Ctrl Pts',(-94.6032580293202,1074.83751173097,
484.051780330783));
#112131=CARTESIAN_POINT('Ctrl Pts',(-94.6031280517499,1074.83752651018,
484.051780330783));
#112132=CARTESIAN_POINT('Ctrl Pts',(-94.6029980713456,1074.83754128593,
484.051780382445));
#112133=CARTESIAN_POINT('Ctrl Pts',(-94.6028680881373,1074.83755605823,
484.051780485771));
#112134=CARTESIAN_POINT('Ctrl Pts',(-94.5376062273942,1074.84497292011,
484.051832363816));
#112135=CARTESIAN_POINT('Ctrl Pts',(-94.4728961004285,1074.85137516962,
484.064907529361));
#112136=CARTESIAN_POINT('Ctrl Pts',(-94.3531213898483,1074.86132287037,
484.115443377367));
#112137=CARTESIAN_POINT('Ctrl Pts',(-94.2991328186827,1074.86480920347,
484.152037997717));
#112138=CARTESIAN_POINT('Ctrl Pts',(-94.2090502874632,1074.86844628791,
484.243508428265));
#112139=CARTESIAN_POINT('Ctrl Pts',(-94.1736130737808,1074.8686093583,484.297178339696));
#112140=CARTESIAN_POINT('Ctrl Pts',(-94.1252124831204,1074.86563134578,
484.415148274704));
#112141=CARTESIAN_POINT('Ctrl Pts',(-94.1127692976782,1074.86251619174,
484.47826283707));
#112142=CARTESIAN_POINT('Ctrl Pts',(-94.1126651952564,1074.85335524365,
484.606063527551));
#112143=CARTESIAN_POINT('Ctrl Pts',(-94.1251918226818,1074.84737857733,
484.669483302672));
#112144=CARTESIAN_POINT('Ctrl Pts',(-94.1743606068894,1074.83316915046,
484.789244988087));
#112145=CARTESIAN_POINT('Ctrl Pts',(-94.2111091104492,1074.82502408753,
484.844185383084));
#112146=CARTESIAN_POINT('Ctrl Pts',(-94.3040475266962,1074.80774374707,
484.93654810885));
#112147=CARTESIAN_POINT('Ctrl Pts',(-94.3594406529071,1074.79876839697,
484.973010432572));
#112148=CARTESIAN_POINT('Ctrl Pts',(-94.4784676554407,1074.78165605926,
485.020839280529));
#112149=CARTESIAN_POINT('Ctrl Pts',(-94.5405529418956,1074.77365088853,
485.03286182824));
#112150=CARTESIAN_POINT('Ctrl Pts',(-94.6032580293198,1074.76643751182,
485.03286182824));
#112151=CARTESIAN_POINT('Origin',(-40.034544989914,1067.7251047501,504.732111464453));
#112152=CARTESIAN_POINT('',(-40.0345449899334,1076.70230022208,503.25380833226));
#112153=CARTESIAN_POINT('',(-40.034544989914,1067.7251047501,503.25380833226));
#112154=CARTESIAN_POINT('Ctrl Pts',(-41.5126544848484,1076.65353483496,
504.756037843979));
#112155=CARTESIAN_POINT('Ctrl Pts',(-41.5157829477054,1076.65862947213,
504.562769545764));
#112156=CARTESIAN_POINT('Ctrl Pts',(-41.4809754826117,1076.66395691137,
504.370751622908));
#112157=CARTESIAN_POINT('Ctrl Pts',(-41.3748386768931,1076.671697424,504.100980925426));
#112158=CARTESIAN_POINT('Ctrl Pts',(-41.3307415283915,1076.67421835813,
504.014763411445));
#112159=CARTESIAN_POINT('Ctrl Pts',(-41.1728328279325,1076.68155683822,
503.768798538432));
#112160=CARTESIAN_POINT('Ctrl Pts',(-41.035460762808,1076.68599837266,503.626739159453));
#112161=CARTESIAN_POINT('Ctrl Pts',(-40.7141068724518,1076.69359618941,
503.404889210497));
#112162=CARTESIAN_POINT('Ctrl Pts',(-40.5334941467736,1076.69669063987,
503.326984693202));
#112163=CARTESIAN_POINT('Ctrl Pts',(-40.1516574964021,1076.70149343388,
503.245527793793));
#112164=CARTESIAN_POINT('Ctrl Pts',(-39.9541267344701,1076.70315709624,
503.243090353066));
#112165=CARTESIAN_POINT('Ctrl Pts',(-39.5687072605579,1076.70511465722,
503.315426844983));
#112166=CARTESIAN_POINT('Ctrl Pts',(-39.3847114872663,1076.70538783021,
503.389830836801));
#112167=CARTESIAN_POINT('Ctrl Pts',(-39.0569614391553,1076.70454797393,
503.60598480715));
#112168=CARTESIAN_POINT('Ctrl Pts',(-38.9163742522714,1076.70344403643,
503.745439270994));
#112169=CARTESIAN_POINT('Ctrl Pts',(-38.6984245787826,1076.69978090374,
504.070154914735));
#112170=CARTESIAN_POINT('Ctrl Pts',(-38.6228580340899,1076.69725797628,
504.251968490841));
#112171=CARTESIAN_POINT('Ctrl Pts',(-38.5466193189783,1076.69074840334,
504.634528523447));
#112172=CARTESIAN_POINT('Ctrl Pts',(-38.5467436536565,1076.68681682594,
504.83152478639));
#112173=CARTESIAN_POINT('Ctrl Pts',(-38.6039355625039,1076.68008029063,
505.116702268898));
#112174=CARTESIAN_POINT('Ctrl Pts',(-38.6318496719947,1076.67773785312,
505.208554792672));
#112175=CARTESIAN_POINT('Ctrl Pts',(-38.7057448878917,1076.67281221251,
505.387240795265));
#112176=CARTESIAN_POINT('Ctrl Pts',(-38.7518781659053,1076.67023730474,
505.473508302114));
#112177=CARTESIAN_POINT('Ctrl Pts',(-38.9141030826265,1076.66239782396,
505.715789219588));
#112178=CARTESIAN_POINT('Ctrl Pts',(-39.0527146610104,1076.65705882752,
505.854173265541));
#112179=CARTESIAN_POINT('Ctrl Pts',(-39.375534020827,1076.64695840291,506.069553768881));
#112180=CARTESIAN_POINT('Ctrl Pts',(-39.556634319814,1076.64230177121,506.144435499386));
#112181=CARTESIAN_POINT('Ctrl Pts',(-39.9373270307768,1076.63464626945,
506.219916336102));
#112182=CARTESIAN_POINT('Ctrl Pts',(-40.1332117643458,1076.63172763579,
506.219824770339));
#112183=CARTESIAN_POINT('Ctrl Pts',(-40.5133943389907,1076.6283043857,506.144052600482));
#112184=CARTESIAN_POINT('Ctrl Pts',(-40.6940222587757,1076.62783155312,
506.069260076883));
#112185=CARTESIAN_POINT('Ctrl Pts',(-41.0158209134949,1076.62945747136,
505.854525767654));
#112186=CARTESIAN_POINT('Ctrl Pts',(-41.1539607251774,1076.63153330559,
505.716802225688));
#112187=CARTESIAN_POINT('Ctrl Pts',(-41.3693507204397,1076.63778327435,
505.396152827116));
#112188=CARTESIAN_POINT('Ctrl Pts',(-41.4445668953704,1076.64188997198,
505.216346606781));
#112189=CARTESIAN_POINT('Ctrl Pts',(-41.5012863953776,1076.64880143344,
504.937907114078));
#112190=CARTESIAN_POINT('Ctrl Pts',(-41.5111798515923,1076.65113342516,
504.847136851046));
#112191=CARTESIAN_POINT('Ctrl Pts',(-41.5126544848484,1076.65353483496,
504.756037843979));
#112192=CARTESIAN_POINT('Origin',(-40.034544989914,1067.7251047501,504.732111464453));
#112193=CARTESIAN_POINT('',(-40.034544989914,1076.65067043007,505.610414596646));
#112194=CARTESIAN_POINT('',(-40.0345449899148,1076.69158153387,503.85380833226));
#112195=CARTESIAN_POINT('Ctrl Pts',(-40.034544989914,1076.65067043007,505.610414596647));
#112196=CARTESIAN_POINT('Ctrl Pts',(-40.099230217787,1076.64979703943,505.610414596647));
#112197=CARTESIAN_POINT('Ctrl Pts',(-40.1638735490618,1076.64911108635,
505.603268574889));
#112198=CARTESIAN_POINT('Ctrl Pts',(-40.3394889650877,1076.64779221792,
505.563768045686));
#112199=CARTESIAN_POINT('Ctrl Pts',(-40.4456532701006,1076.64762563924,
505.51673487539));
#112200=CARTESIAN_POINT('Ctrl Pts',(-40.6337073127725,1076.64867381101,
505.384505414016));
#112201=CARTESIAN_POINT('Ctrl Pts',(-40.7138042450954,1076.64987607597,
505.300633618999));
#112202=CARTESIAN_POINT('Ctrl Pts',(-40.8371524395397,1076.65342653398,
505.106847831021));
#112203=CARTESIAN_POINT('Ctrl Pts',(-40.8792192419791,1076.65573802481,
504.998809249611));
#112204=CARTESIAN_POINT('Ctrl Pts',(-40.9194065315618,1076.66105587421,
504.772613146271));
#112205=CARTESIAN_POINT('Ctrl Pts',(-40.9171097966551,1076.66400893629,
504.656628413306));
#112206=CARTESIAN_POINT('Ctrl Pts',(-40.8802800239126,1076.66855499991,
504.488298378343));
#112207=CARTESIAN_POINT('Ctrl Pts',(-40.8625390204781,1076.67007872801,
504.433550794752));
#112208=CARTESIAN_POINT('Ctrl Pts',(-40.8166453557619,1076.67309430675,
504.328346280406));
#112209=CARTESIAN_POINT('Ctrl Pts',(-40.7886109472355,1076.67457894721,
504.278137862969));
#112210=CARTESIAN_POINT('Ctrl Pts',(-40.6893417422963,1076.6789503985,504.13523618805));
#112211=CARTESIAN_POINT('Ctrl Pts',(-40.6043812201753,1076.68165548887,
504.053651109645));
#112212=CARTESIAN_POINT('Ctrl Pts',(-40.4077164533096,1076.68637261445,
503.928545470762));
#112213=CARTESIAN_POINT('Ctrl Pts',(-40.2980076229507,1076.68834162645,
503.886200266871));
#112214=CARTESIAN_POINT('Ctrl Pts',(-40.1341230671946,1076.69052631114,
503.858049952025));
#112215=CARTESIAN_POINT('Ctrl Pts',(-40.0843834156782,1076.69109675782,
503.853808757965));
#112216=CARTESIAN_POINT('Ctrl Pts',(-40.0345524926856,1076.69158146089,
503.853808332292));
#112217=CARTESIAN_POINT('',(-40.034544989914,1082.7251047501,503.85380833226));
#112218=CARTESIAN_POINT('',(-40.034544989914,1067.7251047501,503.85380833226));
#112219=CARTESIAN_POINT('Origin',(-40.034544989914,1082.7251047501,504.732111464453));
#112220=CARTESIAN_POINT('Ctrl Pts',(-40.0345449899164,1076.69158153387,
503.85380833226));
#112221=CARTESIAN_POINT('Ctrl Pts',(-39.9175261494676,1076.69271975024,
503.85380833226));
#112222=CARTESIAN_POINT('Ctrl Pts',(-39.8016831027087,1076.69337219467,
503.877192551933));
#112223=CARTESIAN_POINT('Ctrl Pts',(-39.5858789949519,1076.69369562175,
503.968022865444));
#112224=CARTESIAN_POINT('Ctrl Pts',(-39.4881051958344,1076.69336295687,
504.034590504819));
#112225=CARTESIAN_POINT('Ctrl Pts',(-39.3247018721275,1076.69171549948,
504.201862509166));
#112226=CARTESIAN_POINT('Ctrl Pts',(-39.2605967479819,1076.69041841276,
504.300784393691));
#112227=CARTESIAN_POINT('Ctrl Pts',(-39.1749142126364,1076.68691720146,
504.517617169565));
#112228=CARTESIAN_POINT('Ctrl Pts',(-39.1540837692115,1076.68474700539,
504.633330225056));
#112229=CARTESIAN_POINT('Ctrl Pts',(-39.1587608620073,1076.67968679998,
504.86650153227));
#112230=CARTESIAN_POINT('Ctrl Pts',(-39.1843734758727,1076.6768426824,504.981639703758));
#112231=CARTESIAN_POINT('Ctrl Pts',(-39.2552755448874,1076.67232959844,
505.141403131959));
#112232=CARTESIAN_POINT('Ctrl Pts',(-39.28399682815,1076.67080152637,505.191956959883));
#112233=CARTESIAN_POINT('Ctrl Pts',(-39.3839984221867,1076.66621825487,
505.333335029321));
#112234=CARTESIAN_POINT('Ctrl Pts',(-39.4683574262096,1076.66318463493,
505.413370284416));
#112235=CARTESIAN_POINT('Ctrl Pts',(-39.6631621868751,1076.65757214213,
505.536324749776));
#112236=CARTESIAN_POINT('Ctrl Pts',(-39.7717249270997,1076.65505002948,
505.578050817571));
#112237=CARTESIAN_POINT('Ctrl Pts',(-39.9346746491659,1076.65213011358,
505.606158255156));
#112238=CARTESIAN_POINT('Ctrl Pts',(-39.9846222978553,1076.65134449451,
505.610414596647));
#112239=CARTESIAN_POINT('Ctrl Pts',(-40.034544989914,1076.65067043007,505.610414596647));
#112240=CARTESIAN_POINT('Origin',(-52.5439991194437,1067.7251047501,505.838291381042));
#112241=CARTESIAN_POINT('',(-52.5439991194708,1076.41132893179,504.562847259905));
#112242=CARTESIAN_POINT('',(-52.5439991194437,1067.7251047501,504.562847259905));
#112243=CARTESIAN_POINT('Ctrl Pts',(-52.5448754729142,1076.27282192338,
507.113735201108));
#112244=CARTESIAN_POINT('Ctrl Pts',(-52.7120708255886,1076.26653123827,
507.113620321703));
#112245=CARTESIAN_POINT('Ctrl Pts',(-52.8776731502766,1076.26216701088,
507.08063083869));
#112246=CARTESIAN_POINT('Ctrl Pts',(-53.1862263402415,1076.25794216686,
506.952781983516));
#112247=CARTESIAN_POINT('Ctrl Pts',(-53.3262292977647,1076.25810841153,
506.85939843974));
#112248=CARTESIAN_POINT('Ctrl Pts',(-53.5621686327428,1076.26296163143,
506.624279190074));
#112249=CARTESIAN_POINT('Ctrl Pts',(-53.6558776560769,1076.2675914453,506.484926632456));
#112250=CARTESIAN_POINT('Ctrl Pts',(-53.7845871745367,1076.28059635365,
506.178029184282));
#112251=CARTESIAN_POINT('Ctrl Pts',(-53.8182701685065,1076.2888463096,506.013417708415));
#112252=CARTESIAN_POINT('Ctrl Pts',(-53.8205595391109,1076.30771904487,
505.680191254166));
#112253=CARTESIAN_POINT('Ctrl Pts',(-53.7889494086595,1076.31816396595,
505.514755483463));
#112254=CARTESIAN_POINT('Ctrl Pts',(-53.6637610991126,1076.33972761712,
505.205183755935));
#112255=CARTESIAN_POINT('Ctrl Pts',(-53.5712476554929,1076.35064011546,
505.064042953511));
#112256=CARTESIAN_POINT('Ctrl Pts',(-53.3355031310887,1076.37159041586,
504.823916099185));
#112257=CARTESIAN_POINT('Ctrl Pts',(-53.1939404166316,1076.38141052102,
504.727864515446));
#112258=CARTESIAN_POINT('Ctrl Pts',(-52.8822616770613,1076.3985626049,504.597019981783));
#112259=CARTESIAN_POINT('Ctrl Pts',(-52.715362969147,1076.40574306297,504.56320249138));
#112260=CARTESIAN_POINT('Ctrl Pts',(-52.3778389214085,1076.41674546459,
504.562497332901));
#112261=CARTESIAN_POINT('Ctrl Pts',(-52.2105725882794,1076.42046023434,
504.595668260933));
#112262=CARTESIAN_POINT('Ctrl Pts',(-51.8984330780026,1076.42403563,504.725366919091));
#112263=CARTESIAN_POINT('Ctrl Pts',(-51.7567208113037,1076.42385755791,
504.820672643409));
#112264=CARTESIAN_POINT('Ctrl Pts',(-51.5189065640949,1076.41958346645,
505.060821615217));
#112265=CARTESIAN_POINT('Ctrl Pts',(-51.425118593829,1076.41553343089,505.203191024268));
#112266=CARTESIAN_POINT('Ctrl Pts',(-51.2984594434416,1076.40391402638,
505.51602663548));
#112267=CARTESIAN_POINT('Ctrl Pts',(-51.2668218078869,1076.3964565273,505.683371240081));
#112268=CARTESIAN_POINT('Ctrl Pts',(-51.2704451220595,1076.37884131952,
506.021523645012));
#112269=CARTESIAN_POINT('Ctrl Pts',(-51.3060590868485,1076.36883879867,
506.188982377302));
#112270=CARTESIAN_POINT('Ctrl Pts',(-51.4068094233405,1076.3528790641,506.421963701217));
#112271=CARTESIAN_POINT('Ctrl Pts',(-51.4478889292366,1076.34745324099,
506.49587366197));
#112272=CARTESIAN_POINT('Ctrl Pts',(-51.591489026787,1076.33111484934,506.702918265949));
#112273=CARTESIAN_POINT('Ctrl Pts',(-51.7132521954594,1076.32022615565,
506.820496694586));
#112274=CARTESIAN_POINT('Ctrl Pts',(-51.9952958290798,1076.29976031084,
507.001813900014));
#112275=CARTESIAN_POINT('Ctrl Pts',(-52.1528580501541,1076.29038355797,
507.063815480095));
#112276=CARTESIAN_POINT('Ctrl Pts',(-52.3928309469499,1076.27892838407,
507.107028210238));
#112277=CARTESIAN_POINT('Ctrl Pts',(-52.4687717021975,1076.27568530953,
507.113787491771));
#112278=CARTESIAN_POINT('Ctrl Pts',(-52.5448754729142,1076.27282192338,
507.113735201108));
#112279=CARTESIAN_POINT('Origin',(-52.5439991194437,1067.7251047501,505.838291381042));
#112280=CARTESIAN_POINT('',(-52.5439991194437,1076.3076507295,506.513735502178));
#112281=CARTESIAN_POINT('',(-52.543999119444,1076.38098512892,505.162847259905));
#112282=CARTESIAN_POINT('Ctrl Pts',(-52.5439991194437,1076.3076507295,506.513735502178));
#112283=CARTESIAN_POINT('Ctrl Pts',(-52.5941445622273,1076.30582150806,
506.513735502178));
#112284=CARTESIAN_POINT('Ctrl Pts',(-52.6442631377859,1076.30430342464,
506.508151231897));
#112285=CARTESIAN_POINT('Ctrl Pts',(-52.7795876422319,1076.30108395938,
506.477455207571));
#112286=CARTESIAN_POINT('Ctrl Pts',(-52.8611026658913,1076.30014727865,
506.441185788444));
#112287=CARTESIAN_POINT('Ctrl Pts',(-53.005413680361,1076.30062591086,506.339393634614));
#112288=CARTESIAN_POINT('Ctrl Pts',(-53.0668314323192,1076.30203198681,
506.274923252499));
#112289=CARTESIAN_POINT('Ctrl Pts',(-53.1614262452317,1076.30699175589,
506.126026444978));
#112290=CARTESIAN_POINT('Ctrl Pts',(-53.1936708617585,1076.31049710481,
506.043041214527));
#112291=CARTESIAN_POINT('Ctrl Pts',(-53.2244955888446,1076.31911280663,
505.869235450439));
#112292=CARTESIAN_POINT('Ctrl Pts',(-53.2226986656671,1076.32414260447,
505.780072386387));
#112293=CARTESIAN_POINT('Ctrl Pts',(-53.1943537621746,1076.33229664811,
505.650627069925));
#112294=CARTESIAN_POINT('Ctrl Pts',(-53.180681692702,1076.33509882485,505.608479093141));
#112295=CARTESIAN_POINT('Ctrl Pts',(-53.1452919845341,1076.34078421601,
505.527441243967));
#112296=CARTESIAN_POINT('Ctrl Pts',(-53.1236531670261,1076.34365396815,
505.488745897926));
#112297=CARTESIAN_POINT('Ctrl Pts',(-53.047789446097,1076.35222361264,505.379744018297));
#112298=CARTESIAN_POINT('Ctrl Pts',(-52.983370784426,1076.35779279807,505.317686780181));
#112299=CARTESIAN_POINT('Ctrl Pts',(-52.8331743764977,1076.36809886091,
505.221302044327));
#112300=CARTESIAN_POINT('Ctrl Pts',(-52.7485973774765,1076.37272189553,
505.188330179835));
#112301=CARTESIAN_POINT('Ctrl Pts',(-52.621857827715,1076.3781787059,505.166232553107));
#112302=CARTESIAN_POINT('Ctrl Pts',(-52.5831920692139,1076.37966146313,
505.162873039544));
#112303=CARTESIAN_POINT('Ctrl Pts',(-52.5444459373632,1076.38097004623,
505.162847408246));
#112304=CARTESIAN_POINT('Ctrl Pts',(-52.5442969956814,1076.38097507648,
505.162847309719));
#112305=CARTESIAN_POINT('Ctrl Pts',(-52.5441480563678,1076.38098010406,
505.162847259905));
#112306=CARTESIAN_POINT('Ctrl Pts',(-52.5439991194442,1076.38098512892,
505.162847259905));
#112307=CARTESIAN_POINT('',(-52.5439991194437,1082.7251047501,505.162847259905));
#112308=CARTESIAN_POINT('',(-52.5439991194437,1067.7251047501,505.162847259905));
#112309=CARTESIAN_POINT('Origin',(-52.5439991194437,1082.7251047501,505.838291381042));
#112310=CARTESIAN_POINT('Ctrl Pts',(-52.5439991194442,1076.38098512892,
505.162847259905));
#112311=CARTESIAN_POINT('Ctrl Pts',(-52.454389053301,1076.38400840739,505.162847259905));
#112312=CARTESIAN_POINT('Ctrl Pts',(-52.3656445614433,1076.38605774787,
505.180680000485));
#112313=CARTESIAN_POINT('Ctrl Pts',(-52.200111080427,1076.38801101988,505.250044928404));
#112314=CARTESIAN_POINT('Ctrl Pts',(-52.1250195665029,1076.38789171826,
505.300938128183));
#112315=CARTESIAN_POINT('Ctrl Pts',(-51.999162401815,1076.38547113493,505.429094455614));
#112316=CARTESIAN_POINT('Ctrl Pts',(-51.9496627855191,1076.38319411869,
505.505057357832));
#112317=CARTESIAN_POINT('Ctrl Pts',(-51.883228099544,1076.37672581559,505.671920978432));
#112318=CARTESIAN_POINT('Ctrl Pts',(-51.8669938531162,1076.37259614805,
505.76116031435));
#112319=CARTESIAN_POINT('Ctrl Pts',(-51.8703596771028,1076.36295358499,
505.941075171903));
#112320=CARTESIAN_POINT('Ctrl Pts',(-51.8900794118279,1076.35753006859,
506.029954351681));
#112321=CARTESIAN_POINT('Ctrl Pts',(-51.9447688812763,1076.34898179335,
506.153163881526));
#112322=CARTESIAN_POINT('Ctrl Pts',(-51.9669056362615,1076.34609765802,
506.19210538115));
#112323=CARTESIAN_POINT('Ctrl Pts',(-52.0439818174159,1076.33746234889,
506.300975951162));
#112324=CARTESIAN_POINT('Ctrl Pts',(-52.1090127195029,1076.33176781271,
506.362586846487));
#112325=CARTESIAN_POINT('Ctrl Pts',(-52.2591523583701,1076.32115888301,
506.457122883992));
#112326=CARTESIAN_POINT('Ctrl Pts',(-52.3428061494639,1076.31634712274,
506.489154634628));
#112327=CARTESIAN_POINT('Ctrl Pts',(-52.4679363166643,1076.31060366373,
506.510524761264));
#112328=CARTESIAN_POINT('Ctrl Pts',(-52.5059754427173,1076.3090377693,506.513735502178));
#112329=CARTESIAN_POINT('Ctrl Pts',(-52.5439991194437,1076.3076507295,506.513735502178));
#112330=CARTESIAN_POINT('Origin',(-66.3937896239306,1067.7251047501,505.798797233579));
#112331=CARTESIAN_POINT('',(-66.3937896239305,1075.74217416993,504.699966097586));
#112332=CARTESIAN_POINT('',(-66.3937896239306,1067.7251047501,504.699966097586));
#112333=CARTESIAN_POINT('Ctrl Pts',(-66.3938922946787,1075.56505891227,
506.897628364774));
#112334=CARTESIAN_POINT('Ctrl Pts',(-66.5377439329708,1075.5553029594,506.897614923805));
#112335=CARTESIAN_POINT('Ctrl Pts',(-66.6803277369447,1075.54793464586,
506.869353627706));
#112336=CARTESIAN_POINT('Ctrl Pts',(-66.9458979690475,1075.53896655866,
506.759593170502));
#112337=CARTESIAN_POINT('Ctrl Pts',(-67.0663498678771,1075.53742419525,
506.679497121772));
#112338=CARTESIAN_POINT('Ctrl Pts',(-67.2695429342651,1075.54039830516,
506.477727005766));
#112339=CARTESIAN_POINT('Ctrl Pts',(-67.3503282205808,1075.54487262748,
506.358150666703));
#112340=CARTESIAN_POINT('Ctrl Pts',(-67.4617465953587,1075.55923551352,
506.094509517608));
#112341=CARTESIAN_POINT('Ctrl Pts',(-67.4911177270138,1075.56899806553,
505.952963071634));
#112342=CARTESIAN_POINT('Ctrl Pts',(-67.4940205904077,1075.59249143215,
505.66594860695));
#112343=CARTESIAN_POINT('Ctrl Pts',(-67.4671709701334,1075.60601842522,
505.523219983919));
#112344=CARTESIAN_POINT('Ctrl Pts',(-67.3868194776427,1075.62770861649,
505.322849447008));
#112345=CARTESIAN_POINT('Ctrl Pts',(-67.3534429135765,1075.63513685526,
505.258707843303));
#112346=CARTESIAN_POINT('Ctrl Pts',(-67.2747200780839,1075.65011148731,
505.138065664204));
#112347=CARTESIAN_POINT('Ctrl Pts',(-67.2295862227784,1075.65762291195,
505.081824883924));
#112348=CARTESIAN_POINT('Ctrl Pts',(-67.0771670909457,1075.68015355567,
504.926015563009));
#112349=CARTESIAN_POINT('Ctrl Pts',(-66.9552034804363,1075.69471965159,
504.842963485428));
#112350=CARTESIAN_POINT('Ctrl Pts',(-66.6864183602497,1075.72108584257,
504.729703518017));
#112351=CARTESIAN_POINT('Ctrl Pts',(-66.5423355880472,1075.7326452051,504.700339722112));
#112352=CARTESIAN_POINT('Ctrl Pts',(-66.2507605417059,1075.75134979152,
504.699599396793));
#112353=CARTESIAN_POINT('Ctrl Pts',(-66.1062000943209,1075.75830783535,
504.72825892625));
#112354=CARTESIAN_POINT('Ctrl Pts',(-65.8376706292063,1075.76667319234,
504.840080292173));
#112355=CARTESIAN_POINT('Ctrl Pts',(-65.7162600264784,1075.76804302978,
504.921657187487));
#112356=CARTESIAN_POINT('Ctrl Pts',(-65.5130971587849,1075.76506869291,
505.126206457029));
#112357=CARTESIAN_POINT('Ctrl Pts',(-65.4329794682159,1075.76081132962,
505.246711156188));
#112358=CARTESIAN_POINT('Ctrl Pts',(-65.3225598718984,1075.74704172745,
505.513900695787));
#112359=CARTESIAN_POINT('Ctrl Pts',(-65.294299520288,1075.73757430082,505.658295646118));
#112360=CARTESIAN_POINT('Ctrl Pts',(-65.2956421914888,1075.71456780327,
505.949730301104));
#112361=CARTESIAN_POINT('Ctrl Pts',(-65.3253509701224,1075.70124560524,
506.093883541034));
#112362=CARTESIAN_POINT('Ctrl Pts',(-65.4101272555891,1075.67978247192,
506.293713601267));
#112363=CARTESIAN_POINT('Ctrl Pts',(-65.4443703142224,1075.67250956308,
506.356589596288));
#112364=CARTESIAN_POINT('Ctrl Pts',(-65.5247093080667,1075.65771823703,
506.475014049654));
#112365=CARTESIAN_POINT('Ctrl Pts',(-65.5706668421235,1075.65023296772,
506.530260184581));
#112366=CARTESIAN_POINT('Ctrl Pts',(-65.72565702693,1075.62758724997,506.683323175303));
#112367=CARTESIAN_POINT('Ctrl Pts',(-65.8491425729377,1075.6127436033,506.76429769867));
#112368=CARTESIAN_POINT('Ctrl Pts',(-66.1148498821844,1075.58616820431,
506.870811005097));
#112369=CARTESIAN_POINT('Ctrl Pts',(-66.2536558097413,1075.57456968708,
506.897641467957));
#112370=CARTESIAN_POINT('Ctrl Pts',(-66.3938922946787,1075.56505891227,
506.897628364774));
#112371=CARTESIAN_POINT('Origin',(-66.3937896239306,1067.7251047501,505.798797233579));
#112372=CARTESIAN_POINT('',(-66.3937896239306,1075.61493016275,506.297628369571));
#112373=CARTESIAN_POINT('',(-66.3937896239315,1075.69533039084,505.299966097586));
#112374=CARTESIAN_POINT('Ctrl Pts',(-66.3937896239305,1075.61493016275,
506.297628369571));
#112375=CARTESIAN_POINT('Ctrl Pts',(-66.3969872526643,1075.61471660334,
506.297628369571));
#112376=CARTESIAN_POINT('Ctrl Pts',(-66.4001864101225,1075.61450543078,
506.2975976233));
#112377=CARTESIAN_POINT('Ctrl Pts',(-66.4686082155845,1075.61004237143,
506.296281008526));
#112378=CARTESIAN_POINT('Ctrl Pts',(-66.5330083204022,1075.60687880481,
506.282243259306));
#112379=CARTESIAN_POINT('Ctrl Pts',(-66.6525296057925,1075.60313393998,
506.230205843174));
#112380=CARTESIAN_POINT('Ctrl Pts',(-66.7065062669411,1075.60257758674,
506.192841425143));
#112381=CARTESIAN_POINT('Ctrl Pts',(-66.7970476739618,1075.60415638336,
506.099526567021));
#112382=CARTESIAN_POINT('Ctrl Pts',(-66.8327242575731,1075.60627324959,
506.044524015442));
#112383=CARTESIAN_POINT('Ctrl Pts',(-66.8810824623255,1075.61291386197,
505.923789671765));
#112384=CARTESIAN_POINT('Ctrl Pts',(-66.8932004913451,1075.61738067694,
505.859208593282));
#112385=CARTESIAN_POINT('Ctrl Pts',(-66.8919947248666,1075.62808638916,
505.728765714233));
#112386=CARTESIAN_POINT('Ctrl Pts',(-66.8785272948644,1075.63423222768,
505.664154900985));
#112387=CARTESIAN_POINT('Ctrl Pts',(-66.8402623969173,1075.64407255818,
505.573936318237));
#112388=CARTESIAN_POINT('Ctrl Pts',(-66.8245795297104,1075.64743432094,
505.545183962969));
#112389=CARTESIAN_POINT('Ctrl Pts',(-66.7878564053252,1075.6542146777,505.49121405238));
#112390=CARTESIAN_POINT('Ctrl Pts',(-66.76690987515,1075.65761753216,505.466115040111));
#112391=CARTESIAN_POINT('Ctrl Pts',(-66.6962780648952,1075.6678554098,505.396612235028));
#112392=CARTESIAN_POINT('Ctrl Pts',(-66.6400176078294,1075.67448591137,
505.359895853247));
#112393=CARTESIAN_POINT('Ctrl Pts',(-66.5195556583078,1075.68618860093,
505.311975903565));
#112394=CARTESIAN_POINT('Ctrl Pts',(-66.4569901306746,1075.69122073777,
505.299966097586));
#112395=CARTESIAN_POINT('Ctrl Pts',(-66.3937896239324,1075.69533039084,
505.299966097586));
#112396=CARTESIAN_POINT('',(-66.3937896239306,1082.7251047501,505.299966097586));
#112397=CARTESIAN_POINT('',(-66.3937896239306,1067.7251047501,505.299966097586));
#112398=CARTESIAN_POINT('Origin',(-66.3937896239306,1082.7251047501,505.798797233579));
#112399=CARTESIAN_POINT('Ctrl Pts',(-66.3937896239324,1075.69533039084,
505.299966097586));
#112400=CARTESIAN_POINT('Ctrl Pts',(-66.393696991604,1075.69533641431,505.299966097586));
#112401=CARTESIAN_POINT('Ctrl Pts',(-66.3936043579098,1075.69534243578,
505.299966123717));
#112402=CARTESIAN_POINT('Ctrl Pts',(-66.3935117228637,1075.69534845529,
505.299966175325));
#112403=CARTESIAN_POINT('Ctrl Pts',(-66.3270385250359,1075.69966794578,
505.300003207775));
#112404=CARTESIAN_POINT('Ctrl Pts',(-66.2611841876149,1075.70288158026,
505.313327059998));
#112405=CARTESIAN_POINT('Ctrl Pts',(-66.1399497147479,1075.7066846604,505.36448891194));
#112406=CARTESIAN_POINT('Ctrl Pts',(-66.0855609170226,1075.70729683034,
505.401234133577));
#112407=CARTESIAN_POINT('Ctrl Pts',(-65.9939189543823,1075.70592073745,
505.493562152881));
#112408=CARTESIAN_POINT('Ctrl Pts',(-65.9575867145451,1075.70394500289,
505.548231953087));
#112409=CARTESIAN_POINT('Ctrl Pts',(-65.907358753142,1075.69755912678,505.669784714922));
#112410=CARTESIAN_POINT('Ctrl Pts',(-65.8945322385433,1075.69315748623,
505.735676699996));
#112411=CARTESIAN_POINT('Ctrl Pts',(-65.8954070785054,1075.68250522403,
505.868595325266));
#112412=CARTESIAN_POINT('Ctrl Pts',(-65.9091428791379,1075.67635739562,
505.934295742771));
#112413=CARTESIAN_POINT('Ctrl Pts',(-65.9481199830954,1075.66650768815,
506.025223447394));
#112414=CARTESIAN_POINT('Ctrl Pts',(-65.9638238820153,1075.6631813765,506.053785225724));
#112415=CARTESIAN_POINT('Ctrl Pts',(-66.0005904751435,1075.65644016903,
506.107484303071));
#112416=CARTESIAN_POINT('Ctrl Pts',(-66.0215782871409,1075.65304063377,
506.132491675586));
#112417=CARTESIAN_POINT('Ctrl Pts',(-66.0926231435377,1075.64273371705,
506.202033754521));
#112418=CARTESIAN_POINT('Ctrl Pts',(-66.1493354797772,1075.63599973081,
506.238743969495));
#112419=CARTESIAN_POINT('Ctrl Pts',(-66.2696390533603,1075.6241684572,506.285932949106));
#112420=CARTESIAN_POINT('Ctrl Pts',(-66.3314235794298,1075.61909539169,
506.297628369571));
#112421=CARTESIAN_POINT('Ctrl Pts',(-66.3937896239305,1075.61493016275,
506.297628369571));
#112422=CARTESIAN_POINT('Origin',(-80.0774492048019,1067.7251047501,502.902003229021));
#112423=CARTESIAN_POINT('',(-80.0774492048019,1074.90384407591,501.811462480293));
#112424=CARTESIAN_POINT('',(-80.0774492048019,1067.7251047501,501.811462480293));
#112425=CARTESIAN_POINT('Ctrl Pts',(-80.0775556651706,1074.69741082091,
503.992543972553));
#112426=CARTESIAN_POINT('Ctrl Pts',(-80.2203939055204,1074.68335242624,
503.992530028451));
#112427=CARTESIAN_POINT('Ctrl Pts',(-80.3620774576235,1074.67206368809,
503.964453024161));
#112428=CARTESIAN_POINT('Ctrl Pts',(-80.6255874212788,1074.65654223953,
503.855395313021));
#112429=CARTESIAN_POINT('Ctrl Pts',(-80.7449440196709,1074.6523996033,503.776028182163));
#112430=CARTESIAN_POINT('Ctrl Pts',(-80.9461808540607,1074.65181168185,
503.576243475235));
#112431=CARTESIAN_POINT('Ctrl Pts',(-81.0261661284762,1074.6553392513,503.458044660765));
#112432=CARTESIAN_POINT('Ctrl Pts',(-81.1367694022258,1074.66961052421,
503.197374581285));
#112433=CARTESIAN_POINT('Ctrl Pts',(-81.1660809474431,1074.68023672022,
503.057438861993));
#112434=CARTESIAN_POINT('Ctrl Pts',(-81.1697363998317,1074.70723981908,
502.773232310702));
#112435=CARTESIAN_POINT('Ctrl Pts',(-81.1435079619441,1074.72340672621,
502.631697216134));
#112436=CARTESIAN_POINT('Ctrl Pts',(-81.0368996889042,1074.75947744905,
502.363331420954));
#112437=CARTESIAN_POINT('Ctrl Pts',(-80.9560413553554,1074.77912227993,
502.239633765539));
#112438=CARTESIAN_POINT('Ctrl Pts',(-80.8032700801437,1074.80856466224,
502.084978808424));
#112439=CARTESIAN_POINT('Ctrl Pts',(-80.7484058314527,1074.81817637982,
502.039352859407));
#112440=CARTESIAN_POINT('Ctrl Pts',(-80.5697774790657,1074.84681222231,
501.918231233593));
#112441=CARTESIAN_POINT('Ctrl Pts',(-80.4349776991283,1074.86505126372,
501.861586297577));
#112442=CARTESIAN_POINT('Ctrl Pts',(-80.1513251869895,1074.89748746044,
501.804428811488));
#112443=CARTESIAN_POINT('Ctrl Pts',(-80.0052807514068,1074.91138774107,
501.804252305455));
#112444=CARTESIAN_POINT('Ctrl Pts',(-79.7225931968404,1074.93295007086,
501.86088327094));
#112445=CARTESIAN_POINT('Ctrl Pts',(-79.5887155205554,1074.94045724399,
501.916564990387));
#112446=CARTESIAN_POINT('Ctrl Pts',(-79.351804312291,1074.94814247841,502.075700378908));
#112447=CARTESIAN_POINT('Ctrl Pts',(-79.2507353332974,1074.94835107219,
502.176824798993));
#112448=CARTESIAN_POINT('Ctrl Pts',(-79.0927212169076,1074.94152693975,
502.412358619853));
#112449=CARTESIAN_POINT('Ctrl Pts',(-79.0374909897089,1074.93454479757,
502.54445607692));
#112450=CARTESIAN_POINT('Ctrl Pts',(-78.9800102013773,1074.91397284501,
502.825200418115));
#112451=CARTESIAN_POINT('Ctrl Pts',(-78.9795713602911,1074.90044714542,
502.971264433429));
#112452=CARTESIAN_POINT('Ctrl Pts',(-79.0355385610595,1074.86860672502,
503.255142309305));
#112453=CARTESIAN_POINT('Ctrl Pts',(-79.0915985444302,1074.8505849915,503.390141249739));
#112454=CARTESIAN_POINT('Ctrl Pts',(-79.2534617935822,1074.81229849349,
503.631076731761));
#112455=CARTESIAN_POINT('Ctrl Pts',(-79.3581097527856,1074.79237972676,
503.73449679173));
#112456=CARTESIAN_POINT('Ctrl Pts',(-79.602566463531,1074.75337675315,503.894598889858));
#112457=CARTESIAN_POINT('Ctrl Pts',(-79.7402559800462,1074.73467195852,
503.949457322082));
#112458=CARTESIAN_POINT('Ctrl Pts',(-79.9483999920536,1074.71066669124,
503.986804683043));
#112459=CARTESIAN_POINT('Ctrl Pts',(-80.0128883498499,1074.70377549355,
503.992550285482));
#112460=CARTESIAN_POINT('Ctrl Pts',(-80.0775556651706,1074.69741082091,
503.992543972553));
#112461=CARTESIAN_POINT('Origin',(-80.0774492048019,1067.7251047501,502.902003229021));
#112462=CARTESIAN_POINT('',(-80.077449204802,1074.75547652074,503.39254397775));
#112463=CARTESIAN_POINT('',(-80.0774492048019,1074.84832662855,502.411462480293));
#112464=CARTESIAN_POINT('Ctrl Pts',(-80.077449204802,1074.75547652074,503.39254397775));
#112465=CARTESIAN_POINT('Ctrl Pts',(-80.0804386977064,1074.75518491478,
503.39254397775));
#112466=CARTESIAN_POINT('Ctrl Pts',(-80.0834296668131,1074.75489575047,
503.392516649627));
#112467=CARTESIAN_POINT('Ctrl Pts',(-80.1505817358878,1074.74846175269,
503.391288156812));
#112468=CARTESIAN_POINT('Ctrl Pts',(-80.2139925467697,1074.74357852497,
503.377534158872));
#112469=CARTESIAN_POINT('Ctrl Pts',(-80.3315251714612,1074.73697045175,
503.326437741991));
#112470=CARTESIAN_POINT('Ctrl Pts',(-80.3845436293575,1074.73528448238,
503.289821015878));
#112471=CARTESIAN_POINT('Ctrl Pts',(-80.4734725583864,1074.73532796221,
503.198397642156));
#112472=CARTESIAN_POINT('Ctrl Pts',(-80.5085290514065,1074.73704629545,
503.144580661257));
#112473=CARTESIAN_POINT('Ctrl Pts',(-80.5562437403426,1074.74367979716,
503.026372118594));
#112474=CARTESIAN_POINT('Ctrl Pts',(-80.5683167302978,1074.74854254875,
502.963124043407));
#112475=CARTESIAN_POINT('Ctrl Pts',(-80.5676464698705,1074.76081522022,
502.83512323168));
#112476=CARTESIAN_POINT('Ctrl Pts',(-80.5546684257742,1074.76812935686,
502.771608449677));
#112477=CARTESIAN_POINT('Ctrl Pts',(-80.5045169611936,1074.78438363024,
502.65188725358));
#112478=CARTESIAN_POINT('Ctrl Pts',(-80.4672435467254,1074.79320189596,
502.597053187483));
#112479=CARTESIAN_POINT('Ctrl Pts',(-80.3735738883454,1074.81093511663,
502.505500458746));
#112480=CARTESIAN_POINT('Ctrl Pts',(-80.318121606227,1074.81968358517,502.469576653714));
#112481=CARTESIAN_POINT('Ctrl Pts',(-80.2000500020039,1074.83544850608,
502.423073813707));
#112482=CARTESIAN_POINT('Ctrl Pts',(-80.1390813375835,1074.84240529864,
502.411464629318));
#112483=CARTESIAN_POINT('Ctrl Pts',(-80.0774663116128,1074.84832498503,
502.411462480594));
#112484=CARTESIAN_POINT('Ctrl Pts',(-80.0774606093383,1074.84832553288,
502.411462480395));
#112485=CARTESIAN_POINT('Ctrl Pts',(-80.0774549070681,1074.84832608072,
502.411462480293));
#112486=CARTESIAN_POINT('Ctrl Pts',(-80.0774492048019,1074.84832662855,
502.411462480293));
#112487=CARTESIAN_POINT('',(-80.0774492048019,1082.7251047501,502.411462480293));
#112488=CARTESIAN_POINT('',(-80.0774492048019,1067.7251047501,502.411462480293));
#112489=CARTESIAN_POINT('Origin',(-80.0774492048019,1082.7251047501,502.902003229021));
#112490=CARTESIAN_POINT('Ctrl Pts',(-80.0774492048019,1074.84832662855,
502.411462480293));
#112491=CARTESIAN_POINT('Ctrl Pts',(-80.0127825915629,1074.8545392838,502.411462480293));
#112492=CARTESIAN_POINT('Ctrl Pts',(-79.9486491232316,1074.8594902095,502.424249728139));
#112493=CARTESIAN_POINT('Ctrl Pts',(-79.8299151493609,1074.86623401415,
502.473724313552));
#112494=CARTESIAN_POINT('Ctrl Pts',(-79.7763608843544,1074.86801171817,
502.509508066976));
#112495=CARTESIAN_POINT('Ctrl Pts',(-79.686013081107,1074.86823282458,502.599566153324));
#112496=CARTESIAN_POINT('Ctrl Pts',(-79.6501060045928,1074.86668059872,
502.652887070509));
#112497=CARTESIAN_POINT('Ctrl Pts',(-79.6005542127742,1074.86041180784,
502.770495814349));
#112498=CARTESIAN_POINT('Ctrl Pts',(-79.5875240977248,1074.85574220163,
502.833649874922));
#112499=CARTESIAN_POINT('Ctrl Pts',(-79.5863199589662,1074.84372459065,
502.962872637271));
#112500=CARTESIAN_POINT('Ctrl Pts',(-79.5988104681922,1074.83643155972,
503.027665799191));
#112501=CARTESIAN_POINT('Ctrl Pts',(-79.6483757697716,1074.82025748681,
503.148603427903));
#112502=CARTESIAN_POINT('Ctrl Pts',(-79.685057162547,1074.81152653033,503.203552594586));
#112503=CARTESIAN_POINT('Ctrl Pts',(-79.777881940359,1074.79379699465,503.295948849467));
#112504=CARTESIAN_POINT('Ctrl Pts',(-79.8332183009218,1074.78496473368,
503.332462500812));
#112505=CARTESIAN_POINT('Ctrl Pts',(-79.952341812871,1074.76882355205,503.380454685222));
#112506=CARTESIAN_POINT('Ctrl Pts',(-80.0145689753705,1074.76161008594,
503.39254397775));
#112507=CARTESIAN_POINT('Ctrl Pts',(-80.077449204802,1074.75547652074,503.39254397775));
#112508=CARTESIAN_POINT('Origin',(-22.5035000139863,1067.7251047501,511.305124859599));
#112509=CARTESIAN_POINT('',(-22.5035000140048,1076.70430247523,509.826821727406));
#112510=CARTESIAN_POINT('',(-22.5035000139863,1067.7251047501,509.826821727406));
#112511=CARTESIAN_POINT('Ctrl Pts',(-22.5035327361191,1076.6298518624,512.78342799143));
#112512=CARTESIAN_POINT('Ctrl Pts',(-22.697188336794,1076.62822043967,512.783423704877));
#112513=CARTESIAN_POINT('Ctrl Pts',(-22.8889703125145,1076.62783250898,
512.745366885901));
#112514=CARTESIAN_POINT('Ctrl Pts',(-23.2464818143271,1076.62962273074,
512.597668356197));
#112515=CARTESIAN_POINT('Ctrl Pts',(-23.4088197788964,1076.63177508635,
512.489640658617));
#112516=CARTESIAN_POINT('Ctrl Pts',(-23.6826202279391,1076.63815172445,
512.217423455911));
#112517=CARTESIAN_POINT('Ctrl Pts',(-23.7914950365478,1076.6423068606,512.055904652138));
#112518=CARTESIAN_POINT('Ctrl Pts',(-23.9411046906667,1076.65176378763,
511.700044378558));
#112519=CARTESIAN_POINT('Ctrl Pts',(-23.9803420008756,1076.65696882156,
511.509089417913));
#112520=CARTESIAN_POINT('Ctrl Pts',(-23.9824739336125,1076.66484283965,
511.219425695112));
#112521=CARTESIAN_POINT('Ctrl Pts',(-23.9737183561377,1076.6674612293,511.123008031829));
#112522=CARTESIAN_POINT('Ctrl Pts',(-23.9375214641077,1076.6725935507,510.933245449221));
#112523=CARTESIAN_POINT('Ctrl Pts',(-23.9101636017548,1076.67509510596,
510.840355902925));
#112524=CARTESIAN_POINT('Ctrl Pts',(-23.8004027713136,1076.68237077316,
510.568997838307));
#112525=CARTESIAN_POINT('Ctrl Pts',(-23.6914150010189,1076.68675194435,
510.403622117564));
#112526=CARTESIAN_POINT('Ctrl Pts',(-23.4161126676759,1076.69419979021,
510.12592921612));
#112527=CARTESIAN_POINT('Ctrl Pts',(-23.2528652196348,1076.69720855228,
510.016007307325));
#112528=CARTESIAN_POINT('Ctrl Pts',(-22.8927823991851,1076.70183240506,
509.865689241871));
#112529=CARTESIAN_POINT('Ctrl Pts',(-22.6994323131464,1076.70340777433,
509.826906152296));
#112530=CARTESIAN_POINT('Ctrl Pts',(-22.3082658034494,1076.70519399336,
509.826737328439));
#112531=CARTESIAN_POINT('Ctrl Pts',(-22.1143143021181,1076.70538769376,
509.865582884672));
#112532=CARTESIAN_POINT('Ctrl Pts',(-21.7531812058628,1076.70439475941,
510.016471427184));
#112533=CARTESIAN_POINT('Ctrl Pts',(-21.5895165689669,1076.70321779961,
510.126890158071));
#112534=CARTESIAN_POINT('Ctrl Pts',(-21.3150766651475,1076.69940842177,
510.404560234275));
#112535=CARTESIAN_POINT('Ctrl Pts',(-21.2068326793722,1076.69681002284,
510.568909243009));
#112536=CARTESIAN_POINT('Ctrl Pts',(-21.0600685816595,1076.69014662445,
510.930764109334));
#112537=CARTESIAN_POINT('Ctrl Pts',(-21.0232572846915,1076.68613413807,
511.12481342175));
#112538=CARTESIAN_POINT('Ctrl Pts',(-21.0272970997305,1076.67695082874,
511.516256004342));
#112539=CARTESIAN_POINT('Ctrl Pts',(-21.0682305948924,1076.67186587121,
511.709780751801));
#112540=CARTESIAN_POINT('Ctrl Pts',(-21.2224183718107,1076.66134236978,
512.067928084707));
#112541=CARTESIAN_POINT('Ctrl Pts',(-21.3335069705477,1076.65601271149,
512.229331198209));
#112542=CARTESIAN_POINT('Ctrl Pts',(-21.6117872969745,1076.64600420641,
512.500090524125));
#112543=CARTESIAN_POINT('Ctrl Pts',(-21.7763186727178,1076.64142975664,
512.606782500528));
#112544=CARTESIAN_POINT('Ctrl Pts',(-22.1307308239509,1076.63413695962,
512.747857579243));
#112545=CARTESIAN_POINT('Ctrl Pts',(-22.3162777347941,1076.63142936424,
512.783432136306));
#112546=CARTESIAN_POINT('Ctrl Pts',(-22.5035327361191,1076.6298518624,512.78342799143));
#112547=CARTESIAN_POINT('Origin',(-22.5035000139863,1067.7251047501,511.305124859599));
#112548=CARTESIAN_POINT('',(-22.5035000139863,1076.64871264505,512.183427991792));
#112549=CARTESIAN_POINT('',(-22.5035000139663,1076.69297254634,510.426821727406));
#112550=CARTESIAN_POINT('Ctrl Pts',(-22.5035000139863,1076.64871264505,
512.183427991792));
#112551=CARTESIAN_POINT('Ctrl Pts',(-22.6136921936282,1076.64786711526,
512.183427991792));
#112552=CARTESIAN_POINT('Ctrl Pts',(-22.7229531368515,1076.64763898538,
512.162690172106));
#112553=CARTESIAN_POINT('Ctrl Pts',(-22.9324051162973,1076.64847486863,
512.080139744173));
#112554=CARTESIAN_POINT('Ctrl Pts',(-23.0299618966429,1076.64958430376,
512.017475159969));
#112555=CARTESIAN_POINT('Ctrl Pts',(-23.195370245027,1076.65297330517,511.858212204119));
#112556=CARTESIAN_POINT('Ctrl Pts',(-23.2616434659143,1076.65521736704,
511.763169348596));
#112557=CARTESIAN_POINT('Ctrl Pts',(-23.3539103754164,1076.66043671566,
511.552927523711));
#112558=CARTESIAN_POINT('Ctrl Pts',(-23.3789889237328,1076.66335970471,
511.439738840843));
#112559=CARTESIAN_POINT('Ctrl Pts',(-23.3828746159423,1076.66789018712,
511.267554586315));
#112560=CARTESIAN_POINT('Ctrl Pts',(-23.3785409393564,1076.66941398011,
511.210179675387));
#112561=CARTESIAN_POINT('Ctrl Pts',(-23.3587389585038,1076.67244001584,
511.09708961534));
#112562=CARTESIAN_POINT('Ctrl Pts',(-23.3433162721398,1076.67393497921,
511.041645943522));
#112563=CARTESIAN_POINT('Ctrl Pts',(-23.2803642688379,1076.67835615271,
510.878995148548));
#112564=CARTESIAN_POINT('Ctrl Pts',(-23.216753876109,1076.6811106595,510.779409748454));
#112565=CARTESIAN_POINT('Ctrl Pts',(-23.0546047170834,1076.68593465301,
510.611387941601));
#112566=CARTESIAN_POINT('Ctrl Pts',(-22.9578292528528,1076.68796173538,
510.54448344382));
#112567=CARTESIAN_POINT('Ctrl Pts',(-22.7437560177297,1076.6911466657,510.452317512047));
#112568=CARTESIAN_POINT('Ctrl Pts',(-22.6285772038153,1076.69227539346,
510.427992582682));
#112569=CARTESIAN_POINT('Ctrl Pts',(-22.5091734568623,1076.69294175239,
510.426835467202));
#112570=CARTESIAN_POINT('Ctrl Pts',(-22.5063364099955,1076.69295729554,
510.426821727405));
#112571=CARTESIAN_POINT('Ctrl Pts',(-22.5035000139464,1076.69297254634,
510.426821727406));
#112572=CARTESIAN_POINT('',(-22.5035000139863,1082.7251047501,510.426821727406));
#112573=CARTESIAN_POINT('',(-22.5035000139863,1067.7251047501,510.426821727406));
#112574=CARTESIAN_POINT('Origin',(-22.5035000139863,1082.7251047501,511.305124859599));
#112575=CARTESIAN_POINT('Ctrl Pts',(-22.5035000139464,1076.69297254634,
510.426821727406));
#112576=CARTESIAN_POINT('Ctrl Pts',(-22.389645575796,1076.69358472169,510.426821727411));
#112577=CARTESIAN_POINT('Ctrl Pts',(-22.2768397969015,1076.69372982667,
510.448960806448));
#112578=CARTESIAN_POINT('Ctrl Pts',(-22.0634032383318,1076.69307529407,
510.536140253258));
#112579=CARTESIAN_POINT('Ctrl Pts',(-21.9652822146936,1076.69225884732,
510.601319054443));
#112580=CARTESIAN_POINT('Ctrl Pts',(-21.8003577505346,1076.68967204169,
510.766074764882));
#112581=CARTESIAN_POINT('Ctrl Pts',(-21.735149768211,1076.68792596669,510.863968325622));
#112582=CARTESIAN_POINT('Ctrl Pts',(-21.6493793336339,1076.68373279841,
511.073003965486));
#112583=CARTESIAN_POINT('Ctrl Pts',(-21.6271245598466,1076.68136863704,
511.181166429725));
#112584=CARTESIAN_POINT('Ctrl Pts',(-21.6253166699448,1076.6787531034,511.290619472025));
#112585=CARTESIAN_POINT('Ctrl Pts',(-21.6243587796215,1076.67736729205,
511.348611947101));
#112586=CARTESIAN_POINT('Ctrl Pts',(-21.6291477183368,1076.67592112488,
511.406555672307));
#112587=CARTESIAN_POINT('Ctrl Pts',(-21.6499798988723,1076.67295937525,
511.520115905184));
#112588=CARTESIAN_POINT('Ctrl Pts',(-21.6658677631083,1076.6714516809,511.57547613968));
#112589=CARTESIAN_POINT('Ctrl Pts',(-21.729513563702,1076.66688656265,511.735976408328));
#112590=CARTESIAN_POINT('Ctrl Pts',(-21.7926384809357,1076.66383645352,
511.833674838728));
#112591=CARTESIAN_POINT('Ctrl Pts',(-21.9530348133738,1076.65814954945,
511.999162481131));
#112592=CARTESIAN_POINT('Ctrl Pts',(-22.048766413592,1076.65557036805,512.065336018375));
#112593=CARTESIAN_POINT('Ctrl Pts',(-22.2602774764295,1076.65135643461,
512.156907125427));
#112594=CARTESIAN_POINT('Ctrl Pts',(-22.3739937884222,1076.64976462194,
512.181436332894));
#112595=CARTESIAN_POINT('Ctrl Pts',(-22.4939718080278,1076.64878689139,
512.183389243752));
#112596=CARTESIAN_POINT('Ctrl Pts',(-22.4987367810559,1076.64874919442,
512.183427991792));
#112597=CARTESIAN_POINT('Ctrl Pts',(-22.5035000139863,1076.64871264505,
512.183427991792));
#112598=CARTESIAN_POINT('Origin',(-34.5096048204688,1067.7251047501,514.987993850267));
#112599=CARTESIAN_POINT('',(-34.5096048204686,1076.41851054042,513.712549729131));
#112600=CARTESIAN_POINT('',(-34.5096048204688,1067.7251047501,513.712549729131));
#112601=CARTESIAN_POINT('Ctrl Pts',(-34.510210550676,1076.26444406336,516.263437827568));
#112602=CARTESIAN_POINT('Ctrl Pts',(-34.6770761418107,1076.26029120131,
516.263358580238));
#112603=CARTESIAN_POINT('Ctrl Pts',(-34.8423390931997,1076.25829883923,
516.230534091237));
#112604=CARTESIAN_POINT('Ctrl Pts',(-35.1505137202821,1076.25893043407,
516.103217369855));
#112605=CARTESIAN_POINT('Ctrl Pts',(-35.2904555944617,1076.26153711202,
516.010118411505));
#112606=CARTESIAN_POINT('Ctrl Pts',(-35.5266628802956,1076.27094966102,
515.775442346978));
#112607=CARTESIAN_POINT('Ctrl Pts',(-35.6206174798617,1076.27766188471,
515.636136749945));
#112608=CARTESIAN_POINT('Ctrl Pts',(-35.7498704340647,1076.29416258726,
515.329053401729));
#112609=CARTESIAN_POINT('Ctrl Pts',(-35.7837744926969,1076.30379557645,
515.164160424993));
#112610=CARTESIAN_POINT('Ctrl Pts',(-35.7862560111193,1076.32454585444,
514.830372499115));
#112611=CARTESIAN_POINT('Ctrl Pts',(-35.7546458658456,1076.33546533049,
514.664655541728));
#112612=CARTESIAN_POINT('Ctrl Pts',(-35.6284501149868,1076.3571975243,514.352646635918));
#112613=CARTESIAN_POINT('Ctrl Pts',(-35.534206291959,1076.36779288197,514.209727796389));
#112614=CARTESIAN_POINT('Ctrl Pts',(-35.2960069591467,1076.38707298587,
513.9697917652));
#112615=CARTESIAN_POINT('Ctrl Pts',(-35.1546820135756,1076.39558365587,
513.874853901345));
#112616=CARTESIAN_POINT('Ctrl Pts',(-34.8429315588452,1076.40962934384,
513.745341652921));
#112617=CARTESIAN_POINT('Ctrl Pts',(-34.6755586727011,1076.41502554586,
513.712146813909));
#112618=CARTESIAN_POINT('Ctrl Pts',(-34.3368750129064,1076.4221382511,513.712961563743));
#112619=CARTESIAN_POINT('Ctrl Pts',(-34.1689685251534,1076.42377274472,
513.74721915866));
#112620=CARTESIAN_POINT('Ctrl Pts',(-33.8564683098246,1076.42306559179,
513.879418325012));
#112621=CARTESIAN_POINT('Ctrl Pts',(-33.7150198072083,1076.42073260849,
513.975993466824));
#112622=CARTESIAN_POINT('Ctrl Pts',(-33.4786776417656,1076.412295967,514.218271328925));
#112623=CARTESIAN_POINT('Ctrl Pts',(-33.3859622956867,1076.40628728116,
514.361357255944));
#112624=CARTESIAN_POINT('Ctrl Pts',(-33.2616665770459,1076.39116443452,
514.675143622838));
#112625=CARTESIAN_POINT('Ctrl Pts',(-33.2312922293419,1076.38219590285,
514.842728733327));
#112626=CARTESIAN_POINT('Ctrl Pts',(-33.2358846722379,1076.36736587868,
515.093961251048));
#112627=CARTESIAN_POINT('Ctrl Pts',(-33.2454281379424,1076.36228606157,
515.176265123999));
#112628=CARTESIAN_POINT('Ctrl Pts',(-33.2803741619054,1076.35183445363,
515.338193358098));
#112629=CARTESIAN_POINT('Ctrl Pts',(-33.3057626507355,1076.34648603911,
515.417423922129));
#112630=CARTESIAN_POINT('Ctrl Pts',(-33.4057693169067,1076.33011967124,
515.649021362422));
#112631=CARTESIAN_POINT('Ctrl Pts',(-33.5031513467196,1076.31914258526,
515.789539701725));
#112632=CARTESIAN_POINT('Ctrl Pts',(-33.7458423042442,1076.29869782582,
516.023121450383));
#112633=CARTESIAN_POINT('Ctrl Pts',(-33.8883025592264,1076.28941582096,
516.114425004076));
#112634=CARTESIAN_POINT('Ctrl Pts',(-34.1927603496154,1076.27427812612,
516.233688459787));
#112635=CARTESIAN_POINT('Ctrl Pts',(-34.350758296486,1076.26841242621,516.263513554176));
#112636=CARTESIAN_POINT('Ctrl Pts',(-34.510210550676,1076.26444406336,516.263437827568));
#112637=CARTESIAN_POINT('Origin',(-34.5096048204688,1067.7251047501,514.987993850267));
#112638=CARTESIAN_POINT('',(-34.5096048204688,1076.30335139737,515.663437971403));
#112639=CARTESIAN_POINT('',(-34.5096048204687,1076.38494400861,514.312549729131));
#112640=CARTESIAN_POINT('Ctrl Pts',(-34.5096048204688,1076.30335139737,
515.663437971403));
#112641=CARTESIAN_POINT('Ctrl Pts',(-34.5147607200677,1076.3032273638,515.663437971403));
#112642=CARTESIAN_POINT('Ctrl Pts',(-34.5199192890106,1076.30310696305,
515.663378936453));
#112643=CARTESIAN_POINT('Ctrl Pts',(-34.6133832608504,1076.30099273748,
515.66123707454));
#112644=CARTESIAN_POINT('Ctrl Pts',(-34.700448866802,1076.30011145474,515.641911819858));
#112645=CARTESIAN_POINT('Ctrl Pts',(-34.8621113822095,1076.30069909558,
515.57087383221));
#112646=CARTESIAN_POINT('Ctrl Pts',(-34.9351405015941,1076.30215908264,
515.519899188168));
#112647=CARTESIAN_POINT('Ctrl Pts',(-35.0575110263185,1076.30721945871,
515.392736761286));
#112648=CARTESIAN_POINT('Ctrl Pts',(-35.1056388675218,1076.31077147118,
515.317765781211));
#112649=CARTESIAN_POINT('Ctrl Pts',(-35.170418690475,1076.31946619841,515.153431373832));
#112650=CARTESIAN_POINT('Ctrl Pts',(-35.1863680819962,1076.32452759051,
515.065619221493));
#112651=CARTESIAN_POINT('Ctrl Pts',(-35.1842608595915,1076.3327125846,514.933044487346));
#112652=CARTESIAN_POINT('Ctrl Pts',(-35.1792178233148,1076.33552155445,
514.889009034933));
#112653=CARTESIAN_POINT('Ctrl Pts',(-35.160605440651,1076.34121170766,514.802586854367));
#112654=CARTESIAN_POINT('Ctrl Pts',(-35.1470845835084,1076.34407935344,
514.760404110216));
#112655=CARTESIAN_POINT('Ctrl Pts',(-35.0938308440773,1076.35272825597,
514.637285988837));
#112656=CARTESIAN_POINT('Ctrl Pts',(-35.0419779334543,1076.3583648964,514.562668436976));
#112657=CARTESIAN_POINT('Ctrl Pts',(-34.9122336573852,1076.36866166981,
514.438295951173));
#112658=CARTESIAN_POINT('Ctrl Pts',(-34.8356972543447,1076.37322379078,
514.389701805251));
#112659=CARTESIAN_POINT('Ctrl Pts',(-34.6746757044643,1076.38041569092,
514.327831209519));
#112660=CARTESIAN_POINT('Ctrl Pts',(-34.5926654537101,1076.38310991803,
514.312588592663));
#112661=CARTESIAN_POINT('Ctrl Pts',(-34.509921460243,1076.38493702107,514.312549803324));
#112662=CARTESIAN_POINT('Ctrl Pts',(-34.5098159124342,1076.38493935172,
514.312549753845));
#112663=CARTESIAN_POINT('Ctrl Pts',(-34.5097103658399,1076.38494168089,
514.312549729131));
#112664=CARTESIAN_POINT('Ctrl Pts',(-34.5096048204686,1076.38494400861,
514.312549729131));
#112665=CARTESIAN_POINT('',(-34.5096048204688,1082.7251047501,514.312549729131));
#112666=CARTESIAN_POINT('',(-34.5096048204688,1067.7251047501,514.312549729131));
#112667=CARTESIAN_POINT('Origin',(-34.5096048204688,1082.7251047501,514.987993850267));
#112668=CARTESIAN_POINT('Ctrl Pts',(-34.5096048204686,1076.38494400861,
514.312549729131));
#112669=CARTESIAN_POINT('Ctrl Pts',(-34.4195797209484,1076.38692943473,
514.312549729131));
#112670=CARTESIAN_POINT('Ctrl Pts',(-34.3304444186114,1076.38785074114,
514.330548069844));
#112671=CARTESIAN_POINT('Ctrl Pts',(-34.1643896087766,1076.38747560109,
514.400478078721));
#112672=CARTESIAN_POINT('Ctrl Pts',(-34.0891738841783,1076.38618084193,
514.451728079472));
#112673=CARTESIAN_POINT('Ctrl Pts',(-33.963441665068,1076.38150815206,514.580546241006));
#112674=CARTESIAN_POINT('Ctrl Pts',(-33.9141407280796,1076.37818083265,
514.656755276528));
#112675=CARTESIAN_POINT('Ctrl Pts',(-33.848269512731,1076.36987453135,514.823899897506));
#112676=CARTESIAN_POINT('Ctrl Pts',(-33.832345532267,1076.36497759429,514.913161534974));
#112677=CARTESIAN_POINT('Ctrl Pts',(-33.8352940715305,1076.35696281089,
515.046819095554));
#112678=CARTESIAN_POINT('Ctrl Pts',(-33.8405471527631,1076.35423184587,
515.090543327369));
#112679=CARTESIAN_POINT('Ctrl Pts',(-33.8594872938482,1076.34864452046,
515.176435539951));
#112680=CARTESIAN_POINT('Ctrl Pts',(-33.8731482725201,1076.3458010522,515.218397487686));
#112681=CARTESIAN_POINT('Ctrl Pts',(-33.9267185940827,1076.33714899981,
515.340841430359));
#112682=CARTESIAN_POINT('Ctrl Pts',(-33.9786358918692,1076.33140337561,
515.415000511813));
#112683=CARTESIAN_POINT('Ctrl Pts',(-34.1076721876445,1076.32078808864,
515.538020849947));
#112684=CARTESIAN_POINT('Ctrl Pts',(-34.1832562655626,1076.31601221174,
515.585980243906));
#112685=CARTESIAN_POINT('Ctrl Pts',(-34.3437014148138,1076.30830828351,
515.648028036408));
#112686=CARTESIAN_POINT('Ctrl Pts',(-34.4263047253469,1076.30535531691,
515.663437971403));
#112687=CARTESIAN_POINT('Ctrl Pts',(-34.5096048204688,1076.30335139737,
515.663437971403));
#112688=CARTESIAN_POINT('Origin',(-48.0649554680751,1067.7251047501,517.828896105943));
#112689=CARTESIAN_POINT('',(-48.064955468075,1075.7548763624,516.73006496995));
#112690=CARTESIAN_POINT('',(-48.0649554680751,1067.7251047501,516.73006496995));
#112691=CARTESIAN_POINT('Ctrl Pts',(-48.0649893420775,1075.55153228081,
518.927727241413));
#112692=CARTESIAN_POINT('Ctrl Pts',(-48.2084938936629,1075.54445758504,
518.927722817555));
#112693=CARTESIAN_POINT('Ctrl Pts',(-48.3506973821094,1075.54011567547,
518.899606749943));
#112694=CARTESIAN_POINT('Ctrl Pts',(-48.6158197749301,1075.53747767521,
518.79037881918));
#112695=CARTESIAN_POINT('Ctrl Pts',(-48.7361648149422,1075.5391837126,518.710576143554));
#112696=CARTESIAN_POINT('Ctrl Pts',(-48.9395756994896,1075.54841917822,
518.509307741398));
#112697=CARTESIAN_POINT('Ctrl Pts',(-49.0205871483468,1075.55586065419,
518.389803671339));
#112698=CARTESIAN_POINT('Ctrl Pts',(-49.1325649150761,1075.5754767029,518.126018496399));
#112699=CARTESIAN_POINT('Ctrl Pts',(-49.1621703363378,1075.58748310855,
517.984173555892));
#112700=CARTESIAN_POINT('Ctrl Pts',(-49.1652837174281,1075.61442205228,
517.69652035456));
#112701=CARTESIAN_POINT('Ctrl Pts',(-49.1384171214939,1075.62911403942,
517.553423285889));
#112702=CARTESIAN_POINT('Ctrl Pts',(-49.0579586152795,1075.65158960913,
517.352929660374));
#112703=CARTESIAN_POINT('Ctrl Pts',(-49.0246954806973,1075.65909376488,
517.28898935585));
#112704=CARTESIAN_POINT('Ctrl Pts',(-48.9057044795966,1075.68157591868,
517.106486232892));
#112705=CARTESIAN_POINT('Ctrl Pts',(-48.8023667811879,1075.69607284841,
517.001241563726));
#112706=CARTESIAN_POINT('Ctrl Pts',(-48.5609641233725,1075.72224327897,
516.837651228932));
#112707=CARTESIAN_POINT('Ctrl Pts',(-48.4254097032791,1075.73367717674,
516.780685382225));
#112708=CARTESIAN_POINT('Ctrl Pts',(-48.1395762712534,1075.75208870326,
516.72294128722));
#112709=CARTESIAN_POINT('Ctrl Pts',(-47.9921652529731,1075.75888045524,
516.722789674877));
#112710=CARTESIAN_POINT('Ctrl Pts',(-47.7069256019333,1075.76688907848,
516.779981637933));
#112711=CARTESIAN_POINT('Ctrl Pts',(-47.5719153765225,1075.76807339262,
516.836257764457));
#112712=CARTESIAN_POINT('Ctrl Pts',(-47.3326842943825,1075.76473349722,
516.997162265414));
#112713=CARTESIAN_POINT('Ctrl Pts',(-47.2305532509364,1075.76029878756,
517.099697161617));
#112714=CARTESIAN_POINT('Ctrl Pts',(-47.0700490322263,1075.74619951358,
517.340164075618));
#112715=CARTESIAN_POINT('Ctrl Pts',(-47.0141195650448,1075.73658401839,
517.476247390196));
#112716=CARTESIAN_POINT('Ctrl Pts',(-46.9584863513016,1075.71333331429,
517.762313849099));
#112717=CARTESIAN_POINT('Ctrl Pts',(-46.9594505166007,1075.69991724618,
517.909490060293));
#112718=CARTESIAN_POINT('Ctrl Pts',(-47.0035391842712,1075.67836579534,
518.122033215604));
#112719=CARTESIAN_POINT('Ctrl Pts',(-47.0248343869156,1075.67107227863,
518.190389843968));
#112720=CARTESIAN_POINT('Ctrl Pts',(-47.0804823842841,1075.65625767349,
518.322234520378));
#112721=CARTESIAN_POINT('Ctrl Pts',(-47.1147586064389,1075.64876984785,
518.385399115621));
#112722=CARTESIAN_POINT('Ctrl Pts',(-47.2368435396587,1075.62614696949,
518.565790955365));
#112723=CARTESIAN_POINT('Ctrl Pts',(-47.3421142764355,1075.61135807081,
518.669330549812));
#112724=CARTESIAN_POINT('Ctrl Pts',(-47.5856008105526,1075.58455096299,
518.828148616589));
#112725=CARTESIAN_POINT('Ctrl Pts',(-47.7210591086514,1075.57275791273,
518.88251120031));
#112726=CARTESIAN_POINT('Ctrl Pts',(-47.9297854064988,1075.55879087764,
518.921476688485));
#112727=CARTESIAN_POINT('Ctrl Pts',(-47.9972990103319,1075.55486937707,
518.927729328124));
#112728=CARTESIAN_POINT('Ctrl Pts',(-48.0649893420775,1075.55153228081,
518.927727241413));
#112729=CARTESIAN_POINT('Origin',(-48.0649554680751,1067.7251047501,517.828896105943));
#112730=CARTESIAN_POINT('',(-48.0649554680751,1075.60888786087,518.327727241935));
#112731=CARTESIAN_POINT('',(-48.0649554680755,1075.70120171291,517.33006496995));
#112732=CARTESIAN_POINT('Ctrl Pts',(-48.0649554680751,1075.60888786087,
518.327727241935));
#112733=CARTESIAN_POINT('Ctrl Pts',(-48.0992071391453,1075.60722863437,
518.327727241935));
#112734=CARTESIAN_POINT('Ctrl Pts',(-48.1334637973026,1075.60589929547,
518.324199567418));
#112735=CARTESIAN_POINT('Ctrl Pts',(-48.2308120936188,1075.60309465836,
518.303818200272));
#112736=CARTESIAN_POINT('Ctrl Pts',(-48.2912423276458,1075.60257430731,
518.278180242568));
#112737=CARTESIAN_POINT('Ctrl Pts',(-48.3988286987254,1075.60422377285,
518.205172799759));
#112738=CARTESIAN_POINT('Ctrl Pts',(-48.4449216152782,1075.60637486178,
518.158549147097));
#112739=CARTESIAN_POINT('Ctrl Pts',(-48.5167682161754,1075.61307782021,
518.050127754965));
#112740=CARTESIAN_POINT('Ctrl Pts',(-48.5417351328201,1075.61757231021,
517.989341218083));
#112741=CARTESIAN_POINT('Ctrl Pts',(-48.5670113254588,1075.6283229294,517.861353012332));
#112742=CARTESIAN_POINT('Ctrl Pts',(-48.5669260928725,1075.63448554066,
517.795346963405));
#112743=CARTESIAN_POINT('Ctrl Pts',(-48.547749762996,1075.64433990826,517.699244525297));
#112744=CARTESIAN_POINT('Ctrl Pts',(-48.5382257162028,1075.64770385252,
517.667916543383));
#112745=CARTESIAN_POINT('Ctrl Pts',(-48.5132180523867,1075.65448488088,
517.607635886622));
#112746=CARTESIAN_POINT('Ctrl Pts',(-48.4978024745126,1075.65788623618,
517.578818041224));
#112747=CARTESIAN_POINT('Ctrl Pts',(-48.4427527368316,1075.66811484334,
517.496451774604));
#112748=CARTESIAN_POINT('Ctrl Pts',(-48.3951237054828,1075.67473242701,
517.449093957106));
#112749=CARTESIAN_POINT('Ctrl Pts',(-48.2841578640708,1075.68669618333,
517.375918605308));
#112750=CARTESIAN_POINT('Ctrl Pts',(-48.2219505162228,1075.69192852252,
517.350766227478));
#112751=CARTESIAN_POINT('Ctrl Pts',(-48.1263765506259,1075.69805613701,
517.332908445803));
#112752=CARTESIAN_POINT('Ctrl Pts',(-48.0957077644681,1075.69975700063,
517.330065222216));
#112753=CARTESIAN_POINT('Ctrl Pts',(-48.0649595603431,1075.70120152066,
517.330064969967));
#112754=CARTESIAN_POINT('',(-48.0649554680751,1082.7251047501,517.33006496995));
#112755=CARTESIAN_POINT('',(-48.0649554680751,1067.7251047501,517.33006496995));
#112756=CARTESIAN_POINT('Origin',(-48.0649554680751,1082.7251047501,517.828896105943));
#112757=CARTESIAN_POINT('Ctrl Pts',(-48.0649554680764,1075.70120171291,
517.33006496995));
#112758=CARTESIAN_POINT('Ctrl Pts',(-47.9999044611301,1075.70425769564,
517.33006496995));
#112759=CARTESIAN_POINT('Ctrl Pts',(-47.9354476847099,1075.70612243468,
517.342788618147));
#112760=CARTESIAN_POINT('Ctrl Pts',(-47.8151009740486,1075.70726495575,
517.392282464125));
#112761=CARTESIAN_POINT('Ctrl Pts',(-47.760399983833,1075.70653554622,517.428519769089));
#112762=CARTESIAN_POINT('Ctrl Pts',(-47.6678714445977,1075.70255080872,
517.520024927186));
#112763=CARTESIAN_POINT('Ctrl Pts',(-47.6310077010242,1075.69932836894,
517.574430432736));
#112764=CARTESIAN_POINT('Ctrl Pts',(-47.5796961761757,1075.69068537271,
517.695559617548));
#112765=CARTESIAN_POINT('Ctrl Pts',(-47.5662879622311,1075.68530429028,
517.761303506675));
#112766=CARTESIAN_POINT('Ctrl Pts',(-47.5659632347747,1075.67311728063,
517.89423329901));
#112767=CARTESIAN_POINT('Ctrl Pts',(-47.5791216868771,1075.66642707446,
517.960113186052));
#112768=CARTESIAN_POINT('Ctrl Pts',(-47.6173529427976,1075.65616205148,
518.051482856452));
#112769=CARTESIAN_POINT('Ctrl Pts',(-47.6328336540704,1075.65276309956,
518.08021984393));
#112770=CARTESIAN_POINT('Ctrl Pts',(-47.6882984438738,1075.64246312669,
518.162706048491));
#112771=CARTESIAN_POINT('Ctrl Pts',(-47.7363836679969,1075.63574105283,
518.210144475302));
#112772=CARTESIAN_POINT('Ctrl Pts',(-47.8472836194192,1075.62365372496,
518.282482986071));
#112773=CARTESIAN_POINT('Ctrl Pts',(-47.9087082971881,1075.61837852881,
518.307148991997));
#112774=CARTESIAN_POINT('Ctrl Pts',(-48.0035260426066,1075.61212913645,
518.324890046688));
#112775=CARTESIAN_POINT('Ctrl Pts',(-48.0342387500439,1075.61037584645,
518.327727241935));
#112776=CARTESIAN_POINT('Ctrl Pts',(-48.0649554680751,1075.60888786087,
518.327727241935));
#112777=CARTESIAN_POINT('Origin',(-62.0518715958007,1067.7251047501,517.840396800599));
#112778=CARTESIAN_POINT('',(-62.0518715958006,1074.92317040789,516.749856051871));
#112779=CARTESIAN_POINT('',(-62.0518715958007,1067.7251047501,516.749856051871));
#112780=CARTESIAN_POINT('Ctrl Pts',(-62.0518921470758,1074.67736430787,
518.930937549134));
#112781=CARTESIAN_POINT('Ctrl Pts',(-62.1942603310177,1074.6664724145,518.930934866201));
#112782=CARTESIAN_POINT('Ctrl Pts',(-62.3354342418161,1074.6588514615,518.903053580556));
#112783=CARTESIAN_POINT('Ctrl Pts',(-62.5982952366624,1074.65116544269,
518.794728005698));
#112784=CARTESIAN_POINT('Ctrl Pts',(-62.7174536596923,1074.65112062037,
518.715798377873));
#112785=CARTESIAN_POINT('Ctrl Pts',(-62.9188964488192,1074.65860121385,
518.516843327924));
#112786=CARTESIAN_POINT('Ctrl Pts',(-62.9991504226547,1074.66604642403,
518.398857898355));
#112787=CARTESIAN_POINT('Ctrl Pts',(-63.1105553117035,1074.68748139238,
518.138225299841));
#112788=CARTESIAN_POINT('Ctrl Pts',(-63.1402390812243,1074.70130458149,
517.997983712585));
#112789=CARTESIAN_POINT('Ctrl Pts',(-63.144377361419,1074.73354656551,517.712985785065));
#112790=CARTESIAN_POINT('Ctrl Pts',(-63.1182120614598,1074.75170339004,
517.570905749583));
#112791=CARTESIAN_POINT('Ctrl Pts',(-63.0390351988826,1074.78026899616,
517.37143452765));
#112792=CARTESIAN_POINT('Ctrl Pts',(-63.0060882392591,1074.7899634778,517.307588148536));
#112793=CARTESIAN_POINT('Ctrl Pts',(-62.9283002311598,1074.80933903494,
517.187518129765));
#112794=CARTESIAN_POINT('Ctrl Pts',(-62.8836767151113,1074.81897657058,
517.131537294117));
#112795=CARTESIAN_POINT('Ctrl Pts',(-62.7328609165993,1074.84765366419,
516.976368806949));
#112796=CARTESIAN_POINT('Ctrl Pts',(-62.6119908311008,1074.8658884934,516.893476149168));
#112797=CARTESIAN_POINT('Ctrl Pts',(-62.3453452480775,1074.89822042974,
516.780205972353));
#112798=CARTESIAN_POINT('Ctrl Pts',(-62.2023159366344,1074.91203054126,
516.750609636004));
#112799=CARTESIAN_POINT('Ctrl Pts',(-61.9128168598515,1074.93346996096,
516.749132190848));
#112800=CARTESIAN_POINT('Ctrl Pts',(-61.7693157896017,1074.94089276304,
516.777169066897));
#112801=CARTESIAN_POINT('Ctrl Pts',(-61.5044467524128,1074.94824448377,
516.886631823903));
#112802=CARTESIAN_POINT('Ctrl Pts',(-61.3853260643093,1074.94826687542,
516.965720359438));
#112803=CARTESIAN_POINT('Ctrl Pts',(-61.183773745132,1074.94107926119,517.165238963778));
#112804=CARTESIAN_POINT('Ctrl Pts',(-61.1034687898453,1074.93392550071,
517.283733177875));
#112805=CARTESIAN_POINT('Ctrl Pts',(-60.9914678374334,1074.91304234065,
517.547458667016));
#112806=CARTESIAN_POINT('Ctrl Pts',(-60.96206910612,1074.89937940805,517.690526211221));
#112807=CARTESIAN_POINT('Ctrl Pts',(-60.9606156081248,1074.86728232888,
517.980207661109));
#112808=CARTESIAN_POINT('Ctrl Pts',(-60.9889230114392,1074.84913335557,
518.123987149514));
#112809=CARTESIAN_POINT('Ctrl Pts',(-61.0716553509557,1074.82055740719,
518.323638730849));
#112810=CARTESIAN_POINT('Ctrl Pts',(-61.105274860867,1074.8109653838,518.386562580986));
#112811=CARTESIAN_POINT('Ctrl Pts',(-61.2261573621606,1074.7814783898,518.567700229877));
#112812=CARTESIAN_POINT('Ctrl Pts',(-61.3313523951008,1074.7617213709,518.672068189386));
#112813=CARTESIAN_POINT('Ctrl Pts',(-61.5743947133541,1074.72519418999,
518.83134188934));
#112814=CARTESIAN_POINT('Ctrl Pts',(-61.7092633476778,1074.70871466609,
518.885721882607));
#112815=CARTESIAN_POINT('Ctrl Pts',(-61.9172146951714,1074.68838082161,
518.924684432473));
#112816=CARTESIAN_POINT('Ctrl Pts',(-61.984452321395,1074.68252379905,518.930938820039));
#112817=CARTESIAN_POINT('Ctrl Pts',(-62.0518921470758,1074.67736430787,
518.930937549134));
#112818=CARTESIAN_POINT('Origin',(-62.0518715958007,1067.7251047501,517.840396800599));
#112819=CARTESIAN_POINT('',(-62.0518715958007,1074.74654397689,518.330937549327));
#112820=CARTESIAN_POINT('',(-62.0518715957997,1074.85711166046,517.34985605187));
#112821=CARTESIAN_POINT('Ctrl Pts',(-62.0518715958007,1074.74654397689,
518.330937549327));
#112822=CARTESIAN_POINT('Ctrl Pts',(-62.0866933977911,1074.7439081959,518.330937549327));
#112823=CARTESIAN_POINT('Ctrl Pts',(-62.1215275249672,1074.74169147073,
518.327229946954));
#112824=CARTESIAN_POINT('Ctrl Pts',(-62.2181304218292,1074.73675502954,
518.306292312785));
#112825=CARTESIAN_POINT('Ctrl Pts',(-62.277288270712,1074.73517998283,518.280734905449));
#112826=CARTESIAN_POINT('Ctrl Pts',(-62.3823615920401,1074.73544743233,
518.208445189124));
#112827=CARTESIAN_POINT('Ctrl Pts',(-62.4272491252186,1074.73727582866,
518.162520707078));
#112828=CARTESIAN_POINT('Ctrl Pts',(-62.4971238766243,1074.7441125856,518.055941661903));
#112829=CARTESIAN_POINT('Ctrl Pts',(-62.5213179376707,1074.74906609204,
517.996293967899));
#112830=CARTESIAN_POINT('Ctrl Pts',(-62.5456795632218,1074.76148918912,
517.870678112267));
#112831=CARTESIAN_POINT('Ctrl Pts',(-62.545375877548,1074.76886150459,517.805874706433));
#112832=CARTESIAN_POINT('Ctrl Pts',(-62.5195854725174,1074.7852194219,517.678491490727));
#112833=CARTESIAN_POINT('Ctrl Pts',(-62.4936505331052,1074.79408514107,
517.617258120011));
#112834=CARTESIAN_POINT('Ctrl Pts',(-62.4193661503622,1074.81186524658,
517.508920862243));
#112835=CARTESIAN_POINT('Ctrl Pts',(-62.3717968856127,1074.82061190484,
517.462787413382));
#112836=CARTESIAN_POINT('Ctrl Pts',(-62.2615240094876,1074.83677645864,
517.392131814308));
#112837=CARTESIAN_POINT('Ctrl Pts',(-62.1999590077581,1074.84404634731,
517.368175631442));
#112838=CARTESIAN_POINT('Ctrl Pts',(-62.1078295525999,1074.85268291733,
517.352255748845));
#112839=CARTESIAN_POINT('Ctrl Pts',(-62.0798907785677,1074.8550288411,517.34985605187));
#112840=CARTESIAN_POINT('Ctrl Pts',(-62.0518715957983,1074.85711166046,
517.34985605187));
#112841=CARTESIAN_POINT('',(-62.0518715958007,1082.7251047501,517.349856051871));
#112842=CARTESIAN_POINT('',(-62.0518715958007,1067.7251047501,517.349856051871));
#112843=CARTESIAN_POINT('Origin',(-62.0518715958007,1082.7251047501,517.840396800599));
#112844=CARTESIAN_POINT('Ctrl Pts',(-62.0518636614512,1074.85711225026,
517.349856051935));
#112845=CARTESIAN_POINT('Ctrl Pts',(-61.9873582813733,1074.86190717157,
517.34985709529));
#112846=CARTESIAN_POINT('Ctrl Pts',(-61.9234066217985,1074.86523466756,
517.362581724588));
#112847=CARTESIAN_POINT('Ctrl Pts',(-61.8048657531118,1074.86854214945,
517.411821523904));
#112848=CARTESIAN_POINT('Ctrl Pts',(-61.7513535549066,1074.8685370349,517.447487760785));
#112849=CARTESIAN_POINT('Ctrl Pts',(-61.6608927591218,1074.86523161019,
517.537351112991));
#112850=CARTESIAN_POINT('Ctrl Pts',(-61.624887274215,1074.8619598069,517.590663062806));
#112851=CARTESIAN_POINT('Ctrl Pts',(-61.574577695082,1074.85241793378,517.70959785811));
#112852=CARTESIAN_POINT('Ctrl Pts',(-61.561443420754,1074.84616349522,517.774295153346));
#112853=CARTESIAN_POINT('Ctrl Pts',(-61.5612191536718,1074.83152276947,
517.905144090354));
#112854=CARTESIAN_POINT('Ctrl Pts',(-61.5742603948211,1074.82327037349,
517.970007685616));
#112855=CARTESIAN_POINT('Ctrl Pts',(-61.6120158739641,1074.81033229964,
518.059910237568));
#112856=CARTESIAN_POINT('Ctrl Pts',(-61.6273052580951,1074.80600235113,
518.08819086711));
#112857=CARTESIAN_POINT('Ctrl Pts',(-61.6820460903651,1074.79275149702,
518.16931808239));
#112858=CARTESIAN_POINT('Ctrl Pts',(-61.7294769085497,1074.78391794939,
518.215940335845));
#112859=CARTESIAN_POINT('Ctrl Pts',(-61.8393283348014,1074.767568359,518.28726613734));
#112860=CARTESIAN_POINT('Ctrl Pts',(-61.9005188251533,1074.76019322307,
518.311550515567));
#112861=CARTESIAN_POINT('Ctrl Pts',(-61.9935655083327,1074.7512518364,518.328337882215));
#112862=CARTESIAN_POINT('Ctrl Pts',(-62.0227142309869,1074.7487509973,518.330937549327));
#112863=CARTESIAN_POINT('Ctrl Pts',(-62.0518715958007,1074.74654397689,
518.330937549327));
#112864=CARTESIAN_POINT('Origin',(-3.98894410367368,1067.7251047501,514.089592938904));
#112865=CARTESIAN_POINT('',(-3.98894410369425,1076.70513022417,512.611289806711));
#112866=CARTESIAN_POINT('',(-3.98894410367368,1067.7251047501,512.611289806711));
#112867=CARTESIAN_POINT('',(-3.98894410367368,1076.62830575618,515.567896071097));
#112868=CARTESIAN_POINT('Ctrl Pts',(-3.98894410367368,1076.62830575618,
515.567896071097));
#112869=CARTESIAN_POINT('Ctrl Pts',(-4.03382380580244,1076.62823827216,
515.567896071097));
#112870=CARTESIAN_POINT('Ctrl Pts',(-4.07835975006978,1076.62823966801,
515.565856602404));
#112871=CARTESIAN_POINT('Ctrl Pts',(-4.12255616830439,1076.62830843885,
515.561845623343));
#112872=CARTESIAN_POINT('Ctrl Pts',(-4.16719148972908,1076.62837789263,
515.557794812287));
#112873=CARTESIAN_POINT('Ctrl Pts',(-4.21148143877147,1076.62851606623,
515.551733139065));
#112874=CARTESIAN_POINT('Ctrl Pts',(-4.25543363066647,1076.6287214095,515.54367804049));
#112875=CARTESIAN_POINT('Ctrl Pts',(-4.26269409923196,1076.62875533018,
515.54234741766));
#112876=CARTESIAN_POINT('Ctrl Pts',(-4.2699453401395,1076.62879108377,515.540962283859));
#112877=CARTESIAN_POINT('Ctrl Pts',(-4.27718736869677,1076.62882866329,
515.539522582308));
#112878=CARTESIAN_POINT('Ctrl Pts',(-4.3152789658614,1076.6290263239,515.531950044988));
#112879=CARTESIAN_POINT('Ctrl Pts',(-4.3532804804579,1076.62927674603,515.522830609595));
#112880=CARTESIAN_POINT('Ctrl Pts',(-4.39093485348061,1076.62957750851,
515.512190418067));
#112881=CARTESIAN_POINT('Ctrl Pts',(-4.42855367177372,1076.62987798701,
515.501560273424));
#112882=CARTESIAN_POINT('Ctrl Pts',(-4.46582540448601,1076.63022871084,
515.489412364288));
#112883=CARTESIAN_POINT('Ctrl Pts',(-4.50250499970203,1076.63062726572,
515.475823567884));
#112884=CARTESIAN_POINT('Ctrl Pts',(-4.52018651723302,1076.63081939038,
515.469273044619));
#112885=CARTESIAN_POINT('Ctrl Pts',(-4.53773066102735,1076.63102262981,
515.462388439635));
#112886=CARTESIAN_POINT('Ctrl Pts',(-4.55511153485945,1076.63123671354,
515.455182405221));
#112887=CARTESIAN_POINT('Ctrl Pts',(-4.59683648483769,1076.63175064817,
515.437883423113));
#112888=CARTESIAN_POINT('Ctrl Pts',(-4.63755429334944,1076.63232447203,
515.418765655002));
#112889=CARTESIAN_POINT('Ctrl Pts',(-4.67728134605977,1076.6329563068,515.397863549824));
#112890=CARTESIAN_POINT('Ctrl Pts',(-4.71710436732038,1076.6335896679,515.376910951478));
#112891=CARTESIAN_POINT('Ctrl Pts',(-4.75593268733475,1076.63428132053,
515.354164962572));
#112892=CARTESIAN_POINT('Ctrl Pts',(-4.79376065554514,1076.63502937274,
515.329613288933));
#112893=CARTESIAN_POINT('Ctrl Pts',(-4.79916555013926,1076.63513625512,
515.326105323414));
#112894=CARTESIAN_POINT('Ctrl Pts',(-4.80454997336945,1076.6352442889,515.322560423272));
#112895=CARTESIAN_POINT('Ctrl Pts',(-4.8099138564203,1076.63535346856,515.318978482876));
#112896=CARTESIAN_POINT('Ctrl Pts',(-4.84006919053791,1076.63596726809,
515.298841092034));
#112897=CARTESIAN_POINT('Ctrl Pts',(-4.86963875872755,1076.63661969767,
515.277485372765));
#112898=CARTESIAN_POINT('Ctrl Pts',(-4.89840452092768,1076.63730478053,
515.255037875441));
#112899=CARTESIAN_POINT('Ctrl Pts',(-4.92717801125513,1076.63799004744,
515.232584347438));
#112900=CARTESIAN_POINT('Ctrl Pts',(-4.9551467821994,1076.6387079852,515.209038795042));
#112901=CARTESIAN_POINT('Ctrl Pts',(-4.9821237700803,1076.63945261223,515.18456978838));
#112902=CARTESIAN_POINT('Ctrl Pts',(-5.00004363908716,1076.63994724191,
515.168315883532));
#112903=CARTESIAN_POINT('Ctrl Pts',(-5.01752654789864,1076.64045364818,
515.151655371139));
#112904=CARTESIAN_POINT('Ctrl Pts',(-5.03452671334026,1076.64097007782,
515.13464660117));
#112905=CARTESIAN_POINT('Ctrl Pts',(-5.06961887939331,1076.64203610477,
515.099536673436));
#112906=CARTESIAN_POINT('Ctrl Pts',(-5.10302181777584,1076.64315559168,
515.062573790306));
#112907=CARTESIAN_POINT('Ctrl Pts',(-5.13450312720013,1076.64431787742,
515.023977588965));
#112908=CARTESIAN_POINT('Ctrl Pts',(-5.16596650616121,1076.64547950116,
514.985403370438));
#112909=CARTESIAN_POINT('Ctrl Pts',(-5.19551002466464,1076.64668387499,
514.945198147337));
#112910=CARTESIAN_POINT('Ctrl Pts',(-5.22294001512885,1076.64792035598,
514.903616428224));
#112911=CARTESIAN_POINT('Ctrl Pts',(-5.25039095889401,1076.64915778149,
514.862002945546));
#112912=CARTESIAN_POINT('Ctrl Pts',(-5.27572480832945,1076.65042736322,
514.819011384178));
#112913=CARTESIAN_POINT('Ctrl Pts',(-5.29879155836087,1076.65171843384,
514.774924826461));
#112914=CARTESIAN_POINT('Ctrl Pts',(-5.31922564937179,1076.65286215172,
514.735869964743));
#112915=CARTESIAN_POINT('Ctrl Pts',(-5.3378811359444,1076.65402273325,514.695956452106));
#112916=CARTESIAN_POINT('Ctrl Pts',(-5.35468532261741,1076.65519276256,
514.65539420572));
#112917=CARTESIAN_POINT('Ctrl Pts',(-5.37357582673536,1076.65650805641,
514.609795968965));
#112918=CARTESIAN_POINT('Ctrl Pts',(-5.39023224656117,1076.65784178247,
514.563120864991));
#112919=CARTESIAN_POINT('Ctrl Pts',(-5.40451833901832,1076.65918391593,
514.515656003345));
#112920=CARTESIAN_POINT('Ctrl Pts',(-5.41879401809223,1076.66052507109,
514.468225739669));
#112921=CARTESIAN_POINT('Ctrl Pts',(-5.43070259306572,1076.6618746214,514.420007443696));
#112922=CARTESIAN_POINT('Ctrl Pts',(-5.4401565240363,1076.66322256394,514.37130673274));
#112923=CARTESIAN_POINT('Ctrl Pts',(-5.44961550628525,1076.6645712267,514.322580000773));
#112924=CARTESIAN_POINT('Ctrl Pts',(-5.45661709319358,1076.66591827998,
514.27337094645));
#112925=CARTESIAN_POINT('Ctrl Pts',(-5.46112479268709,1076.66725370484,
514.223995950583));
#112926=CARTESIAN_POINT('Ctrl Pts',(-5.46519159746117,1076.66845851279,
514.179450286169));
#112927=CARTESIAN_POINT('Ctrl Pts',(-5.46722916015916,1076.66965385581,
514.134770005097));
#112928=CARTESIAN_POINT('Ctrl Pts',(-5.46724711596372,1076.67083237661,
514.090188343358));
#112929=CARTESIAN_POINT('Ctrl Pts',(-5.46726177561919,1076.67179455621,
514.053790542343));
#112930=CARTESIAN_POINT('Ctrl Pts',(-5.46592795458365,1076.67275310273,
514.017175204292));
#112931=CARTESIAN_POINT('Ctrl Pts',(-5.46322340498931,1076.67370161935,
513.980594350085));
#112932=CARTESIAN_POINT('Ctrl Pts',(-5.46052021283035,1076.6746496599,513.944031856106));
#112933=CARTESIAN_POINT('Ctrl Pts',(-5.45644767069605,1076.67558768062,
513.907504402001));
#112934=CARTESIAN_POINT('Ctrl Pts',(-5.4510356663401,1076.67650929431,513.871261967597));
#112935=CARTESIAN_POINT('Ctrl Pts',(-5.44752072436303,1076.67710785603,
513.847723543446));
#112936=CARTESIAN_POINT('Ctrl Pts',(-5.44344185186923,1076.67769949705,
513.824305287228));
#112937=CARTESIAN_POINT('Ctrl Pts',(-5.43881882267849,1076.67828246757,
513.801073529084));
#112938=CARTESIAN_POINT('Ctrl Pts',(-5.43000622466527,1076.67939374864,
513.756788248326));
#112939=CARTESIAN_POINT('Ctrl Pts',(-5.41920433510385,1076.68047665497,
513.713083925439));
#112940=CARTESIAN_POINT('Ctrl Pts',(-5.40643602623801,1076.68153210232,
513.669954046382));
#112941=CARTESIAN_POINT('Ctrl Pts',(-5.3936828518979,1076.68258629864,513.626875290013));
#112942=CARTESIAN_POINT('Ctrl Pts',(-5.37896763951009,1076.68361310103,
513.584368714443));
#112943=CARTESIAN_POINT('Ctrl Pts',(-5.36226378135259,1076.68461342204,
513.542442855698));
#112944=CARTESIAN_POINT('Ctrl Pts',(-5.35989519129212,1076.68475526654,
513.536497811663));
#112945=CARTESIAN_POINT('Ctrl Pts',(-5.35748653872257,1076.68489657858,
513.530564481821));
#112946=CARTESIAN_POINT('Ctrl Pts',(-5.3550376727605,1076.68503736076,513.524642931247));
#112947=CARTESIAN_POINT('Ctrl Pts',(-5.34042728288203,1076.68587729344,
513.489313858967));
#112948=CARTESIAN_POINT('Ctrl Pts',(-5.32439017493919,1076.6866972177,513.454426945205));
#112949=CARTESIAN_POINT('Ctrl Pts',(-5.30701842434866,1076.68749315242,
513.420219921948));
#112950=CARTESIAN_POINT('Ctrl Pts',(-5.28963199199989,1076.68828975983,
513.385983988579));
#112951=CARTESIAN_POINT('Ctrl Pts',(-5.27090892993038,1076.68906233713,
513.352429639599));
#112952=CARTESIAN_POINT('Ctrl Pts',(-5.25098810610052,1076.68980689311,
513.319771474803));
#112953=CARTESIAN_POINT('Ctrl Pts',(-5.24039444818967,1076.69020283915,
513.302404249994));
#112954=CARTESIAN_POINT('Ctrl Pts',(-5.22946282924075,1076.6905908608,513.285290012385));
#112955=CARTESIAN_POINT('Ctrl Pts',(-5.21821901558114,1076.69097035782,
513.268457541051));
#112956=CARTESIAN_POINT('Ctrl Pts',(-5.19335281033031,1076.69180963273,
513.231231765194));
#112957=CARTESIAN_POINT('Ctrl Pts',(-5.16683758555087,1076.69261257175,
513.195190469683));
#112958=CARTESIAN_POINT('Ctrl Pts',(-5.13866486638326,1076.69338071947,
513.160333923104));
#112959=CARTESIAN_POINT('Ctrl Pts',(-5.11073634250464,1076.69414220905,
513.125779505843));
#112960=CARTESIAN_POINT('Ctrl Pts',(-5.08117830263898,1076.69486950784,
513.092388723484));
#112961=CARTESIAN_POINT('Ctrl Pts',(-5.04994673371333,1076.69556412063,
513.06019817998));
#112962=CARTESIAN_POINT('Ctrl Pts',(-5.04488406308498,1076.6956767181,513.05498005855));
#112963=CARTESIAN_POINT('Ctrl Pts',(-5.03977735273785,1076.69578845669,
513.049793565901));
#112964=CARTESIAN_POINT('Ctrl Pts',(-5.03462634377255,1076.69589934281,
513.044638967002));
#112965=CARTESIAN_POINT('Ctrl Pts',(-4.98509132459662,1076.69696568653,
512.995069424986));
#112966=CARTESIAN_POINT('Ctrl Pts',(-4.93233611087355,1076.69793441364,
512.949321540321));
#112967=CARTESIAN_POINT('Ctrl Pts',(-4.87678398576265,1076.69880913241,
512.907594421805));
#112968=CARTESIAN_POINT('Ctrl Pts',(-4.81842086903492,1076.69972811281,
512.863755870467));
#112969=CARTESIAN_POINT('Ctrl Pts',(-4.7569688942424,1076.70054333035,512.824353182086));
#112970=CARTESIAN_POINT('Ctrl Pts',(-4.69286914438583,1076.70125896924,
512.789643059982));
#112971=CARTESIAN_POINT('Ctrl Pts',(-4.64805083877426,1076.70175934128,
512.765373872289));
#112972=CARTESIAN_POINT('Ctrl Pts',(-4.60193692810212,1076.70221103177,
512.743399379173));
#112973=CARTESIAN_POINT('Ctrl Pts',(-4.55467309415124,1076.70261547096,
512.723821779454));
#112974=CARTESIAN_POINT('Ctrl Pts',(-4.51294825012113,1076.7029725127,512.706538537143));
#112975=CARTESIAN_POINT('Ctrl Pts',(-4.47065903441898,1076.70328996082,
512.69125696259));
#112976=CARTESIAN_POINT('Ctrl Pts',(-4.42781932239519,1076.70356952053,
512.677938344804));
#112977=CARTESIAN_POINT('Ctrl Pts',(-4.38484404374123,1076.7038499649,512.66457758014));
#112978=CARTESIAN_POINT('Ctrl Pts',(-4.34131388393893,1076.7040922807,512.653191908722));
#112979=CARTESIAN_POINT('Ctrl Pts',(-4.29722472367035,1076.70429818939,
512.643791012641));
#112980=CARTESIAN_POINT('Ctrl Pts',(-4.29088399272208,1076.70432780237,
512.642439012458));
#112981=CARTESIAN_POINT('Ctrl Pts',(-4.28453168290618,1076.70435666234,
512.641128149906));
#112982=CARTESIAN_POINT('Ctrl Pts',(-4.27816776842535,1076.70438477442,
512.639858541713));
#112983=CARTESIAN_POINT('Ctrl Pts',(-4.2427823506189,1076.70454108667,512.632799110526));
#112984=CARTESIAN_POINT('Ctrl Pts',(-4.20694315657351,1076.704673918,512.627000670701));
#112985=CARTESIAN_POINT('Ctrl Pts',(-4.17089333556487,1076.70478300393,
512.622529672488));
#112986=CARTESIAN_POINT('Ctrl Pts',(-4.13483990415784,1076.70489210079,
512.618058226504));
#112987=CARTESIAN_POINT('Ctrl Pts',(-4.09857638220709,1076.70497744749,
512.614914591586));
#112988=CARTESIAN_POINT('Ctrl Pts',(-4.06235386956601,1076.7050387795,512.613113627527));
#112989=CARTESIAN_POINT('Ctrl Pts',(-4.03783906398118,1076.70508028799,
512.611894764435));
#112990=CARTESIAN_POINT('Ctrl Pts',(-4.01334319964393,1076.70511079689,
512.611289806711));
#112991=CARTESIAN_POINT('Ctrl Pts',(-3.98894410369425,1076.70513022417,
512.611289806711));
#112992=CARTESIAN_POINT('Ctrl Pts',(-3.98894410369425,1076.70513022417,
512.611289806711));
#112993=CARTESIAN_POINT('Ctrl Pts',(-3.89010227930185,1076.70520892495,
512.61128980671));
#112994=CARTESIAN_POINT('Ctrl Pts',(-3.7915191632709,1076.70511108275,512.621201580718));
#112995=CARTESIAN_POINT('Ctrl Pts',(-3.59467449494741,1076.70455073789,
512.661188086013));
#112996=CARTESIAN_POINT('Ctrl Pts',(-3.49706431916902,1076.704078049,512.691793644763));
#112997=CARTESIAN_POINT('Ctrl Pts',(-3.23483687727456,1076.702211287,512.804914607444));
#112998=CARTESIAN_POINT('Ctrl Pts',(-3.08130018423767,1076.70040097121,
512.908384151165));
#112999=CARTESIAN_POINT('Ctrl Pts',(-2.81189620632753,1076.69531749021,
513.1742069126));
#113000=CARTESIAN_POINT('Ctrl Pts',(-2.70159427009519,1076.69200279032,
513.33720003985));
#113001=CARTESIAN_POINT('Ctrl Pts',(-2.55003143068424,1076.68399367258,
513.697863740724));
#113002=CARTESIAN_POINT('Ctrl Pts',(-2.51078829823382,1076.67936288322,
513.892190254648));
#113003=CARTESIAN_POINT('Ctrl Pts',(-2.51049475856978,1076.66927561583,
514.284400974555));
#113004=CARTESIAN_POINT('Ctrl Pts',(-2.54929534796991,1076.66392059558,
514.47840051194));
#113005=CARTESIAN_POINT('Ctrl Pts',(-2.69956374535934,1076.65337255126,
514.838293157373));
#113006=CARTESIAN_POINT('Ctrl Pts',(-2.80890085393043,1076.64828624815,
515.000942899898));
#113007=CARTESIAN_POINT('Ctrl Pts',(-3.07721597011864,1076.639554502,515.26776677021));
#113008=CARTESIAN_POINT('Ctrl Pts',(-3.23105328591043,1076.63593165891,
515.372150493012));
#113009=CARTESIAN_POINT('Ctrl Pts',(-3.49427595121394,1076.6317746266,515.486454209748));
#113010=CARTESIAN_POINT('Ctrl Pts',(-3.59244187907109,1076.63059411286,
515.517425376927));
#113011=CARTESIAN_POINT('Ctrl Pts',(-3.79040983355065,1076.62894293207,
515.557872175624));
#113012=CARTESIAN_POINT('Ctrl Pts',(-3.88954463142303,1076.62845521963,
515.567896071097));
#113013=CARTESIAN_POINT('Ctrl Pts',(-3.98894410367368,1076.62830575618,
515.567896071097));
#113014=CARTESIAN_POINT('Origin',(-3.98894410367368,1067.7251047501,514.089592938904));
#113015=CARTESIAN_POINT('',(-3.98894410367369,1076.64787682225,514.967896071097));
#113016=CARTESIAN_POINT('',(-3.98894410328192,1076.69355479191,513.211289806711));
#113017=CARTESIAN_POINT('Ctrl Pts',(-3.98894410367369,1076.64787682225,
514.967896071097));
#113018=CARTESIAN_POINT('Ctrl Pts',(-4.04149225305876,1076.64780501974,
514.967896071097));
#113019=CARTESIAN_POINT('Ctrl Pts',(-4.09405915061969,1076.64787785117,
514.963180256518));
#113020=CARTESIAN_POINT('Ctrl Pts',(-4.25901867059246,1076.64857049626,
514.93319827929));
#113021=CARTESIAN_POINT('Ctrl Pts',(-4.36690585428157,1076.64972588111,
514.890687485131));
#113022=CARTESIAN_POINT('Ctrl Pts',(-4.56015184895358,1076.65319497187,
514.766585953667));
#113023=CARTESIAN_POINT('Ctrl Pts',(-4.6436542891775,1076.65547258593,514.686207246268));
#113024=CARTESIAN_POINT('Ctrl Pts',(-4.77504221070995,1076.66074118729,
514.497835356852));
#113025=CARTESIAN_POINT('Ctrl Pts',(-4.82163796085241,1076.66367938196,
514.391637552296));
#113026=CARTESIAN_POINT('Ctrl Pts',(-4.85888449665252,1076.66821809082,
514.223442198093));
#113027=CARTESIAN_POINT('Ctrl Pts',(-4.86577146008994,1076.66974202842,
514.166311287477));
#113028=CARTESIAN_POINT('Ctrl Pts',(-4.86829784916898,1076.67276384636,
514.051520487883));
#113029=CARTESIAN_POINT('Ctrl Pts',(-4.86393018775512,1076.67425446059,
513.994135845765));
#113030=CARTESIAN_POINT('Ctrl Pts',(-4.83377771086896,1076.67865188257,
513.822539379258));
#113031=CARTESIAN_POINT('Ctrl Pts',(-4.79081030033423,1076.68138199551,
513.712664687311));
#113032=CARTESIAN_POINT('Ctrl Pts',(-4.66459751953398,1076.6861530925,513.516467774466));
#113033=CARTESIAN_POINT('Ctrl Pts',(-4.58272850939619,1076.68815139934,
513.432019243722));
#113034=CARTESIAN_POINT('Ctrl Pts',(-4.39063234601568,1076.69127697328,
513.299858850111));
#113035=CARTESIAN_POINT('Ctrl Pts',(-4.28226733965402,1076.69237443015,
513.253532640986));
#113036=CARTESIAN_POINT('Ctrl Pts',(-4.10897180875891,1076.69331089348,
513.217441882773));
#113037=CARTESIAN_POINT('Ctrl Pts',(-4.04896272635834,1076.69349799811,
513.211289806658));
#113038=CARTESIAN_POINT('Ctrl Pts',(-3.98894410289016,1076.69355479191,
513.211289806711));
#113039=CARTESIAN_POINT('',(-3.98894410367368,1082.7251047501,513.211289806711));
#113040=CARTESIAN_POINT('',(-3.98894410367368,1067.7251047501,513.211289806711));
#113041=CARTESIAN_POINT('Origin',(-3.98894410367368,1082.7251047501,514.089592938904));
#113042=CARTESIAN_POINT('Ctrl Pts',(-3.98894410289016,1076.69355479191,
513.211289806711));
#113043=CARTESIAN_POINT('Ctrl Pts',(-3.93259196053329,1076.69360811622,
513.211289806761));
#113044=CARTESIAN_POINT('Ctrl Pts',(-3.87623140718768,1076.69354653842,
513.216713139767));
#113045=CARTESIAN_POINT('Ctrl Pts',(-3.70602832970331,1076.69300108805,
513.249941693398));
#113046=CARTESIAN_POINT('Ctrl Pts',(-3.59701492633745,1076.69214788553,
513.294957478828));
#113047=CARTESIAN_POINT('Ctrl Pts',(-3.40322866750269,1076.68948920037,
513.424818703465));
#113048=CARTESIAN_POINT('Ctrl Pts',(-3.32032214304025,1076.68770970805,
513.508276215716));
#113049=CARTESIAN_POINT('Ctrl Pts',(-3.19180681534375,1076.68332366884,
513.702810789303));
#113050=CARTESIAN_POINT('Ctrl Pts',(-3.14753761985142,1076.68075664216,
513.811995534928));
#113051=CARTESIAN_POINT('Ctrl Pts',(-3.11660159621135,1076.67670312101,
513.975829298708));
#113052=CARTESIAN_POINT('Ctrl Pts',(-3.1115356003055,1076.67544402827,514.025735618899));
#113053=CARTESIAN_POINT('Ctrl Pts',(-3.11074928295003,1076.67415562567,
514.07579986548));
#113054=CARTESIAN_POINT('Ctrl Pts',(-3.10983848239562,1076.67266325392,
514.133789865604));
#113055=CARTESIAN_POINT('Ctrl Pts',(-3.11467382062161,1076.67113829599,
514.191727200505));
#113056=CARTESIAN_POINT('Ctrl Pts',(-3.14605896703041,1076.66655651049,
514.362043412921));
#113057=CARTESIAN_POINT('Ctrl Pts',(-3.18901660653344,1076.6635141462,514.470121302242));
#113058=CARTESIAN_POINT('Ctrl Pts',(-3.31421419718697,1076.65786322126,
514.66355454975));
#113059=CARTESIAN_POINT('Ctrl Pts',(-3.39525158639593,1076.65531186279,
514.747031234788));
#113060=CARTESIAN_POINT('Ctrl Pts',(-3.58489355607944,1076.65116968365,
514.877898170841));
#113061=CARTESIAN_POINT('Ctrl Pts',(-3.69164387888887,1076.64962103285,
514.924037620655));
#113062=CARTESIAN_POINT('Ctrl Pts',(-3.8650972758057,1076.64824710587,514.961344519471));
#113063=CARTESIAN_POINT('Ctrl Pts',(-3.92700766681083,1076.64796145305,
514.967896071097));
#113064=CARTESIAN_POINT('Ctrl Pts',(-3.98894410367369,1076.64787682225,
514.967896071097));
#113065=CARTESIAN_POINT('Origin',(-14.9669751953831,1067.7251047501,520.188191956395));
#113066=CARTESIAN_POINT('',(-14.9669751954018,1076.42256169839,518.912747835258));
#113067=CARTESIAN_POINT('',(-14.9669751953831,1067.7251047501,518.912747835258));
#113068=CARTESIAN_POINT('Ctrl Pts',(-14.9670021241791,1076.25965984465,
521.463636077246));
#113069=CARTESIAN_POINT('Ctrl Pts',(-15.1336635644875,1076.25785153312,
521.463632558478));
#113070=CARTESIAN_POINT('Ctrl Pts',(-15.2987115911046,1076.25832656805,
521.430963338145));
#113071=CARTESIAN_POINT('Ctrl Pts',(-15.6066713015969,1076.26376895275,
521.304096002063));
#113072=CARTESIAN_POINT('Ctrl Pts',(-15.7466054890221,1076.26867493645,
521.21122325551));
#113073=CARTESIAN_POINT('Ctrl Pts',(-15.9830506727415,1076.28215836799,
520.976919933069));
#113074=CARTESIAN_POINT('Ctrl Pts',(-16.0772095673545,1076.29060690936,
520.837681537416));
#113075=CARTESIAN_POINT('Ctrl Pts',(-16.2068907476775,1076.30977042356,
520.530582611396));
#113076=CARTESIAN_POINT('Ctrl Pts',(-16.2409974736705,1076.32030446555,
520.365577861591));
#113077=CARTESIAN_POINT('Ctrl Pts',(-16.2437565496537,1076.34192696332,
520.03158437749));
#113078=CARTESIAN_POINT('Ctrl Pts',(-16.2122673467434,1076.35280840907,
519.865772543202));
#113079=CARTESIAN_POINT('Ctrl Pts',(-16.0863865872732,1076.37357572541,
519.553944418207));
#113080=CARTESIAN_POINT('Ctrl Pts',(-15.9925110914523,1076.38324688577,
519.411233388948));
#113081=CARTESIAN_POINT('Ctrl Pts',(-15.7548895327075,1076.40004536789,
519.171152346095));
#113082=CARTESIAN_POINT('Ctrl Pts',(-15.6136669424916,1076.40702126391,
519.075982913399));
#113083=CARTESIAN_POINT('Ctrl Pts',(-15.3019561978232,1076.41757526725,
518.945969105108));
#113084=CARTESIAN_POINT('Ctrl Pts',(-15.1345246872508,1076.42104616242,
518.912542548849));
#113085=CARTESIAN_POINT('Ctrl Pts',(-14.7960739890186,1076.42410766345,
518.912955312285));
#113086=CARTESIAN_POINT('Ctrl Pts',(-14.628456499764,1076.42366363939,518.946887187125));
#113087=CARTESIAN_POINT('Ctrl Pts',(-14.3166047174734,1076.41886072836,
519.078086691963));
#113088=CARTESIAN_POINT('Ctrl Pts',(-14.175446968428,1076.41455533409,519.173909391717));
#113089=CARTESIAN_POINT('Ctrl Pts',(-13.9388582324749,1076.40246837647,
519.414760269681));
#113090=CARTESIAN_POINT('Ctrl Pts',(-13.8457245853666,1076.39480575976,
519.557338223495));
#113091=CARTESIAN_POINT('Ctrl Pts',(-13.7199886720594,1076.37686140203,
519.871161458313));
#113092=CARTESIAN_POINT('Ctrl Pts',(-13.6889596529711,1076.36673965532,
520.039439402739));
#113093=CARTESIAN_POINT('Ctrl Pts',(-13.6930612725026,1076.3506808469,520.293154918816));
#113094=CARTESIAN_POINT('Ctrl Pts',(-13.7027893854653,1076.3452340051,520.377154043451));
#113095=CARTESIAN_POINT('Ctrl Pts',(-13.7564001201965,1076.32887787121,
520.62334720139));
#113096=CARTESIAN_POINT('Ctrl Pts',(-13.8240053407547,1076.31803638244,
520.778519821053));
#113097=CARTESIAN_POINT('Ctrl Pts',(-14.0153576593589,1076.29778936615,
521.053794890939));
#113098=CARTESIAN_POINT('Ctrl Pts',(-14.1372416223797,1076.28858188701,
521.171262865823));
#113099=CARTESIAN_POINT('Ctrl Pts',(-14.4192662617666,1076.27327573536,
521.352138307294));
#113100=CARTESIAN_POINT('Ctrl Pts',(-14.5765772173206,1076.26732318967,
521.413911181364));
#113101=CARTESIAN_POINT('Ctrl Pts',(-14.8158415454656,1076.26176583286,
521.456907181747));
#113102=CARTESIAN_POINT('Ctrl Pts',(-14.8913430558827,1076.26048076139,
521.463637674657));
#113103=CARTESIAN_POINT('Ctrl Pts',(-14.9670021241791,1076.25965984465,
521.463636077246));
#113104=CARTESIAN_POINT('Origin',(-14.9669751953831,1067.7251047501,520.188191956395));
#113105=CARTESIAN_POINT('',(-14.9669751953831,1076.30090002967,520.863636077531));
#113106=CARTESIAN_POINT('',(-14.9669751953831,1076.38718569293,519.512747835259));
#113107=CARTESIAN_POINT('Ctrl Pts',(-14.9669751953831,1076.30090002967,
520.863636077531));
#113108=CARTESIAN_POINT('Ctrl Pts',(-15.0159124905779,1076.30038825754,
520.863636077531));
#113109=CARTESIAN_POINT('Ctrl Pts',(-15.0648239295839,1076.30023170671,
520.858317612946));
#113110=CARTESIAN_POINT('Ctrl Pts',(-15.1989748452287,1076.30081025746,
520.828647733869));
#113111=CARTESIAN_POINT('Ctrl Pts',(-15.2805325350751,1076.30234596997,
520.79290915802));
#113112=CARTESIAN_POINT('Ctrl Pts',(-15.4253275056845,1076.30754318032,
520.692102076889));
#113113=CARTESIAN_POINT('Ctrl Pts',(-15.4871425503217,1076.31115458539,
520.627994392063));
#113114=CARTESIAN_POINT('Ctrl Pts',(-15.5827342408467,1076.31994379382,
520.479532668925));
#113115=CARTESIAN_POINT('Ctrl Pts',(-15.6155204543622,1076.32503940514,
520.396560635829));
#113116=CARTESIAN_POINT('Ctrl Pts',(-15.6393585190988,1076.33325478884,
520.266168602466));
#113117=CARTESIAN_POINT('Ctrl Pts',(-15.6430195310319,1076.33607071421,
520.222002421342));
#113118=CARTESIAN_POINT('Ctrl Pts',(-15.6416588370593,1076.34177054242,
520.133573441364));
#113119=CARTESIAN_POINT('Ctrl Pts',(-15.6366356806778,1076.34464093559,
520.089520542491));
#113120=CARTESIAN_POINT('Ctrl Pts',(-15.6084041255894,1076.35329360248,
519.95815266914));
#113121=CARTESIAN_POINT('Ctrl Pts',(-15.5720124726391,1076.35891932012,
519.874685772055));
#113122=CARTESIAN_POINT('Ctrl Pts',(-15.4687950299649,1076.36915635785,
519.72725219796));
#113123=CARTESIAN_POINT('Ctrl Pts',(-15.4031181994801,1076.37367156808,
519.664665599285));
#113124=CARTESIAN_POINT('Ctrl Pts',(-15.2511143303541,1076.38104185865,
519.568874191581));
#113125=CARTESIAN_POINT('Ctrl Pts',(-15.1663229962618,1076.38382570443,
519.536609231153));
#113126=CARTESIAN_POINT('Ctrl Pts',(-15.0410966181079,1076.38629232625,
519.515803738376));
#113127=CARTESIAN_POINT('Ctrl Pts',(-15.0040740883286,1076.38683176229,
519.512748425204));
#113128=CARTESIAN_POINT('Ctrl Pts',(-14.9669859361834,1076.38718559046,
519.512747835446));
#113129=CARTESIAN_POINT('Ctrl Pts',(-14.9669823559152,1076.38718562461,
519.512747835389));
#113130=CARTESIAN_POINT('Ctrl Pts',(-14.9669787756485,1076.38718565877,
519.512747835259));
#113131=CARTESIAN_POINT('Ctrl Pts',(-14.9669751953832,1076.38718569293,
519.512747835259));
#113132=CARTESIAN_POINT('',(-14.9669751953831,1082.7251047501,519.512747835259));
#113133=CARTESIAN_POINT('',(-14.9669751953831,1067.7251047501,519.512747835259));
#113134=CARTESIAN_POINT('Origin',(-14.9669751953831,1082.7251047501,520.188191956395));
#113135=CARTESIAN_POINT('Ctrl Pts',(-14.9669751953832,1076.38718569293,
519.512747835259));
#113136=CARTESIAN_POINT('Ctrl Pts',(-14.8770304130865,1076.38804369637,
519.512747835259));
#113137=CARTESIAN_POINT('Ctrl Pts',(-14.7879875438153,1076.38779961628,
519.530713998948));
#113138=CARTESIAN_POINT('Ctrl Pts',(-14.6222355938098,1076.38513168314,
519.600435473661));
#113139=CARTESIAN_POINT('Ctrl Pts',(-14.5471950195292,1076.38273558835,
519.651462301316));
#113140=CARTESIAN_POINT('Ctrl Pts',(-14.4214950009639,1076.37605308584,
519.779844122122));
#113141=CARTESIAN_POINT('Ctrl Pts',(-14.372100867259,1076.37183209441,519.855913435516));
#113142=CARTESIAN_POINT('Ctrl Pts',(-14.3058422523083,1076.36204990605,
520.023132686935));
#113143=CARTESIAN_POINT('Ctrl Pts',(-14.2897540825696,1076.35658048938,
520.112664605299));
#113144=CARTESIAN_POINT('Ctrl Pts',(-14.2926457301874,1076.34799942994,
520.247364448804));
#113145=CARTESIAN_POINT('Ctrl Pts',(-14.2980359096252,1076.34510915037,
520.291833557599));
#113146=CARTESIAN_POINT('Ctrl Pts',(-14.3271149076484,1076.33647555813,
520.422012246066));
#113147=CARTESIAN_POINT('Ctrl Pts',(-14.3633213046354,1076.33080807973,
520.503945350285));
#113148=CARTESIAN_POINT('Ctrl Pts',(-14.465315504119,1076.32030516021,520.649085801352));
#113149=CARTESIAN_POINT('Ctrl Pts',(-14.5300989395078,1076.3155711368,520.710912154196));
#113150=CARTESIAN_POINT('Ctrl Pts',(-14.6797494835211,1076.30774429653,
520.805899496244));
#113151=CARTESIAN_POINT('Ctrl Pts',(-14.7631174696826,1076.30472505357,
520.838202974895));
#113152=CARTESIAN_POINT('Ctrl Pts',(-14.8889629914079,1076.30194121674,
520.860258709262));
#113153=CARTESIAN_POINT('Ctrl Pts',(-14.9279773035416,1076.30130785838,
520.863636077531));
#113154=CARTESIAN_POINT('Ctrl Pts',(-14.9669751953831,1076.30090002967,
520.863636077531));
#113155=CARTESIAN_POINT('Origin',(-27.6354521170191,1067.7251047501,525.785329554474));
#113156=CARTESIAN_POINT('',(-27.6354521170396,1075.76324447263,524.686498418482));
#113157=CARTESIAN_POINT('',(-27.6354521170191,1067.7251047501,524.686498418482));
#113158=CARTESIAN_POINT('Ctrl Pts',(-27.6354652325881,1075.54255375362,
526.884160690388));
#113159=CARTESIAN_POINT('Ctrl Pts',(-27.7787046764732,1075.53848270391,
526.884158980693));
#113160=CARTESIAN_POINT('Ctrl Pts',(-27.9205917190107,1075.53736076137,
526.856149463651));
#113161=CARTESIAN_POINT('Ctrl Pts',(-28.1854094989536,1075.54116058917,
526.747323595548));
#113162=CARTESIAN_POINT('Ctrl Pts',(-28.3057312819153,1075.54603270978,
526.667690377292));
#113163=CARTESIAN_POINT('Ctrl Pts',(-28.5094053471864,1075.56111303089,
526.466639419499));
#113164=CARTESIAN_POINT('Ctrl Pts',(-28.5906269865123,1075.57118904213,
526.347055459459));
#113165=CARTESIAN_POINT('Ctrl Pts',(-28.7029706979218,1075.59518245946,
526.082924025914));
#113166=CARTESIAN_POINT('Ctrl Pts',(-28.7326929653438,1075.60889119952,
525.940755182517));
#113167=CARTESIAN_POINT('Ctrl Pts',(-28.7349881424606,1075.63073750512,
525.724867493293));
#113168=CARTESIAN_POINT('Ctrl Pts',(-28.728647938235,1075.63819784828,525.652834322231));
#113169=CARTESIAN_POINT('Ctrl Pts',(-28.7019715325416,1075.65320332144,
525.511192800037));
#113170=CARTESIAN_POINT('Ctrl Pts',(-28.6817206106976,1075.66071353583,
525.4419084292));
#113171=CARTESIAN_POINT('Ctrl Pts',(-28.6002762760136,1075.68317816295,
525.239525837309));
#113172=CARTESIAN_POINT('Ctrl Pts',(-28.5191792744387,1075.69761865733,
525.11609989725));
#113173=CARTESIAN_POINT('Ctrl Pts',(-28.3138232725783,1075.72358285087,
524.908736133025));
#113174=CARTESIAN_POINT('Ctrl Pts',(-28.1918083061117,1075.73487172659,
524.826604577536));
#113175=CARTESIAN_POINT('Ctrl Pts',(-27.9226159359435,1075.7529270516,524.714721275686));
#113176=CARTESIAN_POINT('Ctrl Pts',(-27.7781589010898,1075.7595168294,524.686073495363));
#113177=CARTESIAN_POINT('Ctrl Pts',(-27.486117459956,1075.76714618751,524.686933330395));
#113178=CARTESIAN_POINT('Ctrl Pts',(-27.3415408701877,1075.76810258596,
524.716497676236));
#113179=CARTESIAN_POINT('Ctrl Pts',(-27.0724953047898,1075.764197711,524.830428100375));
#113180=CARTESIAN_POINT('Ctrl Pts',(-26.9507918943143,1075.75937986775,
524.913579353033));
#113181=CARTESIAN_POINT('Ctrl Pts',(-26.7471198413149,1075.74451321898,
525.122343925765));
#113182=CARTESIAN_POINT('Ctrl Pts',(-26.6671944704052,1075.73461570059,
525.245811191617));
#113183=CARTESIAN_POINT('Ctrl Pts',(-26.5599362661046,1075.71088579724,
525.516943428423));
#113184=CARTESIAN_POINT('Ctrl Pts',(-26.5338673749122,1075.69727107743,
525.662008759801));
#113185=CARTESIAN_POINT('Ctrl Pts',(-26.5383155148456,1075.67551881133,
525.879379334709));
#113186=CARTESIAN_POINT('Ctrl Pts',(-26.5467697760468,1075.6681729337,525.950620268285));
#113187=CARTESIAN_POINT('Ctrl Pts',(-26.5774672516633,1075.65328667062,
526.090718627744));
#113188=CARTESIAN_POINT('Ctrl Pts',(-26.5996988288234,1075.6457799459,526.159241031157));
#113189=CARTESIAN_POINT('Ctrl Pts',(-26.6869345144187,1075.62319814399,
526.358993781912));
#113190=CARTESIAN_POINT('Ctrl Pts',(-26.7715637127726,1075.60852924894,
526.47996836697));
#113191=CARTESIAN_POINT('Ctrl Pts',(-26.9820307799952,1075.5821082306,526.68050016929));
#113192=CARTESIAN_POINT('Ctrl Pts',(-27.1053264362455,1075.57057670524,
526.758643785125));
#113193=CARTESIAN_POINT('Ctrl Pts',(-27.3663317956198,1075.55279443144,
526.859213399613));
#113194=CARTESIAN_POINT('Ctrl Pts',(-27.5002648809074,1075.54639632195,
526.88416230413));
#113195=CARTESIAN_POINT('Ctrl Pts',(-27.6354652325881,1075.54255375362,
526.884160690388));
#113196=CARTESIAN_POINT('Origin',(-27.6354521170191,1067.7251047501,525.785329554474));
#113197=CARTESIAN_POINT('',(-27.6354521170191,1075.60488526556,526.284160690467));
#113198=CARTESIAN_POINT('',(-27.6354521170191,1075.70507826342,525.286498418482));
#113199=CARTESIAN_POINT('Ctrl Pts',(-27.6354521170191,1075.60488526556,
526.284160690467));
#113200=CARTESIAN_POINT('Ctrl Pts',(-27.637581719016,1075.60482587619,526.284160690467));
#113201=CARTESIAN_POINT('Ctrl Pts',(-27.6397120058775,1075.60476785828,
526.28414705299));
#113202=CARTESIAN_POINT('Ctrl Pts',(-27.7068531308022,1075.60298317991,
526.283286809497));
#113203=CARTESIAN_POINT('Ctrl Pts',(-27.7710854290312,1075.60257302789,
526.269752069927));
#113204=CARTESIAN_POINT('Ctrl Pts',(-27.8906979085476,1075.60443883698,
526.218808743026));
#113205=CARTESIAN_POINT('Ctrl Pts',(-27.9448925263289,1075.60669375515,
526.181928547868));
#113206=CARTESIAN_POINT('Ctrl Pts',(-28.0362447104239,1075.61358359968,
526.089372519587));
#113207=CARTESIAN_POINT('Ctrl Pts',(-28.0724372738785,1075.61815928623,
526.034536383933));
#113208=CARTESIAN_POINT('Ctrl Pts',(-28.121868734487,1075.62903903416,525.913825428912));
#113209=CARTESIAN_POINT('Ctrl Pts',(-28.134490643121,1075.63524834314,525.849045650563));
#113210=CARTESIAN_POINT('Ctrl Pts',(-28.1341755161321,1075.64514708704,
525.75101151662));
#113211=CARTESIAN_POINT('Ctrl Pts',(-28.1308523712347,1075.64852408539,
525.718391545539));
#113212=CARTESIAN_POINT('Ctrl Pts',(-28.1178815982617,1075.65532165104,
525.654330654986));
#113213=CARTESIAN_POINT('Ctrl Pts',(-28.1082734017101,1075.65872643261,
525.623036102101));
#113214=CARTESIAN_POINT('Ctrl Pts',(-28.0700028005121,1075.66894646184,
525.531504301829));
#113215=CARTESIAN_POINT('Ctrl Pts',(-28.0322844342556,1075.67553482616,
525.47581880527));
#113216=CARTESIAN_POINT('Ctrl Pts',(-27.9373027258572,1075.68739031963,
525.38268004294));
#113217=CARTESIAN_POINT('Ctrl Pts',(-27.8810450351777,1075.69254604396,
525.346077979356));
#113218=CARTESIAN_POINT('Ctrl Pts',(-27.760754306957,1075.7005204626,525.298416886474));
#113219=CARTESIAN_POINT('Ctrl Pts',(-27.6984115041873,1075.70337998349,
525.286498576198));
#113220=CARTESIAN_POINT('Ctrl Pts',(-27.6354533666297,1075.70507822971,
525.286498418483));
#113221=CARTESIAN_POINT('',(-27.6354521170191,1082.7251047501,525.286498418482));
#113222=CARTESIAN_POINT('',(-27.6354521170191,1067.7251047501,525.286498418482));
#113223=CARTESIAN_POINT('Origin',(-27.6354521170191,1082.7251047501,525.785329554474));
#113224=CARTESIAN_POINT('Ctrl Pts',(-27.6354521170192,1075.70507826342,
525.286498418482));
#113225=CARTESIAN_POINT('Ctrl Pts',(-27.5704411122387,1075.70683186801,
525.286498418482));
#113226=CARTESIAN_POINT('Ctrl Pts',(-27.5060446831974,1075.70731322558,
525.299207181009));
#113227=CARTESIAN_POINT('Ctrl Pts',(-27.3857177316477,1075.70567854251,
525.348640197058));
#113228=CARTESIAN_POINT('Ctrl Pts',(-27.330991362886,1075.70357758552,525.384881156227));
#113229=CARTESIAN_POINT('Ctrl Pts',(-27.2374708795837,1075.6969610597,525.477323575225));
#113230=CARTESIAN_POINT('Ctrl Pts',(-27.2000417531703,1075.69245724965,
525.533025441205));
#113231=CARTESIAN_POINT('Ctrl Pts',(-27.1491348021389,1075.68163327302,
525.655863927699));
#113232=CARTESIAN_POINT('Ctrl Pts',(-27.1362363999838,1075.67541537829,
525.721805829603));
#113233=CARTESIAN_POINT('Ctrl Pts',(-27.1368224186861,1075.66549628098,
525.820850957811));
#113234=CARTESIAN_POINT('Ctrl Pts',(-27.1402045434783,1075.66215223877,
525.853317933819));
#113235=CARTESIAN_POINT('Ctrl Pts',(-27.1532576068827,1075.65538745492,
525.917183579509));
#113236=CARTESIAN_POINT('Ctrl Pts',(-27.1629115826284,1075.65198218319,
525.948432418141));
#113237=CARTESIAN_POINT('Ctrl Pts',(-27.2014706749091,1075.64168178599,
526.040227892965));
#113238=CARTESIAN_POINT('Ctrl Pts',(-27.2395677639214,1075.63498222398,
526.096133854981));
#113239=CARTESIAN_POINT('Ctrl Pts',(-27.3345534635558,1075.62299136117,
526.188546074565));
#113240=CARTESIAN_POINT('Ctrl Pts',(-27.3900931550745,1075.61778677211,
526.224578420605));
#113241=CARTESIAN_POINT('Ctrl Pts',(-27.5097210762046,1075.60961542773,
526.272163085955));
#113242=CARTESIAN_POINT('Ctrl Pts',(-27.5722853209087,1075.60664683237,
526.284160690467));
#113243=CARTESIAN_POINT('Ctrl Pts',(-27.6354521170191,1075.60488526556,
526.284160690467));
#113244=CARTESIAN_POINT('Origin',(-41.3143294401472,1067.7251047501,528.704622312801));
#113245=CARTESIAN_POINT('',(-41.314329440147,1074.93718437437,527.614081564072));
#113246=CARTESIAN_POINT('',(-41.3143294401472,1067.7251047501,527.614081564072));
#113247=CARTESIAN_POINT('Ctrl Pts',(-41.3147349368617,1074.66272114928,
529.795162986141));
#113248=CARTESIAN_POINT('Ctrl Pts',(-41.4565839003635,1074.65548636531,
529.795110242314));
#113249=CARTESIAN_POINT('Ctrl Pts',(-41.5971570089355,1074.65186733571,
529.767382442196));
#113250=CARTESIAN_POINT('Ctrl Pts',(-41.8594095745204,1074.6523287955,529.659704010895));
#113251=CARTESIAN_POINT('Ctrl Pts',(-41.9784831358845,1074.65637448485,
529.581057138748));
#113252=CARTESIAN_POINT('Ctrl Pts',(-42.1803317397281,1074.67161051664,
529.382452429747));
#113253=CARTESIAN_POINT('Ctrl Pts',(-42.2609179997288,1074.68267674667,
529.264316016156));
#113254=CARTESIAN_POINT('Ctrl Pts',(-42.3729390913502,1074.71042386179,
529.00300705716));
#113255=CARTESIAN_POINT('Ctrl Pts',(-42.4027939265198,1074.72688791419,
528.862132421517));
#113256=CARTESIAN_POINT('Ctrl Pts',(-42.4067926729944,1074.76336581939,
528.573317249071));
#113257=CARTESIAN_POINT('Ctrl Pts',(-42.3793156828108,1074.78311131342,
528.428083368655));
#113258=CARTESIAN_POINT('Ctrl Pts',(-42.26924765968,1074.822552856,528.158298115756));
#113259=CARTESIAN_POINT('Ctrl Pts',(-42.1881133129265,1074.84187982289,
528.036113619881));
#113260=CARTESIAN_POINT('Ctrl Pts',(-41.9832034495463,1074.87754647936,
527.831273672055));
#113261=CARTESIAN_POINT('Ctrl Pts',(-41.8616520587045,1074.89356728745,
527.75031640009));
#113262=CARTESIAN_POINT('Ctrl Pts',(-41.5937742418405,1074.9202727164,527.640618985392));
#113263=CARTESIAN_POINT('Ctrl Pts',(-41.4501718347894,1074.93070054373,
527.612897211704));
#113264=CARTESIAN_POINT('Ctrl Pts',(-41.1634517280726,1074.94439594919,
527.61531515592));
#113265=CARTESIAN_POINT('Ctrl Pts',(-41.0232724842316,1074.94768751226,
527.644111186203));
#113266=CARTESIAN_POINT('Ctrl Pts',(-40.7617525825489,1074.94696346259,
527.753815837843));
#113267=CARTESIAN_POINT('Ctrl Pts',(-40.6430599502034,1074.94295948973,
527.833577653202));
#113268=CARTESIAN_POINT('Ctrl Pts',(-40.4423049032428,1074.92805447489,
528.034446428386));
#113269=CARTESIAN_POINT('Ctrl Pts',(-40.3624894630061,1074.91726146972,
528.153766950873));
#113270=CARTESIAN_POINT('Ctrl Pts',(-40.2520633692188,1074.88993585858,
528.418517953024));
#113271=CARTESIAN_POINT('Ctrl Pts',(-40.2235815203424,1074.87356315,528.561774659589));
#113272=CARTESIAN_POINT('Ctrl Pts',(-40.2238920221908,1074.84669833597,
528.777049214715));
#113273=CARTESIAN_POINT('Ctrl Pts',(-40.2308990529131,1074.83752097588,
528.847689597252));
#113274=CARTESIAN_POINT('Ctrl Pts',(-40.2585333116757,1074.81871742584,
528.986791992705));
#113275=CARTESIAN_POINT('Ctrl Pts',(-40.2791468108806,1074.80913181389,
529.054934175923));
#113276=CARTESIAN_POINT('Ctrl Pts',(-40.3620343381846,1074.77970044653,
529.255819191466));
#113277=CARTESIAN_POINT('Ctrl Pts',(-40.4445223765027,1074.76002862967,
529.378546440448));
#113278=CARTESIAN_POINT('Ctrl Pts',(-40.6512227926117,1074.72372088479,
529.582245716887));
#113279=CARTESIAN_POINT('Ctrl Pts',(-40.7726856396383,1074.70737583042,
529.662059071412));
#113280=CARTESIAN_POINT('Ctrl Pts',(-41.0359626757278,1074.68040361457,
529.768254314931));
#113281=CARTESIAN_POINT('Ctrl Pts',(-41.1745848054429,1074.66986928699,
529.79521509829));
#113282=CARTESIAN_POINT('Ctrl Pts',(-41.3147349368616,1074.66272114928,
529.795162986141));
#113283=CARTESIAN_POINT('Origin',(-41.3143294401472,1067.7251047501,528.704622312801));
#113284=CARTESIAN_POINT('',(-41.3143294401472,1074.74003968768,529.195163061529));
#113285=CARTESIAN_POINT('',(-41.3143294401478,1074.86349252611,528.214081564072));
#113286=CARTESIAN_POINT('Ctrl Pts',(-41.3143294401473,1074.74003968768,
529.195163061529));
#113287=CARTESIAN_POINT('Ctrl Pts',(-41.3149650648345,1074.74000762129,
529.195163061529));
#113288=CARTESIAN_POINT('Ctrl Pts',(-41.315600759631,1074.73997570815,529.1951618261));
#113289=CARTESIAN_POINT('Ctrl Pts',(-41.3800205074441,1074.7367576039,529.194911378812));
#113290=CARTESIAN_POINT('Ctrl Pts',(-41.4431861274814,1074.73518157134,
529.18222505377));
#113291=CARTESIAN_POINT('Ctrl Pts',(-41.5609956021098,1074.735445482,529.133387891354));
#113292=CARTESIAN_POINT('Ctrl Pts',(-41.6144628987129,1074.73727251931,
529.097805368761));
#113293=CARTESIAN_POINT('Ctrl Pts',(-41.7050067635757,1074.74410843458,
529.008075075171));
#113294=CARTESIAN_POINT('Ctrl Pts',(-41.7410924447216,1074.74906329865,
528.954742912866));
#113295=CARTESIAN_POINT('Ctrl Pts',(-41.7910608480751,1074.76149153383,
528.836887829166));
#113296=CARTESIAN_POINT('Ctrl Pts',(-41.8042382686789,1074.76886763768,
528.773407019333));
#113297=CARTESIAN_POINT('Ctrl Pts',(-41.8054729513215,1074.78521111985,
528.643568446466));
#113298=CARTESIAN_POINT('Ctrl Pts',(-41.792884918473,1074.79405545382,528.578431307186));
#113299=CARTESIAN_POINT('Ctrl Pts',(-41.742954636749,1074.8117951711,528.457257189193));
#113300=CARTESIAN_POINT('Ctrl Pts',(-41.7061682231797,1074.82052396794,
528.402324735324));
#113301=CARTESIAN_POINT('Ctrl Pts',(-41.6132936582189,1074.83667516872,
528.310276378473));
#113302=CARTESIAN_POINT('Ctrl Pts',(-41.5581693039621,1074.84394813471,
528.273974587247));
#113303=CARTESIAN_POINT('Ctrl Pts',(-41.4393192886644,1074.85580739449,
528.226153185481));
#113304=CARTESIAN_POINT('Ctrl Pts',(-41.3771671640389,1074.86038580463,
528.214082208443));
#113305=CARTESIAN_POINT('Ctrl Pts',(-41.3143344706058,1074.8634922774,528.214081564098));
#113306=CARTESIAN_POINT('',(-41.3143294401472,1082.7251047501,528.214081564072));
#113307=CARTESIAN_POINT('',(-41.3143294401472,1067.7251047501,528.214081564072));
#113308=CARTESIAN_POINT('Origin',(-41.3143294401472,1082.7251047501,528.704622312801));
#113309=CARTESIAN_POINT('Ctrl Pts',(-41.3143294401492,1074.86349252611,
528.214081564072));
#113310=CARTESIAN_POINT('Ctrl Pts',(-41.2505739327455,1074.8666445416,528.214081564072));
#113311=CARTESIAN_POINT('Ctrl Pts',(-41.1873927330606,1074.86821828261,
528.22650978009));
#113312=CARTESIAN_POINT('Ctrl Pts',(-41.0693622129366,1074.86802962759,
528.274875616737));
#113313=CARTESIAN_POINT('Ctrl Pts',(-41.0157058632845,1074.86627445234,
528.310281568565));
#113314=CARTESIAN_POINT('Ctrl Pts',(-40.9247150070383,1074.85962435634,
528.399785349406));
#113315=CARTESIAN_POINT('Ctrl Pts',(-40.8883875279695,1074.85477936378,
528.453079629283));
#113316=CARTESIAN_POINT('Ctrl Pts',(-40.8375628576031,1074.84245873064,
528.571924129615));
#113317=CARTESIAN_POINT('Ctrl Pts',(-40.8241704833866,1074.83504196565,
528.636556360447));
#113318=CARTESIAN_POINT('Ctrl Pts',(-40.8236135986097,1074.82288413253,
528.733788934864));
#113319=CARTESIAN_POINT('Ctrl Pts',(-40.826557553515,1074.81873561267,528.765690725002));
#113320=CARTESIAN_POINT('Ctrl Pts',(-40.838608761746,1074.81024794443,528.828494391202));
#113321=CARTESIAN_POINT('Ctrl Pts',(-40.8477001013119,1074.80592749524,
528.859253514476));
#113322=CARTESIAN_POINT('Ctrl Pts',(-40.8843820828532,1074.79270684827,
528.949746165404));
#113323=CARTESIAN_POINT('Ctrl Pts',(-40.9210270111728,1074.78389469495,
529.005063318077));
#113324=CARTESIAN_POINT('Ctrl Pts',(-41.0135485047486,1074.76756439382,
529.097556825592));
#113325=CARTESIAN_POINT('Ctrl Pts',(-41.0683544996801,1074.7601897016,529.134028548398));
#113326=CARTESIAN_POINT('Ctrl Pts',(-41.187608901482,1074.74800778374,529.182752351033));
#113327=CARTESIAN_POINT('Ctrl Pts',(-41.2506169667632,1074.74325389345,
529.195163061529));
#113328=CARTESIAN_POINT('Ctrl Pts',(-41.3143294401473,1074.74003968768,
529.195163061529));
#113329=CARTESIAN_POINT('Origin',(14.699947805047,1067.7251047501,512.963821085944));
#113330=CARTESIAN_POINT('',(14.6999478050656,1078.7051236444,511.48551795375));
#113331=CARTESIAN_POINT('Ctrl Pts',(14.6998978962583,1078.63014559736,514.442124217295));
#113332=CARTESIAN_POINT('Ctrl Pts',(14.7496044544337,1078.62987399772,514.442125895431));
#113333=CARTESIAN_POINT('Ctrl Pts',(14.7992797757492,1078.62968442711,514.439620569293));
#113334=CARTESIAN_POINT('Ctrl Pts',(14.8867432338949,1078.62949662964,514.430772707963));
#113335=CARTESIAN_POINT('Ctrl Pts',(14.9245886139143,1078.62946433203,514.425455823912));
#113336=CARTESIAN_POINT('Ctrl Pts',(15.0019500580471,1078.62949962489,514.411511448347));
#113337=CARTESIAN_POINT('Ctrl Pts',(15.0414039587513,1078.62957306913,514.402716643483));
#113338=CARTESIAN_POINT('Ctrl Pts',(15.1394856411381,1078.62989562152,514.376591201779));
#113339=CARTESIAN_POINT('Ctrl Pts',(15.1974912031204,1078.63021516986,514.357221000039));
#113340=CARTESIAN_POINT('Ctrl Pts',(15.4035757752251,1078.63182159784,514.273887294396));
#113341=CARTESIAN_POINT('Ctrl Pts',(15.5421258678977,1078.6338279638,514.189421381273));
#113342=CARTESIAN_POINT('Ctrl Pts',(15.7838834832569,1078.63917809705,513.981347624014));
#113343=CARTESIAN_POINT('Ctrl Pts',(15.8862203321114,1078.64245604748,513.859939276477));
#113344=CARTESIAN_POINT('Ctrl Pts',(16.0556452944737,1078.65016884252,513.577701386725));
#113345=CARTESIAN_POINT('Ctrl Pts',(16.1176355195055,1078.65461735318,513.416503796587));
#113346=CARTESIAN_POINT('Ctrl Pts',(16.1859615775165,1078.6641002794,513.068083803391));
#113347=CARTESIAN_POINT('Ctrl Pts',(16.1874129211241,1078.66906717691,512.882845505973));
#113348=CARTESIAN_POINT('Ctrl Pts',(16.1199743296375,1078.67885443951,512.507956087882));
#113349=CARTESIAN_POINT('Ctrl Pts',(16.0465448510673,1078.6835367153,512.322749055966));
#113350=CARTESIAN_POINT('Ctrl Pts',(15.8341517173147,1078.69160227121,511.996423613929));
#113351=CARTESIAN_POINT('Ctrl Pts',(15.6989852787079,1078.69494534877,511.85738138296));
#113352=CARTESIAN_POINT('Ctrl Pts',(15.3932749645222,1078.7001245418,511.645889081803));
#113353=CARTESIAN_POINT('Ctrl Pts',(15.2281463969002,1078.70200751748,511.571464109408));
#113354=CARTESIAN_POINT('Ctrl Pts',(14.9434586716088,1078.70413388698,511.501296026986));
#113355=CARTESIAN_POINT('Ctrl Pts',(14.8304271962009,1078.70471829418,511.486914601018));
#113356=CARTESIAN_POINT('Ctrl Pts',(14.6701871029876,1078.70521821483,511.485080473285));
#113357=CARTESIAN_POINT('Ctrl Pts',(14.6235074471387,1078.70532451767,511.486757652073));
#113358=CARTESIAN_POINT('Ctrl Pts',(14.5422261995786,1078.7054420807,511.493541971162));
#113359=CARTESIAN_POINT('Ctrl Pts',(14.5075803961572,1078.70547052923,511.497672538586));
#113360=CARTESIAN_POINT('Ctrl Pts',(14.4357582627616,1078.70548442937,511.508825184092));
#113361=CARTESIAN_POINT('Ctrl Pts',(14.3986395576713,1078.70546607648,511.516056420283));
#113362=CARTESIAN_POINT('Ctrl Pts',(14.3125787790289,1078.70536324443,511.536275676784));
#113363=CARTESIAN_POINT('Ctrl Pts',(14.2639453551362,1078.70525857253,511.550370519949));
#113364=CARTESIAN_POINT('Ctrl Pts',(14.1147636199825,1078.70478791188,511.602040062133));
#113365=CARTESIAN_POINT('Ctrl Pts',(14.0175193639402,1078.70426268457,511.648078300942));
#113366=CARTESIAN_POINT('Ctrl Pts',(13.7582214073901,1078.7021689885,511.807378320523));
#113367=CARTESIAN_POINT('Ctrl Pts',(13.6126375009139,1078.70011826636,511.943057109904));
#113368=CARTESIAN_POINT('Ctrl Pts',(13.3993942633451,1078.69491711075,512.240911669003));
#113369=CARTESIAN_POINT('Ctrl Pts',(13.3252263044758,1078.69199545058,512.394459501776));
#113370=CARTESIAN_POINT('Ctrl Pts',(13.2285668949958,1078.68489306036,512.73231598474));
#113371=CARTESIAN_POINT('Ctrl Pts',(13.2112626086718,1078.68068972132,512.915183813181));
#113372=CARTESIAN_POINT('Ctrl Pts',(13.2451812497772,1078.67119428078,513.291373738735));
#113373=CARTESIAN_POINT('Ctrl Pts',(13.3012324075905,1078.66593646387,513.480762428237));
#113374=CARTESIAN_POINT('Ctrl Pts',(13.4826791150468,1078.6555137632,513.824614664237));
#113375=CARTESIAN_POINT('Ctrl Pts',(13.605481449819,1078.65045374298,513.976173883456));
#113376=CARTESIAN_POINT('Ctrl Pts',(13.8908753439773,1078.64178715355,514.213831471779));
#113377=CARTESIAN_POINT('Ctrl Pts',(14.0472891538332,1078.63817437732,514.302167165923));
#113378=CARTESIAN_POINT('Ctrl Pts',(14.3495968267505,1078.63320320409,514.406988811613));
#113379=CARTESIAN_POINT('Ctrl Pts',(14.4895365839382,1078.63156162662,514.433926464569));
#113380=CARTESIAN_POINT('Ctrl Pts',(14.6540613618039,1078.63041344773,514.441589638889));
#113381=CARTESIAN_POINT('Ctrl Pts',(14.6769780156839,1078.63027083297,514.4421234435));
#113382=CARTESIAN_POINT('Ctrl Pts',(14.6998978962583,1078.63014559736,514.442124217295));
#113383=CARTESIAN_POINT('',(14.6999478050287,1076.70479703066,511.48551795375));
#113384=CARTESIAN_POINT('',(14.699947805047,1067.7251047501,511.485517953751));
#113385=CARTESIAN_POINT('Ctrl Pts',(14.7001358865113,1076.6289311992,514.442124206172));
#113386=CARTESIAN_POINT('Ctrl Pts',(14.507008105989,1076.62999761294,514.442148777423));
#113387=CARTESIAN_POINT('Ctrl Pts',(14.3157483578776,1076.63231146501,514.404327824439));
#113388=CARTESIAN_POINT('Ctrl Pts',(13.9587634920547,1076.6389578427,514.25736482587));
#113389=CARTESIAN_POINT('Ctrl Pts',(13.7964514000899,1076.64321875908,514.149693054514));
#113390=CARTESIAN_POINT('Ctrl Pts',(13.5222436425071,1076.65281493507,513.87797884017));
#113391=CARTESIAN_POINT('Ctrl Pts',(13.4130296203176,1076.65805219814,513.716488948897));
#113392=CARTESIAN_POINT('Ctrl Pts',(13.3004013968247,1076.6659230134,513.449597277797));
#113393=CARTESIAN_POINT('Ctrl Pts',(13.2716601826682,1076.66853181555,513.35714476367));
#113394=CARTESIAN_POINT('Ctrl Pts',(13.2326215889435,1076.67363038448,513.167942887925));
#113395=CARTESIAN_POINT('Ctrl Pts',(13.2224206474366,1076.6761078662,513.071646428809));
#113396=CARTESIAN_POINT('Ctrl Pts',(13.2201992174956,1076.68329114308,512.779032057933));
#113397=CARTESIAN_POINT('Ctrl Pts',(13.2577112268904,1076.68758814285,512.584656160735));
#113398=CARTESIAN_POINT('Ctrl Pts',(13.4059486805338,1076.69485270936,512.222925245413));
#113399=CARTESIAN_POINT('Ctrl Pts',(13.5147872705394,1076.69776396805,512.058966000734));
#113400=CARTESIAN_POINT('Ctrl Pts',(13.7900865941845,1076.7021931983,511.782434420035));
#113401=CARTESIAN_POINT('Ctrl Pts',(13.9539504277458,1076.70367307539,511.672692175678));
#113402=CARTESIAN_POINT('Ctrl Pts',(14.3153297364348,1076.70527006636,511.523058786727));
#113403=CARTESIAN_POINT('Ctrl Pts',(14.5093533614346,1076.70537192508,511.48483457621));
#113404=CARTESIAN_POINT('Ctrl Pts',(14.9005962585822,1076.70419215139,511.486218398268));
#113405=CARTESIAN_POINT('Ctrl Pts',(15.0939490284075,1076.70292187599,511.525652441588));
#113406=CARTESIAN_POINT('Ctrl Pts',(15.4536207665189,1076.69892134873,511.677220962288));
#113407=CARTESIAN_POINT('Ctrl Pts',(15.6164807544368,1076.69622620615,511.78767363118));
#113408=CARTESIAN_POINT('Ctrl Pts',(15.8905787292192,1076.68937498994,512.065991252439));
#113409=CARTESIAN_POINT('Ctrl Pts',(15.9988665664837,1076.68527236375,512.231358863645));
#113410=CARTESIAN_POINT('Ctrl Pts',(16.1447883504337,1076.67594711465,512.594781835267));
#113411=CARTESIAN_POINT('Ctrl Pts',(16.1809202016486,1076.67081308396,512.789268333462));
#113412=CARTESIAN_POINT('Ctrl Pts',(16.1753005948981,1076.66025649441,513.179181144081));
#113413=CARTESIAN_POINT('Ctrl Pts',(16.1343164117519,1076.65494289453,513.370804310472));
#113414=CARTESIAN_POINT('Ctrl Pts',(15.9806014887991,1076.6450430403,513.727382427962));
#113415=CARTESIAN_POINT('Ctrl Pts',(15.8693138868247,1076.64056031446,513.888858337136));
#113416=CARTESIAN_POINT('Ctrl Pts',(15.5907757988116,1076.63338473419,514.159425483661));
#113417=CARTESIAN_POINT('Ctrl Pts',(15.4262833660638,1076.63076665523,514.265931546221));
#113418=CARTESIAN_POINT('Ctrl Pts',(15.0722278865958,1076.62805579513,514.406636173868));
#113419=CARTESIAN_POINT('Ctrl Pts',(14.8870272186761,1076.62789922191,514.442100428373));
#113420=CARTESIAN_POINT('Ctrl Pts',(14.7001358865113,1076.6289311992,514.442124206172));
#113421=CARTESIAN_POINT('Origin',(14.699947805047,1067.7251047501,512.963821085944));
#113422=CARTESIAN_POINT('',(14.699947805047,1076.64821521145,513.842124218137));
#113423=CARTESIAN_POINT('',(14.699947805044,1076.69331989119,512.085517953751));
#113424=CARTESIAN_POINT('Ctrl Pts',(14.699947805047,1076.64821521145,513.842124218137));
#113425=CARTESIAN_POINT('Ctrl Pts',(14.5902341892714,1076.64876664723,513.842124218137));
#113426=CARTESIAN_POINT('Ctrl Pts',(14.4814440862202,1076.6499345,513.821566166036));
#113427=CARTESIAN_POINT('Ctrl Pts',(14.2723884424619,1076.65339518764,513.739567009876));
#113428=CARTESIAN_POINT('Ctrl Pts',(14.1747942053337,1076.65570057739,513.677122346968));
#113429=CARTESIAN_POINT('Ctrl Pts',(14.0090981910953,1076.66100818296,513.518195556117));
#113430=CARTESIAN_POINT('Ctrl Pts',(13.9426126809805,1076.66395730214,513.423218232298));
#113431=CARTESIAN_POINT('Ctrl Pts',(13.8731309645065,1076.66850029281,513.265624382355));
#113432=CARTESIAN_POINT('Ctrl Pts',(13.8551785910615,1076.67002381275,513.2109573044));
#113433=CARTESIAN_POINT('Ctrl Pts',(13.8301966195557,1076.67304115965,513.098896023708));
#113434=CARTESIAN_POINT('Ctrl Pts',(13.8232286368745,1076.674527731,513.041770144096));
#113435=CARTESIAN_POINT('Ctrl Pts',(13.8191479878038,1076.67891209652,512.86743340148));
#113436=CARTESIAN_POINT('Ctrl Pts',(13.8397991282349,1076.68162769075,512.751109826172));
#113437=CARTESIAN_POINT('Ctrl Pts',(13.9252803318556,1076.68635655882,512.533848931459));
#113438=CARTESIAN_POINT('Ctrl Pts',(13.98907440702,1076.68832843462,512.435003694698));
#113439=CARTESIAN_POINT('Ctrl Pts',(14.1515572663527,1076.69139454872,512.26792630332));
#113440=CARTESIAN_POINT('Ctrl Pts',(14.2486471533298,1076.69246080991,512.201370193172));
#113441=CARTESIAN_POINT('Ctrl Pts',(14.4632835550863,1076.69363475109,512.109989242052));
#113442=CARTESIAN_POINT('Ctrl Pts',(14.5787157912715,1076.69373093964,512.086129931039));
#113443=CARTESIAN_POINT('Ctrl Pts',(14.696936129852,1076.69333034212,512.085521825869));
#113444=CARTESIAN_POINT('Ctrl Pts',(14.6984420617311,1076.69332515727,512.085517953751));
#113445=CARTESIAN_POINT('Ctrl Pts',(14.6999478050411,1076.69331989119,512.085517953751));
#113446=CARTESIAN_POINT('',(14.699947805047,1082.7251047501,512.085517953751));
#113447=CARTESIAN_POINT('',(14.699947805047,1067.7251047501,512.085517953751));
#113448=CARTESIAN_POINT('Origin',(14.699947805047,1082.7251047501,512.963821085944));
#113449=CARTESIAN_POINT('Ctrl Pts',(14.6999478050411,1076.69331989119,512.08551795375));
#113450=CARTESIAN_POINT('Ctrl Pts',(14.8150174298463,1076.69291745447,512.08551795375));
#113451=CARTESIAN_POINT('Ctrl Pts',(14.9289858052922,1076.69204383407,512.108131785945));
#113452=CARTESIAN_POINT('Ctrl Pts',(15.1430067031942,1076.68935404349,512.196564529957));
#113453=CARTESIAN_POINT('Ctrl Pts',(15.2407356916632,1076.68755084412,512.262016733255));
#113454=CARTESIAN_POINT('Ctrl Pts',(15.4052186375597,1076.68311950555,512.427480302874));
#113455=CARTESIAN_POINT('Ctrl Pts',(15.4702298040019,1076.68053016571,512.525950177848));
#113456=CARTESIAN_POINT('Ctrl Pts',(15.554784697244,1076.6750258843,512.734816095846));
#113457=CARTESIAN_POINT('Ctrl Pts',(15.5765117015373,1076.67219414545,512.842067512456));
#113458=CARTESIAN_POINT('Ctrl Pts',(15.5781507156001,1076.66932269893,512.950553082464));
#113459=CARTESIAN_POINT('Ctrl Pts',(15.5798911289057,1076.66627360751,513.065750220667));
#113460=CARTESIAN_POINT('Ctrl Pts',(15.5589484464421,1076.66323751492,513.180174989549));
#113461=CARTESIAN_POINT('Ctrl Pts',(15.474065251113,1076.65761621789,513.394453181141));
#113462=CARTESIAN_POINT('Ctrl Pts',(15.410929900768,1076.6550880753,513.492224212286));
#113463=CARTESIAN_POINT('Ctrl Pts',(15.2505387101093,1076.65100759029,513.657751439642));
#113464=CARTESIAN_POINT('Ctrl Pts',(15.1548601169707,1076.64949675587,513.723918305029));
#113465=CARTESIAN_POINT('Ctrl Pts',(14.9435839893325,1076.64779756826,513.815460695151));
#113466=CARTESIAN_POINT('Ctrl Pts',(14.8300703324198,1076.64762466531,513.840015801074));
#113467=CARTESIAN_POINT('Ctrl Pts',(14.7100170574461,1076.64816590382,513.842080945559));
#113468=CARTESIAN_POINT('Ctrl Pts',(14.7049814592775,1076.64818991161,513.842124218137));
#113469=CARTESIAN_POINT('Ctrl Pts',(14.699947805047,1076.64821521145,513.842124218137));
#113470=CARTESIAN_POINT('Origin',(5.22978306525629,1067.7251047501,521.211612088867));
#113471=CARTESIAN_POINT('',(5.22978306527375,1078.42681724135,519.93616796773));
#113472=CARTESIAN_POINT('Ctrl Pts',(5.22976567235167,1078.26387350206,522.487056209884));
#113473=CARTESIAN_POINT('Ctrl Pts',(5.26411870576279,1078.26374442239,522.487056678348));
#113474=CARTESIAN_POINT('Ctrl Pts',(5.29845782220942,1078.26371167916,522.485669241599));
#113475=CARTESIAN_POINT('Ctrl Pts',(5.37080415501917,1078.263846266,522.479812496659));
#113476=CARTESIAN_POINT('Ctrl Pts',(5.40875071914021,1078.26403652399,522.475016106612));
#113477=CARTESIAN_POINT('Ctrl Pts',(5.50661975544815,1078.26483891144,522.458147427206));
#113478=CARTESIAN_POINT('Ctrl Pts',(5.56598875477243,1078.26563426326,522.443461796757));
#113479=CARTESIAN_POINT('Ctrl Pts',(5.78523223648911,1078.26974512755,522.372194104605));
#113480=CARTESIAN_POINT('Ctrl Pts',(5.93428652750519,1078.27499035138,522.288231812167));
#113481=CARTESIAN_POINT('Ctrl Pts',(6.16926122574186,1078.28795175423,522.085675624277));
#113482=CARTESIAN_POINT('Ctrl Pts',(6.25995812646026,1078.29501207729,521.976673495429));
#113483=CARTESIAN_POINT('Ctrl Pts',(6.40771455656613,1078.31141104809,521.723822559312));
#113484=CARTESIAN_POINT('Ctrl Pts',(6.46032483203251,1078.32075402018,521.579890482998));
#113485=CARTESIAN_POINT('Ctrl Pts',(6.51426712829598,1078.34078288177,521.269706019815));
#113486=CARTESIAN_POINT('Ctrl Pts',(6.51118749253278,1078.35133335968,521.105399802076));
#113487=CARTESIAN_POINT('Ctrl Pts',(6.44221569650749,1078.37200478621,520.781317782674));
#113488=CARTESIAN_POINT('Ctrl Pts',(6.37482325455214,1078.38189802412,520.625044644336));
#113489=CARTESIAN_POINT('Ctrl Pts',(6.18661662569876,1078.39911299917,520.352774478781));
#113490=CARTESIAN_POINT('Ctrl Pts',(6.06956700635826,1078.4063627812,520.237994042669));
#113491=CARTESIAN_POINT('Ctrl Pts',(5.79905804478788,1078.41785855085,520.058828454279));
#113492=CARTESIAN_POINT('Ctrl Pts',(5.64820256977495,1078.42201393506,519.99590853225));
#113493=CARTESIAN_POINT('Ctrl Pts',(5.42983939844212,1078.42535424372,519.950478556129));
#113494=CARTESIAN_POINT('Ctrl Pts',(5.36928763696347,1078.42601801755,519.942352673398));
#113495=CARTESIAN_POINT('Ctrl Pts',(5.27062000758902,1078.42668331406,519.936260500062));
#113496=CARTESIAN_POINT('Ctrl Pts',(5.23276961374977,1078.4268402678,519.935610335759));
#113497=CARTESIAN_POINT('Ctrl Pts',(5.16100456457109,1078.42695218217,519.937571229624));
#113498=CARTESIAN_POINT('Ctrl Pts',(5.12711364669926,1078.42692617282,519.939853630472));
#113499=CARTESIAN_POINT('Ctrl Pts',(5.05124133802895,1078.42669038935,519.948016191585));
#113500=CARTESIAN_POINT('Ctrl Pts',(5.00938081825521,1078.4264368938,519.954641736164));
#113501=CARTESIAN_POINT('Ctrl Pts',(4.8895661263475,1078.42535140423,519.979775649532));
#113502=CARTESIAN_POINT('Ctrl Pts',(4.81293137931116,1078.4242079663,520.003555250756));
#113503=CARTESIAN_POINT('Ctrl Pts',(4.58267075101719,1078.41932327351,520.099540578291));
#113504=CARTESIAN_POINT('Ctrl Pts',(4.44089451496295,1078.41415836311,520.195207371471));
#113505=CARTESIAN_POINT('Ctrl Pts',(4.22049218825775,1078.40154123029,520.418542072107));
#113506=CARTESIAN_POINT('Ctrl Pts',(4.13725392248797,1078.39462437085,520.537830179254));
#113507=CARTESIAN_POINT('Ctrl Pts',(4.00946983763835,1078.37842393442,520.809327539929));
#113508=CARTESIAN_POINT('Ctrl Pts',(3.96953552233366,1078.369129991,520.961113743919));
#113509=CARTESIAN_POINT('Ctrl Pts',(3.94541821257091,1078.34887208769,521.28291686476));
#113510=CARTESIAN_POINT('Ctrl Pts',(3.96579518517392,1078.33802735926,521.450380534731));
#113511=CARTESIAN_POINT('Ctrl Pts',(4.07008287336911,1078.31687155432,521.768310256668));
#113512=CARTESIAN_POINT('Ctrl Pts',(4.15315534560916,1078.30676716075,521.915686450277));
#113513=CARTESIAN_POINT('Ctrl Pts',(4.36504648521359,1078.28939875751,522.16229956733));
#113514=CARTESIAN_POINT('Ctrl Pts',(4.48900779682275,1078.28215291433,522.261786289363));
#113515=CARTESIAN_POINT('Ctrl Pts',(4.74619359579404,1078.27175418726,522.399410159));
#113516=CARTESIAN_POINT('Ctrl Pts',(4.87363429925156,1078.26821717801,522.443642503963));
#113517=CARTESIAN_POINT('Ctrl Pts',(5.06037071587576,1078.26520873888,522.476976489007));
#113518=CARTESIAN_POINT('Ctrl Pts',(5.11567542033187,1078.26457243175,522.483157480549));
#113519=CARTESIAN_POINT('Ctrl Pts',(5.1907150622956,1078.26405133865,522.486607255741));
#113520=CARTESIAN_POINT('Ctrl Pts',(5.21023899255782,1078.2639468725,522.487055943604));
#113521=CARTESIAN_POINT('Ctrl Pts',(5.22976567235167,1078.26387350206,522.487056209884));
#113522=CARTESIAN_POINT('',(5.22978306523924,1076.42335637261,519.93616796773));
#113523=CARTESIAN_POINT('',(5.22978306525629,1067.7251047501,519.936167967731));
#113524=CARTESIAN_POINT('Ctrl Pts',(5.22980079484193,1076.2587132809,522.487056209879));
#113525=CARTESIAN_POINT('Ctrl Pts',(5.06334132967647,1076.25934481001,522.487058523785));
#113526=CARTESIAN_POINT('Ctrl Pts',(4.89851973416088,1076.26225948526,522.454474761201));
#113527=CARTESIAN_POINT('Ctrl Pts',(4.59076760731962,1076.27222559529,522.327899665305));
#113528=CARTESIAN_POINT('Ctrl Pts',(4.45082336662027,1076.27917657429,522.235143334438));
#113529=CARTESIAN_POINT('Ctrl Pts',(4.21418460098485,1076.29605216036,522.000976871181));
#113530=CARTESIAN_POINT('Ctrl Pts',(4.11987400053696,1076.30581788062,521.861691349361));
#113531=CARTESIAN_POINT('Ctrl Pts',(4.02251851690844,1076.32148184635,521.63141390347));
#113532=CARTESIAN_POINT('Ctrl Pts',(3.99764721524802,1076.32684141485,521.551554199838));
#113533=CARTESIAN_POINT('Ctrl Pts',(3.9638497969926,1076.33765889563,521.388082127266));
#113534=CARTESIAN_POINT('Ctrl Pts',(3.95501449308845,1076.34309116847,521.304854850028));
#113535=CARTESIAN_POINT('Ctrl Pts',(3.95309841160809,1076.35922309317,521.054214952404));
#113536=CARTESIAN_POINT('Ctrl Pts',(3.98469064664019,1076.36958810969,520.888396373723));
#113537=CARTESIAN_POINT('Ctrl Pts',(4.1106920745005,1076.38852965609,520.576876803706));
#113538=CARTESIAN_POINT('Ctrl Pts',(4.20445407101636,1076.39690587049,520.434440461867));
#113539=CARTESIAN_POINT('Ctrl Pts',(4.44186123868912,1076.41059644603,520.194584052986));
#113540=CARTESIAN_POINT('Ctrl Pts',(4.58304544841294,1076.41578739126,520.099437952901));
#113541=CARTESIAN_POINT('Ctrl Pts',(4.89450892846827,1076.42247147271,519.969495721745));
#113542=CARTESIAN_POINT('Ctrl Pts',(5.06170769696453,1076.42389732787,519.936064006097));
#113543=CARTESIAN_POINT('Ctrl Pts',(5.39938269945827,1076.42281054014,519.936272384284));
#113544=CARTESIAN_POINT('Ctrl Pts',(5.56647947264613,1076.42030932585,519.969890272096));
#113545=CARTESIAN_POINT('Ctrl Pts',(5.87772196664879,1076.41157710857,520.100139449533));
#113546=CARTESIAN_POINT('Ctrl Pts',(6.01878590088497,1076.40543149535,520.195426699665));
#113547=CARTESIAN_POINT('Ctrl Pts',(6.25611337178095,1076.39004924351,520.435704605549));
#113548=CARTESIAN_POINT('Ctrl Pts',(6.34983577046797,1076.38094815867,520.578502077093));
#113549=CARTESIAN_POINT('Ctrl Pts',(6.44397685863669,1076.36595130184,520.812380823332));
#113550=CARTESIAN_POINT('Ctrl Pts',(6.46738234656901,1076.36081768811,520.892242468003));
#113551=CARTESIAN_POINT('Ctrl Pts',(6.49858790273712,1076.35021220659,521.05667062681));
#113552=CARTESIAN_POINT('Ctrl Pts',(6.50605498115587,1076.34476192239,521.140893103485));
#113553=CARTESIAN_POINT('Ctrl Pts',(6.50336458026901,1076.32840192542,521.392865411299));
#113554=CARTESIAN_POINT('Ctrl Pts',(6.46854063521812,1076.317569398,521.558538406778));
#113555=CARTESIAN_POINT('Ctrl Pts',(6.33677561685729,1076.29736433717,521.866926855902));
#113556=CARTESIAN_POINT('Ctrl Pts',(6.24111209788622,1076.28819005243,522.00667543937));
#113557=CARTESIAN_POINT('Ctrl Pts',(6.00134838792477,1076.27297537825,522.240916764585));
#113558=CARTESIAN_POINT('Ctrl Pts',(5.85969373012418,1076.26708029017,522.333233951461));
#113559=CARTESIAN_POINT('Ctrl Pts',(5.55335213624406,1076.25966852185,522.4559852736));
#113560=CARTESIAN_POINT('Ctrl Pts',(5.39233178566741,1076.25809665599,522.487053950582));
#113561=CARTESIAN_POINT('Ctrl Pts',(5.22980079484193,1076.2587132809,522.487056209879));
#113562=CARTESIAN_POINT('Origin',(5.22978306525629,1067.7251047501,521.211612088867));
#113563=CARTESIAN_POINT('',(5.22978306525628,1076.30041692086,521.887056210003));
#113564=CARTESIAN_POINT('',(5.22978306525629,1076.38762615333,520.536167967731));
#113565=CARTESIAN_POINT('Ctrl Pts',(5.22978306525629,1076.30041692086,521.887056210003));
#113566=CARTESIAN_POINT('Ctrl Pts',(5.22636307154697,1076.30042942372,521.887056210003));
#113567=CARTESIAN_POINT('Ctrl Pts',(5.22294188876261,1076.30044368456,521.887030235228));
#113568=CARTESIAN_POINT('Ctrl Pts',(5.13132690531383,1076.30087259974,521.885638000346));
#113569=CARTESIAN_POINT('Ctrl Pts',(5.04426484962881,1076.30244826036,521.867036420831));
#113570=CARTESIAN_POINT('Ctrl Pts',(4.88220300795897,1076.30771664338,521.797439252864));
#113571=CARTESIAN_POINT('Ctrl Pts',(4.80878446062561,1076.31135809685,521.747105820346));
#113572=CARTESIAN_POINT('Ctrl Pts',(4.6853157352251,1076.3201938069,521.620985871368));
#113573=CARTESIAN_POINT('Ctrl Pts',(4.63651184212421,1076.32530547997,521.546351967946));
#113574=CARTESIAN_POINT('Ctrl Pts',(4.58690612046484,1076.33353431322,521.423480691079));
#113575=CARTESIAN_POINT('Ctrl Pts',(4.57442202372235,1076.33635337301,521.380964969194));
#113576=CARTESIAN_POINT('Ctrl Pts',(4.55793561504524,1076.34205598278,521.294085861446));
#113577=CARTESIAN_POINT('Ctrl Pts',(4.55397770763807,1076.34492602243,521.249927569434));
#113578=CARTESIAN_POINT('Ctrl Pts',(4.55514010358894,1076.35347245615,521.117123388698));
#113579=CARTESIAN_POINT('Ctrl Pts',(4.57333251787838,1076.35899405347,521.029538666631));
#113580=CARTESIAN_POINT('Ctrl Pts',(4.64300463506706,1076.36914822281,520.865213839047));
#113581=CARTESIAN_POINT('Ctrl Pts',(4.69425883575052,1076.37366755107,520.790273191389));
#113582=CARTESIAN_POINT('Ctrl Pts',(4.82297891891141,1076.38103583083,520.665006597796));
#113583=CARTESIAN_POINT('Ctrl Pts',(4.89908587152979,1076.3838173038,520.615863343598));
#113584=CARTESIAN_POINT('Ctrl Pts',(5.06132194296739,1076.38721072309,520.55206546916));
#113585=CARTESIAN_POINT('Ctrl Pts',(5.14517421313421,1076.38790802239,520.536167967731));
#113586=CARTESIAN_POINT('Ctrl Pts',(5.2297830652563,1076.38762615333,520.536167967731));
#113587=CARTESIAN_POINT('',(5.22978306525629,1082.7251047501,520.536167967731));
#113588=CARTESIAN_POINT('',(5.22978306525629,1067.7251047501,520.536167967731));
#113589=CARTESIAN_POINT('Origin',(5.22978306525629,1082.7251047501,521.211612088867));
#113590=CARTESIAN_POINT('Ctrl Pts',(5.22978353114544,1076.38762615178,520.536167967731));
#113591=CARTESIAN_POINT('Ctrl Pts',(5.31949312756942,1076.38732728611,520.536168029608));
#113592=CARTESIAN_POINT('Ctrl Pts',(5.40829400123085,1076.38593355036,520.554040101875));
#113593=CARTESIAN_POINT('Ctrl Pts',(5.57378252673664,1076.3810882742,520.623438541529));
#113594=CARTESIAN_POINT('Ctrl Pts',(5.64879219423385,1076.37768222906,520.674300510113));
#113595=CARTESIAN_POINT('Ctrl Pts',(5.77476330846205,1076.36923107347,520.802549715811));
#113596=CARTESIAN_POINT('Ctrl Pts',(5.82436604459513,1076.36426296791,520.878752565947));
#113597=CARTESIAN_POINT('Ctrl Pts',(5.87406002213901,1076.35612839439,521.003936693618));
#113598=CARTESIAN_POINT('Ctrl Pts',(5.88638390275323,1076.35333417558,521.047002303802));
#113599=CARTESIAN_POINT('Ctrl Pts',(5.90226938780586,1076.34766152172,521.134506038321));
#113600=CARTESIAN_POINT('Ctrl Pts',(5.90587551991134,1076.34479763704,521.17871891908));
#113601=CARTESIAN_POINT('Ctrl Pts',(5.90364065959751,1076.33619212936,521.311671849643));
#113602=CARTESIAN_POINT('Ctrl Pts',(5.88468608857278,1076.33053182074,521.399237546016));
#113603=CARTESIAN_POINT('Ctrl Pts',(5.81400676365003,1076.32005684067,521.562005230839));
#113604=CARTESIAN_POINT('Ctrl Pts',(5.76298003150811,1076.31534364291,521.635646812019));
#113605=CARTESIAN_POINT('Ctrl Pts',(5.63545941022927,1076.30757189409,521.758873402087));
#113606=CARTESIAN_POINT('Ctrl Pts',(5.56026352919896,1076.30458642456,521.807314975803));
#113607=CARTESIAN_POINT('Ctrl Pts',(5.3988307917615,1076.3008809691,521.871052324356));
#113608=CARTESIAN_POINT('Ctrl Pts',(5.31467323103817,1076.30010657814,521.887056210003));
#113609=CARTESIAN_POINT('Ctrl Pts',(5.22978306525629,1076.30041692086,521.887056210003));
#113610=CARTESIAN_POINT('Origin',(-5.99814689883715,1067.7251047501,529.320363258268));
#113611=CARTESIAN_POINT('',(-5.99814689886821,1075.76695399575,528.221532122276));
#113612=CARTESIAN_POINT('',(-5.99814689883715,1067.7251047501,528.221532122276));
#113613=CARTESIAN_POINT('Ctrl Pts',(-5.99814221872999,1075.53855676448,
530.419194394251));
#113614=CARTESIAN_POINT('Ctrl Pts',(-6.14120201009968,1075.53767312577,
530.419195003567));
#113615=CARTESIAN_POINT('Ctrl Pts',(-6.28284864094654,1075.53981354691,
530.391258873147));
#113616=CARTESIAN_POINT('Ctrl Pts',(-6.5475753084573,1075.54986582568,530.282678498626));
#113617=CARTESIAN_POINT('Ctrl Pts',(-6.66800732574684,1075.5576831081,530.203049841736));
#113618=CARTESIAN_POINT('Ctrl Pts',(-6.8720519362554,1075.5779410052,530.001808475949));
#113619=CARTESIAN_POINT('Ctrl Pts',(-6.95347628374648,1075.59020773967,
529.881918882545));
#113620=CARTESIAN_POINT('Ctrl Pts',(-7.06594680082405,1075.6175154686,529.61710135549));
#113621=CARTESIAN_POINT('Ctrl Pts',(-7.0956189940278,1075.63231181689,529.474535113313));
#113622=CARTESIAN_POINT('Ctrl Pts',(-7.09758769177086,1075.6548203051,529.258453798557));
#113623=CARTESIAN_POINT('Ctrl Pts',(-7.09118015406157,1075.66231536263,
529.18663729525));
#113624=CARTESIAN_POINT('Ctrl Pts',(-7.05063852966411,1075.68470750054,
528.972498566485));
#113625=CARTESIAN_POINT('Ctrl Pts',(-6.99513672767571,1075.69906109191,
528.835785138501));
#113626=CARTESIAN_POINT('Ctrl Pts',(-6.83413894957984,1075.72479847781,
528.592548127098));
#113627=CARTESIAN_POINT('Ctrl Pts',(-6.73045584163645,1075.73594775202,
528.488255337386));
#113628=CARTESIAN_POINT('Ctrl Pts',(-6.48813180567354,1075.75368495786,
528.326076586428));
#113629=CARTESIAN_POINT('Ctrl Pts',(-6.35192389613001,1075.76009563144,
528.269841643617));
#113630=CARTESIAN_POINT('Ctrl Pts',(-6.06508096297714,1075.76733907375,
528.21386801996));
#113631=CARTESIAN_POINT('Ctrl Pts',(-5.91738958264268,1075.76809081394,
528.214787290593));
#113632=CARTESIAN_POINT('Ctrl Pts',(-5.63115141807019,1075.76377400335,
528.274373072617));
#113633=CARTESIAN_POINT('Ctrl Pts',(-5.49555571288412,1075.75875452978,
528.332369224935));
#113634=CARTESIAN_POINT('Ctrl Pts',(-5.25520570932623,1075.74351803806,
528.497730718745));
#113635=CARTESIAN_POINT('Ctrl Pts',(-5.1528562515381,1075.73345837417,528.603363975249));
#113636=CARTESIAN_POINT('Ctrl Pts',(-4.99509660502515,1075.70946886991,
528.848516262205));
#113637=CARTESIAN_POINT('Ctrl Pts',(-4.94140800577116,1075.69576066359,
528.98572124902));
#113638=CARTESIAN_POINT('Ctrl Pts',(-4.90361508272451,1075.67392971182,
529.199742450141));
#113639=CARTESIAN_POINT('Ctrl Pts',(-4.89808675040854,1075.66656836557,
529.271236972101));
#113640=CARTESIAN_POINT('Ctrl Pts',(-4.9010069329658,1075.65167221851,529.414558490779));
#113641=CARTESIAN_POINT('Ctrl Pts',(-4.90950759888245,1075.64417115885,
529.486055197811));
#113642=CARTESIAN_POINT('Ctrl Pts',(-4.95627999852536,1075.6216317123,529.698892705372));
#113643=CARTESIAN_POINT('Ctrl Pts',(-5.01579579578355,1075.6070316305,529.833987059212));
#113644=CARTESIAN_POINT('Ctrl Pts',(-5.18327558174302,1075.58082906822,
530.071537681488));
#113645=CARTESIAN_POINT('Ctrl Pts',(-5.28901001441675,1075.56944370285,
530.172118720282));
#113646=CARTESIAN_POINT('Ctrl Pts',(-5.53287583850086,1075.5514482599,530.326156258603));
#113647=CARTESIAN_POINT('Ctrl Pts',(-5.66840793539604,1075.54498741651,
530.378396404296));
#113648=CARTESIAN_POINT('Ctrl Pts',(-5.87230887821545,1075.53991780616,
530.413779398576));
#113649=CARTESIAN_POINT('Ctrl Pts',(-5.93516279572556,1075.53894577005,
530.419194126011));
#113650=CARTESIAN_POINT('Ctrl Pts',(-5.99814221873,1075.53855676448,530.419194394251));
#113651=CARTESIAN_POINT('Origin',(-5.99814689883715,1067.7251047501,529.320363258268));
#113652=CARTESIAN_POINT('',(-5.99814689883715,1075.60310529676,529.819194394261));
#113653=CARTESIAN_POINT('',(-5.99814689883715,1075.70679891916,528.821532122276));
#113654=CARTESIAN_POINT('Ctrl Pts',(-5.99814689883716,1075.60310529676,
529.819194394261));
#113655=CARTESIAN_POINT('Ctrl Pts',(-6.03252410608921,1075.60289709975,
529.819194394261));
#113656=CARTESIAN_POINT('Ctrl Pts',(-6.0668923489677,1075.60306468037,529.815640697523));
#113657=CARTESIAN_POINT('Ctrl Pts',(-6.16429428135216,1075.60463756082,
529.79517970399));
#113658=CARTESIAN_POINT('Ctrl Pts',(-6.22462787047192,1075.60698346613,
529.769530387408));
#113659=CARTESIAN_POINT('Ctrl Pts',(-6.33224176667914,1075.61403827695,
529.696474753279));
#113660=CARTESIAN_POINT('Ctrl Pts',(-6.37840974236614,1075.61868677132,
529.649699848775));
#113661=CARTESIAN_POINT('Ctrl Pts',(-6.45036121560613,1075.6296835713,529.540855683966));
#113662=CARTESIAN_POINT('Ctrl Pts',(-6.47532694324519,1075.6359358906,529.479740397663));
#113663=CARTESIAN_POINT('Ctrl Pts',(-6.49404293736756,1075.6458684236,529.38351500831));
#113664=CARTESIAN_POINT('Ctrl Pts',(-6.49711397960339,1075.64924946972,
529.350896666296));
#113665=CARTESIAN_POINT('Ctrl Pts',(-6.49683309921706,1075.65604511042,
529.285593986273));
#113666=CARTESIAN_POINT('Ctrl Pts',(-6.49349267468341,1075.65944396227,
529.253060472506));
#113667=CARTESIAN_POINT('Ctrl Pts',(-6.47376400397003,1075.66963383704,
529.155915340796));
#113668=CARTESIAN_POINT('Ctrl Pts',(-6.44762122171576,1075.67618441246,
529.094002601275));
#113669=CARTESIAN_POINT('Ctrl Pts',(-6.37262348355696,1075.68793821837,
528.984198403479));
#113670=CARTESIAN_POINT('Ctrl Pts',(-6.32457509952072,1075.69303023553,
528.937346833578));
#113671=CARTESIAN_POINT('Ctrl Pts',(-6.21340227194694,1075.70103774583,
528.865579339296));
#113672=CARTESIAN_POINT('Ctrl Pts',(-6.15155160596148,1075.70389643969,
528.841152365395));
#113673=CARTESIAN_POINT('Ctrl Pts',(-6.05747564078982,1075.70618097767,
528.824183865406));
#113674=CARTESIAN_POINT('Ctrl Pts',(-6.02784296238916,1075.70662516651,
528.821532122276));
#113675=CARTESIAN_POINT('Ctrl Pts',(-5.99814689883715,1075.70679891916,
528.821532122276));
#113676=CARTESIAN_POINT('',(-5.99814689883715,1082.7251047501,528.821532122276));
#113677=CARTESIAN_POINT('',(-5.99814689883715,1067.7251047501,528.821532122276));
#113678=CARTESIAN_POINT('Origin',(-5.99814689883715,1082.7251047501,529.320363258268));
#113679=CARTESIAN_POINT('Ctrl Pts',(-5.99814673263117,1075.70679892014,
528.821532122276));
#113680=CARTESIAN_POINT('Ctrl Pts',(-5.93313362101752,1075.70717931179,
528.821532143938));
#113681=CARTESIAN_POINT('Ctrl Pts',(-5.86876118686279,1075.70625867822,
528.834241700176));
#113682=CARTESIAN_POINT('Ctrl Pts',(-5.74837980993453,1075.70190989668,
528.88367758071));
#113683=CARTESIAN_POINT('Ctrl Pts',(-5.69359049502711,1075.69851786768,
528.91997694178));
#113684=CARTESIAN_POINT('Ctrl Pts',(-5.60005316507632,1075.68957579206,
529.012501767536));
#113685=CARTESIAN_POINT('Ctrl Pts',(-5.56264141879102,1075.68406867106,
529.068221741975));
#113686=CARTESIAN_POINT('Ctrl Pts',(-5.51176420879098,1075.67169092605,
529.191122729049));
#113687=CARTESIAN_POINT('Ctrl Pts',(-5.49888335354078,1075.66493707847,
529.25713215309));
#113688=CARTESIAN_POINT('Ctrl Pts',(-5.49954408692235,1075.65463529819,
529.356290523305));
#113689=CARTESIAN_POINT('Ctrl Pts',(-5.5029573133427,1075.65123350083,529.388795264001));
#113690=CARTESIAN_POINT('Ctrl Pts',(-5.52297899150482,1075.64095736565,
529.486265039177));
#113691=CARTESIAN_POINT('Ctrl Pts',(-5.54949426896431,1075.63429345119,
529.548463741102));
#113692=CARTESIAN_POINT('Ctrl Pts',(-5.6247105130087,1075.6224060827,529.657507757935));
#113693=CARTESIAN_POINT('Ctrl Pts',(-5.67218601133138,1075.6172679483,529.703622592007));
#113694=CARTESIAN_POINT('Ctrl Pts',(-5.78205417802778,1075.60911836451,
529.774664701286));
#113695=CARTESIAN_POINT('Ctrl Pts',(-5.84327982710687,1075.60617454501,
529.799023140969));
#113696=CARTESIAN_POINT('Ctrl Pts',(-5.93747642234815,1075.60376521422,
529.816427903331));
#113697=CARTESIAN_POINT('Ctrl Pts',(-5.96781514998269,1075.60328899345,
529.819194394261));
#113698=CARTESIAN_POINT('Ctrl Pts',(-5.99814689883716,1075.60310529676,
529.819194394261));
#113699=CARTESIAN_POINT('Origin',(-18.7711528398113,1067.7251047501,535.019860978405));
#113700=CARTESIAN_POINT('',(-18.7711528398381,1074.94531439476,533.929320229677));
#113701=CARTESIAN_POINT('',(-18.7711528398113,1067.7251047501,533.929320229677));
#113702=CARTESIAN_POINT('Ctrl Pts',(-18.7711547684023,1074.65422624396,
536.110401727132));
#113703=CARTESIAN_POINT('Ctrl Pts',(-18.9127131527175,1074.65093863987,
536.11040147679));
#113704=CARTESIAN_POINT('Ctrl Pts',(-19.0529112739059,1074.65144815089,
536.082839303297));
#113705=CARTESIAN_POINT('Ctrl Pts',(-19.3149494445529,1074.65999650034,
535.975688086813));
#113706=CARTESIAN_POINT('Ctrl Pts',(-19.4341264139645,1074.6679489259,535.89717792505));
#113707=CARTESIAN_POINT('Ctrl Pts',(-19.636505420761,1074.69028812969,535.698608584391));
#113708=CARTESIAN_POINT('Ctrl Pts',(-19.7174230174435,1074.70450182111,
535.580191978784));
#113709=CARTESIAN_POINT('Ctrl Pts',(-19.8298594761071,1074.73735176127,
535.318125738536));
#113710=CARTESIAN_POINT('Ctrl Pts',(-19.8597900299775,1074.75571916076,
535.176709440408));
#113711=CARTESIAN_POINT('Ctrl Pts',(-19.8634602527513,1074.79438921212,
534.887640108292));
#113712=CARTESIAN_POINT('Ctrl Pts',(-19.8359479568745,1074.81435732531,
534.742657657127));
#113713=CARTESIAN_POINT('Ctrl Pts',(-19.7258905597185,1074.85260860472,
534.473289331668));
#113714=CARTESIAN_POINT('Ctrl Pts',(-19.6448535671405,1074.8705466394,534.351265782043));
#113715=CARTESIAN_POINT('Ctrl Pts',(-19.4400133171832,1074.90207526721,
534.146502177501));
#113716=CARTESIAN_POINT('Ctrl Pts',(-19.3184540089299,1074.91538485099,
534.065539747917));
#113717=CARTESIAN_POINT('Ctrl Pts',(-19.0505079984785,1074.93567743386,
533.955827468364));
#113718=CARTESIAN_POINT('Ctrl Pts',(-18.9069088925942,1074.94246286451,
533.92813471574));
#113719=CARTESIAN_POINT('Ctrl Pts',(-18.6203036704244,1074.94849365463,
533.930555427321));
#113720=CARTESIAN_POINT('Ctrl Pts',(-18.4802603852379,1074.94784777991,
533.959335194944));
#113721=CARTESIAN_POINT('Ctrl Pts',(-18.2186702056287,1074.93936104051,
534.068960620253));
#113722=CARTESIAN_POINT('Ctrl Pts',(-18.0998305093355,1074.9315850408,534.148839297154));
#113723=CARTESIAN_POINT('Ctrl Pts',(-17.897283572241,1074.90957296588,534.351561473377));
#113724=CARTESIAN_POINT('Ctrl Pts',(-17.8165022098086,1074.89541815361,
534.473257285375));
#113725=CARTESIAN_POINT('Ctrl Pts',(-17.7067821425449,1074.8625410088,534.741437244337));
#113726=CARTESIAN_POINT('Ctrl Pts',(-17.6792550977401,1074.84411004723,
534.885446175479));
#113727=CARTESIAN_POINT('Ctrl Pts',(-17.6813553440007,1074.81530924104,
535.101679459));
#113728=CARTESIAN_POINT('Ctrl Pts',(-17.6890237594445,1074.80567512096,
535.172656662161));
#113729=CARTESIAN_POINT('Ctrl Pts',(-17.7334786396821,1074.7761677942,535.385953587735));
#113730=CARTESIAN_POINT('Ctrl Pts',(-17.7920876144873,1074.75654137926,
535.522139528844));
#113731=CARTESIAN_POINT('Ctrl Pts',(-17.9580613663079,1074.72056985167,
535.760683714768));
#113732=CARTESIAN_POINT('Ctrl Pts',(-18.0627989601439,1074.70450255018,
535.861468498097));
#113733=CARTESIAN_POINT('Ctrl Pts',(-18.3046595839089,1074.67794315162,
536.015874947154));
#113734=CARTESIAN_POINT('Ctrl Pts',(-18.439095365224,1074.66765942824,536.068441902923));
#113735=CARTESIAN_POINT('Ctrl Pts',(-18.6431240172495,1074.65797102832,
536.104752084804));
#113736=CARTESIAN_POINT('Ctrl Pts',(-18.7070637566873,1074.65571471724,
536.110401840475));
#113737=CARTESIAN_POINT('Ctrl Pts',(-18.7711547684023,1074.65422624396,
536.110401727132));
#113738=CARTESIAN_POINT('Origin',(-18.7711528398113,1067.7251047501,535.019860978405));
#113739=CARTESIAN_POINT('',(-18.7711528398113,1074.73625576269,535.510401727133));
#113740=CARTESIAN_POINT('',(-18.7711528398123,1074.86719845859,534.529320229677));
#113741=CARTESIAN_POINT('Ctrl Pts',(-18.7711528398114,1074.73625576269,
535.510401727133));
#113742=CARTESIAN_POINT('Ctrl Pts',(-18.8052066733967,1074.73547473995,
535.510401727133));
#113743=CARTESIAN_POINT('Ctrl Pts',(-18.8392574174682,1074.73517201613,
535.506855701214));
#113744=CARTESIAN_POINT('Ctrl Pts',(-18.9350338741057,1074.73571041669,
535.486580018099));
#113745=CARTESIAN_POINT('Ctrl Pts',(-18.9941097748032,1074.73775213253,
535.461405442099));
#113746=CARTESIAN_POINT('Ctrl Pts',(-19.0995598509404,1074.74498546157,
535.389808231347));
#113747=CARTESIAN_POINT('Ctrl Pts',(-19.1448107129023,1074.75011964075,
535.344000007114));
#113748=CARTESIAN_POINT('Ctrl Pts',(-19.2155424766701,1074.76284773375,
535.237311807002));
#113749=CARTESIAN_POINT('Ctrl Pts',(-19.2401396458003,1074.77034151344,
535.177322032859));
#113750=CARTESIAN_POINT('Ctrl Pts',(-19.2587048565978,1074.78258398033,
535.082793576055));
#113751=CARTESIAN_POINT('Ctrl Pts',(-19.261781551059,1074.78681388689,535.050669961364));
#113752=CARTESIAN_POINT('Ctrl Pts',(-19.2616018415929,1074.79542137452,
534.98632695665));
#113753=CARTESIAN_POINT('Ctrl Pts',(-19.258348824959,1074.79977944901,534.954252870605));
#113754=CARTESIAN_POINT('Ctrl Pts',(-19.2390031904703,1074.81299654071,
534.858484243277));
#113755=CARTESIAN_POINT('Ctrl Pts',(-19.2132684912105,1074.82170607306,
534.797434470212));
#113756=CARTESIAN_POINT('Ctrl Pts',(-19.1394197922584,1074.83774227509,
534.689294666574));
#113757=CARTESIAN_POINT('Ctrl Pts',(-19.0921328220124,1074.84492216286,
534.643172922295));
#113758=CARTESIAN_POINT('Ctrl Pts',(-18.9822466284785,1074.8567815164,534.572280588167));
#113759=CARTESIAN_POINT('Ctrl Pts',(-18.9208165985547,1074.86135101369,
534.548146307163));
#113760=CARTESIAN_POINT('Ctrl Pts',(-18.8282424568846,1074.86558707483,
534.531817674485));
#113761=CARTESIAN_POINT('Ctrl Pts',(-18.7997335851328,1074.86655681678,
534.529320597696));
#113762=CARTESIAN_POINT('Ctrl Pts',(-18.7711591569468,1074.86719831677,
534.529320229717));
#113763=CARTESIAN_POINT('',(-18.7711528398113,1082.7251047501,534.529320229677));
#113764=CARTESIAN_POINT('',(-18.7711528398113,1067.7251047501,534.529320229677));
#113765=CARTESIAN_POINT('Origin',(-18.7711528398113,1082.7251047501,535.019860978405));
#113766=CARTESIAN_POINT('Ctrl Pts',(-18.7711528398145,1074.86719845859,
534.529320229677));
#113767=CARTESIAN_POINT('Ctrl Pts',(-18.7074504788267,1074.86862847736,
534.529320229676));
#113768=CARTESIAN_POINT('Ctrl Pts',(-18.6443653971043,1074.86840674218,
534.541727296054));
#113769=CARTESIAN_POINT('Ctrl Pts',(-18.5263471574557,1074.86468127263,
534.59000816825));
#113770=CARTESIAN_POINT('Ctrl Pts',(-18.4726342372528,1074.86120870885,
534.625436830946));
#113771=CARTESIAN_POINT('Ctrl Pts',(-18.3805410345879,1074.85130297252,
534.715984699392));
#113772=CARTESIAN_POINT('Ctrl Pts',(-18.3435923279513,1074.84489038946,
534.770698752533));
#113773=CARTESIAN_POINT('Ctrl Pts',(-18.2931913483521,1074.83000282662,
534.891464050108));
#113774=CARTESIAN_POINT('Ctrl Pts',(-18.2803538904494,1074.82166400125,
534.95638013702));
#113775=CARTESIAN_POINT('Ctrl Pts',(-18.280744529368,1074.80866099614,535.053908368051));
#113776=CARTESIAN_POINT('Ctrl Pts',(-18.2840201429532,1074.80432025391,
535.085896769819));
#113777=CARTESIAN_POINT('Ctrl Pts',(-18.3034686683672,1074.79107069298,
535.181823794996));
#113778=CARTESIAN_POINT('Ctrl Pts',(-18.3293979746482,1074.78228336716,
535.243077568395));
#113779=CARTESIAN_POINT('Ctrl Pts',(-18.4034963443633,1074.76611618187,
535.351058366833));
#113780=CARTESIAN_POINT('Ctrl Pts',(-18.4506742638047,1074.75887395473,
535.396933453209));
#113781=CARTESIAN_POINT('Ctrl Pts',(-18.5594922362588,1074.74695625201,
535.467015424092));
#113782=CARTESIAN_POINT('Ctrl Pts',(-18.6198148560792,1074.74235630109,
535.490890599223));
#113783=CARTESIAN_POINT('Ctrl Pts',(-18.7122310511654,1074.737965022,535.507747898848));
#113784=CARTESIAN_POINT('Ctrl Pts',(-18.741693101653,1074.73693142012,535.510401727133));
#113785=CARTESIAN_POINT('Ctrl Pts',(-18.7711528398114,1074.73625576269,
535.510401727133));
#113786=CARTESIAN_POINT('Origin',(32.7463814565115,1067.7251047501,507.977010932744));
#113787=CARTESIAN_POINT('',(32.7463814565274,1078.70364178837,506.498707800551));
#113788=CARTESIAN_POINT('Ctrl Pts',(32.746381249705,1078.63286819012,509.455314064938));
#113789=CARTESIAN_POINT('Ctrl Pts',(32.8530883738035,1078.63158555358,509.455314079865));
#113790=CARTESIAN_POINT('Ctrl Pts',(32.9594854661601,1078.63064964346,509.443760592605));
#113791=CARTESIAN_POINT('Ctrl Pts',(33.1088409948913,1078.62984872399,509.410935027859));
#113792=CARTESIAN_POINT('Ctrl Pts',(33.1534811694462,1078.62967771172,509.398905830537));
#113793=CARTESIAN_POINT('Ctrl Pts',(33.2287140077989,1078.62950852055,509.37479878059));
#113794=CARTESIAN_POINT('Ctrl Pts',(33.259601718698,1078.62947461873,509.363755510969));
#113795=CARTESIAN_POINT('Ctrl Pts',(33.3212695661467,1078.6294797426,509.339364625878));
#113796=CARTESIAN_POINT('Ctrl Pts',(33.3520141050007,1078.6295204057,509.325978320393));
#113797=CARTESIAN_POINT('Ctrl Pts',(33.425732677801,1078.62971187988,509.290852331071));
#113798=CARTESIAN_POINT('Ctrl Pts',(33.4681509056471,1078.62990288716,509.268036147716));
#113799=CARTESIAN_POINT('Ctrl Pts',(33.6098471373868,1078.63082348265,509.182650210039));
#113800=CARTESIAN_POINT('Ctrl Pts',(33.7027488741016,1078.63193032042,509.11036813935));
#113801=CARTESIAN_POINT('Ctrl Pts',(33.8919237564726,1078.6353742331,508.923194780199));
#113802=CARTESIAN_POINT('Ctrl Pts',(33.9813026708042,1078.63794233723,508.803143557609));
#113803=CARTESIAN_POINT('Ctrl Pts',(34.1286423123368,1078.64438119282,508.526425675508));
#113804=CARTESIAN_POINT('Ctrl Pts',(34.1812054924937,1078.6483141616,508.369153075442));
#113805=CARTESIAN_POINT('Ctrl Pts',(34.2343278509573,1078.65708324799,508.031074808779));
#113806=CARTESIAN_POINT('Ctrl Pts',(34.2300629419761,1078.66189058216,507.852131119818));
#113807=CARTESIAN_POINT('Ctrl Pts',(34.1557398485126,1078.67172127962,507.491972217516));
#113808=CARTESIAN_POINT('Ctrl Pts',(34.0817114223846,1078.67664045808,507.314852952749));
#113809=CARTESIAN_POINT('Ctrl Pts',(33.8681203401151,1078.6857116655,506.994677135991));
#113810=CARTESIAN_POINT('Ctrl Pts',(33.7291469399183,1078.68975641361,506.855646134404));
#113811=CARTESIAN_POINT('Ctrl Pts',(33.4132955946416,1078.69637206553,506.644772208427));
#113812=CARTESIAN_POINT('Ctrl Pts',(33.2414232158748,1078.69895404166,506.571815420625));
#113813=CARTESIAN_POINT('Ctrl Pts',(32.8835406774432,1078.70283010831,506.493978948077));
#113814=CARTESIAN_POINT('Ctrl Pts',(32.7009432313531,1078.70412328656,506.488342087204));
#113815=CARTESIAN_POINT('Ctrl Pts',(32.4619675773265,1078.70507352566,506.525059311246));
#113816=CARTESIAN_POINT('Ctrl Pts',(32.4026747434072,1078.70524517313,506.537941612906));
#113817=CARTESIAN_POINT('Ctrl Pts',(32.3096229670037,1078.70541410203,506.564239275755));
#113818=CARTESIAN_POINT('Ctrl Pts',(32.2752761156426,1078.70545376003,506.575318564671));
#113819=CARTESIAN_POINT('Ctrl Pts',(32.2116579319089,1078.70548445708,506.598442732447));
#113820=CARTESIAN_POINT('Ctrl Pts',(32.1823008671319,1078.70548089485,506.610192503226));
#113821=CARTESIAN_POINT('Ctrl Pts',(32.117910599325,1078.70543316381,506.638391945824));
#113822=CARTESIAN_POINT('Ctrl Pts',(32.0831007699214,1078.70538011835,506.655294194597));
#113823=CARTESIAN_POINT('Ctrl Pts',(31.985606327637,1078.70515161966,506.707456083407));
#113824=CARTESIAN_POINT('Ctrl Pts',(31.9247770463984,1078.70491063041,506.745948620394));
#113825=CARTESIAN_POINT('Ctrl Pts',(31.708943380727,1078.70365917296,506.905674696418));
#113826=CARTESIAN_POINT('Ctrl Pts',(31.5758116824482,1078.70205794334,507.052997358032));
#113827=CARTESIAN_POINT('Ctrl Pts',(31.3919564298537,1078.69776982583,507.362510617041));
#113828=CARTESIAN_POINT('Ctrl Pts',(31.3323784741342,1078.69533634334,507.51585072257));
#113829=CARTESIAN_POINT('Ctrl Pts',(31.2630177861554,1078.68923740537,507.849126498867));
#113830=CARTESIAN_POINT('Ctrl Pts',(31.2583746304162,1078.68553075635,508.027517520772));
#113831=CARTESIAN_POINT('Ctrl Pts',(31.3143545699072,1078.67691354226,508.390286025321));
#113832=CARTESIAN_POINT('Ctrl Pts',(31.3792849940979,1078.67201134422,508.570760718543));
#113833=CARTESIAN_POINT('Ctrl Pts',(31.5763581202034,1078.66173191473,508.901341125006));
#113834=CARTESIAN_POINT('Ctrl Pts',(31.7082342859328,1078.65644880754,509.047335078825));
#113835=CARTESIAN_POINT('Ctrl Pts',(31.9687314017846,1078.64821972533,509.240919661813));
#113836=CARTESIAN_POINT('Ctrl Pts',(32.0825776875407,1078.64512142271,509.304253367899));
#113837=CARTESIAN_POINT('Ctrl Pts',(32.3761476239361,1078.63836207545,509.42022797339));
#113838=CARTESIAN_POINT('Ctrl Pts',(32.5604272617905,1078.63510338651,509.455314038924));
#113839=CARTESIAN_POINT('Ctrl Pts',(32.746381249705,1078.63286819012,509.455314064938));
#113840=CARTESIAN_POINT('',(32.7463814564926,1076.70329713523,506.498707800551));
#113841=CARTESIAN_POINT('',(32.7463814565115,1067.7251047501,506.498707800551));
#113842=CARTESIAN_POINT('Ctrl Pts',(32.7473303221479,1076.6316750193,509.455313760417));
#113843=CARTESIAN_POINT('Ctrl Pts',(32.5543036171815,1076.63401833412,509.455437656823));
#113844=CARTESIAN_POINT('Ctrl Pts',(32.363125508151,1076.63747722987,509.417754613386));
#113845=CARTESIAN_POINT('Ctrl Pts',(32.0060300173876,1076.64594260234,509.271048238892));
#113846=CARTESIAN_POINT('Ctrl Pts',(31.843551984202,1076.65086126279,509.163410266948));
#113847=CARTESIAN_POINT('Ctrl Pts',(31.5690105217389,1076.6612031598,508.891632046527));
#113848=CARTESIAN_POINT('Ctrl Pts',(31.4596450000888,1076.6665218222,508.73003448844));
#113849=CARTESIAN_POINT('Ctrl Pts',(31.3469010632648,1076.67414465603,508.46298095179));
#113850=CARTESIAN_POINT('Ctrl Pts',(31.3181416154283,1076.67660949418,508.370513264503));
#113851=CARTESIAN_POINT('Ctrl Pts',(31.2590373252825,1076.68373889658,508.084222303228));
#113852=CARTESIAN_POINT('Ctrl Pts',(31.2579203683751,1076.68798848716,507.8865678999));
#113853=CARTESIAN_POINT('Ctrl Pts',(31.3325849906484,1076.6951592245,507.503164611125));
#113854=CARTESIAN_POINT('Ctrl Pts',(31.4072871625381,1076.69802331024,507.321126044623));
#113855=CARTESIAN_POINT('Ctrl Pts',(31.6233655336458,1076.70236155665,506.995967508178));
#113856=CARTESIAN_POINT('Ctrl Pts',(31.7628279883748,1076.70379658765,506.856190921005));
#113857=CARTESIAN_POINT('Ctrl Pts',(32.0885502051469,1076.70530205959,506.638689396146));
#113858=CARTESIAN_POINT('Ctrl Pts',(32.2717140624998,1076.70535737953,506.563314533295));
#113859=CARTESIAN_POINT('Ctrl Pts',(32.6562536171745,1076.70407841855,506.488548271379));
#113860=CARTESIAN_POINT('Ctrl Pts',(32.8537795626229,1076.70275703919,506.489695857962));
#113861=CARTESIAN_POINT('Ctrl Pts',(33.2362057872882,1076.69865085437,506.568666071004));
#113862=CARTESIAN_POINT('Ctrl Pts',(33.4173962178751,1076.6959035228,506.645434850156));
#113863=CARTESIAN_POINT('Ctrl Pts',(33.7401441385592,1076.68895573799,506.865221058208));
#113864=CARTESIAN_POINT('Ctrl Pts',(33.8783610276179,1076.68481087431,507.006313388783));
#113865=CARTESIAN_POINT('Ctrl Pts',(34.0920129432897,1076.67541942983,507.334338046798));
#113866=CARTESIAN_POINT('Ctrl Pts',(34.1652348325223,1076.67026148756,507.518097419006));
#113867=CARTESIAN_POINT('Ctrl Pts',(34.2354602451169,1076.65969232901,507.901645069903));
#113868=CARTESIAN_POINT('Ctrl Pts',(34.2324865839961,1076.65439006213,508.097553038576));
#113869=CARTESIAN_POINT('Ctrl Pts',(34.1510038145265,1076.6445529373,508.477125912479));
#113870=CARTESIAN_POINT('Ctrl Pts',(34.0732448440796,1076.64012091762,508.657101987969));
#113871=CARTESIAN_POINT('Ctrl Pts',(33.8526860802714,1076.63307811178,508.976566882754));
#113872=CARTESIAN_POINT('Ctrl Pts',(33.7120890361442,1076.63054061637,509.112986843496));
#113873=CARTESIAN_POINT('Ctrl Pts',(33.3866049505424,1076.62795519261,509.323474590133));
#113874=CARTESIAN_POINT('Ctrl Pts',(33.2049862459164,1076.62792892676,509.395648404247));
#113875=CARTESIAN_POINT('Ctrl Pts',(32.9264542257899,1076.62974528757,509.447042578769));
#113876=CARTESIAN_POINT('Ctrl Pts',(32.8369865558007,1076.63058660627,509.455256213535));
#113877=CARTESIAN_POINT('Ctrl Pts',(32.7473303221479,1076.6316750193,509.455313760417));
#113878=CARTESIAN_POINT('Origin',(32.7463814565115,1067.7251047501,507.977010932744));
#113879=CARTESIAN_POINT('',(32.7463814565115,1076.64970661189,508.855314064937));
#113880=CARTESIAN_POINT('',(32.7463814541604,1076.69227114044,507.098707800551));
#113881=CARTESIAN_POINT('Ctrl Pts',(32.7463814565115,1076.64970661189,508.855314064937));
#113882=CARTESIAN_POINT('Ctrl Pts',(32.6369671703856,1076.65092157723,508.855314064937));
#113883=CARTESIAN_POINT('Ctrl Pts',(32.5284680697616,1076.65269351219,508.834867999844));
#113884=CARTESIAN_POINT('Ctrl Pts',(32.3195549767455,1076.65718584503,508.753168717285));
#113885=CARTESIAN_POINT('Ctrl Pts',(32.2218529608895,1076.65990155956,508.690781557422));
#113886=CARTESIAN_POINT('Ctrl Pts',(32.0559289775466,1076.66574613851,508.531895820681));
#113887=CARTESIAN_POINT('Ctrl Pts',(31.9893304978876,1076.66881699953,508.4368970313));
#113888=CARTESIAN_POINT('Ctrl Pts',(31.919725082527,1076.67333812372,508.279255429859));
#113889=CARTESIAN_POINT('Ctrl Pts',(31.9017403200052,1076.67482018496,508.224587282085));
#113890=CARTESIAN_POINT('Ctrl Pts',(31.8637451809236,1076.67918147736,508.054559231728));
#113891=CARTESIAN_POINT('Ctrl Pts',(31.8612648616058,1076.68187406866,507.936611800604));
#113892=CARTESIAN_POINT('Ctrl Pts',(31.9025351075754,1076.6865534672,507.707002540313));
#113893=CARTESIAN_POINT('Ctrl Pts',(31.945736976525,1076.68849857901,507.597599996767));
#113894=CARTESIAN_POINT('Ctrl Pts',(32.0724188694461,1076.69150946777,507.401854109998));
#113895=CARTESIAN_POINT('Ctrl Pts',(32.1547058196195,1076.69254664494,507.317501460307));
#113896=CARTESIAN_POINT('Ctrl Pts',(32.3476041347743,1076.69365919543,507.185772822873));
#113897=CARTESIAN_POINT('Ctrl Pts',(32.4563357059021,1076.69372312936,507.139780570975));
#113898=CARTESIAN_POINT('Ctrl Pts',(32.6287768372029,1076.6930768903,507.104613294972));
#113899=CARTESIAN_POINT('Ctrl Pts',(32.687577791763,1076.6927351604,507.098707800866));
#113900=CARTESIAN_POINT('Ctrl Pts',(32.7463814518093,1076.69227114044,507.098707800551));
#113901=CARTESIAN_POINT('',(32.7463814565115,1082.7251047501,507.098707800551));
#113902=CARTESIAN_POINT('',(32.7463814565115,1067.7251047501,507.098707800551));
#113903=CARTESIAN_POINT('Origin',(32.7463814565115,1082.7251047501,507.977010932744));
#113904=CARTESIAN_POINT('Ctrl Pts',(32.7463814518093,1076.69227114044,507.098707800551));
#113905=CARTESIAN_POINT('Ctrl Pts',(32.8037342847657,1076.69181856897,507.098707800244));
#113906=CARTESIAN_POINT('Ctrl Pts',(32.8610896909645,1076.6912496181,507.104325473822));
#113907=CARTESIAN_POINT('Ctrl Pts',(33.0318664443822,1076.6891790374,507.138271654048));
#113908=CARTESIAN_POINT('Ctrl Pts',(33.1404587774664,1076.68734536723,507.183483765153));
#113909=CARTESIAN_POINT('Ctrl Pts',(33.3338825170799,1076.68286219988,507.313771296859));
#113910=CARTESIAN_POINT('Ctrl Pts',(33.4167316120568,1076.68025276808,507.397638929314));
#113911=CARTESIAN_POINT('Ctrl Pts',(33.5445984446936,1076.67452752786,507.592548806499));
#113912=CARTESIAN_POINT('Ctrl Pts',(33.5884622035893,1076.67146883894,507.701583623083));
#113913=CARTESIAN_POINT('Ctrl Pts',(33.6188854603855,1076.66707695697,507.864716278004));
#113914=CARTESIAN_POINT('Ctrl Pts',(33.6238316626777,1076.66576974659,507.914125891656));
#113915=CARTESIAN_POINT('Ctrl Pts',(33.6245835404832,1076.66448388031,507.963688330589));
#113916=CARTESIAN_POINT('Ctrl Pts',(33.6263312369102,1076.66149495858,508.078893350336));
#113917=CARTESIAN_POINT('Ctrl Pts',(33.6053926774398,1076.65866150851,508.193330375199));
#113918=CARTESIAN_POINT('Ctrl Pts',(33.5205254249345,1076.65373818431,508.407583827307));
#113919=CARTESIAN_POINT('Ctrl Pts',(33.457423506089,1076.65169860574,508.505324214213));
#113920=CARTESIAN_POINT('Ctrl Pts',(33.2971618619861,1076.64881045897,508.670773621486));
#113921=CARTESIAN_POINT('Ctrl Pts',(33.2015962164759,1076.64799048993,508.736910425619));
#113922=CARTESIAN_POINT('Ctrl Pts',(32.9905663110002,1076.64774301643,508.828479114546));
#113923=CARTESIAN_POINT('Ctrl Pts',(32.8771803110057,1076.64831579393,508.853090008474));
#113924=CARTESIAN_POINT('Ctrl Pts',(32.7569785132388,1076.64959026502,508.855266137898));
#113925=CARTESIAN_POINT('Ctrl Pts',(32.7516789122271,1076.64964778753,508.855314064937));
#113926=CARTESIAN_POINT('Ctrl Pts',(32.7463814565115,1076.64970661189,508.855314064937));
#113927=CARTESIAN_POINT('Origin',(25.1979747106606,1067.7251047501,518.01352587698));
#113928=CARTESIAN_POINT('',(25.1979747106869,1078.42435733551,516.738081755843));
#113929=CARTESIAN_POINT('Ctrl Pts',(25.1979750950576,1078.26679961873,519.288969998116));
#113930=CARTESIAN_POINT('Ctrl Pts',(25.2538393015146,1078.26579106381,519.288969981279));
#113931=CARTESIAN_POINT('Ctrl Pts',(25.3096465254065,1078.26502788217,519.285299707378));
#113932=CARTESIAN_POINT('Ctrl Pts',(25.4010411064822,1078.26418420223,519.273224544298));
#113933=CARTESIAN_POINT('Ctrl Pts',(25.4368271213489,1078.2639586333,519.266931763596));
#113934=CARTESIAN_POINT('Ctrl Pts',(25.5003877095324,1078.26374726128,519.252933592203));
#113935=CARTESIAN_POINT('Ctrl Pts',(25.5282618165064,1078.26372140327,519.245798388078));
#113936=CARTESIAN_POINT('Ctrl Pts',(25.586444312872,1078.26380940973,519.228788689061));
#113937=CARTESIAN_POINT('Ctrl Pts',(25.6166718909598,1078.2639385447,519.218708420609));
#113938=CARTESIAN_POINT('Ctrl Pts',(25.6945526056013,1078.26449138403,519.189452778603));
#113939=CARTESIAN_POINT('Ctrl Pts',(25.7414790230461,1078.26504649876,519.168513444252));
#113940=CARTESIAN_POINT('Ctrl Pts',(25.9260914974776,1078.26814830043,519.072388647803));
#113941=CARTESIAN_POINT('Ctrl Pts',(26.0505866156886,1078.27241995435,518.974966830462));
#113942=CARTESIAN_POINT('Ctrl Pts',(26.2451124389318,1078.2835438971,518.754541932419));
#113943=CARTESIAN_POINT('Ctrl Pts',(26.318703829592,1078.28993503851,518.637659794602));
#113944=CARTESIAN_POINT('Ctrl Pts',(26.4304963335197,1078.30513914723,518.373966420577));
#113945=CARTESIAN_POINT('Ctrl Pts',(26.4641657543368,1078.31399651465,518.227450752337));
#113946=CARTESIAN_POINT('Ctrl Pts',(26.4799168977178,1078.33333109839,517.918627028371));
#113947=CARTESIAN_POINT('Ctrl Pts',(26.4579020625722,1078.34370757868,517.758650210284));
#113948=CARTESIAN_POINT('Ctrl Pts',(26.3530264885736,1078.36461965783,517.446826788575));
#113949=CARTESIAN_POINT('Ctrl Pts',(26.2678889976152,1078.37492787065,517.298960884281));
#113950=CARTESIAN_POINT('Ctrl Pts',(26.0477565847437,1078.39334316983,517.04826449496));
#113951=CARTESIAN_POINT('Ctrl Pts',(25.9161673302562,1078.40133192517,516.946709932133));
#113952=CARTESIAN_POINT('Ctrl Pts',(25.6296781349704,1078.41405877237,516.803314624226));
#113953=CARTESIAN_POINT('Ctrl Pts',(25.4788848365716,1078.41884855583,516.75969362844));
#113954=CARTESIAN_POINT('Ctrl Pts',(25.2363989338142,1078.4239129098,516.73562992413));
#113955=CARTESIAN_POINT('Ctrl Pts',(25.1481978933723,1078.42523121994,516.736020716809));
#113956=CARTESIAN_POINT('Ctrl Pts',(25.0252452362049,1078.42634945222,516.749327920288));
#113957=CARTESIAN_POINT('Ctrl Pts',(24.9899323035213,1078.42658557129,516.754657184705));
#113958=CARTESIAN_POINT('Ctrl Pts',(24.9287486053121,1078.42684587648,516.766535865982));
#113959=CARTESIAN_POINT('Ctrl Pts',(24.9027734278071,1078.4269085968,516.772428379401));
#113960=CARTESIAN_POINT('Ctrl Pts',(24.8490422379368,1078.42693814154,516.786399794905));
#113961=CARTESIAN_POINT('Ctrl Pts',(24.8213379317463,1078.42689636598,516.79461775101));
#113962=CARTESIAN_POINT('Ctrl Pts',(24.7570842598639,1078.42666449705,516.81607737707));
#113963=CARTESIAN_POINT('Ctrl Pts',(24.7208140096023,1078.42642834775,516.830062793949));
#113964=CARTESIAN_POINT('Ctrl Pts',(24.608458401249,1078.42535811319,516.879391873892));
#113965=CARTESIAN_POINT('Ctrl Pts',(24.5351947032948,1078.42415122644,516.920589534214));
#113966=CARTESIAN_POINT('Ctrl Pts',(24.3276737151788,1078.41910089287,517.065867488017));
#113967=CARTESIAN_POINT('Ctrl Pts',(24.2096353141831,1078.41387644729,517.189734969079));
#113968=CARTESIAN_POINT('Ctrl Pts',(24.0422909167752,1078.40116928911,517.454990295583));
#113969=CARTESIAN_POINT('Ctrl Pts',(23.9865992335089,1078.39422538086,517.589131640078));
#113970=CARTESIAN_POINT('Ctrl Pts',(23.9198634616342,1078.37797480244,517.881485069862));
#113971=CARTESIAN_POINT('Ctrl Pts',(23.9133094938973,1078.36865652168,518.038319665684));
#113972=CARTESIAN_POINT('Ctrl Pts',(23.9586008571845,1078.34835863445,518.358046825016));
#113973=CARTESIAN_POINT('Ctrl Pts',(24.0144221101813,1078.33749956753,518.517454730633));
#113974=CARTESIAN_POINT('Ctrl Pts',(24.1844466729048,1078.316366862,518.805694049332));
#113975=CARTESIAN_POINT('Ctrl Pts',(24.2970534952695,1078.30629829287,518.931753178497));
#113976=CARTESIAN_POINT('Ctrl Pts',(24.5554693101356,1078.28909535356,519.126307262868));
#113977=CARTESIAN_POINT('Ctrl Pts',(24.6963139681842,1078.2819553323,519.196517368932));
#113978=CARTESIAN_POINT('Ctrl Pts',(24.9606808418641,1078.27219239906,519.272329347048));
#113979=CARTESIAN_POINT('Ctrl Pts',(25.0790222205508,1078.26894715674,519.288970033966));
#113980=CARTESIAN_POINT('Ctrl Pts',(25.1979750950576,1078.26679961873,519.288969998116));
#113981=CARTESIAN_POINT('',(25.197974710641,1076.42087024281,516.738081755844));
#113982=CARTESIAN_POINT('',(25.1979747106606,1067.7251047501,516.738081755843));
#113983=CARTESIAN_POINT('Ctrl Pts',(25.1980044361408,1076.26166889074,519.288969997769));
#113984=CARTESIAN_POINT('Ctrl Pts',(25.031537606726,1076.26470468843,519.288973877443));
#113985=CARTESIAN_POINT('Ctrl Pts',(24.8667318546538,1076.26990561849,519.256389121415));
#113986=CARTESIAN_POINT('Ctrl Pts',(24.5587436286835,1076.28389738122,519.129732630649));
#113987=CARTESIAN_POINT('Ctrl Pts',(24.4185795947314,1076.29255534022,519.036772507589));
#113988=CARTESIAN_POINT('Ctrl Pts',(24.1816428518619,1076.31202071232,518.802017551005));
#113989=CARTESIAN_POINT('Ctrl Pts',(24.087263209789,1076.32264379334,518.66233126658));
#113990=CARTESIAN_POINT('Ctrl Pts',(23.9900737635484,1076.33888785251,518.431504929377));
#113991=CARTESIAN_POINT('Ctrl Pts',(23.9653043796319,1076.34431759179,518.351543066889));
#113992=CARTESIAN_POINT('Ctrl Pts',(23.9145150247131,1076.36055618046,518.103859956947));
#113993=CARTESIAN_POINT('Ctrl Pts',(23.9138627054195,1076.37099485117,517.932819995292));
#113994=CARTESIAN_POINT('Ctrl Pts',(23.9792829582952,1076.38983033526,517.601276433598));
#113995=CARTESIAN_POINT('Ctrl Pts',(24.0443684741143,1076.39805683879,517.44397031636));
#113996=CARTESIAN_POINT('Ctrl Pts',(24.232245828346,1076.41144415945,517.163416124712));
#113997=CARTESIAN_POINT('Ctrl Pts',(24.3532884105665,1076.41647058397,517.043032546197));
#113998=CARTESIAN_POINT('Ctrl Pts',(24.6358632193602,1076.42279156108,516.856120911585));
#113999=CARTESIAN_POINT('Ctrl Pts',(24.7946853442826,1076.424012382,516.791673881075));
#114000=CARTESIAN_POINT('Ctrl Pts',(25.1280767874121,1076.42247563035,516.728761698703));
#114001=CARTESIAN_POINT('Ctrl Pts',(25.2992647614757,1076.41973682242,516.730862473475));
#114002=CARTESIAN_POINT('Ctrl Pts',(25.6300874785057,1076.4105383985,516.801692798854));
#114003=CARTESIAN_POINT('Ctrl Pts',(25.7864647294093,1076.40418066329,516.869453557925));
#114004=CARTESIAN_POINT('Ctrl Pts',(26.0637479056959,1076.38845202921,517.061852664176));
#114005=CARTESIAN_POINT('Ctrl Pts',(26.1818977119738,1076.37923043119,517.184609950215));
#114006=CARTESIAN_POINT('Ctrl Pts',(26.3172690778288,1076.36412954347,517.396450065671));
#114007=CARTESIAN_POINT('Ctrl Pts',(26.354924744394,1076.35897736963,517.470326050818));
#114008=CARTESIAN_POINT('Ctrl Pts',(26.4155329911697,1076.34841954437,517.624662810669));
#114009=CARTESIAN_POINT('Ctrl Pts',(26.438274306961,1076.34303766751,517.704789000514));
#114010=CARTESIAN_POINT('Ctrl Pts',(26.4831811410849,1076.32665049629,517.953108160057));
#114011=CARTESIAN_POINT('Ctrl Pts',(26.4798530782244,1076.31575718523,518.124032056819));
#114012=CARTESIAN_POINT('Ctrl Pts',(26.407016890058,1076.29567121162,518.452882314315));
#114013=CARTESIAN_POINT('Ctrl Pts',(26.3389131487456,1076.28665897991,518.607764461718));
#114014=CARTESIAN_POINT('Ctrl Pts',(26.1468440263256,1076.27184899657,518.882070442686));
#114015=CARTESIAN_POINT('Ctrl Pts',(26.0248815138126,1076.26619180919,518.998913384367));
#114016=CARTESIAN_POINT('Ctrl Pts',(25.7431482078447,1076.25919072888,519.17858641003));
#114017=CARTESIAN_POINT('Ctrl Pts',(25.5862626857221,1076.25790385133,519.239830662437));
#114018=CARTESIAN_POINT('Ctrl Pts',(25.3480749433583,1076.25937840023,519.282332473962));
#114019=CARTESIAN_POINT('Ctrl Pts',(25.2731103698183,1076.26029920995,519.288968247352));
#114020=CARTESIAN_POINT('Ctrl Pts',(25.1980044361408,1076.26166889074,519.288969997769));
#114021=CARTESIAN_POINT('Origin',(25.1979747106606,1067.7251047501,518.01352587698));
#114022=CARTESIAN_POINT('',(25.1979747106606,1076.3019258569,518.688969998116));
#114023=CARTESIAN_POINT('',(25.1979747106607,1076.38624898044,517.338081755843));
#114024=CARTESIAN_POINT('Ctrl Pts',(25.1979747106606,1076.3019258569,518.688969998116));
#114025=CARTESIAN_POINT('Ctrl Pts',(25.1506482879843,1076.30275829312,518.688969998116));
#114026=CARTESIAN_POINT('Ctrl Pts',(25.1033458087688,1076.30391372793,518.683995895215));
#114027=CARTESIAN_POINT('Ctrl Pts',(24.9705154872112,1076.30808645208,518.655617822141));
#114028=CARTESIAN_POINT('Ctrl Pts',(24.8886594604942,1076.31179806768,518.620429280826));
#114029=CARTESIAN_POINT('Ctrl Pts',(24.7429745164403,1076.32075060247,518.52049903454));
#114030=CARTESIAN_POINT('Ctrl Pts',(24.6805960922587,1076.3259077255,518.456647167304));
#114031=CARTESIAN_POINT('Ctrl Pts',(24.6081303200936,1076.33417911531,518.345586287252));
#114032=CARTESIAN_POINT('Ctrl Pts',(24.5876614884424,1076.33700701395,518.306267672777));
#114033=CARTESIAN_POINT('Ctrl Pts',(24.5547233750118,1076.34271386765,518.224247033879));
#114034=CARTESIAN_POINT('Ctrl Pts',(24.5423232870404,1076.3455792421,518.181742945173));
#114035=CARTESIAN_POINT('Ctrl Pts',(24.5175462711231,1076.35419315865,518.049961454994));
#114036=CARTESIAN_POINT('Ctrl Pts',(24.5187402570958,1076.3597677743,517.959134452175));
#114037=CARTESIAN_POINT('Ctrl Pts',(24.5566081677011,1076.36987625386,517.783466779294));
#114038=CARTESIAN_POINT('Ctrl Pts',(24.5928209289011,1076.37431376896,517.700349972542));
#114039=CARTESIAN_POINT('Ctrl Pts',(24.6957495694736,1076.38151050216,517.553002240948));
#114040=CARTESIAN_POINT('Ctrl Pts',(24.761473338734,1076.38419657027,517.490277855503));
#114041=CARTESIAN_POINT('Ctrl Pts',(24.913824288656,1076.38747633607,517.394162825976));
#114042=CARTESIAN_POINT('Ctrl Pts',(24.998940634694,1076.38803361555,517.361805249456));
#114043=CARTESIAN_POINT('Ctrl Pts',(25.1242863879005,1076.38725323819,517.34110121662));
#114044=CARTESIAN_POINT('Ctrl Pts',(25.1610987811129,1076.38684187574,517.338081755843));
#114045=CARTESIAN_POINT('Ctrl Pts',(25.1979747106609,1076.38624898044,517.338081755843));
#114046=CARTESIAN_POINT('',(25.1979747106606,1082.7251047501,517.338081755844));
#114047=CARTESIAN_POINT('',(25.1979747106606,1067.7251047501,517.338081755844));
#114048=CARTESIAN_POINT('Origin',(25.1979747106606,1082.7251047501,518.01352587698));
#114049=CARTESIAN_POINT('Ctrl Pts',(25.19797846324,1076.3862489201,517.338081755854));
#114050=CARTESIAN_POINT('Ctrl Pts',(25.2879847978612,1076.38480175833,517.338082255904));
#114051=CARTESIAN_POINT('Ctrl Pts',(25.3770617771146,1076.38229506456,517.356072898381));
#114052=CARTESIAN_POINT('Ctrl Pts',(25.5427548319197,1076.3754154159,517.425803272491));
#114053=CARTESIAN_POINT('Ctrl Pts',(25.6177287943988,1076.37111298612,517.476789791512));
#114054=CARTESIAN_POINT('Ctrl Pts',(25.7434527121999,1076.36121280296,517.605155566688));
#114055=CARTESIAN_POINT('Ctrl Pts',(25.7929021281417,1076.35570964023,517.681312341625));
#114056=CARTESIAN_POINT('Ctrl Pts',(25.842204694364,1076.34714948523,517.805841920776));
#114057=CARTESIAN_POINT('Ctrl Pts',(25.8543735968277,1076.34429679249,517.848282997687));
#114058=CARTESIAN_POINT('Ctrl Pts',(25.8785009286614,1076.33564934978,517.979752579884));
#114059=CARTESIAN_POINT('Ctrl Pts',(25.8769764775005,1076.32994791322,518.070261173533));
#114060=CARTESIAN_POINT('Ctrl Pts',(25.8388866316471,1076.31949889079,518.244415281066));
#114061=CARTESIAN_POINT('Ctrl Pts',(25.8030912747009,1076.31484265673,518.326453675911));
#114062=CARTESIAN_POINT('Ctrl Pts',(25.7019184575798,1076.30720792409,518.471885516939));
#114063=CARTESIAN_POINT('Ctrl Pts',(25.6375923832873,1076.30430091073,518.533910326504));
#114064=CARTESIAN_POINT('Ctrl Pts',(25.4888078416967,1076.30068727313,518.629513160756));
#114065=CARTESIAN_POINT('Ctrl Pts',(25.4058557840819,1076.30001124025,518.66222657909));
#114066=CARTESIAN_POINT('Ctrl Pts',(25.2789384875224,1076.3007382741,518.685332295366));
#114067=CARTESIAN_POINT('Ctrl Pts',(25.2384478437601,1076.30121396489,518.688969998116));
#114068=CARTESIAN_POINT('Ctrl Pts',(25.1979747106606,1076.3019258569,518.688969998116));
#114069=CARTESIAN_POINT('Origin',(15.9013061211262,1067.7251047501,528.279499281495));
#114070=CARTESIAN_POINT('',(15.9013061211524,1077.7757685569,527.180668145503));
#114071=CARTESIAN_POINT('Ctrl Pts',(15.9013326495842,1077.55169183437,529.378330417168));
#114072=CARTESIAN_POINT('Ctrl Pts',(15.9354256569584,1077.55113887753,529.37832959408));
#114073=CARTESIAN_POINT('Ctrl Pts',(15.9695020621221,1077.55075385341,529.376742086929));
#114074=CARTESIAN_POINT('Ctrl Pts',(16.029515268272,1077.55037270998,529.371139118324));
#114075=CARTESIAN_POINT('Ctrl Pts',(16.0554842451758,1077.55030715702,529.367775098043));
#114076=CARTESIAN_POINT('Ctrl Pts',(16.1086468112226,1077.55037833515,529.358947147593));
#114077=CARTESIAN_POINT('Ctrl Pts',(16.1358030166974,1077.55052712521,529.353374972161));
#114078=CARTESIAN_POINT('Ctrl Pts',(16.2035708404945,1077.55118325342,529.336776399701));
#114079=CARTESIAN_POINT('Ctrl Pts',(16.2438107469713,1077.55183579649,529.324434107133));
#114080=CARTESIAN_POINT('Ctrl Pts',(16.3891161115835,1077.55517364205,529.270570068469));
#114081=CARTESIAN_POINT('Ctrl Pts',(16.4882512437389,1077.55941166206,529.215259687026));
#114082=CARTESIAN_POINT('Ctrl Pts',(16.6682412594859,1077.57129161793,529.074846892129));
#114083=CARTESIAN_POINT('Ctrl Pts',(16.747456369472,1077.57893596218,528.989959815292));
#114084=CARTESIAN_POINT('Ctrl Pts',(16.8827256923866,1077.59771871991,528.789625379511));
#114085=CARTESIAN_POINT('Ctrl Pts',(16.9348048549741,1077.60898213919,528.673509045357));
#114086=CARTESIAN_POINT('Ctrl Pts',(16.999660649027,1077.63425695103,528.419360210446));
#114087=CARTESIAN_POINT('Ctrl Pts',(17.0085147312245,1077.64820041578,528.282456567556));
#114088=CARTESIAN_POINT('Ctrl Pts',(16.9746020120754,1077.6773431011,528.00226985882));
#114089=CARTESIAN_POINT('Ctrl Pts',(16.928208735083,1077.69227684009,527.861977254396));
#114090=CARTESIAN_POINT('Ctrl Pts',(16.7846063607034,1077.71980272233,527.61035041876));
#114091=CARTESIAN_POINT('Ctrl Pts',(16.6898083768046,1077.73218082522,527.500836219454));
#114092=CARTESIAN_POINT('Ctrl Pts',(16.4752200190605,1077.75204122725,527.333699230502));
#114093=CARTESIAN_POINT('Ctrl Pts',(16.3607950054836,1077.7597518177,527.273100731741));
#114094=CARTESIAN_POINT('Ctrl Pts',(16.1445012200799,1077.7698800982,527.203386909236));
#114095=CARTESIAN_POINT('Ctrl Pts',(16.0469208706027,1077.77306530005,527.185893563921));
#114096=CARTESIAN_POINT('Ctrl Pts',(15.9076554089286,1077.77574512915,527.179934289773));
#114097=CARTESIAN_POINT('Ctrl Pts',(15.8669595666641,1077.77630629531,527.180452286059));
#114098=CARTESIAN_POINT('Ctrl Pts',(15.7992131197838,1077.77687110405,527.185082288483));
#114099=CARTESIAN_POINT('Ctrl Pts',(15.7721208064804,1077.77699748216,527.187948667648));
#114100=CARTESIAN_POINT('Ctrl Pts',(15.7193785141611,1077.77704836196,527.19552016244));
#114101=CARTESIAN_POINT('Ctrl Pts',(15.6937344163041,1077.77698139936,527.20013727113));
#114102=CARTESIAN_POINT('Ctrl Pts',(15.6340903930987,1077.77660958155,527.213080265684));
#114103=CARTESIAN_POINT('Ctrl Pts',(15.6002773735579,1077.77623122058,527.222127440125));
#114104=CARTESIAN_POINT('Ctrl Pts',(15.495412242424,1077.7745240779,527.255623958176));
#114105=CARTESIAN_POINT('Ctrl Pts',(15.4264180411923,1077.77260781199,527.285745643577));
#114106=CARTESIAN_POINT('Ctrl Pts',(15.2338561401924,1077.76482640166,527.394470233332));
#114107=CARTESIAN_POINT('Ctrl Pts',(15.1223636790291,1077.75702154368,527.49086557591));
#114108=CARTESIAN_POINT('Ctrl Pts',(14.9565098520058,1077.73834614646,527.7047233275));
#114109=CARTESIAN_POINT('Ctrl Pts',(14.8974468985504,1077.72821473454,527.815577532673));
#114110=CARTESIAN_POINT('Ctrl Pts',(14.8158476309181,1077.70479454011,528.061823640231));
#114111=CARTESIAN_POINT('Ctrl Pts',(14.7973756669171,1077.69150865683,528.196429485797));
#114112=CARTESIAN_POINT('Ctrl Pts',(14.8104669248276,1077.66292978698,528.475759623976));
#114113=CARTESIAN_POINT('Ctrl Pts',(14.8458485901493,1077.64783030156,528.617828310167));
#114114=CARTESIAN_POINT('Ctrl Pts',(14.9693941473493,1077.61892051957,528.879297428913));
#114115=CARTESIAN_POINT('Ctrl Pts',(15.0560976649763,1077.60537610607,528.996370963454));
#114116=CARTESIAN_POINT('Ctrl Pts',(15.2617877721368,1077.58260204064,529.182945196387));
#114117=CARTESIAN_POINT('Ctrl Pts',(15.3760890202089,1077.5733101814,529.253876705106));
#114118=CARTESIAN_POINT('Ctrl Pts',(15.6070877152219,1077.56004953077,529.34438782175));
#114119=CARTESIAN_POINT('Ctrl Pts',(15.7196873345586,1077.55559543575,529.369268368028));
#114120=CARTESIAN_POINT('Ctrl Pts',(15.8565206111492,1077.55249107862,529.377645982359));
#114121=CARTESIAN_POINT('Ctrl Pts',(15.8789233143288,1077.55205529292,529.378330958184));
#114122=CARTESIAN_POINT('Ctrl Pts',(15.9013326495842,1077.55169183437,529.378330417168));
#114123=CARTESIAN_POINT('',(15.9013061211098,1075.76586229356,527.180668145503));
#114124=CARTESIAN_POINT('',(15.9013061211262,1067.7251047501,527.180668145503));
#114125=CARTESIAN_POINT('Ctrl Pts',(15.9013205982293,1075.53973398927,529.378330417393));
#114126=CARTESIAN_POINT('Ctrl Pts',(15.7583042502497,1075.54207465006,529.378332301633));
#114127=CARTESIAN_POINT('Ctrl Pts',(15.6167585256812,1075.54737091471,529.350415482922));
#114128=CARTESIAN_POINT('Ctrl Pts',(15.3519511202224,1075.56321196787,529.241887338351));
#114129=CARTESIAN_POINT('Ctrl Pts',(15.2313566414536,1075.57361833005,529.162146819059));
#114130=CARTESIAN_POINT('Ctrl Pts',(15.0270198064597,1075.5981335215,528.960519269506));
#114131=CARTESIAN_POINT('Ctrl Pts',(14.9454746476426,1075.61202853342,528.840293754353));
#114132=CARTESIAN_POINT('Ctrl Pts',(14.8612892957594,1075.63402729201,528.641439964089));
#114133=CARTESIAN_POINT('Ctrl Pts',(14.8397758507011,1075.64151639324,528.572393654757));
#114134=CARTESIAN_POINT('Ctrl Pts',(14.8106159174879,1075.65653838638,528.431201920474));
#114135=CARTESIAN_POINT('Ctrl Pts',(14.8030172675462,1075.66403638592,528.359388136089));
#114136=CARTESIAN_POINT('Ctrl Pts',(14.8014594959151,1075.68639799958,528.141163889383));
#114137=CARTESIAN_POINT('Ctrl Pts',(14.8295960057726,1075.70068345627,527.996135575297));
#114138=CARTESIAN_POINT('Ctrl Pts',(14.9408226164428,1075.7261872287,527.726257167342));
#114139=CARTESIAN_POINT('Ctrl Pts',(15.0225028353466,1075.73717649953,527.603930820679));
#114140=CARTESIAN_POINT('Ctrl Pts',(15.2289890933845,1075.75452775864,527.398229518589));
#114141=CARTESIAN_POINT('Ctrl Pts',(15.3516751352132,1075.76072223674,527.31689178922));
#114142=CARTESIAN_POINT('Ctrl Pts',(15.6219424740288,1075.76751920701,527.206796633006));
#114143=CARTESIAN_POINT('Ctrl Pts',(15.7667576394102,1075.76804937915,527.179209577086));
#114144=CARTESIAN_POINT('Ctrl Pts',(16.0586305848033,1075.7633177527,527.182244737854));
#114145=CARTESIAN_POINT('Ctrl Pts',(16.202679044292,1075.75810682931,527.212803301843));
#114146=CARTESIAN_POINT('Ctrl Pts',(16.4703467320378,1075.74252796372,527.328250825835));
#114147=CARTESIAN_POINT('Ctrl Pts',(16.5912471421057,1075.73231345017,527.411985403997));
#114148=CARTESIAN_POINT('Ctrl Pts',(16.793751260426,1075.70805565276,527.621964298198));
#114149=CARTESIAN_POINT('Ctrl Pts',(16.8731493277795,1075.69423139713,527.74633383078));
#114150=CARTESIAN_POINT('Ctrl Pts',(16.9791153025329,1075.66465804811,528.019792617817));
#114151=CARTESIAN_POINT('Ctrl Pts',(17.0041757197176,1075.64918170966,528.166409856263));
#114152=CARTESIAN_POINT('Ctrl Pts',(16.9951178013447,1075.6190763178,528.458291803031));
#114153=CARTESIAN_POINT('Ctrl Pts',(16.9620684160472,1075.60472218162,528.60079010185));
#114154=CARTESIAN_POINT('Ctrl Pts',(16.8426819748313,1075.57895916141,528.864388687406));
#114155=CARTESIAN_POINT('Ctrl Pts',(16.7576903529827,1075.56778863589,528.983043762542));
#114156=CARTESIAN_POINT('Ctrl Pts',(16.5470403842023,1075.55030847844,529.180124481898));
#114157=CARTESIAN_POINT('Ctrl Pts',(16.4237153657142,1075.54414224892,529.256868179455));
#114158=CARTESIAN_POINT('Ctrl Pts',(16.1650890549829,1075.53797233457,529.354386493475));
#114159=CARTESIAN_POINT('Ctrl Pts',(16.0337516693691,1075.53756657121,529.378328672613));
#114160=CARTESIAN_POINT('Ctrl Pts',(15.9013205982293,1075.53973398927,529.378330417393));
#114161=CARTESIAN_POINT('Origin',(15.9013061211262,1067.7251047501,528.279499281495));
#114162=CARTESIAN_POINT('',(15.9013061211262,1075.60362949862,528.778330417488));
#114163=CARTESIAN_POINT('',(15.9013061211261,1075.70629239322,527.780668145503));
#114164=CARTESIAN_POINT('Ctrl Pts',(15.9013061211262,1075.60362949862,528.778330417488));
#114165=CARTESIAN_POINT('Ctrl Pts',(15.8995926060343,1075.60365700516,528.778330417488));
#114166=CARTESIAN_POINT('Ctrl Pts',(15.8978786789049,1075.60368544188,528.778321588453));
#114167=CARTESIAN_POINT('Ctrl Pts',(15.8311908049592,1075.60482786782,528.777634164962));
#114168=CARTESIAN_POINT('Ctrl Pts',(15.7670166584918,1075.60725579324,528.764277247047));
#114169=CARTESIAN_POINT('Ctrl Pts',(15.647217236971,1075.61445686718,528.713683958102));
#114170=CARTESIAN_POINT('Ctrl Pts',(15.5928041508971,1075.61916809108,528.676849510168));
#114171=CARTESIAN_POINT('Ctrl Pts',(15.5009685292575,1075.63026307702,528.584200793289));
#114172=CARTESIAN_POINT('Ctrl Pts',(15.4645337217032,1075.636549945,528.529160128414));
#114173=CARTESIAN_POINT('Ctrl Pts',(15.4273353345171,1075.646515274,528.438420401918));
#114174=CARTESIAN_POINT('Ctrl Pts',(15.4179313081546,1075.64990696243,528.406984517297));
#114175=CARTESIAN_POINT('Ctrl Pts',(15.4054270487921,1075.65671629965,528.342780497876));
#114176=CARTESIAN_POINT('Ctrl Pts',(15.4023465654893,1075.66011814095,528.310162979115));
#114177=CARTESIAN_POINT('Ctrl Pts',(15.4027490443541,1075.67030039173,528.210890973561));
#114178=CARTESIAN_POINT('Ctrl Pts',(15.416348788394,1075.67682638207,528.144983077483));
#114179=CARTESIAN_POINT('Ctrl Pts',(15.4685914924221,1075.68848859448,528.02259721819));
#114180=CARTESIAN_POINT('Ctrl Pts',(15.5066139908239,1075.69351612248,527.967287481599));
#114181=CARTESIAN_POINT('Ctrl Pts',(15.602125880045,1075.7014060213,527.87486300747));
#114182=CARTESIAN_POINT('Ctrl Pts',(15.6586046110204,1075.70419329947,527.838650013437));
#114183=CARTESIAN_POINT('Ctrl Pts',(15.7781887853578,1075.70704013822,527.792163073099));
#114184=CARTESIAN_POINT('Ctrl Pts',(15.8394782944546,1075.70725159426,527.780668145503));
#114185=CARTESIAN_POINT('Ctrl Pts',(15.9013061211261,1075.70629239322,527.780668145503));
#114186=CARTESIAN_POINT('',(15.9013061211262,1082.7251047501,527.780668145503));
#114187=CARTESIAN_POINT('',(15.9013061211262,1067.7251047501,527.780668145503));
#114188=CARTESIAN_POINT('Origin',(15.9013061211262,1082.7251047501,528.279499281495));
#114189=CARTESIAN_POINT('Ctrl Pts',(15.9013061211261,1075.70629239322,527.780668145503));
#114190=CARTESIAN_POINT('Ctrl Pts',(15.9013960893017,1075.70629099745,527.780668145503));
#114191=CARTESIAN_POINT('Ctrl Pts',(15.9014860586171,1075.70628959919,527.78066816984));
#114192=CARTESIAN_POINT('Ctrl Pts',(15.9015760290626,1075.70628819846,527.780668218521));
#114193=CARTESIAN_POINT('Ctrl Pts',(15.9666371127217,1075.70527527467,527.78070342183));
#114194=CARTESIAN_POINT('Ctrl Pts',(16.0310242090725,1075.70298577075,527.793466033217));
#114195=CARTESIAN_POINT('Ctrl Pts',(16.1526245906639,1075.69602260248,527.843500270199));
#114196=CARTESIAN_POINT('Ctrl Pts',(16.208388263226,1075.69136503836,527.880827323484));
#114197=CARTESIAN_POINT('Ctrl Pts',(16.3021419088947,1075.6802886557,527.975190243344));
#114198=CARTESIAN_POINT('Ctrl Pts',(16.3391258504495,1075.67397312267,528.031359182079));
#114199=CARTESIAN_POINT('Ctrl Pts',(16.3761786504636,1075.66396426213,528.12332023625));
#114200=CARTESIAN_POINT('Ctrl Pts',(16.3853682646411,1075.66059943618,528.154683383715));
#114201=CARTESIAN_POINT('Ctrl Pts',(16.3975088511561,1075.65381222211,528.218813718927));
#114202=CARTESIAN_POINT('Ctrl Pts',(16.4004178469543,1075.6504054272,528.251435472857));
#114203=CARTESIAN_POINT('Ctrl Pts',(16.3995033647169,1075.64020624374,528.350409933561));
#114204=CARTESIAN_POINT('Ctrl Pts',(16.3856771876017,1075.6336357142,528.415971570707));
#114205=CARTESIAN_POINT('Ctrl Pts',(16.3334741559357,1075.62188942714,528.537091545518));
#114206=CARTESIAN_POINT('Ctrl Pts',(16.2959262991265,1075.61680913897,528.591613097222));
#114207=CARTESIAN_POINT('Ctrl Pts',(16.2020522544986,1075.60879854306,528.682784560787));
#114208=CARTESIAN_POINT('Ctrl Pts',(16.1467618635846,1075.60593434293,528.718648108494));
#114209=CARTESIAN_POINT('Ctrl Pts',(16.0272885556594,1075.60286717747,528.766292040893));
#114210=CARTESIAN_POINT('Ctrl Pts',(15.9645782347285,1075.60261381045,528.778330417488));
#114211=CARTESIAN_POINT('Ctrl Pts',(15.9013061211262,1075.60362949862,528.778330417488));
#114212=CARTESIAN_POINT('Origin',(4.59241321360915,1067.7251047501,536.510106563848));
#114213=CARTESIAN_POINT('',(4.59241321363791,1076.96429318502,535.41956581512));
#114214=CARTESIAN_POINT('Ctrl Pts',(4.59240250088817,1076.67169975394,537.600647312524));
#114215=CARTESIAN_POINT('Ctrl Pts',(4.61963247439736,1076.67154620407,537.600647580012));
#114216=CARTESIAN_POINT('Ctrl Pts',(4.64685300256101,1076.67153279158,537.599627980395));
#114217=CARTESIAN_POINT('Ctrl Pts',(4.70549323594633,1076.67180653428,537.595228218623));
#114218=CARTESIAN_POINT('Ctrl Pts',(4.73686019260232,1076.67214185057,537.591499610811));
#114219=CARTESIAN_POINT('Ctrl Pts',(4.8212936532487,1076.67355782825,537.57772381268));
#114220=CARTESIAN_POINT('Ctrl Pts',(4.87383513915931,1076.67499652859,537.565090685447));
#114221=CARTESIAN_POINT('Ctrl Pts',(5.06278565836851,1076.68224245367,537.504540531177));
#114222=CARTESIAN_POINT('Ctrl Pts',(5.19003205201556,1076.69125446614,537.433624909088));
#114223=CARTESIAN_POINT('Ctrl Pts',(5.39141840175913,1076.71358022889,537.262032278697));
#114224=CARTESIAN_POINT('Ctrl Pts',(5.46942358282502,1076.72579078015,537.169327646511));
#114225=CARTESIAN_POINT('Ctrl Pts',(5.59728131715015,1076.75441431509,536.953500808567));
#114226=CARTESIAN_POINT('Ctrl Pts',(5.64306854302756,1076.77087507896,536.830124400968));
#114227=CARTESIAN_POINT('Ctrl Pts',(5.69066752396957,1076.80657850383,536.56345818499));
#114228=CARTESIAN_POINT('Ctrl Pts',(5.68840329148452,1076.82562331359,536.421706105464));
#114229=CARTESIAN_POINT('Ctrl Pts',(5.62939229014925,1076.8632037199,536.142902448811));
#114230=CARTESIAN_POINT('Ctrl Pts',(5.57162448245924,1076.8813589666,536.008702819453));
#114231=CARTESIAN_POINT('Ctrl Pts',(5.41074873767791,1076.91301931469,535.776200414741));
#114232=CARTESIAN_POINT('Ctrl Pts',(5.31137146010354,1076.92642833287,535.67853602913));
#114233=CARTESIAN_POINT('Ctrl Pts',(5.08104817907621,1076.94780594154,535.525407532778));
#114234=CARTESIAN_POINT('Ctrl Pts',(4.952255495658,1076.95557909134,535.471357107651));
#114235=CARTESIAN_POINT('Ctrl Pts',(4.76774845647982,1076.96164638735,535.432595106691));
#114236=CARTESIAN_POINT('Ctrl Pts',(4.71821492839048,1076.96281553606,535.425694566824));
#114237=CARTESIAN_POINT('Ctrl Pts',(4.63798156785976,1076.96397957258,535.420092438433));
#114238=CARTESIAN_POINT('Ctrl Pts',(4.60751297418011,1076.96425410189,535.419244769929));
#114239=CARTESIAN_POINT('Ctrl Pts',(4.55268802689552,1076.96444744263,535.420017331621));
#114240=CARTESIAN_POINT('Ctrl Pts',(4.52834697868929,1076.96442646147,535.421176751332));
#114241=CARTESIAN_POINT('Ctrl Pts',(4.4718632457097,1076.96412909794,535.42576775435));
#114242=CARTESIAN_POINT('Ctrl Pts',(4.43979539215814,1076.96377179973,535.429814710541));
#114243=CARTESIAN_POINT('Ctrl Pts',(4.35106232444018,1076.96225556588,535.445042637426));
#114244=CARTESIAN_POINT('Ctrl Pts',(4.29504854230218,1076.96068966126,535.45930588876));
#114245=CARTESIAN_POINT('Ctrl Pts',(4.10334867623869,1076.95315814647,535.524675273155));
#114246=CARTESIAN_POINT('Ctrl Pts',(3.97712810276218,1076.94420063445,535.598200444191));
#114247=CARTESIAN_POINT('Ctrl Pts',(3.7780751300857,1076.92205486763,535.774645184438));
#114248=CARTESIAN_POINT('Ctrl Pts',(3.70137286321866,1076.90992097153,535.869782155043));
#114249=CARTESIAN_POINT('Ctrl Pts',(3.57730582055464,1076.88138656195,536.090322205786));
#114250=CARTESIAN_POINT('Ctrl Pts',(3.53410557316563,1076.86493327179,536.215874053228));
#114251=CARTESIAN_POINT('Ctrl Pts',(3.49293824102599,1076.82905342546,536.486223339413));
#114252=CARTESIAN_POINT('Ctrl Pts',(3.49916302609928,1076.80981614048,536.629329151069));
#114253=CARTESIAN_POINT('Ctrl Pts',(3.566618010933,1076.77195854236,536.907380496889));
#114254=CARTESIAN_POINT('Ctrl Pts',(3.62813324410225,1076.75370500083,537.039578244589));
#114255=CARTESIAN_POINT('Ctrl Pts',(3.79463716522226,1076.72197923598,537.266068360592));
#114256=CARTESIAN_POINT('Ctrl Pts',(3.8955964316538,1076.70857371197,537.360101223211));
#114257=CARTESIAN_POINT('Ctrl Pts',(4.12289767311567,1076.68772612295,537.503156829554));
#114258=CARTESIAN_POINT('Ctrl Pts',(4.24616653037819,1076.68024739971,537.55259854802));
#114259=CARTESIAN_POINT('Ctrl Pts',(4.42333613990684,1076.67431155834,537.588569314053));
#114260=CARTESIAN_POINT('Ctrl Pts',(4.47185480341855,1076.67314588631,537.595065869767));
#114261=CARTESIAN_POINT('Ctrl Pts',(4.5445379155475,1076.67207790489,537.599858788991));
#114262=CARTESIAN_POINT('Ctrl Pts',(4.56846640826851,1076.67183472961,537.600647077392));
#114263=CARTESIAN_POINT('Ctrl Pts',(4.59240250088817,1076.67169975394,537.600647312524));
#114264=CARTESIAN_POINT('',(4.59241321359178,1074.94723115222,535.41956581512));
#114265=CARTESIAN_POINT('',(4.59241321360915,1067.7251047501,535.41956581512));
#114266=CARTESIAN_POINT('Ctrl Pts',(4.59241350730773,1074.65221523953,537.600647312576));
#114267=CARTESIAN_POINT('Ctrl Pts',(4.45097247351488,1074.65301913803,537.600647350669));
#114268=CARTESIAN_POINT('Ctrl Pts',(4.31099418018631,1074.6576275787,537.573133182937));
#114269=CARTESIAN_POINT('Ctrl Pts',(4.04892093847275,1074.67389907727,537.466148598073));
#114270=CARTESIAN_POINT('Ctrl Pts',(3.92953334655367,1074.68542816297,537.387524090739));
#114271=CARTESIAN_POINT('Ctrl Pts',(3.7266755056389,1074.71394090407,537.18846756568));
#114272=CARTESIAN_POINT('Ctrl Pts',(3.64553305693232,1074.73070049125,537.069547156246));
#114273=CARTESIAN_POINT('Ctrl Pts',(3.56138277177411,1074.75804181118,536.872606487432));
#114274=CARTESIAN_POINT('Ctrl Pts',(3.53977837373126,1074.76750128965,536.804013876899));
#114275=CARTESIAN_POINT('Ctrl Pts',(3.51034273845369,1074.78673962673,536.66358020759));
#114276=CARTESIAN_POINT('Ctrl Pts',(3.50259049049914,1074.79647502727,536.592055365455));
#114277=CARTESIAN_POINT('Ctrl Pts',(3.50055916703735,1074.82587855887,536.374630470324));
#114278=CARTESIAN_POINT('Ctrl Pts',(3.52839677931706,1074.84517135384,536.230039212452));
#114279=CARTESIAN_POINT('Ctrl Pts',(3.63894992867444,1074.88053853766,535.961383359238));
#114280=CARTESIAN_POINT('Ctrl Pts',(3.72011828051353,1074.89630388714,535.839714909502));
#114281=CARTESIAN_POINT('Ctrl Pts',(3.92518913613577,1074.92231188485,535.635506876668));
#114282=CARTESIAN_POINT('Ctrl Pts',(4.04682534609737,1074.93232348045,535.554822731648));
#114283=CARTESIAN_POINT('Ctrl Pts',(4.31474911424055,1074.94529735909,535.445644685266));
#114284=CARTESIAN_POINT('Ctrl Pts',(4.45820555561252,1074.94813479584,535.418225528271));
#114285=CARTESIAN_POINT('Ctrl Pts',(4.74464142728425,1074.94622035816,535.420978564132));
#114286=CARTESIAN_POINT('Ctrl Pts',(4.88465939827589,1074.94164078346,535.449962376807));
#114287=CARTESIAN_POINT('Ctrl Pts',(5.14860256833081,1074.9255281304,535.560951332028));
#114288=CARTESIAN_POINT('Ctrl Pts',(5.26934107995339,1074.91400444726,535.642996236302));
#114289=CARTESIAN_POINT('Ctrl Pts',(5.47222927006135,1074.88540823187,535.849582890718));
#114290=CARTESIAN_POINT('Ctrl Pts',(5.55210927611159,1074.86858646151,535.972308997168));
#114291=CARTESIAN_POINT('Ctrl Pts',(5.63195595118891,1074.84122470969,536.172926716412));
#114292=CARTESIAN_POINT('Ctrl Pts',(5.65171985197724,1074.83190547949,536.24140586266));
#114293=CARTESIAN_POINT('Ctrl Pts',(5.67769575715397,1074.81287411049,536.381499008862));
#114294=CARTESIAN_POINT('Ctrl Pts',(5.68378522507747,1074.80320323547,536.45281027509));
#114295=CARTESIAN_POINT('Ctrl Pts',(5.68098327565191,1074.77384035403,536.669684489158));
#114296=CARTESIAN_POINT('Ctrl Pts',(5.65000381268211,1074.75443997486,536.813447584097));
#114297=CARTESIAN_POINT('Ctrl Pts',(5.53404430120954,1074.71883253648,537.078678969888));
#114298=CARTESIAN_POINT('Ctrl Pts',(5.45088611797357,1074.70292233435,537.197930594038));
#114299=CARTESIAN_POINT('Ctrl Pts',(5.24362006982905,1074.67675924409,537.396444401062));
#114300=CARTESIAN_POINT('Ctrl Pts',(5.12195193450283,1074.66671014128,537.474148409721));
#114301=CARTESIAN_POINT('Ctrl Pts',(4.86232331778747,1074.65418471931,537.575364659058));
#114302=CARTESIAN_POINT('Ctrl Pts',(4.72799470805854,1074.65144464615,537.600647276063));
#114303=CARTESIAN_POINT('Ctrl Pts',(4.59241350730772,1074.65221523953,537.600647312576));
#114304=CARTESIAN_POINT('Origin',(4.59241321360915,1067.7251047501,536.510106563848));
#114305=CARTESIAN_POINT('',(4.59241321360915,1074.73536251872,537.000647312576));
#114306=CARTESIAN_POINT('',(4.59241321360923,1074.8680726283,536.01956581512));
#114307=CARTESIAN_POINT('Ctrl Pts',(4.59241321360915,1074.73536251872,537.000647312576));
#114308=CARTESIAN_POINT('Ctrl Pts',(4.59111296646291,1074.73536981555,537.000647312576));
#114309=CARTESIAN_POINT('Ctrl Pts',(4.58981246310562,1074.73537782066,537.000642142847));
#114310=CARTESIAN_POINT('Ctrl Pts',(4.52485381758119,1074.73581300135,537.000125482655));
#114311=CARTESIAN_POINT('Ctrl Pts',(4.46195359926289,1074.73792920154,536.987233759357));
#114312=CARTESIAN_POINT('Ctrl Pts',(4.34436934018267,1074.74529884748,536.938107046314));
#114313=CARTESIAN_POINT('Ctrl Pts',(4.29090598636675,1074.75049324738,536.902251505426));
#114314=CARTESIAN_POINT('Ctrl Pts',(4.20033795354942,1074.76331991499,536.811838149889));
#114315=CARTESIAN_POINT('Ctrl Pts',(4.16427511206219,1074.77085110083,536.757974648325));
#114316=CARTESIAN_POINT('Ctrl Pts',(4.12720605980857,1074.78313632965,536.669018569248));
#114317=CARTESIAN_POINT('Ctrl Pts',(4.11777072189871,1074.78738233221,536.638104710596));
#114318=CARTESIAN_POINT('Ctrl Pts',(4.10510359199887,1074.79601709625,536.57490114595));
#114319=CARTESIAN_POINT('Ctrl Pts',(4.10190044694374,1074.80038628712,536.542754657397));
#114320=CARTESIAN_POINT('Ctrl Pts',(4.10181599721064,1074.81362343086,536.444861376876));
#114321=CARTESIAN_POINT('Ctrl Pts',(4.11494634489056,1074.82232886225,536.379791782595));
#114322=CARTESIAN_POINT('Ctrl Pts',(4.16597308217532,1074.83830918791,536.259011817999));
#114323=CARTESIAN_POINT('Ctrl Pts',(4.20321540052522,1074.84543949873,536.204406608515));
#114324=CARTESIAN_POINT('Ctrl Pts',(4.29688139158837,1074.85716195678,536.113192568182));
#114325=CARTESIAN_POINT('Ctrl Pts',(4.35225336206347,1074.86164989832,536.077408196333));
#114326=CARTESIAN_POINT('Ctrl Pts',(4.47020097331052,1074.86720243615,536.031090224403));
#114327=CARTESIAN_POINT('Ctrl Pts',(4.53102029027343,1074.86840975228,536.01956581512));
#114328=CARTESIAN_POINT('Ctrl Pts',(4.59241321360938,1074.8680726283,536.01956581512));
#114329=CARTESIAN_POINT('',(4.59241321360915,1082.7251047501,536.01956581512));
#114330=CARTESIAN_POINT('',(4.59241321360915,1067.7251047501,536.01956581512));
#114331=CARTESIAN_POINT('Origin',(4.59241321360915,1082.7251047501,536.510106563848));
#114332=CARTESIAN_POINT('Ctrl Pts',(4.59241494804499,1074.86807261878,536.019565815123));
#114333=CARTESIAN_POINT('Ctrl Pts',(4.65613540139557,1074.8677226836,536.019566040424));
#114334=CARTESIAN_POINT('Ctrl Pts',(4.71919903687055,1074.86571598349,536.031981090877));
#114335=CARTESIAN_POINT('Ctrl Pts',(4.83730193509805,1074.85859856745,536.080278813853));
#114336=CARTESIAN_POINT('Ctrl Pts',(4.89110933749994,1074.85354264986,536.115799904315));
#114337=CARTESIAN_POINT('Ctrl Pts',(4.98330162341501,1074.84084878979,536.206561222789));
#114338=CARTESIAN_POINT('Ctrl Pts',(5.02027070079791,1074.83326895952,536.261418717346));
#114339=CARTESIAN_POINT('Ctrl Pts',(5.05769302124054,1074.82093012762,536.351441427919));
#114340=CARTESIAN_POINT('Ctrl Pts',(5.06706788991385,1074.81672948397,536.382196172587));
#114341=CARTESIAN_POINT('Ctrl Pts',(5.0796970982866,1074.80815704409,536.445156596179));
#114342=CARTESIAN_POINT('Ctrl Pts',(5.08290513911219,1074.80380415207,536.477223963017));
#114343=CARTESIAN_POINT('Ctrl Pts',(5.083052418277,1074.7905296475,536.57530599089));
#114344=CARTESIAN_POINT('Ctrl Pts',(5.06985629252667,1074.78174088848,536.640640133447));
#114345=CARTESIAN_POINT('Ctrl Pts',(5.0187255712267,1074.76562260392,536.761342540552));
#114346=CARTESIAN_POINT('Ctrl Pts',(4.98164835173554,1074.75842705477,536.815696300057));
#114347=CARTESIAN_POINT('Ctrl Pts',(4.88898788677217,1074.74662133191,536.906077212551));
#114348=CARTESIAN_POINT('Ctrl Pts',(4.83462408568439,1074.74208631009,536.941508679684));
#114349=CARTESIAN_POINT('Ctrl Pts',(4.71686744409228,1074.73629900908,536.988694094649));
#114350=CARTESIAN_POINT('Ctrl Pts',(4.65493653762755,1074.73501164518,537.000647312576));
#114351=CARTESIAN_POINT('Ctrl Pts',(4.59241321360915,1074.73536251872,537.000647312576));
#114352=CARTESIAN_POINT('Origin',(49.3616411037544,1067.7251047501,499.347110012371));
#114353=CARTESIAN_POINT('',(49.3616411037703,1078.70098643656,497.868806880177));
#114354=CARTESIAN_POINT('Ctrl Pts',(50.8397772837836,1078.64997002067,499.369326761487));
#114355=CARTESIAN_POINT('Ctrl Pts',(50.8424068823753,1078.65432609598,499.194372955374));
#114356=CARTESIAN_POINT('Ctrl Pts',(50.8139541383063,1078.65901118556,499.020338179437));
#114357=CARTESIAN_POINT('Ctrl Pts',(50.6933755445324,1078.66874765754,498.678513848796));
#114358=CARTESIAN_POINT('Ctrl Pts',(50.5979231326937,1078.67370907481,498.515155430946));
#114359=CARTESIAN_POINT('Ctrl Pts',(50.3459846066139,1078.68309182049,498.227039440132));
#114360=CARTESIAN_POINT('Ctrl Pts',(50.1896261463433,1078.68739095086,498.106972871076));
#114361=CARTESIAN_POINT('Ctrl Pts',(49.8454398767191,1078.69459396784,497.937569631812));
#114362=CARTESIAN_POINT('Ctrl Pts',(49.6620657588907,1078.69748205776,497.887446512515));
#114363=CARTESIAN_POINT('Ctrl Pts',(49.2896157478694,1078.70192809518,497.859000632821));
#114364=CARTESIAN_POINT('Ctrl Pts',(49.1039909490667,1078.70347537265,497.879705027883));
#114365=CARTESIAN_POINT('Ctrl Pts',(48.8507729174781,1078.70481731323,497.957592848052));
#114366=CARTESIAN_POINT('Ctrl Pts',(48.7765461814908,1078.70510525467,497.98718048505));
#114367=CARTESIAN_POINT('Ctrl Pts',(48.6718521247516,1078.70536039302,498.039078707383));
#114368=CARTESIAN_POINT('Ctrl Pts',(48.6392653583714,1078.70541663073,498.05678911477));
#114369=CARTESIAN_POINT('Ctrl Pts',(48.583042040328,1078.70547240393,498.090143670295));
#114370=CARTESIAN_POINT('Ctrl Pts',(48.5591247209862,1078.70548219651,498.105277357441));
#114371=CARTESIAN_POINT('Ctrl Pts',(48.5108578570887,1078.70547284712,498.137795280551));
#114372=CARTESIAN_POINT('Ctrl Pts',(48.4865717984161,1078.70545203616,498.155250975752));
#114373=CARTESIAN_POINT('Ctrl Pts',(48.4267098417356,1078.70535912999,498.201093564839));
#114374=CARTESIAN_POINT('Ctrl Pts',(48.3918841440097,1078.70526601773,498.230408804135));
#114375=CARTESIAN_POINT('Ctrl Pts',(48.2664622690791,1078.70477650681,498.346283727692));
#114376=CARTESIAN_POINT('Ctrl Pts',(48.1856347557062,1078.70413810346,498.442633210835));
#114377=CARTESIAN_POINT('Ctrl Pts',(48.0373344179074,1078.70210163806,498.67344752563));
#114378=CARTESIAN_POINT('Ctrl Pts',(47.9761814572351,1078.70059316131,498.810352642049));
#114379=CARTESIAN_POINT('Ctrl Pts',(47.8924765415345,1078.6965091591,499.113855164203));
#114380=CARTESIAN_POINT('Ctrl Pts',(47.875595619189,1078.69385899944,499.279908399778));
#114381=CARTESIAN_POINT('Ctrl Pts',(47.898502127747,1078.68730940719,499.624106142555));
#114382=CARTESIAN_POINT('Ctrl Pts',(47.9428257315769,1078.68337551964,499.799280688149));
#114383=CARTESIAN_POINT('Ctrl Pts',(48.0975032165717,1078.67434615777,500.137299861922));
#114384=CARTESIAN_POINT('Ctrl Pts',(48.2110409173425,1078.66926963615,500.295033527205));
#114385=CARTESIAN_POINT('Ctrl Pts',(48.4933837520922,1078.65888588427,500.559218340279));
#114386=CARTESIAN_POINT('Ctrl Pts',(48.6599163753638,1078.65368157732,500.662657050314));
#114387=CARTESIAN_POINT('Ctrl Pts',(49.0124902482889,1078.64443898008,500.795132753));
#114388=CARTESIAN_POINT('Ctrl Pts',(49.1937308847251,1078.64043452576,500.827141052003));
#114389=CARTESIAN_POINT('Ctrl Pts',(49.5581299687267,1078.63406328938,500.823547169656));
#114390=CARTESIAN_POINT('Ctrl Pts',(49.7381667272288,1078.6317503759,500.788189944642));
#114391=CARTESIAN_POINT('Ctrl Pts',(49.9590648889496,1078.63013700081,500.700465722135));
#114392=CARTESIAN_POINT('Ctrl Pts',(50.0096629034765,1078.62986059048,500.676980200575));
#114393=CARTESIAN_POINT('Ctrl Pts',(50.0877975385495,1078.6295871773,500.635192812644));
#114394=CARTESIAN_POINT('Ctrl Pts',(50.1162560963385,1078.62952212581,500.618729723957));
#114395=CARTESIAN_POINT('Ctrl Pts',(50.167830319471,1078.62946945633,500.586552886558));
#114396=CARTESIAN_POINT('Ctrl Pts',(50.1910949554386,1078.6294716644,500.571105926506));
#114397=CARTESIAN_POINT('Ctrl Pts',(50.2414641234579,1078.62953481524,500.535566558212));
#114398=CARTESIAN_POINT('Ctrl Pts',(50.2683466198659,1078.62960785773,500.515186466865));
#114399=CARTESIAN_POINT('Ctrl Pts',(50.3417913497394,1078.62992029996,500.455442400916));
#114400=CARTESIAN_POINT('Ctrl Pts',(50.3866497236217,1078.63024616515,500.414092842344));
#114401=CARTESIAN_POINT('Ctrl Pts',(50.5651229817255,1078.63213805046,500.227907847569));
#114402=CARTESIAN_POINT('Ctrl Pts',(50.6716282390872,1078.63483689903,500.05991866479));
#114403=CARTESIAN_POINT('Ctrl Pts',(50.80410847851,1078.64173387056,499.714149024615));
#114404=CARTESIAN_POINT('Ctrl Pts',(50.8371724553628,1078.64565497852,499.542632545847));
#114405=CARTESIAN_POINT('Ctrl Pts',(50.8397772837836,1078.64997002067,499.369326761487));
#114406=CARTESIAN_POINT('',(49.3616411037368,1076.7006095282,497.868806880177));
#114407=CARTESIAN_POINT('',(49.3616411037544,1067.7251047501,497.868806880177));
#114408=CARTESIAN_POINT('Ctrl Pts',(49.3624292594544,1076.63635835644,500.825412934462));
#114409=CARTESIAN_POINT('Ctrl Pts',(49.169353872364,1076.63981814556,500.825515872408));
#114410=CARTESIAN_POINT('Ctrl Pts',(48.9781312245865,1076.64418702791,500.787792900627));
#114411=CARTESIAN_POINT('Ctrl Pts',(48.6208591844163,1076.65392418461,500.64092682057));
#114412=CARTESIAN_POINT('Ctrl Pts',(48.4582674877644,1076.65919298524,500.533125372586));
#114413=CARTESIAN_POINT('Ctrl Pts',(48.1836868704222,1076.66968175505,500.260998222324));
#114414=CARTESIAN_POINT('Ctrl Pts',(48.0743734531646,1076.67479716143,500.099250538524));
#114415=CARTESIAN_POINT('Ctrl Pts',(47.923449534576,1076.68421023618,499.741004657796));
#114416=CARTESIAN_POINT('Ctrl Pts',(47.8840332144445,1076.68840827999,499.547690141379));
#114417=CARTESIAN_POINT('Ctrl Pts',(47.8826628493512,1076.69547892568,499.157450850087));
#114418=CARTESIAN_POINT('Ctrl Pts',(47.920509380774,1076.69829323977,498.964364345255));
#114419=CARTESIAN_POINT('Ctrl Pts',(48.069289066609,1076.70253581002,498.60309569489));
#114420=CARTESIAN_POINT('Ctrl Pts',(48.1791084959194,1076.70392346639,498.438621398773));
#114421=CARTESIAN_POINT('Ctrl Pts',(48.4569428659271,1076.70533126823,498.161562221212));
#114422=CARTESIAN_POINT('Ctrl Pts',(48.622387596233,1076.70533637046,498.051924027819));
#114423=CARTESIAN_POINT('Ctrl Pts',(48.9858236698055,1076.70394944997,497.904023210739));
#114424=CARTESIAN_POINT('Ctrl Pts',(49.1801007082442,1076.70257225397,497.866982469837));
#114425=CARTESIAN_POINT('Ctrl Pts',(49.5707994477516,1076.69835099485,497.870760125806));
#114426=CARTESIAN_POINT('Ctrl Pts',(49.7633720973987,1076.69554737456,497.911157079714));
#114427=CARTESIAN_POINT('Ctrl Pts',(50.1222140806546,1076.68849710468,498.06450259862));
#114428=CARTESIAN_POINT('Ctrl Pts',(50.2848734023975,1076.68430861636,498.176133635553));
#114429=CARTESIAN_POINT('Ctrl Pts',(50.5589386098338,1076.67480716416,498.457775948561));
#114430=CARTESIAN_POINT('Ctrl Pts',(50.666967154968,1076.66957478604,498.625615433594));
#114431=CARTESIAN_POINT('Ctrl Pts',(50.8093329902586,1076.65894549525,498.990446072193));
#114432=CARTESIAN_POINT('Ctrl Pts',(50.8435982120277,1076.65366044596,499.183318187261));
#114433=CARTESIAN_POINT('Ctrl Pts',(50.8356722690318,1076.64391066459,499.571349616223));
#114434=CARTESIAN_POINT('Ctrl Pts',(50.7935307746048,1076.63954780243,499.762747796716));
#114435=CARTESIAN_POINT('Ctrl Pts',(50.6377522610623,1076.63268400824,500.118170230531));
#114436=CARTESIAN_POINT('Ctrl Pts',(50.5256942373236,1076.63025439825,500.278766550657));
#114437=CARTESIAN_POINT('Ctrl Pts',(50.2462547107407,1076.62789959202,500.54723333446));
#114438=CARTESIAN_POINT('Ctrl Pts',(50.0817088218061,1076.62799406049,500.65261346529));
#114439=CARTESIAN_POINT('Ctrl Pts',(49.7297753855395,1076.63064111655,500.790682492722));
#114440=CARTESIAN_POINT('Ctrl Pts',(49.5469155692401,1076.63305247816,500.825314575773));
#114441=CARTESIAN_POINT('Ctrl Pts',(49.3624292594544,1076.63635835644,500.825412934462));
#114442=CARTESIAN_POINT('Origin',(49.3616411037544,1067.7251047501,499.347110012371));
#114443=CARTESIAN_POINT('',(49.3616411037544,1076.65225835227,500.225413144564));
#114444=CARTESIAN_POINT('',(49.3616411037542,1076.69042463418,498.468806880177));
#114445=CARTESIAN_POINT('Ctrl Pts',(49.3616411037544,1076.65225835227,500.225413144564));
#114446=CARTESIAN_POINT('Ctrl Pts',(49.2526397446302,1076.65405656161,500.225413144564));
#114447=CARTESIAN_POINT('Ctrl Pts',(49.1445390094345,1076.656318982,500.205121031533));
#114448=CARTESIAN_POINT('Ctrl Pts',(48.9358138895393,1076.661577456,500.123828754696));
#114449=CARTESIAN_POINT('Ctrl Pts',(48.837959421548,1076.66455181297,500.06151639355));
#114450=CARTESIAN_POINT('Ctrl Pts',(48.7133726407549,1076.66910586258,499.942475946899));
#114451=CARTESIAN_POINT('Ctrl Pts',(48.6758510030616,1076.67062826025,499.898838728586));
#114452=CARTESIAN_POINT('Ctrl Pts',(48.6099016312046,1076.67363340817,499.804922924166));
#114453=CARTESIAN_POINT('Ctrl Pts',(48.5816210798479,1076.67510900197,499.754876943453));
#114454=CARTESIAN_POINT('Ctrl Pts',(48.5112459995488,1076.6794443307,499.59579115308));
#114455=CARTESIAN_POINT('Ctrl Pts',(48.4857749565104,1076.68211321505,499.480809663299));
#114456=CARTESIAN_POINT('Ctrl Pts',(48.4812371815133,1076.68674331669,499.247776609224));
#114457=CARTESIAN_POINT('Ctrl Pts',(48.5021492347113,1076.68866226052,499.132040380882));
#114458=CARTESIAN_POINT('Ctrl Pts',(48.5880483514483,1076.69161962061,498.91510906484));
#114459=CARTESIAN_POINT('Ctrl Pts',(48.6523218104215,1076.69262848295,498.816131172533));
#114460=CARTESIAN_POINT('Ctrl Pts',(48.8160266865626,1076.69368053487,498.648939949345));
#114461=CARTESIAN_POINT('Ctrl Pts',(48.9138959172231,1076.69371222786,498.582478836269));
#114462=CARTESIAN_POINT('Ctrl Pts',(49.1294936780044,1076.69278723447,498.49204620934));
#114463=CARTESIAN_POINT('Ctrl Pts',(49.2449904043857,1076.69184255343,498.468806880177));
#114464=CARTESIAN_POINT('Ctrl Pts',(49.361641103754,1076.69042463418,498.468806880177));
#114465=CARTESIAN_POINT('',(49.3616411037544,1082.7251047501,498.468806880177));
#114466=CARTESIAN_POINT('',(49.3616411037544,1067.7251047501,498.468806880177));
#114467=CARTESIAN_POINT('Origin',(49.3616411037544,1082.7251047501,499.347110012371));
#114468=CARTESIAN_POINT('Ctrl Pts',(49.361641103754,1076.69042463418,498.468806880177));
#114469=CARTESIAN_POINT('Ctrl Pts',(49.3618661819275,1076.6904218983,498.468806880177));
#114470=CARTESIAN_POINT('Ctrl Pts',(49.362091264397,1076.69041916064,498.468806966697));
#114471=CARTESIAN_POINT('Ctrl Pts',(49.478798580427,1076.68899876853,498.468896692359));
#114472=CARTESIAN_POINT('Ctrl Pts',(49.5941007023354,1076.68713463047,498.492157345844));
#114473=CARTESIAN_POINT('Ctrl Pts',(49.8090051354294,1076.68260080841,498.582338809127));
#114474=CARTESIAN_POINT('Ctrl Pts',(49.9064550787002,1076.67997265236,498.648408157275));
#114475=CARTESIAN_POINT('Ctrl Pts',(50.0704006515689,1076.67419715182,498.815275564623));
#114476=CARTESIAN_POINT('Ctrl Pts',(50.1350381480216,1076.67110351319,498.914624450601));
#114477=CARTESIAN_POINT('Ctrl Pts',(50.2172975299658,1076.66519369211,499.122345575253));
#114478=CARTESIAN_POINT('Ctrl Pts',(50.238166604033,1076.66242934611,499.227229665931));
#114479=CARTESIAN_POINT('Ctrl Pts',(50.2398355216052,1076.65987444592,499.333291312131));
#114480=CARTESIAN_POINT('Ctrl Pts',(50.2416478298962,1076.65710003281,499.448465604721));
#114481=CARTESIAN_POINT('Ctrl Pts',(50.2207851993397,1076.65462615942,499.562887367419));
#114482=CARTESIAN_POINT('Ctrl Pts',(50.1360989378208,1076.65068256021,499.777096010322));
#114483=CARTESIAN_POINT('Ctrl Pts',(50.0731216638255,1076.64925290657,499.874813993407));
#114484=CARTESIAN_POINT('Ctrl Pts',(49.9131483865159,1076.64772752428,500.040277564078));
#114485=CARTESIAN_POINT('Ctrl Pts',(49.817748553446,1076.64764590949,500.106456927186));
#114486=CARTESIAN_POINT('Ctrl Pts',(49.606992395841,1076.64885773552,500.198235456417));
#114487=CARTESIAN_POINT('Ctrl Pts',(49.4936990042523,1076.65013703494,500.22299217993));
#114488=CARTESIAN_POINT('Ctrl Pts',(49.3731201546009,1076.65207030756,500.225356909283));
#114489=CARTESIAN_POINT('Ctrl Pts',(49.3673793811915,1076.65216368718,500.225413144564));
#114490=CARTESIAN_POINT('Ctrl Pts',(49.3616411037544,1076.65225835227,500.225413144564));
#114491=CARTESIAN_POINT('Origin',(44.0648939479111,1067.7251047501,510.733705034314));
#114492=CARTESIAN_POINT('',(44.0648939479365,1078.41872688014,509.458260913177));
#114493=CARTESIAN_POINT('Ctrl Pts',(44.0649233283352,1078.2734319431,512.009149155111));
#114494=CARTESIAN_POINT('Ctrl Pts',(44.1880264249484,1078.26956806541,512.009146319377));
#114495=CARTESIAN_POINT('Ctrl Pts',(44.3105075695597,1078.26679874672,511.991321125002));
#114496=CARTESIAN_POINT('Ctrl Pts',(44.4706129032522,1078.26467957244,511.943695046355));
#114497=CARTESIAN_POINT('Ctrl Pts',(44.5120048987952,1078.2642773326,511.9290191121));
#114498=CARTESIAN_POINT('Ctrl Pts',(44.5778908661641,1078.26387834022,511.901756163488));
#114499=CARTESIAN_POINT('Ctrl Pts',(44.6028782862815,1078.26378615623,511.890460043791));
#114500=CARTESIAN_POINT('Ctrl Pts',(44.649880058208,1078.26372736872,511.867359211077));
#114501=CARTESIAN_POINT('Ctrl Pts',(44.6719497463567,1078.26375025698,511.855696029825));
#114502=CARTESIAN_POINT('Ctrl Pts',(44.7213945258687,1078.26391820128,511.82767973288));
#114503=CARTESIAN_POINT('Ctrl Pts',(44.7485269043753,1078.26409530375,511.810932759244));
#114504=CARTESIAN_POINT('Ctrl Pts',(44.8279271463046,1078.26487358262,511.757715417644));
#114505=CARTESIAN_POINT('Ctrl Pts',(44.8781154099761,1078.26572063921,511.718330187519));
#114506=CARTESIAN_POINT('Ctrl Pts',(45.0507311696377,1078.26999998016,511.560636833786));
#114507=CARTESIAN_POINT('Ctrl Pts',(45.1520574044804,1078.27534724355,511.421983108299));
#114508=CARTESIAN_POINT('Ctrl Pts',(45.2819500075955,1078.28844959601,511.140179486435));
#114509=CARTESIAN_POINT('Ctrl Pts',(45.3192377794129,1078.29552900789,511.003968227667));
#114510=CARTESIAN_POINT('Ctrl Pts',(45.3491961468539,1078.31195951831,510.713331211856));
#114511=CARTESIAN_POINT('Ctrl Pts',(45.3376373286404,1078.32131821746,510.560639240082));
#114512=CARTESIAN_POINT('Ctrl Pts',(45.2586193967198,1078.34136818601,510.255859826798));
#114513=CARTESIAN_POINT('Ctrl Pts',(45.1878593661594,1078.351922742,510.107390558694));
#114514=CARTESIAN_POINT('Ctrl Pts',(44.9910598959799,1078.372559519,509.840769415868));
#114515=CARTESIAN_POINT('Ctrl Pts',(44.8651708735293,1078.38241474774,509.726378471745));
#114516=CARTESIAN_POINT('Ctrl Pts',(44.5822331974789,1078.399487038,509.556776761719));
#114517=CARTESIAN_POINT('Ctrl Pts',(44.4292741045652,1078.4066482895,509.500796653613));
#114518=CARTESIAN_POINT('Ctrl Pts',(44.1077587594526,1078.41811353863,509.448441447054));
#114519=CARTESIAN_POINT('Ctrl Pts',(43.9420068574355,1078.42226273415,509.453601435726));
#114520=CARTESIAN_POINT('Ctrl Pts',(43.7241966059722,1078.42547987196,509.50318937737));
#114521=CARTESIAN_POINT('Ctrl Pts',(43.6676063820261,1078.42609572361,509.520277400153));
#114522=CARTESIAN_POINT('Ctrl Pts',(43.5837247291025,1078.42667113737,509.552106674066));
#114523=CARTESIAN_POINT('Ctrl Pts',(43.5554490856828,1078.42680364945,509.564019406702));
#114524=CARTESIAN_POINT('Ctrl Pts',(43.5053387657168,1078.42692640291,509.587293325476));
#114525=CARTESIAN_POINT('Ctrl Pts',(43.4833511983387,1078.42693965304,509.598288881504));
#114526=CARTESIAN_POINT('Ctrl Pts',(43.4373926283563,1078.42687998455,509.622957282948));
#114527=CARTESIAN_POINT('Ctrl Pts',(43.4135198271369,1078.42679635528,509.636786527848));
#114528=CARTESIAN_POINT('Ctrl Pts',(43.351564860165,1078.4264373479,509.675412539031));
#114529=CARTESIAN_POINT('Ctrl Pts',(43.3143278474008,1078.42607319779,509.7014881403));
#114530=CARTESIAN_POINT('Ctrl Pts',(43.1618407086329,1078.42392450151,509.820890749726));
#114531=CARTESIAN_POINT('Ctrl Pts',(43.0619659177488,1078.42081023532,509.93192354757));
#114532=CARTESIAN_POINT('Ctrl Pts',(42.9117438614676,1078.41221661889,510.172208468626));
#114533=CARTESIAN_POINT('Ctrl Pts',(42.8587785837881,1078.40702155248,510.297472526595));
#114534=CARTESIAN_POINT('Ctrl Pts',(42.7910462855203,1078.39412783417,510.572457283003));
#114535=CARTESIAN_POINT('Ctrl Pts',(42.7809518465782,1078.38633227265,510.721279006368));
#114536=CARTESIAN_POINT('Ctrl Pts',(42.81343049477,1078.36854609626,511.026987087462));
#114537=CARTESIAN_POINT('Ctrl Pts',(42.8598463718235,1078.35858523557,511.180937499236));
#114538=CARTESIAN_POINT('Ctrl Pts',(43.011419943816,1078.33754469861,511.472307774161));
#114539=CARTESIAN_POINT('Ctrl Pts',(43.1185007686512,1078.32663889876,511.605308130303));
#114540=CARTESIAN_POINT('Ctrl Pts',(43.3445464540617,1078.30871969167,511.793665775114));
#114541=CARTESIAN_POINT('Ctrl Pts',(43.4519755230289,1078.30152981722,511.859211086788));
#114542=CARTESIAN_POINT('Ctrl Pts',(43.6364119537953,1078.29115151849,511.937367251213));
#114543=CARTESIAN_POINT('Ctrl Pts',(43.708037897756,1078.28753344912,511.960512913644));
#114544=CARTESIAN_POINT('Ctrl Pts',(43.8743255501986,1078.28006013478,511.998436522319));
#114545=CARTESIAN_POINT('Ctrl Pts',(43.9694626892088,1078.27642819782,512.00915135409));
#114546=CARTESIAN_POINT('Ctrl Pts',(44.0649233283352,1078.2734319431,512.009149155111));
#114547=CARTESIAN_POINT('',(44.0648939478931,1076.41517983612,509.458260913177));
#114548=CARTESIAN_POINT('',(44.0648939479111,1067.7251047501,509.458260913177));
#114549=CARTESIAN_POINT('Ctrl Pts',(44.0649289142737,1076.26836941018,512.009149154971));
#114550=CARTESIAN_POINT('Ctrl Pts',(43.898466721868,1076.27364765281,512.00915371854));
#114551=CARTESIAN_POINT('Ctrl Pts',(43.7336757635041,1076.28085793182,511.976571532619));
#114552=CARTESIAN_POINT('Ctrl Pts',(43.4255980312565,1076.29814802138,511.849892034166));
#114553=CARTESIAN_POINT('Ctrl Pts',(43.2853292344771,1076.30806503659,511.756845973201));
#114554=CARTESIAN_POINT('Ctrl Pts',(43.1076795744347,1076.32385879801,511.580738504689));
#114555=CARTESIAN_POINT('Ctrl Pts',(43.0543151174143,1076.3292440124,511.516299408341));
#114556=CARTESIAN_POINT('Ctrl Pts',(42.9609252978987,1076.34007978619,511.377897182119));
#114557=CARTESIAN_POINT('Ctrl Pts',(42.92112790914,1076.34550463083,511.304257657007));
#114558=CARTESIAN_POINT('Ctrl Pts',(42.8231671228517,1076.36172686774,511.070827742348));
#114559=CARTESIAN_POINT('Ctrl Pts',(42.7893682881464,1076.37212929197,510.902822386907));
#114560=CARTESIAN_POINT('Ctrl Pts',(42.789531130527,1076.39082207213,510.564461885871));
#114561=CARTESIAN_POINT('Ctrl Pts',(42.8230537282854,1076.39894628175,510.397448781163));
#114562=CARTESIAN_POINT('Ctrl Pts',(42.9532536253702,1076.41208001526,510.086009985341));
#114563=CARTESIAN_POINT('Ctrl Pts',(43.0486587750672,1076.41696331781,509.944685561946));
#114564=CARTESIAN_POINT('Ctrl Pts',(43.2893362834614,1076.42298691131,509.707095303306));
#114565=CARTESIAN_POINT('Ctrl Pts',(43.4323053363089,1076.42406124075,509.613322596213));
#114566=CARTESIAN_POINT('Ctrl Pts',(43.7463888061328,1076.42225126093,509.487137638111));
#114567=CARTESIAN_POINT('Ctrl Pts',(43.9143232162407,1076.4193875216,509.455939848884));
#114568=CARTESIAN_POINT('Ctrl Pts',(44.2521255034383,1076.40996404624,509.460845403669));
#114569=CARTESIAN_POINT('Ctrl Pts',(44.4186228177448,1076.40350198033,509.496747470433));
#114570=CARTESIAN_POINT('Ctrl Pts',(44.7283047831834,1076.38758170073,509.631334097181));
#114571=CARTESIAN_POINT('Ctrl Pts',(44.8683568598277,1076.37826864388,509.728844772274));
#114572=CARTESIAN_POINT('Ctrl Pts',(45.0427133406882,1076.36305942859,509.910598795777));
#114573=CARTESIAN_POINT('Ctrl Pts',(45.0941421083455,1076.35787432204,509.975892416633));
#114574=CARTESIAN_POINT('Ctrl Pts',(45.1843665778088,1076.34719554529,510.116733352278));
#114575=CARTESIAN_POINT('Ctrl Pts',(45.2227080714411,1076.34172394529,510.1920977003));
#114576=CARTESIAN_POINT('Ctrl Pts',(45.314177609022,1076.32536347,510.426875244866));
#114577=CARTESIAN_POINT('Ctrl Pts',(45.3436560276373,1076.31461218309,510.593560774999));
#114578=CARTESIAN_POINT('Ctrl Pts',(45.3364295434161,1076.29473867435,510.928736467631));
#114579=CARTESIAN_POINT('Ctrl Pts',(45.2998322220975,1076.28581091494,511.093997874046));
#114580=CARTESIAN_POINT('Ctrl Pts',(45.1648858177163,1076.27122059476,511.400608487779));
#114581=CARTESIAN_POINT('Ctrl Pts',(45.0680041547839,1076.26569628253,511.539032561309));
#114582=CARTESIAN_POINT('Ctrl Pts',(44.8266311050491,1076.25898953484,511.770209463768));
#114583=CARTESIAN_POINT('Ctrl Pts',(44.6846746230433,1076.25785997188,511.860854687224));
#114584=CARTESIAN_POINT('Ctrl Pts',(44.3812706408253,1076.2601490384,511.979465613399));
#114585=CARTESIAN_POINT('Ctrl Pts',(44.223776818423,1076.26333260411,512.009144800148));
#114586=CARTESIAN_POINT('Ctrl Pts',(44.0649289142737,1076.26836941018,512.009149154971));
#114587=CARTESIAN_POINT('Origin',(44.0648939479111,1067.7251047501,510.733705034314));
#114588=CARTESIAN_POINT('',(44.0648939479111,1076.3053526307,511.40914915545));
#114589=CARTESIAN_POINT('',(44.0648939479122,1076.38310559156,510.058260913177));
#114590=CARTESIAN_POINT('Ctrl Pts',(44.0648939479111,1076.3053526307,511.40914915545));
#114591=CARTESIAN_POINT('Ctrl Pts',(44.0633527628547,1076.30539988211,511.40914915545));
#114592=CARTESIAN_POINT('Ctrl Pts',(44.0618113343601,1076.30544745384,511.409143880586));
#114593=CARTESIAN_POINT('Ctrl Pts',(43.9720188605801,1076.30823686737,511.408529124494));
#114594=CARTESIAN_POINT('Ctrl Pts',(43.884773315559,1076.31197309278,511.390635615152));
#114595=CARTESIAN_POINT('Ctrl Pts',(43.721946257568,1076.32096316671,511.322285843355));
#114596=CARTESIAN_POINT('Ctrl Pts',(43.6479630276562,1076.32613292064,511.272406572667));
#114597=CARTESIAN_POINT('Ctrl Pts',(43.5545347528908,1076.33441434733,511.17835484543));
#114598=CARTESIAN_POINT('Ctrl Pts',(43.5265300258902,1076.33724450606,511.144002164113));
#114599=CARTESIAN_POINT('Ctrl Pts',(43.4776284811296,1076.34295724576,511.070306507139));
#114600=CARTESIAN_POINT('Ctrl Pts',(43.4568510945842,1076.34582627713,511.031136155473));
#114601=CARTESIAN_POINT('Ctrl Pts',(43.4058321641746,1076.3544500931,510.906858046465));
#114602=CARTESIAN_POINT('Ctrl Pts',(43.3886279945003,1076.3600251194,510.817468897038));
#114603=CARTESIAN_POINT('Ctrl Pts',(43.3903285823292,1076.37010972279,510.637534695334));
#114604=CARTESIAN_POINT('Ctrl Pts',(43.4090728930029,1076.37452473097,510.548778109158));
#114605=CARTESIAN_POINT('Ctrl Pts',(43.480211565499,1076.38165860269,510.383795285743));
#114606=CARTESIAN_POINT('Ctrl Pts',(43.5318752711781,1076.38430833495,510.309215794991));
#114607=CARTESIAN_POINT('Ctrl Pts',(43.6614488871979,1076.38751506255,510.184574883999));
#114608=CARTESIAN_POINT('Ctrl Pts',(43.7380667818616,1076.38803887879,510.135793679277));
#114609=CARTESIAN_POINT('Ctrl Pts',(43.8995060293051,1076.38692014794,510.073574062566));
#114610=CARTESIAN_POINT('Ctrl Pts',(43.9818499782334,1076.38544930888,510.058260913177));
#114611=CARTESIAN_POINT('Ctrl Pts',(44.0648939479144,1076.38310559156,510.058260913177));
#114612=CARTESIAN_POINT('',(44.0648939479111,1082.7251047501,510.058260913177));
#114613=CARTESIAN_POINT('',(44.0648939479111,1067.7251047501,510.058260913177));
#114614=CARTESIAN_POINT('Origin',(44.0648939479111,1082.7251047501,510.733705034314));
#114615=CARTESIAN_POINT('Ctrl Pts',(44.0649019425061,1076.38310536593,510.058260913225));
#114616=CARTESIAN_POINT('Ctrl Pts',(44.1547346152825,1076.38056999439,510.058261976489));
#114617=CARTESIAN_POINT('Ctrl Pts',(44.2436360023306,1076.37706156818,510.076183629503));
#114618=CARTESIAN_POINT('Ctrl Pts',(44.4093391643003,1076.36844335467,510.145765016121));
#114619=CARTESIAN_POINT('Ctrl Pts',(44.4844585717707,1076.36341511981,510.19679661222));
#114620=CARTESIAN_POINT('Ctrl Pts',(44.5781912597982,1076.35526119709,510.292467494895));
#114621=CARTESIAN_POINT('Ctrl Pts',(44.6058611629681,1076.35249267579,510.326865469975));
#114622=CARTESIAN_POINT('Ctrl Pts',(44.6544610113736,1076.34681628114,510.40109094345));
#114623=CARTESIAN_POINT('Ctrl Pts',(44.6751678808445,1076.34392071567,510.440810837595));
#114624=CARTESIAN_POINT('Ctrl Pts',(44.7248188201033,1076.33529466325,510.564612268263));
#114625=CARTESIAN_POINT('Ctrl Pts',(44.7413041669408,1076.32966310519,510.652660939925));
#114626=CARTESIAN_POINT('Ctrl Pts',(44.7392854090862,1076.31929313078,510.830041948944));
#114627=CARTESIAN_POINT('Ctrl Pts',(44.7208320987569,1076.31465481247,510.917666177242));
#114628=CARTESIAN_POINT('Ctrl Pts',(44.6511545552143,1076.30706721385,511.080631198303));
#114629=CARTESIAN_POINT('Ctrl Pts',(44.6006845645422,1076.30418898174,511.154416852484));
#114630=CARTESIAN_POINT('Ctrl Pts',(44.4742704873603,1076.30064035351,511.278165817368));
#114631=CARTESIAN_POINT('Ctrl Pts',(44.3996341008144,1076.29999935545,511.326982776317));
#114632=CARTESIAN_POINT('Ctrl Pts',(44.2373389937831,1076.30105501513,511.392491591372));
#114633=CARTESIAN_POINT('Ctrl Pts',(44.1515008222423,1076.30269733816,511.40914915545));
#114634=CARTESIAN_POINT('Ctrl Pts',(44.0648939479111,1076.3053526307,511.40914915545));
#114635=CARTESIAN_POINT('Origin',(37.1057957606637,1067.7251047501,522.70822837456));
#114636=CARTESIAN_POINT('',(37.1057957606635,1077.76997147869,521.609397238568));
#114637=CARTESIAN_POINT('Ctrl Pts',(37.105796071773,1077.55793163415,523.807059510553));
#114638=CARTESIAN_POINT('Ctrl Pts',(37.1819019257861,1077.55505615697,523.807059489005));
#114639=CARTESIAN_POINT('Ctrl Pts',(37.2578238143658,1077.55297387967,523.799152773324));
#114640=CARTESIAN_POINT('Ctrl Pts',(37.3645577570114,1077.55118390574,523.776664777783));
#114641=CARTESIAN_POINT('Ctrl Pts',(37.396458676761,1077.55080014837,523.768430913599));
#114642=CARTESIAN_POINT('Ctrl Pts',(37.4476618495431,1077.5504329526,523.752729609035));
#114643=CARTESIAN_POINT('Ctrl Pts',(37.4672065256664,1077.55035358048,523.746128913403));
#114644=CARTESIAN_POINT('Ctrl Pts',(37.5075398463782,1077.55031767467,523.731229867817));
#114645=CARTESIAN_POINT('Ctrl Pts',(37.5282838381324,1077.55037212107,523.722838729423));
#114646=CARTESIAN_POINT('Ctrl Pts',(37.576364206958,1077.55067151241,523.701659422828));
#114647=CARTESIAN_POINT('Ctrl Pts',(37.6034576390165,1077.5509760974,523.688367344859));
#114648=CARTESIAN_POINT('Ctrl Pts',(37.6879499798836,1077.55236676043,523.64250806257));
#114649=CARTESIAN_POINT('Ctrl Pts',(37.7429664517361,1077.5539485014,523.605887400888));
#114650=CARTESIAN_POINT('Ctrl Pts',(37.9084498148921,1077.5609896708,523.472826242117));
#114651=CARTESIAN_POINT('Ctrl Pts',(38.002957898368,1077.56875414734,523.359294711216));
#114652=CARTESIAN_POINT('Ctrl Pts',(38.130756243618,1077.58742059887,523.122862458955));
#114653=CARTESIAN_POINT('Ctrl Pts',(38.1705473439029,1077.59748236801,523.006086264765));
#114654=CARTESIAN_POINT('Ctrl Pts',(38.2116478943223,1077.62070901741,522.754324456711));
#114655=CARTESIAN_POINT('Ctrl Pts',(38.2091216107585,1077.63387499693,522.620656571859));
#114656=CARTESIAN_POINT('Ctrl Pts',(38.1546822006451,1077.66205431621,522.351051892117));
#114657=CARTESIAN_POINT('Ctrl Pts',(38.0995662146793,1077.67687387527,522.218158104341));
#114658=CARTESIAN_POINT('Ctrl Pts',(37.9403429117606,1077.70553180493,521.978880915739));
#114659=CARTESIAN_POINT('Ctrl Pts',(37.8369620251451,1077.71907922308,521.875235883165));
#114660=CARTESIAN_POINT('Ctrl Pts',(37.6029661902064,1077.74218224825,521.718863919753));
#114661=CARTESIAN_POINT('Ctrl Pts',(37.4763834979393,1077.75173227366,521.664795578838));
#114662=CARTESIAN_POINT('Ctrl Pts',(37.2111042970911,1077.76657770235,521.6061438797));
#114663=CARTESIAN_POINT('Ctrl Pts',(37.0748600856621,1077.77179152888,521.601536093843));
#114664=CARTESIAN_POINT('Ctrl Pts',(36.8986797266645,1077.77549923438,521.628239431293));
#114665=CARTESIAN_POINT('Ctrl Pts',(36.8566407122039,1077.77614728576,521.637156220384));
#114666=CARTESIAN_POINT('Ctrl Pts',(36.7910551103268,1077.77678054124,521.655139366435));
#114667=CARTESIAN_POINT('Ctrl Pts',(36.7671154058867,1077.77692917591,521.662592777791));
#114668=CARTESIAN_POINT('Ctrl Pts',(36.7229586896977,1077.77704792792,521.678016348418));
#114669=CARTESIAN_POINT('Ctrl Pts',(36.7026828497048,1077.77703927433,521.685779833696));
#114670=CARTESIAN_POINT('Ctrl Pts',(36.6583937387185,1077.77687919045,521.704260186241));
#114671=CARTESIAN_POINT('Ctrl Pts',(36.6345086993071,1077.77669809368,521.71524845123));
#114672=CARTESIAN_POINT('Ctrl Pts',(36.5679567870713,1077.77592044874,521.748808033854));
#114673=CARTESIAN_POINT('Ctrl Pts',(36.5263547884368,1077.77510407087,521.773345870686));
#114674=CARTESIAN_POINT('Ctrl Pts',(36.3656670996843,1077.77056903018,521.882978084723));
#114675=CARTESIAN_POINT('Ctrl Pts',(36.2625918330275,1077.76437348841,521.988662511923));
#114676=CARTESIAN_POINT('Ctrl Pts',(36.1179449472872,1077.74858960728,522.212217070053));
#114677=CARTESIAN_POINT('Ctrl Pts',(36.0697035921556,1077.7399034487,522.323075230964));
#114678=CARTESIAN_POINT('Ctrl Pts',(36.0083464475759,1077.71914163,522.566278725154));
#114679=CARTESIAN_POINT('Ctrl Pts',(35.9992758314291,1077.70699385866,522.697733005839));
#114680=CARTESIAN_POINT('Ctrl Pts',(36.0287616905797,1077.68013756808,522.967549583484));
#114681=CARTESIAN_POINT('Ctrl Pts',(36.0708063740701,1077.66554281071,523.103237129484));
#114682=CARTESIAN_POINT('Ctrl Pts',(36.2060059036698,1077.63611499291,523.355511024951));
#114683=CARTESIAN_POINT('Ctrl Pts',(36.2995553167718,1077.62157094099,523.46889853725));
#114684=CARTESIAN_POINT('Ctrl Pts',(36.4915780543861,1077.59907319862,523.625037468314));
#114685=CARTESIAN_POINT('Ctrl Pts',(36.5792029394156,1077.59056060109,523.678038219772));
#114686=CARTESIAN_POINT('Ctrl Pts',(36.7311004545636,1077.57841278622,523.743137440291));
#114687=CARTESIAN_POINT('Ctrl Pts',(36.7913285133599,1077.57417549172,523.76300372559));
#114688=CARTESIAN_POINT('Ctrl Pts',(36.9357690856537,1077.56534056385,523.797155110267));
#114689=CARTESIAN_POINT('Ctrl Pts',(37.0206155941158,1077.56114997422,523.80705953467));
#114690=CARTESIAN_POINT('Ctrl Pts',(37.105796071773,1077.55793163415,523.807059510553));
#114691=CARTESIAN_POINT('',(37.1057957606431,1075.76001126608,521.609397238568));
#114692=CARTESIAN_POINT('',(37.1057957606637,1067.7251047501,521.609397238568));
#114693=CARTESIAN_POINT('Ctrl Pts',(37.1058085229615,1075.54602936729,523.807059510479));
#114694=CARTESIAN_POINT('Ctrl Pts',(36.962618776904,1075.55148807702,523.807061173546));
#114695=CARTESIAN_POINT('Ctrl Pts',(36.820944062981,1075.55969809754,523.779077062919));
#114696=CARTESIAN_POINT('Ctrl Pts',(36.5557180154681,1075.58062367947,523.670262608626));
#114697=CARTESIAN_POINT('Ctrl Pts',(36.4348455022318,1075.59315951082,523.590183173545));
#114698=CARTESIAN_POINT('Ctrl Pts',(36.2302689579569,1075.62084154858,523.387724464143));
#114699=CARTESIAN_POINT('Ctrl Pts',(36.1487230710439,1075.63573855628,523.267014954714));
#114700=CARTESIAN_POINT('Ctrl Pts',(36.0649907979957,1075.65825363871,523.067833724736));
#114701=CARTESIAN_POINT('Ctrl Pts',(36.0437090753994,1075.66572117715,522.999028954527));
#114702=CARTESIAN_POINT('Ctrl Pts',(36.0000341115014,1075.68797032344,522.785712403809));
#114703=CARTESIAN_POINT('Ctrl Pts',(35.9995046517734,1075.70214461371,522.638284032741));
#114704=CARTESIAN_POINT('Ctrl Pts',(36.0560928927073,1075.72739320482,522.352250426399));
#114705=CARTESIAN_POINT('Ctrl Pts',(36.1124217679349,1075.73823577623,522.216408218919));
#114706=CARTESIAN_POINT('Ctrl Pts',(36.275083603449,1075.75526553076,521.974312345321));
#114707=CARTESIAN_POINT('Ctrl Pts',(36.3798167189253,1075.76127923228,521.870535446229));
#114708=CARTESIAN_POINT('Ctrl Pts',(36.6228750045003,1075.76764624752,521.710633225511));
#114709=CARTESIAN_POINT('Ctrl Pts',(36.7584387976241,1075.7679844608,521.65572882712));
#114710=CARTESIAN_POINT('Ctrl Pts',(37.0443266705674,1075.76294126561,521.60142655478));
#114711=CARTESIAN_POINT('Ctrl Pts',(37.1918160398829,1075.75755997854,521.603088103954));
#114712=CARTESIAN_POINT('Ctrl Pts',(37.4771699604814,1075.7416667549,521.663831536216));
#114713=CARTESIAN_POINT('Ctrl Pts',(37.6121558493899,1075.73131925553,521.722225884631));
#114714=CARTESIAN_POINT('Ctrl Pts',(37.8517472187289,1075.70686501772,521.888286373147));
#114715=CARTESIAN_POINT('Ctrl Pts',(37.9538798086312,1075.69298431231,521.994479518879));
#114716=CARTESIAN_POINT('Ctrl Pts',(38.1112913603744,1075.66337753341,522.241314981971));
#114717=CARTESIAN_POINT('Ctrl Pts',(38.1646495489176,1075.6479250309,522.379822325483));
#114718=CARTESIAN_POINT('Ctrl Pts',(38.2135845009188,1075.61776955795,522.668693638895));
#114719=CARTESIAN_POINT('Ctrl Pts',(38.209043326696,1075.6033529045,522.816211823732));
#114720=CARTESIAN_POINT('Ctrl Pts',(38.142835677807,1075.57771197269,523.099136293412));
#114721=CARTESIAN_POINT('Ctrl Pts',(38.0825476903773,1075.56669678043,523.231966100617));
#114722=CARTESIAN_POINT('Ctrl Pts',(37.9143117441168,1075.5495760996,523.466106350132));
#114723=CARTESIAN_POINT('Ctrl Pts',(37.8083228233454,1075.54361032715,523.565312995936));
#114724=CARTESIAN_POINT('Ctrl Pts',(37.5645628638608,1075.53761517467,523.716918627914));
#114725=CARTESIAN_POINT('Ctrl Pts',(37.4293911130489,1075.53761606337,523.768044094385));
#114726=CARTESIAN_POINT('Ctrl Pts',(37.2279325124291,1075.54188513668,523.801960689426));
#114727=CARTESIAN_POINT('Ctrl Pts',(37.1669160619767,1075.54369981279,523.80705880075));
#114728=CARTESIAN_POINT('Ctrl Pts',(37.1058085229615,1075.54602936729,523.807059510479));
#114729=CARTESIAN_POINT('Origin',(37.1057957606637,1067.7251047501,522.70822837456));
#114730=CARTESIAN_POINT('',(37.1057957606637,1075.60643384366,523.207059510553));
#114731=CARTESIAN_POINT('',(37.1057957606638,1075.70357965628,522.209397238568));
#114732=CARTESIAN_POINT('Ctrl Pts',(37.1057957606637,1075.60643384366,523.207059510553));
#114733=CARTESIAN_POINT('Ctrl Pts',(37.0715278617885,1075.60771635452,523.207059510553));
#114734=CARTESIAN_POINT('Ctrl Pts',(37.0372821742987,1075.60934665592,523.203528331015));
#114735=CARTESIAN_POINT('Ctrl Pts',(36.9397986981363,1075.61500489314,523.183125618715));
#114736=CARTESIAN_POINT('Ctrl Pts',(36.8792909601871,1075.61980011443,523.157406655478));
#114737=CARTESIAN_POINT('Ctrl Pts',(36.7713261037424,1075.6310295087,523.084057867589));
#114738=CARTESIAN_POINT('Ctrl Pts',(36.7249865915008,1075.63736525146,523.036998776482));
#114739=CARTESIAN_POINT('Ctrl Pts',(36.6711059659364,1075.64736299764,522.95509753201));
#114740=CARTESIAN_POINT('Ctrl Pts',(36.6558783678005,1075.65075368797,522.926112470758));
#114741=CARTESIAN_POINT('Ctrl Pts',(36.6313332594527,1075.65754877975,522.86564658854));
#114742=CARTESIAN_POINT('Ctrl Pts',(36.6220612865006,1075.66093749477,522.834309770799));
#114743=CARTESIAN_POINT('Ctrl Pts',(36.6033808891434,1075.67106949781,522.737020463842));
#114744=CARTESIAN_POINT('Ctrl Pts',(36.6040095655807,1075.6775436533,522.669854002592));
#114745=CARTESIAN_POINT('Ctrl Pts',(36.6315873077625,1075.68908235576,522.539806990181));
#114746=CARTESIAN_POINT('Ctrl Pts',(36.6581982056893,1075.69403710896,522.478199419826));
#114747=CARTESIAN_POINT('Ctrl Pts',(36.7337017348081,1075.70172462878,522.36954278163));
#114748=CARTESIAN_POINT('Ctrl Pts',(36.7815977993668,1075.704404469,522.32343008279));
#114749=CARTESIAN_POINT('Ctrl Pts',(36.8918809489161,1075.70715944505,522.252928195246));
#114750=CARTESIAN_POINT('Ctrl Pts',(36.9529692099161,1075.70724196444,522.228955747049));
#114751=CARTESIAN_POINT('Ctrl Pts',(37.0462652018157,1075.70548062127,522.212066026661));
#114752=CARTESIAN_POINT('Ctrl Pts',(37.0760029825362,1075.70465924766,522.209397238568));
#114753=CARTESIAN_POINT('Ctrl Pts',(37.1057957606639,1075.70357965628,522.209397238568));
#114754=CARTESIAN_POINT('',(37.1057957606637,1082.7251047501,522.209397238568));
#114755=CARTESIAN_POINT('',(37.1057957606637,1067.7251047501,522.209397238568));
#114756=CARTESIAN_POINT('Origin',(37.1057957606637,1082.7251047501,522.70822837456));
#114757=CARTESIAN_POINT('Ctrl Pts',(37.1057981350553,1075.70357957024,522.209397238574));
#114758=CARTESIAN_POINT('Ctrl Pts',(37.1709760170612,1075.70121771037,522.209397548814));
#114759=CARTESIAN_POINT('Ctrl Pts',(37.2354654141579,1075.69765473122,522.22217096653));
#114760=CARTESIAN_POINT('Ctrl Pts',(37.3571418365381,1075.68841522189,522.272245048994));
#114761=CARTESIAN_POINT('Ctrl Pts',(37.4129068670046,1075.68278623442,522.309577632184));
#114762=CARTESIAN_POINT('Ctrl Pts',(37.5066358474258,1075.6702348421,522.403931631854));
#114763=CARTESIAN_POINT('Ctrl Pts',(37.5436188803242,1075.6634310619,522.460091045283));
#114764=CARTESIAN_POINT('Ctrl Pts',(37.5806691086318,1075.65311475641,522.552054126811));
#114765=CARTESIAN_POINT('Ctrl Pts',(37.5898582728438,1075.64971799561,522.583413152199));
#114766=CARTESIAN_POINT('Ctrl Pts',(37.6083628897596,1075.63948692928,522.681164147311));
#114767=CARTESIAN_POINT('Ctrl Pts',(37.6074680466773,1075.63289357422,522.74876246245));
#114768=CARTESIAN_POINT('Ctrl Pts',(37.5793307466939,1075.62121979839,522.878177227253));
#114769=CARTESIAN_POINT('Ctrl Pts',(37.552951258777,1075.61622087836,522.938851680759));
#114770=CARTESIAN_POINT('Ctrl Pts',(37.4783575255633,1075.60839855439,523.046282286457));
#114771=CARTESIAN_POINT('Ctrl Pts',(37.4310075752998,1075.60563935457,523.092067615194));
#114772=CARTESIAN_POINT('Ctrl Pts',(37.3215124375085,1075.60274958377,523.162676949381));
#114773=CARTESIAN_POINT('Ctrl Pts',(37.2605243187527,1075.60263640758,523.186889878728));
#114774=CARTESIAN_POINT('Ctrl Pts',(37.1665751422606,1075.60443311762,523.204284112385));
#114775=CARTESIAN_POINT('Ctrl Pts',(37.1361767225813,1075.60529680536,523.207059510553));
#114776=CARTESIAN_POINT('Ctrl Pts',(37.1057957606637,1075.60643384366,523.207059510553));
#114777=CARTESIAN_POINT('Origin',(27.7552687727514,1067.7251047501,533.110228186055));
#114778=CARTESIAN_POINT('',(27.7552687727512,1076.95995571924,532.019687437326));
#114779=CARTESIAN_POINT('Ctrl Pts',(27.7552666781061,1076.67624978494,534.200768934781));
#114780=CARTESIAN_POINT('Ctrl Pts',(27.800749602656,1076.67470112636,534.200769022142));
#114781=CARTESIAN_POINT('Ctrl Pts',(27.8461978020645,1076.67353183618,534.197923695252));
#114782=CARTESIAN_POINT('Ctrl Pts',(27.9202859703263,1076.67224859531,534.188606269179));
#114783=CARTESIAN_POINT('Ctrl Pts',(27.9490713776196,1076.67190703409,534.183806659105));
#114784=CARTESIAN_POINT('Ctrl Pts',(28.000031619331,1076.67158427493,534.173192816812));
#114785=CARTESIAN_POINT('Ctrl Pts',(28.022279584309,1076.6715413264,534.167823525971));
#114786=CARTESIAN_POINT('Ctrl Pts',(28.0685879420242,1076.67165897254,534.155093009102));
#114787=CARTESIAN_POINT('Ctrl Pts',(28.0925949574108,1076.67184008849,534.147591363473));
#114788=CARTESIAN_POINT('Ctrl Pts',(28.1542564602887,1076.67262044846,534.125956624133));
#114789=CARTESIAN_POINT('Ctrl Pts',(28.1914219166206,1076.67340452834,534.110560598595));
#114790=CARTESIAN_POINT('Ctrl Pts',(28.3376377751246,1076.67777938803,534.040291359133));
#114791=CARTESIAN_POINT('Ctrl Pts',(28.4378636452712,1076.68380228948,533.969400135769));
#114792=CARTESIAN_POINT('Ctrl Pts',(28.6057555957578,1076.70026506997,533.802450261603));
#114793=CARTESIAN_POINT('Ctrl Pts',(28.6738386372743,1076.71033096995,533.70910811931));
#114794=CARTESIAN_POINT('Ctrl Pts',(28.7835396313896,1076.73495241998,533.494739986341));
#114795=CARTESIAN_POINT('Ctrl Pts',(28.8210108220568,1076.74967109205,533.373481699937));
#114796=CARTESIAN_POINT('Ctrl Pts',(28.8542567229034,1076.78264658264,533.113742631473));
#114797=CARTESIAN_POINT('Ctrl Pts',(28.8461184918472,1076.8008176166,532.976827028232));
#114798=CARTESIAN_POINT('Ctrl Pts',(28.7774301812217,1076.83874892362,532.702876802798));
#114799=CARTESIAN_POINT('Ctrl Pts',(28.7134872748216,1076.85816056167,532.569277953425));
#114800=CARTESIAN_POINT('Ctrl Pts',(28.5394386091861,1076.89354471149,532.33922403747));
#114801=CARTESIAN_POINT('Ctrl Pts',(28.4325676500709,1076.90928968887,532.243765569968));
#114802=CARTESIAN_POINT('Ctrl Pts',(28.198283894545,1076.93465255479,532.105284488169));
#114803=CARTESIAN_POINT('Ctrl Pts',(28.0753043849492,1076.94447690571,532.059588121092));
#114804=CARTESIAN_POINT('Ctrl Pts',(27.8571232945171,1076.95652961713,532.020623011117));
#114805=CARTESIAN_POINT('Ctrl Pts',(27.7655359639275,1076.96010199512,532.015911833822));
#114806=CARTESIAN_POINT('Ctrl Pts',(27.6380366991379,1076.96303829024,532.025394453301));
#114807=CARTESIAN_POINT('Ctrl Pts',(27.6018434293981,1076.96363909349,532.029918589574));
#114808=CARTESIAN_POINT('Ctrl Pts',(27.5421593853192,1076.96424144684,532.040440048664));
#114809=CARTESIAN_POINT('Ctrl Pts',(27.5185228853992,1076.96437664828,532.045421295655));
#114810=CARTESIAN_POINT('Ctrl Pts',(27.4727721014839,1076.96443550985,532.056661862207));
#114811=CARTESIAN_POINT('Ctrl Pts',(27.4506523051707,1076.96436923202,532.062843274559));
#114812=CARTESIAN_POINT('Ctrl Pts',(27.3994327987842,1076.96399247307,532.078916562617));
#114813=CARTESIAN_POINT('Ctrl Pts',(27.3705249246315,1076.96360721627,532.089348751169));
#114814=CARTESIAN_POINT('Ctrl Pts',(27.2809730208945,1076.96186225852,532.126010163014));
#114815=CARTESIAN_POINT('Ctrl Pts',(27.2222685165802,1076.95989538189,532.156526763776));
#114816=CARTESIAN_POINT('Ctrl Pts',(27.044554732498,1076.95119820474,532.270456348092));
#114817=CARTESIAN_POINT('Ctrl Pts',(26.9394344356685,1076.94167724829,532.372237845655));
#114818=CARTESIAN_POINT('Ctrl Pts',(26.7879367113717,1076.91856004502,532.592059044527));
#114819=CARTESIAN_POINT('Ctrl Pts',(26.7360734287624,1076.90598935935,532.703547791886));
#114820=CARTESIAN_POINT('Ctrl Pts',(26.6685710651777,1076.87665623319,532.949064822446));
#114821=CARTESIAN_POINT('Ctrl Pts',(26.6570743079382,1076.85985871735,533.082220851289));
#114822=CARTESIAN_POINT('Ctrl Pts',(26.6832874301669,1076.82346282728,533.356326910267));
#114823=CARTESIAN_POINT('Ctrl Pts',(26.7247353072037,1076.80407814151,533.494563715906));
#114824=CARTESIAN_POINT('Ctrl Pts',(26.8590102789459,1076.76643226086,533.747944510667));
#114825=CARTESIAN_POINT('Ctrl Pts',(26.9509091231919,1076.7485268945,533.860606582479));
#114826=CARTESIAN_POINT('Ctrl Pts',(27.1658328961315,1076.71793165164,534.037511776423));
#114827=CARTESIAN_POINT('Ctrl Pts',(27.284473001473,1076.70522493337,534.103080083893));
#114828=CARTESIAN_POINT('Ctrl Pts',(27.5227928918663,1076.68665474553,534.182044894166));
#114829=CARTESIAN_POINT('Ctrl Pts',(27.638588818275,1076.68022257627,534.200768710673));
#114830=CARTESIAN_POINT('Ctrl Pts',(27.7552666781061,1076.67624978494,534.200768934781));
#114831=CARTESIAN_POINT('',(27.7552687727293,1074.94285725241,532.019687437326));
#114832=CARTESIAN_POINT('',(27.7552687727514,1067.7251047501,532.019687437326));
#114833=CARTESIAN_POINT('Ctrl Pts',(27.755275424151,1074.65680217842,534.200768934763));
#114834=CARTESIAN_POINT('Ctrl Pts',(27.6136253996526,1074.66166448356,534.200769798711));
#114835=CARTESIAN_POINT('Ctrl Pts',(27.4735280043461,1074.67017283515,534.173176636777));
#114836=CARTESIAN_POINT('Ctrl Pts',(27.2108671662123,1074.69350273941,534.065845243065));
#114837=CARTESIAN_POINT('Ctrl Pts',(27.0910484391902,1074.70814472328,533.986729086362));
#114838=CARTESIAN_POINT('Ctrl Pts',(26.8877068762176,1074.74165627613,533.786390102643));
#114839=CARTESIAN_POINT('Ctrl Pts',(26.8064892950006,1074.76024863888,533.666639584316));
#114840=CARTESIAN_POINT('Ctrl Pts',(26.7229560449997,1074.7890820409,533.468988528123));
#114841=CARTESIAN_POINT('Ctrl Pts',(26.7016858388308,1074.79877338609,533.400642763769));
#114842=CARTESIAN_POINT('Ctrl Pts',(26.6579396846555,1074.82800508257,533.188738752911));
#114843=CARTESIAN_POINT('Ctrl Pts',(26.6572064079259,1074.84713066521,533.042212086953));
#114844=CARTESIAN_POINT('Ctrl Pts',(26.7131036243726,1074.8821553278,532.758073590742));
#114845=CARTESIAN_POINT('Ctrl Pts',(26.7688679879507,1074.89774018205,532.623125712085));
#114846=CARTESIAN_POINT('Ctrl Pts',(26.9301219154371,1074.92339221948,532.382665414629));
#114847=CARTESIAN_POINT('Ctrl Pts',(27.033942798244,1074.9332082023,532.279551635639));
#114848=CARTESIAN_POINT('Ctrl Pts',(27.2733725151368,1074.94557923062,532.121733319789));
#114849=CARTESIAN_POINT('Ctrl Pts',(27.4057662935109,1074.94817794078,532.067525467788));
#114850=CARTESIAN_POINT('Ctrl Pts',(27.6840218614343,1074.94606974451,532.012817250953));
#114851=CARTESIAN_POINT('Ctrl Pts',(27.8270551253356,1074.94138305118,532.012880236067));
#114852=CARTESIAN_POINT('Ctrl Pts',(28.1082300688142,1074.92505604725,532.068249721328));
#114853=CARTESIAN_POINT('Ctrl Pts',(28.2432401627996,1074.91342028451,532.124300675689));
#114854=CARTESIAN_POINT('Ctrl Pts',(28.4834925723629,1074.88467231471,532.285634813647));
#114855=CARTESIAN_POINT('Ctrl Pts',(28.5862764841568,1074.86783197128,532.389418357372));
#114856=CARTESIAN_POINT('Ctrl Pts',(28.7047763799925,1074.84049411415,532.569176746184));
#114857=CARTESIAN_POINT('Ctrl Pts',(28.7379040672622,1074.83119757991,532.631980612322));
#114858=CARTESIAN_POINT('Ctrl Pts',(28.7915935595026,1074.81223324189,532.763298958413));
#114859=CARTESIAN_POINT('Ctrl Pts',(28.8119899361011,1074.80260655093,532.831539942821));
#114860=CARTESIAN_POINT('Ctrl Pts',(28.8536452009153,1074.77317887653,533.044908497349));
#114861=CARTESIAN_POINT('Ctrl Pts',(28.8525099084244,1074.75368525076,533.192844219449));
#114862=CARTESIAN_POINT('Ctrl Pts',(28.7923690303293,1074.7180903992,533.476735824113));
#114863=CARTESIAN_POINT('Ctrl Pts',(28.7350936718625,1074.70226461112,533.610210217195));
#114864=CARTESIAN_POINT('Ctrl Pts',(28.5724437477429,1074.67629286926,533.846332736054));
#114865=CARTESIAN_POINT('Ctrl Pts',(28.469141521979,1074.66634798717,533.946967242136));
#114866=CARTESIAN_POINT('Ctrl Pts',(28.2302627188289,1074.6537424931,534.10207169616));
#114867=CARTESIAN_POINT('Ctrl Pts',(28.0974024754569,1074.65114515647,534.155385465907));
#114868=CARTESIAN_POINT('Ctrl Pts',(27.8911442059687,1074.65299064074,534.194408051689));
#114869=CARTESIAN_POINT('Ctrl Pts',(27.8232750413236,1074.65446801089,534.200768520021));
#114870=CARTESIAN_POINT('Ctrl Pts',(27.755275424151,1074.65680217842,534.200768934763));
#114871=CARTESIAN_POINT('Origin',(27.7552687727514,1067.7251047501,533.110228186055));
#114872=CARTESIAN_POINT('',(27.7552687727514,1074.73740020174,533.600768934783));
#114873=CARTESIAN_POINT('',(27.7552687727514,1074.86607808781,532.619687437326));
#114874=CARTESIAN_POINT('Ctrl Pts',(27.7552687727514,1074.73740020174,533.600768934783));
#114875=CARTESIAN_POINT('Ctrl Pts',(27.7217220514107,1074.73853763052,533.600768934783));
#114876=CARTESIAN_POINT('Ctrl Pts',(27.6881995638384,1074.74013005689,533.597327622873));
#114877=CARTESIAN_POINT('Ctrl Pts',(27.5926310129866,1074.74600435434,533.577420134648));
#114878=CARTESIAN_POINT('Ctrl Pts',(27.5332872568249,1074.75133989622,533.552288455029));
#114879=CARTESIAN_POINT('Ctrl Pts',(27.427153033961,1074.76440786162,533.480519027331));
#114880=CARTESIAN_POINT('Ctrl Pts',(27.3815200989915,1074.7720368498,533.434363159037));
#114881=CARTESIAN_POINT('Ctrl Pts',(27.3283822682814,1074.78440280468,533.35401244561));
#114882=CARTESIAN_POINT('Ctrl Pts',(27.3133399123249,1074.7886527102,533.325542322099));
#114883=CARTESIAN_POINT('Ctrl Pts',(27.2890584726604,1074.79727255547,533.266133892481));
#114884=CARTESIAN_POINT('Ctrl Pts',(27.2798663335074,1074.80162300998,533.235331970339));
#114885=CARTESIAN_POINT('Ctrl Pts',(27.2612704923806,1074.81478286354,533.139694328085));
#114886=CARTESIAN_POINT('Ctrl Pts',(27.2617330322699,1074.82340768767,533.073626534165));
#114887=CARTESIAN_POINT('Ctrl Pts',(27.2885631672471,1074.83921156428,532.945689302679));
#114888=CARTESIAN_POINT('Ctrl Pts',(27.3145829076547,1074.84624380939,532.885037407387));
#114889=CARTESIAN_POINT('Ctrl Pts',(27.388561934187,1074.85769618983,532.778069288628));
#114890=CARTESIAN_POINT('Ctrl Pts',(27.4354966049048,1074.86203580859,532.7326397653));
#114891=CARTESIAN_POINT('Ctrl Pts',(27.5435969923283,1074.86746688699,532.663141308034));
#114892=CARTESIAN_POINT('Ctrl Pts',(27.603431634089,1074.86855547558,532.639437617623));
#114893=CARTESIAN_POINT('Ctrl Pts',(27.6955543522107,1074.86770593739,532.622418338912));
#114894=CARTESIAN_POINT('Ctrl Pts',(27.7253834821696,1074.86707024684,532.619687437326));
#114895=CARTESIAN_POINT('Ctrl Pts',(27.7552687727515,1074.86607808781,532.619687437326));
#114896=CARTESIAN_POINT('',(27.7552687727514,1082.7251047501,532.619687437326));
#114897=CARTESIAN_POINT('',(27.7552687727514,1067.7251047501,532.619687437326));
#114898=CARTESIAN_POINT('Origin',(27.7552687727514,1082.7251047501,533.110228186055));
#114899=CARTESIAN_POINT('Ctrl Pts',(27.7552701015566,1074.86607804369,532.619687437328));
#114900=CARTESIAN_POINT('Ctrl Pts',(27.8191337024483,1074.86395781937,532.619687610326));
#114901=CARTESIAN_POINT('Ctrl Pts',(27.8822994455548,1074.86024186908,532.63215767805));
#114902=CARTESIAN_POINT('Ctrl Pts',(28.0018273593798,1074.84989940556,532.681129971462));
#114903=CARTESIAN_POINT('Ctrl Pts',(28.0567224362022,1074.84330132016,532.717782421802));
#114904=CARTESIAN_POINT('Ctrl Pts',(28.1489781808369,1074.82814462366,532.81038119986));
#114905=CARTESIAN_POINT('Ctrl Pts',(28.1853811897379,1074.81972767506,532.865482372977));
#114906=CARTESIAN_POINT('Ctrl Pts',(28.2219278451578,1074.80668908636,532.955684646427));
#114907=CARTESIAN_POINT('Ctrl Pts',(28.2310129009365,1074.80235096542,532.986447773686));
#114908=CARTESIAN_POINT('Ctrl Pts',(28.2493971918684,1074.78914652732,533.082348995895));
#114909=CARTESIAN_POINT('Ctrl Pts',(28.2486991028959,1074.78044035288,533.148707651386));
#114910=CARTESIAN_POINT('Ctrl Pts',(28.2212979116833,1074.76451019408,533.276587597903));
#114911=CARTESIAN_POINT('Ctrl Pts',(28.1951436695123,1074.75742307522,533.336935756115));
#114912=CARTESIAN_POINT('Ctrl Pts',(28.1212511010678,1074.74588577366,533.443088602389));
#114913=CARTESIAN_POINT('Ctrl Pts',(28.0746167460702,1074.74150513762,533.488090561853));
#114914=CARTESIAN_POINT('Ctrl Pts',(27.9669175562519,1074.73598171402,533.557328621623));
#114915=CARTESIAN_POINT('Ctrl Pts',(27.907062940919,1074.73486832538,533.581035451629));
#114916=CARTESIAN_POINT('Ctrl Pts',(27.8148661819697,1074.7357389034,533.598055532107));
#114917=CARTESIAN_POINT('Ctrl Pts',(27.7850579233091,1074.73639017645,533.600768934783));
#114918=CARTESIAN_POINT('Ctrl Pts',(27.7552687727514,1074.73740020174,533.600768934783));
#114919=CARTESIAN_POINT('Origin',(63.8195601713296,1067.7251047501,487.451286405902));
#114920=CARTESIAN_POINT('',(63.8195601713476,1078.69713855509,485.972983273709));
#114921=CARTESIAN_POINT('Ctrl Pts',(63.8195894624746,1078.64371854035,488.929589537805));
#114922=CARTESIAN_POINT('Ctrl Pts',(63.9840898466471,1078.64006414708,488.929586278389));
#114923=CARTESIAN_POINT('Ctrl Pts',(64.147453182996,1078.63693311643,488.902125535132));
#114924=CARTESIAN_POINT('Ctrl Pts',(64.437514187406,1078.63248760894,488.801765362934));
#114925=CARTESIAN_POINT('Ctrl Pts',(64.5646691439413,1078.63100970525,488.73599521947));
#114926=CARTESIAN_POINT('Ctrl Pts',(64.7189173791907,1078.62993169095,488.625499302091));
#114927=CARTESIAN_POINT('Ctrl Pts',(64.7560404026802,1078.62973703954,488.596111347511));
#114928=CARTESIAN_POINT('Ctrl Pts',(64.8133215019525,1078.62954551861,488.546111962442));
#114929=CARTESIAN_POINT('Ctrl Pts',(64.8343982379717,1078.62950100682,488.526604165847));
#114930=CARTESIAN_POINT('Ctrl Pts',(64.8731922603131,1078.62946960111,488.488540842801));
#114931=CARTESIAN_POINT('Ctrl Pts',(64.8910209072986,1078.62947704804,488.470113788901));
#114932=CARTESIAN_POINT('Ctrl Pts',(64.9300915952786,1078.62954395193,488.427571284039));
#114933=CARTESIAN_POINT('Ctrl Pts',(64.951044729482,1078.62961608325,488.403208089341));
#114934=CARTESIAN_POINT('Ctrl Pts',(65.0104014475364,1078.62993091023,488.329459941845));
#114935=CARTESIAN_POINT('Ctrl Pts',(65.0464836543618,1078.63027019842,488.278299281655));
#114936=CARTESIAN_POINT('Ctrl Pts',(65.1824631487881,1078.63220921733,488.056918116752));
#114937=CARTESIAN_POINT('Ctrl Pts',(65.2510196528309,1078.63493719783,487.869863677846));
#114938=CARTESIAN_POINT('Ctrl Pts',(65.3051133784915,1078.64163702959,487.516357727991));
#114939=CARTESIAN_POINT('Ctrl Pts',(65.3034107651073,1078.64523225297,487.354934841883));
#114940=CARTESIAN_POINT('Ctrl Pts',(65.2458715016793,1078.65347085552,487.025462902417));
#114941=CARTESIAN_POINT('Ctrl Pts',(65.1858597232329,1078.6581094606,486.860598750576));
#114942=CARTESIAN_POINT('Ctrl Pts',(65.0049664543459,1078.6678008949,486.548496327283));
#114943=CARTESIAN_POINT('Ctrl Pts',(64.8816253042141,1078.67276842342,486.406183838743));
#114944=CARTESIAN_POINT('Ctrl Pts',(64.5816898614871,1078.68223686314,486.169608074433));
#114945=CARTESIAN_POINT('Ctrl Pts',(64.4058327386662,1078.68661221552,486.080215823895));
#114946=CARTESIAN_POINT('Ctrl Pts',(64.0355180964178,1078.69399347682,485.976661019645));
#114947=CARTESIAN_POINT('Ctrl Pts',(63.8452519507421,1078.69697667558,485.961150441436));
#114948=CARTESIAN_POINT('Ctrl Pts',(63.4806169621885,1078.70150019059,486.001434944975));
#114949=CARTESIAN_POINT('Ctrl Pts',(63.3089580462608,1078.70308592756,486.052629611219));
#114950=CARTESIAN_POINT('Ctrl Pts',(63.0679258473507,1078.70464054665,486.174962862035));
#114951=CARTESIAN_POINT('Ctrl Pts',(62.9894673987184,1078.70501590523,486.224541866277));
#114952=CARTESIAN_POINT('Ctrl Pts',(62.8854961345996,1078.70533108904,486.3048110849));
#114953=CARTESIAN_POINT('Ctrl Pts',(62.855770519636,1078.70539704804,486.32968451552));
#114954=CARTESIAN_POINT('Ctrl Pts',(62.8093655331422,1078.70546021506,486.371723182413));
#114955=CARTESIAN_POINT('Ctrl Pts',(62.7920654195967,1078.70547408171,486.388175642058));
#114956=CARTESIAN_POINT('Ctrl Pts',(62.7570371306505,1078.70548167735,486.423141733429));
#114957=CARTESIAN_POINT('Ctrl Pts',(62.7393766658493,1078.70547385276,486.441712102762));
#114958=CARTESIAN_POINT('Ctrl Pts',(62.6993217611342,1078.7054281524,486.486085583627));
#114959=CARTESIAN_POINT('Ctrl Pts',(62.6773212730456,1078.70538115618,486.512224630403));
#114960=CARTESIAN_POINT('Ctrl Pts',(62.6108178240106,1078.70516671632,486.597036886666));
#114961=CARTESIAN_POINT('Ctrl Pts',(62.5697811297559,1078.70492332943,486.658284164334));
#114962=CARTESIAN_POINT('Ctrl Pts',(62.4364455080255,1078.70366707218,486.893526027989));
#114963=CARTESIAN_POINT('Ctrl Pts',(62.3745669326555,1078.70206694927,487.082378659631));
#114964=CARTESIAN_POINT('Ctrl Pts',(62.3323635385775,1078.69778701519,487.439490572911));
#114965=CARTESIAN_POINT('Ctrl Pts',(62.3401010365273,1078.69536513719,487.603237256047));
#114966=CARTESIAN_POINT('Ctrl Pts',(62.4115688765271,1078.68929086434,487.935217194669));
#114967=CARTESIAN_POINT('Ctrl Pts',(62.479466096613,1078.6855952386,488.099953815447));
#114968=CARTESIAN_POINT('Ctrl Pts',(62.6772738206339,1078.67699747554,488.408695407246));
#114969=CARTESIAN_POINT('Ctrl Pts',(62.8095884730262,1078.67210254672,488.547371017869));
#114970=CARTESIAN_POINT('Ctrl Pts',(63.0788837150454,1078.66328789451,488.738313396836));
#114971=CARTESIAN_POINT('Ctrl Pts',(63.2042225570539,1078.65949593348,488.802730111167));
#114972=CARTESIAN_POINT('Ctrl Pts',(63.4920619879084,1078.65148856653,488.902192161214));
#114973=CARTESIAN_POINT('Ctrl Pts',(63.6552496452803,1078.6473693666,488.92959279404));
#114974=CARTESIAN_POINT('Ctrl Pts',(63.8195894624746,1078.64371854035,488.929589537805));
#114975=CARTESIAN_POINT('',(63.8195601713054,1076.69671505693,485.972983273709));
#114976=CARTESIAN_POINT('',(63.8195601713296,1067.7251047501,485.972983273709));
#114977=CARTESIAN_POINT('Ctrl Pts',(63.8196790295888,1076.64266067219,488.929589533317));
#114978=CARTESIAN_POINT('Ctrl Pts',(63.6266637061908,1076.64699817558,488.9296050521));
#114979=CARTESIAN_POINT('Ctrl Pts',(63.4355114909343,1076.65198209469,488.891818924218));
#114980=CARTESIAN_POINT('Ctrl Pts',(63.0783218190941,1076.66237653906,488.744844186407));
#114981=CARTESIAN_POINT('Ctrl Pts',(62.9157480424437,1076.6676822105,488.636972471792));
#114982=CARTESIAN_POINT('Ctrl Pts',(62.6412573598861,1076.67776335618,488.364723487194));
#114983=CARTESIAN_POINT('Ctrl Pts',(62.5320074252481,1076.6824408189,488.20293863512));
#114984=CARTESIAN_POINT('Ctrl Pts',(62.3813117723216,1076.69069166442,487.844855465753));
#114985=CARTESIAN_POINT('Ctrl Pts',(62.3419715931296,1076.69417867454,487.651775912808));
#114986=CARTESIAN_POINT('Ctrl Pts',(62.3405622868592,1076.69976087682,487.261618709333));
#114987=CARTESIAN_POINT('Ctrl Pts',(62.3784511593684,1076.70181077384,487.068377724351));
#114988=CARTESIAN_POINT('Ctrl Pts',(62.5273030519845,1076.70453642962,486.707150006348));
#114989=CARTESIAN_POINT('Ctrl Pts',(62.6370364788583,1076.70518710588,486.542822342158));
#114990=CARTESIAN_POINT('Ctrl Pts',(62.9141008093992,1076.70512360841,486.266464209322));
#114991=CARTESIAN_POINT('Ctrl Pts',(63.0786857269495,1076.70441004859,486.157159896911));
#114992=CARTESIAN_POINT('Ctrl Pts',(63.4402417057163,1076.70155480918,486.009231475747));
#114993=CARTESIAN_POINT('Ctrl Pts',(63.633551754434,1076.69943928384,485.971827051054));
#114994=CARTESIAN_POINT('Ctrl Pts',(64.0237269139951,1076.69372595064,485.974195249882));
#114995=CARTESIAN_POINT('Ctrl Pts',(64.2167544746152,1076.69017424572,486.014028607335));
#114996=CARTESIAN_POINT('Ctrl Pts',(64.4846573373595,1076.68391175077,486.127578245854));
#114997=CARTESIAN_POINT('Ctrl Pts',(64.5690151412844,1076.68170928521,486.173446959145));
#114998=CARTESIAN_POINT('Ctrl Pts',(64.8105570368171,1076.67463682357,486.336978368092));
#114999=CARTESIAN_POINT('Ctrl Pts',(64.9493321941796,1076.66944502775,486.477958746744));
#115000=CARTESIAN_POINT('Ctrl Pts',(65.1628585102578,1076.65885899044,486.804291013134));
#115001=CARTESIAN_POINT('Ctrl Pts',(65.2361140013734,1076.65357364652,486.986063387697));
#115002=CARTESIAN_POINT('Ctrl Pts',(65.3082193662151,1076.64382909709,487.367639770847));
#115003=CARTESIAN_POINT('Ctrl Pts',(65.3063239173843,1076.63947208179,487.563750204927));
#115004=CARTESIAN_POINT('Ctrl Pts',(65.2268400786758,1076.63262870979,487.943828373376));
#115005=CARTESIAN_POINT('Ctrl Pts',(65.150105079873,1076.6302132747,488.12411224945));
#115006=CARTESIAN_POINT('Ctrl Pts',(64.9316461160177,1076.62789251368,488.444316314171));
#115007=CARTESIAN_POINT('Ctrl Pts',(64.7922171890342,1076.6280053344,488.581233911691));
#115008=CARTESIAN_POINT('Ctrl Pts',(64.4689266284222,1076.63074726386,488.793293728351));
#115009=CARTESIAN_POINT('Ctrl Pts',(64.2882973189173,1076.633340972,488.86653745439));
#115010=CARTESIAN_POINT('Ctrl Pts',(64.0067526630902,1076.63861956661,488.920677163634));
#115011=CARTESIAN_POINT('Ctrl Pts',(63.9133200171384,1076.64055634134,488.929582004412));
#115012=CARTESIAN_POINT('Ctrl Pts',(63.8196790295888,1076.64266067219,488.929589533317));
#115013=CARTESIAN_POINT('Origin',(63.8195601713296,1067.7251047501,487.451286405902));
#115014=CARTESIAN_POINT('',(63.8195601713296,1076.65571487055,488.329589538096));
#115015=CARTESIAN_POINT('',(63.819560171333,1076.68781395203,486.572983273709));
#115016=CARTESIAN_POINT('Ctrl Pts',(63.8195601713296,1076.65571487055,488.329589538096));
#115017=CARTESIAN_POINT('Ctrl Pts',(63.7107697804043,1076.65798824794,488.329589538096));
#115018=CARTESIAN_POINT('Ctrl Pts',(63.6028716162922,1076.66061090128,488.309375843125));
#115019=CARTESIAN_POINT('Ctrl Pts',(63.39429164515,1076.66634768013,488.228309470195));
#115020=CARTESIAN_POINT('Ctrl Pts',(63.2963987561866,1076.66942216486,488.166073090089));
#115021=CARTESIAN_POINT('Ctrl Pts',(63.1300943178984,1076.6754291516,488.007405178066));
#115022=CARTESIAN_POINT('Ctrl Pts',(63.063300272878,1076.67830344724,487.912485291315));
#115023=CARTESIAN_POINT('Ctrl Pts',(62.9694049578448,1076.68354215884,487.700790544189));
#115024=CARTESIAN_POINT('Ctrl Pts',(62.9438210601612,1076.68584838576,487.58582423722));
#115025=CARTESIAN_POINT('Ctrl Pts',(62.9390622631114,1076.68964004189,487.352764181843));
#115026=CARTESIAN_POINT('Ctrl Pts',(62.9598730251725,1076.69109192874,487.23698824714));
#115027=CARTESIAN_POINT('Ctrl Pts',(63.045517073269,1076.69306253932,487.020145887916));
#115028=CARTESIAN_POINT('Ctrl Pts',(63.1095607462142,1076.69356254242,486.921261308762));
#115029=CARTESIAN_POINT('Ctrl Pts',(63.2725389825084,1076.69358373261,486.754296937428));
#115030=CARTESIAN_POINT('Ctrl Pts',(63.3698504694939,1076.69310471028,486.687881665862));
#115031=CARTESIAN_POINT('Ctrl Pts',(63.5845665079714,1076.69117522368,486.597024029905));
#115032=CARTESIAN_POINT('Ctrl Pts',(63.6998086185617,1076.6897431168,486.573423475287));
#115033=CARTESIAN_POINT('Ctrl Pts',(63.8173780549111,1076.68784921539,486.572985306547));
#115034=CARTESIAN_POINT('Ctrl Pts',(63.818469163189,1076.6878316016,486.572983273709));
#115035=CARTESIAN_POINT('Ctrl Pts',(63.8195601713365,1076.68781395203,486.572983273709));
#115036=CARTESIAN_POINT('',(63.8195601713296,1082.7251047501,486.572983273709));
#115037=CARTESIAN_POINT('',(63.8195601713296,1067.7251047501,486.572983273709));
#115038=CARTESIAN_POINT('Origin',(63.8195601713296,1082.7251047501,487.451286405902));
#115039=CARTESIAN_POINT('Ctrl Pts',(63.8195601713365,1076.68781395203,486.572983273709));
#115040=CARTESIAN_POINT('Ctrl Pts',(63.9350701010665,1076.68594531276,486.572983273709));
#115041=CARTESIAN_POINT('Ctrl Pts',(64.0494576024828,1076.68367400261,486.595770247173));
#115042=CARTESIAN_POINT('Ctrl Pts',(64.2645360000653,1076.67843271753,486.685008814363));
#115043=CARTESIAN_POINT('Ctrl Pts',(64.3628089626602,1076.67550321216,486.751241238968));
#115044=CARTESIAN_POINT('Ctrl Pts',(64.5260112993656,1076.66942713559,486.916859920746));
#115045=CARTESIAN_POINT('Ctrl Pts',(64.589937036861,1076.66634467399,487.014016877144));
#115046=CARTESIAN_POINT('Ctrl Pts',(64.6741808433638,1076.66060693963,487.221404317127));
#115047=CARTESIAN_POINT('Ctrl Pts',(64.6960422229002,1076.65798862615,487.328795694996));
#115048=CARTESIAN_POINT('Ctrl Pts',(64.6977542871803,1076.65571755183,487.437448526525));
#115049=CARTESIAN_POINT('Ctrl Pts',(64.6995701042535,1076.65330884816,487.55268582739));
#115050=CARTESIAN_POINT('Ctrl Pts',(64.6786861551085,1076.6513385752,487.667169847103));
#115051=CARTESIAN_POINT('Ctrl Pts',(64.5939433460243,1076.64861220933,487.881400968346));
#115052=CARTESIAN_POINT('Ctrl Pts',(64.5309643521006,1076.64788279605,487.979087238798));
#115053=CARTESIAN_POINT('Ctrl Pts',(64.3710574006373,1076.64781958489,488.144446523562));
#115054=CARTESIAN_POINT('Ctrl Pts',(64.2757425146998,1076.64848382618,488.210573030146));
#115055=CARTESIAN_POINT('Ctrl Pts',(64.0651859252744,1076.6510846175,488.302319929318));
#115056=CARTESIAN_POINT('Ctrl Pts',(63.9519985665621,1076.65299295402,488.327098272006));
#115057=CARTESIAN_POINT('Ctrl Pts',(63.8313589702029,1076.65546939683,488.329530126905));
#115058=CARTESIAN_POINT('Ctrl Pts',(63.8254582594845,1076.65559161903,488.329589538096));
#115059=CARTESIAN_POINT('Ctrl Pts',(63.8195601713296,1076.65571487055,488.329589538096));
#115060=CARTESIAN_POINT('Origin',(61.0059658728171,1067.7251047501,499.690312664149));
#115061=CARTESIAN_POINT('',(61.0059658728373,1078.41010379242,498.414868543013));
#115062=CARTESIAN_POINT('Ctrl Pts',(61.0060185765775,1078.28341943821,500.965756784196));
#115063=CARTESIAN_POINT('Ctrl Pts',(61.1593612507269,1078.27681519819,500.965750447787));
#115064=CARTESIAN_POINT('Ctrl Pts',(61.3115040629282,1078.27167163102,500.938090417076));
#115065=CARTESIAN_POINT('Ctrl Pts',(61.5294627507336,1078.26656240556,500.856081999369));
#115066=CARTESIAN_POINT('Ctrl Pts',(61.6010381099983,1078.26530678887,500.821223191467));
#115067=CARTESIAN_POINT('Ctrl Pts',(61.6976461112628,1078.26424350508,500.762444921767));
#115068=CARTESIAN_POINT('Ctrl Pts',(61.7256796492391,1078.26401878141,500.743831194445));
#115069=CARTESIAN_POINT('Ctrl Pts',(61.7698766977493,1078.26380403502,500.711896878635));
#115070=CARTESIAN_POINT('Ctrl Pts',(61.7865053405924,1078.26375737041,500.699248837616));
#115071=CARTESIAN_POINT('Ctrl Pts',(61.8204286188542,1078.26373448196,500.672105388278));
#115072=CARTESIAN_POINT('Ctrl Pts',(61.8376643467884,1078.26376418367,500.657547982924));
#115073=CARTESIAN_POINT('Ctrl Pts',(61.8771326449426,1078.26393115789,500.622377443948));
#115074=CARTESIAN_POINT('Ctrl Pts',(61.8990341574984,1078.26410183812,500.601413804347));
#115075=CARTESIAN_POINT('Ctrl Pts',(61.9664003251663,1078.26488344987,500.532167311465));
#115076=CARTESIAN_POINT('Ctrl Pts',(62.0088536330547,1078.265775407,500.481115101989));
#115077=CARTESIAN_POINT('Ctrl Pts',(62.1453603527211,1078.27018479766,500.288186707831));
#115078=CARTESIAN_POINT('Ctrl Pts',(62.2147960369423,1078.27558509874,500.13117825464));
#115079=CARTESIAN_POINT('Ctrl Pts',(62.2816743671612,1078.28876887451,499.828216932716));
#115080=CARTESIAN_POINT('Ctrl Pts',(62.2890924237342,1078.29588017964,499.687178604723));
#115081=CARTESIAN_POINT('Ctrl Pts',(62.256439448631,1078.31236603524,499.396730274855));
#115082=CARTESIAN_POINT('Ctrl Pts',(62.2125768553997,1078.32174728379,499.249920461796));
#115083=CARTESIAN_POINT('Ctrl Pts',(62.0702775780052,1078.34182773481,498.968781844095));
#115084=CARTESIAN_POINT('Ctrl Pts',(61.9693673546002,1078.35238842155,498.838708946376));
#115085=CARTESIAN_POINT('Ctrl Pts',(61.7200846157815,1078.37300114546,498.620202575887));
#115086=CARTESIAN_POINT('Ctrl Pts',(61.5727161461335,1078.38282688788,498.535354569588));
#115087=CARTESIAN_POINT('Ctrl Pts',(61.260545411812,1078.3998060434,498.430212896559));
#115088=CARTESIAN_POINT('Ctrl Pts',(61.0996084303574,1078.40691089988,498.408154756107));
#115089=CARTESIAN_POINT('Ctrl Pts',(60.7774262686565,1078.41819074401,498.425151614357));
#115090=CARTESIAN_POINT('Ctrl Pts',(60.6191169232872,1078.42225765181,498.46424738999));
#115091=CARTESIAN_POINT('Ctrl Pts',(60.4175197813752,1078.4254743782,498.557119647779));
#115092=CARTESIAN_POINT('Ctrl Pts',(60.3645978106156,1078.42610383578,498.586209932429));
#115093=CARTESIAN_POINT('Ctrl Pts',(60.2898897929974,1078.42666703254,498.634466124367));
#115094=CARTESIAN_POINT('Ctrl Pts',(60.2663773999814,1078.42679236439,498.65080038069));
#115095=CARTESIAN_POINT('Ctrl Pts',(60.2256701710816,1078.42691530889,498.681160831159));
#115096=CARTESIAN_POINT('Ctrl Pts',(60.2082543284669,1078.42693534288,498.694870501367));
#115097=CARTESIAN_POINT('Ctrl Pts',(60.1729246832527,1078.42690717033,498.724204699766));
#115098=CARTESIAN_POINT('Ctrl Pts',(60.1550725821967,1078.42685394242,498.739890219775));
#115099=CARTESIAN_POINT('Ctrl Pts',(60.1106336194392,1078.42661942927,498.781192129821));
#115100=CARTESIAN_POINT('Ctrl Pts',(60.0847019742475,1078.42638369646,498.80748044149));
#115101=CARTESIAN_POINT('Ctrl Pts',(59.9880828274185,1078.42510196671,498.914328021156));
#115102=CARTESIAN_POINT('Ctrl Pts',(59.9265263277214,1078.42337382139,499.00253129405));
#115103=CARTESIAN_POINT('Ctrl Pts',(59.8175027708732,1078.4179502462,499.210164535695));
#115104=CARTESIAN_POINT('Ctrl Pts',(59.7755245946314,1078.4139748903,499.331166481984));
#115105=CARTESIAN_POINT('Ctrl Pts',(59.7260759691088,1078.40357059609,499.596148970225));
#115106=CARTESIAN_POINT('Ctrl Pts',(59.7235616529909,1078.39698056187,499.739296046524));
#115107=CARTESIAN_POINT('Ctrl Pts',(59.7675829640332,1078.38138825678,500.032233432546));
#115108=CARTESIAN_POINT('Ctrl Pts',(59.8179011397374,1078.37235473804,500.179167782539));
#115109=CARTESIAN_POINT('Ctrl Pts',(59.9740981591699,1078.35249435977,500.458066544377));
#115110=CARTESIAN_POINT('Ctrl Pts',(60.0824211082803,1078.3417682257,500.585442094107));
#115111=CARTESIAN_POINT('Ctrl Pts',(60.3125864214195,1078.3230338029,500.768497513091));
#115112=CARTESIAN_POINT('Ctrl Pts',(60.4246410377411,1078.31506352744,500.832823128112));
#115113=CARTESIAN_POINT('Ctrl Pts',(60.6915600712771,1078.2984543899,500.936433156734));
#115114=CARTESIAN_POINT('Ctrl Pts',(60.8480764598553,1078.29022176935,500.965763310663));
#115115=CARTESIAN_POINT('Ctrl Pts',(61.0060185765775,1078.28341943821,500.965756784196));
#115116=CARTESIAN_POINT('',(61.0059658727952,1076.40646512577,498.414868543013));
#115117=CARTESIAN_POINT('',(61.0059658728171,1067.7251047501,498.414868543013));
#115118=CARTESIAN_POINT('Ctrl Pts',(61.0060409438501,1076.27845846789,500.965756783076));
#115119=CARTESIAN_POINT('Ctrl Pts',(60.8393532119705,1076.28571097349,500.965766594105));
#115120=CARTESIAN_POINT('Ctrl Pts',(60.6743383448293,1076.29456922384,500.933101074979));
#115121=CARTESIAN_POINT('Ctrl Pts',(60.3658759786924,1076.31431410998,500.806082350595));
#115122=CARTESIAN_POINT('Ctrl Pts',(60.2254417397641,1076.32501352991,500.712770698471));
#115123=CARTESIAN_POINT('Ctrl Pts',(60.0477651021946,1076.34127535239,500.536232428695));
#115124=CARTESIAN_POINT('Ctrl Pts',(59.9944560145889,1076.34669397231,500.471707366279));
#115125=CARTESIAN_POINT('Ctrl Pts',(59.8533562014058,1076.3628483696,500.262049498931));
#115126=CARTESIAN_POINT('Ctrl Pts',(59.7877280301588,1076.37316917685,500.104218976959));
#115127=CARTESIAN_POINT('Ctrl Pts',(59.7220854218885,1076.39168201607,499.772829033881));
#115128=CARTESIAN_POINT('Ctrl Pts',(59.7224140897275,1076.39970620851,499.602593824359));
#115129=CARTESIAN_POINT('Ctrl Pts',(59.789407417764,1076.41262948071,499.27159316087));
#115130=CARTESIAN_POINT('Ctrl Pts',(59.8555699434147,1076.41739720942,499.114151420653));
#115131=CARTESIAN_POINT('Ctrl Pts',(60.0458503641121,1076.42316730663,498.833723887449));
#115132=CARTESIAN_POINT('Ctrl Pts',(60.1682419741281,1076.42410175589,498.713690040939));
#115133=CARTESIAN_POINT('Ctrl Pts',(60.4526371074538,1076.42199349074,498.528710937925));
#115134=CARTESIAN_POINT('Ctrl Pts',(60.611715179383,1076.41897648336,498.46555300937));
#115135=CARTESIAN_POINT('Ctrl Pts',(60.9445258790086,1076.40925873538,498.405216296368));
#115136=CARTESIAN_POINT('Ctrl Pts',(61.1148816736779,1076.40266455816,498.408382360996));
#115137=CARTESIAN_POINT('Ctrl Pts',(61.4445191497671,1076.3865296403,498.480795906462));
#115138=CARTESIAN_POINT('Ctrl Pts',(61.6005313489561,1076.37714081322,498.54938606952));
#115139=CARTESIAN_POINT('Ctrl Pts',(61.8063860563556,1076.36186638373,498.693850425921));
#115140=CARTESIAN_POINT('Ctrl Pts',(61.8693451359274,1076.35666909398,498.747878073002));
#115141=CARTESIAN_POINT('Ctrl Pts',(61.9850024580324,1076.34597130689,498.868508828113));
#115142=CARTESIAN_POINT('Ctrl Pts',(62.0371982269214,1076.340492805,498.935042374393));
#115143=CARTESIAN_POINT('Ctrl Pts',(62.1723241765287,1076.32413980981,499.147679462465));
#115144=CARTESIAN_POINT('Ctrl Pts',(62.2334714492597,1076.31342738866,499.305484806729));
#115145=CARTESIAN_POINT('Ctrl Pts',(62.2911976389649,1076.29370015856,499.635615898861));
#115146=CARTESIAN_POINT('Ctrl Pts',(62.2872777130916,1076.28487779503,499.804751501161));
#115147=CARTESIAN_POINT('Ctrl Pts',(62.2142893581537,1076.27054739291,500.13152385481));
#115148=CARTESIAN_POINT('Ctrl Pts',(62.1460960247155,1076.26517470197,500.286010253355));
#115149=CARTESIAN_POINT('Ctrl Pts',(61.9541860296279,1076.25879133627,500.559478245958));
#115150=CARTESIAN_POINT('Ctrl Pts',(61.8325311071289,1076.2578313534,500.675892842116));
#115151=CARTESIAN_POINT('Ctrl Pts',(61.5515524611975,1076.26050472866,500.855134842823));
#115152=CARTESIAN_POINT('Ctrl Pts',(61.3950511192112,1076.26410238746,500.916306047607));
#115153=CARTESIAN_POINT('Ctrl Pts',(61.1569191730779,1076.27223850714,500.95904288288));
#115154=CARTESIAN_POINT('Ctrl Pts',(61.0815476100229,1076.275173208,500.965752338849));
#115155=CARTESIAN_POINT('Ctrl Pts',(61.0060409438501,1076.27845846789,500.965756783076));
#115156=CARTESIAN_POINT('Origin',(61.0059658728171,1067.7251047501,499.690312664149));
#115157=CARTESIAN_POINT('',(61.0059658728171,1076.31052966192,500.365756785285));
#115158=CARTESIAN_POINT('',(61.005965872817,1076.37831455598,499.014868543013));
#115159=CARTESIAN_POINT('Ctrl Pts',(61.0059658728171,1076.31052966192,500.365756785285));
#115160=CARTESIAN_POINT('Ctrl Pts',(60.9602270007978,1076.31246147104,500.365756785285));
#115161=CARTESIAN_POINT('Ctrl Pts',(60.9145063088114,1076.314628575,500.361110802308));
#115162=CARTESIAN_POINT('Ctrl Pts',(60.782887332266,1076.32155472217,500.333962078073));
#115163=CARTESIAN_POINT('Ctrl Pts',(60.7006346737792,1076.32676762466,500.299255965846));
#115164=CARTESIAN_POINT('Ctrl Pts',(60.5907950691867,1076.33508722384,500.22492833398));
#115165=CARTESIAN_POINT('Ctrl Pts',(60.5566920535575,1076.33792506562,500.196606332976));
#115166=CARTESIAN_POINT('Ctrl Pts',(60.4945641776638,1076.34363858974,500.133756645256));
#115167=CARTESIAN_POINT('Ctrl Pts',(60.4666770488451,1076.3465006828,500.099387198059));
#115168=CARTESIAN_POINT('Ctrl Pts',(60.3928025512871,1076.35508766922,499.987528047546));
#115169=CARTESIAN_POINT('Ctrl Pts',(60.3587199228918,1076.36062081203,499.903354392186));
#115170=CARTESIAN_POINT('Ctrl Pts',(60.3255613131223,1076.37060790071,499.726756820627));
#115171=CARTESIAN_POINT('Ctrl Pts',(60.3267372252089,1076.37496650124,499.636099560964));
#115172=CARTESIAN_POINT('Ctrl Pts',(60.364532008823,1076.38197773769,499.460361040129));
#115173=CARTESIAN_POINT('Ctrl Pts',(60.4008255387522,1076.38455869322,499.377055787549));
#115174=CARTESIAN_POINT('Ctrl Pts',(60.5040542188223,1076.38761361433,499.229402268924));
#115175=CARTESIAN_POINT('Ctrl Pts',(60.5699940769635,1076.38805350169,499.166591258357));
#115176=CARTESIAN_POINT('Ctrl Pts',(60.7225779565673,1076.38671338192,499.070609103443));
#115177=CARTESIAN_POINT('Ctrl Pts',(60.8076510813114,1076.38494860617,499.038388159638));
#115178=CARTESIAN_POINT('Ctrl Pts',(60.9327006851329,1076.38104556125,499.017853175409));
#115179=CARTESIAN_POINT('Ctrl Pts',(60.9693057062944,1076.37975511911,499.014868543013));
#115180=CARTESIAN_POINT('Ctrl Pts',(61.0059658728168,1076.37831455598,499.014868543013));
#115181=CARTESIAN_POINT('',(61.0059658728171,1082.7251047501,499.014868543013));
#115182=CARTESIAN_POINT('',(61.0059658728171,1067.7251047501,499.014868543013));
#115183=CARTESIAN_POINT('Origin',(61.0059658728171,1082.7251047501,499.690312664149));
#115184=CARTESIAN_POINT('Ctrl Pts',(61.0059658728168,1076.37831455598,499.014868543013));
#115185=CARTESIAN_POINT('Ctrl Pts',(61.006088218702,1076.37830974839,499.014868543013));
#115186=CARTESIAN_POINT('Ctrl Pts',(61.0062105652016,1076.37830493914,499.014868576095));
#115187=CARTESIAN_POINT('Ctrl Pts',(61.0063329123016,1076.3783001282,499.014868642579));
#115188=CARTESIAN_POINT('Ctrl Pts',(61.0961419167745,1076.37476865911,499.014917445233));
#115189=CARTESIAN_POINT('Ctrl Pts',(61.1850092423183,1076.3703858054,499.032876840093));
#115190=CARTESIAN_POINT('Ctrl Pts',(61.3506539455567,1076.36036131963,499.102515794653));
#115191=CARTESIAN_POINT('Ctrl Pts',(61.4257566948979,1076.35481535028,499.15357903573));
#115192=CARTESIAN_POINT('Ctrl Pts',(61.5194648340624,1076.34622638151,499.249308564313));
#115193=CARTESIAN_POINT('Ctrl Pts',(61.5471291275999,1076.3433698427,499.283731790389));
#115194=CARTESIAN_POINT('Ctrl Pts',(61.6202954907906,1076.33473058531,499.395601181472));
#115195=CARTESIAN_POINT('Ctrl Pts',(61.6539441512043,1076.32905986884,499.479632579587));
#115196=CARTESIAN_POINT('Ctrl Pts',(61.6862786245079,1076.31871981181,499.654937752871));
#115197=CARTESIAN_POINT('Ctrl Pts',(61.6850535659793,1076.3141402482,499.744430501955));
#115198=CARTESIAN_POINT('Ctrl Pts',(61.6481138312494,1076.30669523748,499.917682732522));
#115199=CARTESIAN_POINT('Ctrl Pts',(61.6128399843051,1076.3038992998,499.999772676156));
#115200=CARTESIAN_POINT('Ctrl Pts',(61.512718568371,1076.30052576457,500.145531948238));
#115201=CARTESIAN_POINT('Ctrl Pts',(61.4489237809329,1076.29997641375,500.20781971664));
#115202=CARTESIAN_POINT('Ctrl Pts',(61.3010433856369,1076.30122143156,500.304266069869));
#115203=CARTESIAN_POINT('Ctrl Pts',(61.2184267132202,1076.30300096174,500.33750867518));
#115204=CARTESIAN_POINT('Ctrl Pts',(61.0901970097171,1076.30717218938,500.361819299098));
#115205=CARTESIAN_POINT('Ctrl Pts',(61.0480737369782,1076.30875121064,500.365756785285));
#115206=CARTESIAN_POINT('Ctrl Pts',(61.0059658728171,1076.31052966192,500.365756785285));
#115207=CARTESIAN_POINT('Origin',(56.6885840720975,1067.7251047501,512.850041810019));
#115208=CARTESIAN_POINT('',(56.6885840720974,1077.75968243012,511.751210674027));
#115209=CARTESIAN_POINT('Ctrl Pts',(56.6886081290873,1077.56894204485,513.948872945749));
#115210=CARTESIAN_POINT('Ctrl Pts',(56.8261231132141,1077.56103093171,513.948869935098));
#115211=CARTESIAN_POINT('Ctrl Pts',(56.9625179305558,1077.55546951976,513.923052854808));
#115212=CARTESIAN_POINT('Ctrl Pts',(57.1274950322521,1077.55176837792,513.858184947821));
#115213=CARTESIAN_POINT('Ctrl Pts',(57.1635121568085,1077.55116671106,513.841726874955));
#115214=CARTESIAN_POINT('Ctrl Pts',(57.2187463512769,1077.55057719113,513.812786266466));
#115215=CARTESIAN_POINT('Ctrl Pts',(57.2385936460081,1077.55043736053,513.801587100646));
#115216=CARTESIAN_POINT('Ctrl Pts',(57.274530730328,1077.55031926557,513.779808688972));
#115217=CARTESIAN_POINT('Ctrl Pts',(57.2907180079139,1077.55031925992,513.769408253724));
#115218=CARTESIAN_POINT('Ctrl Pts',(57.3254383039349,1077.55043724832,513.745789730864));
#115219=CARTESIAN_POINT('Ctrl Pts',(57.3438502323476,1077.55057679087,513.732410137908));
#115220=CARTESIAN_POINT('Ctrl Pts',(57.3938577369024,1077.55117441997,513.693641767044));
#115221=CARTESIAN_POINT('Ctrl Pts',(57.4244816451797,1077.55179569627,513.667064454835));
#115222=CARTESIAN_POINT('Ctrl Pts',(57.5580686446764,1077.55572960633,513.537514192885));
#115223=CARTESIAN_POINT('Ctrl Pts',(57.6413148447348,1077.56180565762,513.416489384173));
#115224=CARTESIAN_POINT('Ctrl Pts',(57.7450816461198,1077.57750896273,513.17436109799));
#115225=CARTESIAN_POINT('Ctrl Pts',(57.7737566562579,1077.58614944444,513.05914475885));
#115226=CARTESIAN_POINT('Ctrl Pts',(57.7943342947576,1077.60680865319,512.813268635681));
#115227=CARTESIAN_POINT('Ctrl Pts',(57.7824020047724,1077.61890753672,512.684053791606));
#115228=CARTESIAN_POINT('Ctrl Pts',(57.7118340754916,1077.64552211447,512.426249200563));
#115229=CARTESIAN_POINT('Ctrl Pts',(57.6502812306567,1077.65992011515,512.300707521847));
#115230=CARTESIAN_POINT('Ctrl Pts',(57.4794488624528,1077.68910225513,512.07336758671));
#115231=CARTESIAN_POINT('Ctrl Pts',(57.3694753385046,1077.7035880436,511.975327672765));
#115232=CARTESIAN_POINT('Ctrl Pts',(57.1215812723172,1077.72954363832,511.830291800281));
#115233=CARTESIAN_POINT('Ctrl Pts',(56.9869522514092,1077.74086067208,511.783071169242));
#115234=CARTESIAN_POINT('Ctrl Pts',(56.7198346616448,1077.7586006036,511.744170714597));
#115235=CARTESIAN_POINT('Ctrl Pts',(56.5903714491967,1077.76524234396,511.748075249157));
#115236=CARTESIAN_POINT('Ctrl Pts',(56.3865624964544,1077.7726436181,511.790541123025));
#115237=CARTESIAN_POINT('Ctrl Pts',(56.3106526789005,1077.77465788857,511.815182822459));
#115238=CARTESIAN_POINT('Ctrl Pts',(56.2097457973579,1077.77628301304,511.860543376455));
#115239=CARTESIAN_POINT('Ctrl Pts',(56.1819869597731,1077.77660963499,511.87446363521));
#115240=CARTESIAN_POINT('Ctrl Pts',(56.1369670513964,1077.77693574781,511.89948026704));
#115241=CARTESIAN_POINT('Ctrl Pts',(56.1193613932389,1077.77700871986,511.909917274788));
#115242=CARTESIAN_POINT('Ctrl Pts',(56.0856188660735,1077.77704051168,511.931216084456));
#115243=CARTESIAN_POINT('Ctrl Pts',(56.0694587463262,1077.7770048533,511.942026624961));
#115244=CARTESIAN_POINT('Ctrl Pts',(56.0323237123983,1077.77680174403,511.968321068902));
#115245=CARTESIAN_POINT('Ctrl Pts',(56.0115965806802,1077.77659359619,511.984133625794));
#115246=CARTESIAN_POINT('Ctrl Pts',(55.9476059417592,1077.77564186145,512.03665456934));
#115247=CARTESIAN_POINT('Ctrl Pts',(55.9066186050281,1077.7745579944,512.075977497988));
#115248=CARTESIAN_POINT('Ctrl Pts',(55.7718916726251,1077.76918120536,512.226900584202));
#115249=CARTESIAN_POINT('Ctrl Pts',(55.6975541818714,1077.76257849438,512.353628038415));
#115250=CARTESIAN_POINT('Ctrl Pts',(55.6104694429214,1077.74608656393,512.605545779289));
#115251=CARTESIAN_POINT('Ctrl Pts',(55.5901279684423,1077.7370413497,512.725719525586));
#115252=CARTESIAN_POINT('Ctrl Pts',(55.5893552004997,1077.71560635979,512.978428314551));
#115253=CARTESIAN_POINT('Ctrl Pts',(55.6126484753009,1077.70316050526,513.109084826551));
#115254=CARTESIAN_POINT('Ctrl Pts',(55.707782491818,1077.67583170941,513.36537363583));
#115255=CARTESIAN_POINT('Ctrl Pts',(55.7823949292631,1077.66108130366,513.487498046795));
#115256=CARTESIAN_POINT('Ctrl Pts',(55.967260464845,1077.63306249184,513.689412387421));
#115257=CARTESIAN_POINT('Ctrl Pts',(56.0732526704201,1077.61998236202,513.769963117753));
#115258=CARTESIAN_POINT('Ctrl Pts',(56.2594534447348,1077.60103419945,513.86451717195));
#115259=CARTESIAN_POINT('Ctrl Pts',(56.3313290710501,1077.5944937807,513.892008434028));
#115260=CARTESIAN_POINT('Ctrl Pts',(56.497805996776,1077.5810230906,513.936391378811));
#115261=CARTESIAN_POINT('Ctrl Pts',(56.59296919302,1077.57444406668,513.948875039596));
#115262=CARTESIAN_POINT('Ctrl Pts',(56.6886081290873,1077.56894204485,513.948872945749));
#115263=CARTESIAN_POINT('',(56.6885840720726,1075.74962658425,511.751210674027));
#115264=CARTESIAN_POINT('',(56.6885840720975,1067.7251047501,511.751210674027));
#115265=CARTESIAN_POINT('Ctrl Pts',(56.688665939873,1075.55713627063,513.948872942962));
#115266=CARTESIAN_POINT('Ctrl Pts',(56.545178338593,1075.56546486824,513.948883633423));
#115267=CARTESIAN_POINT('Ctrl Pts',(56.4032254515711,1075.57621265454,513.920792057026));
#115268=CARTESIAN_POINT('Ctrl Pts',(56.137487060598,1075.60126725074,513.81154703054));
#115269=CARTESIAN_POINT('Ctrl Pts',(56.0163641408127,1075.61535423461,513.731100016272));
#115270=CARTESIAN_POINT('Ctrl Pts',(55.863120128512,1075.63749302432,513.578898554677));
#115271=CARTESIAN_POINT('Ctrl Pts',(55.8171142560329,1075.64499509613,513.523214503998));
#115272=CARTESIAN_POINT('Ctrl Pts',(55.7368450001395,1075.65997707953,513.403909826976));
#115273=CARTESIAN_POINT('Ctrl Pts',(55.7027169832874,1075.66742250756,513.340598178089));
#115274=CARTESIAN_POINT('Ctrl Pts',(55.6187164697901,1075.68957947368,513.139965011894));
#115275=CARTESIAN_POINT('Ctrl Pts',(55.5896951964811,1075.70365286938,512.995563315431));
#115276=CARTESIAN_POINT('Ctrl Pts',(55.5898106614579,1075.72864668678,512.704120985872));
#115277=CARTESIAN_POINT('Ctrl Pts',(55.618761220439,1075.73933512329,512.559942790098));
#115278=CARTESIAN_POINT('Ctrl Pts',(55.7314955667793,1075.75601604001,512.290817644665));
#115279=CARTESIAN_POINT('Ctrl Pts',(55.814231570036,1075.76183417675,512.168634566489));
#115280=CARTESIAN_POINT('Ctrl Pts',(56.0206828343934,1075.76774660283,511.965823938307));
#115281=CARTESIAN_POINT('Ctrl Pts',(56.1414700414339,1075.7678990289,511.886402274529));
#115282=CARTESIAN_POINT('Ctrl Pts',(56.4070000636937,1075.76263714728,511.778250402562));
#115283=CARTESIAN_POINT('Ctrl Pts',(56.5491486730179,1075.75726195637,511.750709334383));
#115284=CARTESIAN_POINT('Ctrl Pts',(56.8382667326121,1075.74143131156,511.751734533559));
#115285=CARTESIAN_POINT('Ctrl Pts',(56.9823492838177,1075.73104815858,511.781255765029));
#115286=CARTESIAN_POINT('Ctrl Pts',(57.25077628193,1075.70654473072,511.894709152754));
#115287=CARTESIAN_POINT('Ctrl Pts',(57.372416941745,1075.69265311821,511.977671978499));
#115288=CARTESIAN_POINT('Ctrl Pts',(57.5769230252388,1075.6630478409,512.186834707922));
#115289=CARTESIAN_POINT('Ctrl Pts',(57.6574878086284,1075.64760781311,512.31133209373));
#115290=CARTESIAN_POINT('Ctrl Pts',(57.7646463823465,1075.61747936737,512.583870217935));
#115291=CARTESIAN_POINT('Ctrl Pts',(57.7904938275083,1075.60307749624,512.729172590082));
#115292=CARTESIAN_POINT('Ctrl Pts',(57.7837973641008,1075.57748263647,513.019629825418));
#115293=CARTESIAN_POINT('Ctrl Pts',(57.7520835582338,1075.56649753112,513.161980597539));
#115294=CARTESIAN_POINT('Ctrl Pts',(57.6355578208295,1075.54944468611,513.425637637228));
#115295=CARTESIAN_POINT('Ctrl Pts',(57.5522289267554,1075.54351604955,513.544482780541));
#115296=CARTESIAN_POINT('Ctrl Pts',(57.3448504471021,1075.53759642069,513.742922434999));
#115297=CARTESIAN_POINT('Ctrl Pts',(57.2230770502388,1075.53763572485,513.820731366586));
#115298=CARTESIAN_POINT('Ctrl Pts',(56.9619228712105,1075.54357025731,513.923162562141));
#115299=CARTESIAN_POINT('Ctrl Pts',(56.825850053433,1075.5491735528,513.948862722139));
#115300=CARTESIAN_POINT('Ctrl Pts',(56.688665939873,1075.55713627063,513.948872942962));
#115301=CARTESIAN_POINT('Origin',(56.6885840720975,1067.7251047501,512.850041810019));
#115302=CARTESIAN_POINT('',(56.6885840720975,1075.61138997104,513.348872946012));
#115303=CARTESIAN_POINT('',(56.6885840720978,1075.69877322724,512.351210674027));
#115304=CARTESIAN_POINT('Ctrl Pts',(56.6885840720976,1075.61138997104,513.348872946012));
#115305=CARTESIAN_POINT('Ctrl Pts',(56.6856353917996,1075.61155830615,513.348872946012));
#115306=CARTESIAN_POINT('Ctrl Pts',(56.6826856497571,1075.61172901146,513.348846800787));
#115307=CARTESIAN_POINT('Ctrl Pts',(56.6145283054266,1075.6157267927,513.347637551156));
#115308=CARTESIAN_POINT('Ctrl Pts',(56.550247139395,1075.6206265607,513.333706769179));
#115309=CARTESIAN_POINT('Ctrl Pts',(56.4304095372942,1075.63202017548,513.28185968679));
#115310=CARTESIAN_POINT('Ctrl Pts',(56.3760567804463,1075.63841378756,513.244295287237));
#115311=CARTESIAN_POINT('Ctrl Pts',(56.2841232541272,1075.65193539467,513.149517112086));
#115312=CARTESIAN_POINT('Ctrl Pts',(56.247773763792,1075.65894372933,513.092860533435));
#115313=CARTESIAN_POINT('Ctrl Pts',(56.1995769763763,1075.67247229934,512.968843972007));
#115314=CARTESIAN_POINT('Ctrl Pts',(56.1881045044952,1075.67886399388,512.902720402242));
#115315=CARTESIAN_POINT('Ctrl Pts',(56.1917799382474,1075.69018089434,512.769881583919));
#115316=CARTESIAN_POINT('Ctrl Pts',(56.2068480293014,1075.69499713634,512.704481362263));
#115317=CARTESIAN_POINT('Ctrl Pts',(56.2615232716968,1075.70236414649,512.583997057215));
#115318=CARTESIAN_POINT('Ctrl Pts',(56.3003133012152,1075.70486596451,512.530013671785));
#115319=CARTESIAN_POINT('Ctrl Pts',(56.3960612796101,1075.70725109424,512.440788863679));
#115320=CARTESIAN_POINT('Ctrl Pts',(56.4518198103308,1075.70714518084,512.406195279986));
#115321=CARTESIAN_POINT('Ctrl Pts',(56.5688319756226,1075.70446970291,512.362088715319));
#115322=CARTESIAN_POINT('Ctrl Pts',(56.6283527037088,1075.70211063064,512.351241331275));
#115323=CARTESIAN_POINT('Ctrl Pts',(56.6883296349369,1075.69878733113,512.351210739033));
#115324=CARTESIAN_POINT('Ctrl Pts',(56.6884144485161,1075.69878263164,512.351210695772));
#115325=CARTESIAN_POINT('Ctrl Pts',(56.6884992609062,1075.69877793035,512.351210674027));
#115326=CARTESIAN_POINT('Ctrl Pts',(56.688584072098,1075.69877322724,512.351210674027));
#115327=CARTESIAN_POINT('',(56.6885840720975,1082.7251047501,512.351210674027));
#115328=CARTESIAN_POINT('',(56.6885840720975,1067.7251047501,512.351210674027));
#115329=CARTESIAN_POINT('Origin',(56.6885840720975,1082.7251047501,512.850041810019));
#115330=CARTESIAN_POINT('Ctrl Pts',(56.688584072098,1075.69877322724,512.351210674027));
#115331=CARTESIAN_POINT('Ctrl Pts',(56.7550184269763,1075.69508918153,512.351210674027));
#115332=CARTESIAN_POINT('Ctrl Pts',(56.8207179252903,1075.69029351969,512.364480756885));
#115333=CARTESIAN_POINT('Ctrl Pts',(56.9431511449826,1075.67900838172,512.41593311774));
#115334=CARTESIAN_POINT('Ctrl Pts',(56.9986424001624,1075.6726255336,512.453676334347));
#115335=CARTESIAN_POINT('Ctrl Pts',(57.0917047797326,1075.65910658288,512.548764302263));
#115336=CARTESIAN_POINT('Ctrl Pts',(57.1283045669644,1075.65209891217,512.605257041306));
#115337=CARTESIAN_POINT('Ctrl Pts',(57.1772166247705,1075.63842106371,512.729462828353));
#115338=CARTESIAN_POINT('Ctrl Pts',(57.188976740676,1075.63188566127,512.795998323866));
#115339=CARTESIAN_POINT('Ctrl Pts',(57.1855601054695,1075.62037662518,512.928332734584));
#115340=CARTESIAN_POINT('Ctrl Pts',(57.17101361606,1075.61548204284,512.992847771813));
#115341=CARTESIAN_POINT('Ctrl Pts',(57.1178833131381,1075.60790188226,513.112304719604));
#115342=CARTESIAN_POINT('Ctrl Pts',(57.0799660849343,1075.60527804921,513.166130164001));
#115343=CARTESIAN_POINT('Ctrl Pts',(56.9856739717083,1075.60267072458,513.255989818789));
#115344=CARTESIAN_POINT('Ctrl Pts',(56.9303155975767,1075.60270252346,513.291201547692));
#115345=CARTESIAN_POINT('Ctrl Pts',(56.8119498459242,1075.6053660802,513.337344559212));
#115346=CARTESIAN_POINT('Ctrl Pts',(56.750501019099,1075.60785523846,513.348872946012));
#115347=CARTESIAN_POINT('Ctrl Pts',(56.6885840720976,1075.61138997104,513.348872946012));
#115348=CARTESIAN_POINT('Origin',(49.7050859019682,1067.7251047501,524.96881684456));
#115349=CARTESIAN_POINT('',(49.7050859019681,1076.94955520377,523.878276095832));
#115350=CARTESIAN_POINT('Ctrl Pts',(49.7051010956667,1076.68713161255,526.059357593183));
#115351=CARTESIAN_POINT('Ctrl Pts',(49.8088196058972,1076.68081788784,526.059356148149));
#115352=CARTESIAN_POINT('Ctrl Pts',(49.9120885769206,1076.67634163785,526.044558198505));
#115353=CARTESIAN_POINT('Ctrl Pts',(50.0459481856418,1076.67300727781,526.005330350595));
#115354=CARTESIAN_POINT('Ctrl Pts',(50.0796158220323,1076.67239233822,525.993646226015));
#115355=CARTESIAN_POINT('Ctrl Pts',(50.132975025126,1076.67178502937,525.972146286058));
#115356=CARTESIAN_POINT('Ctrl Pts',(50.1530443720276,1076.67164427072,525.963348054894));
#115357=CARTESIAN_POINT('Ctrl Pts',(50.1906690054537,1076.67154917841,525.945483576024));
#115358=CARTESIAN_POINT('Ctrl Pts',(50.2082691325682,1076.6715777997,525.936533477392));
#115359=CARTESIAN_POINT('Ctrl Pts',(50.2475560463489,1076.67180942963,525.915193424795));
#115360=CARTESIAN_POINT('Ctrl Pts',(50.2690788279477,1076.67205652408,525.902526837374));
#115361=CARTESIAN_POINT('Ctrl Pts',(50.3317132132919,1076.67313964998,525.862709087758));
#115362=CARTESIAN_POINT('Ctrl Pts',(50.3714324424752,1076.67431347612,525.83350483112));
#115363=CARTESIAN_POINT('Ctrl Pts',(50.5193153002078,1076.68068267819,525.708518676353));
#115364=CARTESIAN_POINT('Ctrl Pts',(50.6098380401068,1076.68920035861,525.594469904896));
#115365=CARTESIAN_POINT('Ctrl Pts',(50.7297357974363,1076.71059995738,525.360591608081));
#115366=CARTESIAN_POINT('Ctrl Pts',(50.7662173654937,1076.72230872815,525.246873664953));
#115367=CARTESIAN_POINT('Ctrl Pts',(50.8027980978875,1076.75001560668,525.001616850204));
#115368=CARTESIAN_POINT('Ctrl Pts',(50.7989167301965,1076.76609517129,524.871305558032));
#115369=CARTESIAN_POINT('Ctrl Pts',(50.7437473135572,1076.80123160075,524.608400609267));
#115370=CARTESIAN_POINT('Ctrl Pts',(50.6892153615724,1076.82011769004,524.47871760199));
#115371=CARTESIAN_POINT('Ctrl Pts',(50.5313246102264,1076.85783773953,524.242481790271));
#115372=CARTESIAN_POINT('Ctrl Pts',(50.4276399916915,1076.87628991027,524.139216212707));
#115373=CARTESIAN_POINT('Ctrl Pts',(50.1911042395142,1076.90880615558,523.982787576683));
#115374=CARTESIAN_POINT('Ctrl Pts',(50.0618738851153,1076.92274392356,523.928965892714));
#115375=CARTESIAN_POINT('Ctrl Pts',(49.7950978369668,1076.94484043791,523.873833716397));
#115376=CARTESIAN_POINT('Ctrl Pts',(49.6603852961936,1076.95301660898,523.871010226687));
#115377=CARTESIAN_POINT('Ctrl Pts',(49.4669169638779,1076.96054213026,523.9027808114));
#115378=CARTESIAN_POINT('Ctrl Pts',(49.4064240516526,1076.96225868753,523.91812041938));
#115379=CARTESIAN_POINT('Ctrl Pts',(49.3242060255788,1076.96368973258,523.946652212118));
#115380=CARTESIAN_POINT('Ctrl Pts',(49.3011368386674,1076.96398683188,523.955547236706));
#115381=CARTESIAN_POINT('Ctrl Pts',(49.2615022695362,1076.9643131366,523.972398566672));
#115382=CARTESIAN_POINT('Ctrl Pts',(49.2447994750683,1076.96439158913,523.980003289559));
#115383=CARTESIAN_POINT('Ctrl Pts',(49.2104144860873,1076.96442869639,523.996718783239));
#115384=CARTESIAN_POINT('Ctrl Pts',(49.192773902446,1076.96437678838,524.005898961466));
#115385=CARTESIAN_POINT('Ctrl Pts',(49.1519569226844,1076.96408778106,524.028579440257));
#115386=CARTESIAN_POINT('Ctrl Pts',(49.1290090154073,1076.9637925443,524.042461993219));
#115387=CARTESIAN_POINT('Ctrl Pts',(49.057371330461,1076.96243744104,524.089491811313));
#115388=CARTESIAN_POINT('Ctrl Pts',(49.0108570925859,1076.96088780839,524.125733641707));
#115389=CARTESIAN_POINT('Ctrl Pts',(48.8612232473619,1076.95345476994,524.263129374957));
#115390=CARTESIAN_POINT('Ctrl Pts',(48.7755058867875,1076.94462518507,524.380708499751));
#115391=CARTESIAN_POINT('Ctrl Pts',(48.6645189513374,1076.92276844206,524.620881359219));
#115392=CARTESIAN_POINT('Ctrl Pts',(48.6325026062703,1076.91080305764,524.737897999566));
#115393=CARTESIAN_POINT('Ctrl Pts',(48.6068359257461,1076.8825797593,524.98826281284));
#115394=CARTESIAN_POINT('Ctrl Pts',(48.6171692821046,1076.8662535282,525.120123908447));
#115395=CARTESIAN_POINT('Ctrl Pts',(48.6866792696424,1076.83056210063,525.383751228586));
#115396=CARTESIAN_POINT('Ctrl Pts',(48.7490851406893,1076.81137652074,525.51230254272));
#115397=CARTESIAN_POINT('Ctrl Pts',(48.9188277218414,1076.7739993112,525.737448347857));
#115398=CARTESIAN_POINT('Ctrl Pts',(49.0243149715656,1076.75612946937,525.832315979849));
#115399=CARTESIAN_POINT('Ctrl Pts',(49.2171396635911,1076.73042006772,525.947716364382));
#115400=CARTESIAN_POINT('Ctrl Pts',(49.2940365919188,1076.72152431293,525.982425429634));
#115401=CARTESIAN_POINT('Ctrl Pts',(49.4810873207852,1076.70289412714,526.041979076823));
#115402=CARTESIAN_POINT('Ctrl Pts',(49.592681813386,1076.69397498504,526.059359159437));
#115403=CARTESIAN_POINT('Ctrl Pts',(49.7051010956667,1076.68713161255,526.059357593183));
#115404=CARTESIAN_POINT('',(49.7050859019402,1074.93236944137,523.878276095832));
#115405=CARTESIAN_POINT('',(49.7050859019682,1067.7251047501,523.878276095832));
#115406=CARTESIAN_POINT('Ctrl Pts',(49.7045327815809,1074.66780810413,526.059357453018));
#115407=CARTESIAN_POINT('Ctrl Pts',(49.5625720018367,1074.67652953238,526.059285450746));
#115408=CARTESIAN_POINT('Ctrl Pts',(49.4222337317669,1074.6885690479,526.03149985231));
#115409=CARTESIAN_POINT('Ctrl Pts',(49.1590551093703,1074.7179348791,525.923575693812));
#115410=CARTESIAN_POINT('Ctrl Pts',(49.0389404221457,1074.73502905751,525.843944797542));
#115411=CARTESIAN_POINT('Ctrl Pts',(48.8866461967813,1074.76269718284,525.693103719675));
#115412=CARTESIAN_POINT('Ctrl Pts',(48.8407632584335,1074.77223284,525.637677149076));
#115413=CARTESIAN_POINT('Ctrl Pts',(48.7606636865352,1074.7915328718,525.518791458315));
#115414=CARTESIAN_POINT('Ctrl Pts',(48.7266027627846,1074.80125310818,525.455618460512));
#115415=CARTESIAN_POINT('Ctrl Pts',(48.6429153207276,1074.8305179077,525.255502964398));
#115416=CARTESIAN_POINT('Ctrl Pts',(48.6141566330179,1074.84959607476,525.11145403381));
#115417=CARTESIAN_POINT('Ctrl Pts',(48.6149386387002,1074.88435927607,524.821397837244));
#115418=CARTESIAN_POINT('Ctrl Pts',(48.6440366075017,1074.89973770998,524.678190775981));
#115419=CARTESIAN_POINT('Ctrl Pts',(48.7566128360411,1074.92484835885,524.411541627296));
#115420=CARTESIAN_POINT('Ctrl Pts',(48.838790490427,1074.93434730158,524.290726991862));
#115421=CARTESIAN_POINT('Ctrl Pts',(49.0447128969339,1074.94613771329,524.08921518635));
#115422=CARTESIAN_POINT('Ctrl Pts',(49.1658542694596,1074.9483909307,524.010144969033));
#115423=CARTESIAN_POINT('Ctrl Pts',(49.4304649275366,1074.94544904026,523.903936701423));
#115424=CARTESIAN_POINT('Ctrl Pts',(49.570991037753,1074.94036278595,523.877332045742));
#115425=CARTESIAN_POINT('Ctrl Pts',(49.857416713149,1074.92329557957,523.879293889884));
#115426=CARTESIAN_POINT('Ctrl Pts',(50.0003887150679,1074.9113327437,523.909133788143));
#115427=CARTESIAN_POINT('Ctrl Pts',(50.2666680223075,1074.88201441875,524.022791742783));
#115428=CARTESIAN_POINT('Ctrl Pts',(50.3872229444195,1074.86492275914,524.105737641097));
#115429=CARTESIAN_POINT('Ctrl Pts',(50.5374275697886,1074.83730943705,524.260624802096));
#115430=CARTESIAN_POINT('Ctrl Pts',(50.5817735933465,1074.82793436821,524.316329727833));
#115431=CARTESIAN_POINT('Ctrl Pts',(50.6591441952577,1074.80884541381,524.435772126998));
#115432=CARTESIAN_POINT('Ctrl Pts',(50.6919459063807,1074.7991730995,524.499274702747));
#115433=CARTESIAN_POINT('Ctrl Pts',(50.7725931602685,1074.76968516607,524.70188856101));
#115434=CARTESIAN_POINT('Ctrl Pts',(50.7988337714617,1074.7502503453,524.847940784062));
#115435=CARTESIAN_POINT('Ctrl Pts',(50.7918754877078,1074.71502421092,525.13852279965));
#115436=CARTESIAN_POINT('Ctrl Pts',(50.7600934763545,1074.6994930169,525.280276126511));
#115437=CARTESIAN_POINT('Ctrl Pts',(50.6435681777698,1074.67425178988,525.542296465004));
#115438=CARTESIAN_POINT('Ctrl Pts',(50.5605041258705,1074.66473437469,525.660196468658));
#115439=CARTESIAN_POINT('Ctrl Pts',(50.3541867038513,1074.65305420016,525.856532132437));
#115440=CARTESIAN_POINT('Ctrl Pts',(50.233396864555,1074.6509444254,525.93333098338));
#115441=CARTESIAN_POINT('Ctrl Pts',(49.9746818113774,1074.65433161193,526.034203506374));
#115442=CARTESIAN_POINT('Ctrl Pts',(49.8401329657222,1074.6594774421,526.059426229206));
#115443=CARTESIAN_POINT('Ctrl Pts',(49.7045327815809,1074.66780810413,526.059357453018));
#115444=CARTESIAN_POINT('Origin',(49.7050859019682,1067.7251047501,524.96881684456));
#115445=CARTESIAN_POINT('',(49.7050859019682,1074.74227702453,525.459357593288));
#115446=CARTESIAN_POINT('',(49.7050859019685,1074.86129916363,524.478276095832));
#115447=CARTESIAN_POINT('Ctrl Pts',(49.7050859019682,1074.74227702453,525.459357593288));
#115448=CARTESIAN_POINT('Ctrl Pts',(49.7042385243676,1074.74232843758,525.459357593288));
#115449=CARTESIAN_POINT('Ctrl Pts',(49.7033910526429,1074.74238012467,525.459355397603));
#115450=CARTESIAN_POINT('Ctrl Pts',(49.6386219609656,1074.74635089057,525.459019703593));
#115451=CARTESIAN_POINT('Ctrl Pts',(49.5754894174681,1074.75174807733,525.446200007164));
#115452=CARTESIAN_POINT('Ctrl Pts',(49.4572417247623,1074.76491503881,525.397005248761));
#115453=CARTESIAN_POINT('Ctrl Pts',(49.403354017794,1074.77258043984,525.360871069239));
#115454=CARTESIAN_POINT('Ctrl Pts',(49.3352444927388,1074.78498960951,525.292676140412));
#115455=CARTESIAN_POINT('Ctrl Pts',(49.3147929353546,1074.78925799106,525.267710480105));
#115456=CARTESIAN_POINT('Ctrl Pts',(49.279098864582,1074.79791017122,525.214173023116));
#115457=CARTESIAN_POINT('Ctrl Pts',(49.2639332817146,1074.80227438928,525.18572430995));
#115458=CARTESIAN_POINT('Ctrl Pts',(49.2266561959728,1074.81545990107,525.095424886765));
#115459=CARTESIAN_POINT('Ctrl Pts',(49.2140178972823,1074.82408227959,525.03039670124));
#115460=CARTESIAN_POINT('Ctrl Pts',(49.2151031724537,1074.83982449383,524.899459650653));
#115461=CARTESIAN_POINT('Ctrl Pts',(49.2286758037565,1074.84680058392,524.834821027198));
#115462=CARTESIAN_POINT('Ctrl Pts',(49.2801672148551,1074.85810553264,524.715348895732));
#115463=CARTESIAN_POINT('Ctrl Pts',(49.3172319860543,1074.86235798359,524.661579615519));
#115464=CARTESIAN_POINT('Ctrl Pts',(49.4095276776769,1074.86760490442,524.572157907458));
#115465=CARTESIAN_POINT('Ctrl Pts',(49.4635318492254,1074.86859727634,524.537133276184));
#115466=CARTESIAN_POINT('Ctrl Pts',(49.5807062159694,1074.86726255741,524.490217355236));
#115467=CARTESIAN_POINT('Ctrl Pts',(49.6425127344436,1074.86501864792,524.478307291072));
#115468=CARTESIAN_POINT('Ctrl Pts',(49.7048408686823,1074.86131373627,524.478276157118));
#115469=CARTESIAN_POINT('Ctrl Pts',(49.7049225476157,1074.86130888111,524.478276116317));
#115470=CARTESIAN_POINT('Ctrl Pts',(49.7050042253808,1074.86130402357,524.478276095832));
#115471=CARTESIAN_POINT('Ctrl Pts',(49.7050859019687,1074.86129916363,524.478276095832));
#115472=CARTESIAN_POINT('',(49.7050859019682,1082.7251047501,524.478276095832));
#115473=CARTESIAN_POINT('',(49.7050859019682,1067.7251047501,524.478276095832));
#115474=CARTESIAN_POINT('Origin',(49.7050859019682,1082.7251047501,524.96881684456));
#115475=CARTESIAN_POINT('Ctrl Pts',(49.7050859019687,1074.86129916363,524.478276095832));
#115476=CARTESIAN_POINT('Ctrl Pts',(49.7690222839905,1074.85749480846,524.478276095832));
#115477=CARTESIAN_POINT('Ctrl Pts',(49.8322378137251,1074.8522284988,524.490773982374));
#115478=CARTESIAN_POINT('Ctrl Pts',(49.9518571609206,1074.83918388506,524.539828474315));
#115479=CARTESIAN_POINT('Ctrl Pts',(50.0068143051841,1074.83146919783,524.576564320064));
#115480=CARTESIAN_POINT('Ctrl Pts',(50.0755035950335,1074.81900529293,524.645632418096));
#115481=CARTESIAN_POINT('Ctrl Pts',(50.0958136304354,1074.8147772041,524.670508815552));
#115482=CARTESIAN_POINT('Ctrl Pts',(50.1313241442475,1074.80617701668,524.723905292744));
#115483=CARTESIAN_POINT('Ctrl Pts',(50.1464325591112,1074.80182393296,524.752313818214));
#115484=CARTESIAN_POINT('Ctrl Pts',(50.1837270944111,1074.78858807754,524.842856832629));
#115485=CARTESIAN_POINT('Ctrl Pts',(50.1963126327165,1074.7798774798,524.908201722288));
#115486=CARTESIAN_POINT('Ctrl Pts',(50.1948930021439,1074.76399887641,525.039146675381));
#115487=CARTESIAN_POINT('Ctrl Pts',(50.1812690455078,1074.75696291534,525.103481856568));
#115488=CARTESIAN_POINT('Ctrl Pts',(50.129968273002,1074.74554619808,525.222227936558));
#115489=CARTESIAN_POINT('Ctrl Pts',(50.093202375989,1074.74123492869,525.275625525989));
#115490=CARTESIAN_POINT('Ctrl Pts',(50.0013970852732,1074.73586449067,525.364916401852));
#115491=CARTESIAN_POINT('Ctrl Pts',(49.9474434653618,1074.73483245957,525.400052791796));
#115492=CARTESIAN_POINT('Ctrl Pts',(49.8299711124248,1074.73616947686,525.447336148879));
#115493=CARTESIAN_POINT('Ctrl Pts',(49.7677861562045,1074.73847280419,525.459357593288));
#115494=CARTESIAN_POINT('Ctrl Pts',(49.7050859019682,1074.74227702453,525.459357593288));
#115495=CARTESIAN_POINT('Origin',(75.4882582191912,1067.7251047501,472.809444687437));
#115496=CARTESIAN_POINT('',(75.4882582192226,1078.69210669589,471.331141555243));
#115497=CARTESIAN_POINT('Ctrl Pts',(75.4883591791963,1078.65110304669,474.287747816183));
#115498=CARTESIAN_POINT('Ctrl Pts',(75.6738846076919,1078.64642022966,474.287735145812));
#115499=CARTESIAN_POINT('Ctrl Pts',(75.8577731642089,1078.64215344441,474.25279772366));
#115500=CARTESIAN_POINT('Ctrl Pts',(76.2028476993047,1078.63519237295,474.116771245797));
#115501=CARTESIAN_POINT('Ctrl Pts',(76.3609960447903,1078.63256354019,474.016954115307));
#115502=CARTESIAN_POINT('Ctrl Pts',(76.5486284066885,1078.63044231687,473.84194790386));
#115503=CARTESIAN_POINT('Ctrl Pts',(76.5971122148997,1078.63001746006,473.789695126768));
#115504=CARTESIAN_POINT('Ctrl Pts',(76.6599317411793,1078.62965774124,473.711340567205));
#115505=CARTESIAN_POINT('Ctrl Pts',(76.6775400349786,1078.62958172096,473.687991095779));
#115506=CARTESIAN_POINT('Ctrl Pts',(76.7085227237751,1078.62949534906,473.644266605918));
#115507=CARTESIAN_POINT('Ctrl Pts',(76.7221080656931,1078.62947615609,473.624053584186));
#115508=CARTESIAN_POINT('Ctrl Pts',(76.7485175895551,1078.62947796131,473.582582632352));
#115509=CARTESIAN_POINT('Ctrl Pts',(76.7613180723559,1078.62949973388,473.56131872677));
#115510=CARTESIAN_POINT('Ctrl Pts',(76.7912100487528,1078.62960359524,473.508709076028));
#115511=CARTESIAN_POINT('Ctrl Pts',(76.8077130885578,1078.62970791169,473.47704710312));
#115512=CARTESIAN_POINT('Ctrl Pts',(76.8612782639026,1078.6302211234,473.364517282206));
#115513=CARTESIAN_POINT('Ctrl Pts',(76.8921774655035,1078.63085155159,473.2809314245));
#115514=CARTESIAN_POINT('Ctrl Pts',(76.9476616566716,1078.63295707426,473.075600852574));
#115515=CARTESIAN_POINT('Ctrl Pts',(76.9648138863255,1078.63465835563,472.952545948046));
#115516=CARTESIAN_POINT('Ctrl Pts',(76.9684843419805,1078.63942569333,472.672302980661));
#115517=CARTESIAN_POINT('Ctrl Pts',(76.945666676569,1078.64270286122,472.516474557731));
#115518=CARTESIAN_POINT('Ctrl Pts',(76.8476704098332,1078.65041112291,472.203941880989));
#115519=CARTESIAN_POINT('Ctrl Pts',(76.7685599201206,1078.65485959935,472.050855059878));
#115520=CARTESIAN_POINT('Ctrl Pts',(76.5539017011356,1078.66433878016,471.768528614668));
#115521=CARTESIAN_POINT('Ctrl Pts',(76.4164840386204,1078.66930162597,471.644326190103));
#115522=CARTESIAN_POINT('Ctrl Pts',(76.0912980893407,1078.67907857565,471.445345791837));
#115523=CARTESIAN_POINT('Ctrl Pts',(75.9037669536843,1078.68375251818,471.377039649236));
#115524=CARTESIAN_POINT('Ctrl Pts',(75.5189195473925,1078.6917736033,471.319095987988));
#115525=CARTESIAN_POINT('Ctrl Pts',(75.3257234847783,1078.69508675301,471.327665340448));
#115526=CARTESIAN_POINT('Ctrl Pts',(74.9743722653524,1078.70008698208,471.412953117287));
#115527=CARTESIAN_POINT('Ctrl Pts',(74.8173451207834,1078.70188330224,471.481232786763));
#115528=CARTESIAN_POINT('Ctrl Pts',(74.5666181739271,1078.70413599813,471.646296258331));
#115529=CARTESIAN_POINT('Ctrl Pts',(74.4677945957722,1078.70479808836,471.731952485555));
#115530=CARTESIAN_POINT('Ctrl Pts',(74.3528508500848,1078.70527814465,471.861766235987));
#115531=CARTESIAN_POINT('Ctrl Pts',(74.3256580871193,1078.70536409373,471.89533020559));
#115532=CARTESIAN_POINT('Ctrl Pts',(74.2843529187854,1078.70544864801,471.951143061264));
#115533=CARTESIAN_POINT('Ctrl Pts',(74.2692975379912,1078.70546825953,471.972662450159));
#115534=CARTESIAN_POINT('Ctrl Pts',(74.2418698223851,1078.70548202789,472.014178476528));
#115535=CARTESIAN_POINT('Ctrl Pts',(74.2293856857682,1078.70547863999,472.034091653993));
#115536=CARTESIAN_POINT('Ctrl Pts',(74.2022918730305,1078.70544866441,472.079689031923));
#115537=CARTESIAN_POINT('Ctrl Pts',(74.1879667654673,1078.70541634643,472.105530705662));
#115538=CARTESIAN_POINT('Ctrl Pts',(74.147897836739,1078.70527436976,472.183215423094));
#115539=CARTESIAN_POINT('Ctrl Pts',(74.1244130703106,1078.70512045451,472.236159924138));
#115540=CARTESIAN_POINT('Ctrl Pts',(74.0347841579004,1078.70417420876,472.475152694407));
#115541=CARTESIAN_POINT('Ctrl Pts',(74.0031867137151,1078.70275493028,472.671979498503));
#115542=CARTESIAN_POINT('Ctrl Pts',(74.0176317392622,1078.69883959814,473.029132484725));
#115543=CARTESIAN_POINT('Ctrl Pts',(74.0500373477484,1078.69661836051,473.186965030117));
#115544=CARTESIAN_POINT('Ctrl Pts',(74.1693318751837,1078.69096939555,473.499570856544));
#115545=CARTESIAN_POINT('Ctrl Pts',(74.2599415360653,1078.68749082197,473.650320590085));
#115546=CARTESIAN_POINT('Ctrl Pts',(74.4981372593134,1078.67929894864,473.923108964409));
#115547=CARTESIAN_POINT('Ctrl Pts',(74.6473337685029,1078.67458300061,474.039659012687));
#115548=CARTESIAN_POINT('Ctrl Pts',(74.9138363613299,1078.66667163302,474.176163692336));
#115549=CARTESIAN_POINT('Ctrl Pts',(75.0188120815975,1078.66365965535,474.215681286133));
#115550=CARTESIAN_POINT('Ctrl Pts',(75.2453036469157,1078.65739862494,474.272721080618));
#115551=CARTESIAN_POINT('Ctrl Pts',(75.3665981398743,1078.65417639719,474.287756131795));
#115552=CARTESIAN_POINT('Ctrl Pts',(75.4883591791963,1078.65110304669,474.287747816183));
#115553=CARTESIAN_POINT('',(75.4882582191714,1076.6916225261,471.331141555244));
#115554=CARTESIAN_POINT('',(75.4882582191912,1067.7251047501,471.331141555244));
#115555=CARTESIAN_POINT('Ctrl Pts',(75.487416119239,1076.65015733518,474.287747579784));
#115556=CARTESIAN_POINT('Ctrl Pts',(75.2941477495985,1076.65509390806,474.287637486456));
#115557=CARTESIAN_POINT('Ctrl Pts',(75.1027674812067,1076.66038695946,474.249627667376));
#115558=CARTESIAN_POINT('Ctrl Pts',(74.7454004369792,1076.67085061937,474.102089954927));
#115559=CARTESIAN_POINT('Ctrl Pts',(74.582864262089,1076.67591723991,473.993943445776));
#115560=CARTESIAN_POINT('Ctrl Pts',(74.3073819627376,1076.68518114485,473.719940057585));
#115561=CARTESIAN_POINT('Ctrl Pts',(74.1976138837424,1076.68928141582,473.556249372343));
#115562=CARTESIAN_POINT('Ctrl Pts',(74.048125694059,1076.69614758041,473.195944211236));
#115563=CARTESIAN_POINT('Ctrl Pts',(74.0097657378391,1076.69885579239,473.00291543298));
#115564=CARTESIAN_POINT('Ctrl Pts',(74.0101469157191,1076.70288797094,472.611989528244));
#115565=CARTESIAN_POINT('Ctrl Pts',(74.0493216181602,1076.70417222778,472.417951918973));
#115566=CARTESIAN_POINT('Ctrl Pts',(74.2013211842234,1076.70537226395,472.055889894595));
#115567=CARTESIAN_POINT('Ctrl Pts',(74.3128635434451,1076.70527492564,471.891567320269));
#115568=CARTESIAN_POINT('Ctrl Pts',(74.5931205500648,1076.7036766014,471.616773061266));
#115569=CARTESIAN_POINT('Ctrl Pts',(74.7588236214776,1076.70219294848,471.50880710114));
#115570=CARTESIAN_POINT('Ctrl Pts',(75.1217122397172,1076.6977548676,471.364112829601));
#115571=CARTESIAN_POINT('Ctrl Pts',(75.3151722554871,1076.69484316653,471.328440445533));
#115572=CARTESIAN_POINT('Ctrl Pts',(75.7053422696635,1076.68758955606,471.33416999898));
#115573=CARTESIAN_POINT('Ctrl Pts',(75.898212919866,1076.68330767376,471.37574715457));
#115574=CARTESIAN_POINT('Ctrl Pts',(76.1654707024127,1076.67615770782,471.491877270918));
#115575=CARTESIAN_POINT('Ctrl Pts',(76.2495993877647,1076.67369664673,471.538634153267));
#115576=CARTESIAN_POINT('Ctrl Pts',(76.4897797850506,1076.66599625282,471.704583745673));
#115577=CARTESIAN_POINT('Ctrl Pts',(76.6272274923538,1076.66059878149,471.846890075095));
#115578=CARTESIAN_POINT('Ctrl Pts',(76.8376279573087,1076.65019591766,472.175223471903));
#115579=CARTESIAN_POINT('Ctrl Pts',(76.9091447621676,1076.64529430033,472.357642143143));
#115580=CARTESIAN_POINT('Ctrl Pts',(76.9776049539143,1076.63692598836,472.739650764687));
#115581=CARTESIAN_POINT('Ctrl Pts',(76.9739027906418,1076.63354729511,472.935528786523));
#115582=CARTESIAN_POINT('Ctrl Pts',(76.891101144393,1076.62908213527,473.314360346499));
#115583=CARTESIAN_POINT('Ctrl Pts',(76.8129350538818,1076.62803950129,473.493655297899));
#115584=CARTESIAN_POINT('Ctrl Pts',(76.5921399911397,1076.62854799809,473.811538877061));
#115585=CARTESIAN_POINT('Ctrl Pts',(76.4517926810517,1076.63008793845,473.947136320226));
#115586=CARTESIAN_POINT('Ctrl Pts',(76.1270588505246,1076.63541758085,474.156515194196));
#115587=CARTESIAN_POINT('Ctrl Pts',(75.9458490738619,1076.63914850194,474.228339926111));
#115588=CARTESIAN_POINT('Ctrl Pts',(75.6673873722677,1076.64564977036,474.279617326469));
#115589=CARTESIAN_POINT('Ctrl Pts',(75.5774921057094,1076.64785656205,474.287798890638));
#115590=CARTESIAN_POINT('Ctrl Pts',(75.487416119239,1076.65015733518,474.287747579784));
#115591=CARTESIAN_POINT('Origin',(75.4882582191912,1067.7251047501,472.809444687437));
#115592=CARTESIAN_POINT('',(75.4882582191912,1076.65987181774,473.68774781963));
#115593=CARTESIAN_POINT('',(75.4882582191939,1076.68449717364,471.931141555244));
#115594=CARTESIAN_POINT('Ctrl Pts',(75.4882582191911,1076.65987181774,473.68774781963));
#115595=CARTESIAN_POINT('Ctrl Pts',(75.3795548737725,1076.66248986587,473.68774781963));
#115596=CARTESIAN_POINT('Ctrl Pts',(75.2717368513576,1076.66532867394,473.667566390282));
#115597=CARTESIAN_POINT('Ctrl Pts',(75.0631502138089,1076.67124953729,473.586564628072));
#115598=CARTESIAN_POINT('Ctrl Pts',(74.9651901345204,1076.67427623391,473.52431053641));
#115599=CARTESIAN_POINT('Ctrl Pts',(74.7976946551806,1076.67998948559,473.364526163751));
#115600=CARTESIAN_POINT('Ctrl Pts',(74.7302215487056,1076.68261510257,473.268113306397));
#115601=CARTESIAN_POINT('Ctrl Pts',(74.6368674030413,1076.68714518856,473.054628849557));
#115602=CARTESIAN_POINT('Ctrl Pts',(74.6118897284744,1076.68900781701,472.939686161403));
#115603=CARTESIAN_POINT('Ctrl Pts',(74.6082293322471,1076.6918454184,472.706296121146));
#115604=CARTESIAN_POINT('Ctrl Pts',(74.6297641493946,1076.69279138027,472.590172895777));
#115605=CARTESIAN_POINT('Ctrl Pts',(74.7171461708703,1076.69371340958,472.372934854634));
#115606=CARTESIAN_POINT('Ctrl Pts',(74.7822155095578,1076.6936791762,472.274039933481));
#115607=CARTESIAN_POINT('Ctrl Pts',(74.9471113267483,1076.6926208934,472.107843477452));
#115608=CARTESIAN_POINT('Ctrl Pts',(75.0451981403042,1076.69160862419,472.042124578511));
#115609=CARTESIAN_POINT('Ctrl Pts',(75.2595247999158,1076.68866381459,471.953692750837));
#115610=CARTESIAN_POINT('Ctrl Pts',(75.3733480631393,1076.68677275628,471.931141555244));
#115611=CARTESIAN_POINT('Ctrl Pts',(75.4882582191967,1076.68449717364,471.931141555244));
#115612=CARTESIAN_POINT('',(75.4882582191912,1082.7251047501,471.931141555244));
#115613=CARTESIAN_POINT('',(75.4882582191912,1067.7251047501,471.931141555244));
#115614=CARTESIAN_POINT('Origin',(75.4882582191912,1082.7251047501,472.809444687437));
#115615=CARTESIAN_POINT('Ctrl Pts',(75.4882582191967,1076.68449717364,471.931141555244));
#115616=CARTESIAN_POINT('Ctrl Pts',(75.4897687748842,1076.68446725989,471.931141555244));
#115617=CARTESIAN_POINT('Ctrl Pts',(75.4912795183942,1076.68443727978,471.931145452152));
#115618=CARTESIAN_POINT('Ctrl Pts',(75.6093545818292,1076.68208921839,471.93175475067));
#115619=CARTESIAN_POINT('Ctrl Pts',(75.7246341896332,1076.67941978365,471.955555118033));
#115620=CARTESIAN_POINT('Ctrl Pts',(75.884478497529,1076.67508939696,472.023511770839));
#115621=CARTESIAN_POINT('Ctrl Pts',(75.9347534318612,1076.67361895054,472.050944275815));
#115622=CARTESIAN_POINT('Ctrl Pts',(76.0782617178249,1076.6690746825,472.148492106724));
#115623=CARTESIAN_POINT('Ctrl Pts',(76.1605597090188,1076.6659615896,472.232406066685));
#115624=CARTESIAN_POINT('Ctrl Pts',(76.2869862583745,1076.66005651707,472.42641082651));
#115625=CARTESIAN_POINT('Ctrl Pts',(76.3302816653696,1076.65732080599,472.534342839857));
#115626=CARTESIAN_POINT('Ctrl Pts',(76.3606717240375,1076.65399831874,472.696395274421));
#115627=CARTESIAN_POINT('Ctrl Pts',(76.3656697823108,1076.65308034466,472.745924848059));
#115628=CARTESIAN_POINT('Ctrl Pts',(76.3664524173893,1076.65226038285,472.795612035064));
#115629=CARTESIAN_POINT('Ctrl Pts',(76.3682654495979,1076.6503608805,472.910716089134));
#115630=CARTESIAN_POINT('Ctrl Pts',(76.3474312203528,1076.64901622478,473.025068011928));
#115631=CARTESIAN_POINT('Ctrl Pts',(76.2628817863424,1076.64767305316,473.239092129448));
#115632=CARTESIAN_POINT('Ctrl Pts',(76.2000401080296,1076.64768681701,473.336706577559));
#115633=CARTESIAN_POINT('Ctrl Pts',(76.0403984525932,1076.64908105315,473.502087076357));
#115634=CARTESIAN_POINT('Ctrl Pts',(75.9451775833408,1076.65044569815,473.568281919729));
#115635=CARTESIAN_POINT('Ctrl Pts',(75.7346737785574,1076.65427288339,473.660261316522));
#115636=CARTESIAN_POINT('Ctrl Pts',(75.6214226622723,1076.65669614696,473.685157609897));
#115637=CARTESIAN_POINT('Ctrl Pts',(75.5004853717269,1076.65957810674,473.687684017164));
#115638=CARTESIAN_POINT('Ctrl Pts',(75.494370395865,1076.65972461001,473.68774781963));
#115639=CARTESIAN_POINT('Ctrl Pts',(75.4882582191911,1076.65987181774,473.68774781963));
#115640=CARTESIAN_POINT('Origin',(75.2807843499779,1067.7251047501,485.365998005138));
#115641=CARTESIAN_POINT('',(75.2807843500077,1078.39877300636,484.090553884001));
#115642=CARTESIAN_POINT('Ctrl Pts',(75.2809045366249,1078.29623865226,486.641442120612));
#115643=CARTESIAN_POINT('Ctrl Pts',(75.4339105238594,1078.2882023348,486.641427702672));
#115644=CARTESIAN_POINT('Ctrl Pts',(75.5857297123117,1078.28130556259,486.613880856192));
#115645=CARTESIAN_POINT('Ctrl Pts',(75.870023368324,1078.27070260712,486.507146698662));
#115646=CARTESIAN_POINT('Ctrl Pts',(76.0005273852905,1078.26703110727,486.429678545514));
#115647=CARTESIAN_POINT('Ctrl Pts',(76.1462977300508,1078.26464544065,486.303765465089));
#115648=CARTESIAN_POINT('Ctrl Pts',(76.1767035328239,1078.26426694378,486.274761038957));
#115649=CARTESIAN_POINT('Ctrl Pts',(76.222190991114,1078.26389723177,486.226863869023));
#115650=CARTESIAN_POINT('Ctrl Pts',(76.2382613847249,1078.26380971897,486.208953664539));
#115651=CARTESIAN_POINT('Ctrl Pts',(76.2669222035402,1078.2637355859,486.175133845931));
#115652=CARTESIAN_POINT('Ctrl Pts',(76.2796581257944,1078.26373526559,486.159357857223));
#115653=CARTESIAN_POINT('Ctrl Pts',(76.3066136640089,1078.26380783491,486.124289470864));
#115654=CARTESIAN_POINT('Ctrl Pts',(76.3206764811848,1078.26389403399,486.104886405074));
#115655=CARTESIAN_POINT('Ctrl Pts',(76.3582619371465,1078.26426397549,486.049828044096));
#115656=CARTESIAN_POINT('Ctrl Pts',(76.3805521187458,1078.26464929531,486.013371236718));
#115657=CARTESIAN_POINT('Ctrl Pts',(76.4819964712389,1078.26729100411,485.827041527426));
#115658=CARTESIAN_POINT('Ctrl Pts',(76.5325310650515,1078.27168449475,485.663600881729));
#115659=CARTESIAN_POINT('Ctrl Pts',(76.5634527384567,1078.28312828342,485.35973230746));
#115660=CARTESIAN_POINT('Ctrl Pts',(76.555468701051,1078.28941048786,485.223055576913));
#115661=CARTESIAN_POINT('Ctrl Pts',(76.493947627413,1078.30441416594,484.945199741084));
#115662=CARTESIAN_POINT('Ctrl Pts',(76.4367295935245,1078.31319121105,484.80688854445));
#115663=CARTESIAN_POINT('Ctrl Pts',(76.2713755449846,1078.33240508195,484.546870966901));
#115664=CARTESIAN_POINT('Ctrl Pts',(76.1611861636037,1078.34274706974,484.429446477995));
#115665=CARTESIAN_POINT('Ctrl Pts',(75.8956885425243,1078.36366888313,484.235866696622));
#115666=CARTESIAN_POINT('Ctrl Pts',(75.740707945171,1078.37402252915,484.16441542305));
#115667=CARTESIAN_POINT('Ctrl Pts',(75.416129209437,1078.39256448877,484.087115759469));
#115668=CARTESIAN_POINT('Ctrl Pts',(75.2500504972073,1078.400632639,484.080326399211));
#115669=CARTESIAN_POINT('Ctrl Pts',(74.9448587649636,1078.41307129196,484.127185420217));
#115670=CARTESIAN_POINT('Ctrl Pts',(74.8071835967028,1078.41769217654,484.173007260694));
#115671=CARTESIAN_POINT('Ctrl Pts',(74.5863103151216,1078.42343536162,484.290936006579));
#115672=CARTESIAN_POINT('Ctrl Pts',(74.4991717021453,1078.42513500507,484.352519283816));
#115673=CARTESIAN_POINT('Ctrl Pts',(74.393953385885,1078.42639080901,484.448611206889));
#115674=CARTESIAN_POINT('Ctrl Pts',(74.3682783263774,1078.42662066942,484.474145699792));
#115675=CARTESIAN_POINT('Ctrl Pts',(74.3285856906966,1078.42684757054,484.517132085187));
#115676=CARTESIAN_POINT('Ctrl Pts',(74.3138804350274,1078.42690004787,484.533920807439));
#115677=CARTESIAN_POINT('Ctrl Pts',(74.286734267309,1078.42693505528,484.566605058894));
#115678=CARTESIAN_POINT('Ctrl Pts',(74.2742153570082,1078.42692380996,484.582427006257));
#115679=CARTESIAN_POINT('Ctrl Pts',(74.2466507154517,1078.42683500459,484.619015682967));
#115680=CARTESIAN_POINT('Ctrl Pts',(74.2318454130292,1078.42674032887,484.63995251557));
#115681=CARTESIAN_POINT('Ctrl Pts',(74.1894275853905,1078.42632234144,484.703945707616));
#115682=CARTESIAN_POINT('Ctrl Pts',(74.1637638439162,1078.42586570848,484.748229684603));
#115683=CARTESIAN_POINT('Ctrl Pts',(74.0648826850275,1078.42313516236,484.945270423876));
#115684=CARTESIAN_POINT('Ctrl Pts',(74.0198471286397,1078.41913259009,485.110188562167));
#115685=CARTESIAN_POINT('Ctrl Pts',(73.9988927945721,1078.40868075659,485.416812705358));
#115686=CARTESIAN_POINT('Ctrl Pts',(74.0119178351324,1078.40288387409,485.555162740193));
#115687=CARTESIAN_POINT('Ctrl Pts',(74.0849456541348,1078.38880698269,485.834418461351));
#115688=CARTESIAN_POINT('Ctrl Pts',(74.1485603018477,1078.38045633912,485.972207522359));
#115689=CARTESIAN_POINT('Ctrl Pts',(74.3273945550068,1078.36171231311,486.228590057464));
#115690=CARTESIAN_POINT('Ctrl Pts',(74.444574647628,1078.35137807255,486.34260277014));
#115691=CARTESIAN_POINT('Ctrl Pts',(74.6771583592216,1078.33348784218,486.495571379258));
#115692=CARTESIAN_POINT('Ctrl Pts',(74.7826912782624,1078.3260535696,486.54591668702));
#115693=CARTESIAN_POINT('Ctrl Pts',(75.0187903984343,1078.31079932443,486.621140681863));
#115694=CARTESIAN_POINT('Ctrl Pts',(75.1494377303241,1078.30314366958,486.641454508888));
#115695=CARTESIAN_POINT('Ctrl Pts',(75.2809045366249,1078.29623865226,486.641442120612));
#115696=CARTESIAN_POINT('',(75.280784349959,1076.3950142966,484.090553884002));
#115697=CARTESIAN_POINT('',(75.2807843499779,1067.7251047501,484.090553884002));
#115698=CARTESIAN_POINT('Ctrl Pts',(75.2808777508431,1076.29141182132,486.641442122854));
#115699=CARTESIAN_POINT('Ctrl Pts',(75.1140408641621,1076.30026491392,486.641454340332));
#115700=CARTESIAN_POINT('Ctrl Pts',(74.9488638013435,1076.31032003874,486.60873234125));
#115701=CARTESIAN_POINT('Ctrl Pts',(74.7175248930847,1076.32622456351,486.513371472444));
#115702=CARTESIAN_POINT('Ctrl Pts',(74.6436555185119,1076.3316297301,486.474056100849));
#115703=CARTESIAN_POINT('Ctrl Pts',(74.5046433536862,1076.34247314129,486.381545150379));
#115704=CARTESIAN_POINT('Ctrl Pts',(74.4398334068195,1076.34788563694,486.32856406927));
#115705=CARTESIAN_POINT('Ctrl Pts',(74.2606645043229,1076.36400774368,486.150091497939));
#115706=CARTESIAN_POINT('Ctrl Pts',(74.1656350644278,1076.37427869745,486.007807887029));
#115707=CARTESIAN_POINT('Ctrl Pts',(74.0370711249052,1076.39263302296,485.695166642793));
#115708=CARTESIAN_POINT('Ctrl Pts',(74.0044762480409,1076.40055173042,485.528028987161));
#115709=CARTESIAN_POINT('Ctrl Pts',(74.0062403464886,1076.41322435377,485.190386718522));
#115710=CARTESIAN_POINT('Ctrl Pts',(74.0406838301846,1076.41785252816,485.023239054337));
#115711=CARTESIAN_POINT('Ctrl Pts',(74.1729601823872,1076.42333201726,484.711620713509));
#115712=CARTESIAN_POINT('Ctrl Pts',(74.2696286622621,1076.42412110499,484.570351064309));
#115713=CARTESIAN_POINT('Ctrl Pts',(74.5123785638704,1076.42173533607,484.334025774632));
#115714=CARTESIAN_POINT('Ctrl Pts',(74.655952339171,1076.41858835557,484.241286129291));
#115715=CARTESIAN_POINT('Ctrl Pts',(74.9703980447938,1076.40863309289,484.117442564739));
#115716=CARTESIAN_POINT('Ctrl Pts',(75.1380594259484,1076.40192964516,484.087397190795));
#115717=CARTESIAN_POINT('Ctrl Pts',(75.4756191035355,1076.38560017553,484.094242855806));
#115718=CARTESIAN_POINT('Ctrl Pts',(75.6421777359095,1076.3761242814,484.131219186376));
#115719=CARTESIAN_POINT('Ctrl Pts',(75.8724659623747,1076.360753094,484.233062024092));
#115720=CARTESIAN_POINT('Ctrl Pts',(75.9448308854703,1076.35552822348,484.273903400199));
#115721=CARTESIAN_POINT('Ctrl Pts',(76.0817938114949,1076.34479762919,484.369877130782));
#115722=CARTESIAN_POINT('Ctrl Pts',(76.1459002725335,1076.33931456702,484.425016201848));
#115723=CARTESIAN_POINT('Ctrl Pts',(76.3197225732954,1076.32296952879,484.60740907976));
#115724=CARTESIAN_POINT('Ctrl Pts',(76.4103329637795,1076.31229321409,484.750375695436));
#115725=CARTESIAN_POINT('Ctrl Pts',(76.531015683909,1076.29270145854,485.063100721387));
#115726=CARTESIAN_POINT('Ctrl Pts',(76.5599740863891,1076.28397745739,485.229825189004));
#115727=CARTESIAN_POINT('Ctrl Pts',(76.5517185072052,1076.26989613149,485.564613960329));
#115728=CARTESIAN_POINT('Ctrl Pts',(76.5147572621712,1076.26467144202,485.729414367033));
#115729=CARTESIAN_POINT('Ctrl Pts',(76.3794759900474,1076.25861045035,486.034912615537));
#115730=CARTESIAN_POINT('Ctrl Pts',(76.2826908660345,1076.25782084881,486.172695017995));
#115731=CARTESIAN_POINT('Ctrl Pts',(76.0418008954033,1076.26082762739,486.402974827879));
#115732=CARTESIAN_POINT('Ctrl Pts',(75.9001483641354,1076.26458439457,486.493307150367));
#115733=CARTESIAN_POINT('Ctrl Pts',(75.597171675997,1076.27580070577,486.611757669751));
#115734=CARTESIAN_POINT('Ctrl Pts',(75.4396886644151,1076.28298462186,486.64143049312));
#115735=CARTESIAN_POINT('Ctrl Pts',(75.280877750843,1076.29141182132,486.641442122854));
#115736=CARTESIAN_POINT('Origin',(75.2807843499779,1067.7251047501,485.365998005138));
#115737=CARTESIAN_POINT('',(75.2807843499779,1076.31720630032,486.041442126274));
#115738=CARTESIAN_POINT('',(75.2807843499785,1076.3720597734,484.690553884002));
#115739=CARTESIAN_POINT('Ctrl Pts',(75.2807843499779,1076.31720630032,486.041442126274));
#115740=CARTESIAN_POINT('Ctrl Pts',(75.2805672485108,1076.31721754179,486.041442126274));
#115741=CARTESIAN_POINT('Ctrl Pts',(75.2803501421419,1076.31722878769,486.041442021603));
#115742=CARTESIAN_POINT('Ctrl Pts',(75.1917003815966,1076.32182247007,486.041356538139));
#115743=CARTESIAN_POINT('Ctrl Pts',(75.1041680787943,1076.32705182337,486.02390559196));
#115744=CARTESIAN_POINT('Ctrl Pts',(74.9816429630424,1076.33538467202,485.973200491599));
#115745=CARTESIAN_POINT('Ctrl Pts',(74.9425425067788,1076.33822522788,485.952319110587));
#115746=CARTESIAN_POINT('Ctrl Pts',(74.868992635477,1076.3439444394,485.90321982519));
#115747=CARTESIAN_POINT('Ctrl Pts',(74.8347173484263,1076.3468095166,485.875118918327));
#115748=CARTESIAN_POINT('Ctrl Pts',(74.7397583913188,1076.35539801353,485.780263711893));
#115749=CARTESIAN_POINT('Ctrl Pts',(74.6894174042909,1076.36092308838,485.704551273704));
#115750=CARTESIAN_POINT('Ctrl Pts',(74.6214844176693,1076.37087259255,485.538063460784));
#115751=CARTESIAN_POINT('Ctrl Pts',(74.6044647353718,1076.37520300687,485.448984739103));
#115752=CARTESIAN_POINT('Ctrl Pts',(74.6062854402542,1076.38214292305,485.269286881598));
#115753=CARTESIAN_POINT('Ctrl Pts',(74.6251235199639,1076.38468343182,485.180471439936));
#115754=CARTESIAN_POINT('Ctrl Pts',(74.6965420898417,1076.38765532396,485.015297584075));
#115755=CARTESIAN_POINT('Ctrl Pts',(74.7484371702031,1076.38805488841,484.940630010926));
#115756=CARTESIAN_POINT('Ctrl Pts',(74.8784083840739,1076.38664140941,484.8160754338));
#115757=CARTESIAN_POINT('Ctrl Pts',(74.9551487084894,1076.3848437304,484.767436661445));
#115758=CARTESIAN_POINT('Ctrl Pts',(75.1163020148837,1076.37946891737,484.70569604598));
#115759=CARTESIAN_POINT('Ctrl Pts',(75.1982066679893,1076.37609316992,484.690553884002));
#115760=CARTESIAN_POINT('Ctrl Pts',(75.2807843499796,1076.3720597734,484.690553884002));
#115761=CARTESIAN_POINT('',(75.2807843499779,1082.7251047501,484.690553884002));
#115762=CARTESIAN_POINT('',(75.2807843499779,1067.7251047501,484.690553884002));
#115763=CARTESIAN_POINT('Origin',(75.2807843499779,1082.7251047501,485.365998005138));
#115764=CARTESIAN_POINT('Ctrl Pts',(75.280789999719,1076.37205949745,484.690553884025));
#115765=CARTESIAN_POINT('Ctrl Pts',(75.3707000073535,1076.36766793225,484.690554636076));
#115766=CARTESIAN_POINT('Ctrl Pts',(75.4596792503472,1076.36257979634,484.70850687006));
#115767=CARTESIAN_POINT('Ctrl Pts',(75.583088663004,1076.3543701819,484.760379032669));
#115768=CARTESIAN_POINT('Ctrl Pts',(75.6218987573435,1076.35158916811,484.781359211578));
#115769=CARTESIAN_POINT('Ctrl Pts',(75.6949764250228,1076.34593312118,484.830631809924));
#115770=CARTESIAN_POINT('Ctrl Pts',(75.72905860543,1076.3430712256,484.858827298119));
#115771=CARTESIAN_POINT('Ctrl Pts',(75.8232814843969,1076.33443099212,484.953744755188));
#115772=CARTESIAN_POINT('Ctrl Pts',(75.8731450516467,1076.32877074794,485.029291833927));
#115773=CARTESIAN_POINT('Ctrl Pts',(75.9400871324703,1076.31846592261,485.194532351811));
#115774=CARTESIAN_POINT('Ctrl Pts',(75.9568871292005,1076.31391088546,485.282465231146));
#115775=CARTESIAN_POINT('Ctrl Pts',(75.9555319465901,1076.3065277786,485.459647670252));
#115776=CARTESIAN_POINT('Ctrl Pts',(75.9374739089418,1076.30376858818,485.54717153329));
#115777=CARTESIAN_POINT('Ctrl Pts',(75.8686767856061,1076.30047573724,485.710100362392));
#115778=CARTESIAN_POINT('Ctrl Pts',(75.8186964139097,1076.29996918873,485.783941474256));
#115779=CARTESIAN_POINT('Ctrl Pts',(75.6932153305394,1076.30129870733,485.908131174528));
#115780=CARTESIAN_POINT('Ctrl Pts',(75.6189735970548,1076.30311868741,485.957291787176));
#115781=CARTESIAN_POINT('Ctrl Pts',(75.4559510433341,1076.30882414188,486.024250034985));
#115782=CARTESIAN_POINT('Ctrl Pts',(75.3687702480181,1076.31265041163,486.041442126274));
#115783=CARTESIAN_POINT('Ctrl Pts',(75.2807843499779,1076.31720630032,486.041442126274));
#115784=CARTESIAN_POINT('Origin',(73.793809237574,1067.7251047501,499.135789645571));
#115785=CARTESIAN_POINT('',(73.7938092375738,1077.74530255756,498.036958509579));
#115786=CARTESIAN_POINT('Ctrl Pts',(73.7933312060954,1077.58423708672,500.234620677583));
#115787=CARTESIAN_POINT('Ctrl Pts',(73.9124417122508,1077.57535459326,500.234672494987));
#115788=CARTESIAN_POINT('Ctrl Pts',(74.0308689479815,1077.56794487714,500.215357137192));
#115789=CARTESIAN_POINT('Ctrl Pts',(74.2455323814251,1077.55730469832,500.143192444516));
#115790=CARTESIAN_POINT('Ctrl Pts',(74.3416181649181,1077.55378480492,500.094351536102));
#115791=CARTESIAN_POINT('Ctrl Pts',(74.4565106494304,1077.55132489931,500.012934102364));
#115792=CARTESIAN_POINT('Ctrl Pts',(74.4829842327755,1077.55090110402,499.99229046815));
#115793=CARTESIAN_POINT('Ctrl Pts',(74.5235558786957,1077.55048740021,499.957552367046));
#115794=CARTESIAN_POINT('Ctrl Pts',(74.5382860581984,1077.55039106666,499.944231613654));
#115795=CARTESIAN_POINT('Ctrl Pts',(74.5651350992939,1077.55031863288,499.918595112909));
#115796=CARTESIAN_POINT('Ctrl Pts',(74.5773400221384,1077.55032849672,499.906378700872));
#115797=CARTESIAN_POINT('Ctrl Pts',(74.6040202414769,1077.55044811783,499.878383895092));
#115798=CARTESIAN_POINT('Ctrl Pts',(74.6183322385584,1077.5505812347,499.862460048817));
#115799=CARTESIAN_POINT('Ctrl Pts',(74.6583280431628,1077.55115878803,499.815255968473));
#115800=CARTESIAN_POINT('Ctrl Pts',(74.6827587200317,1077.55177444295,499.782964649903));
#115801=CARTESIAN_POINT('Ctrl Pts',(74.7871428356671,1077.55570285974,499.627898763944));
#115802=CARTESIAN_POINT('Ctrl Pts',(74.8437564074959,1077.56181746199,499.491359554758));
#115803=CARTESIAN_POINT('Ctrl Pts',(74.8947463817484,1077.5775952898,499.232123340022));
#115804=CARTESIAN_POINT('Ctrl Pts',(74.8987087598206,1077.58623675781,499.113576373838));
#115805=CARTESIAN_POINT('Ctrl Pts',(74.8675108231822,1077.60689745236,498.868971232424));
#115806=CARTESIAN_POINT('Ctrl Pts',(74.8288763505096,1077.6189982519,498.745127096819));
#115807=CARTESIAN_POINT('Ctrl Pts',(74.7060676945397,1077.64561593364,498.50775612588));
#115808=CARTESIAN_POINT('Ctrl Pts',(74.6196650193212,1077.66001519281,498.397824330894));
#115809=CARTESIAN_POINT('Ctrl Pts',(74.4051453040325,1077.6891943188,498.211151157411));
#115810=CARTESIAN_POINT('Ctrl Pts',(74.2771365204911,1077.70367567654,498.138227235733));
#115811=CARTESIAN_POINT('Ctrl Pts',(74.0045179663677,1077.72961144853,498.04815261718));
#115812=CARTESIAN_POINT('Ctrl Pts',(73.8630878151982,1077.74091504749,498.03006538966));
#115813=CARTESIAN_POINT('Ctrl Pts',(73.5963567766027,1077.75846984418,498.047537720141));
#115814=CARTESIAN_POINT('Ctrl Pts',(73.4729816321844,1077.76500965731,498.07730234913));
#115815=CARTESIAN_POINT('Ctrl Pts',(73.2807891581509,1077.77257860996,498.160501310288));
#115816=CARTESIAN_POINT('Ctrl Pts',(73.2082936732639,1077.77469880566,498.202218013958));
#115817=CARTESIAN_POINT('Ctrl Pts',(73.1171600973508,1077.77631811587,498.269493681862));
#115818=CARTESIAN_POINT('Ctrl Pts',(73.0938526270263,1077.77662537978,498.288214489695));
#115819=CARTESIAN_POINT('Ctrl Pts',(73.0570919810898,1077.77693018569,498.320292888793));
#115820=CARTESIAN_POINT('Ctrl Pts',(73.0431705850289,1077.77699998709,498.333088641093));
#115821=CARTESIAN_POINT('Ctrl Pts',(73.0170663092033,1077.77704117233,498.358355477605));
#115822=CARTESIAN_POINT('Ctrl Pts',(73.0048365180837,1077.77701983419,498.3707697071));
#115823=CARTESIAN_POINT('Ctrl Pts',(72.9774240097596,1077.7768764149,498.399952407309));
#115824=CARTESIAN_POINT('Ctrl Pts',(72.9624537206654,1077.77672625258,498.41690909654));
#115825=CARTESIAN_POINT('Ctrl Pts',(72.9181924867336,1077.77605439487,498.470276373843));
#115826=CARTESIAN_POINT('Ctrl Pts',(72.8906941389063,1077.77530802723,498.50809954657));
#115827=CARTESIAN_POINT('Ctrl Pts',(72.7876611654125,1077.77103914359,498.670665207963));
#115828=CARTESIAN_POINT('Ctrl Pts',(72.7349598832007,1077.76503245415,498.807987674773));
#115829=CARTESIAN_POINT('Ctrl Pts',(72.6905343401532,1077.74961802217,499.069095452969));
#115830=CARTESIAN_POINT('Ctrl Pts',(72.689826709024,1077.74112156295,499.189088494081));
#115831=CARTESIAN_POINT('Ctrl Pts',(72.7286200299827,1077.72071914054,499.43538852032));
#115832=CARTESIAN_POINT('Ctrl Pts',(72.7715699371,1077.70872794931,499.559305581308));
#115833=CARTESIAN_POINT('Ctrl Pts',(72.9036580323554,1077.68212244327,499.795134127343));
#115834=CARTESIAN_POINT('Ctrl Pts',(72.9949874731787,1077.66761150533,499.903233977721));
#115835=CARTESIAN_POINT('Ctrl Pts',(73.1930481878229,1077.64141292084,500.062914038606));
#115836=CARTESIAN_POINT('Ctrl Pts',(73.2926259662991,1077.62985494095,500.12032369341));
#115837=CARTESIAN_POINT('Ctrl Pts',(73.5249304671283,1077.60607303618,500.209686272067));
#115838=CARTESIAN_POINT('Ctrl Pts',(73.6584913990223,1077.59429257002,500.234562017361));
#115839=CARTESIAN_POINT('Ctrl Pts',(73.7933312060954,1077.58423708672,500.234620677583));
#115840=CARTESIAN_POINT('',(73.7938092375516,1075.73511330977,498.036958509579));
#115841=CARTESIAN_POINT('',(73.793809237574,1067.7251047501,498.036958509579));
#115842=CARTESIAN_POINT('Ctrl Pts',(73.7943431628175,1075.57249684997,500.234620651846));
#115843=CARTESIAN_POINT('Ctrl Pts',(73.6506175246825,1075.58330219327,500.23469048856));
#115844=CARTESIAN_POINT('Ctrl Pts',(73.5084060437648,1075.59608072594,500.206563734191));
#115845=CARTESIAN_POINT('Ctrl Pts',(73.2422667990826,1075.62408715031,500.097069246554));
#115846=CARTESIAN_POINT('Ctrl Pts',(73.120965264772,1075.63906256478,500.016420972424));
#115847=CARTESIAN_POINT('Ctrl Pts',(72.9676850470399,1075.66158528276,499.863893253268));
#115848=CARTESIAN_POINT('Ctrl Pts',(72.9217478532435,1075.6690461048,499.808194085901));
#115849=CARTESIAN_POINT('Ctrl Pts',(72.8001152687884,1075.69119911753,499.627072426163));
#115850=CARTESIAN_POINT('Ctrl Pts',(72.7435967681914,1075.70521824599,499.490618477095));
#115851=CARTESIAN_POINT('Ctrl Pts',(72.6874998082093,1075.72998009466,499.204202457804));
#115852=CARTESIAN_POINT('Ctrl Pts',(72.6881438427515,1075.74050139934,499.05713036763));
#115853=CARTESIAN_POINT('Ctrl Pts',(72.7468740496821,1075.75677397741,498.77169592508));
#115854=CARTESIAN_POINT('Ctrl Pts',(72.8043087950933,1075.76236876971,498.636207548035));
#115855=CARTESIAN_POINT('Ctrl Pts',(72.9688874035406,1075.76790839337,498.395375264388));
#115856=CARTESIAN_POINT('Ctrl Pts',(73.0743576562249,1075.76779510899,498.292523538431));
#115857=CARTESIAN_POINT('Ctrl Pts',(73.3192403672629,1075.76181406095,498.134053144044));
#115858=CARTESIAN_POINT('Ctrl Pts',(73.4561199949375,1075.75600891844,498.08004344579));
#115859=CARTESIAN_POINT('Ctrl Pts',(73.7429349984395,1075.7393569208,498.028496799552));
#115860=CARTESIAN_POINT('Ctrl Pts',(73.8899851476081,1075.72866956609,498.031546297141));
#115861=CARTESIAN_POINT('Ctrl Pts',(74.174944804702,1075.70364040769,498.094830441354));
#115862=CARTESIAN_POINT('Ctrl Pts',(74.3099702953708,1075.68952223951,498.154781690339));
#115863=CARTESIAN_POINT('Ctrl Pts',(74.4878092140052,1075.66731262955,498.280834008654));
#115864=CARTESIAN_POINT('Ctrl Pts',(74.5421696666241,1075.65986224754,498.327990547762));
#115865=CARTESIAN_POINT('Ctrl Pts',(74.6920987469502,1075.63714734461,498.486260647984));
#115866=CARTESIAN_POINT('Ctrl Pts',(74.7705033963861,1075.62200641361,498.61146960579));
#115867=CARTESIAN_POINT('Ctrl Pts',(74.8730752789762,1075.59392129564,498.883739892678));
#115868=CARTESIAN_POINT('Ctrl Pts',(74.8968920458942,1075.58122242146,499.027943543766));
#115869=CARTESIAN_POINT('Ctrl Pts',(74.8871731536858,1075.56000737385,499.316724330229));
#115870=CARTESIAN_POINT('Ctrl Pts',(74.8540577792207,1075.55167687336,499.458485925363));
#115871=CARTESIAN_POINT('Ctrl Pts',(74.7351518794729,1075.54063425143,499.720481415376));
#115872=CARTESIAN_POINT('Ctrl Pts',(74.6508834236155,1075.5379977505,499.838244773477));
#115873=CARTESIAN_POINT('Ctrl Pts',(74.4421058838755,1075.53880709932,500.034452359883));
#115874=CARTESIAN_POINT('Ctrl Pts',(74.3198178645823,1075.54222455647,500.111064665783));
#115875=CARTESIAN_POINT('Ctrl Pts',(74.061089762638,1075.55425587424,500.210023985928));
#115876=CARTESIAN_POINT('Ctrl Pts',(73.9282217980015,1075.56243180778,500.23455559982));
#115877=CARTESIAN_POINT('Ctrl Pts',(73.7943431628175,1075.57249684997,500.234620651846));
#115878=CARTESIAN_POINT('Origin',(73.793809237574,1067.7251047501,499.135789645571));
#115879=CARTESIAN_POINT('',(73.793809237574,1075.61827177418,499.634620781564));
#115880=CARTESIAN_POINT('',(73.7938092375747,1075.69207332612,498.636958509579));
#115881=CARTESIAN_POINT('Ctrl Pts',(73.7938092375739,1075.61827177418,499.634620781564));
#115882=CARTESIAN_POINT('Ctrl Pts',(73.7913850280998,1075.61845153324,499.634620781564));
#115883=CARTESIAN_POINT('Ctrl Pts',(73.7889601060211,1075.61863265287,499.634603109896));
#115884=CARTESIAN_POINT('Ctrl Pts',(73.721225695092,1075.62372835527,499.633615217395));
#115885=CARTESIAN_POINT('Ctrl Pts',(73.6567987396114,1075.62952376564,499.619846996068));
#115886=CARTESIAN_POINT('Ctrl Pts',(73.5366576718624,1075.64222522068,499.568229107957));
#115887=CARTESIAN_POINT('Ctrl Pts',(73.4821309605372,1075.64901660974,499.530734949376));
#115888=CARTESIAN_POINT('Ctrl Pts',(73.3898621684334,1075.66278401858,499.43597876458));
#115889=CARTESIAN_POINT('Ctrl Pts',(73.3533473110501,1075.66962750127,499.379280500382));
#115890=CARTESIAN_POINT('Ctrl Pts',(73.3049263756146,1075.68227121177,499.255132621402));
#115891=CARTESIAN_POINT('Ctrl Pts',(73.2933698982706,1075.6879534161,499.188952422037));
#115892=CARTESIAN_POINT('Ctrl Pts',(73.2969399182935,1075.69740214851,499.056065581121));
#115893=CARTESIAN_POINT('Ctrl Pts',(73.3119394658212,1075.70108093001,498.990695929044));
#115894=CARTESIAN_POINT('Ctrl Pts',(73.366709024541,1075.70594176922,498.869661300972));
#115895=CARTESIAN_POINT('Ctrl Pts',(73.4058829075062,1075.70707737461,498.815231302157));
#115896=CARTESIAN_POINT('Ctrl Pts',(73.502255851258,1075.70663762081,498.725841807686));
#115897=CARTESIAN_POINT('Ctrl Pts',(73.5580969989074,1075.70512317638,498.69138749117));
#115898=CARTESIAN_POINT('Ctrl Pts',(73.6749146300443,1075.69988437989,498.647662390977));
#115899=CARTESIAN_POINT('Ctrl Pts',(73.7341467464272,1075.69639019611,498.636958509579));
#115900=CARTESIAN_POINT('Ctrl Pts',(73.7938092375755,1075.69207332612,498.636958509579));
#115901=CARTESIAN_POINT('',(73.793809237574,1082.7251047501,498.636958509579));
#115902=CARTESIAN_POINT('',(73.793809237574,1067.7251047501,498.636958509579));
#115903=CARTESIAN_POINT('Origin',(73.793809237574,1082.7251047501,499.135789645571));
#115904=CARTESIAN_POINT('Ctrl Pts',(73.7938092375755,1075.69207332612,498.636958509579));
#115905=CARTESIAN_POINT('Ctrl Pts',(73.7938800001328,1075.6920682061,498.636958509579));
#115906=CARTESIAN_POINT('Ctrl Pts',(73.7939507632939,1075.69206308491,498.636958524932));
#115907=CARTESIAN_POINT('Ctrl Pts',(73.7940215270573,1075.69205796258,498.636958555047));
#115908=CARTESIAN_POINT('Ctrl Pts',(73.8606121962174,1075.68723770921,498.636986894369));
#115909=CARTESIAN_POINT('Ctrl Pts',(73.9264607334969,1075.68148464659,498.650347571099));
#115910=CARTESIAN_POINT('Ctrl Pts',(74.0492569028667,1075.66874103527,498.70215111076));
#115911=CARTESIAN_POINT('Ctrl Pts',(74.1049458244209,1075.66186959979,498.74021065917));
#115912=CARTESIAN_POINT('Ctrl Pts',(74.1981819534008,1075.64794210248,498.836115794799));
#115913=CARTESIAN_POINT('Ctrl Pts',(74.2347495868739,1075.64102167646,498.893096125891));
#115914=CARTESIAN_POINT('Ctrl Pts',(74.282658541406,1075.62827460122,499.016788074975));
#115915=CARTESIAN_POINT('Ctrl Pts',(74.2940762066304,1075.62254889527,499.082087367716));
#115916=CARTESIAN_POINT('Ctrl Pts',(74.2909250966268,1075.6129706565,499.21310637812));
#115917=CARTESIAN_POINT('Ctrl Pts',(74.2765328430183,1075.60920138255,499.277548944007));
#115918=CARTESIAN_POINT('Ctrl Pts',(74.2237659659103,1075.604155167,499.3969506414));
#115919=CARTESIAN_POINT('Ctrl Pts',(74.1860540023914,1075.60291434053,499.450778478515));
#115920=CARTESIAN_POINT('Ctrl Pts',(74.0921557874047,1075.60313681649,499.540810307316));
#115921=CARTESIAN_POINT('Ctrl Pts',(74.0369543903032,1075.6045910064,499.576159751426));
#115922=CARTESIAN_POINT('Ctrl Pts',(73.9182848271023,1075.60991048372,499.622883923426));
#115923=CARTESIAN_POINT('Ctrl Pts',(73.8562836600276,1075.61363919447,499.634620781564));
#115924=CARTESIAN_POINT('Ctrl Pts',(73.7938092375739,1075.61827177418,499.634620781564));
#115925=CARTESIAN_POINT('Origin',(69.4825522658044,1067.7251047501,512.441691281815));
#115926=CARTESIAN_POINT('',(69.4825522658043,1076.93351373127,511.351150533087));
#115927=CARTESIAN_POINT('Ctrl Pts',(69.4826078971758,1076.70383791337,513.532232029124));
#115928=CARTESIAN_POINT('Ctrl Pts',(69.6122669881504,1076.69283316808,513.53222541487));
#115929=CARTESIAN_POINT('Ctrl Pts',(69.741060928863,1076.68435581015,513.509095376724));
#115930=CARTESIAN_POINT('Ctrl Pts',(69.9252523092832,1076.67604351272,513.440551985081));
#115931=CARTESIAN_POINT('Ctrl Pts',(69.9853778208891,1076.67402815309,513.411680414185));
#115932=CARTESIAN_POINT('Ctrl Pts',(70.0659665877485,1076.67235331882,513.363457985195));
#115933=CARTESIAN_POINT('Ctrl Pts',(70.0888854128759,1076.67200602563,513.348546524656));
#115934=CARTESIAN_POINT('Ctrl Pts',(70.124835040167,1076.67167395825,513.323184078409));
#115935=CARTESIAN_POINT('Ctrl Pts',(70.1382272484212,1076.67160062657,513.313268612612));
#115936=CARTESIAN_POINT('Ctrl Pts',(70.1654174322554,1076.67155755931,513.292155757156));
#115937=CARTESIAN_POINT('Ctrl Pts',(70.1791792986112,1076.67159500289,513.280920348107));
#115938=CARTESIAN_POINT('Ctrl Pts',(70.2104971720501,1076.6718205056,513.254050609814));
#115939=CARTESIAN_POINT('Ctrl Pts',(70.2278337040877,1076.67205325521,513.238175394666));
#115940=CARTESIAN_POINT('Ctrl Pts',(70.2805377597367,1076.67310876059,513.186685545547));
#115941=CARTESIAN_POINT('Ctrl Pts',(70.313961178618,1076.6743000496,513.149189903141));
#115942=CARTESIAN_POINT('Ctrl Pts',(70.433096754109,1076.68071441277,512.995396899938));
#115943=CARTESIAN_POINT('Ctrl Pts',(70.4978496578637,1076.68924152534,512.864994581949));
#115944=CARTESIAN_POINT('Ctrl Pts',(70.5663203402181,1076.71064373906,512.61141627984));
#115945=CARTESIAN_POINT('Ctrl Pts',(70.5783051673573,1076.72234162312,512.492743699219));
#115946=CARTESIAN_POINT('Ctrl Pts',(70.563071319087,1076.75002822772,512.245448508246));
#115947=CARTESIAN_POINT('Ctrl Pts',(70.5321875212895,1076.76610081385,512.118852361795));
#115948=CARTESIAN_POINT('Ctrl Pts',(70.423597375804,1076.80122707127,511.873231550895));
#115949=CARTESIAN_POINT('Ctrl Pts',(70.343309627338,1076.82011063196,511.757732408011));
#115950=CARTESIAN_POINT('Ctrl Pts',(70.1397826128885,1076.85782792288,511.559489641262));
#115951=CARTESIAN_POINT('Ctrl Pts',(70.0169040425762,1076.87627986179,511.480032211021));
#115952=CARTESIAN_POINT('Ctrl Pts',(69.7531366181056,1076.90878354048,511.376224666224));
#115953=CARTESIAN_POINT('Ctrl Pts',(69.6156653127265,1076.92271222959,511.350437098259));
#115954=CARTESIAN_POINT('Ctrl Pts',(69.346538439072,1076.94455379086,511.351849166121));
#115955=CARTESIAN_POINT('Ctrl Pts',(69.217258819437,1076.95260568815,511.37587845933));
#115956=CARTESIAN_POINT('Ctrl Pts',(69.0345315832573,1076.96033083147,511.445315644274));
#115957=CARTESIAN_POINT('Ctrl Pts',(68.976051749935,1076.96216491322,511.47372976735));
#115958=CARTESIAN_POINT('Ctrl Pts',(68.8973958977383,1076.96369723817,511.521042754245));
#115959=CARTESIAN_POINT('Ctrl Pts',(68.8748803697039,1076.96401668945,511.535746077119));
#115960=CARTESIAN_POINT('Ctrl Pts',(68.8394765478094,1076.96432238444,511.560780253401));
#115961=CARTESIAN_POINT('Ctrl Pts',(68.8262402256117,1076.96438970056,511.57059706391));
#115962=CARTESIAN_POINT('Ctrl Pts',(68.7993082234047,1076.96442783105,511.591533821189));
#115963=CARTESIAN_POINT('Ctrl Pts',(68.7856498519398,1076.96439152585,511.602693579264));
#115964=CARTESIAN_POINT('Ctrl Pts',(68.7544786491073,1076.96417654197,511.62944897881));
#115965=CARTESIAN_POINT('Ctrl Pts',(68.7371868096006,1076.96395496499,511.645287492151));
#115966=CARTESIAN_POINT('Ctrl Pts',(68.684337732467,1076.96294594852,511.696924573239));
#115967=CARTESIAN_POINT('Ctrl Pts',(68.6507528556428,1076.96180203104,511.734632888165));
#115968=CARTESIAN_POINT('Ctrl Pts',(68.5315755127396,1076.95565562866,511.888728652044));
#115969=CARTESIAN_POINT('Ctrl Pts',(68.4669153471803,1076.94750162141,512.019194209781));
#115970=CARTESIAN_POINT('Ctrl Pts',(68.3985531773248,1076.92686605912,512.273197251867));
#115971=CARTESIAN_POINT('Ctrl Pts',(68.3866861996268,1076.91552292664,512.392249928602));
#115972=CARTESIAN_POINT('Ctrl Pts',(68.4024229816617,1076.88846020786,512.640424938139));
#115973=CARTESIAN_POINT('Ctrl Pts',(68.4337620374989,1076.87263882435,512.767474808657));
#115974=CARTESIAN_POINT('Ctrl Pts',(68.5436959760718,1076.8377331556,513.013954870388));
#115975=CARTESIAN_POINT('Ctrl Pts',(68.6249513056033,1076.81879458981,513.12975867381));
#115976=CARTESIAN_POINT('Ctrl Pts',(68.815604926498,1076.78344747383,513.313466635032));
#115977=CARTESIAN_POINT('Ctrl Pts',(68.919582257624,1076.76723503197,513.383988540194));
#115978=CARTESIAN_POINT('Ctrl Pts',(69.0976126242619,1076.74366820895,513.464471225474));
#115979=CARTESIAN_POINT('Ctrl Pts',(69.1646234271701,1076.73558041456,513.487250429895));
#115980=CARTESIAN_POINT('Ctrl Pts',(69.3150133891904,1076.71909139178,513.522539992064));
#115981=CARTESIAN_POINT('Ctrl Pts',(69.3986264979972,1076.71096578925,513.532236313237));
#115982=CARTESIAN_POINT('Ctrl Pts',(69.4826078971757,1076.70383791337,513.532232029124));
#115983=CARTESIAN_POINT('',(69.4825522657769,1074.91619351132,511.351150533086));
#115984=CARTESIAN_POINT('',(69.4825522658044,1067.7251047501,511.351150533086));
#115985=CARTESIAN_POINT('Ctrl Pts',(69.4820444016945,1074.68466440541,513.532231912287));
#115986=CARTESIAN_POINT('Ctrl Pts',(69.3394705209171,1074.69687223284,513.532165515717));
#115987=CARTESIAN_POINT('Ctrl Pts',(69.1985379162362,1074.71192877342,513.504145529219));
#115988=CARTESIAN_POINT('Ctrl Pts',(68.9344311812239,1074.74606446002,513.395339502725));
#115989=CARTESIAN_POINT('Ctrl Pts',(68.8139383864327,1074.76485862075,513.315053679255));
#115990=CARTESIAN_POINT('Ctrl Pts',(68.6619976213376,1074.79379438774,513.163531925989));
#115991=CARTESIAN_POINT('Ctrl Pts',(68.6165657547483,1074.80347559918,513.108348181927));
#115992=CARTESIAN_POINT('Ctrl Pts',(68.4961976649056,1074.8325900277,512.92887515516));
#115993=CARTESIAN_POINT('Ctrl Pts',(68.4402223128954,1074.85151852095,512.793644469373));
#115994=CARTESIAN_POINT('Ctrl Pts',(68.3846015740659,1074.88595897511,512.509637830926));
#115995=CARTESIAN_POINT('Ctrl Pts',(68.3852108393213,1074.90115966746,512.363650922729));
#115996=CARTESIAN_POINT('Ctrl Pts',(68.443601734931,1074.92589973294,512.079989476065));
#115997=CARTESIAN_POINT('Ctrl Pts',(68.5007943994584,1074.93519072691,511.945190126555));
#115998=CARTESIAN_POINT('Ctrl Pts',(68.6628914927086,1074.94642867149,511.708550178006));
#115999=CARTESIAN_POINT('Ctrl Pts',(68.764964210655,1074.94843806051,511.60836412095));
#116000=CARTESIAN_POINT('Ctrl Pts',(69.0019088635042,1074.94515900181,511.452559146278));
#116001=CARTESIAN_POINT('Ctrl Pts',(69.1343968809284,1074.93989756299,511.398561240073));
#116002=CARTESIAN_POINT('Ctrl Pts',(69.4156680715146,1074.9224947882,511.343590363771));
#116003=CARTESIAN_POINT('Ctrl Pts',(69.5618379405238,1074.91037210208,511.344477112535));
#116004=CARTESIAN_POINT('Ctrl Pts',(69.8451847015609,1074.88081983878,511.403062532666));
#116005=CARTESIAN_POINT('Ctrl Pts',(69.9795342445981,1074.86367019389,511.460293514152));
#116006=CARTESIAN_POINT('Ctrl Pts',(70.1571436095353,1074.83603585489,511.581909187756));
#116007=CARTESIAN_POINT('Ctrl Pts',(70.2115395624646,1074.8266691463,511.627523778567));
#116008=CARTESIAN_POINT('Ctrl Pts',(70.3108605259358,1074.80762135251,511.728787369085));
#116009=CARTESIAN_POINT('Ctrl Pts',(70.3555302526697,1074.79798169931,511.784245543407));
#116010=CARTESIAN_POINT('Ctrl Pts',(70.4747269729781,1074.76860477466,511.966004496857));
#116011=CARTESIAN_POINT('Ctrl Pts',(70.5295976336062,1074.74926883606,512.103373722146));
#116012=CARTESIAN_POINT('Ctrl Pts',(70.5812274960528,1074.71422832265,512.388845353581));
#116013=CARTESIAN_POINT('Ctrl Pts',(70.5786812208422,1074.69878838845,512.533982227166));
#116014=CARTESIAN_POINT('Ctrl Pts',(70.517467466125,1074.67375549784,512.813910243385));
#116015=CARTESIAN_POINT('Ctrl Pts',(70.4599660560575,1074.66435260242,512.946048139922));
#116016=CARTESIAN_POINT('Ctrl Pts',(70.2976701742277,1074.65290348342,513.179891536469));
#116017=CARTESIAN_POINT('Ctrl Pts',(70.1949339328048,1074.65091110759,513.279484386364));
#116018=CARTESIAN_POINT('Ctrl Pts',(69.9572467919293,1074.65459479166,513.433643157594));
#116019=CARTESIAN_POINT('Ctrl Pts',(69.8247872974603,1074.66021707146,513.486728871373));
#116020=CARTESIAN_POINT('Ctrl Pts',(69.6187299662236,1074.67364883709,513.525862309228));
#116021=CARTESIAN_POINT('Ctrl Pts',(69.5504341427086,1074.67880856315,513.532263761348));
#116022=CARTESIAN_POINT('Ctrl Pts',(69.4820444016944,1074.68466440541,513.532231912287));
#116023=CARTESIAN_POINT('Origin',(69.4825522658044,1067.7251047501,512.441691281815));
#116024=CARTESIAN_POINT('',(69.4825522658045,1074.74977363876,512.932232030543));
#116025=CARTESIAN_POINT('',(69.4825522658044,1074.85393827482,511.951150533086));
#116026=CARTESIAN_POINT('Ctrl Pts',(69.4825522658045,1074.74977363876,512.932232030543));
#116027=CARTESIAN_POINT('Ctrl Pts',(69.449079001942,1074.75260930569,512.932232030543));
#116028=CARTESIAN_POINT('Ctrl Pts',(69.4156422604509,1074.75580684056,512.928805735255));
#116029=CARTESIAN_POINT('Ctrl Pts',(69.3196946475562,1074.76605381396,512.908872049097));
#116030=CARTESIAN_POINT('Ctrl Pts',(69.2599081233851,1074.7738132317,512.883491244156));
#116031=CARTESIAN_POINT('Ctrl Pts',(69.1802249341963,1074.78629861362,512.829324110509));
#116032=CARTESIAN_POINT('Ctrl Pts',(69.1555178518989,1074.79057166016,512.808717383512));
#116033=CARTESIAN_POINT('Ctrl Pts',(69.1105321240183,1074.79921186373,512.763028191438));
#116034=CARTESIAN_POINT('Ctrl Pts',(69.090346984417,1074.80355955703,512.738054954091));
#116035=CARTESIAN_POINT('Ctrl Pts',(69.0368499035733,1074.81667515841,512.656736030347));
#116036=CARTESIAN_POINT('Ctrl Pts',(69.0121780541397,1074.82522094721,512.595505966556));
#116037=CARTESIAN_POINT('Ctrl Pts',(68.9883421325934,1074.84078388337,512.467035695293));
#116038=CARTESIAN_POINT('Ctrl Pts',(68.9893356107765,1074.8476554736,512.401053500535));
#116039=CARTESIAN_POINT('Ctrl Pts',(69.017058142962,1074.85872061286,512.27401364987));
#116040=CARTESIAN_POINT('Ctrl Pts',(69.0431699591804,1074.86283865761,512.214168299575));
#116041=CARTESIAN_POINT('Ctrl Pts',(69.1166676980363,1074.86779966899,512.108797235077));
#116042=CARTESIAN_POINT('Ctrl Pts',(69.1629663043581,1074.86864416037,512.064120133381));
#116043=CARTESIAN_POINT('Ctrl Pts',(69.2701100198263,1074.86700441952,511.994964613161));
#116044=CARTESIAN_POINT('Ctrl Pts',(69.3298661792914,1074.86453637549,511.971192686971));
#116045=CARTESIAN_POINT('Ctrl Pts',(69.4221751405219,1074.858671246,511.953941216856));
#116046=CARTESIAN_POINT('Ctrl Pts',(69.4523419826411,1074.85645423452,511.951150631426));
#116047=CARTESIAN_POINT('Ctrl Pts',(69.4825506689621,1074.85393840781,511.951150533089));
#116048=CARTESIAN_POINT('',(69.4825522658044,1082.7251047501,511.951150533086));
#116049=CARTESIAN_POINT('',(69.4825522658044,1067.7251047501,511.951150533086));
#116050=CARTESIAN_POINT('Origin',(69.4825522658044,1082.7251047501,512.441691281815));
#116051=CARTESIAN_POINT('Ctrl Pts',(69.4825522658042,1074.85393827482,511.951150533086));
#116052=CARTESIAN_POINT('Ctrl Pts',(69.5480076026392,1074.8484870293,511.951150533086));
#116053=CARTESIAN_POINT('Ctrl Pts',(69.6126865705572,1074.84171403297,511.964248612907));
#116054=CARTESIAN_POINT('Ctrl Pts',(69.7331209623984,1074.82629764847,512.014929237526));
#116055=CARTESIAN_POINT('Ctrl Pts',(69.7876777637123,1074.81779887447,512.052086079148));
#116056=CARTESIAN_POINT('Ctrl Pts',(69.8556816419551,1074.80471537265,512.121648042885));
#116057=CARTESIAN_POINT('Ctrl Pts',(69.8757492299989,1074.80037531797,512.146650205093));
#116058=CARTESIAN_POINT('Ctrl Pts',(69.9291246522644,1074.78720272623,512.228362682958));
#116059=CARTESIAN_POINT('Ctrl Pts',(69.9536570560271,1074.77856974081,512.289994969465));
#116060=CARTESIAN_POINT('Ctrl Pts',(69.9768429254042,1074.76288232822,512.418650406565));
#116061=CARTESIAN_POINT('Ctrl Pts',(69.9755636053974,1074.7559614686,512.484375975875));
#116062=CARTESIAN_POINT('Ctrl Pts',(69.9475407365004,1074.74482450298,512.61056883289));
#116063=CARTESIAN_POINT('Ctrl Pts',(69.9215175585826,1074.74067272418,512.669872078126));
#116064=CARTESIAN_POINT('Ctrl Pts',(69.8482518897609,1074.73563614165,512.774790752987));
#116065=CARTESIAN_POINT('Ctrl Pts',(69.8019190784616,1074.73477696069,512.819450070359));
#116066=CARTESIAN_POINT('Ctrl Pts',(69.6947818169604,1074.7364624146,512.888508879183));
#116067=CARTESIAN_POINT('Ctrl Pts',(69.6350868502195,1074.7389856868,512.912228790736));
#116068=CARTESIAN_POINT('Ctrl Pts',(69.542803701313,1074.744964776,512.929459774938));
#116069=CARTESIAN_POINT('Ctrl Pts',(69.5126632077471,1074.74722280885,512.932232030543));
#116070=CARTESIAN_POINT('Ctrl Pts',(69.4825522658045,1074.74977363876,512.932232030543));
#116071=CARTESIAN_POINT('Origin',(83.8577571500221,1067.7251047501,456.061503599423));
#116072=CARTESIAN_POINT('',(83.8577571500471,1078.68595559847,454.58320046723));
#116073=CARTESIAN_POINT('Ctrl Pts',(83.857895722855,1078.6591843157,457.539806725122));
#116074=CARTESIAN_POINT('Ctrl Pts',(84.0501826867988,1078.65404884633,457.539788700571));
#116075=CARTESIAN_POINT('Ctrl Pts',(84.2406408333334,1078.64908129588,457.502253888277));
#116076=CARTESIAN_POINT('Ctrl Pts',(84.5743214387011,1078.64088084795,457.365440788119));
#116077=CARTESIAN_POINT('Ctrl Pts',(84.718037646745,1078.63757322054,457.275440178014));
#116078=CARTESIAN_POINT('Ctrl Pts',(84.9597562330392,1078.63267847603,457.059157454937));
#116079=CARTESIAN_POINT('Ctrl Pts',(85.0588207078151,1078.6310153872,456.937383861936));
#116080=CARTESIAN_POINT('Ctrl Pts',(85.1596304165353,1078.62990767214,456.7633181193));
#116081=CARTESIAN_POINT('Ctrl Pts',(85.1804514808721,1078.6297267007,456.723241749134));
#116082=CARTESIAN_POINT('Ctrl Pts',(85.2104913314188,1078.62954871999,456.658317834723));
#116083=CARTESIAN_POINT('Ctrl Pts',(85.2209326799639,1078.62950655315,456.634067548322));
#116084=CARTESIAN_POINT('Ctrl Pts',(85.239011086755,1078.62947224598,456.588777709061));
#116085=CARTESIAN_POINT('Ctrl Pts',(85.2468305538254,1078.6294734533,456.567819215659));
#116086=CARTESIAN_POINT('Ctrl Pts',(85.2630399000802,1078.62951352662,456.521167252621));
#116087=CARTESIAN_POINT('Ctrl Pts',(85.27120684045,1078.62956017016,456.495404797611));
#116088=CARTESIAN_POINT('Ctrl Pts',(85.292214551982,1078.62976095209,456.422230426666));
#116089=CARTESIAN_POINT('Ctrl Pts',(85.3034053828301,1078.6299716987,456.37438217292));
#116090=CARTESIAN_POINT('Ctrl Pts',(85.3473339019269,1078.63142373511,456.132884567486));
#116091=CARTESIAN_POINT('Ctrl Pts',(85.3436337191116,1078.63385382327,455.934638312188));
#116092=CARTESIAN_POINT('Ctrl Pts',(85.2673723068792,1078.6400585357,455.589076190886));
#116093=CARTESIAN_POINT('Ctrl Pts',(85.2090444140144,1078.64342875293,455.441649644837));
#116094=CARTESIAN_POINT('Ctrl Pts',(85.0407378233742,1078.65129476155,455.15846130064));
#116095=CARTESIAN_POINT('Ctrl Pts',(84.9278135471952,1078.65580171458,455.027142050148));
#116096=CARTESIAN_POINT('Ctrl Pts',(84.6521900266623,1078.66535009839,454.801228067949));
#116097=CARTESIAN_POINT('Ctrl Pts',(84.4888587419943,1078.67031854076,454.712010624993));
#116098=CARTESIAN_POINT('Ctrl Pts',(84.1272415690971,1078.67997968496,454.594866421756));
#116099=CARTESIAN_POINT('Ctrl Pts',(83.9310060435655,1078.68454131793,454.572111169916));
#116100=CARTESIAN_POINT('Ctrl Pts',(83.5456899038228,1078.69237044383,454.60394709358));
#116101=CARTESIAN_POINT('Ctrl Pts',(83.3601782355851,1078.69559819491,454.65641279354));
#116102=CARTESIAN_POINT('Ctrl Pts',(83.0422820629693,1078.70038697822,454.81743061677));
#116103=CARTESIAN_POINT('Ctrl Pts',(82.9083529441599,1078.70208456588,454.916360716088));
#116104=CARTESIAN_POINT('Ctrl Pts',(82.7052131785727,1078.70421724732,455.127035596776));
#116105=CARTESIAN_POINT('Ctrl Pts',(82.6290517179936,1078.70484431844,455.229715316369));
#116106=CARTESIAN_POINT('Ctrl Pts',(82.5467639482396,1078.70529344552,455.377107029814));
#116107=CARTESIAN_POINT('Ctrl Pts',(82.5280715782491,1078.70537283249,455.414172053926));
#116108=CARTESIAN_POINT('Ctrl Pts',(82.5006240037821,1078.70545074768,455.474819214385));
#116109=CARTESIAN_POINT('Ctrl Pts',(82.4908677776319,1078.70546882236,455.49792362392));
#116110=CARTESIAN_POINT('Ctrl Pts',(82.4743523585173,1078.70548110583,455.539990396581));
#116111=CARTESIAN_POINT('Ctrl Pts',(82.4673837486615,1078.70547932534,455.558863924635));
#116112=CARTESIAN_POINT('Ctrl Pts',(82.4519822322641,1078.70545819374,455.60335088314));
#116113=CARTESIAN_POINT('Ctrl Pts',(82.4438605960793,1078.70543307706,455.629064511982));
#116114=CARTESIAN_POINT('Ctrl Pts',(82.4227439641766,1078.70532439608,455.702894709613));
#116115=CARTESIAN_POINT('Ctrl Pts',(82.4114723624004,1078.70520943202,455.751465743107));
#116116=CARTESIAN_POINT('Ctrl Pts',(82.3679412476656,1078.70441873335,455.994161466607));
#116117=CARTESIAN_POINT('Ctrl Pts',(82.3722126048156,1078.70310566954,456.192805463357));
#116118=CARTESIAN_POINT('Ctrl Pts',(82.4498696732354,1078.69940825983,456.539333448924));
#116119=CARTESIAN_POINT('Ctrl Pts',(82.5091214958284,1078.69730138823,456.687320321736));
#116120=CARTESIAN_POINT('Ctrl Pts',(82.6799381027615,1078.69189796453,456.971514598402));
#116121=CARTESIAN_POINT('Ctrl Pts',(82.7945553185853,1078.68854615125,457.103124026201));
#116122=CARTESIAN_POINT('Ctrl Pts',(83.0589086833123,1078.68103416303,457.316474892323));
#116123=CARTESIAN_POINT('Ctrl Pts',(83.2052366795662,1078.67696202899,457.398411926288));
#116124=CARTESIAN_POINT('Ctrl Pts',(83.5212696691922,1078.66826446424,457.510881285026));
#116125=CARTESIAN_POINT('Ctrl Pts',(83.6889634141074,1078.66369604484,457.539822560459));
#116126=CARTESIAN_POINT('Ctrl Pts',(83.857895722855,1078.6591843157,457.539806725122));
#116127=CARTESIAN_POINT('',(83.8577571500032,1076.68539762474,454.58320046723));
#116128=CARTESIAN_POINT('',(83.8577571500221,1067.7251047501,454.58320046723));
#116129=CARTESIAN_POINT('Ctrl Pts',(83.8571954838192,1076.65832806552,457.539806624917));
#116130=CARTESIAN_POINT('Ctrl Pts',(83.6639119834466,1076.66355105368,457.539733188816));
#116131=CARTESIAN_POINT('Ctrl Pts',(83.4725026434182,1076.66883992384,457.5017536051));
#116132=CARTESIAN_POINT('Ctrl Pts',(83.1151092303283,1076.67882739148,457.354265983379));
#116133=CARTESIAN_POINT('Ctrl Pts',(82.9525718107223,1076.68342942717,457.246159064353));
#116134=CARTESIAN_POINT('Ctrl Pts',(82.6771709865733,1076.69149751766,456.972338653538));
#116135=CARTESIAN_POINT('Ctrl Pts',(82.5674425843615,1076.69487994061,456.808833048692));
#116136=CARTESIAN_POINT('Ctrl Pts',(82.4177379379093,1076.7002538874,456.44854537559));
#116137=CARTESIAN_POINT('Ctrl Pts',(82.3792750403163,1076.70220032726,456.255288785364));
#116138=CARTESIAN_POINT('Ctrl Pts',(82.3796349258613,1076.70472115355,455.864260269205));
#116139=CARTESIAN_POINT('Ctrl Pts',(82.4187468703183,1076.70527147427,455.670349959404));
#116140=CARTESIAN_POINT('Ctrl Pts',(82.5702395422862,1076.70500246619,455.309168589201));
#116141=CARTESIAN_POINT('Ctrl Pts',(82.6810802262658,1076.70418581685,455.145458431561));
#116142=CARTESIAN_POINT('Ctrl Pts',(82.9595479947621,1076.70111661657,454.871279807384));
#116143=CARTESIAN_POINT('Ctrl Pts',(83.1242181473936,1076.69889278287,454.7633022341));
#116144=CARTESIAN_POINT('Ctrl Pts',(83.4861185286791,1076.69296530367,454.61742433396));
#116145=CARTESIAN_POINT('Ctrl Pts',(83.6798175416097,1076.68931013321,454.581027832075));
#116146=CARTESIAN_POINT('Ctrl Pts',(83.9707694676161,1076.68291524758,454.584416412143));
#116147=CARTESIAN_POINT('Ctrl Pts',(84.0662279375089,1076.68067306608,454.594841687333));
#116148=CARTESIAN_POINT('Ctrl Pts',(84.2555261586187,1076.67591578607,454.634379563519));
#116149=CARTESIAN_POINT('Ctrl Pts',(84.3488386880646,1076.67340794898,454.663740659378));
#116150=CARTESIAN_POINT('Ctrl Pts',(84.6169810283324,1076.66569950907,454.778304904097));
#116151=CARTESIAN_POINT('Ctrl Pts',(84.7786502908841,1076.66035445157,454.888910304203));
#116152=CARTESIAN_POINT('Ctrl Pts',(85.0501368360057,1076.65001067064,455.166344833762));
#116153=CARTESIAN_POINT('Ctrl Pts',(85.1572813234135,1076.6451186208,455.330528614358));
#116154=CARTESIAN_POINT('Ctrl Pts',(85.3019583596872,1076.63678412459,455.690892624565));
#116155=CARTESIAN_POINT('Ctrl Pts',(85.3381013789166,1076.63342948226,455.883563481951));
#116156=CARTESIAN_POINT('Ctrl Pts',(85.3338456226123,1076.62902403533,456.271481836929));
#116157=CARTESIAN_POINT('Ctrl Pts',(85.2936440839372,1076.62801568502,456.46295270076));
#116158=CARTESIAN_POINT('Ctrl Pts',(85.1418631734501,1076.62859370268,456.819001944414));
#116159=CARTESIAN_POINT('Ctrl Pts',(85.031945038628,1076.63016690374,456.980202608986));
#116160=CARTESIAN_POINT('Ctrl Pts',(84.7565214178857,1076.63555268389,457.250976790726));
#116161=CARTESIAN_POINT('Ctrl Pts',(84.5937449471793,1076.63930519792,457.358011815409));
#116162=CARTESIAN_POINT('Ctrl Pts',(84.237882256376,1076.64816033336,457.502844080452));
#116163=CARTESIAN_POINT('Ctrl Pts',(84.0484294235124,1076.65316046145,457.539879282308));
#116164=CARTESIAN_POINT('Ctrl Pts',(83.8571954838192,1076.65832806552,457.539806624917));
#116165=CARTESIAN_POINT('Origin',(83.8577571500221,1067.7251047501,456.061503599423));
#116166=CARTESIAN_POINT('',(83.8577571500221,1076.66449392106,456.939806731617));
#116167=CARTESIAN_POINT('',(83.8577571500243,1076.68056431803,455.18320046723));
#116168=CARTESIAN_POINT('Ctrl Pts',(83.8577571500221,1076.66449392106,456.939806731616));
#116169=CARTESIAN_POINT('Ctrl Pts',(83.7491563869114,1076.66731144614,456.939806731616));
#116170=CARTESIAN_POINT('Ctrl Pts',(83.64143436695,1076.67021713204,456.919663328342));
#116171=CARTESIAN_POINT('Ctrl Pts',(83.4329170859451,1076.67603402612,456.838768819911));
#116172=CARTESIAN_POINT('Ctrl Pts',(83.3349402934638,1076.67887787434,456.776552656778));
#116173=CARTESIAN_POINT('Ctrl Pts',(83.1673710954663,1076.68403158457,456.616811491697));
#116174=CARTESIAN_POINT('Ctrl Pts',(83.0998519482754,1076.68628429903,456.520396479986));
#116175=CARTESIAN_POINT('Ctrl Pts',(83.0064065376708,1076.68996027735,456.306855913284));
#116176=CARTESIAN_POINT('Ctrl Pts',(82.9813977169083,1076.69135025765,456.19185765644));
#116177=CARTESIAN_POINT('Ctrl Pts',(82.9777244290133,1076.69319196447,455.958576204661));
#116178=CARTESIAN_POINT('Ctrl Pts',(82.9991882680623,1076.69362560699,455.842615681471));
#116179=CARTESIAN_POINT('Ctrl Pts',(83.0861994999065,1076.69351107157,455.625904651252));
#116180=CARTESIAN_POINT('Ctrl Pts',(83.1508707555719,1076.69296406066,455.527314243881));
#116181=CARTESIAN_POINT('Ctrl Pts',(83.3148040429077,1076.69090032807,455.361364456753));
#116182=CARTESIAN_POINT('Ctrl Pts',(83.4123680647117,1076.68940369389,455.295593094294));
#116183=CARTESIAN_POINT('Ctrl Pts',(83.6269699886546,1076.68554041562,455.206164115548));
#116184=CARTESIAN_POINT('Ctrl Pts',(83.7418004079885,1076.68321289986,455.18320046723));
#116185=CARTESIAN_POINT('Ctrl Pts',(83.8577571500265,1076.68056431803,455.18320046723));
#116186=CARTESIAN_POINT('',(83.8577571500221,1082.7251047501,455.18320046723));
#116187=CARTESIAN_POINT('',(83.8577571500221,1067.7251047501,455.18320046723));
#116188=CARTESIAN_POINT('Origin',(83.8577571500221,1082.7251047501,456.061503599423));
#116189=CARTESIAN_POINT('Ctrl Pts',(83.8577571500264,1076.68056431803,455.18320046723));
#116190=CARTESIAN_POINT('Ctrl Pts',(83.8583775614648,1076.68055014713,455.18320046723));
#116191=CARTESIAN_POINT('Ctrl Pts',(83.8589980051472,1076.68053596712,455.183201124595));
#116192=CARTESIAN_POINT('Ctrl Pts',(83.9167484364247,1076.67921531978,455.183323511558));
#116193=CARTESIAN_POINT('Ctrl Pts',(83.973729065245,1076.67784084955,455.189018396919));
#116194=CARTESIAN_POINT('Ctrl Pts',(84.0866258061812,1076.67496599451,455.211562807171));
#116195=CARTESIAN_POINT('Ctrl Pts',(84.142235845964,1076.67347102156,455.228525885965));
#116196=CARTESIAN_POINT('Ctrl Pts',(84.3020804656356,1076.66893066948,455.295174012744));
#116197=CARTESIAN_POINT('Ctrl Pts',(84.398644774739,1076.6658514267,455.359987187322));
#116198=CARTESIAN_POINT('Ctrl Pts',(84.5612830577236,1076.65998142773,455.523221426675));
#116199=CARTESIAN_POINT('Ctrl Pts',(84.6257688330966,1076.65724973988,455.620076851781));
#116200=CARTESIAN_POINT('Ctrl Pts',(84.7117989206522,1076.65271883418,455.828666388698));
#116201=CARTESIAN_POINT('Ctrl Pts',(84.7342768823954,1076.65092765027,455.937741862609));
#116202=CARTESIAN_POINT('Ctrl Pts',(84.7359583932156,1076.64970293009,456.048125689504));
#116203=CARTESIAN_POINT('Ctrl Pts',(84.7377114048492,1076.64842613264,456.163203231901));
#116204=CARTESIAN_POINT('Ctrl Pts',(84.7168283306949,1076.64779110094,456.277514211922));
#116205=CARTESIAN_POINT('Ctrl Pts',(84.632235179076,1076.64791761215,456.491389717655));
#116206=CARTESIAN_POINT('Ctrl Pts',(84.5694184676888,1076.64867542544,456.588907253751));
#116207=CARTESIAN_POINT('Ctrl Pts',(84.4098843528329,1076.65144475292,456.75414263032));
#116208=CARTESIAN_POINT('Ctrl Pts',(84.3147370841928,1076.65342659934,456.820291355855));
#116209=CARTESIAN_POINT('Ctrl Pts',(84.1043647865005,1076.65825257172,456.91225928783));
#116210=CARTESIAN_POINT('Ctrl Pts',(83.9911573508748,1076.66104800146,456.937175987832));
#116211=CARTESIAN_POINT('Ctrl Pts',(83.8701655771886,1076.66417236966,456.93974102359));
#116212=CARTESIAN_POINT('Ctrl Pts',(83.8639599301777,1076.66433299688,456.939806731616));
#116213=CARTESIAN_POINT('Ctrl Pts',(83.8577571500221,1076.66449392106,456.939806731616));
#116214=CARTESIAN_POINT('Origin',(86.2654713137628,1067.7251047501,468.386802343567));
#116215=CARTESIAN_POINT('',(86.2654713137801,1078.38513071259,467.111358222431));
#116216=CARTESIAN_POINT('Ctrl Pts',(86.2657852622204,1078.31122975657,469.662246426064));
#116217=CARTESIAN_POINT('Ctrl Pts',(86.4293026174469,1078.30152800511,469.662206176537));
#116218=CARTESIAN_POINT('Ctrl Pts',(86.5913564979556,1078.29272124248,469.630720814669));
#116219=CARTESIAN_POINT('Ctrl Pts',(86.8771104038815,1078.27890818702,469.51531799073));
#116220=CARTESIAN_POINT('Ctrl Pts',(87.0010080273735,1078.27368093332,469.438782944172));
#116221=CARTESIAN_POINT('Ctrl Pts',(87.1845084955334,1078.26743513783,469.276830663847));
#116222=CARTESIAN_POINT('Ctrl Pts',(87.2515171699036,1078.26563813553,469.20197029594));
#116223=CARTESIAN_POINT('Ctrl Pts',(87.3287326703871,1078.26430944613,469.092069028911));
#116224=CARTESIAN_POINT('Ctrl Pts',(87.3472491563598,1078.26406575919,469.063324775724));
#116225=CARTESIAN_POINT('Ctrl Pts',(87.3753205107532,1078.26382535787,469.015642474366));
#116226=CARTESIAN_POINT('Ctrl Pts',(87.3855968720574,1078.26376994913,468.997149697114));
#116227=CARTESIAN_POINT('Ctrl Pts',(87.4043122313338,1078.2637340015,468.961404405957));
#116228=CARTESIAN_POINT('Ctrl Pts',(87.4128308217793,1078.26374701227,468.944200157969));
#116229=CARTESIAN_POINT('Ctrl Pts',(87.4313377728443,1078.26384518279,468.904599750075));
#116230=CARTESIAN_POINT('Ctrl Pts',(87.4410750442437,1078.2639493232,468.882094785677));
#116231=CARTESIAN_POINT('Ctrl Pts',(87.468463229481,1078.26441083778,468.813428202348));
#116232=CARTESIAN_POINT('Ctrl Pts',(87.4840856653855,1078.26491761532,468.766509914351));
#116233=CARTESIAN_POINT('Ctrl Pts',(87.5410400564051,1078.26802511382,468.555253403917));
#116234=CARTESIAN_POINT('Ctrl Pts',(87.552098884957,1078.27269527593,468.38460081847));
#116235=CARTESIAN_POINT('Ctrl Pts',(87.5112581261407,1078.28461173621,468.080880886857));
#116236=CARTESIAN_POINT('Ctrl Pts',(87.4711738657788,1078.29112017823,467.948819592391));
#116237=CARTESIAN_POINT('Ctrl Pts',(87.3451063275319,1078.30653492293,467.691463710751));
#116238=CARTESIAN_POINT('Ctrl Pts',(87.2562627253326,1078.31548411419,467.569846163314));
#116239=CARTESIAN_POINT('Ctrl Pts',(87.0325714867284,1078.3349540528,467.355253190721));
#116240=CARTESIAN_POINT('Ctrl Pts',(86.8967577700272,1078.34536821816,467.266975472739));
#116241=CARTESIAN_POINT('Ctrl Pts',(86.5918757201393,1078.36623672665,467.142326464495));
#116242=CARTESIAN_POINT('Ctrl Pts',(86.4244251035465,1078.37646189505,467.110079125792));
#116243=CARTESIAN_POINT('Ctrl Pts',(86.0917677391716,1078.39460656449,467.112674756566));
#116244=CARTESIAN_POINT('Ctrl Pts',(85.9297263499821,1078.40242275936,467.145477650272));
#116245=CARTESIAN_POINT('Ctrl Pts',(85.6438360406098,1078.41444363172,467.263641401564));
#116246=CARTESIAN_POINT('Ctrl Pts',(85.5198491895828,1078.41886952241,467.341818930712));
#116247=CARTESIAN_POINT('Ctrl Pts',(85.3396895087518,1078.42398312233,467.504144282614));
#116248=CARTESIAN_POINT('Ctrl Pts',(85.275289481429,1078.42540855033,467.577048896656));
#116249=CARTESIAN_POINT('Ctrl Pts',(85.2005866668197,1078.4264705406,467.684021425547));
#116250=CARTESIAN_POINT('Ctrl Pts',(85.1824928022474,1078.42666681158,467.712237347808));
#116251=CARTESIAN_POINT('Ctrl Pts',(85.1549758934935,1078.42686075099,467.759114244863));
#116252=CARTESIAN_POINT('Ctrl Pts',(85.1448634543236,1078.42690540145,467.777351395219));
#116253=CARTESIAN_POINT('Ctrl Pts',(85.1264023954751,1078.42693384648,467.812659132235));
#116254=CARTESIAN_POINT('Ctrl Pts',(85.1179792311707,1078.4269227042,467.829684450228));
#116255=CARTESIAN_POINT('Ctrl Pts',(85.099630581685,1078.42684091163,467.868954728429));
#116256=CARTESIAN_POINT('Ctrl Pts',(85.0899558199228,1078.42675437259,467.891308574778));
#116257=CARTESIAN_POINT('Ctrl Pts',(85.0626207102447,1078.42636969244,467.959782320886));
#116258=CARTESIAN_POINT('Ctrl Pts',(85.0469932150047,1078.42594586247,468.006662213625));
#116259=CARTESIAN_POINT('Ctrl Pts',(84.9899689910333,1078.42333734457,468.217856632479));
#116260=CARTESIAN_POINT('Ctrl Pts',(84.9788404704766,1078.41940782907,468.388513222671));
#116261=CARTESIAN_POINT('Ctrl Pts',(85.0196343830212,1078.40909248344,468.692729001687));
#116262=CARTESIAN_POINT('Ctrl Pts',(85.0598810477708,1078.40336881025,468.825243477131));
#116263=CARTESIAN_POINT('Ctrl Pts',(85.1866963835772,1078.38943448805,469.083644742128));
#116264=CARTESIAN_POINT('Ctrl Pts',(85.2762164602593,1078.38114900311,469.20576072949));
#116265=CARTESIAN_POINT('Ctrl Pts',(85.501864338204,1078.36251506303,469.421121871411));
#116266=CARTESIAN_POINT('Ctrl Pts',(85.639015606967,1078.35222191931,469.509500663051));
#116267=CARTESIAN_POINT('Ctrl Pts',(85.9405155358859,1078.33133210487,469.630926748259));
#116268=CARTESIAN_POINT('Ctrl Pts',(86.1023854601413,1078.3209245334,469.662286646656));
#116269=CARTESIAN_POINT('Ctrl Pts',(86.2657852622204,1078.31122975657,469.662246426064));
#116270=CARTESIAN_POINT('',(86.2654713137447,1076.38122798592,467.111358222431));
#116271=CARTESIAN_POINT('',(86.2654713137628,1067.7251047501,467.111358222431));
#116272=CARTESIAN_POINT('Ctrl Pts',(86.2659892652717,1076.3065438716,469.662246359534));
#116273=CARTESIAN_POINT('Ctrl Pts',(86.0990110388632,1076.31655262552,469.662314168567));
#116274=CARTESIAN_POINT('Ctrl Pts',(85.9336598964842,1076.3273118429,469.629591248244));
#116275=CARTESIAN_POINT('Ctrl Pts',(85.7021327202753,1076.34357417979,469.534138393049));
#116276=CARTESIAN_POINT('Ctrl Pts',(85.6282420575696,1076.34897918251,469.494805264416));
#116277=CARTESIAN_POINT('Ctrl Pts',(85.4175456889382,1076.3650722077,469.354553963634));
#116278=CARTESIAN_POINT('Ctrl Pts',(85.2964793286387,1076.37529935133,469.233328924411));
#116279=CARTESIAN_POINT('Ctrl Pts',(85.1094441551327,1076.39350676399,468.951419131407));
#116280=CARTESIAN_POINT('Ctrl Pts',(85.0449708655218,1076.40132620614,468.793756169916));
#116281=CARTESIAN_POINT('Ctrl Pts',(84.9811268117638,1076.41376165968,468.462324009853));
#116282=CARTESIAN_POINT('Ctrl Pts',(84.9824054704497,1076.41825857064,468.291845287455));
#116283=CARTESIAN_POINT('Ctrl Pts',(85.0513882282358,1076.42346813979,467.960915715412));
#116284=CARTESIAN_POINT('Ctrl Pts',(85.1185202239477,1076.4241245211,467.803805578061));
#116285=CARTESIAN_POINT('Ctrl Pts',(85.3100788862593,1076.42149000419,467.52509062931));
#116286=CARTESIAN_POINT('Ctrl Pts',(85.4325239584889,1076.41822820435,467.406242546533));
#116287=CARTESIAN_POINT('Ctrl Pts',(85.7163259414703,1076.40806435727,467.223335420329));
#116288=CARTESIAN_POINT('Ctrl Pts',(85.8748006196462,1076.40126404783,467.161015982234));
#116289=CARTESIAN_POINT('Ctrl Pts',(86.207338620264,1076.38475895787,467.101491973826));
#116290=CARTESIAN_POINT('Ctrl Pts',(86.3781587396811,1076.37520173521,467.105136950802));
#116291=CARTESIAN_POINT('Ctrl Pts',(86.6243099064432,1076.35973799447,467.160061550193));
#116292=CARTESIAN_POINT('Ctrl Pts',(86.7034162619302,1076.35448602985,467.186027677112));
#116293=CARTESIAN_POINT('Ctrl Pts',(86.8566195534566,1076.34372468397,467.2534819613));
#116294=CARTESIAN_POINT('Ctrl Pts',(86.9302484684515,1076.33823863164,467.295041298377));
#116295=CARTESIAN_POINT('Ctrl Pts',(87.1363509583598,1076.32190336354,467.440003227648));
#116296=CARTESIAN_POINT('Ctrl Pts',(87.2531466267127,1076.31126142937,467.562557477571));
#116297=CARTESIAN_POINT('Ctrl Pts',(87.4325825032181,1076.29179595377,467.845790468995));
#116298=CARTESIAN_POINT('Ctrl Pts',(87.4935301684182,1076.28316302257,468.003711654092));
#116299=CARTESIAN_POINT('Ctrl Pts',(87.5507426137669,1076.26931200386,468.333770842427));
#116300=CARTESIAN_POINT('Ctrl Pts',(87.5466236263288,1076.26422399356,468.50265306745));
#116301=CARTESIAN_POINT('Ctrl Pts',(87.4734851819258,1076.25846048254,468.828699693846));
#116302=CARTESIAN_POINT('Ctrl Pts',(87.4054162907907,1076.25782771373,468.982706349862));
#116303=CARTESIAN_POINT('Ctrl Pts',(87.2140597338252,1076.26114034261,469.255500400334));
#116304=CARTESIAN_POINT('Ctrl Pts',(87.0927642320039,1076.26504221223,469.371694400366));
#116305=CARTESIAN_POINT('Ctrl Pts',(86.8123871363491,1076.27677433783,469.550998739777));
#116306=CARTESIAN_POINT('Ctrl Pts',(86.6559935268662,1076.28449022634,469.612329798631));
#116307=CARTESIAN_POINT('Ctrl Pts',(86.4176130659882,1076.29763161351,469.655412796818));
#116308=CARTESIAN_POINT('Ctrl Pts',(86.3418720166314,1076.30199542357,469.662215543924));
#116309=CARTESIAN_POINT('Ctrl Pts',(86.2659892652717,1076.3065438716,469.662246359534));
#116310=CARTESIAN_POINT('Origin',(86.2654713137628,1067.7251047501,468.386802343567));
#116311=CARTESIAN_POINT('',(86.2654713137628,1076.32506388483,469.062246464703));
#116312=CARTESIAN_POINT('',(86.265471313763,1076.36458696229,467.711358222431));
#116313=CARTESIAN_POINT('Ctrl Pts',(86.2654713137628,1076.32506388483,469.062246464703));
#116314=CARTESIAN_POINT('Ctrl Pts',(86.221131644048,1076.3276742955,469.062246464703));
#116315=CARTESIAN_POINT('Ctrl Pts',(86.176799990606,1076.33040428046,469.057880406972));
#116316=CARTESIAN_POINT('Ctrl Pts',(86.0897630260982,1076.33600127725,469.040489378451));
#116317=CARTESIAN_POINT('Ctrl Pts',(86.0473582127218,1076.33884722441,469.027588123505));
#116318=CARTESIAN_POINT('Ctrl Pts',(85.9656683713897,1076.344570484,468.993679184451));
#116319=CARTESIAN_POINT('Ctrl Pts',(85.9265785304812,1076.34743421304,468.972748761436));
#116320=CARTESIAN_POINT('Ctrl Pts',(85.8149132408429,1076.35601217159,468.898021572604));
#116321=CARTESIAN_POINT('Ctrl Pts',(85.7507762389027,1076.36151517799,468.833394967447));
#116322=CARTESIAN_POINT('Ctrl Pts',(85.6518576691523,1076.37138378073,468.683054671894));
#116323=CARTESIAN_POINT('Ctrl Pts',(85.617934073741,1076.37565746368,468.598922112967));
#116324=CARTESIAN_POINT('Ctrl Pts',(85.5850142199041,1076.38245893128,468.422331719813));
#116325=CARTESIAN_POINT('Ctrl Pts',(85.586316150721,1076.38492157503,468.331651468764));
#116326=CARTESIAN_POINT('Ctrl Pts',(85.6243420134699,1076.38773247282,468.156037181576));
#116327=CARTESIAN_POINT('Ctrl Pts',(85.660695250463,1076.38805223879,468.07288106433));
#116328=CARTESIAN_POINT('Ctrl Pts',(85.7637996490437,1076.3864893365,467.925692998336));
#116329=CARTESIAN_POINT('Ctrl Pts',(85.8294991820277,1076.3846226682,467.863144660363));
#116330=CARTESIAN_POINT('Ctrl Pts',(85.9814878905492,1076.37889956016,467.767410140476));
#116331=CARTESIAN_POINT('Ctrl Pts',(86.0662529747926,1076.37509888885,467.735194004088));
#116332=CARTESIAN_POINT('Ctrl Pts',(86.1913820877741,1076.36867438578,467.714410473312));
#116333=CARTESIAN_POINT('Ctrl Pts',(86.2283981852657,1076.36667970469,467.711358222431));
#116334=CARTESIAN_POINT('Ctrl Pts',(86.2654713137633,1076.36458696229,467.711358222431));
#116335=CARTESIAN_POINT('',(86.2654713137628,1082.7251047501,467.711358222431));
#116336=CARTESIAN_POINT('',(86.2654713137628,1067.7251047501,467.711358222431));
#116337=CARTESIAN_POINT('Origin',(86.2654713137628,1082.7251047501,468.386802343567));
#116338=CARTESIAN_POINT('Ctrl Pts',(86.2654713137633,1076.36458696229,467.711358222431));
#116339=CARTESIAN_POINT('Ctrl Pts',(86.2655409522252,1076.36458303127,467.711358222431));
#116340=CARTESIAN_POINT('Ctrl Pts',(86.2656105908878,1076.36457909989,467.711358233502));
#116341=CARTESIAN_POINT('Ctrl Pts',(86.2656802297497,1076.36457516817,467.711358255042));
#116342=CARTESIAN_POINT('Ctrl Pts',(86.355911849862,1076.35948081317,467.711386163862));
#116343=CARTESIAN_POINT('Ctrl Pts',(86.4452075118274,1076.3538758243,467.729494157835));
#116344=CARTESIAN_POINT('Ctrl Pts',(86.5694496717781,1076.34520358804,467.781973253651));
#116345=CARTESIAN_POINT('Ctrl Pts',(86.6087819724189,1076.34230438781,467.803399558533));
#116346=CARTESIAN_POINT('Ctrl Pts',(86.7190276781068,1076.33369870382,467.878490567791));
#116347=CARTESIAN_POINT('Ctrl Pts',(86.7818100803589,1076.32812258751,467.942398193927));
#116348=CARTESIAN_POINT('Ctrl Pts',(86.8790362657067,1076.31794553537,468.090789963433));
#116349=CARTESIAN_POINT('Ctrl Pts',(86.9125709066619,1076.3134428523,468.173824515392));
#116350=CARTESIAN_POINT('Ctrl Pts',(86.9455813375285,1076.30618997006,468.347959352503));
#116351=CARTESIAN_POINT('Ctrl Pts',(86.9448195947062,1076.30350728791,468.437345199056));
#116352=CARTESIAN_POINT('Ctrl Pts',(86.9088741993592,1076.30038067367,468.610537551847));
#116353=CARTESIAN_POINT('Ctrl Pts',(86.8741385265952,1076.29996176381,468.69266301623));
#116354=CARTESIAN_POINT('Ctrl Pts',(86.7750897341507,1076.30146354208,468.838791458384));
#116355=CARTESIAN_POINT('Ctrl Pts',(86.7117868827548,1076.3033659806,468.901389393473));
#116356=CARTESIAN_POINT('Ctrl Pts',(86.56467718958,1076.30922539268,468.998757270787));
#116357=CARTESIAN_POINT('Ctrl Pts',(86.4822796861326,1076.3131263705,469.0325537748));
#116358=CARTESIAN_POINT('Ctrl Pts',(86.3527307934431,1076.32004288636,469.058019934114));
#116359=CARTESIAN_POINT('Ctrl Pts',(86.3090971729148,1076.32249549835,469.062246464703));
#116360=CARTESIAN_POINT('Ctrl Pts',(86.2654713137628,1076.32506388483,469.062246464703));
#116361=CARTESIAN_POINT('Origin',(87.6738908373847,1067.7251047501,482.164850509085));
#116362=CARTESIAN_POINT('',(87.6738908373846,1077.72740193357,481.066019373093));
#116363=CARTESIAN_POINT('Ctrl Pts',(87.6740206312035,1077.60297233385,483.263681637412));
#116364=CARTESIAN_POINT('Ctrl Pts',(87.8111078912392,1077.59090326144,483.263665444679));
#116365=CARTESIAN_POINT('Ctrl Pts',(87.947120297585,1077.58034241541,483.237995402536));
#116366=CARTESIAN_POINT('Ctrl Pts',(88.2018528738531,1077.56352493692,483.138120241511));
#116367=CARTESIAN_POINT('Ctrl Pts',(88.3184574072474,1077.5573852086,483.065176719914));
#116368=CARTESIAN_POINT('Ctrl Pts',(88.4570329518924,1077.55249541496,482.937395245085));
#116369=CARTESIAN_POINT('Ctrl Pts',(88.4927347895459,1077.55152977756,482.899447681179));
#116370=CARTESIAN_POINT('Ctrl Pts',(88.5385563920844,1077.55073133453,482.8432329801));
#116371=CARTESIAN_POINT('Ctrl Pts',(88.5510499554212,1077.55056682287,482.826999449908));
#116372=CARTESIAN_POINT('Ctrl Pts',(88.572016367431,1077.55038679093,482.798121078688));
#116373=CARTESIAN_POINT('Ctrl Pts',(88.5806936239008,1077.55034382916,482.785632108351));
#116374=CARTESIAN_POINT('Ctrl Pts',(88.5982462673749,1077.55032467976,482.759215300122));
#116375=CARTESIAN_POINT('Ctrl Pts',(88.6070724459055,1077.55035454002,482.745259456535));
#116376=CARTESIAN_POINT('Ctrl Pts',(88.6271168118163,1077.55051865362,482.711925668892));
#116377=CARTESIAN_POINT('Ctrl Pts',(88.638063627853,1077.55068623542,482.692393653871));
#116378=CARTESIAN_POINT('Ctrl Pts',(88.6715312240695,1077.55146427346,482.628152446531));
#116379=CARTESIAN_POINT('Ctrl Pts',(88.6915935803461,1077.5523652021,482.582241053861));
#116380=CARTESIAN_POINT('Ctrl Pts',(88.7575650094331,1077.55728247949,482.397915688518));
#116381=CARTESIAN_POINT('Ctrl Pts',(88.7788497727581,1077.56391333966,482.252414060837));
#116382=CARTESIAN_POINT('Ctrl Pts',(88.7649338993396,1077.58057500221,481.98795427312));
#116383=CARTESIAN_POINT('Ctrl Pts',(88.7393040393277,1077.58966491729,481.870717581574));
#116384=CARTESIAN_POINT('Ctrl Pts',(88.6475136601557,1077.61115073085,481.639123730004));
#116385=CARTESIAN_POINT('Ctrl Pts',(88.578579094557,1077.62360428328,481.527806123344));
#116386=CARTESIAN_POINT('Ctrl Pts',(88.3985409779626,1077.65076097294,481.327081251066));
#116387=CARTESIAN_POINT('Ctrl Pts',(88.2861888347545,1077.66532303483,481.241778560504));
#116388=CARTESIAN_POINT('Ctrl Pts',(88.0303906645026,1077.69441375866,481.115314135174));
#116389=CARTESIAN_POINT('Ctrl Pts',(87.8882923742511,1077.70863879979,481.077328391473));
#116390=CARTESIAN_POINT('Ctrl Pts',(87.6032966241837,1077.73374848996,481.05941248711));
#116391=CARTESIAN_POINT('Ctrl Pts',(87.4632323965882,1077.74452188966,481.077343357942));
#116392=CARTESIAN_POINT('Ctrl Pts',(87.2081666536232,1077.76124407805,481.161338661643));
#116393=CARTESIAN_POINT('Ctrl Pts',(87.0940421833216,1077.76738954126,481.22264216562));
#116394=CARTESIAN_POINT('Ctrl Pts',(86.9373214824395,1077.77366309305,481.346352945659));
#116395=CARTESIAN_POINT('Ctrl Pts',(86.885966737377,1077.77523806423,481.39566106034));
#116396=CARTESIAN_POINT('Ctrl Pts',(86.8223721562136,1077.77647482148,481.469827931667));
#116397=CARTESIAN_POINT('Ctrl Pts',(86.8057621118243,1077.77671668394,481.490689508232));
#116398=CARTESIAN_POINT('Ctrl Pts',(86.7796539289241,1077.77695716748,481.526047486838));
#116399=CARTESIAN_POINT('Ctrl Pts',(86.7697109074471,1077.77701135261,481.540200517127));
#116400=CARTESIAN_POINT('Ctrl Pts',(86.7510753823337,1077.77703794793,481.568104417005));
#116401=CARTESIAN_POINT('Ctrl Pts',(86.7423460381145,1077.77701505015,481.581825170085));
#116402=CARTESIAN_POINT('Ctrl Pts',(86.7227395151829,1077.77687846258,481.614207800903));
#116403=CARTESIAN_POINT('Ctrl Pts',(86.7121018345921,1077.77673747912,481.633006445475));
#116404=CARTESIAN_POINT('Ctrl Pts',(86.6803193986995,1077.77609440414,481.693247465911));
#116405=CARTESIAN_POINT('Ctrl Pts',(86.661250042485,1077.77536405011,481.735721841062));
#116406=CARTESIAN_POINT('Ctrl Pts',(86.5937730347837,1077.77115622372,481.915791865297));
#116407=CARTESIAN_POINT('Ctrl Pts',(86.5703289296778,1077.76518874474,482.061035824494));
#116408=CARTESIAN_POINT('Ctrl Pts',(86.580366437141,1077.74984985467,482.325527842935));
#116409=CARTESIAN_POINT('Ctrl Pts',(86.6041948654783,1077.74139736497,482.442911986737));
#116410=CARTESIAN_POINT('Ctrl Pts',(86.6923952079399,1077.72107857569,482.675748734811));
#116411=CARTESIAN_POINT('Ctrl Pts',(86.759674563606,1077.70912391434,482.788156688546));
#116412=CARTESIAN_POINT('Ctrl Pts',(86.9369334168585,1077.68257735879,482.991871882107));
#116413=CARTESIAN_POINT('Ctrl Pts',(87.0482874353572,1077.66808642387,483.079002105188));
#116414=CARTESIAN_POINT('Ctrl Pts',(87.2468622285877,1077.64510456924,483.180709496343));
#116415=CARTESIAN_POINT('Ctrl Pts',(87.3248255496704,1077.6366457401,483.210069231924));
#116416=CARTESIAN_POINT('Ctrl Pts',(87.4931599888644,1077.61951268012,483.252491707867));
#116417=CARTESIAN_POINT('Ctrl Pts',(87.5833947489484,1077.61095097705,483.263692342132));
#116418=CARTESIAN_POINT('Ctrl Pts',(87.6740206312035,1077.60297233385,483.263681637412));
#116419=CARTESIAN_POINT('',(87.6738908373588,1075.71704703142,481.066019373093));
#116420=CARTESIAN_POINT('',(87.6738908373847,1067.7251047501,481.066019373093));
#116421=CARTESIAN_POINT('Ctrl Pts',(87.6734764141951,1075.59152636934,483.263681566928));
#116422=CARTESIAN_POINT('Ctrl Pts',(87.5292769610456,1075.60434077903,483.263627182228));
#116423=CARTESIAN_POINT('Ctrl Pts',(87.3865888632646,1075.61859675302,483.235190481196));
#116424=CARTESIAN_POINT('Ctrl Pts',(87.1181456506469,1075.64852695256,483.124041830118));
#116425=CARTESIAN_POINT('Ctrl Pts',(86.9953185741151,1075.66393157655,483.041462726015));
#116426=CARTESIAN_POINT('Ctrl Pts',(86.7900265506239,1075.69343560738,482.833719639797));
#116427=CARTESIAN_POINT('Ctrl Pts',(86.7092408291913,1075.70726261736,482.710851473547));
#116428=CARTESIAN_POINT('Ctrl Pts',(86.6003467446628,1075.73162894803,482.440728071573));
#116429=CARTESIAN_POINT('Ctrl Pts',(86.5732339670936,1075.74193644529,482.296159388352));
#116430=CARTESIAN_POINT('Ctrl Pts',(86.5770822421847,1075.75775246956,482.004127373511));
#116431=CARTESIAN_POINT('Ctrl Pts',(86.6081899068073,1075.76308729527,481.859634643593));
#116432=CARTESIAN_POINT('Ctrl Pts',(86.7240214239792,1075.76797693463,481.594163314984));
#116433=CARTESIAN_POINT('Ctrl Pts',(86.8063947943622,1075.76760933368,481.475370492346));
#116434=CARTESIAN_POINT('Ctrl Pts',(87.0123398616821,1075.76133151365,481.275807533555));
#116435=CARTESIAN_POINT('Ctrl Pts',(87.1339717779872,1075.75546724528,481.19713241487));
#116436=CARTESIAN_POINT('Ctrl Pts',(87.4025778338071,1075.73874752703,481.090112345591));
#116437=CARTESIAN_POINT('Ctrl Pts',(87.5472218895445,1075.7279777464,481.063694070379));
#116438=CARTESIAN_POINT('Ctrl Pts',(87.8384255124702,1075.7028704515,481.068670891156));
#116439=CARTESIAN_POINT('Ctrl Pts',(87.982128630667,1075.68876933436,481.10013883438));
#116440=CARTESIAN_POINT('Ctrl Pts',(88.1808335292629,1075.66663079743,481.187333292501));
#116441=CARTESIAN_POINT('Ctrl Pts',(88.2432738679707,1075.65921506883,481.222337088777));
#116442=CARTESIAN_POINT('Ctrl Pts',(88.4227006748425,1075.63643163934,481.347296047487));
#116443=CARTESIAN_POINT('Ctrl Pts',(88.5254396337985,1075.62120195041,481.454914625536));
#116444=CARTESIAN_POINT('Ctrl Pts',(88.68086350819,1075.5931267396,481.701915668365));
#116445=CARTESIAN_POINT('Ctrl Pts',(88.7330142254566,1075.58050893989,481.838294430055));
#116446=CARTESIAN_POINT('Ctrl Pts',(88.7813084100526,1075.55948538804,482.122868329802));
#116447=CARTESIAN_POINT('Ctrl Pts',(88.777306778482,1075.55126245121,482.268226562851));
#116448=CARTESIAN_POINT('Ctrl Pts',(88.7134875328229,1075.54043862233,482.548523774093));
#116449=CARTESIAN_POINT('Ctrl Pts',(88.6546335203854,1075.53791396469,482.680736199129));
#116450=CARTESIAN_POINT('Ctrl Pts',(88.4895906495717,1075.53894046124,482.914869217121));
#116451=CARTESIAN_POINT('Ctrl Pts',(88.3851680557,1075.54246634591,483.014521711206));
#116452=CARTESIAN_POINT('Ctrl Pts',(88.1438160023445,1075.55509807103,483.168414464634));
#116453=CARTESIAN_POINT('Ctrl Pts',(88.009185497361,1075.56409226403,483.221007869021));
#116454=CARTESIAN_POINT('Ctrl Pts',(87.8040425953351,1075.58024751605,483.257904290828));
#116455=CARTESIAN_POINT('Ctrl Pts',(87.7388081660356,1075.58572060645,483.263706206742));
#116456=CARTESIAN_POINT('Ctrl Pts',(87.6734764141951,1075.59152636934,483.263681566928));
#116457=CARTESIAN_POINT('Origin',(87.6738908373847,1067.7251047501,482.164850509085));
#116458=CARTESIAN_POINT('',(87.6738908373847,1075.62676689012,482.663681645078));
#116459=CARTESIAN_POINT('',(87.6738908373844,1075.68376086233,481.666019373093));
#116460=CARTESIAN_POINT('Ctrl Pts',(87.6738908373847,1075.62676689012,482.663681645078));
#116461=CARTESIAN_POINT('Ctrl Pts',(87.6405437266238,1075.62969674438,482.663681645078));
#116462=CARTESIAN_POINT('Ctrl Pts',(87.6072155162424,1075.63281359472,482.660337682329));
#116463=CARTESIAN_POINT('Ctrl Pts',(87.5090710985346,1075.6425588954,482.640364150143));
#116464=CARTESIAN_POINT('Ctrl Pts',(87.4470775639424,1075.64947758236,482.614104143471));
#116465=CARTESIAN_POINT('Ctrl Pts',(87.3373126205476,1075.66331998747,482.538955909657));
#116466=CARTESIAN_POINT('Ctrl Pts',(87.2905424987636,1075.67011069185,482.490874696734));
#116467=CARTESIAN_POINT('Ctrl Pts',(87.2186324786873,1075.68265728098,482.379260249585));
#116468=CARTESIAN_POINT('Ctrl Pts',(87.1941545739213,1075.68829322328,482.316842132766));
#116469=CARTESIAN_POINT('Ctrl Pts',(87.1710842150568,1075.6976622135,482.185889203247));
#116470=CARTESIAN_POINT('Ctrl Pts',(87.1727519968497,1075.70129929393,482.118670489896));
#116471=CARTESIAN_POINT('Ctrl Pts',(87.2020814466865,1075.7059997038,481.99033977916));
#116472=CARTESIAN_POINT('Ctrl Pts',(87.2288175142528,1075.70707762621,481.93038736364));
#116473=CARTESIAN_POINT('Ctrl Pts',(87.3038208703414,1075.70662936817,481.824099411465));
#116474=CARTESIAN_POINT('Ctrl Pts',(87.3513394876768,1075.7051076779,481.778823797502));
#116475=CARTESIAN_POINT('Ctrl Pts',(87.4612261556118,1075.69962458665,481.708930741842));
#116476=CARTESIAN_POINT('Ctrl Pts',(87.5225600535927,1075.69570776398,481.685087421994));
#116477=CARTESIAN_POINT('Ctrl Pts',(87.6154826379312,1075.68864767134,481.668587802623));
#116478=CARTESIAN_POINT('Ctrl Pts',(87.6446651300579,1075.68628043382,481.666019373093));
#116479=CARTESIAN_POINT('Ctrl Pts',(87.6738908373842,1075.68376086233,481.666019373093));
#116480=CARTESIAN_POINT('',(87.6738908373847,1082.7251047501,481.666019373093));
#116481=CARTESIAN_POINT('',(87.6738908373847,1067.7251047501,481.666019373093));
#116482=CARTESIAN_POINT('Origin',(87.6738908373847,1082.7251047501,482.164850509085));
#116483=CARTESIAN_POINT('Ctrl Pts',(87.6738908373842,1075.68376086233,481.666019373093));
#116484=CARTESIAN_POINT('Ctrl Pts',(87.6738972500494,1075.68376030949,481.666019373093));
#116485=CARTESIAN_POINT('Ctrl Pts',(87.6739036627171,1075.68375975665,481.666019373132));
#116486=CARTESIAN_POINT('Ctrl Pts',(87.6739100753865,1075.68375920379,481.66601937338));
#116487=CARTESIAN_POINT('Ctrl Pts',(87.7403307301844,1075.67803287809,481.666021934973));
#116488=CARTESIAN_POINT('Ctrl Pts',(87.8060356353594,1075.67160013665,481.67928947701));
#116489=CARTESIAN_POINT('Ctrl Pts',(87.8971153636982,1075.66151731301,481.717572405829));
#116490=CARTESIAN_POINT('Ctrl Pts',(87.9257468068423,1075.6581462725,481.733046125472));
#116491=CARTESIAN_POINT('Ctrl Pts',(88.0079443108267,1075.64782497327,481.788441285301));
#116492=CARTESIAN_POINT('Ctrl Pts',(88.0552181071588,1075.64094345281,481.836411863289));
#116493=CARTESIAN_POINT('Ctrl Pts',(88.1278106129164,1075.62818139214,481.947676929813));
#116494=CARTESIAN_POINT('Ctrl Pts',(88.1526103480024,1075.62241655307,482.009764891465));
#116495=CARTESIAN_POINT('Ctrl Pts',(88.1763173761705,1075.61284437028,482.139150533971));
#116496=CARTESIAN_POINT('Ctrl Pts',(88.1753770175085,1075.60910239877,482.205101727012));
#116497=CARTESIAN_POINT('Ctrl Pts',(88.1481307969692,1075.60410850654,482.332658491556));
#116498=CARTESIAN_POINT('Ctrl Pts',(88.1222289247291,1075.60289338895,482.393021430533));
#116499=CARTESIAN_POINT('Ctrl Pts',(88.0487332535141,1075.60316451165,482.500331856297));
#116500=CARTESIAN_POINT('Ctrl Pts',(88.0019108728425,1075.60464340461,482.546230003847));
#116501=CARTESIAN_POINT('Ctrl Pts',(87.8931985020239,1075.61011317454,482.617594768251));
#116502=CARTESIAN_POINT('Ctrl Pts',(87.8323409444093,1075.6140569638,482.642292553746));
#116503=CARTESIAN_POINT('Ctrl Pts',(87.7372504496691,1075.62137033106,482.660665506466));
#116504=CARTESIAN_POINT('Ctrl Pts',(87.7055621192307,1075.62398427304,482.663681645078));
#116505=CARTESIAN_POINT('Ctrl Pts',(87.6738908373847,1075.62676689012,482.663681645078));
#116506=CARTESIAN_POINT('Origin',(86.2232976813476,1067.7251047501,496.076346996727));
#116507=CARTESIAN_POINT('',(86.2232976813475,1076.9124877279,494.985806247999));
#116508=CARTESIAN_POINT('Ctrl Pts',(86.2234201885755,1076.72559507709,497.166887738574));
#116509=CARTESIAN_POINT('Ctrl Pts',(86.3524097961115,1076.71205555844,497.166873248369));
#116510=CARTESIAN_POINT('Ctrl Pts',(86.480576174896,1076.70055077558,497.143973457267));
#116511=CARTESIAN_POINT('Ctrl Pts',(86.7226977502226,1076.68283926357,497.054338875221));
#116512=CARTESIAN_POINT('Ctrl Pts',(86.8347360052163,1076.67675512922,496.988530372314));
#116513=CARTESIAN_POINT('Ctrl Pts',(86.9563728152243,1076.67302111874,496.884336703862));
#116514=CARTESIAN_POINT('Ctrl Pts',(86.9791203061111,1076.67247634535,496.863099231561));
#116515=CARTESIAN_POINT('Ctrl Pts',(87.0150778334672,1076.67187843183,496.826527300309));
#116516=CARTESIAN_POINT('Ctrl Pts',(87.0288231866282,1076.67171992683,496.811748253903));
#116517=CARTESIAN_POINT('Ctrl Pts',(87.0527719620715,1076.67157337985,496.784520813728));
#116518=CARTESIAN_POINT('Ctrl Pts',(87.0631246265751,1076.67155727495,496.772212245553));
#116519=CARTESIAN_POINT('Ctrl Pts',(87.0844921179883,1076.67162681908,496.745636138793));
#116520=CARTESIAN_POINT('Ctrl Pts',(87.0954329115812,1076.67172494994,496.731315646235));
#116521=CARTESIAN_POINT('Ctrl Pts',(87.1235095640396,1076.67214795092,496.69261431479));
#116522=CARTESIAN_POINT('Ctrl Pts',(87.1400083661517,1076.67257890471,496.667792751873));
#116523=CARTESIAN_POINT('Ctrl Pts',(87.2083308298922,1076.67521735423,496.555265770314));
#116524=CARTESIAN_POINT('Ctrl Pts',(87.2486980622296,1076.67918721935,496.461287481939));
#116525=CARTESIAN_POINT('Ctrl Pts',(87.3041125094595,1076.69113009959,496.257998890933));
#116526=CARTESIAN_POINT('Ctrl Pts',(87.3168160464308,1076.69929813708,496.149273692147));
#116527=CARTESIAN_POINT('Ctrl Pts',(87.3092617857711,1076.72018567046,495.918906240303));
#116528=CARTESIAN_POINT('Ctrl Pts',(87.2849248909177,1076.73318443667,495.798910476036));
#116529=CARTESIAN_POINT('Ctrl Pts',(87.1940481680738,1076.76321722936,495.562156814412));
#116530=CARTESIAN_POINT('Ctrl Pts',(87.1246914887283,1076.78026547521,495.448512857642));
#116531=CARTESIAN_POINT('Ctrl Pts',(86.9420708702739,1076.81680859389,495.243947432705));
#116532=CARTESIAN_POINT('Ctrl Pts',(86.8274301421062,1076.83606120584,495.157344153586));
#116533=CARTESIAN_POINT('Ctrl Pts',(86.5699757981875,1076.87316869743,495.032423992116));
#116534=CARTESIAN_POINT('Ctrl Pts',(86.4292727160451,1076.89066379218,494.995771917294));
#116535=CARTESIAN_POINT('Ctrl Pts',(86.1520096037281,1076.92024691669,494.979977090931));
#116536=CARTESIAN_POINT('Ctrl Pts',(86.0182260605291,1076.9323936938,494.996919913663));
#116537=CARTESIAN_POINT('Ctrl Pts',(85.754889645979,1076.95197768784,495.081258135025));
#116538=CARTESIAN_POINT('Ctrl Pts',(85.6287943502149,1076.95886674519,495.151003283154));
#116539=CARTESIAN_POINT('Ctrl Pts',(85.4948783411836,1076.96291995805,495.264106667049));
#116540=CARTESIAN_POINT('Ctrl Pts',(85.4710646908169,1076.96348255808,495.286109662743));
#116541=CARTESIAN_POINT('Ctrl Pts',(85.4338410843614,1076.96409366395,495.32371313831));
#116542=CARTESIAN_POINT('Ctrl Pts',(85.4198312838338,1076.96425497732,495.338687696573));
#116543=CARTESIAN_POINT('Ctrl Pts',(85.3956531535167,1076.96440748111,495.366037406025));
#116544=CARTESIAN_POINT('Ctrl Pts',(85.3853198319258,1076.96442822542,495.378257956122));
#116545=CARTESIAN_POINT('Ctrl Pts',(85.3642047971045,1076.96437496726,495.404374023749));
#116546=CARTESIAN_POINT('Ctrl Pts',(85.3534828868134,1076.96429141355,495.4183116884));
#116547=CARTESIAN_POINT('Ctrl Pts',(85.3263965849636,1076.96392829633,495.45534115173));
#116548=CARTESIAN_POINT('Ctrl Pts',(85.3105867106407,1076.96356046012,495.478820164385));
#116549=CARTESIAN_POINT('Ctrl Pts',(85.2481877839852,1076.9614176983,495.579752102493));
#116550=CARTESIAN_POINT('Ctrl Pts',(85.2104302273405,1076.95833555419,495.662187103763));
#116551=CARTESIAN_POINT('Ctrl Pts',(85.1510913618141,1076.94858126176,495.850301666348));
#116552=CARTESIAN_POINT('Ctrl Pts',(85.1341308980016,1076.94140598426,495.956389671081));
#116553=CARTESIAN_POINT('Ctrl Pts',(85.1313766008971,1076.92258946607,496.183610851459));
#116554=CARTESIAN_POINT('Ctrl Pts',(85.1498936846263,1076.91062344118,496.303330037062));
#116555=CARTESIAN_POINT('Ctrl Pts',(85.2285475665924,1076.88239890454,496.542169211195));
#116556=CARTESIAN_POINT('Ctrl Pts',(85.2917526328625,1076.86606951276,496.658298576247));
#116557=CARTESIAN_POINT('Ctrl Pts',(85.4627335065793,1076.83037150634,496.870620253821));
#116558=CARTESIAN_POINT('Ctrl Pts',(85.5721659738896,1076.811182402,496.962545314751));
#116559=CARTESIAN_POINT('Ctrl Pts',(85.7716424590892,1076.78098187998,497.07270832065));
#116560=CARTESIAN_POINT('Ctrl Pts',(85.8519245211287,1076.76980240617,497.105340155335));
#116561=CARTESIAN_POINT('Ctrl Pts',(86.0290587067681,1076.74710795817,497.153847856076));
#116562=CARTESIAN_POINT('Ctrl Pts',(86.1259690214058,1076.7358241329,497.16689868587));
#116563=CARTESIAN_POINT('Ctrl Pts',(86.2234201885755,1076.72559507709,497.166887738574));
#116564=CARTESIAN_POINT('',(86.223297681327,1074.89499160754,494.985806247999));
#116565=CARTESIAN_POINT('',(86.2232976813476,1067.7251047501,494.985806247999));
#116566=CARTESIAN_POINT('Ctrl Pts',(86.2233659408369,1074.70655738266,497.166887743319));
#116567=CARTESIAN_POINT('Ctrl Pts',(86.0803109173772,1074.72169708915,497.166896697467));
#116568=CARTESIAN_POINT('Ctrl Pts',(85.938853039836,1074.739081694,497.138761309409));
#116569=CARTESIAN_POINT('Ctrl Pts',(85.7406870749057,1074.76700945455,497.056914296415));
#116570=CARTESIAN_POINT('Ctrl Pts',(85.6772676320875,1074.77659254706,497.023062448602));
#116571=CARTESIAN_POINT('Ctrl Pts',(85.5582047487984,1074.7959229432,496.943549312242));
#116572=CARTESIAN_POINT('Ctrl Pts',(85.5028064575396,1074.80562619512,496.898102180657));
#116573=CARTESIAN_POINT('Ctrl Pts',(85.3496454429075,1074.83475784732,496.744974796333));
#116574=CARTESIAN_POINT('Ctrl Pts',(85.2684330580968,1074.85363670812,496.62283397562));
#116575=CARTESIAN_POINT('Ctrl Pts',(85.1589809956636,1074.8878324657,496.354495851551));
#116576=CARTESIAN_POINT('Ctrl Pts',(85.1314496167889,1074.90284549871,496.211037453975));
#116577=CARTESIAN_POINT('Ctrl Pts',(85.1341568903704,1074.92710203794,495.921551916974));
#116578=CARTESIAN_POINT('Ctrl Pts',(85.164257561941,1074.93611353415,495.778461490953));
#116579=CARTESIAN_POINT('Ctrl Pts',(85.27756399223,1074.94679051999,495.515157651623));
#116580=CARTESIAN_POINT('Ctrl Pts',(85.358395700729,1074.94851346881,495.397146356174));
#116581=CARTESIAN_POINT('Ctrl Pts',(85.5608242107753,1074.94466507112,495.198550289736));
#116582=CARTESIAN_POINT('Ctrl Pts',(85.6803908911938,1074.93912728222,495.120010733015));
#116583=CARTESIAN_POINT('Ctrl Pts',(85.9456637895418,1074.9212164551,495.011831856432));
#116584=CARTESIAN_POINT('Ctrl Pts',(86.0891610405896,1074.90887126502,494.984492764252));
#116585=CARTESIAN_POINT('Ctrl Pts',(86.37863716269,1074.87892711957,494.987222700849));
#116586=CARTESIAN_POINT('Ctrl Pts',(86.5217505346063,1074.86160048812,495.017512633713));
#116587=CARTESIAN_POINT('Ctrl Pts',(86.7198448431444,1074.83377040269,495.102815010389));
#116588=CARTESIAN_POINT('Ctrl Pts',(86.7821549224923,1074.8243469137,495.137201058864));
#116589=CARTESIAN_POINT('Ctrl Pts',(86.8994061884456,1074.80520795178,495.217723154351));
#116590=CARTESIAN_POINT('Ctrl Pts',(86.9540537293406,1074.79553430232,495.26372613206));
#116591=CARTESIAN_POINT('Ctrl Pts',(87.1062621169359,1074.76611453062,495.419712469126));
#116592=CARTESIAN_POINT('Ctrl Pts',(87.1865717931367,1074.74682286749,495.544391033771));
#116593=CARTESIAN_POINT('Ctrl Pts',(87.2917921724487,1074.71205820369,495.815179799298));
#116594=CARTESIAN_POINT('Ctrl Pts',(87.3169440053454,1074.6968373674,495.958177480026));
#116595=CARTESIAN_POINT('Ctrl Pts',(87.3101560755106,1074.67234277346,496.244694824896));
#116596=CARTESIAN_POINT('Ctrl Pts',(87.2788618340179,1074.66325286937,496.385379091055));
#116597=CARTESIAN_POINT('Ctrl Pts',(87.1640524130299,1074.65247828509,496.645852898545));
#116598=CARTESIAN_POINT('Ctrl Pts',(87.0821614426303,1074.65083964695,496.763174927283));
#116599=CARTESIAN_POINT('Ctrl Pts',(86.8782047774325,1074.65521976434,496.959746556909));
#116600=CARTESIAN_POINT('Ctrl Pts',(86.7583012027278,1074.6611775755,497.037070803745));
#116601=CARTESIAN_POINT('Ctrl Pts',(86.4984665135315,1074.67969380481,497.140652703391));
#116602=CARTESIAN_POINT('Ctrl Pts',(86.3614278650871,1074.6919461026,497.166879101701));
#116603=CARTESIAN_POINT('Ctrl Pts',(86.2233659408369,1074.70655738266,497.166887743319));
#116604=CARTESIAN_POINT('Origin',(86.2232976813476,1067.7251047501,496.076346996727));
#116605=CARTESIAN_POINT('',(86.2232976813475,1074.75955377087,496.566887745455));
#116606=CARTESIAN_POINT('',(86.2232976813475,1074.84430822541,495.585806247999));
#116607=CARTESIAN_POINT('Ctrl Pts',(86.2232976813475,1074.75955377087,496.566887745455));
#116608=CARTESIAN_POINT('Ctrl Pts',(86.2226440593275,1074.75962237626,496.566887745455));
#116609=CARTESIAN_POINT('Ctrl Pts',(86.2219903858984,1074.75969109957,496.566886439075));
#116610=CARTESIAN_POINT('Ctrl Pts',(86.156936183418,1074.76654170787,496.566626372241));
#116611=CARTESIAN_POINT('Ctrl Pts',(86.0933076663028,1074.77433382017,496.553691462151));
#116612=CARTESIAN_POINT('Ctrl Pts',(86.0043705346255,1074.78685722683,496.516501857578));
#116613=CARTESIAN_POINT('Ctrl Pts',(85.9759897465591,1074.79114664136,496.50120329209));
#116614=CARTESIAN_POINT('Ctrl Pts',(85.9226764809709,1074.79981475687,496.465305525912));
#116615=CARTESIAN_POINT('Ctrl Pts',(85.8978599907607,1074.80417389155,496.444792691315));
#116616=CARTESIAN_POINT('Ctrl Pts',(85.8291081585573,1074.81730799618,496.375560257888));
#116617=CARTESIAN_POINT('Ctrl Pts',(85.7927021199992,1074.82584734057,496.320310092879));
#116618=CARTESIAN_POINT('Ctrl Pts',(85.7438543031066,1074.84134511513,496.198921929108));
#116619=CARTESIAN_POINT('Ctrl Pts',(85.7317757644832,1074.84816107792,496.134009919116));
#116620=CARTESIAN_POINT('Ctrl Pts',(85.7338479894099,1074.85908486631,496.003971718148));
#116621=CARTESIAN_POINT('Ctrl Pts',(85.7476145889624,1074.86312067503,495.940158239953));
#116622=CARTESIAN_POINT('Ctrl Pts',(85.7988303780936,1074.86790886816,495.822341948628));
#116623=CARTESIAN_POINT('Ctrl Pts',(85.8353891435477,1074.86866356488,495.769389890237));
#116624=CARTESIAN_POINT('Ctrl Pts',(85.9267488713175,1074.86684566662,495.680424992944));
#116625=CARTESIAN_POINT('Ctrl Pts',(85.9806190019375,1074.86429169331,495.645316174372));
#116626=CARTESIAN_POINT('Ctrl Pts',(86.0980899150621,1074.85622254089,495.597883000476));
#116627=CARTESIAN_POINT('Ctrl Pts',(86.1604532385391,1074.85081360277,495.585806247999));
#116628=CARTESIAN_POINT('Ctrl Pts',(86.2232976813474,1074.84430822541,495.585806247999));
#116629=CARTESIAN_POINT('',(86.2232976813476,1082.7251047501,495.585806247999));
#116630=CARTESIAN_POINT('',(86.2232976813476,1067.7251047501,495.585806247999));
#116631=CARTESIAN_POINT('Origin',(86.2232976813476,1082.7251047501,496.076346996727));
#116632=CARTESIAN_POINT('Ctrl Pts',(86.2232976813474,1074.84430822541,495.585806247999));
#116633=CARTESIAN_POINT('Ctrl Pts',(86.2233019494077,1074.8443077836,495.585806247999));
#116634=CARTESIAN_POINT('Ctrl Pts',(86.2233062174703,1074.84430734178,495.585806248042));
#116635=CARTESIAN_POINT('Ctrl Pts',(86.2233104855349,1074.84430689996,495.585806248154));
#116636=CARTESIAN_POINT('Ctrl Pts',(86.2888311471117,1074.8375243441,495.585807958388));
#116637=CARTESIAN_POINT('Ctrl Pts',(86.3535917320136,1074.82968248953,495.598934670239));
#116638=CARTESIAN_POINT('Ctrl Pts',(86.4433153117649,1074.81710255258,495.6367467866));
#116639=CARTESIAN_POINT('Ctrl Pts',(86.4715312206027,1074.8128490095,495.652041918061));
#116640=CARTESIAN_POINT('Ctrl Pts',(86.5246181303704,1074.80422349754,495.687933598277));
#116641=CARTESIAN_POINT('Ctrl Pts',(86.5493630162513,1074.79987063099,495.708460720927));
#116642=CARTESIAN_POINT('Ctrl Pts',(86.6181958536365,1074.78667374477,495.777999013993));
#116643=CARTESIAN_POINT('Ctrl Pts',(86.6546383624893,1074.77804081921,495.833618109012));
#116644=CARTESIAN_POINT('Ctrl Pts',(86.7030654206161,1074.76240822645,495.955203405332));
#116645=CARTESIAN_POINT('Ctrl Pts',(86.7149169782775,1074.75553756712,496.019854259707));
#116646=CARTESIAN_POINT('Ctrl Pts',(86.7126255587337,1074.74451778519,496.149112216989));
#116647=CARTESIAN_POINT('Ctrl Pts',(86.6989445841481,1074.74043286006,496.212433045587));
#116648=CARTESIAN_POINT('Ctrl Pts',(86.6480524086574,1074.73554231507,496.329873683035));
#116649=CARTESIAN_POINT('Ctrl Pts',(86.6115468864515,1074.73476019736,496.382875657183));
#116650=CARTESIAN_POINT('Ctrl Pts',(86.5203271726244,1074.7365981839,496.471896694175));
#116651=CARTESIAN_POINT('Ctrl Pts',(86.4665679794862,1074.73919466779,496.507032781713));
#116652=CARTESIAN_POINT('Ctrl Pts',(86.3489982345556,1074.74740833894,496.554716480634));
#116653=CARTESIAN_POINT('Ctrl Pts',(86.2863874353879,1074.7529317518,496.566887745455));
#116654=CARTESIAN_POINT('Ctrl Pts',(86.2232976813475,1074.75955377087,496.566887745455));
#116655=CARTESIAN_POINT('Origin',(88.5622696992333,1067.7251047501,437.939428532945));
#116656=CARTESIAN_POINT('',(88.5622696992515,1078.67883079978,436.461125400751));
#116657=CARTESIAN_POINT('Ctrl Pts',(88.5624504403869,1078.66748248367,439.417731654089));
#116658=CARTESIAN_POINT('Ctrl Pts',(88.757345015015,1078.66228612236,439.417707825776));
#116659=CARTESIAN_POINT('Ctrl Pts',(88.9503273060786,1078.6569937597,439.379142881179));
#116660=CARTESIAN_POINT('Ctrl Pts',(89.3025589141094,1078.64726732473,439.232555684521));
#116661=CARTESIAN_POINT('Ctrl Pts',(89.4597375327993,1078.64289971757,439.128868216047));
#116662=CARTESIAN_POINT('Ctrl Pts',(89.7209953868401,1078.6358690912,438.874527370835));
#116663=CARTESIAN_POINT('Ctrl Pts',(89.8250665607932,1078.63319830216,438.72835683181));
#116664=CARTESIAN_POINT('Ctrl Pts',(89.9360868402136,1078.63073122799,438.491667515965));
#116665=CARTESIAN_POINT('Ctrl Pts',(89.9650602475366,1078.63016532841,438.413264597878));
#116666=CARTESIAN_POINT('Ctrl Pts',(89.9963785571602,1078.62969541958,438.299823872625));
#116667=CARTESIAN_POINT('Ctrl Pts',(90.0043425517052,1078.62959797718,438.266504855865));
#116668=CARTESIAN_POINT('Ctrl Pts',(90.0152946475143,1078.6295048698,438.212441453156));
#116669=CARTESIAN_POINT('Ctrl Pts',(90.0190116220425,1078.62948435833,438.191857783571));
#116670=CARTESIAN_POINT('Ctrl Pts',(90.0257937762046,1078.62947257754,438.149134691943));
#116671=CARTESIAN_POINT('Ctrl Pts',(90.0287961599801,1078.62948340464,438.126990619487));
#116672=CARTESIAN_POINT('Ctrl Pts',(90.0346138172216,1078.62954793693,438.075307226615));
#116673=CARTESIAN_POINT('Ctrl Pts',(90.0370440215606,1078.62961451857,438.045734279213));
#116674=CARTESIAN_POINT('Ctrl Pts',(90.0418964547107,1078.62991783137,437.952310614242));
#116675=CARTESIAN_POINT('Ctrl Pts',(90.0410711413001,1078.63026201202,437.888365873144));
#116676=CARTESIAN_POINT('Ctrl Pts',(90.0208508646909,1078.63220780497,437.628662782334));
#116677=CARTESIAN_POINT('Ctrl Pts',(89.9666401589069,1078.63492363913,437.437664654653));
#116678=CARTESIAN_POINT('Ctrl Pts',(89.8034269765363,1078.64159556978,437.120572201635));
#116679=CARTESIAN_POINT('Ctrl Pts',(89.7075560654635,1078.64517893324,436.991109043046));
#116680=CARTESIAN_POINT('Ctrl Pts',(89.4681195341764,1078.65339775563,436.758298803338));
#116681=CARTESIAN_POINT('Ctrl Pts',(89.3229983760408,1078.65802967811,436.660006815832));
#116682=CARTESIAN_POINT('Ctrl Pts',(88.9937644666912,1078.66771358045,436.513248057597));
#116683=CARTESIAN_POINT('Ctrl Pts',(88.810531607163,1078.67268076812,436.470228677978));
#116684=CARTESIAN_POINT('Ctrl Pts',(88.4289595182711,1078.68215611944,436.454244500458));
#116685=CARTESIAN_POINT('Ctrl Pts',(88.2340670620951,1078.6865383815,436.484837421534));
#116686=CARTESIAN_POINT('Ctrl Pts',(87.8733545189762,1078.69393353298,436.617865550892));
#116687=CARTESIAN_POINT('Ctrl Pts',(87.7101300913676,1078.69692399872,436.71672727955));
#116688=CARTESIAN_POINT('Ctrl Pts',(87.4425068272208,1078.70139236637,436.959082917338));
#116689=CARTESIAN_POINT('Ctrl Pts',(87.3361587463948,1078.70295379596,437.09586366536));
#116690=CARTESIAN_POINT('Ctrl Pts',(87.2083715890297,1078.70459376192,437.337282044604));
#116691=CARTESIAN_POINT('Ctrl Pts',(87.1703383730882,1078.70501319292,437.431345881074));
#116692=CARTESIAN_POINT('Ctrl Pts',(87.1319459917568,1078.7053363797,437.564037213949));
#116693=CARTESIAN_POINT('Ctrl Pts',(87.1230131209069,1078.70539825704,437.59989199811));
#116694=CARTESIAN_POINT('Ctrl Pts',(87.1105851978113,1078.70545965385,437.659160541457));
#116695=CARTESIAN_POINT('Ctrl Pts',(87.1062925734953,1078.70547360007,437.682390308681));
#116696=CARTESIAN_POINT('Ctrl Pts',(87.0990865422115,1078.70548123484,437.727396825959));
#116697=CARTESIAN_POINT('Ctrl Pts',(87.0960983146865,1078.70547627664,437.749155395497));
#116698=CARTESIAN_POINT('Ctrl Pts',(87.0903143381137,1078.70544484624,437.799582626489));
#116699=CARTESIAN_POINT('Ctrl Pts',(87.0878694684239,1078.70541216515,437.828282591387));
#116700=CARTESIAN_POINT('Ctrl Pts',(87.0828839198283,1078.70526441035,437.91759478844));
#116701=CARTESIAN_POINT('Ctrl Pts',(87.083233658455,1078.7050984122,437.978304538025));
#116702=CARTESIAN_POINT('Ctrl Pts',(87.1005846110692,1078.70410859516,438.235789588208));
#116703=CARTESIAN_POINT('Ctrl Pts',(87.1531793757567,1078.70266328467,438.428114147403));
#116704=CARTESIAN_POINT('Ctrl Pts',(87.3140974976532,1078.69869682965,438.747605160651));
#116705=CARTESIAN_POINT('Ctrl Pts',(87.4090274351938,1078.69644991752,438.878103900114));
#116706=CARTESIAN_POINT('Ctrl Pts',(87.6473447712769,1078.69074624572,439.113669287901));
#116707=CARTESIAN_POINT('Ctrl Pts',(87.7924536974861,1078.68723915733,439.213518635821));
#116708=CARTESIAN_POINT('Ctrl Pts',(88.0476778660629,1078.68086743532,439.329285867746));
#116709=CARTESIAN_POINT('Ctrl Pts',(88.1481322858348,1078.67831845493,439.362452438779));
#116710=CARTESIAN_POINT('Ctrl Pts',(88.3535252766991,1078.67301211949,439.406653678577));
#116711=CARTESIAN_POINT('Ctrl Pts',(88.4578420533073,1078.67027159659,439.417744443781));
#116712=CARTESIAN_POINT('Ctrl Pts',(88.5624504403869,1078.66748248367,439.417731654089));
#116713=CARTESIAN_POINT('',(88.5622696992118,1076.67818780051,436.461125400751));
#116714=CARTESIAN_POINT('',(88.5622696992333,1067.7251047501,436.461125400751));
#116715=CARTESIAN_POINT('Ctrl Pts',(88.5617352524017,1076.66672428354,439.41773156853));
#116716=CARTESIAN_POINT('Ctrl Pts',(88.3683809758935,1076.67194009027,439.41766166569));
#116717=CARTESIAN_POINT('Ctrl Pts',(88.1768972564217,1076.67695651917,439.379657888919));
#116718=CARTESIAN_POINT('Ctrl Pts',(87.8176643094205,1076.68608108643,439.231354792517));
#116719=CARTESIAN_POINT('Ctrl Pts',(87.6536988854534,1076.69009296818,439.121807155248));
#116720=CARTESIAN_POINT('Ctrl Pts',(87.3780890166092,1076.69676616586,438.845568983184));
#116721=CARTESIAN_POINT('Ctrl Pts',(87.2690504815552,1076.69937242687,438.681699088468));
#116722=CARTESIAN_POINT('Ctrl Pts',(87.1204864835168,1076.70320006966,438.320226613705));
#116723=CARTESIAN_POINT('Ctrl Pts',(87.0827691330013,1076.70438483802,438.126049449173));
#116724=CARTESIAN_POINT('Ctrl Pts',(87.0852248910072,1076.70538860172,437.733826789366));
#116725=CARTESIAN_POINT('Ctrl Pts',(87.1255605943168,1076.70519705504,437.539678770042));
#116726=CARTESIAN_POINT('Ctrl Pts',(87.2794221082317,1076.70340929647,437.179207364597));
#116727=CARTESIAN_POINT('Ctrl Pts',(87.3911426333467,1076.70183157579,437.016340666353));
#116728=CARTESIAN_POINT('Ctrl Pts',(87.6709541381621,1076.69720280529,436.744061410256));
#116729=CARTESIAN_POINT('Ctrl Pts',(87.8360887993002,1076.69419419588,436.637123174694));
#116730=CARTESIAN_POINT('Ctrl Pts',(88.1991432641097,1076.68675386757,436.493110421715));
#116731=CARTESIAN_POINT('Ctrl Pts',(88.3936214801836,1076.68238210076,436.457792522723));
#116732=CARTESIAN_POINT('Ctrl Pts',(88.6868856082326,1076.67509357414,436.463157910341));
#116733=CARTESIAN_POINT('Ctrl Pts',(88.7840415346486,1076.67256602926,436.474600731023));
#116734=CARTESIAN_POINT('Ctrl Pts',(89.0688325908674,1076.66481721658,436.537142277561));
#116735=CARTESIAN_POINT('Ctrl Pts',(89.2482781730382,1076.65946977958,436.615644168988));
#116736=CARTESIAN_POINT('Ctrl Pts',(89.5666905284698,1076.64918330829,436.837523430681));
#116737=CARTESIAN_POINT('Ctrl Pts',(89.7025484344164,1076.64435046856,436.978788202611));
#116738=CARTESIAN_POINT('Ctrl Pts',(89.9118735393716,1076.6361906598,437.305702102426));
#116739=CARTESIAN_POINT('Ctrl Pts',(89.9833289645815,1076.6329495055,437.488161197479));
#116740=CARTESIAN_POINT('Ctrl Pts',(90.0515895250753,1076.62880161083,437.869913486374));
#116741=CARTESIAN_POINT('Ctrl Pts',(90.0478755907697,1076.62793474189,438.065464302928));
#116742=CARTESIAN_POINT('Ctrl Pts',(89.9653350825308,1076.62879179068,438.443550743642));
#116743=CARTESIAN_POINT('Ctrl Pts',(89.8874864742292,1076.63050034395,438.622454655504));
#116744=CARTESIAN_POINT('Ctrl Pts',(89.6674995590258,1076.63612200071,438.939984840519));
#116745=CARTESIAN_POINT('Ctrl Pts',(89.527548801666,1076.63997328647,439.075593198019));
#116746=CARTESIAN_POINT('Ctrl Pts',(89.203370742823,1076.64901305868,439.285412825144));
#116747=CARTESIAN_POINT('Ctrl Pts',(89.022228488455,1076.65410849205,439.357566614862));
#116748=CARTESIAN_POINT('Ctrl Pts',(88.7431027765002,1076.66180103145,439.409435422911));
#116749=CARTESIAN_POINT('Ctrl Pts',(88.6525139055784,1076.6642754941,439.417764387486));
#116750=CARTESIAN_POINT('Ctrl Pts',(88.5617352524017,1076.66672428354,439.41773156853));
#116751=CARTESIAN_POINT('Origin',(88.5622696992333,1067.7251047501,437.939428532945));
#116752=CARTESIAN_POINT('',(88.5622696992333,1076.6693343871,438.817731665138));
#116753=CARTESIAN_POINT('',(88.5622696993117,1076.67614304338,437.061125400752));
#116754=CARTESIAN_POINT('Ctrl Pts',(88.5622696992333,1076.6693343871,438.817731665138));
#116755=CARTESIAN_POINT('Ctrl Pts',(88.4536517533704,1076.67220897669,438.817731665138));
#116756=CARTESIAN_POINT('Ctrl Pts',(88.3459099310249,1076.67504496281,438.797581873877));
#116757=CARTESIAN_POINT('Ctrl Pts',(88.1358308853606,1076.68054698191,438.71606497484));
#116758=CARTESIAN_POINT('Ctrl Pts',(88.0365939392436,1076.68313022806,438.652648202581));
#116759=CARTESIAN_POINT('Ctrl Pts',(87.8687859378155,1076.68755634743,438.490849384969));
#116760=CARTESIAN_POINT('Ctrl Pts',(87.8018434510697,1076.68935896266,438.394114717533));
#116761=CARTESIAN_POINT('Ctrl Pts',(87.7094694558756,1076.69206732777,438.179843760435));
#116762=CARTESIAN_POINT('Ctrl Pts',(87.6850841716801,1076.69294615635,438.064388079985));
#116763=CARTESIAN_POINT('Ctrl Pts',(87.6829222669053,1076.69373261675,437.830517802458));
#116764=CARTESIAN_POINT('Ctrl Pts',(87.7052427320025,1076.69363180558,437.714443996672));
#116765=CARTESIAN_POINT('Ctrl Pts',(87.7939562708241,1076.69244392786,437.498129167194));
#116766=CARTESIAN_POINT('Ctrl Pts',(87.8593627160175,1076.6913694884,437.400011721706));
#116767=CARTESIAN_POINT('Ctrl Pts',(88.0244931402338,1076.68828756065,437.235314081606));
#116768=CARTESIAN_POINT('Ctrl Pts',(88.1224915206422,1076.68631006592,437.170290791429));
#116769=CARTESIAN_POINT('Ctrl Pts',(88.335721505322,1076.68163482803,437.083241244989));
#116770=CARTESIAN_POINT('Ctrl Pts',(88.4484747365534,1076.67899668761,437.061125400731));
#116771=CARTESIAN_POINT('Ctrl Pts',(88.56226969939,1076.67614304338,437.061125400751));
#116772=CARTESIAN_POINT('',(88.5622696992333,1082.7251047501,437.061125400751));
#116773=CARTESIAN_POINT('',(88.5622696992333,1067.7251047501,437.061125400751));
#116774=CARTESIAN_POINT('Origin',(88.5622696992333,1082.7251047501,437.939428532945));
#116775=CARTESIAN_POINT('Ctrl Pts',(88.56226969939,1076.67614304338,437.061125400751));
#116776=CARTESIAN_POINT('Ctrl Pts',(88.5651433688951,1076.67607098017,437.061125400752));
#116777=CARTESIAN_POINT('Ctrl Pts',(88.5680177027814,1076.6759987816,437.061139504034));
#116778=CARTESIAN_POINT('Ctrl Pts',(88.6288907643527,1076.67446722831,437.06173716517));
#116779=CARTESIAN_POINT('Ctrl Pts',(88.6866892952071,1076.67296430677,437.068050272989));
#116780=CARTESIAN_POINT('Ctrl Pts',(88.8561391256731,1076.6684109272,437.103771672063));
#116781=CARTESIAN_POINT('Ctrl Pts',(88.9630724197748,1076.66533696018,437.149466870854));
#116782=CARTESIAN_POINT('Ctrl Pts',(89.1532244248137,1076.65950966314,437.279534086036));
#116783=CARTESIAN_POINT('Ctrl Pts',(89.2345977229757,1076.65681496627,437.362656120586));
#116784=CARTESIAN_POINT('Ctrl Pts',(89.3605927294946,1076.65228848288,437.555549579377));
#116785=CARTESIAN_POINT('Ctrl Pts',(89.4040047099736,1076.6505028898,437.663442066641));
#116786=CARTESIAN_POINT('Ctrl Pts',(89.4346526918423,1076.648845267,437.825935577347));
#116787=CARTESIAN_POINT('Ctrl Pts',(89.4397101202682,1076.6484648082,437.875936544235));
#116788=CARTESIAN_POINT('Ctrl Pts',(89.4404716297984,1076.64821331939,437.926095822328));
#116789=CARTESIAN_POINT('Ctrl Pts',(89.442217060216,1076.64763689034,438.041064218952));
#116790=CARTESIAN_POINT('Ctrl Pts',(89.4213693793535,1076.64774924074,438.155263251906));
#116791=CARTESIAN_POINT('Ctrl Pts',(89.3369086710337,1076.6493305304,438.369011200203));
#116792=CARTESIAN_POINT('Ctrl Pts',(89.2741615572938,1076.65078152744,438.466508778896));
#116793=CARTESIAN_POINT('Ctrl Pts',(89.1147209668251,1076.65475310104,438.63181621552));
#116794=CARTESIAN_POINT('Ctrl Pts',(89.019566207292,1076.65723294942,438.698032125079));
#116795=CARTESIAN_POINT('Ctrl Pts',(88.8091103257634,1076.66278330872,438.790128042062));
#116796=CARTESIAN_POINT('Ctrl Pts',(88.6958206984086,1076.66579840644,438.81508978528));
#116797=CARTESIAN_POINT('Ctrl Pts',(88.574718553124,1076.66900488633,438.817665528259));
#116798=CARTESIAN_POINT('Ctrl Pts',(88.5684926881341,1076.66916969481,438.817731665138));
#116799=CARTESIAN_POINT('Ctrl Pts',(88.5622696992333,1076.6693343871,438.817731665138));
#116800=CARTESIAN_POINT('Origin',(93.479943233478,1067.7251047501,449.494798005067));
#116801=CARTESIAN_POINT('',(93.4799432334968,1078.36968470723,448.219353883931));
#116802=CARTESIAN_POINT('Ctrl Pts',(93.4801826298566,1078.32767378068,450.770242103737));
#116803=CARTESIAN_POINT('Ctrl Pts',(93.6475477114777,1078.31708652496,450.770210689898));
#116804=CARTESIAN_POINT('Ctrl Pts',(93.8133273471716,1078.30697943726,450.737236796184));
#116805=CARTESIAN_POINT('Ctrl Pts',(94.1110529047082,1078.2897292958,450.613914363091));
#116806=CARTESIAN_POINT('Ctrl Pts',(94.2421511453505,1078.28256593783,450.52910739579));
#116807=CARTESIAN_POINT('Ctrl Pts',(94.47314148915,1078.27107922897,450.311336576597));
#116808=CARTESIAN_POINT('Ctrl Pts',(94.5690466207419,1078.2670225275,450.178217006567));
#116809=CARTESIAN_POINT('Ctrl Pts',(94.6529474756453,1078.26462949725,449.996986510507));
#116810=CARTESIAN_POINT('Ctrl Pts',(94.6670491949256,1078.26429572532,449.962678154495));
#116811=CARTESIAN_POINT('Ctrl Pts',(94.6876349920122,1078.26393260025,449.905642734319));
#116812=CARTESIAN_POINT('Ctrl Pts',(94.695017938818,1078.26383669483,449.88326454698));
#116813=CARTESIAN_POINT('Ctrl Pts',(94.7070736130371,1078.2637464853,449.843007189547));
#116814=CARTESIAN_POINT('Ctrl Pts',(94.7119856793705,1078.26373470009,449.825206870223));
#116815=CARTESIAN_POINT('Ctrl Pts',(94.7215007826988,1078.26376851037,449.787556473735));
#116816=CARTESIAN_POINT('Ctrl Pts',(94.7260180969208,1078.26382015393,449.767690103934));
#116817=CARTESIAN_POINT('Ctrl Pts',(94.7365988617227,1078.2640440848,449.715393549379));
#116818=CARTESIAN_POINT('Ctrl Pts',(94.7418832817774,1078.26427119927,449.682821937226));
#116819=CARTESIAN_POINT('Ctrl Pts',(94.7589553049056,1078.26561079862,449.543642638043));
#116820=CARTESIAN_POINT('Ctrl Pts',(94.7585335793055,1078.26756089624,449.435996084373));
#116821=CARTESIAN_POINT('Ctrl Pts',(94.7284219549179,1078.27366930619,449.205341470702));
#116822=CARTESIAN_POINT('Ctrl Pts',(94.6939422154392,1078.27811235492,449.084100176053));
#116823=CARTESIAN_POINT('Ctrl Pts',(94.5844834156256,1078.28959207689,448.84170975938));
#116824=CARTESIAN_POINT('Ctrl Pts',(94.505828263565,1078.29679879806,448.724040549938));
#116825=CARTESIAN_POINT('Ctrl Pts',(94.3052850705498,1078.31345024192,448.510525371881));
#116826=CARTESIAN_POINT('Ctrl Pts',(94.1819070491363,1078.32289717681,448.419061114382));
#116827=CARTESIAN_POINT('Ctrl Pts',(93.8987475672184,1078.34306554176,448.279021051198));
#116828=CARTESIAN_POINT('Ctrl Pts',(93.7395370223165,1078.35364313157,448.235382198108));
#116829=CARTESIAN_POINT('Ctrl Pts',(93.4086729706007,1078.37418974403,448.210282468943));
#116830=CARTESIAN_POINT('Ctrl Pts',(93.2400015141554,1078.3839347676,448.230867165947));
#116831=CARTESIAN_POINT('Ctrl Pts',(92.9282270374595,1078.40067106426,448.333779738091));
#116832=CARTESIAN_POINT('Ctrl Pts',(92.7870323122245,1078.40763067077,448.412086778063));
#116833=CARTESIAN_POINT('Ctrl Pts',(92.5426094346535,1078.41853937265,448.615536314068));
#116834=CARTESIAN_POINT('Ctrl Pts',(92.4410186940592,1078.42243686271,448.738256576007));
#116835=CARTESIAN_POINT('Ctrl Pts',(92.3353775377774,1078.42553735098,448.928833482709));
#116836=CARTESIAN_POINT('Ctrl Pts',(92.3100600450754,1078.42614826811,448.983211849712));
#116837=CARTESIAN_POINT('Ctrl Pts',(92.2791929794852,1078.42667705712,449.063916897381));
#116838=CARTESIAN_POINT('Ctrl Pts',(92.2705014079795,1078.42679127977,449.088952966193));
#116839=CARTESIAN_POINT('Ctrl Pts',(92.2570433252745,1078.42690397541,449.132003527251));
#116840=CARTESIAN_POINT('Ctrl Pts',(92.2518801726277,1078.42692676637,449.149884769434));
#116841=CARTESIAN_POINT('Ctrl Pts',(92.2422504584826,1078.42692490095,449.186198345056));
#116842=CARTESIAN_POINT('Ctrl Pts',(92.2378000171455,1078.42689934546,449.204630150487));
#116843=CARTESIAN_POINT('Ctrl Pts',(92.2279502619266,1078.42677699351,449.249816463611));
#116844=CARTESIAN_POINT('Ctrl Pts',(92.2229956135971,1078.42665386618,449.276658109654));
#116845=CARTESIAN_POINT('Ctrl Pts',(92.2086628326856,1078.42604427424,449.371207953038));
#116846=CARTESIAN_POINT('Ctrl Pts',(92.2038678680935,1078.42529103033,449.43948895891));
#116847=CARTESIAN_POINT('Ctrl Pts',(92.2063028295234,1078.42156955022,449.677955713005));
#116848=CARTESIAN_POINT('Ctrl Pts',(92.2420651811146,1078.41701467454,449.845987096239));
#116849=CARTESIAN_POINT('Ctrl Pts',(92.3655792799109,1078.40555094395,450.130958778107));
#116850=CARTESIAN_POINT('Ctrl Pts',(92.4423770957565,1078.39926377994,450.249741709368));
#116851=CARTESIAN_POINT('Ctrl Pts',(92.639781211349,1078.38424392151,450.466503842991));
#116852=CARTESIAN_POINT('Ctrl Pts',(92.7620390281582,1078.37546379632,450.560007998539));
#116853=CARTESIAN_POINT('Ctrl Pts',(92.9872034922823,1078.35992787438,450.6754956304));
#116854=CARTESIAN_POINT('Ctrl Pts',(93.0816361975551,1078.3535620404,450.710605327249));
#116855=CARTESIAN_POINT('Ctrl Pts',(93.2777354264199,1078.34062038903,450.758186876195));
#116856=CARTESIAN_POINT('Ctrl Pts',(93.3787783042975,1078.33408846118,450.770261136972));
#116857=CARTESIAN_POINT('Ctrl Pts',(93.4801826298566,1078.32767378068,450.770242103737));
#116858=CARTESIAN_POINT('',(93.4799432334501,1076.36561958492,448.219353883931));
#116859=CARTESIAN_POINT('',(93.479943233478,1067.7251047501,448.219353883931));
#116860=CARTESIAN_POINT('Ctrl Pts',(93.4801397319905,1076.32317311768,450.770242111067));
#116861=CARTESIAN_POINT('Ctrl Pts',(93.3966391800305,1076.32851006915,450.770254975397));
#116862=CARTESIAN_POINT('Ctrl Pts',(93.3133414971078,1076.3339303567,450.762067917032));
#116863=CARTESIAN_POINT('Ctrl Pts',(93.1497499971195,1076.34475870276,450.729572381437));
#116864=CARTESIAN_POINT('Ctrl Pts',(93.0698354885403,1076.35014117197,450.705379818211));
#116865=CARTESIAN_POINT('Ctrl Pts',(92.836739106239,1076.36612940808,450.609059066668));
#116866=CARTESIAN_POINT('Ctrl Pts',(92.6949442321963,1076.37625737627,450.514159482743));
#116867=CARTESIAN_POINT('Ctrl Pts',(92.456901802598,1076.39427452854,450.274886685455));
#116868=CARTESIAN_POINT('Ctrl Pts',(92.3628568939185,1076.40199774594,450.133007941772));
#116869=CARTESIAN_POINT('Ctrl Pts',(92.2351340378411,1076.41424292262,449.820165117067));
#116870=CARTESIAN_POINT('Ctrl Pts',(92.202969309497,1076.41863513552,449.652218865655));
#116871=CARTESIAN_POINT('Ctrl Pts',(92.2061462687408,1076.42360522909,449.312901654591));
#116872=CARTESIAN_POINT('Ctrl Pts',(92.2416938301822,1076.42412210169,449.144959103998));
#116873=CARTESIAN_POINT('Ctrl Pts',(92.376375543339,1076.42117660296,448.83324001666));
#116874=CARTESIAN_POINT('Ctrl Pts',(92.4740078374944,1076.41775112604,448.692557144687));
#116875=CARTESIAN_POINT('Ctrl Pts',(92.7179325220569,1076.40727311881,448.458181072377));
#116876=CARTESIAN_POINT('Ctrl Pts',(92.8615712173566,1076.40033668268,448.366608964887));
#116877=CARTESIAN_POINT('Ctrl Pts',(93.176148830756,1076.38362615321,448.244617868714));
#116878=CARTESIAN_POINT('Ctrl Pts',(93.3440045530336,1076.37400987909,448.215452292248));
#116879=CARTESIAN_POINT('Ctrl Pts',(93.6826596272493,1076.35313032174,448.224129279082));
#116880=CARTESIAN_POINT('Ctrl Pts',(93.8501126669127,1076.34205873386,448.262460176437));
#116881=CARTESIAN_POINT('Ctrl Pts',(94.1577977508267,1076.32020256933,448.401478309504));
#116882=CARTESIAN_POINT('Ctrl Pts',(94.2954475977977,1076.30962762166,448.499905468882));
#116883=CARTESIAN_POINT('Ctrl Pts',(94.5246944317019,1076.29039063412,448.744273655185));
#116884=CARTESIAN_POINT('Ctrl Pts',(94.6141375007907,1076.28191586489,448.887805261111));
#116885=CARTESIAN_POINT('Ctrl Pts',(94.7322757779242,1076.2684440228,449.200946253375));
#116886=CARTESIAN_POINT('Ctrl Pts',(94.7599828200759,1076.26357300931,449.367436284188));
#116887=CARTESIAN_POINT('Ctrl Pts',(94.7495666775411,1076.25826497393,449.701213616718));
#116888=CARTESIAN_POINT('Ctrl Pts',(94.7117462240708,1076.25786835316,449.865224565764));
#116889=CARTESIAN_POINT('Ctrl Pts',(94.5752357038917,1076.26163815408,450.169195636705));
#116890=CARTESIAN_POINT('Ctrl Pts',(94.4779667113281,1076.26575996905,450.306213464761));
#116891=CARTESIAN_POINT('Ctrl Pts',(94.236224075899,1076.27788545298,450.535259222229));
#116892=CARTESIAN_POINT('Ctrl Pts',(94.0940336295003,1076.28577278385,450.625005130405));
#116893=CARTESIAN_POINT('Ctrl Pts',(93.7923508974505,1076.3035555458,450.74129559664));
#116894=CARTESIAN_POINT('Ctrl Pts',(93.6368948719087,1076.31315408721,450.770217960928));
#116895=CARTESIAN_POINT('Ctrl Pts',(93.4801397319905,1076.32317311768,450.770242111067));
#116896=CARTESIAN_POINT('Origin',(93.479943233478,1067.7251047501,449.494798005067));
#116897=CARTESIAN_POINT('',(93.479943233478,1076.33373423278,450.170242126204));
#116898=CARTESIAN_POINT('',(93.4799432334781,1076.35619778296,448.819353883931));
#116899=CARTESIAN_POINT('Ctrl Pts',(93.479943233478,1076.33373423278,450.170242126204));
#116900=CARTESIAN_POINT('Ctrl Pts',(93.4371754633824,1076.33643869804,450.170242126204));
#116901=CARTESIAN_POINT('Ctrl Pts',(93.3945029447023,1076.33919408693,450.166180168351));
#116902=CARTESIAN_POINT('Ctrl Pts',(93.3092123998598,1076.34481486458,450.149793282562));
#116903=CARTESIAN_POINT('Ctrl Pts',(93.2668405035828,1076.34766755124,450.137258346407));
#116904=CARTESIAN_POINT('Ctrl Pts',(93.1427944673026,1076.35620649091,450.086927080627));
#116905=CARTESIAN_POINT('Ctrl Pts',(93.0671353424771,1076.36167909722,450.036908765151));
#116906=CARTESIAN_POINT('Ctrl Pts',(92.9398637726623,1076.3715038067,449.910238678341));
#116907=CARTESIAN_POINT('Ctrl Pts',(92.8894860433503,1076.37576103081,449.834870332213));
#116908=CARTESIAN_POINT('Ctrl Pts',(92.8210536335252,1076.38253942125,449.668565823741));
#116909=CARTESIAN_POINT('Ctrl Pts',(92.8037738169076,1076.38498913436,449.57926606267));
#116910=CARTESIAN_POINT('Ctrl Pts',(92.8052559516844,1076.38773096296,449.400921098179));
#116911=CARTESIAN_POINT('Ctrl Pts',(92.8232839999973,1076.38803946154,449.313647021995));
#116912=CARTESIAN_POINT('Ctrl Pts',(92.8919407583486,1076.38652986799,449.15086205297));
#116913=CARTESIAN_POINT('Ctrl Pts',(92.9419423208957,1076.38472322065,449.076961826822));
#116914=CARTESIAN_POINT('Ctrl Pts',(93.0685981587866,1076.3791301043,448.951570441442));
#116915=CARTESIAN_POINT('Ctrl Pts',(93.144416855151,1076.37536546497,448.901745636581));
#116916=CARTESIAN_POINT('Ctrl Pts',(93.3079194127563,1076.3664986175,448.835930620374));
#116917=CARTESIAN_POINT('Ctrl Pts',(93.3935461910011,1076.36153221488,448.819353883931));
#116918=CARTESIAN_POINT('Ctrl Pts',(93.4799432334782,1076.35619778296,448.819353883931));
#116919=CARTESIAN_POINT('',(93.479943233478,1082.7251047501,448.819353883931));
#116920=CARTESIAN_POINT('',(93.479943233478,1067.7251047501,448.819353883931));
#116921=CARTESIAN_POINT('Origin',(93.479943233478,1082.7251047501,449.494798005067));
#116922=CARTESIAN_POINT('Ctrl Pts',(93.4799432334782,1076.35619778296,448.819353883931));
#116923=CARTESIAN_POINT('Ctrl Pts',(93.4799582875746,1076.35619685347,448.819353883931));
#116924=CARTESIAN_POINT('Ctrl Pts',(93.4799733416942,1076.35619592397,448.819353884573));
#116925=CARTESIAN_POINT('Ctrl Pts',(93.4799883958374,1076.35619499446,448.81935388558));
#116926=CARTESIAN_POINT('Ctrl Pts',(93.5239130761171,1076.35348288653,448.819356822524));
#116927=CARTESIAN_POINT('Ctrl Pts',(93.5677293071545,1076.35069484535,448.823644427834));
#116928=CARTESIAN_POINT('Ctrl Pts',(93.6539989035039,1076.34503745886,448.840682570169));
#116929=CARTESIAN_POINT('Ctrl Pts',(93.6962459378029,1076.34218124833,448.853412412776));
#116930=CARTESIAN_POINT('Ctrl Pts',(93.819820025376,1076.33356167836,448.904257531836));
#116931=CARTESIAN_POINT('Ctrl Pts',(93.8950974830939,1076.32793422957,448.954512861949));
#116932=CARTESIAN_POINT('Ctrl Pts',(94.0209077297674,1076.31774179405,449.080757673004));
#116933=CARTESIAN_POINT('Ctrl Pts',(94.0705124222885,1076.31326426424,449.155221544693));
#116934=CARTESIAN_POINT('Ctrl Pts',(94.1380576308787,1076.30606768474,449.318924767482));
#116935=CARTESIAN_POINT('Ctrl Pts',(94.1554180377051,1076.30341556689,449.406537685414));
#116936=CARTESIAN_POINT('Ctrl Pts',(94.1553566605395,1076.30034980644,449.583324463453));
#116937=CARTESIAN_POINT('Ctrl Pts',(94.1380145459098,1076.29996170617,449.670764062105));
#116938=CARTESIAN_POINT('Ctrl Pts',(94.0706868754874,1076.30152307186,449.833963248197));
#116939=CARTESIAN_POINT('Ctrl Pts',(94.0213835798089,1076.30345527971,449.90813282625));
#116940=CARTESIAN_POINT('Ctrl Pts',(93.8970065888715,1076.30937099208,450.03339265262));
#116941=CARTESIAN_POINT('Ctrl Pts',(93.82310625867,1076.31329879062,450.083230605174));
#116942=CARTESIAN_POINT('Ctrl Pts',(93.6601858134117,1076.3225953758,450.151735095738));
#116943=CARTESIAN_POINT('Ctrl Pts',(93.572697535404,1076.32787696942,450.16966190179));
#116944=CARTESIAN_POINT('Ctrl Pts',(93.4828271644317,1076.33355192919,450.170237509001));
#116945=CARTESIAN_POINT('Ctrl Pts',(93.4813851448154,1076.33364305199,450.170242126204));
#116946=CARTESIAN_POINT('Ctrl Pts',(93.479943233478,1076.33373423278,450.170242126204));
#116947=CARTESIAN_POINT('Origin',(97.7222027015969,1067.7251047501,462.678935876427));
#116948=CARTESIAN_POINT('',(97.7222027015967,1077.70670509264,461.580104740434));
#116949=CARTESIAN_POINT('Ctrl Pts',(97.7223774853707,1077.62439637431,463.777766998518));
#116950=CARTESIAN_POINT('Ctrl Pts',(97.8652488471286,1077.61047146469,463.777744272919));
#116951=CARTESIAN_POINT('Ctrl Pts',(98.0068778787342,1077.59763005528,463.749857219864));
#116952=CARTESIAN_POINT('Ctrl Pts',(98.2526249076054,1077.57726328201,463.649034000485));
#116953=CARTESIAN_POINT('Ctrl Pts',(98.3574905237846,1077.56938265876,463.583865810438));
#116954=CARTESIAN_POINT('Ctrl Pts',(98.5370653843179,1077.55767770435,463.425313758873));
#116955=CARTESIAN_POINT('Ctrl Pts',(98.6118031240287,1077.55375460285,463.334466346593));
#116956=CARTESIAN_POINT('Ctrl Pts',(98.6868906872435,1077.55125604233,463.206021931477));
#116957=CARTESIAN_POINT('Ctrl Pts',(98.7017513688048,1077.55086778332,463.177861979705));
#116958=CARTESIAN_POINT('Ctrl Pts',(98.723157007946,1077.55048929999,463.132644603069));
#116959=CARTESIAN_POINT('Ctrl Pts',(98.7305347726689,1077.55039988936,463.116002901385));
#116960=CARTESIAN_POINT('Ctrl Pts',(98.7433633565128,1077.55032428066,463.085009950598));
#116961=CARTESIAN_POINT('Ctrl Pts',(98.7489333403759,1077.5503240831,463.070713150755));
#116962=CARTESIAN_POINT('Ctrl Pts',(98.7604385804056,1077.55039873526,463.039249475392));
#116963=CARTESIAN_POINT('Ctrl Pts',(98.7662512017515,1077.55048736259,463.022042773026));
#116964=CARTESIAN_POINT('Ctrl Pts',(98.7812747130292,1077.55086882627,462.973645347321));
#116965=CARTESIAN_POINT('Ctrl Pts',(98.7895309708941,1077.55126752842,462.942179720779));
#116966=CARTESIAN_POINT('Ctrl Pts',(98.8256759145672,1077.55417681668,462.774435855143));
#116967=CARTESIAN_POINT('Ctrl Pts',(98.8288759297638,1077.55930118692,462.634237323956));
#116968=CARTESIAN_POINT('Ctrl Pts',(98.7868430771987,1077.57316198976,462.383526553364));
#116969=CARTESIAN_POINT('Ctrl Pts',(98.7500126803987,1077.58104747223,462.273609643655));
#116970=CARTESIAN_POINT('Ctrl Pts',(98.6383090863358,1077.60028657507,462.059057600028));
#116971=CARTESIAN_POINT('Ctrl Pts',(98.560797625596,1077.61176560098,461.957680001032));
#116972=CARTESIAN_POINT('Ctrl Pts',(98.3674511948929,1077.63739383679,461.779071930105));
#116973=CARTESIAN_POINT('Ctrl Pts',(98.2506922038987,1077.65146467942,461.705910199451));
#116974=CARTESIAN_POINT('Ctrl Pts',(97.9865450051201,1077.68074653231,461.602266454776));
#116975=CARTESIAN_POINT('Ctrl Pts',(97.8400508784254,1077.69567544329,461.576554671687));
#116976=CARTESIAN_POINT('Ctrl Pts',(97.5502102397836,1077.72284129563,461.584316882894));
#116977=CARTESIAN_POINT('Ctrl Pts',(97.409604703891,1077.73489848313,461.615861291594));
#116978=CARTESIAN_POINT('Ctrl Pts',(97.1698005802234,1077.75347127226,461.721600828075));
#116979=CARTESIAN_POINT('Ctrl Pts',(97.069200000847,1077.76045186913,461.787157714475));
#116980=CARTESIAN_POINT('Ctrl Pts',(96.8984418442197,1077.77065893617,461.943156169815));
#116981=CARTESIAN_POINT('Ctrl Pts',(96.8277981069749,1077.77403230737,462.030850174253));
#116982=CARTESIAN_POINT('Ctrl Pts',(96.7560163178606,1077.77621092353,462.154645142902));
#116983=CARTESIAN_POINT('Ctrl Pts',(96.7415657161512,1077.77655464805,462.182198335974));
#116984=CARTESIAN_POINT('Ctrl Pts',(96.72065487641,1077.77689079144,462.22654950586));
#116985=CARTESIAN_POINT('Ctrl Pts',(96.7134051362498,1077.7769702779,462.242955417096));
#116986=CARTESIAN_POINT('Ctrl Pts',(96.7013379646493,1077.77703368948,462.272177657662));
#116987=CARTESIAN_POINT('Ctrl Pts',(96.696352470503,1077.77703579725,462.28492018693));
#116988=CARTESIAN_POINT('Ctrl Pts',(96.685532330415,1077.77698284557,462.314174342721));
#116989=CARTESIAN_POINT('Ctrl Pts',(96.6798518613852,1077.77691163816,462.330738878175));
#116990=CARTESIAN_POINT('Ctrl Pts',(96.6655000931725,1077.77660560186,462.376093948235));
#116991=CARTESIAN_POINT('Ctrl Pts',(96.6576109573208,1077.77629020204,462.405114944635));
#116992=CARTESIAN_POINT('Ctrl Pts',(96.6255903096901,1077.77419969049,462.545405709047));
#116993=CARTESIAN_POINT('Ctrl Pts',(96.6176693930722,1077.77082065323,462.659606965961));
#116994=CARTESIAN_POINT('Ctrl Pts',(96.6369579321418,1077.76091280199,462.884263300539));
#116995=CARTESIAN_POINT('Ctrl Pts',(96.6634346560488,1077.75449909266,462.993405676657));
#116996=CARTESIAN_POINT('Ctrl Pts',(96.7530884914899,1077.7381816032,463.211563535045));
#116997=CARTESIAN_POINT('Ctrl Pts',(96.8194456910075,1077.72808106501,463.317570621166));
#116998=CARTESIAN_POINT('Ctrl Pts',(96.991592198616,1077.70471527976,463.510655144333));
#116999=CARTESIAN_POINT('Ctrl Pts',(97.0988195395435,1077.69144661683,463.593759639793));
#117000=CARTESIAN_POINT('Ctrl Pts',(97.2945945973171,1077.66893027088,463.694785591453));
#117001=CARTESIAN_POINT('Ctrl Pts',(97.3752305141564,1077.66003853043,463.725075789592));
#117002=CARTESIAN_POINT('Ctrl Pts',(97.5448563663803,1077.64207150673,463.766998119792));
#117003=CARTESIAN_POINT('Ctrl Pts',(97.6334417894073,1077.63306446226,463.777781144929));
#117004=CARTESIAN_POINT('Ctrl Pts',(97.7223774853707,1077.62439637431,463.777766998518));
#117005=CARTESIAN_POINT('',(97.7222027015771,1075.6961592181,461.580104740434));
#117006=CARTESIAN_POINT('',(97.7222027015969,1067.7251047501,461.580104740434));
#117007=CARTESIAN_POINT('Ctrl Pts',(97.7213962340406,1075.61319330111,463.777766716473));
#117008=CARTESIAN_POINT('Ctrl Pts',(97.5770261561073,1075.62739687131,463.777660758595));
#117009=CARTESIAN_POINT('Ctrl Pts',(97.4341242719184,1075.64244589601,463.749104628276));
#117010=CARTESIAN_POINT('Ctrl Pts',(97.1656082188661,1075.67268771489,463.637621917011));
#117011=CARTESIAN_POINT('Ctrl Pts',(97.0428695849892,1075.68758788676,463.554963927471));
#117012=CARTESIAN_POINT('Ctrl Pts',(96.837686314047,1075.71492195647,463.346959379739));
#117013=CARTESIAN_POINT('Ctrl Pts',(96.756960917834,1075.72710923841,463.223924830604));
#117014=CARTESIAN_POINT('Ctrl Pts',(96.6483007962585,1075.7472871335,462.953466622021));
#117015=CARTESIAN_POINT('Ctrl Pts',(96.6213648162697,1075.75508627585,462.8087842277));
#117016=CARTESIAN_POINT('Ctrl Pts',(96.6256133146802,1075.76531543224,462.516949278297));
#117017=CARTESIAN_POINT('Ctrl Pts',(96.656816480121,1075.76763690043,462.372790660382));
#117018=CARTESIAN_POINT('Ctrl Pts',(96.7738060454817,1075.76644992584,462.105082237661));
#117019=CARTESIAN_POINT('Ctrl Pts',(96.8583708276482,1075.76295468752,461.984297679999));
#117020=CARTESIAN_POINT('Ctrl Pts',(97.0695415973137,1075.75052545678,461.782986595226));
#117021=CARTESIAN_POINT('Ctrl Pts',(97.1939544639372,1075.7417206361,461.704478040095));
#117022=CARTESIAN_POINT('Ctrl Pts',(97.4662404315634,1075.71981663867,461.600412100679));
#117023=CARTESIAN_POINT('Ctrl Pts',(97.6114601384691,1075.70692132068,461.576034860562));
#117024=CARTESIAN_POINT('Ctrl Pts',(97.8285214474085,1075.68587135561,461.582926702863));
#117025=CARTESIAN_POINT('Ctrl Pts',(97.8995578343671,1075.67869690786,461.592161096067));
#117026=CARTESIAN_POINT('Ctrl Pts',(98.0390806357657,1075.66402382542,461.624343517563));
#117027=CARTESIAN_POINT('Ctrl Pts',(98.1072333201016,1075.65655780719,461.647273957167));
#117028=CARTESIAN_POINT('Ctrl Pts',(98.3060072031474,1075.63385069365,461.736611056026));
#117029=CARTESIAN_POINT('Ctrl Pts',(98.4261202769493,1075.6187994765,461.822583420046));
#117030=CARTESIAN_POINT('Ctrl Pts',(98.6244761046872,1075.59106783417,462.03533062314));
#117031=CARTESIAN_POINT('Ctrl Pts',(98.7013213763591,1075.57862690897,462.15957890916));
#117032=CARTESIAN_POINT('Ctrl Pts',(98.802151146019,1075.55805915997,462.430202485468));
#117033=CARTESIAN_POINT('Ctrl Pts',(98.825461828968,1075.55011041699,462.573807692676));
#117034=CARTESIAN_POINT('Ctrl Pts',(98.8152523198532,1075.53989503967,462.861188426707));
#117035=CARTESIAN_POINT('Ctrl Pts',(98.782185188029,1075.53769666475,463.002099720797));
#117036=CARTESIAN_POINT('Ctrl Pts',(98.6638974462999,1075.53937606489,463.26296984945));
#117037=CARTESIAN_POINT('Ctrl Pts',(98.5800032503363,1075.54321998508,463.380378597254));
#117038=CARTESIAN_POINT('Ctrl Pts',(98.3718309816341,1075.55643045529,463.576673547403));
#117039=CARTESIAN_POINT('Ctrl Pts',(98.2495045334886,1075.56567869409,463.653524192746));
#117040=CARTESIAN_POINT('Ctrl Pts',(97.9899832981551,1075.58763380002,463.753158562953));
#117041=CARTESIAN_POINT('Ctrl Pts',(97.8561966645764,1075.59993122211,463.777865650877));
#117042=CARTESIAN_POINT('Ctrl Pts',(97.7213962340406,1075.61319330111,463.777766716473));
#117043=CARTESIAN_POINT('Origin',(97.7222027015969,1067.7251047501,462.678935876427));
#117044=CARTESIAN_POINT('',(97.7222027015969,1075.63649232379,463.177767012419));
#117045=CARTESIAN_POINT('',(97.7222027015972,1075.6741872497,462.180104740434));
#117046=CARTESIAN_POINT('Ctrl Pts',(97.7222027015969,1075.63649232379,463.177767012419));
#117047=CARTESIAN_POINT('Ctrl Pts',(97.6572569350772,1075.64283239013,463.177767012419));
#117048=CARTESIAN_POINT('Ctrl Pts',(97.5929472946405,1075.6495721601,463.165083811798));
#117049=CARTESIAN_POINT('Ctrl Pts',(97.4712302351422,1075.66326292133,463.115154326405));
#117050=CARTESIAN_POINT('Ctrl Pts',(97.4152347351747,1075.67008164955,463.077749631703));
#117051=CARTESIAN_POINT('Ctrl Pts',(97.3214347213736,1075.68266182711,462.983286339805));
#117052=CARTESIAN_POINT('Ctrl Pts',(97.2844710857069,1075.68830516242,462.927233885765));
#117053=CARTESIAN_POINT('Ctrl Pts',(97.2347461427881,1075.69766744456,462.803943202293));
#117054=CARTESIAN_POINT('Ctrl Pts',(97.2224316028057,1075.70129708935,462.737970559391));
#117055=CARTESIAN_POINT('Ctrl Pts',(97.2244011812662,1075.705997423,462.606444795298));
#117056=CARTESIAN_POINT('Ctrl Pts',(97.2380806517,1075.70707708838,462.542216119828));
#117057=CARTESIAN_POINT('Ctrl Pts',(97.2893356417546,1075.70663047217,462.422640387586));
#117058=CARTESIAN_POINT('Ctrl Pts',(97.3263853081653,1075.70511021377,462.368480132492));
#117059=CARTESIAN_POINT('Ctrl Pts',(97.4202147779464,1075.69957691317,462.276369805907));
#117060=CARTESIAN_POINT('Ctrl Pts',(97.4764713908016,1075.69556253835,462.239782288104));
#117061=CARTESIAN_POINT('Ctrl Pts',(97.5966624666558,1075.68582134651,462.19207681243));
#117062=CARTESIAN_POINT('Ctrl Pts',(97.6589621544798,1075.68028190558,462.180158261962));
#117063=CARTESIAN_POINT('Ctrl Pts',(97.7217791146744,1075.67422807885,462.180104920357));
#117064=CARTESIAN_POINT('Ctrl Pts',(97.7219203119211,1075.67421447132,462.180104800458));
#117065=CARTESIAN_POINT('Ctrl Pts',(97.7220615075749,1075.67420086161,462.180104740434));
#117066=CARTESIAN_POINT('Ctrl Pts',(97.7222027015975,1075.6741872497,462.180104740434));
#117067=CARTESIAN_POINT('',(97.7222027015969,1082.7251047501,462.180104740434));
#117068=CARTESIAN_POINT('',(97.7222027015969,1067.7251047501,462.180104740434));
#117069=CARTESIAN_POINT('Origin',(97.7222027015969,1082.7251047501,462.678935876427));
#117070=CARTESIAN_POINT('Ctrl Pts',(97.7222027015975,1075.6741872497,462.180104740434));
#117071=CARTESIAN_POINT('Ctrl Pts',(97.754609689393,1075.67106303118,462.180104740434));
#117072=CARTESIAN_POINT('Ctrl Pts',(97.7869307534788,1075.66782351289,462.183262736636));
#117073=CARTESIAN_POINT('Ctrl Pts',(97.850693653922,1075.66118268563,462.19583607518));
#117074=CARTESIAN_POINT('Ctrl Pts',(97.8819805854774,1075.65779584215,462.205263039015));
#117075=CARTESIAN_POINT('Ctrl Pts',(97.973996019334,1075.64743399608,462.243148976887));
#117076=CARTESIAN_POINT('Ctrl Pts',(98.0301420491263,1075.64053600106,462.280827109893));
#117077=CARTESIAN_POINT('Ctrl Pts',(98.1232581986539,1075.62785013386,462.375148449897));
#117078=CARTESIAN_POINT('Ctrl Pts',(98.1597193537219,1075.62216301585,462.430485544627));
#117079=CARTESIAN_POINT('Ctrl Pts',(98.2089844657867,1075.61268012852,462.551883093394));
#117080=CARTESIAN_POINT('Ctrl Pts',(98.2214434684478,1075.60896646353,462.616701334425));
#117081=CARTESIAN_POINT('Ctrl Pts',(98.2206060480949,1075.60403958664,462.747201156494));
#117082=CARTESIAN_POINT('Ctrl Pts',(98.2074623439131,1075.60286166937,462.811581640935));
#117083=CARTESIAN_POINT('Ctrl Pts',(98.1572135606402,1075.60320924604,462.931559153335));
#117084=CARTESIAN_POINT('Ctrl Pts',(98.1206638117141,1075.60472521221,462.985977292797));
#117085=CARTESIAN_POINT('Ctrl Pts',(98.0286985689788,1075.61026144565,463.077844669439));
#117086=CARTESIAN_POINT('Ctrl Pts',(97.9741443597817,1075.61423299495,463.114340784303));
#117087=CARTESIAN_POINT('Ctrl Pts',(97.8538834137291,1075.62412149214,463.164489182562));
#117088=CARTESIAN_POINT('Ctrl Pts',(97.7892776797568,1075.62995335678,463.17752150349));
#117089=CARTESIAN_POINT('Ctrl Pts',(97.7234368912988,1075.63637188279,463.177765867431));
#117090=CARTESIAN_POINT('Ctrl Pts',(97.7228197677316,1075.63643208521,463.177767012419));
#117091=CARTESIAN_POINT('Ctrl Pts',(97.7222027015969,1075.63649232379,463.177767012419));
#117092=CARTESIAN_POINT('Origin',(99.1956712429292,1067.7251047501,476.588028064191));
#117093=CARTESIAN_POINT('',(99.1956712429291,1076.88734730071,475.497487315463));
#117094=CARTESIAN_POINT('Ctrl Pts',(99.1958465811725,1076.75140941306,477.678568798823));
#117095=CARTESIAN_POINT('Ctrl Pts',(99.3351617747574,1076.7346540188,477.678546399586));
#117096=CARTESIAN_POINT('Ctrl Pts',(99.4734108960095,1076.71964145972,477.651828116974));
#117097=CARTESIAN_POINT('Ctrl Pts',(99.7161417774516,1076.69644564892,477.554078976883));
#117098=CARTESIAN_POINT('Ctrl Pts',(99.8209503002571,1076.68780224914,477.489830406464));
#117099=CARTESIAN_POINT('Ctrl Pts',(99.9771448754437,1076.67750000721,477.353420953028));
#117100=CARTESIAN_POINT('Ctrl Pts',(100.034524803286,1076.67455478323,477.290073020182));
#117101=CARTESIAN_POINT('Ctrl Pts',(100.100082677636,1076.67244456217,477.198020799036));
#117102=CARTESIAN_POINT('Ctrl Pts',(100.115331571195,1076.67207042614,477.174778670863));
#117103=CARTESIAN_POINT('Ctrl Pts',(100.13838380948,1076.67170327014,477.136532058407));
#117104=CARTESIAN_POINT('Ctrl Pts',(100.146754487306,1076.67161830386,477.121885998868));
#117105=CARTESIAN_POINT('Ctrl Pts',(100.161250987515,1076.67156200304,477.095097703538));
#117106=CARTESIAN_POINT('Ctrl Pts',(100.167495713823,1076.6715718113,477.083024082478));
#117107=CARTESIAN_POINT('Ctrl Pts',(100.181620291774,1076.67167681384,477.054417309451));
#117108=CARTESIAN_POINT('Ctrl Pts',(100.189312418226,1076.67180046132,477.037796490646));
#117109=CARTESIAN_POINT('Ctrl Pts',(100.210170509832,1076.67233666983,476.98957729023));
#117110=CARTESIAN_POINT('Ctrl Pts',(100.222270962653,1076.67290662092,476.957545393931));
#117111=CARTESIAN_POINT('Ctrl Pts',(100.277467201558,1076.67702217729,476.787656350893));
#117112=CARTESIAN_POINT('Ctrl Pts',(100.294314996694,1076.68419826844,476.642980662656));
#117113=CARTESIAN_POINT('Ctrl Pts',(100.273215456004,1076.70320492643,476.384279417923));
#117114=CARTESIAN_POINT('Ctrl Pts',(100.245620457751,1076.71370283127,476.271565322794));
#117115=CARTESIAN_POINT('Ctrl Pts',(100.151824386149,1076.73914623861,476.04844949399));
#117116=CARTESIAN_POINT('Ctrl Pts',(100.08269373915,1076.75424250037,475.941123726815));
#117117=CARTESIAN_POINT('Ctrl Pts',(99.9039530308407,1076.78783564412,475.74757637163));
#117118=CARTESIAN_POINT('Ctrl Pts',(99.792997548431,1076.80622580733,475.665426877847));
#117119=CARTESIAN_POINT('Ctrl Pts',(99.538988806265,1076.84405326829,475.542793526404));
#117120=CARTESIAN_POINT('Ctrl Pts',(99.3967517492221,1076.86313019544,475.506354948691));
#117121=CARTESIAN_POINT('Ctrl Pts',(99.1107527556563,1076.89770522881,475.491710286497));
#117122=CARTESIAN_POINT('Ctrl Pts',(98.9697771982252,1076.91298595081,475.511822942385));
#117123=CARTESIAN_POINT('Ctrl Pts',(98.7228795308952,1076.93655323769,475.597980489552));
#117124=CARTESIAN_POINT('Ctrl Pts',(98.6165747687278,1076.94538168441,475.656123314795));
#117125=CARTESIAN_POINT('Ctrl Pts',(98.4429096462419,1076.95725957267,475.792600900962));
#117126=CARTESIAN_POINT('Ctrl Pts',(98.3728785958174,1076.96096863199,475.865261488284));
#117127=CARTESIAN_POINT('Ctrl Pts',(98.2965084980456,1076.96344766329,475.970253245765));
#117128=CARTESIAN_POINT('Ctrl Pts',(98.2802182803277,1076.96385410512,475.994660144318));
#117129=CARTESIAN_POINT('Ctrl Pts',(98.2559131364058,1076.96425457595,476.034463937463));
#117130=CARTESIAN_POINT('Ctrl Pts',(98.2472480027526,1076.96434931872,476.04944481332));
#117131=CARTESIAN_POINT('Ctrl Pts',(98.2317871277339,1076.96442531801,476.077705784519));
#117132=CARTESIAN_POINT('Ctrl Pts',(98.224900370466,1076.96442045686,476.090931163826));
#117133=CARTESIAN_POINT('Ctrl Pts',(98.2102834441325,1076.96432123259,476.120464624055));
#117134=CARTESIAN_POINT('Ctrl Pts',(98.202682663047,1076.96420828806,476.136831502438));
#117135=CARTESIAN_POINT('Ctrl Pts',(98.1821749620315,1076.96371932022,476.18402218748));
#117136=CARTESIAN_POINT('Ctrl Pts',(98.1702748581943,1076.96320143568,476.215258297867));
#117137=CARTESIAN_POINT('Ctrl Pts',(98.1147447674314,1076.95939189429,476.383920280059));
#117138=CARTESIAN_POINT('Ctrl Pts',(98.0973062344002,1076.9526395624,476.528286014376));
#117139=CARTESIAN_POINT('Ctrl Pts',(98.1172160619302,1076.93453986928,476.786949066574));
#117140=CARTESIAN_POINT('Ctrl Pts',(98.1443316871356,1076.92447492308,476.899877821638));
#117141=CARTESIAN_POINT('Ctrl Pts',(98.2373240012515,1076.89985495387,477.123773319765));
#117142=CARTESIAN_POINT('Ctrl Pts',(98.3062050670795,1076.88513004011,477.231626860478));
#117143=CARTESIAN_POINT('Ctrl Pts',(98.4848475972005,1076.85201768475,477.426421706207));
#117144=CARTESIAN_POINT('Ctrl Pts',(98.596019935673,1076.83370848726,477.509196004444));
#117145=CARTESIAN_POINT('Ctrl Pts',(98.7912373214412,1076.80456106505,477.603932553809));
#117146=CARTESIAN_POINT('Ctrl Pts',(98.8665394631734,1076.79389458265,477.630767999022));
#117147=CARTESIAN_POINT('Ctrl Pts',(99.0265397562579,1076.77237044624,477.668699342284));
#117148=CARTESIAN_POINT('Ctrl Pts',(99.1110212610301,1076.76161132748,477.678582437124));
#117149=CARTESIAN_POINT('Ctrl Pts',(99.1958465811724,1076.75140941306,477.678568798823));
#117150=CARTESIAN_POINT('',(99.1956712429125,1074.86964135584,475.497487315462));
#117151=CARTESIAN_POINT('',(99.1956712429292,1067.7251047501,475.497487315462));
#117152=CARTESIAN_POINT('Ctrl Pts',(99.1952643927994,1074.73264861964,477.678568737027));
#117153=CARTESIAN_POINT('Ctrl Pts',(99.0517460771263,1074.75005615301,477.67851519437));
#117154=CARTESIAN_POINT('Ctrl Pts',(98.9097698670427,1074.76900244351,477.650133765574));
#117155=CARTESIAN_POINT('Ctrl Pts',(98.7113786882859,1074.79803574604,477.567751158396));
#117156=CARTESIAN_POINT('Ctrl Pts',(98.6481671702273,1074.8077433162,477.533880670059));
#117157=CARTESIAN_POINT('Ctrl Pts',(98.4681042010753,1074.83684315306,477.413257926984));
#117158=CARTESIAN_POINT('Ctrl Pts',(98.3646996972244,1074.85564381212,477.309090431949));
#117159=CARTESIAN_POINT('Ctrl Pts',(98.2053095581982,1074.88957139567,477.066908547697));
#117160=CARTESIAN_POINT('Ctrl Pts',(98.1505262447493,1074.90439905785,476.931469881838));
#117161=CARTESIAN_POINT('Ctrl Pts',(98.0971762665379,1074.92820415866,476.646984446269));
#117162=CARTESIAN_POINT('Ctrl Pts',(98.0990043535727,1074.93695809786,476.500856558028));
#117163=CARTESIAN_POINT('Ctrl Pts',(98.1591409803313,1074.94710326793,476.220670198977));
#117164=CARTESIAN_POINT('Ctrl Pts',(98.2155816401616,1074.94855352414,476.089238716457));
#117165=CARTESIAN_POINT('Ctrl Pts',(98.3757013610401,1074.94416584569,475.855191509198));
#117166=CARTESIAN_POINT('Ctrl Pts',(98.4777903545748,1074.9383661131,475.754977821258));
#117167=CARTESIAN_POINT('Ctrl Pts',(98.7170546997745,1074.91997135385,475.597477159545));
#117168=CARTESIAN_POINT('Ctrl Pts',(98.8525072930294,1074.90741099956,475.542863991436));
#117169=CARTESIAN_POINT('Ctrl Pts',(99.1371075425808,1074.87710181334,475.489426290735));
#117170=CARTESIAN_POINT('Ctrl Pts',(99.2835000073978,1074.85962400353,475.491430677514));
#117171=CARTESIAN_POINT('Ctrl Pts',(99.4945554115769,1074.8316404046,475.536836580004));
#117172=CARTESIAN_POINT('Ctrl Pts',(99.5624190940086,1074.82217675517,475.558550211646));
#117173=CARTESIAN_POINT('Ctrl Pts',(99.6931910602662,1074.80298217493,475.614968030021));
#117174=CARTESIAN_POINT('Ctrl Pts',(99.7557834634978,1074.79329335006,475.649600604602));
#117175=CARTESIAN_POINT('Ctrl Pts',(99.9342486124761,1074.76407509348,475.772602348726));
#117176=CARTESIAN_POINT('Ctrl Pts',(100.036371341694,1074.74503432885,475.878296152674));
#117177=CARTESIAN_POINT('Ctrl Pts',(100.192042063617,1074.71064395715,476.122051110436));
#117178=CARTESIAN_POINT('Ctrl Pts',(100.24479599716,1074.69557213169,476.257324526878));
#117179=CARTESIAN_POINT('Ctrl Pts',(100.294422682368,1074.67143879966,476.539592348336));
#117180=CARTESIAN_POINT('Ctrl Pts',(100.291374202805,1074.66255692892,476.683674581217));
#117181=CARTESIAN_POINT('Ctrl Pts',(100.229978789766,1074.65222651072,476.961607860377));
#117182=CARTESIAN_POINT('Ctrl Pts',(100.172738965682,1074.65081939223,477.092718628694));
#117183=CARTESIAN_POINT('Ctrl Pts',(100.011398926172,1074.6556532975,477.325513495924));
#117184=CARTESIAN_POINT('Ctrl Pts',(99.9090348548584,1074.66182947456,477.424883587504));
#117185=CARTESIAN_POINT('Ctrl Pts',(99.6716504411043,1074.68097646112,477.57944521021));
#117186=CARTESIAN_POINT('Ctrl Pts',(99.5387978489786,1074.69379625042,477.632821930371));
#117187=CARTESIAN_POINT('Ctrl Pts',(99.3322582714828,1074.71642671158,477.672157205324));
#117188=CARTESIAN_POINT('Ctrl Pts',(99.2638100766752,1074.72433461963,477.678594309498));
#117189=CARTESIAN_POINT('Ctrl Pts',(99.1952643927994,1074.73264861964,477.678568737027));
#117190=CARTESIAN_POINT('Origin',(99.1956712429292,1067.7251047501,476.588028064191));
#117191=CARTESIAN_POINT('',(99.1956712429292,1074.77118038462,477.078568812919));
#117192=CARTESIAN_POINT('',(99.1956712429291,1074.8328201009,476.097487315462));
#117193=CARTESIAN_POINT('Ctrl Pts',(99.1956712429292,1074.77118038462,477.078568812919));
#117194=CARTESIAN_POINT('Ctrl Pts',(99.1626961372876,1074.7751548492,477.078568812919));
#117195=CARTESIAN_POINT('Ctrl Pts',(99.1297477646064,1074.7793322153,477.075243758096));
#117196=CARTESIAN_POINT('Ctrl Pts',(99.0657858437502,1074.78785081691,477.062155481617));
#117197=CARTESIAN_POINT('Ctrl Pts',(99.0349616082967,1074.7921556658,477.052611997444));
#117198=CARTESIAN_POINT('Ctrl Pts',(98.9756735887002,1074.80084234471,477.02764702067));
#117199=CARTESIAN_POINT('Ctrl Pts',(98.9473408483259,1074.80520455892,477.012287419544));
#117200=CARTESIAN_POINT('Ctrl Pts',(98.8664725268024,1074.81832574806,476.957552677079));
#117201=CARTESIAN_POINT('Ctrl Pts',(98.8200739716366,1074.82682834479,476.910307871755));
#117202=CARTESIAN_POINT('Ctrl Pts',(98.7487547995675,1074.84219589629,476.8005306581));
#117203=CARTESIAN_POINT('Ctrl Pts',(98.7244136738683,1074.84892064961,476.739145109896));
#117204=CARTESIAN_POINT('Ctrl Pts',(98.7014411623352,1074.85962464656,476.611139004963));
#117205=CARTESIAN_POINT('Ctrl Pts',(98.7026768247695,1074.86353531181,476.545884627614));
#117206=CARTESIAN_POINT('Ctrl Pts',(98.7302649995425,1074.86806023038,476.420433380235));
#117207=CARTESIAN_POINT('Ctrl Pts',(98.7559520265371,1074.86867885329,476.361440805009));
#117208=CARTESIAN_POINT('Ctrl Pts',(98.8284834149077,1074.86659269479,476.256563420427));
#117209=CARTESIAN_POINT('Ctrl Pts',(98.874591640806,1074.86390876541,476.211746241645));
#117210=CARTESIAN_POINT('Ctrl Pts',(98.9815985143537,1074.85553641748,476.142036772301));
#117211=CARTESIAN_POINT('Ctrl Pts',(99.041523297757,1074.84991135535,476.117977723604));
#117212=CARTESIAN_POINT('Ctrl Pts',(99.1344242837301,1074.83994515504,476.100359062507));
#117213=CARTESIAN_POINT('Ctrl Pts',(99.165025857401,1074.8364766822,476.097487315462));
#117214=CARTESIAN_POINT('Ctrl Pts',(99.1956712429291,1074.8328201009,476.097487315462));
#117215=CARTESIAN_POINT('',(99.1956712429292,1082.7251047501,476.097487315462));
#117216=CARTESIAN_POINT('',(99.1956712429292,1067.7251047501,476.097487315462));
#117217=CARTESIAN_POINT('Origin',(99.1956712429292,1082.7251047501,476.588028064191));
#117218=CARTESIAN_POINT('Ctrl Pts',(99.1956712429291,1074.8328201009,476.097487315462));
#117219=CARTESIAN_POINT('Ctrl Pts',(99.1956805572333,1074.83281898953,476.097487315462));
#117220=CARTESIAN_POINT('Ctrl Pts',(99.1956898715415,1074.83281787814,476.097487315729));
#117221=CARTESIAN_POINT('Ctrl Pts',(99.1956991858538,1074.83281676673,476.097487316259));
#117222=CARTESIAN_POINT('Ctrl Pts',(99.2613415340014,1074.82498413957,476.097491055479));
#117223=CARTESIAN_POINT('Ctrl Pts',(99.3262541257414,1074.81639903078,476.11066932637));
#117224=CARTESIAN_POINT('Ctrl Pts',(99.4161889769876,1074.80323755955,476.148672372801));
#117225=CARTESIAN_POINT('Ctrl Pts',(99.4444713012855,1074.79887903672,476.164046852538));
#117226=CARTESIAN_POINT('Ctrl Pts',(99.5255279562476,1074.78568733498,476.21903124286));
#117227=CARTESIAN_POINT('Ctrl Pts',(99.5720685022878,1074.77708580007,476.266615523325));
#117228=CARTESIAN_POINT('Ctrl Pts',(99.6430606853371,1074.76157824561,476.376620403901));
#117229=CARTESIAN_POINT('Ctrl Pts',(99.667154531816,1074.75479754371,476.437754037079));
#117230=CARTESIAN_POINT('Ctrl Pts',(99.68984303202,1074.74399030679,476.565003513488));
#117231=CARTESIAN_POINT('Ctrl Pts',(99.6886378745193,1074.74002593788,476.629767038152));
#117232=CARTESIAN_POINT('Ctrl Pts',(99.6613707160498,1074.73539219092,476.754808810447));
#117233=CARTESIAN_POINT('Ctrl Pts',(99.6357837972584,1074.73474383589,476.813852869771));
#117234=CARTESIAN_POINT('Ctrl Pts',(99.5634706639402,1074.73684468048,476.91879929773));
#117235=CARTESIAN_POINT('Ctrl Pts',(99.5175072957653,1074.73956811237,476.963649574576));
#117236=CARTESIAN_POINT('Ctrl Pts',(99.4108081536497,1074.74805522612,477.033491876358));
#117237=CARTESIAN_POINT('Ctrl Pts',(99.3510457986267,1074.7537529146,477.057659621408));
#117238=CARTESIAN_POINT('Ctrl Pts',(99.257774605815,1074.76387774655,477.075622838188));
#117239=CARTESIAN_POINT('Ctrl Pts',(99.2267110811289,1074.76743917635,477.078568812919));
#117240=CARTESIAN_POINT('Ctrl Pts',(99.1956712429292,1074.77118038462,477.078568812919));
#117241=CARTESIAN_POINT('Origin',(89.3961860936685,1067.7251047501,419.235241127771));
#117242=CARTESIAN_POINT('',(89.396186093693,1078.67097321562,417.756937995578));
#117243=CARTESIAN_POINT('Ctrl Pts',(89.396365151478,1078.67555522044,420.713544249121));
#117244=CARTESIAN_POINT('Ctrl Pts',(89.5926021620978,1078.67059400202,420.713520480133));
#117245=CARTESIAN_POINT('Ctrl Pts',(89.7868803865718,1078.66530429547,420.674422855112));
#117246=CARTESIAN_POINT('Ctrl Pts',(90.1455321466403,1078.65489274438,420.524033233358));
#117247=CARTESIAN_POINT('Ctrl Pts',(90.3069592237574,1078.64987437859,420.415496758054));
#117248=CARTESIAN_POINT('Ctrl Pts',(90.5639905174958,1078.64146838599,420.157719986072));
#117249=CARTESIAN_POINT('Ctrl Pts',(90.6629652919494,1078.63802999079,420.016274572357));
#117250=CARTESIAN_POINT('Ctrl Pts',(90.804684180364,1078.63284103783,419.712966951113));
#117251=CARTESIAN_POINT('Ctrl Pts',(90.848840040397,1078.63105791976,419.554444544646));
#117252=CARTESIAN_POINT('Ctrl Pts',(90.8709486226905,1078.62990837589,419.347020229116));
#117253=CARTESIAN_POINT('Ctrl Pts',(90.8736746801494,1078.62972718661,419.301924041295));
#117254=CARTESIAN_POINT('Ctrl Pts',(90.8747098060535,1078.62955017467,419.230865850681));
#117255=CARTESIAN_POINT('Ctrl Pts',(90.8744060075422,1078.62950828556,419.204952494405));
#117256=CARTESIAN_POINT('Ctrl Pts',(90.872589819542,1078.62947295042,419.157196933325));
#117257=CARTESIAN_POINT('Ctrl Pts',(90.8712730476324,1078.62947298505,419.135354510003));
#117258=CARTESIAN_POINT('Ctrl Pts',(90.8673372935181,1078.62950848713,419.087705502361));
#117259=CARTESIAN_POINT('Ctrl Pts',(90.8645229743418,1078.62955051107,419.061922303702));
#117260=CARTESIAN_POINT('Ctrl Pts',(90.8547740306395,1078.62973121858,418.990165251602));
#117261=CARTESIAN_POINT('Ctrl Pts',(90.8463470880121,1078.62992003612,418.944425048915));
#117262=CARTESIAN_POINT('Ctrl Pts',(90.7911382054936,1078.63128073333,418.707940641688));
#117263=CARTESIAN_POINT('Ctrl Pts',(90.7088465874481,1078.63365394497,418.52753381423));
#117264=CARTESIAN_POINT('Ctrl Pts',(90.5016993951744,1078.63976416674,418.241329873439));
#117265=CARTESIAN_POINT('Ctrl Pts',(90.390004512142,1078.64308916845,418.129647228667));
#117266=CARTESIAN_POINT('Ctrl Pts',(90.1239555920498,1078.65087862969,417.937115791031));
#117267=CARTESIAN_POINT('Ctrl Pts',(89.9686248448788,1078.65535749821,417.86152813034));
#117268=CARTESIAN_POINT('Ctrl Pts',(89.6268884115708,1078.66487281626,417.76349378516));
#117269=CARTESIAN_POINT('Ctrl Pts',(89.4420129126725,1078.66983874007,417.746226030568));
#117270=CARTESIAN_POINT('Ctrl Pts',(89.0639182086915,1078.67953229188,417.781535349483));
#117271=CARTESIAN_POINT('Ctrl Pts',(88.874632708023,1078.68412829493,417.838225318654));
#117272=CARTESIAN_POINT('Ctrl Pts',(88.5329987312695,1078.69204165862,418.019971931558));
#117273=CARTESIAN_POINT('Ctrl Pts',(88.3831434860232,1078.69531632402,418.141749270905));
#117274=CARTESIAN_POINT('Ctrl Pts',(88.1541684632275,1078.70019975614,418.416443957324));
#117275=CARTESIAN_POINT('Ctrl Pts',(88.0699986809484,1078.70194026103,418.561247774263));
#117276=CARTESIAN_POINT('Ctrl Pts',(87.9653313245738,1078.70416950108,418.840871856981));
#117277=CARTESIAN_POINT('Ctrl Pts',(87.935797782561,1078.70483204222,418.97040285699));
#117278=CARTESIAN_POINT('Ctrl Pts',(87.9201609548036,1078.70529363473,419.143353153028));
#117279=CARTESIAN_POINT('Ctrl Pts',(87.9181668201181,1078.70537280198,419.184717394828));
#117280=CARTESIAN_POINT('Ctrl Pts',(87.9177594267779,1078.70545007456,419.250676894304));
#117281=CARTESIAN_POINT('Ctrl Pts',(87.9182200869431,1078.70546803235,419.275243079408));
#117282=CARTESIAN_POINT('Ctrl Pts',(87.9202278843457,1078.70548141821,419.321184556132));
#117283=CARTESIAN_POINT('Ctrl Pts',(87.9216279949986,1078.70547943627,419.342559915636));
#117284=CARTESIAN_POINT('Ctrl Pts',(87.9258105320442,1078.7054565499,419.390436345672));
#117285=CARTESIAN_POINT('Ctrl Pts',(87.9288459703438,1078.705431156,419.416907881017));
#117286=CARTESIAN_POINT('Ctrl Pts',(87.9397257594501,1078.70532051258,419.493448103484));
#117287=CARTESIAN_POINT('Ctrl Pts',(87.9494309089539,1078.70520204724,419.543213467121));
#117288=CARTESIAN_POINT('Ctrl Pts',(88.0093787827409,1078.70439483503,419.784003892429));
#117289=CARTESIAN_POINT('Ctrl Pts',(88.0949997063828,1078.703065199,419.964134396414));
#117290=CARTESIAN_POINT('Ctrl Pts',(88.3085843445926,1078.69933176009,420.248968168345));
#117291=CARTESIAN_POINT('Ctrl Pts',(88.4234942861283,1078.69721030295,420.359690718077));
#117292=CARTESIAN_POINT('Ctrl Pts',(88.6833424792936,1078.69203228291,420.539884312143));
#117293=CARTESIAN_POINT('Ctrl Pts',(88.826444223292,1078.68901136644,420.60842325218));
#117294=CARTESIAN_POINT('Ctrl Pts',(89.1136032323245,1078.68250947261,420.693192330588));
#117295=CARTESIAN_POINT('Ctrl Pts',(89.2546213004758,1078.67913875548,420.713561417686));
#117296=CARTESIAN_POINT('Ctrl Pts',(89.396365151478,1078.67555522044,420.713544249121));
#117297=CARTESIAN_POINT('',(89.3961860936479,1076.67023697645,417.756937995578));
#117298=CARTESIAN_POINT('',(89.3961860936685,1067.7251047501,417.756937995578));
#117299=CARTESIAN_POINT('Ctrl Pts',(89.3958628075866,1076.67488613727,420.713544224615));
#117300=CARTESIAN_POINT('Ctrl Pts',(89.2003037329778,1076.67988828043,420.713501458333));
#117301=CARTESIAN_POINT('Ctrl Pts',(89.0066716658443,1076.68446185602,420.674654572202));
#117302=CARTESIAN_POINT('Ctrl Pts',(88.6465876150618,1076.69236398927,420.52418675266));
#117303=CARTESIAN_POINT('Ctrl Pts',(88.4835370452158,1076.69562704742,420.414375969499));
#117304=CARTESIAN_POINT('Ctrl Pts',(88.2086750915665,1076.70077456957,420.137175558416));
#117305=CARTESIAN_POINT('Ctrl Pts',(88.0998441334391,1076.70260977851,419.972242292839));
#117306=CARTESIAN_POINT('Ctrl Pts',(87.9522924601903,1076.70490671658,419.608479072034));
#117307=CARTESIAN_POINT('Ctrl Pts',(87.915474988846,1076.7053429627,419.413092822487));
#117308=CARTESIAN_POINT('Ctrl Pts',(87.920531048797,1076.70482948334,419.019707987937));
#117309=CARTESIAN_POINT('Ctrl Pts',(87.9622279083649,1076.70388566694,418.82563928336));
#117310=CARTESIAN_POINT('Ctrl Pts',(88.1185225555899,1076.700547807,418.46644147806));
#117311=CARTESIAN_POINT('Ctrl Pts',(88.2310752264399,1076.69818923817,418.30465679144));
#117312=CARTESIAN_POINT('Ctrl Pts',(88.5122114751986,1076.69200409886,418.034448108022));
#117313=CARTESIAN_POINT('Ctrl Pts',(88.6779244245936,1076.68823293265,417.928563692943));
#117314=CARTESIAN_POINT('Ctrl Pts',(88.9483676843181,1076.68169997947,417.823164216011));
#117315=CARTESIAN_POINT('Ctrl Pts',(89.0405086630507,1076.67941956102,417.79718861429));
#117316=CARTESIAN_POINT('Ctrl Pts',(89.2289885462388,1076.67463308011,417.763289757598));
#117317=CARTESIAN_POINT('Ctrl Pts',(89.3248999771645,1076.67213721909,417.755540694822));
#117318=CARTESIAN_POINT('Ctrl Pts',(89.6167681764678,1076.66436230015,417.760417007292));
#117319=CARTESIAN_POINT('Ctrl Pts',(89.8100648471479,1076.65896009628,417.802597665003));
#117320=CARTESIAN_POINT('Ctrl Pts',(90.1672018754771,1076.64866396056,417.959093496439));
#117321=CARTESIAN_POINT('Ctrl Pts',(90.3278536181244,1076.64387183281,418.071186420475));
#117322=CARTESIAN_POINT('Ctrl Pts',(90.5966378383839,1076.63582738994,418.350982375037));
#117323=CARTESIAN_POINT('Ctrl Pts',(90.7021831269147,1076.63265953329,418.515948775082));
#117324=CARTESIAN_POINT('Ctrl Pts',(90.8434262157542,1076.6286746025,418.87694085061));
#117325=CARTESIAN_POINT('Ctrl Pts',(90.8778696214137,1076.62789620056,419.069408129626));
#117326=CARTESIAN_POINT('Ctrl Pts',(90.8705930944519,1076.62892628264,419.456296678916));
#117327=CARTESIAN_POINT('Ctrl Pts',(90.8290910361996,1076.63071870553,419.646965769265));
#117328=CARTESIAN_POINT('Ctrl Pts',(90.6751354860759,1076.63648673964,420.001381795169));
#117329=CARTESIAN_POINT('Ctrl Pts',(90.5642152194989,1076.64039978275,420.161728568667));
#117330=CARTESIAN_POINT('Ctrl Pts',(90.2869293510888,1076.64952914099,420.430775575771));
#117331=CARTESIAN_POINT('Ctrl Pts',(90.1231898942228,1076.65465149798,420.536849901135));
#117332=CARTESIAN_POINT('Ctrl Pts',(89.8570914339161,1076.66242227576,420.642948213038));
#117333=CARTESIAN_POINT('Ctrl Pts',(89.7674132497588,1076.66496255713,420.669208868241));
#117334=CARTESIAN_POINT('Ctrl Pts',(89.5835906501358,1076.66999866792,420.704625199847));
#117335=CARTESIAN_POINT('Ctrl Pts',(89.4898334440527,1076.67248249235,420.713564774798));
#117336=CARTESIAN_POINT('Ctrl Pts',(89.3958628075866,1076.67488613727,420.713544224615));
#117337=CARTESIAN_POINT('Origin',(89.3961860936685,1067.7251047501,419.235241127771));
#117338=CARTESIAN_POINT('',(89.3961860936685,1076.67415347727,420.113544259965));
#117339=CARTESIAN_POINT('',(89.3961860936854,1076.67140064346,418.356937995578));
#117340=CARTESIAN_POINT('Ctrl Pts',(89.3961860936685,1076.67415347727,420.113544259965));
#117341=CARTESIAN_POINT('Ctrl Pts',(89.2860749511209,1076.67698690193,420.113544259965));
#117342=CARTESIAN_POINT('Ctrl Pts',(89.1768740162537,1076.67966401957,420.092836616295));
#117343=CARTESIAN_POINT('Ctrl Pts',(88.9660596953361,1076.68460580211,420.009801445987));
#117344=CARTESIAN_POINT('Ctrl Pts',(88.8673463593847,1076.6867908605,419.946074527012));
#117345=CARTESIAN_POINT('Ctrl Pts',(88.700164984497,1076.690328816,419.783527140741));
#117346=CARTESIAN_POINT('Ctrl Pts',(88.6334878189784,1076.69164609358,419.686191896892));
#117347=CARTESIAN_POINT('Ctrl Pts',(88.5419256009336,1076.69333443435,419.470665020016));
#117348=CARTESIAN_POINT('Ctrl Pts',(88.5181485291833,1076.69368635659,419.354556242671));
#117349=CARTESIAN_POINT('Ctrl Pts',(88.5176220514905,1076.69339780757,419.119972542679));
#117350=CARTESIAN_POINT('Ctrl Pts',(88.5408361739458,1076.69276073735,419.003860581854));
#117351=CARTESIAN_POINT('Ctrl Pts',(88.631242643307,1076.69051636158,418.788156268158));
#117352=CARTESIAN_POINT('Ctrl Pts',(88.697313779647,1076.68893376231,418.690632858346));
#117353=CARTESIAN_POINT('Ctrl Pts',(88.8634648455413,1076.68490757212,418.527314785467));
#117354=CARTESIAN_POINT('Ctrl Pts',(88.9618126163982,1076.68250310554,418.463057119944));
#117355=CARTESIAN_POINT('Ctrl Pts',(89.1226742179782,1076.67846342243,418.398670771847));
#117356=CARTESIAN_POINT('Ctrl Pts',(89.1774695150229,1076.67707208457,418.382702881811));
#117357=CARTESIAN_POINT('Ctrl Pts',(89.2870916290989,1076.67425368401,418.36203000487));
#117358=CARTESIAN_POINT('Ctrl Pts',(89.3415825686882,1076.67283665557,418.356937995576));
#117359=CARTESIAN_POINT('Ctrl Pts',(89.3961860937022,1076.67140064346,418.356937995578));
#117360=CARTESIAN_POINT('',(89.3961860936685,1082.7251047501,418.356937995578));
#117361=CARTESIAN_POINT('',(89.3961860936685,1067.7251047501,418.356937995578));
#117362=CARTESIAN_POINT('Origin',(89.3961860936685,1082.7251047501,419.235241127771));
#117363=CARTESIAN_POINT('Ctrl Pts',(89.3961860937022,1076.67140064346,418.356937995578));
#117364=CARTESIAN_POINT('Ctrl Pts',(89.3986607406576,1076.67133556299,418.356937995578));
#117365=CARTESIAN_POINT('Ctrl Pts',(89.4011356188665,1076.67127044396,418.356948454172));
#117366=CARTESIAN_POINT('Ctrl Pts',(89.5199913397858,1076.66814155448,418.357953214332));
#117367=CARTESIAN_POINT('Ctrl Pts',(89.6350256668046,1076.6650379992,418.382059894481));
#117368=CARTESIAN_POINT('Ctrl Pts',(89.8478551468005,1076.6592102296,418.473224245885));
#117369=CARTESIAN_POINT('Ctrl Pts',(89.9437637384592,1076.65654094439,418.53893899094));
#117370=CARTESIAN_POINT('Ctrl Pts',(90.1047307400064,1076.65208210947,418.703609080853));
#117371=CARTESIAN_POINT('Ctrl Pts',(90.1682412701848,1076.6503379917,418.800957168843));
#117372=CARTESIAN_POINT('Ctrl Pts',(90.2512204196791,1076.64819395911,419.00747937103));
#117373=CARTESIAN_POINT('Ctrl Pts',(90.2726467436591,1076.64773102208,419.113681003135));
#117374=CARTESIAN_POINT('Ctrl Pts',(90.2743755221586,1076.64787624781,419.221108905413));
#117375=CARTESIAN_POINT('Ctrl Pts',(90.2762246161387,1076.64803158062,419.336013323445));
#117376=CARTESIAN_POINT('Ctrl Pts',(90.2555044101713,1076.64887998737,419.450166271211));
#117377=CARTESIAN_POINT('Ctrl Pts',(90.1713002092023,1076.65181242532,419.663974429493));
#117378=CARTESIAN_POINT('Ctrl Pts',(90.108641187565,1076.65386587201,419.76156620233));
#117379=CARTESIAN_POINT('Ctrl Pts',(89.9492837723896,1076.65880378749,419.927128576555));
#117380=CARTESIAN_POINT('Ctrl Pts',(89.8541034515488,1076.66163849817,419.993485350182));
#117381=CARTESIAN_POINT('Ctrl Pts',(89.643558053945,1076.66761007176,420.085795385248));
#117382=CARTESIAN_POINT('Ctrl Pts',(89.5302118704862,1076.67068771278,420.110839572154));
#117383=CARTESIAN_POINT('Ctrl Pts',(89.4089026814889,1076.67382581652,420.113475248774));
#117384=CARTESIAN_POINT('Ctrl Pts',(89.4025428706656,1076.67398990211,420.113544259965));
#117385=CARTESIAN_POINT('Ctrl Pts',(89.3961860936685,1076.67415347727,420.113544259965));
#117386=CARTESIAN_POINT('Origin',(96.608893067355,1067.7251047501,429.515656233126));
#117387=CARTESIAN_POINT('',(96.6088930673831,1078.35304757369,428.24021211199));
#117388=CARTESIAN_POINT('Ctrl Pts',(96.6091598698775,1078.34476504118,430.791100326357));
#117389=CARTESIAN_POINT('Ctrl Pts',(96.7780589842411,1078.33391689068,430.791064995361));
#117390=CARTESIAN_POINT('Ctrl Pts',(96.9453022942696,1078.32309025058,430.757480637883));
#117391=CARTESIAN_POINT('Ctrl Pts',(97.252542525453,1078.30313955902,430.628940999755));
#117392=CARTESIAN_POINT('Ctrl Pts',(97.3903484268822,1078.29416340589,430.536956076821));
#117393=CARTESIAN_POINT('Ctrl Pts',(97.6068876450851,1078.2801769268,430.322235083317));
#117394=CARTESIAN_POINT('Ctrl Pts',(97.6897643941568,1078.27488130207,430.207252763852));
#117395=CARTESIAN_POINT('Ctrl Pts',(97.8017564083411,1078.26794934715,429.980780131298));
#117396=CARTESIAN_POINT('Ctrl Pts',(97.8379361604888,1078.26581462932,429.874437867473));
#117397=CARTESIAN_POINT('Ctrl Pts',(97.8665541867106,1078.26433515541,429.730712377094));
#117398=CARTESIAN_POINT('Ctrl Pts',(97.8719370554832,1078.26408218529,429.696434049079));
#117399=CARTESIAN_POINT('Ctrl Pts',(97.8782736194658,1078.26383542025,429.641564880119));
#117400=CARTESIAN_POINT('Ctrl Pts',(97.8801374016113,1078.26377805036,429.621097325731));
#117401=CARTESIAN_POINT('Ctrl Pts',(97.8826983900408,1078.2637352564,429.582726152118));
#117402=CARTESIAN_POINT('Ctrl Pts',(97.8835144878876,1078.26374153488,429.564835576519));
#117403=CARTESIAN_POINT('Ctrl Pts',(97.8844998735435,1078.26381441373,429.524665335253));
#117404=CARTESIAN_POINT('Ctrl Pts',(97.884462661919,1078.26389534235,429.502386557595));
#117405=CARTESIAN_POINT('Ctrl Pts',(97.8826598355887,1078.26424784371,429.437705113659));
#117406=CARTESIAN_POINT('Ctrl Pts',(97.8793617789237,1078.26462545867,429.395376595322));
#117407=CARTESIAN_POINT('Ctrl Pts',(97.8522924709095,1078.26724264127,429.184464150602));
#117408=CARTESIAN_POINT('Ctrl Pts',(97.7970543993223,1078.27164299534,429.021724858507));
#117409=CARTESIAN_POINT('Ctrl Pts',(97.643273015679,1078.28310168061,428.757184750735));
#117410=CARTESIAN_POINT('Ctrl Pts',(97.5566731991259,1078.28937029402,428.651417211364));
#117411=CARTESIAN_POINT('Ctrl Pts',(97.3439662424416,1078.30434876736,428.462814941456));
#117412=CARTESIAN_POINT('Ctrl Pts',(97.2165371116341,1078.31311606194,428.384483139707));
#117413=CARTESIAN_POINT('Ctrl Pts',(96.9301900342652,1078.33231516005,428.271071750476));
#117414=CARTESIAN_POINT('Ctrl Pts',(96.7721146000858,1078.34265289184,428.240675042645));
#117415=CARTESIAN_POINT('Ctrl Pts',(96.4435935292681,1078.36357468578,428.239732727962));
#117416=CARTESIAN_POINT('Ctrl Pts',(96.2761721401171,1078.37393269022,428.272825621434));
#117417=CARTESIAN_POINT('Ctrl Pts',(95.9680216748652,1078.39248535877,428.400697928381));
#117418=CARTESIAN_POINT('Ctrl Pts',(95.8295845387844,1078.40056007298,428.492638938362));
#117419=CARTESIAN_POINT('Ctrl Pts',(95.6124230489633,1078.41287657546,428.707219678173));
#117420=CARTESIAN_POINT('Ctrl Pts',(95.5294171079926,1078.41742446496,428.821916780123));
#117421=CARTESIAN_POINT('Ctrl Pts',(95.4165788203255,1078.42336782487,429.048889145251));
#117422=CARTESIAN_POINT('Ctrl Pts',(95.3799756824197,1078.42518293578,429.15613878423));
#117423=CARTESIAN_POINT('Ctrl Pts',(95.3512065708384,1078.42643117177,429.300759728285));
#117424=CARTESIAN_POINT('Ctrl Pts',(95.3458379126787,1078.42664263812,429.33496982924));
#117425=CARTESIAN_POINT('Ctrl Pts',(95.3395283160829,1078.42684858651,429.389613878104));
#117426=CARTESIAN_POINT('Ctrl Pts',(95.3376753841892,1078.42689649,429.409924712243));
#117427=CARTESIAN_POINT('Ctrl Pts',(95.3351141541855,1078.42693294889,429.448097447928));
#117428=CARTESIAN_POINT('Ctrl Pts',(95.3342927853368,1078.42692811649,429.465946779611));
#117429=CARTESIAN_POINT('Ctrl Pts',(95.3332975045362,1078.42686857656,429.505792232258));
#117430=CARTESIAN_POINT('Ctrl Pts',(95.3333170549708,1078.42680262111,429.527787446515));
#117431=CARTESIAN_POINT('Ctrl Pts',(95.3350230576038,1078.42651543316,429.591546673648));
#117432=CARTESIAN_POINT('Ctrl Pts',(95.338193352319,1078.4262080599,429.633241306722));
#117433=CARTESIAN_POINT('Ctrl Pts',(95.3646146130976,1078.42404864329,429.843466252332));
#117434=CARTESIAN_POINT('Ctrl Pts',(95.4193650307878,1078.42037893309,430.006253541714));
#117435=CARTESIAN_POINT('Ctrl Pts',(95.5724958984442,1078.41053361279,430.271426216472));
#117436=CARTESIAN_POINT('Ctrl Pts',(95.6590386556319,1078.40506236998,430.37766705163));
#117437=CARTESIAN_POINT('Ctrl Pts',(95.8720884163574,1078.39162279519,430.567380500981));
#117438=CARTESIAN_POINT('Ctrl Pts',(95.9999857653115,1078.38356658276,430.646235777515));
#117439=CARTESIAN_POINT('Ctrl Pts',(96.2883505717373,1078.36529272026,430.760639839526));
#117440=CARTESIAN_POINT('Ctrl Pts',(96.4480465416396,1078.35511312168,430.79113402869));
#117441=CARTESIAN_POINT('Ctrl Pts',(96.6091598698775,1078.34476504118,430.791100326357));
#117442=CARTESIAN_POINT('',(96.6088930673352,1076.3488082978,428.24021211199));
#117443=CARTESIAN_POINT('',(96.608893067355,1067.7251047501,428.24021211199));
#117444=CARTESIAN_POINT('Ctrl Pts',(96.6091161516571,1076.34044219187,430.791100334753));
#117445=CARTESIAN_POINT('Ctrl Pts',(96.5257062042077,1076.34585531859,430.791114923749));
#117446=CARTESIAN_POINT('Ctrl Pts',(96.4424911049163,1076.35123612761,430.782947365478));
#117447=CARTESIAN_POINT('Ctrl Pts',(96.194791856356,1076.3671952592,430.733800607917));
#117448=CARTESIAN_POINT('Ctrl Pts',(96.0370589157469,1076.37727408663,430.66821601593));
#117449=CARTESIAN_POINT('Ctrl Pts',(95.7568651334049,1076.3951358746,430.479614349123));
#117450=CARTESIAN_POINT('Ctrl Pts',(95.6370223540367,1076.40275653031,430.358672128692));
#117451=CARTESIAN_POINT('Ctrl Pts',(95.4510449959223,1076.4147596279,430.076680552373));
#117452=CARTESIAN_POINT('Ctrl Pts',(95.386912852988,1076.41901866201,429.918339734609));
#117453=CARTESIAN_POINT('Ctrl Pts',(95.3241009777672,1076.42371559229,429.585332395619));
#117454=CARTESIAN_POINT('Ctrl Pts',(95.3262351364234,1076.42409823989,429.413985449834));
#117455=CARTESIAN_POINT('Ctrl Pts',(95.3973581420346,1076.42090102356,429.082506550211));
#117456=CARTESIAN_POINT('Ctrl Pts',(95.4654991720177,1076.41735930617,428.925689250503));
#117457=CARTESIAN_POINT('Ctrl Pts',(95.6586502079043,1076.40667050234,428.648325624693));
#117458=CARTESIAN_POINT('Ctrl Pts',(95.7815504819943,1076.39963671498,428.530421550854));
#117459=CARTESIAN_POINT('Ctrl Pts',(96.0663045449067,1076.38275178711,428.349073138491));
#117460=CARTESIAN_POINT('Ctrl Pts',(96.2254321069276,1076.37305628671,428.287552070561));
#117461=CARTESIAN_POINT('Ctrl Pts',(96.5598377418726,1076.35205431126,428.229806745443));
#117462=CARTESIAN_POINT('Ctrl Pts',(96.7319221687995,1076.3409408836,428.234770116977));
#117463=CARTESIAN_POINT('Ctrl Pts',(97.0611532241657,1076.31908585922,428.311370086237));
#117464=CARTESIAN_POINT('Ctrl Pts',(97.2153462197109,1076.30855281656,428.381159049807));
#117465=CARTESIAN_POINT('Ctrl Pts',(97.4877985936292,1076.28945991678,428.576330749339));
#117466=CARTESIAN_POINT('Ctrl Pts',(97.6034704741582,1076.28108626243,428.699771245375));
#117467=CARTESIAN_POINT('Ctrl Pts',(97.7802554189951,1076.26786524973,428.984048732891));
#117468=CARTESIAN_POINT('Ctrl Pts',(97.8397958318671,1076.26314114355,429.142011296511));
#117469=CARTESIAN_POINT('Ctrl Pts',(97.8944277253633,1076.25814920103,429.471480852004));
#117470=CARTESIAN_POINT('Ctrl Pts',(97.8891910980265,1076.25791770276,429.639711562067));
#117471=CARTESIAN_POINT('Ctrl Pts',(97.8143459148466,1076.26200684184,429.964377877794));
#117472=CARTESIAN_POINT('Ctrl Pts',(97.7455690186523,1076.26627897936,430.117655123041));
#117473=CARTESIAN_POINT('Ctrl Pts',(97.5529961184477,1076.27866570818,430.389255396033));
#117474=CARTESIAN_POINT('Ctrl Pts',(97.4309970420768,1076.2866612289,430.504901473221));
#117475=CARTESIAN_POINT('Ctrl Pts',(97.1491933464996,1076.30516104736,430.68300221619));
#117476=CARTESIAN_POINT('Ctrl Pts',(96.9919835153256,1076.31549077737,430.743595488476));
#117477=CARTESIAN_POINT('Ctrl Pts',(96.7554587177488,1076.33092979891,430.784766387279));
#117478=CARTESIAN_POINT('Ctrl Pts',(96.6823552564843,1076.33568913103,430.791087524709));
#117479=CARTESIAN_POINT('Ctrl Pts',(96.6091161516571,1076.34044219187,430.791100334753));
#117480=CARTESIAN_POINT('Origin',(96.608893067355,1067.7251047501,429.515656233126));
#117481=CARTESIAN_POINT('',(96.608893067355,1076.34281999372,430.191100354262));
#117482=CARTESIAN_POINT('',(96.608893067355,1076.34724098047,428.84021211199));
#117483=CARTESIAN_POINT('Ctrl Pts',(96.608893067355,1076.34281999372,430.191100354262));
#117484=CARTESIAN_POINT('Ctrl Pts',(96.5658147920971,1076.34560871382,430.191100354262));
#117485=CARTESIAN_POINT('Ctrl Pts',(96.52283114131,1076.34839238715,430.186979197945));
#117486=CARTESIAN_POINT('Ctrl Pts',(96.3922695285492,1076.35685180461,430.161706409238));
#117487=CARTESIAN_POINT('Ctrl Pts',(96.3082778772544,1076.36229842477,430.127167221171));
#117488=CARTESIAN_POINT('Ctrl Pts',(96.158884077575,1076.3720341645,430.027293685815));
#117489=CARTESIAN_POINT('Ctrl Pts',(96.0949243857349,1076.37623042713,429.963014350603));
#117490=CARTESIAN_POINT('Ctrl Pts',(95.9958047352578,1076.38286170464,429.813040719218));
#117491=CARTESIAN_POINT('Ctrl Pts',(95.9616820843232,1076.38522898994,429.728826775021));
#117492=CARTESIAN_POINT('Ctrl Pts',(95.9284231983361,1076.38783123599,429.551810006037));
#117493=CARTESIAN_POINT('Ctrl Pts',(95.929674749872,1076.3880374266,429.460795811302));
#117494=CARTESIAN_POINT('Ctrl Pts',(95.9678012182744,1076.38623910634,429.284719321792));
#117495=CARTESIAN_POINT('Ctrl Pts',(96.0042519996463,1076.38425464593,429.201439533524));
#117496=CARTESIAN_POINT('Ctrl Pts',(96.1075236577383,1076.37831335311,429.054218441719));
#117497=CARTESIAN_POINT('Ctrl Pts',(96.1732545550311,1076.3744182383,428.99172570101));
#117498=CARTESIAN_POINT('Ctrl Pts',(96.3253360597475,1076.36516534383,428.896058513761));
#117499=CARTESIAN_POINT('Ctrl Pts',(96.4101984234306,1076.35989647234,428.863876652953));
#117500=CARTESIAN_POINT('Ctrl Pts',(96.5352179471671,1076.35196907944,428.843230577298));
#117501=CARTESIAN_POINT('Ctrl Pts',(96.5720256934705,1076.34961643708,428.84021211199));
#117502=CARTESIAN_POINT('Ctrl Pts',(96.6088930673551,1076.34724098047,428.84021211199));
#117503=CARTESIAN_POINT('',(96.608893067355,1082.7251047501,428.84021211199));
#117504=CARTESIAN_POINT('',(96.608893067355,1067.7251047501,428.84021211199));
#117505=CARTESIAN_POINT('Origin',(96.608893067355,1082.7251047501,429.515656233126));
#117506=CARTESIAN_POINT('Ctrl Pts',(96.6088930673551,1076.34724098047,428.84021211199));
#117507=CARTESIAN_POINT('Ctrl Pts',(96.6089025413445,1076.34724037004,428.84021211199));
#117508=CARTESIAN_POINT('Ctrl Pts',(96.6089120153378,1076.34723975961,428.840212112183));
#117509=CARTESIAN_POINT('Ctrl Pts',(96.6089214893351,1076.34723914917,428.840212112582));
#117510=CARTESIAN_POINT('Ctrl Pts',(96.6530279814733,1076.34439724654,428.840213968537));
#117511=CARTESIAN_POINT('Ctrl Pts',(96.6970284556051,1076.34153498234,428.84453604931));
#117512=CARTESIAN_POINT('Ctrl Pts',(96.8281870782537,1076.33292169698,428.870548295092));
#117513=CARTESIAN_POINT('Ctrl Pts',(96.9117602770266,1076.32731966516,428.905301673286));
#117514=CARTESIAN_POINT('Ctrl Pts',(97.0596241144492,1076.31720948098,429.004855233394));
#117515=CARTESIAN_POINT('Ctrl Pts',(97.1227030254683,1076.31278797405,429.068344596971));
#117516=CARTESIAN_POINT('Ctrl Pts',(97.2206312431141,1076.30572917975,429.21594679194));
#117517=CARTESIAN_POINT('Ctrl Pts',(97.2545974685802,1076.30315738567,429.298573106462));
#117518=CARTESIAN_POINT('Ctrl Pts',(97.2886875845159,1076.30026500213,429.47206387651));
#117519=CARTESIAN_POINT('Ctrl Pts',(97.2885599604648,1076.29996784546,429.561209221119));
#117520=CARTESIAN_POINT('Ctrl Pts',(97.2540221793563,1076.30170717808,429.734327758894));
#117521=CARTESIAN_POINT('Ctrl Pts',(97.2199798348334,1076.30372425459,429.816610854075));
#117522=CARTESIAN_POINT('Ctrl Pts',(97.1221665855661,1076.30979055424,429.963509334998));
#117523=CARTESIAN_POINT('Ctrl Pts',(97.0593064093363,1076.31378244562,430.026672537639));
#117524=CARTESIAN_POINT('Ctrl Pts',(96.9127352398344,1076.32317802229,430.125352966867));
#117525=CARTESIAN_POINT('Ctrl Pts',(96.830382000739,1076.32849361908,430.159848746053));
#117526=CARTESIAN_POINT('Ctrl Pts',(96.7004128191174,1076.33689663328,430.186331298869));
#117527=CARTESIAN_POINT('Ctrl Pts',(96.6563141293245,1076.33975020148,430.190883463694));
#117528=CARTESIAN_POINT('Ctrl Pts',(96.6110243655397,1076.34268202248,430.191097832485));
#117529=CARTESIAN_POINT('Ctrl Pts',(96.6099586874942,1076.34275100961,430.191100354262));
#117530=CARTESIAN_POINT('Ctrl Pts',(96.608893067355,1076.34281999372,430.191100354262));
#117531=CARTESIAN_POINT('Origin',(103.499585384595,1067.7251047501,441.529673720836));
#117532=CARTESIAN_POINT('',(103.499585384619,1077.68406953396,440.430842584843));
#117533=CARTESIAN_POINT('Ctrl Pts',(103.499860694173,1077.64747802966,442.628504822339));
#117534=CARTESIAN_POINT('Ctrl Pts',(103.645111118182,1077.63259627413,442.628468430183));
#117535=CARTESIAN_POINT('Ctrl Pts',(103.789010605813,1077.6182221956,442.59963215631));
#117536=CARTESIAN_POINT('Ctrl Pts',(104.050498000161,1077.59291668959,442.490382015408));
#117537=CARTESIAN_POINT('Ctrl Pts',(104.16677498141,1077.58206970272,442.413639589368));
#117538=CARTESIAN_POINT('Ctrl Pts',(104.359583798264,1077.56505944824,442.226046984409));
#117539=CARTESIAN_POINT('Ctrl Pts',(104.436358856901,1077.55881466678,442.11877473147));
#117540=CARTESIAN_POINT('Ctrl Pts',(104.518663846431,1077.55312454052,441.94518193482));
#117541=CARTESIAN_POINT('Ctrl Pts',(104.540205315743,1077.5518391956,441.887836893985));
#117542=CARTESIAN_POINT('Ctrl Pts',(104.563392351372,1077.55080368086,441.805932189706));
#117543=CARTESIAN_POINT('Ctrl Pts',(104.569163545854,1077.55059555095,441.782669040295));
#117544=CARTESIAN_POINT('Ctrl Pts',(104.577163463826,1077.55039678927,441.745221169366));
#117545=CARTESIAN_POINT('Ctrl Pts',(104.579882835002,1077.55035237811,441.731149882642));
#117546=CARTESIAN_POINT('Ctrl Pts',(104.584899611622,1077.55032279103,441.702157590973));
#117547=CARTESIAN_POINT('Ctrl Pts',(104.587166314174,1077.55034089549,441.68723442818));
#117548=CARTESIAN_POINT('Ctrl Pts',(104.591680524313,1077.55045929991,441.652742416295));
#117549=CARTESIAN_POINT('Ctrl Pts',(104.593710695626,1077.55058295171,441.633150648677));
#117550=CARTESIAN_POINT('Ctrl Pts',(104.598359693779,1077.55114022538,441.572398295951));
#117551=CARTESIAN_POINT('Ctrl Pts',(104.599188774366,1077.55176452249,441.531140496396));
#117552=CARTESIAN_POINT('Ctrl Pts',(104.592420560346,1077.55570449242,441.344100048161));
#117553=CARTESIAN_POINT('Ctrl Pts',(104.558150384969,1077.56179060128,441.200883163092));
#117554=CARTESIAN_POINT('Ctrl Pts',(104.447618586277,1077.57749669874,440.96176623425));
#117555=CARTESIAN_POINT('Ctrl Pts',(104.381422833653,1077.58610740631,440.863638806983));
#117556=CARTESIAN_POINT('Ctrl Pts',(104.212974784091,1077.60671063103,440.684055240918));
#117557=CARTESIAN_POINT('Ctrl Pts',(104.109177244887,1077.61878817036,440.606447398284));
#117558=CARTESIAN_POINT('Ctrl Pts',(103.870735432718,1077.64536986028,440.486185842388));
#117559=CARTESIAN_POINT('Ctrl Pts',(103.736382388567,1077.65975812971,440.447760953317));
#117560=CARTESIAN_POINT('Ctrl Pts',(103.453241190359,1077.68893717594,440.422179988729));
#117561=CARTESIAN_POINT('Ctrl Pts',(103.306772389159,1077.70342984835,440.438087269816));
#117562=CARTESIAN_POINT('Ctrl Pts',(103.033089922435,1077.72939661722,440.524821449055));
#117563=CARTESIAN_POINT('Ctrl Pts',(102.907899993219,1077.74071983741,440.593016016293));
#117564=CARTESIAN_POINT('Ctrl Pts',(102.705109527106,1077.75805565959,440.760852622276));
#117565=CARTESIAN_POINT('Ctrl Pts',(102.62474411354,1077.76446595137,440.853676109533));
#117566=CARTESIAN_POINT('Ctrl Pts',(102.514059557075,1077.77241712264,441.035314010731));
#117567=CARTESIAN_POINT('Ctrl Pts',(102.476624965789,1077.77475443465,441.118316870278));
#117568=CARTESIAN_POINT('Ctrl Pts',(102.44146198237,1077.77637828602,441.232009394482));
#117569=CARTESIAN_POINT('Ctrl Pts',(102.43415352809,1077.77665665588,441.259332703226));
#117570=CARTESIAN_POINT('Ctrl Pts',(102.424194427279,1077.77692835425,441.303296789513));
#117571=CARTESIAN_POINT('Ctrl Pts',(102.42085837831,1077.77699146764,441.319768308307));
#117572=CARTESIAN_POINT('Ctrl Pts',(102.41531823909,1077.77703812473,441.350760055114));
#117573=CARTESIAN_POINT('Ctrl Pts',(102.413024933617,1077.77703071548,441.365260435083));
#117574=CARTESIAN_POINT('Ctrl Pts',(102.408525571024,1077.77694853396,441.397940717941));
#117575=CARTESIAN_POINT('Ctrl Pts',(102.406482085994,1077.77685756898,441.416138424035));
#117576=CARTESIAN_POINT('Ctrl Pts',(102.401855078273,1077.77646055183,441.469290527423));
#117577=CARTESIAN_POINT('Ctrl Pts',(102.400487948646,1077.77603414678,441.504326058925));
#117578=CARTESIAN_POINT('Ctrl Pts',(102.4020877338,1077.7729759697,441.685711092669));
#117579=CARTESIAN_POINT('Ctrl Pts',(102.432600355618,1077.76767656071,441.830237547501));
#117580=CARTESIAN_POINT('Ctrl Pts',(102.536710317238,1077.75353427765,442.071868559446));
#117581=CARTESIAN_POINT('Ctrl Pts',(102.599789433246,1077.74570263645,442.171100762973));
#117582=CARTESIAN_POINT('Ctrl Pts',(102.762352164988,1077.72657612096,442.354530854693));
#117583=CARTESIAN_POINT('Ctrl Pts',(102.863580427146,1077.71515985653,442.434853135299));
#117584=CARTESIAN_POINT('Ctrl Pts',(103.057063159085,1077.69398375268,442.539647893311));
#117585=CARTESIAN_POINT('Ctrl Pts',(103.143009302606,1077.68475074002,442.573089765098));
#117586=CARTESIAN_POINT('Ctrl Pts',(103.319643890586,1077.66608556445,442.617424205756));
#117587=CARTESIAN_POINT('Ctrl Pts',(103.409582050061,1077.6567276048,442.628527441443));
#117588=CARTESIAN_POINT('Ctrl Pts',(103.499860694173,1077.64747802966,442.628504822339));
#117589=CARTESIAN_POINT('',(103.499585384576,1075.67331547342,440.430842584843));
#117590=CARTESIAN_POINT('',(103.499585384595,1067.7251047501,440.430842584843));
#117591=CARTESIAN_POINT('Ctrl Pts',(103.499274463467,1075.63644950196,442.62850481284));
#117592=CARTESIAN_POINT('Ctrl Pts',(103.427257073541,1075.64389599565,442.628484435069));
#117593=CARTESIAN_POINT('Ctrl Pts',(103.355417684151,1075.65141634246,442.621384084784));
#117594=CARTESIAN_POINT('Ctrl Pts',(103.141451896906,1075.67409110447,442.578736761835));
#117595=CARTESIAN_POINT('Ctrl Pts',(103.00516743923,1075.68891256557,442.521836809897));
#117596=CARTESIAN_POINT('Ctrl Pts',(102.76346360034,1075.71605248958,442.358359915889));
#117597=CARTESIAN_POINT('Ctrl Pts',(102.660217219451,1075.72812379484,442.25364715078));
#117598=CARTESIAN_POINT('Ctrl Pts',(102.500503022171,1075.74804648779,442.009784639939));
#117599=CARTESIAN_POINT('Ctrl Pts',(102.445632435157,1075.75570175893,441.873078335723));
#117600=CARTESIAN_POINT('Ctrl Pts',(102.392738789125,1075.76556424131,441.587100897914));
#117601=CARTESIAN_POINT('Ctrl Pts',(102.394806535939,1075.76771622652,441.44082761082));
#117602=CARTESIAN_POINT('Ctrl Pts',(102.455286709802,1075.76629090132,441.158968232738));
#117603=CARTESIAN_POINT('Ctrl Pts',(102.51249188648,1075.76278859546,441.026093096148));
#117604=CARTESIAN_POINT('Ctrl Pts',(102.676073269864,1075.75043099469,440.787688685539));
#117605=CARTESIAN_POINT('Ctrl Pts',(102.781666879871,1075.74160185034,440.685144574812));
#117606=CARTESIAN_POINT('Ctrl Pts',(103.026590908685,1075.71966684757,440.527192912908));
#117607=CARTESIAN_POINT('Ctrl Pts',(103.163525373555,1075.70677087799,440.47341623255));
#117608=CARTESIAN_POINT('Ctrl Pts',(103.377100443955,1075.68573219168,440.435359798528));
#117609=CARTESIAN_POINT('Ctrl Pts',(103.44841135433,1075.67856529576,440.429718598257));
#117610=CARTESIAN_POINT('Ctrl Pts',(103.59134490727,1075.66391272026,440.432341345033));
#117611=CARTESIAN_POINT('Ctrl Pts',(103.662639108214,1075.65645961681,440.440651271714));
#117612=CARTESIAN_POINT('Ctrl Pts',(103.876865904172,1075.63361876489,440.48713891478));
#117613=CARTESIAN_POINT('Ctrl Pts',(104.01340727035,1075.61842751581,440.547205576925));
#117614=CARTESIAN_POINT('Ctrl Pts',(104.25201284105,1075.59062294275,440.715939607113));
#117615=CARTESIAN_POINT('Ctrl Pts',(104.352499763948,1075.57822704031,440.821911344669));
#117616=CARTESIAN_POINT('Ctrl Pts',(104.506254203105,1075.5577670559,441.066252704841));
#117617=CARTESIAN_POINT('Ctrl Pts',(104.558300614325,1075.54987967195,441.202048164075));
#117618=CARTESIAN_POINT('Ctrl Pts',(104.606836644657,1075.53979213193,441.485399575454));
#117619=CARTESIAN_POINT('Ctrl Pts',(104.603175506552,1075.53765998793,441.630062853594));
#117620=CARTESIAN_POINT('Ctrl Pts',(104.540538158766,1075.53946911503,441.909550504499));
#117621=CARTESIAN_POINT('Ctrl Pts',(104.482323453435,1075.54337712613,442.041604688478));
#117622=CARTESIAN_POINT('Ctrl Pts',(104.31847971329,1075.55670754947,442.276249936995));
#117623=CARTESIAN_POINT('Ctrl Pts',(104.214335601615,1075.56601176743,442.376441487126));
#117624=CARTESIAN_POINT('Ctrl Pts',(103.973025804153,1075.58875984639,442.531668586423));
#117625=CARTESIAN_POINT('Ctrl Pts',(103.837984657249,1075.6020071227,442.584925014224));
#117626=CARTESIAN_POINT('Ctrl Pts',(103.631515481982,1075.62285393917,442.622563338287));
#117627=CARTESIAN_POINT('Ctrl Pts',(103.565454977384,1075.62960653279,442.62852353903));
#117628=CARTESIAN_POINT('Ctrl Pts',(103.499274463467,1075.63644950196,442.62850481284));
#117629=CARTESIAN_POINT('Origin',(103.499585384595,1067.7251047501,441.529673720836));
#117630=CARTESIAN_POINT('',(103.499585384595,1075.64701319545,442.028504856828));
#117631=CARTESIAN_POINT('',(103.499585384595,1075.66376111901,441.030842584843));
#117632=CARTESIAN_POINT('Ctrl Pts',(103.499585384595,1075.64701319545,442.028504856828));
#117633=CARTESIAN_POINT('Ctrl Pts',(103.499575443353,1075.64701421976,442.028504856828));
#117634=CARTESIAN_POINT('Ctrl Pts',(103.499565502105,1075.64701524408,442.028504856513));
#117635=CARTESIAN_POINT('Ctrl Pts',(103.466919470037,1075.65037901643,442.028502904697));
#117636=CARTESIAN_POINT('Ctrl Pts',(103.434363758874,1075.65378175874,442.025298132306));
#117637=CARTESIAN_POINT('Ctrl Pts',(103.337113753866,1075.66409266761,442.00597215801));
#117638=CARTESIAN_POINT('Ctrl Pts',(103.275087078802,1075.67087185248,441.980080458876));
#117639=CARTESIAN_POINT('Ctrl Pts',(103.164983052293,1075.68334498511,441.905545705399));
#117640=CARTESIAN_POINT('Ctrl Pts',(103.117939128761,1075.68892082593,441.857700281519));
#117641=CARTESIAN_POINT('Ctrl Pts',(103.045358487654,1075.69812876426,441.74629941969));
#117642=CARTESIAN_POINT('Ctrl Pts',(103.020539627964,1075.70166991111,441.683878905855));
#117643=CARTESIAN_POINT('Ctrl Pts',(102.997142800598,1075.70617246218,441.554390485282));
#117644=CARTESIAN_POINT('Ctrl Pts',(102.998198250127,1075.70714788565,441.488746093747));
#117645=CARTESIAN_POINT('Ctrl Pts',(103.025459847927,1075.70649369283,441.361543849802));
#117646=CARTESIAN_POINT('Ctrl Pts',(103.051389544962,1075.70487101264,441.301253869449));
#117647=CARTESIAN_POINT('Ctrl Pts',(103.125004608819,1075.69920085749,441.193851859608));
#117648=CARTESIAN_POINT('Ctrl Pts',(103.172040786718,1075.69520012457,441.147854409471));
#117649=CARTESIAN_POINT('Ctrl Pts',(103.28218497472,1075.68521075879,441.075809535943));
#117650=CARTESIAN_POINT('Ctrl Pts',(103.34451076681,1075.67928094454,441.050933876175));
#117651=CARTESIAN_POINT('Ctrl Pts',(103.439368402523,1075.66988058255,441.033579969333));
#117652=CARTESIAN_POINT('Ctrl Pts',(103.469341848508,1075.66685978171,441.030855574593));
#117653=CARTESIAN_POINT('Ctrl Pts',(103.499370369833,1075.66378314963,441.030842631183));
#117654=CARTESIAN_POINT('Ctrl Pts',(103.499442041806,1075.66377580633,441.03084260029));
#117655=CARTESIAN_POINT('Ctrl Pts',(103.499513713395,1075.66376846279,441.030842584843));
#117656=CARTESIAN_POINT('Ctrl Pts',(103.499585384595,1075.66376111901,441.030842584843));
#117657=CARTESIAN_POINT('',(103.499585384595,1082.7251047501,441.030842584843));
#117658=CARTESIAN_POINT('',(103.499585384595,1067.7251047501,441.030842584843));
#117659=CARTESIAN_POINT('Origin',(103.499585384595,1082.7251047501,441.529673720836));
#117660=CARTESIAN_POINT('Ctrl Pts',(103.499585384595,1075.66376111901,441.030842584843));
#117661=CARTESIAN_POINT('Ctrl Pts',(103.532060611507,1075.66043354591,441.030842584843));
#117662=CARTESIAN_POINT('Ctrl Pts',(103.564455810833,1075.65705545975,441.034013912775));
#117663=CARTESIAN_POINT('Ctrl Pts',(103.661850094858,1075.64671898749,441.053264220225));
#117664=CARTESIAN_POINT('Ctrl Pts',(103.724152924491,1075.6398520434,441.079259655313));
#117665=CARTESIAN_POINT('Ctrl Pts',(103.834235296593,1075.62719741521,441.153887815884));
#117666=CARTESIAN_POINT('Ctrl Pts',(103.881103112898,1075.62152146925,441.201547987854));
#117667=CARTESIAN_POINT('Ctrl Pts',(103.952997527745,1075.61216832407,441.311701420194));
#117668=CARTESIAN_POINT('Ctrl Pts',(103.977634544781,1075.60855460844,441.372897386145));
#117669=CARTESIAN_POINT('Ctrl Pts',(104.001826508974,1075.60384253857,441.50108260297));
#117670=CARTESIAN_POINT('Ctrl Pts',(104.001275424936,1075.60277788747,441.566767408293));
#117671=CARTESIAN_POINT('Ctrl Pts',(103.974984361348,1075.60335067882,441.694141624082));
#117672=CARTESIAN_POINT('Ctrl Pts',(103.949551691095,1075.60497755678,441.75456574776));
#117673=CARTESIAN_POINT('Ctrl Pts',(103.876901269081,1075.61072008804,441.862396457139));
#117674=CARTESIAN_POINT('Ctrl Pts',(103.830337481106,1075.6147859128,441.908697009938));
#117675=CARTESIAN_POINT('Ctrl Pts',(103.721868130933,1075.62483343728,441.9810013349));
#117676=CARTESIAN_POINT('Ctrl Pts',(103.660922918955,1075.63072855163,442.00618346961));
#117677=CARTESIAN_POINT('Ctrl Pts',(103.564858078166,1075.64033609418,442.025295009983));
#117678=CARTESIAN_POINT('Ctrl Pts',(103.532257199036,1075.64364679602,442.028504856828));
#117679=CARTESIAN_POINT('Ctrl Pts',(103.499585384595,1075.64701319545,442.028504856828));
#117680=CARTESIAN_POINT('Origin',(107.832717977554,1067.7251047501,454.828467536887));
#117681=CARTESIAN_POINT('',(107.832717977553,1076.85914687694,453.73792678816));
#117682=CARTESIAN_POINT('Ctrl Pts',(107.832971536831,1076.78010498484,455.919008256138));
#117683=CARTESIAN_POINT('Ctrl Pts',(107.976293244521,1076.76145240728,455.918974932716));
#117684=CARTESIAN_POINT('Ctrl Pts',(108.118399363473,1076.74390174584,455.890688248432));
#117685=CARTESIAN_POINT('Ctrl Pts',(108.37179267808,1076.71451997644,455.785420615026));
#117686=CARTESIAN_POINT('Ctrl Pts',(108.482684606891,1076.70255123353,455.71391068143));
#117687=CARTESIAN_POINT('Ctrl Pts',(108.679564754118,1076.68339266947,455.529442953307));
#117688=CARTESIAN_POINT('Ctrl Pts',(108.76187320898,1076.67670328487,455.416064819364));
#117689=CARTESIAN_POINT('Ctrl Pts',(108.833425746483,1076.67291107026,455.262937671884));
#117690=CARTESIAN_POINT('Ctrl Pts',(108.845007218833,1076.67240572149,455.235224438535));
#117691=CARTESIAN_POINT('Ctrl Pts',(108.861958322215,1076.67185990988,455.189434183184));
#117692=CARTESIAN_POINT('Ctrl Pts',(108.868028563725,1076.67171637646,455.171636064354));
#117693=CARTESIAN_POINT('Ctrl Pts',(108.877981463478,1076.67158017788,455.139780425035));
#117694=CARTESIAN_POINT('Ctrl Pts',(108.882047957335,1076.67156084973,455.125785662428));
#117695=CARTESIAN_POINT('Ctrl Pts',(108.889968807407,1076.67160443307,455.09633576917));
#117696=CARTESIAN_POINT('Ctrl Pts',(108.893767450016,1076.67167513581,455.080869424165));
#117697=CARTESIAN_POINT('Ctrl Pts',(108.902759896149,1076.67198347318,455.040454799156));
#117698=CARTESIAN_POINT('Ctrl Pts',(108.907420149256,1076.67229571784,455.015399081513));
#117699=CARTESIAN_POINT('Ctrl Pts',(108.923198026648,1076.67410834938,454.910190488869));
#117700=CARTESIAN_POINT('Ctrl Pts',(108.926250263164,1076.67670990839,454.829127156987));
#117701=CARTESIAN_POINT('Ctrl Pts',(108.912698862536,1076.68532799887,454.644795911623));
#117702=CARTESIAN_POINT('Ctrl Pts',(108.890287235635,1076.69206269198,454.542818239556));
#117703=CARTESIAN_POINT('Ctrl Pts',(108.812358334415,1076.71000836084,454.33494918969));
#117704=CARTESIAN_POINT('Ctrl Pts',(108.753195588104,1076.72158975816,454.231895257354));
#117705=CARTESIAN_POINT('Ctrl Pts',(108.597336430079,1076.74906156974,454.040231380331));
#117706=CARTESIAN_POINT('Ctrl Pts',(108.498800674608,1076.76504438467,453.955416786063));
#117707=CARTESIAN_POINT('Ctrl Pts',(108.268110439784,1076.80003438503,453.818973439859));
#117708=CARTESIAN_POINT('Ctrl Pts',(108.135890091922,1076.81887779136,453.771717561882));
#117709=CARTESIAN_POINT('Ctrl Pts',(107.855266020332,1076.85661706485,453.728587014278));
#117710=CARTESIAN_POINT('Ctrl Pts',(107.709041231693,1076.87513160685,453.735290159195));
#117711=CARTESIAN_POINT('Ctrl Pts',(107.433875004523,1076.90781956673,453.804067820478));
#117712=CARTESIAN_POINT('Ctrl Pts',(107.306889381564,1076.92186363973,453.863016890868));
#117713=CARTESIAN_POINT('Ctrl Pts',(107.093475367213,1076.94345106512,454.017143888293));
#117714=CARTESIAN_POINT('Ctrl Pts',(107.005775803873,1076.95136420361,454.106687994877));
#117715=CARTESIAN_POINT('Ctrl Pts',(106.892531043737,1076.95985674309,454.270855283648));
#117716=CARTESIAN_POINT('Ctrl Pts',(106.856465869863,1076.9620786582,454.336712183565));
#117717=CARTESIAN_POINT('Ctrl Pts',(106.817521675084,1076.96371792995,454.429332414074));
#117718=CARTESIAN_POINT('Ctrl Pts',(106.808445806467,1076.9640180105,454.453235549723));
#117719=CARTESIAN_POINT('Ctrl Pts',(106.795113662979,1076.96431392402,454.492449893638));
#117720=CARTESIAN_POINT('Ctrl Pts',(106.790337472132,1076.96438197488,454.507572746395));
#117721=CARTESIAN_POINT('Ctrl Pts',(106.781848177851,1076.96442545437,454.536645673666));
#117722=CARTESIAN_POINT('Ctrl Pts',(106.778078965015,1076.96440866715,454.550575672544));
#117723=CARTESIAN_POINT('Ctrl Pts',(106.770110107113,1076.96428478677,454.582528587587));
#117724=CARTESIAN_POINT('Ctrl Pts',(106.766090614728,1076.96415356452,454.600591490269));
#117725=CARTESIAN_POINT('Ctrl Pts',(106.755297878057,1076.96356896003,454.655665996039));
#117726=CARTESIAN_POINT('Ctrl Pts',(106.74997914225,1076.96292322275,454.692930011779));
#117727=CARTESIAN_POINT('Ctrl Pts',(106.73359348296,1076.95857765652,454.874386330028));
#117728=CARTESIAN_POINT('Ctrl Pts',(106.749367691084,1076.9514635675,455.01937028733));
#117729=CARTESIAN_POINT('Ctrl Pts',(106.827870501434,1076.93270628244,455.267901842644));
#117730=CARTESIAN_POINT('Ctrl Pts',(106.880406277064,1076.92232823087,455.372390030318));
#117731=CARTESIAN_POINT('Ctrl Pts',(107.023110276428,1076.89710289102,455.570194855512));
#117732=CARTESIAN_POINT('Ctrl Pts',(107.115460432949,1076.88210142741,455.659781991592));
#117733=CARTESIAN_POINT('Ctrl Pts',(107.311017983575,1076.85224734,455.792273036469));
#117734=CARTESIAN_POINT('Ctrl Pts',(107.409562028757,1076.83785939066,455.839411681416));
#117735=CARTESIAN_POINT('Ctrl Pts',(107.616921296845,1076.80876215893,455.902914512555));
#117736=CARTESIAN_POINT('Ctrl Pts',(107.724632667405,1076.79420472728,455.919033445776));
#117737=CARTESIAN_POINT('Ctrl Pts',(107.832971536831,1076.78010498484,455.919008256138));
#117738=CARTESIAN_POINT('',(107.832717977524,1074.84120620429,453.737926788159));
#117739=CARTESIAN_POINT('',(107.832717977554,1067.7251047501,453.737926788159));
#117740=CARTESIAN_POINT('Ctrl Pts',(107.832913167154,1074.76151756941,455.919008268147));
#117741=CARTESIAN_POINT('Ctrl Pts',(107.761364680361,1074.77090615704,455.919021074199));
#117742=CARTESIAN_POINT('Ctrl Pts',(107.690007241569,1074.7805072353,455.911992639033));
#117743=CARTESIAN_POINT('Ctrl Pts',(107.549993601512,1074.79981575487,455.884129554535));
#117744=CARTESIAN_POINT('Ctrl Pts',(107.481641060263,1074.80947954401,455.863408111629));
#117745=CARTESIAN_POINT('Ctrl Pts',(107.282079838548,1074.83843075412,455.780842033004));
#117746=CARTESIAN_POINT('Ctrl Pts',(107.1605628438,1074.85709833395,455.699395202276));
#117747=CARTESIAN_POINT('Ctrl Pts',(106.956789546625,1074.89075928502,455.493949390514));
#117748=CARTESIAN_POINT('Ctrl Pts',(106.876320330313,1074.9054469374,455.372119822143));
#117749=CARTESIAN_POINT('Ctrl Pts',(106.767561384308,1074.92896688559,455.103616175412));
#117750=CARTESIAN_POINT('Ctrl Pts',(106.740399210943,1074.93755992791,454.959669784576));
#117751=CARTESIAN_POINT('Ctrl Pts',(106.744089173054,1074.94731695781,454.67282620598));
#117752=CARTESIAN_POINT('Ctrl Pts',(106.773480886195,1074.94856290909,454.532882477924));
#117753=CARTESIAN_POINT('Ctrl Pts',(106.884264397555,1074.94377444183,454.271823333038));
#117754=CARTESIAN_POINT('Ctrl Pts',(106.964608960224,1074.93777693391,454.153392027821));
#117755=CARTESIAN_POINT('Ctrl Pts',(107.168200687902,1074.91901003619,453.951710582853));
#117756=CARTESIAN_POINT('Ctrl Pts',(107.290291937445,1074.90627884597,453.87142850615));
#117757=CARTESIAN_POINT('Ctrl Pts',(107.558549872016,1074.87572560015,453.763059868814));
#117758=CARTESIAN_POINT('Ctrl Pts',(107.702131789146,1074.85818938898,453.736178496687));
#117759=CARTESIAN_POINT('Ctrl Pts',(107.917463658781,1074.83019045815,453.738916049534));
#117760=CARTESIAN_POINT('Ctrl Pts',(107.988067088475,1074.82073763901,453.746726052469));
#117761=CARTESIAN_POINT('Ctrl Pts',(108.12696748848,1074.80158989798,453.775969661687));
#117762=CARTESIAN_POINT('Ctrl Pts',(108.194945731411,1074.79193686762,453.797387563067));
#117763=CARTESIAN_POINT('Ctrl Pts',(108.395041151581,1074.76264162941,453.882682931718));
#117764=CARTESIAN_POINT('Ctrl Pts',(108.516929903128,1074.7435246556,453.966693540862));
#117765=CARTESIAN_POINT('Ctrl Pts',(108.718078675198,1074.70925152903,454.175788192346));
#117766=CARTESIAN_POINT('Ctrl Pts',(108.796325451983,1074.69434260757,454.297946150964));
#117767=CARTESIAN_POINT('Ctrl Pts',(108.900425519118,1074.67058456738,454.564710628252));
#117768=CARTESIAN_POINT('Ctrl Pts',(108.925782033253,1074.66191095239,454.706449742708));
#117769=CARTESIAN_POINT('Ctrl Pts',(108.920362005906,1074.65200819628,454.990860435801));
#117770=CARTESIAN_POINT('Ctrl Pts',(108.890099436397,1074.65082000139,455.130630123571));
#117771=CARTESIAN_POINT('Ctrl Pts',(108.777834792077,1074.65607970017,455.390664360931));
#117772=CARTESIAN_POINT('Ctrl Pts',(108.697039268529,1074.66246419161,455.508302532283));
#117773=CARTESIAN_POINT('Ctrl Pts',(108.494652339104,1074.68199695735,455.706727884768));
#117774=CARTESIAN_POINT('Ctrl Pts',(108.37480824893,1074.69499371989,455.785286066671));
#117775=CARTESIAN_POINT('Ctrl Pts',(108.112958319505,1074.72568614054,455.891770153792));
#117776=CARTESIAN_POINT('Ctrl Pts',(107.973506051147,1074.74306898062,455.918983104237));
#117777=CARTESIAN_POINT('Ctrl Pts',(107.832913167154,1074.76151756941,455.919008268147));
#117778=CARTESIAN_POINT('Origin',(107.832717977554,1067.7251047501,454.828467536887));
#117779=CARTESIAN_POINT('',(107.832717977554,1074.78413642061,455.319008285615));
#117780=CARTESIAN_POINT('',(107.832717977554,1074.8199670159,454.337926788159));
#117781=CARTESIAN_POINT('Ctrl Pts',(107.832717977554,1074.78413642061,455.319008285615));
#117782=CARTESIAN_POINT('Ctrl Pts',(107.80132417306,1074.78824117862,455.319008285615));
#117783=CARTESIAN_POINT('Ctrl Pts',(107.77001005431,1074.79244177835,455.315994575158));
#117784=CARTESIAN_POINT('Ctrl Pts',(107.707766885313,1074.80100537068,455.303907485118));
#117785=CARTESIAN_POINT('Ctrl Pts',(107.676999512641,1074.80535060123,455.294737716767));
#117786=CARTESIAN_POINT('Ctrl Pts',(107.586891108525,1074.81842493241,455.257958976559));
#117787=CARTESIAN_POINT('Ctrl Pts',(107.531906586075,1074.82689694455,455.221435086252));
#117788=CARTESIAN_POINT('Ctrl Pts',(107.439558776845,1074.84222992862,455.128988095712));
#117789=CARTESIAN_POINT('Ctrl Pts',(107.403041771232,1074.84894717126,455.074014804486));
#117790=CARTESIAN_POINT('Ctrl Pts',(107.354029797519,1074.85964148896,454.953589742402));
#117791=CARTESIAN_POINT('Ctrl Pts',(107.341703043795,1074.86354839834,454.889494764361));
#117792=CARTESIAN_POINT('Ctrl Pts',(107.342671627679,1074.86806437088,454.761060606083));
#117793=CARTESIAN_POINT('Ctrl Pts',(107.355558844303,1074.868678798,454.698037234446));
#117794=CARTESIAN_POINT('Ctrl Pts',(107.404752322777,1074.8665853144,454.580387569291));
#117795=CARTESIAN_POINT('Ctrl Pts',(107.440572432291,1074.86389653181,454.526963801322));
#117796=CARTESIAN_POINT('Ctrl Pts',(107.530841728602,1074.85551182968,454.43653428028));
#117797=CARTESIAN_POINT('Ctrl Pts',(107.584516325315,1074.84987837628,454.400553573597));
#117798=CARTESIAN_POINT('Ctrl Pts',(107.703501609517,1074.83627639932,454.350799989405));
#117799=CARTESIAN_POINT('Ctrl Pts',(107.767834298285,1074.82840098098,454.337926788159));
#117800=CARTESIAN_POINT('Ctrl Pts',(107.832717977554,1074.8199670159,454.337926788159));
#117801=CARTESIAN_POINT('',(107.832717977554,1082.7251047501,454.337926788159));
#117802=CARTESIAN_POINT('',(107.832717977554,1067.7251047501,454.337926788159));
#117803=CARTESIAN_POINT('Origin',(107.832717977554,1082.7251047501,454.828467536887));
#117804=CARTESIAN_POINT('Ctrl Pts',(107.832717977554,1074.8199670159,454.337926788159));
#117805=CARTESIAN_POINT('Ctrl Pts',(107.832731662808,1074.81996523701,454.337926788159));
#117806=CARTESIAN_POINT('Ctrl Pts',(107.832745348086,1074.81996345809,454.337926788733));
#117807=CARTESIAN_POINT('Ctrl Pts',(107.832759033389,1074.81996167915,454.337926789878));
#117808=CARTESIAN_POINT('Ctrl Pts',(107.864720572838,1074.81580702779,454.337929464901));
#117809=CARTESIAN_POINT('Ctrl Pts',(107.896595272592,1074.81154558869,454.341055820378));
#117810=CARTESIAN_POINT('Ctrl Pts',(107.959313103048,1074.80292319969,454.353465016089));
#117811=CARTESIAN_POINT('Ctrl Pts',(107.990014750329,1074.79858131692,454.362729932292));
#117812=CARTESIAN_POINT('Ctrl Pts',(108.080279548172,1074.78543850234,454.399922020564));
#117813=CARTESIAN_POINT('Ctrl Pts',(108.135392458427,1074.77687321478,454.436877219524));
#117814=CARTESIAN_POINT('Ctrl Pts',(108.22728102955,1074.76141574975,454.52985399325));
#117815=CARTESIAN_POINT('Ctrl Pts',(108.263391166522,1074.75465297741,454.584748587818));
#117816=CARTESIAN_POINT('Ctrl Pts',(108.311662403432,1074.74389147749,454.70460246635));
#117817=CARTESIAN_POINT('Ctrl Pts',(108.323757055971,1074.73995263477,454.768191978922));
#117818=CARTESIAN_POINT('Ctrl Pts',(108.322732874622,1074.73536732846,454.896108010189));
#117819=CARTESIAN_POINT('Ctrl Pts',(108.30981429028,1074.73474283866,454.959130700503));
#117820=CARTESIAN_POINT('Ctrl Pts',(108.260588473304,1074.73688951362,455.076692195476));
#117821=CARTESIAN_POINT('Ctrl Pts',(108.224798394672,1074.73963642042,455.130039055872));
#117822=CARTESIAN_POINT('Ctrl Pts',(108.134656224412,1074.748169808,455.22033612801));
#117823=CARTESIAN_POINT('Ctrl Pts',(108.081081628074,1074.7538909484,455.256271530422));
#117824=CARTESIAN_POINT('Ctrl Pts',(107.962788666784,1074.76759438969,455.305820312635));
#117825=CARTESIAN_POINT('Ctrl Pts',(107.899100568906,1074.77546674313,455.318728063144));
#117826=CARTESIAN_POINT('Ctrl Pts',(107.834120646257,1074.78395307392,455.319006781636));
#117827=CARTESIAN_POINT('Ctrl Pts',(107.833419292021,1074.78404472334,455.319008285615));
#117828=CARTESIAN_POINT('Ctrl Pts',(107.832717977554,1074.78413642061,455.319008285615));
#117829=CARTESIAN_POINT('Origin',(86.323060185316,1067.7251047501,400.766404126158));
#117830=CARTESIAN_POINT('',(86.3230601853348,1078.66271960918,399.288100993964));
#117831=CARTESIAN_POINT('Ctrl Pts',(86.3231885187679,1078.68302856617,402.244707252781));
#117832=CARTESIAN_POINT('Ctrl Pts',(86.511377124993,1078.67873167388,402.244690915879));
#117833=CARTESIAN_POINT('Ctrl Pts',(86.6978340159513,1078.67397014017,402.208740216216));
#117834=CARTESIAN_POINT('Ctrl Pts',(87.0536990953585,1078.66381065772,402.066262785444));
#117835=CARTESIAN_POINT('Ctrl Pts',(87.2187302999287,1078.65849687174,401.95856262917));
#117836=CARTESIAN_POINT('Ctrl Pts',(87.4924700757981,1078.64859018114,401.690140995185));
#117837=CARTESIAN_POINT('Ctrl Pts',(87.6004762133578,1078.64407489731,401.533884827865));
#117838=CARTESIAN_POINT('Ctrl Pts',(87.7457832568328,1078.63684031022,401.203503049251));
#117839=CARTESIAN_POINT('Ctrl Pts',(87.7870777909925,1078.63406309525,401.034465919139));
#117840=CARTESIAN_POINT('Ctrl Pts',(87.8046994174545,1078.63111786495,400.762906393987));
#117841=CARTESIAN_POINT('Ctrl Pts',(87.8011109419465,1078.63034964539,400.66328299183));
#117842=CARTESIAN_POINT('Ctrl Pts',(87.7824754248551,1078.62974695291,400.527928373313));
#117843=CARTESIAN_POINT('Ctrl Pts',(87.776013699419,1078.62962913559,400.491286635201));
#117844=CARTESIAN_POINT('Ctrl Pts',(87.7631011112122,1078.62951198781,400.43137780273));
#117845=CARTESIAN_POINT('Ctrl Pts',(87.7574503625128,1078.62948555144,400.407955625885));
#117846=CARTESIAN_POINT('Ctrl Pts',(87.7453884988887,1078.62947240838,400.362827544823));
#117847=CARTESIAN_POINT('Ctrl Pts',(87.7390463566941,1078.62948337884,400.341110051006));
#117848=CARTESIAN_POINT('Ctrl Pts',(87.7231399691271,1078.62954918519,400.290949855368));
#117849=CARTESIAN_POINT('Ctrl Pts',(87.7132032005472,1078.62961714908,400.262635772914));
#117850=CARTESIAN_POINT('Ctrl Pts',(87.6792290728415,1078.62992641556,400.174509103744));
#117851=CARTESIAN_POINT('Ctrl Pts',(87.6521388856902,1078.63027691097,400.115955521755));
#117852=CARTESIAN_POINT('Ctrl Pts',(87.5272739895007,1078.63224469689,399.886682816148));
#117853=CARTESIAN_POINT('Ctrl Pts',(87.3997291574734,1078.63497295119,399.734506182838));
#117854=CARTESIAN_POINT('Ctrl Pts',(87.1210596675006,1078.64166554795,399.511718491457));
#117855=CARTESIAN_POINT('Ctrl Pts',(86.9805224613034,1078.64525865084,399.432696435072));
#117856=CARTESIAN_POINT('Ctrl Pts',(86.6665992891594,1078.6534933482,399.318078559461));
#117857=CARTESIAN_POINT('Ctrl Pts',(86.4938682118272,1078.65813069637,399.287726539262));
#117858=CARTESIAN_POINT('Ctrl Pts',(86.1332105510088,1078.6678200902,399.288509831046));
#117859=CARTESIAN_POINT('Ctrl Pts',(85.9483204421648,1078.67278681185,399.32425700736));
#117860=CARTESIAN_POINT('Ctrl Pts',(85.5935550584435,1078.68225291729,399.465881124098));
#117861=CARTESIAN_POINT('Ctrl Pts',(85.4282673175356,1078.68662673938,399.573553508469));
#117862=CARTESIAN_POINT('Ctrl Pts',(85.153666317123,1078.69400196367,399.84248969958));
#117863=CARTESIAN_POINT('Ctrl Pts',(85.0452372845045,1078.69698172471,399.999412656643));
#117864=CARTESIAN_POINT('Ctrl Pts',(84.8998834356383,1078.70144204265,400.330738224604));
#117865=CARTESIAN_POINT('Ctrl Pts',(84.8587408193982,1078.70300006463,400.499929000067));
#117866=CARTESIAN_POINT('Ctrl Pts',(84.8414343245999,1078.70461262791,400.771480271008));
#117867=CARTESIAN_POINT('Ctrl Pts',(84.8451197289468,1078.70502006977,400.870966338669));
#117868=CARTESIAN_POINT('Ctrl Pts',(84.863816927806,1078.70533761821,401.005885381117));
#117869=CARTESIAN_POINT('Ctrl Pts',(84.8702500342564,1078.70539915638,401.042238908333));
#117870=CARTESIAN_POINT('Ctrl Pts',(84.8830600391271,1078.70546027805,401.101585490668));
#117871=CARTESIAN_POINT('Ctrl Pts',(84.8886447678288,1078.70547408537,401.124732716756));
#117872=CARTESIAN_POINT('Ctrl Pts',(84.9005335922015,1078.70548116609,401.169262293854));
#117873=CARTESIAN_POINT('Ctrl Pts',(84.9067670820064,1078.70547569812,401.190656947926));
#117874=CARTESIAN_POINT('Ctrl Pts',(84.9223508278997,1078.7054423641,401.239964673893));
#117875=CARTESIAN_POINT('Ctrl Pts',(84.9320559174966,1078.70540788476,401.267755720552));
#117876=CARTESIAN_POINT('Ctrl Pts',(84.9650280379881,1078.70525120238,401.353826576474));
#117877=CARTESIAN_POINT('Ctrl Pts',(84.9911789878627,1078.70507413942,401.41092633258));
#117878=CARTESIAN_POINT('Ctrl Pts',(85.1138777067444,1078.70404785706,401.639247301699));
#117879=CARTESIAN_POINT('Ctrl Pts',(85.2404466466818,1078.70258809057,401.792036317088));
#117880=CARTESIAN_POINT('Ctrl Pts',(85.5180154432927,1078.69859591862,402.016634821358));
#117881=CARTESIAN_POINT('Ctrl Pts',(85.6584935110152,1078.69632929459,402.096637478305));
#117882=CARTESIAN_POINT('Ctrl Pts',(85.9736132389365,1078.69057521564,402.213493079599));
#117883=CARTESIAN_POINT('Ctrl Pts',(86.1477101532214,1078.68703524676,402.24472248629));
#117884=CARTESIAN_POINT('Ctrl Pts',(86.3231885187679,1078.68302856617,402.244707252781));
#117885=CARTESIAN_POINT('',(86.3230601852944,1076.66188598601,399.288100993964));
#117886=CARTESIAN_POINT('',(86.323060185316,1067.7251047501,399.288100993964));
#117887=CARTESIAN_POINT('',(86.323060185316,1076.68243856932,402.244707258351));
#117888=CARTESIAN_POINT('Ctrl Pts',(86.323060185316,1076.68243856932,402.244707258351));
#117889=CARTESIAN_POINT('Ctrl Pts',(86.2781747730325,1076.68347561579,402.244707258351));
#117890=CARTESIAN_POINT('Ctrl Pts',(86.2336323361814,1076.68447645497,402.242667270048));
#117891=CARTESIAN_POINT('Ctrl Pts',(86.1894286980019,1076.68544312929,402.238655047791));
#117892=CARTESIAN_POINT('Ctrl Pts',(86.1447882829812,1076.68641935534,402.234603180704));
#117893=CARTESIAN_POINT('Ctrl Pts',(86.1004924641547,1076.68736073805,402.228539911076));
#117894=CARTESIAN_POINT('Ctrl Pts',(86.0565337239154,1076.688269381,402.220482458307));
#117895=CARTESIAN_POINT('Ctrl Pts',(86.049311585819,1076.68841866519,402.219158670676));
#117896=CARTESIAN_POINT('Ctrl Pts',(86.0420985572702,1076.68856706566,402.217780941709));
#117897=CARTESIAN_POINT('Ctrl Pts',(86.0348946237282,1076.68871459173,402.216349214693));
#117898=CARTESIAN_POINT('Ctrl Pts',(85.996765109473,1076.68949542867,402.208771263655));
#117899=CARTESIAN_POINT('Ctrl Pts',(85.958725481398,1076.69025451741,402.199643312767));
#117900=CARTESIAN_POINT('Ctrl Pts',(85.92103295674,1076.69098826324,402.188991296821));
#117901=CARTESIAN_POINT('Ctrl Pts',(85.8833768031073,1076.69172130105,402.178349559432));
#117902=CARTESIAN_POINT('Ctrl Pts',(85.846067682979,1076.69242904483,402.166186817494));
#117903=CARTESIAN_POINT('Ctrl Pts',(85.8093508310832,1076.69310791027,402.152579746354));
#117904=CARTESIAN_POINT('Ctrl Pts',(85.791761404465,1076.6934331248,402.146061197869));
#117905=CARTESIAN_POINT('Ctrl Pts',(85.7743076779248,1076.69375171191,402.139211922037));
#117906=CARTESIAN_POINT('Ctrl Pts',(85.7570150942891,1076.69406327753,402.132044307749));
#117907=CARTESIAN_POINT('Ctrl Pts',(85.7152840314043,1076.69481515849,402.114747172231));
#117908=CARTESIAN_POINT('Ctrl Pts',(85.6745594924959,1076.6955259268,402.095630482121));
#117909=CARTESIAN_POINT('Ctrl Pts',(85.6348252209055,1076.69619803782,402.0747285448));
#117910=CARTESIAN_POINT('Ctrl Pts',(85.5949967567797,1076.69687174212,402.053777058151));
#117911=CARTESIAN_POINT('Ctrl Pts',(85.5561624134356,1076.69750660564,402.031031427587));
#117912=CARTESIAN_POINT('Ctrl Pts',(85.5183279992,1076.69810510126,402.006479228432));
#117913=CARTESIAN_POINT('Ctrl Pts',(85.5129365550676,1076.69819038752,402.002980514028));
#117914=CARTESIAN_POINT('Ctrl Pts',(85.5075654650637,1076.69827493527,401.999445043196));
#117915=CARTESIAN_POINT('Ctrl Pts',(85.5022147979378,1076.69835875168,401.99587271082));
#117916=CARTESIAN_POINT('Ctrl Pts',(85.4720809220624,1076.69883078871,401.975754056855));
#117917=CARTESIAN_POINT('Ctrl Pts',(85.4425301022561,1076.69927989956,401.954417787375));
#117918=CARTESIAN_POINT('Ctrl Pts',(85.4137805664492,1076.69970448713,401.931990127003));
#117919=CARTESIAN_POINT('Ctrl Pts',(85.3850243052947,1076.70012917403,401.909557220153));
#117920=CARTESIAN_POINT('Ctrl Pts',(85.3570701847616,1076.70052932618,401.886032751249));
#117921=CARTESIAN_POINT('Ctrl Pts',(85.3301054815449,1076.70090334536,401.861584981958));
#117922=CARTESIAN_POINT('Ctrl Pts',(85.3121382809558,1076.70115256293,401.845294872207));
#117923=CARTESIAN_POINT('Ctrl Pts',(85.2946097069164,1076.70139017782,401.828595697225));
#117924=CARTESIAN_POINT('Ctrl Pts',(85.2775660305127,1076.70161571723,401.811546280568));
#117925=CARTESIAN_POINT('Ctrl Pts',(85.2424743437808,1076.70208008641,401.776442775073));
#117926=CARTESIAN_POINT('Ctrl Pts',(85.2090706729493,1076.70249853921,401.73948581198));
#117927=CARTESIAN_POINT('Ctrl Pts',(85.1775876281939,1076.70287118893,401.700894774336));
#117928=CARTESIAN_POINT('Ctrl Pts',(85.1461227436608,1076.70324362368,401.662325996986));
#117929=CARTESIAN_POINT('Ctrl Pts',(85.1165766905558,1076.70357030818,401.622125482738));
#117930=CARTESIAN_POINT('Ctrl Pts',(85.0891433844455,1076.70385135552,401.580547528257));
#117931=CARTESIAN_POINT('Ctrl Pts',(85.0616894197992,1076.7041326145,401.538938263673));
#117932=CARTESIAN_POINT('Ctrl Pts',(85.0363517220966,1076.70436816757,401.495950004178));
#117933=CARTESIAN_POINT('Ctrl Pts',(85.0132805743846,1076.70455812808,401.451865665152));
#117934=CARTESIAN_POINT('Ctrl Pts',(84.9928181668511,1076.70472660905,401.412766105727));
#117935=CARTESIAN_POINT('Ctrl Pts',(84.9741381915511,1076.70485922517,401.372804988911));
#117936=CARTESIAN_POINT('Ctrl Pts',(84.9573137963501,1076.70495605553,401.332192913321));
#117937=CARTESIAN_POINT('Ctrl Pts',(84.9384373945459,1076.70506469592,401.286627539482));
#117938=CARTESIAN_POINT('Ctrl Pts',(84.9217916099113,1076.70512901854,401.23998628075));
#117939=CARTESIAN_POINT('Ctrl Pts',(84.9075126608846,1076.70514893364,401.192555926258));
#117940=CARTESIAN_POINT('Ctrl Pts',(84.8932441338425,1076.70516883421,401.14516019045));
#117941=CARTESIAN_POINT('Ctrl Pts',(84.8813392198776,1076.70514439207,401.096977085023));
#117942=CARTESIAN_POINT('Ctrl Pts',(84.8718854375303,1076.70507551768,401.04831191612));
#117943=CARTESIAN_POINT('Ctrl Pts',(84.8624265602351,1076.70500660617,400.999620519991));
#117944=CARTESIAN_POINT('Ctrl Pts',(84.8554215850028,1076.7048932145,400.950447149187));
#117945=CARTESIAN_POINT('Ctrl Pts',(84.8509069838721,1076.70473525298,400.901107883088));
#117946=CARTESIAN_POINT('Ctrl Pts',(84.8468157491852,1076.70459210465,400.856395512925));
#117947=CARTESIAN_POINT('Ctrl Pts',(84.8447690760854,1076.70441235379,400.811547360364));
#117948=CARTESIAN_POINT('Ctrl Pts',(84.8447571060139,1076.70419593364,400.766799573503));
#117949=CARTESIAN_POINT('Ctrl Pts',(84.8447473670697,1076.70401985251,400.730392422381));
#117950=CARTESIAN_POINT('Ctrl Pts',(84.8460868290201,1076.70381787846,400.693768275429));
#117951=CARTESIAN_POINT('Ctrl Pts',(84.8487976378466,1076.70359075187,400.65717916664));
#117952=CARTESIAN_POINT('Ctrl Pts',(84.8515071072191,1076.70336373751,400.620608137115));
#117953=CARTESIAN_POINT('Ctrl Pts',(84.8555865653958,1076.70311159546,400.584072701866));
#117954=CARTESIAN_POINT('Ctrl Pts',(84.8610060230901,1076.702835065,400.547822842946));
#117955=CARTESIAN_POINT('Ctrl Pts',(84.8645262241826,1076.70265544504,400.524276798273));
#117956=CARTESIAN_POINT('Ctrl Pts',(84.8686107167369,1076.70246553528,400.50085118465));
#117957=CARTESIAN_POINT('Ctrl Pts',(84.8732396922764,1076.70226553832,400.477612352357));
#117958=CARTESIAN_POINT('Ctrl Pts',(84.8820608692554,1076.70188441544,400.433327423501));
#117959=CARTESIAN_POINT('Ctrl Pts',(84.8928711226574,1076.70146702708,400.389624982645));
#117960=CARTESIAN_POINT('Ctrl Pts',(84.9056472680785,1076.7010111334,400.346498454964));
#117961=CARTESIAN_POINT('Ctrl Pts',(84.9184092539294,1076.70055574497,400.303419723631));
#117962=CARTESIAN_POINT('Ctrl Pts',(84.9331330539135,1076.70006193652,400.260914727335));
#117963=CARTESIAN_POINT('Ctrl Pts',(84.9498449798141,1076.69952747563,400.218991895722));
#117964=CARTESIAN_POINT('Ctrl Pts',(84.952221111862,1076.699451485,400.213031231204));
#117965=CARTESIAN_POINT('Ctrl Pts',(84.9546375125551,1076.69937467257,400.207082373412));
#117966=CARTESIAN_POINT('Ctrl Pts',(84.9570943332091,1076.69929703189,400.201145387587));
#117967=CARTESIAN_POINT('Ctrl Pts',(84.9717199476879,1076.69883483188,400.165802121608));
#117968=CARTESIAN_POINT('Ctrl Pts',(84.9877730909188,1076.69834274521,400.130902979445));
#117969=CARTESIAN_POINT('Ctrl Pts',(85.0051613822483,1076.69782306189,400.096685606535));
#117970=CARTESIAN_POINT('Ctrl Pts',(85.0225647163828,1076.69730292899,400.062438631794));
#117971=CARTESIAN_POINT('Ctrl Pts',(85.0413052391773,1076.69675515167,400.028875150433));
#117972=CARTESIAN_POINT('Ctrl Pts',(85.0612437929392,1076.69618202591,399.996209642549));
#117973=CARTESIAN_POINT('Ctrl Pts',(85.0718285068446,1076.69587777253,399.97886861272));
#117974=CARTESIAN_POINT('Ctrl Pts',(85.0827500869924,1076.69556637547,399.961780196826));
#117975=CARTESIAN_POINT('Ctrl Pts',(85.0939828637915,1076.69524817822,399.94497300405));
#117976=CARTESIAN_POINT('Ctrl Pts',(85.1188605168078,1076.69454345481,399.907749482428));
#117977=CARTESIAN_POINT('Ctrl Pts',(85.1453867556051,1076.69380278896,399.871711793279));
#117978=CARTESIAN_POINT('Ctrl Pts',(85.1735698409287,1076.69302336567,399.836860098791));
#117979=CARTESIAN_POINT('Ctrl Pts',(85.2015102136936,1076.69225065478,399.802308546884));
#117980=CARTESIAN_POINT('Ctrl Pts',(85.2310796490996,1076.69143985114,399.768921984926));
#117981=CARTESIAN_POINT('Ctrl Pts',(85.2623219763971,1076.69058821188,399.736736897005));
#117982=CARTESIAN_POINT('Ctrl Pts',(85.2673789151792,1076.69045036403,399.731527361307));
#117983=CARTESIAN_POINT('Ctrl Pts',(85.2724797471146,1076.69031144632,399.726349393422));
#117984=CARTESIAN_POINT('Ctrl Pts',(85.277624729216,1076.69017144712,399.721203256573));
#117985=CARTESIAN_POINT('Ctrl Pts',(85.3270311525582,1076.68882705761,399.671785744376));
#117986=CARTESIAN_POINT('Ctrl Pts',(85.3796355268857,1076.68740530391,399.62617214953));
#117987=CARTESIAN_POINT('Ctrl Pts',(85.4350174597331,1076.68591198077,399.584557999036));
#117988=CARTESIAN_POINT('Ctrl Pts',(85.4932534022695,1076.68434170188,399.5407993371));
#117989=CARTESIAN_POINT('Ctrl Pts',(85.5545622562959,1076.68269228709,399.50146084956));
#117990=CARTESIAN_POINT('Ctrl Pts',(85.618505362964,1076.680970474,399.466795472388));
#117991=CARTESIAN_POINT('Ctrl Pts',(85.6635875331991,1076.67975653438,399.44235514541));
#117992=CARTESIAN_POINT('Ctrl Pts',(85.7099803264848,1076.67850660736,399.420238305068));
#117993=CARTESIAN_POINT('Ctrl Pts',(85.7575354277989,1076.67722305418,399.40054838733));
#117994=CARTESIAN_POINT('Ctrl Pts',(85.7992620443115,1076.67609681682,399.383271720392));
#117995=CARTESIAN_POINT('Ctrl Pts',(85.841552596285,1076.67495402394,399.367996775221));
#117996=CARTESIAN_POINT('Ctrl Pts',(85.8843932112835,1076.67379476451,399.354684806836));
#117997=CARTESIAN_POINT('Ctrl Pts',(85.9273698567947,1076.67263182411,399.34133056936));
#117998=CARTESIAN_POINT('Ctrl Pts',(85.9709009592765,1076.67145231241,399.329951487713));
#117999=CARTESIAN_POINT('Ctrl Pts',(86.0149906391529,1076.67025631923,399.320557209856));
#118000=CARTESIAN_POINT('Ctrl Pts',(86.0212994704472,1076.67008518351,399.319212974327));
#118001=CARTESIAN_POINT('Ctrl Pts',(86.0276197554638,1076.66991371033,399.317909463193));
#118002=CARTESIAN_POINT('Ctrl Pts',(86.0339515196089,1076.66974189995,399.316646791268));
#118003=CARTESIAN_POINT('Ctrl Pts',(86.069346529021,1076.6687814678,399.309588365905));
#118004=CARTESIAN_POINT('Ctrl Pts',(86.1051948127433,1076.66780773598,399.303791735915));
#118005=CARTESIAN_POINT('Ctrl Pts',(86.1412531880335,1076.66682790792,399.299323226414));
#118006=CARTESIAN_POINT('Ctrl Pts',(86.1773155013337,1076.66584797285,399.294854228899));
#118007=CARTESIAN_POINT('Ctrl Pts',(86.2135873733398,1076.6648619402,399.291713745247));
#118008=CARTESIAN_POINT('Ctrl Pts',(86.2498176838234,1076.66387701573,399.289916507982));
#118009=CARTESIAN_POINT('Ctrl Pts',(86.2742766985505,1076.66321209507,399.288703196471));
#118010=CARTESIAN_POINT('Ctrl Pts',(86.2987166153919,1076.66254767947,399.288100993965));
#118011=CARTESIAN_POINT('Ctrl Pts',(86.3230601852944,1076.66188598601,399.288100993964));
#118012=CARTESIAN_POINT('Ctrl Pts',(86.3230601852944,1076.66188598601,399.288100993964));
#118013=CARTESIAN_POINT('Ctrl Pts',(86.5193488915849,1076.65655057493,399.288100993962));
#118014=CARTESIAN_POINT('Ctrl Pts',(86.7136832635768,1076.65127220747,399.327193099627));
#118015=CARTESIAN_POINT('Ctrl Pts',(87.0726851878742,1076.64181642315,399.47772843703));
#118016=CARTESIAN_POINT('Ctrl Pts',(87.2343467825304,1076.63772009232,399.586492581294));
#118017=CARTESIAN_POINT('Ctrl Pts',(87.5068579887354,1076.63149362544,399.860136871519));
#118018=CARTESIAN_POINT('Ctrl Pts',(87.6150361758342,1076.62943100754,400.022425360104));
#118019=CARTESIAN_POINT('Ctrl Pts',(87.7630166637178,1076.62783207451,400.379867168201));
#118020=CARTESIAN_POINT('Ctrl Pts',(87.8012156409061,1076.62831903304,400.571623049732));
#118021=CARTESIAN_POINT('Ctrl Pts',(87.8015097065115,1076.63176047436,400.95836775111));
#118022=CARTESIAN_POINT('Ctrl Pts',(87.7638255065369,1076.63467101274,401.149610492304));
#118023=CARTESIAN_POINT('Ctrl Pts',(87.6171026682516,1076.64228909187,401.506739872023));
#118024=CARTESIAN_POINT('Ctrl Pts',(87.509483419049,1076.646916496,401.669195699455));
#118025=CARTESIAN_POINT('Ctrl Pts',(87.2377712112084,1076.65696241842,401.943698001443));
#118026=CARTESIAN_POINT('Ctrl Pts',(87.07622419366,1076.66227879963,402.053050768127));
#118027=CARTESIAN_POINT('Ctrl Pts',(86.8058328361515,1076.67017479352,402.167250190758));
#118028=CARTESIAN_POINT('Ctrl Pts',(86.7097073453473,1076.67282204102,402.196769066544));
#118029=CARTESIAN_POINT('Ctrl Pts',(86.5164033827763,1076.67783862898,402.235201840842));
#118030=CARTESIAN_POINT('Ctrl Pts',(86.4198549618292,1076.6802021928,402.244707258351));
#118031=CARTESIAN_POINT('Ctrl Pts',(86.323060185316,1076.68243856932,402.244707258351));
#118032=CARTESIAN_POINT('Origin',(86.323060185316,1067.7251047501,400.766404126158));
#118033=CARTESIAN_POINT('',(86.323060185316,1076.67873408293,401.644707258351));
#118034=CARTESIAN_POINT('',(86.3230601934255,1076.66654097378,399.888100993964));
#118035=CARTESIAN_POINT('Ctrl Pts',(86.323060185316,1076.67873408293,401.644707258351));
#118036=CARTESIAN_POINT('Ctrl Pts',(86.2703365558132,1076.67999434393,401.644707258351));
#118037=CARTESIAN_POINT('Ctrl Pts',(86.2175900991985,1076.68120258287,401.639959906646));
#118038=CARTESIAN_POINT('Ctrl Pts',(86.0508799772341,1076.68486336245,401.609553687992));
#118039=CARTESIAN_POINT('Ctrl Pts',(85.9415805432687,1076.6870210946,401.566066376273));
#118040=CARTESIAN_POINT('Ctrl Pts',(85.7462055632267,1076.69049162001,401.438903899627));
#118041=CARTESIAN_POINT('Ctrl Pts',(85.6621011671413,1076.69177193059,401.356448727894));
#118042=CARTESIAN_POINT('Ctrl Pts',(85.5308559925965,1076.69338560833,401.163264956452));
#118043=CARTESIAN_POINT('Ctrl Pts',(85.4851196212203,1076.69370245253,401.054401013379));
#118044=CARTESIAN_POINT('Ctrl Pts',(85.4389747655909,1076.69335051842,400.82523873274));
#118045=CARTESIAN_POINT('Ctrl Pts',(85.4389975443721,1076.69268545099,400.70723855402));
#118046=CARTESIAN_POINT('Ctrl Pts',(85.4851488405695,1076.6903905254,400.478480005544));
#118047=CARTESIAN_POINT('Ctrl Pts',(85.5306973091888,1076.68878349222,400.369977469653));
#118048=CARTESIAN_POINT('Ctrl Pts',(85.6615055835276,1076.6847086655,400.177036919966));
#118049=CARTESIAN_POINT('Ctrl Pts',(85.7454867969112,1076.68227796102,400.094530632461));
#118050=CARTESIAN_POINT('Ctrl Pts',(85.8909526465541,1076.67820342884,399.999617090543));
#118051=CARTESIAN_POINT('Ctrl Pts',(85.9417217547294,1076.67680058898,399.973145035766));
#118052=CARTESIAN_POINT('Ctrl Pts',(86.0484920846018,1076.67388088735,399.930107152951));
#118053=CARTESIAN_POINT('Ctrl Pts',(86.1043003340706,1076.67236973109,399.913805613415));
#118054=CARTESIAN_POINT('Ctrl Pts',(86.2147707440104,1076.66940637569,399.893106551994));
#118055=CARTESIAN_POINT('Ctrl Pts',(86.2689219404621,1076.66796623408,399.888100992965));
#118056=CARTESIAN_POINT('Ctrl Pts',(86.3230602015351,1076.66654097378,399.888100993964));
#118057=CARTESIAN_POINT('',(86.323060185316,1082.7251047501,399.888100993964));
#118058=CARTESIAN_POINT('',(86.323060185316,1067.7251047501,399.888100993964));
#118059=CARTESIAN_POINT('Origin',(86.323060185316,1082.7251047501,400.766404126158));
#118060=CARTESIAN_POINT('Ctrl Pts',(86.3230602015351,1076.66654097378,399.888100993964));
#118061=CARTESIAN_POINT('Ctrl Pts',(86.3835602978918,1076.66494822988,399.888100995082));
#118062=CARTESIAN_POINT('Ctrl Pts',(86.4440442396713,1076.66337405196,399.894352178612));
#118063=CARTESIAN_POINT('Ctrl Pts',(86.6162978831962,1076.65896256379,399.930519125098));
#118064=CARTESIAN_POINT('Ctrl Pts',(86.7233134227448,1076.65631211925,399.97615557805));
#118065=CARTESIAN_POINT('Ctrl Pts',(86.9135845116199,1076.65190698282,400.106126773335));
#118066=CARTESIAN_POINT('Ctrl Pts',(86.9950035821248,1076.65019723603,400.189185963914));
#118067=CARTESIAN_POINT('Ctrl Pts',(87.1210520559765,1076.64805927605,400.381876011175));
#118068=CARTESIAN_POINT('Ctrl Pts',(87.1645076941637,1076.64765153742,400.489600926454));
#118069=CARTESIAN_POINT('Ctrl Pts',(87.195329481483,1076.64806700802,400.652003725408));
#118070=CARTESIAN_POINT('Ctrl Pts',(87.2004447812257,1076.64832486168,400.70208215275));
#118071=CARTESIAN_POINT('Ctrl Pts',(87.2012504124973,1076.64870978558,400.752321622694));
#118072=CARTESIAN_POINT('Ctrl Pts',(87.2030916191839,1076.64958949878,400.867139966079));
#118073=CARTESIAN_POINT('Ctrl Pts',(87.1823974007777,1076.65112258767,400.981204654637));
#118074=CARTESIAN_POINT('Ctrl Pts',(87.0983016656521,1076.65523027365,401.194890512925));
#118075=CARTESIAN_POINT('Ctrl Pts',(87.0357107310818,1076.65776283178,401.292451292755));
#118076=CARTESIAN_POINT('Ctrl Pts',(86.8764915534712,1076.66338249602,401.458019541839));
#118077=CARTESIAN_POINT('Ctrl Pts',(86.7813684669782,1076.6664135884,401.524408367226));
#118078=CARTESIAN_POINT('Ctrl Pts',(86.6236024554262,1076.67097304646,401.593680827278));
#118079=CARTESIAN_POINT('Ctrl Pts',(86.5688985800898,1076.67248410541,401.611552632287));
#118080=CARTESIAN_POINT('Ctrl Pts',(86.4503735200599,1076.67561408443,401.637783076379));
#118081=CARTESIAN_POINT('Ctrl Pts',(86.386733500936,1076.67721208991,401.644707258351));
#118082=CARTESIAN_POINT('Ctrl Pts',(86.323060185316,1076.67873408293,401.644707258351));
#118083=CARTESIAN_POINT('Origin',(95.5155706932862,1067.7251047501,409.322561393736));
#118084=CARTESIAN_POINT('',(95.5155706933088,1078.33592031499,408.047117272599));
#118085=CARTESIAN_POINT('Ctrl Pts',(95.5157708467647,1078.36173587679,410.598005499167));
#118086=CARTESIAN_POINT('Ctrl Pts',(95.6818456189848,1078.35138272575,410.597979437309));
#118087=CARTESIAN_POINT('Ctrl Pts',(95.846320998692,1078.34061900062,410.5655169649));
#118088=CARTESIAN_POINT('Ctrl Pts',(96.1550572043217,1078.31940202197,410.438773886002));
#118089=CARTESIAN_POINT('Ctrl Pts',(96.2961429969713,1078.30915868367,410.345111475783));
#118090=CARTESIAN_POINT('Ctrl Pts',(96.5262341735934,1078.29144359458,410.116223207326));
#118091=CARTESIAN_POINT('Ctrl Pts',(96.6160958137961,1078.28398795017,409.98605322132));
#118092=CARTESIAN_POINT('Ctrl Pts',(96.7478900226055,1078.27185634106,409.691035758722));
#118093=CARTESIAN_POINT('Ctrl Pts',(96.7853912837021,1078.26749239219,409.527434387064));
#118094=CARTESIAN_POINT('Ctrl Pts',(96.7916613111768,1078.26479235547,409.320553344349));
#118095=CARTESIAN_POINT('Ctrl Pts',(96.790948682325,1078.26439437466,409.279870660457));
#118096=CARTESIAN_POINT('Ctrl Pts',(96.7867088842337,1078.26397330139,409.215069130938));
#118097=CARTESIAN_POINT('Ctrl Pts',(96.784433022949,1078.26386384006,409.190897814286));
#118098=CARTESIAN_POINT('Ctrl Pts',(96.7792129087214,1078.26375578654,409.148471473705));
#118099=CARTESIAN_POINT('Ctrl Pts',(96.7765589847555,1078.26373696293,409.130188108744));
#118100=CARTESIAN_POINT('Ctrl Pts',(96.7702825434915,1078.26375561822,409.09269687742));
#118101=CARTESIAN_POINT('Ctrl Pts',(96.7666137692975,1078.26379641053,409.073501680161));
#118102=CARTESIAN_POINT('Ctrl Pts',(96.7562134955821,1078.26397855988,409.025141302091));
#118103=CARTESIAN_POINT('Ctrl Pts',(96.748893867157,1078.26416179124,408.996115116325));
#118104=CARTESIAN_POINT('Ctrl Pts',(96.7167486679843,1078.26514854897,408.885251096893));
#118105=CARTESIAN_POINT('Ctrl Pts',(96.6847417155487,1078.2664698986,408.805739397829));
#118106=CARTESIAN_POINT('Ctrl Pts',(96.5890202668801,1078.27101453864,408.623277459538));
#118107=CARTESIAN_POINT('Ctrl Pts',(96.518173715774,1078.27477282283,408.525024934341));
#118108=CARTESIAN_POINT('Ctrl Pts',(96.3394301153674,1078.28485574914,408.33927001983));
#118109=CARTESIAN_POINT('Ctrl Pts',(96.2289188733061,1078.29139780745,408.256392798646));
#118110=CARTESIAN_POINT('Ctrl Pts',(95.9748429615258,1078.3068731441,408.123305858752));
#118111=CARTESIAN_POINT('Ctrl Pts',(95.8311486695084,1078.3158476971,408.077758970819));
#118112=CARTESIAN_POINT('Ctrl Pts',(95.523583801791,1078.33535479415,408.037058711165));
#118113=CARTESIAN_POINT('Ctrl Pts',(95.3617187997048,1078.34577900403,408.046273854795));
#118114=CARTESIAN_POINT('Ctrl Pts',(95.0420855861173,1078.36663663872,408.126290569185));
#118115=CARTESIAN_POINT('Ctrl Pts',(94.8880501038049,1078.37684060563,408.199396782662));
#118116=CARTESIAN_POINT('Ctrl Pts',(94.6216044936282,1078.39491960971,408.39825515004));
#118117=CARTESIAN_POINT('Ctrl Pts',(94.5105001323017,1078.40269454033,408.520446453725));
#118118=CARTESIAN_POINT('Ctrl Pts',(94.350454285991,1078.41460470566,408.783898272124));
#118119=CARTESIAN_POINT('Ctrl Pts',(94.2969284648118,1078.41897537158,408.919341038538));
#118120=CARTESIAN_POINT('Ctrl Pts',(94.247274087537,1078.42404571228,409.156223439857));
#118121=CARTESIAN_POINT('Ctrl Pts',(94.2382751790723,1078.42546105857,409.253537466283));
#118122=CARTESIAN_POINT('Ctrl Pts',(94.2411673834591,1078.4264927777,409.383527933655));
#118123=CARTESIAN_POINT('Ctrl Pts',(94.2431422157397,1078.42667908012,409.416084339831));
#118124=CARTESIAN_POINT('Ctrl Pts',(94.2483381277004,1078.42686245503,409.468436387324));
#118125=CARTESIAN_POINT('Ctrl Pts',(94.2507819359811,1078.42690480424,409.488293992395));
#118126=CARTESIAN_POINT('Ctrl Pts',(94.2563164209592,1078.42693323704,409.525937795906));
#118127=CARTESIAN_POINT('Ctrl Pts',(94.2593195755141,1078.42692442566,409.543731944702));
#118128=CARTESIAN_POINT('Ctrl Pts',(94.2669889144042,1078.42685384478,409.583953367182));
#118129=CARTESIAN_POINT('Ctrl Pts',(94.2718837455851,1078.42677846831,409.606330647218));
#118130=CARTESIAN_POINT('Ctrl Pts',(94.2883467413373,1078.42644521499,409.672945647874));
#118131=CARTESIAN_POINT('Ctrl Pts',(94.3016931476827,1078.42608061037,409.716704588679));
#118132=CARTESIAN_POINT('Ctrl Pts',(94.3754706640813,1078.42369665795,409.918953739349));
#118133=CARTESIAN_POINT('Ctrl Pts',(94.4647569250254,1078.41989967285,410.065041142623));
#118134=CARTESIAN_POINT('Ctrl Pts',(94.6729760200097,1078.40982746045,410.289788849472));
#118135=CARTESIAN_POINT('Ctrl Pts',(94.7815364596466,1078.40423244603,410.374543694537));
#118136=CARTESIAN_POINT('Ctrl Pts',(95.0000289934117,1078.3923269411,410.49458042913));
#118137=CARTESIAN_POINT('Ctrl Pts',(95.10533012359,1078.38637181487,410.535451565601));
#118138=CARTESIAN_POINT('Ctrl Pts',(95.3132100058356,1078.37417482621,410.585932618435));
#118139=CARTESIAN_POINT('Ctrl Pts',(95.4143185766654,1078.36806044169,410.598021419915));
#118140=CARTESIAN_POINT('Ctrl Pts',(95.5157708467647,1078.36173587679,410.598005499167));
#118141=CARTESIAN_POINT('',(95.515570693267,1076.33150256053,408.0471172726));
#118142=CARTESIAN_POINT('',(95.5155706932862,1067.7251047501,408.0471172726));
#118143=CARTESIAN_POINT('Ctrl Pts',(95.5152393238831,1076.35762093081,410.598005471826));
#118144=CARTESIAN_POINT('Ctrl Pts',(95.3462068216855,1076.3682676787,410.597961555985));
#118145=CARTESIAN_POINT('Ctrl Pts',(95.1788077616908,1076.37827883585,410.56431576052));
#118146=CARTESIAN_POINT('Ctrl Pts',(94.8673437761854,1076.39596881353,410.433853171452));
#118147=CARTESIAN_POINT('Ctrl Pts',(94.7262614520925,1076.40348614202,410.338533835159));
#118148=CARTESIAN_POINT('Ctrl Pts',(94.4889398941508,1076.41525764072,410.09806679161));
#118149=CARTESIAN_POINT('Ctrl Pts',(94.3952089412524,1076.41938944838,409.955172995849));
#118150=CARTESIAN_POINT('Ctrl Pts',(94.2688186385361,1076.4238178205,409.640635468617));
#118151=CARTESIAN_POINT('Ctrl Pts',(94.2376021102377,1076.42406178306,409.472093703902));
#118152=CARTESIAN_POINT('Ctrl Pts',(94.2429641604886,1076.42058948996,409.133059848678));
#118153=CARTESIAN_POINT('Ctrl Pts',(94.2793402074269,1076.41691485914,408.965985053345));
#118154=CARTESIAN_POINT('Ctrl Pts',(94.4149212921026,1076.40598072977,408.656384811212));
#118155=CARTESIAN_POINT('Ctrl Pts',(94.5125647178691,1076.39883715225,408.516857732209));
#118156=CARTESIAN_POINT('Ctrl Pts',(94.756648226872,1076.38176911232,408.283640659087));
#118157=CARTESIAN_POINT('Ctrl Pts',(94.9007928616087,1076.37200195597,408.192370202695));
#118158=CARTESIAN_POINT('Ctrl Pts',(95.2176270772563,1076.35090892827,408.070742322079));
#118159=CARTESIAN_POINT('Ctrl Pts',(95.3874168679025,1076.3397775118,408.042175011207));
#118160=CARTESIAN_POINT('Ctrl Pts',(95.7252721625835,1076.31795289155,408.053361722937));
#118161=CARTESIAN_POINT('Ctrl Pts',(95.8900811076927,1076.30746694685,408.091866282138));
#118162=CARTESIAN_POINT('Ctrl Pts',(96.1952413370978,1076.28852989874,408.230384756731));
#118163=CARTESIAN_POINT('Ctrl Pts',(96.3326784552892,1076.28026335186,408.328990890009));
#118164=CARTESIAN_POINT('Ctrl Pts',(96.561303952101,1076.26730168083,408.573474622017));
#118165=CARTESIAN_POINT('Ctrl Pts',(96.6503925565104,1076.26272699978,408.71683592043));
#118166=CARTESIAN_POINT('Ctrl Pts',(96.7680017223648,1076.25805157737,409.029368217875));
#118167=CARTESIAN_POINT('Ctrl Pts',(96.7955605163017,1076.25798414124,409.195390865539));
#118168=CARTESIAN_POINT('Ctrl Pts',(96.7852559247905,1076.26238928213,409.528395735921));
#118169=CARTESIAN_POINT('Ctrl Pts',(96.7475859808118,1076.26681076826,409.692119201418));
#118170=CARTESIAN_POINT('Ctrl Pts',(96.6114758770957,1076.27945864058,409.995988321167));
#118171=CARTESIAN_POINT('Ctrl Pts',(96.5142708974298,1076.28756378237,410.133156880886));
#118172=CARTESIAN_POINT('Ctrl Pts',(96.272427198426,1076.30622741002,410.362655425657));
#118173=CARTESIAN_POINT('Ctrl Pts',(96.1299714925185,1076.3166096792,410.452655243967));
#118174=CARTESIAN_POINT('Ctrl Pts',(95.9014745265624,1076.33238731036,410.540725233353));
#118175=CARTESIAN_POINT('Ctrl Pts',(95.8262539165507,1076.33746266407,410.562045378037));
#118176=CARTESIAN_POINT('Ctrl Pts',(95.6722912265138,1076.34761456986,410.590778526715));
#118177=CARTESIAN_POINT('Ctrl Pts',(95.5938506946242,1076.35266948399,410.598025895617));
#118178=CARTESIAN_POINT('Ctrl Pts',(95.5152393238831,1076.35762093081,410.598005471826));
#118179=CARTESIAN_POINT('Origin',(95.5155706932862,1067.7251047501,409.322561393736));
#118180=CARTESIAN_POINT('',(95.5155706932862,1076.35191524971,409.998005514872));
#118181=CARTESIAN_POINT('',(95.5155706932863,1076.33810018128,408.6471172726));
#118182=CARTESIAN_POINT('Ctrl Pts',(95.5155706932862,1076.35191524971,409.998005514872));
#118183=CARTESIAN_POINT('Ctrl Pts',(95.4268631047514,1076.3575378307,409.998005514872));
#118184=CARTESIAN_POINT('Ctrl Pts',(95.3389823525427,1076.36287753048,409.980530058774));
#118185=CARTESIAN_POINT('Ctrl Pts',(95.1740512569251,1076.37246855803,409.912176126145));
#118186=CARTESIAN_POINT('Ctrl Pts',(95.0987775398121,1076.37661271161,409.861613003879));
#118187=CARTESIAN_POINT('Ctrl Pts',(94.9722814177744,1076.38312432879,409.733846983442));
#118188=CARTESIAN_POINT('Ctrl Pts',(94.9223727036056,1076.38542472252,409.657887972189));
#118189=CARTESIAN_POINT('Ctrl Pts',(94.8552103879287,1076.38788498739,409.490713375327));
#118190=CARTESIAN_POINT('Ctrl Pts',(94.8386874965241,1076.38801741199,409.401177587466));
#118191=CARTESIAN_POINT('Ctrl Pts',(94.8417602983214,1076.38607341608,409.221013227405));
#118192=CARTESIAN_POINT('Ctrl Pts',(94.8612822612857,1076.38401880293,409.132216377598));
#118193=CARTESIAN_POINT('Ctrl Pts',(94.9338840883269,1076.37795001218,408.967686475133));
#118194=CARTESIAN_POINT('Ctrl Pts',(94.9861728002878,1076.37399904601,408.893584305718));
#118195=CARTESIAN_POINT('Ctrl Pts',(95.1166832878363,1076.36465634994,408.770118356905));
#118196=CARTESIAN_POINT('Ctrl Pts',(95.1936383730592,1076.35935448643,408.722016209618));
#118197=CARTESIAN_POINT('Ctrl Pts',(95.3536793712844,1076.34862033023,408.661802104452));
#118198=CARTESIAN_POINT('Ctrl Pts',(95.4341694303066,1076.3433362448,408.647147294093));
#118199=CARTESIAN_POINT('Ctrl Pts',(95.5153212013006,1076.33811622929,408.647117318678));
#118200=CARTESIAN_POINT('Ctrl Pts',(95.5154043660395,1076.3381108798,408.647117287959));
#118201=CARTESIAN_POINT('Ctrl Pts',(95.5154875300362,1076.33810553046,408.6471172726));
#118202=CARTESIAN_POINT('Ctrl Pts',(95.5155706932864,1076.33810018128,408.6471172726));
#118203=CARTESIAN_POINT('',(95.5155706932862,1082.7251047501,408.6471172726));
#118204=CARTESIAN_POINT('',(95.5155706932862,1067.7251047501,408.6471172726));
#118205=CARTESIAN_POINT('Origin',(95.5155706932862,1082.7251047501,409.322561393736));
#118206=CARTESIAN_POINT('Ctrl Pts',(95.5155706932864,1076.33810018128,408.6471172726));
#118207=CARTESIAN_POINT('Ctrl Pts',(95.6050888462091,1076.33234224998,408.6471172726));
#118208=CARTESIAN_POINT('Ctrl Pts',(95.6937419908893,1076.32676984405,408.664913370058));
#118209=CARTESIAN_POINT('Ctrl Pts',(95.8580878010066,1076.31674152892,408.73370087287));
#118210=CARTESIAN_POINT('Ctrl Pts',(95.93232579778,1076.31237213147,408.783671656049));
#118211=CARTESIAN_POINT('Ctrl Pts',(96.0571375631939,1076.30543870016,408.909338698087));
#118212=CARTESIAN_POINT('Ctrl Pts',(96.1065556297645,1076.30293886113,408.983748504815));
#118213=CARTESIAN_POINT('Ctrl Pts',(96.1738144023741,1076.30019943501,409.147246984151));
#118214=CARTESIAN_POINT('Ctrl Pts',(96.1910713569332,1076.29998186512,409.234699493124));
#118215=CARTESIAN_POINT('Ctrl Pts',(96.1909580358862,1076.30187621358,409.411224565421));
#118216=CARTESIAN_POINT('Ctrl Pts',(96.1736151391932,1076.30396742989,409.498568174232));
#118217=CARTESIAN_POINT('Ctrl Pts',(96.1063230347709,1076.31016595517,409.661729965477));
#118218=CARTESIAN_POINT('Ctrl Pts',(96.0569808708569,1076.31421480077,409.735945468884));
#118219=CARTESIAN_POINT('Ctrl Pts',(95.9324502998172,1076.32369904763,409.86132215265));
#118220=CARTESIAN_POINT('Ctrl Pts',(95.8583941731649,1076.32904547513,409.911216828379));
#118221=CARTESIAN_POINT('Ctrl Pts',(95.7360696308699,1076.33747218958,409.962531130631));
#118222=CARTESIAN_POINT('Ctrl Pts',(95.6937025115112,1076.3403297286,409.975592635954));
#118223=CARTESIAN_POINT('Ctrl Pts',(95.6071250341514,1076.34604948107,409.993225142205));
#118224=CARTESIAN_POINT('Ctrl Pts',(95.5631235614272,1076.34889814964,409.997773289301));
#118225=CARTESIAN_POINT('Ctrl Pts',(95.5178516334647,1076.35177063834,409.998002626737));
#118226=CARTESIAN_POINT('Ctrl Pts',(95.5167110950412,1076.35184296727,409.998005514872));
#118227=CARTESIAN_POINT('Ctrl Pts',(95.5155706932862,1076.35191524971,409.998005514872));
#118228=CARTESIAN_POINT('Origin',(104.753539540173,1067.7251047501,419.641388283931));
#118229=CARTESIAN_POINT('',(104.753539540203,1077.66045630879,418.542557147938));
#118230=CARTESIAN_POINT('Ctrl Pts',(104.753337989031,1077.67124291073,420.740219401439));
#118231=CARTESIAN_POINT('Ctrl Pts',(104.900057040271,1077.65614840032,420.740246313119));
#118232=CARTESIAN_POINT('Ctrl Pts',(105.045339494299,1077.64093797211,420.710887479148));
#118233=CARTESIAN_POINT('Ctrl Pts',(105.312516336785,1077.61248223269,420.598193937028));
#118234=CARTESIAN_POINT('Ctrl Pts',(105.43241877665,1077.59946383205,420.517244645325));
#118235=CARTESIAN_POINT('Ctrl Pts',(105.621401545446,1077.57853531814,420.32683144979));
#118236=CARTESIAN_POINT('Ctrl Pts',(105.693683172648,1077.5703353697,420.223797724618));
#118237=CARTESIAN_POINT('Ctrl Pts',(105.799112991354,1077.55798113396,420.000603992107));
#118238=CARTESIAN_POINT('Ctrl Pts',(105.832489688039,1077.55381500438,419.882548921654));
#118239=CARTESIAN_POINT('Ctrl Pts',(105.848952660687,1077.55129454079,419.732674653752));
#118240=CARTESIAN_POINT('Ctrl Pts',(105.850972785091,1077.55093225463,419.703866746693));
#118241=CARTESIAN_POINT('Ctrl Pts',(105.852428174474,1077.55053513875,419.65632548408));
#118242=CARTESIAN_POINT('Ctrl Pts',(105.852523267621,1077.55042996759,419.63762785047));
#118243=CARTESIAN_POINT('Ctrl Pts',(105.851837017862,1077.55033270959,419.604048396105));
#118244=CARTESIAN_POINT('Ctrl Pts',(105.851230137569,1077.55032197808,419.589167868126));
#118245=CARTESIAN_POINT('Ctrl Pts',(105.849302102183,1077.55036792785,419.557645716235));
#118246=CARTESIAN_POINT('Ctrl Pts',(105.847903805087,1077.5504329001,419.541012705523));
#118247=CARTESIAN_POINT('Ctrl Pts',(105.84318525221,1077.55071337619,419.49693792828));
#118248=CARTESIAN_POINT('Ctrl Pts',(105.83920769182,1077.55099956616,419.469579595451));
#118249=CARTESIAN_POINT('Ctrl Pts',(105.816907725988,1077.55276765661,419.348472261398));
#118250=CARTESIAN_POINT('Ctrl Pts',(105.787446389403,1077.55545267616,419.257233179425));
#118251=CARTESIAN_POINT('Ctrl Pts',(105.700341275358,1077.56380784206,419.073350382954));
#118252=CARTESIAN_POINT('Ctrl Pts',(105.639982010274,1077.5697778904,418.983142259288));
#118253=CARTESIAN_POINT('Ctrl Pts',(105.486013291688,1077.58525013152,418.813360339748));
#118254=CARTESIAN_POINT('Ctrl Pts',(105.390265249364,1077.59499159045,418.73768516913));
#118255=CARTESIAN_POINT('Ctrl Pts',(105.168861991658,1077.61765178481,418.615576761589));
#118256=CARTESIAN_POINT('Ctrl Pts',(105.043079533405,1077.63059258579,418.573254642765));
#118257=CARTESIAN_POINT('Ctrl Pts',(104.772769955003,1077.65846054535,418.533635647527));
#118258=CARTESIAN_POINT('Ctrl Pts',(104.629979601619,1077.67321148739,418.540377563639));
#118259=CARTESIAN_POINT('Ctrl Pts',(104.351458636077,1077.70203924284,418.608521521727));
#118260=CARTESIAN_POINT('Ctrl Pts',(104.218632435707,1077.71581753649,418.670605939101));
#118261=CARTESIAN_POINT('Ctrl Pts',(103.991259135625,1077.73955344112,418.838166468809));
#118262=CARTESIAN_POINT('Ctrl Pts',(103.896959638166,1077.7494780425,418.939550694101));
#118263=CARTESIAN_POINT('Ctrl Pts',(103.751832614709,1077.76505147781,419.169984413909));
#118264=CARTESIAN_POINT('Ctrl Pts',(103.701518069179,1077.77064053063,419.296516377219));
#118265=CARTESIAN_POINT('Ctrl Pts',(103.665516933398,1077.77507197987,419.479338792007));
#118266=CARTESIAN_POINT('Ctrl Pts',(103.659145621184,1077.77594280979,419.530228916064));
#118267=CARTESIAN_POINT('Ctrl Pts',(103.65514842758,1077.7766828898,419.603317531618));
#118268=CARTESIAN_POINT('Ctrl Pts',(103.65460683322,1077.77683993463,419.625283385923));
#118269=CARTESIAN_POINT('Ctrl Pts',(103.654797677955,1077.7769894068,419.661051367562));
#118270=CARTESIAN_POINT('Ctrl Pts',(103.655131283486,1077.77702131537,419.674849047804));
#118271=CARTESIAN_POINT('Ctrl Pts',(103.656372282436,1077.77703413892,419.703683511127));
#118272=CARTESIAN_POINT('Ctrl Pts',(103.657329146783,1077.77701013077,419.718715243145));
#118273=CARTESIAN_POINT('Ctrl Pts',(103.660323033302,1077.7768807378,419.754218226528));
#118274=CARTESIAN_POINT('Ctrl Pts',(103.662626495215,1077.77674883046,419.774661040391));
#118275=CARTESIAN_POINT('Ctrl Pts',(103.672030997665,1077.7761308177,419.841261851752));
#118276=CARTESIAN_POINT('Ctrl Pts',(103.681499536177,1077.77540831961,419.887029439237));
#118277=CARTESIAN_POINT('Ctrl Pts',(103.732479124479,1077.77123006641,420.072889265702));
#118278=CARTESIAN_POINT('Ctrl Pts',(103.798771233643,1077.76527569804,420.20451944097));
#118279=CARTESIAN_POINT('Ctrl Pts',(103.962124804672,1077.74996187958,420.412906061734));
#118280=CARTESIAN_POINT('Ctrl Pts',(104.050155865404,1077.74153430367,420.493904256605));
#118281=CARTESIAN_POINT('Ctrl Pts',(104.242901321601,1077.72272849526,420.620788193795));
#118282=CARTESIAN_POINT('Ctrl Pts',(104.345261722085,1077.71259696246,420.667669086737));
#118283=CARTESIAN_POINT('Ctrl Pts',(104.550623988338,1077.6919728297,420.726094557412));
#118284=CARTESIAN_POINT('Ctrl Pts',(104.651750685918,1077.68169425015,420.740200767968));
#118285=CARTESIAN_POINT('Ctrl Pts',(104.753337989031,1077.67124291073,420.740219401439));
#118286=CARTESIAN_POINT('',(104.753539540154,1075.64948580966,418.542557147938));
#118287=CARTESIAN_POINT('',(104.753539540173,1067.7251047501,418.542557147938));
#118288=CARTESIAN_POINT('Ctrl Pts',(104.753780331061,1075.66032526247,420.740219393541));
#118289=CARTESIAN_POINT('Ctrl Pts',(104.608017390083,1075.67545936333,420.740251335108));
#118290=CARTESIAN_POINT('Ctrl Pts',(104.463616745573,1075.69018993346,420.711279234496));
#118291=CARTESIAN_POINT('Ctrl Pts',(104.194951603842,1075.71712622813,420.598748997557));
#118292=CARTESIAN_POINT('Ctrl Pts',(104.073213737543,1075.72908278922,420.516486776639));
#118293=CARTESIAN_POINT('Ctrl Pts',(103.868511886586,1075.74876355436,420.308816329664));
#118294=CARTESIAN_POINT('Ctrl Pts',(103.787693667013,1075.75628352042,420.185398144544));
#118295=CARTESIAN_POINT('Ctrl Pts',(103.68018647117,1075.76577533426,419.916766300725));
#118296=CARTESIAN_POINT('Ctrl Pts',(103.653464740972,1075.76776781884,419.774714435164));
#118297=CARTESIAN_POINT('Ctrl Pts',(103.656042550634,1075.76614840311,419.488119056161));
#118298=CARTESIAN_POINT('Ctrl Pts',(103.685384927727,1075.76254544142,419.346429673682));
#118299=CARTESIAN_POINT('Ctrl Pts',(103.797781076754,1075.74999313514,419.079899130659));
#118300=CARTESIAN_POINT('Ctrl Pts',(103.880695003253,1075.74106943032,418.95815433516));
#118301=CARTESIAN_POINT('Ctrl Pts',(104.088875957801,1075.71899043143,418.754339373639));
#118302=CARTESIAN_POINT('Ctrl Pts',(104.212042704123,1075.70605456884,418.674258481696));
#118303=CARTESIAN_POINT('Ctrl Pts',(104.413276182018,1075.6849934789,418.594141672999));
#118304=CARTESIAN_POINT('Ctrl Pts',(104.481849030662,1075.67782790398,418.574297114894));
#118305=CARTESIAN_POINT('Ctrl Pts',(104.622050555195,1075.66319241087,418.548117027916));
#118306=CARTESIAN_POINT('Ctrl Pts',(104.69336763863,1075.65575504721,418.54188424412));
#118307=CARTESIAN_POINT('Ctrl Pts',(104.912040589968,1075.63297156441,418.544120805526));
#118308=CARTESIAN_POINT('Ctrl Pts',(105.057573541504,1075.61783475013,418.575217732282));
#118309=CARTESIAN_POINT('Ctrl Pts',(105.325079724885,1075.59013380257,418.691846022237));
#118310=CARTESIAN_POINT('Ctrl Pts',(105.444929098913,1075.57778939103,418.77516108264));
#118311=CARTESIAN_POINT('Ctrl Pts',(105.645011802497,1075.5574505081,418.983060248187));
#118312=CARTESIAN_POINT('Ctrl Pts',(105.723529884179,1075.54963116592,419.105373244616));
#118313=CARTESIAN_POINT('Ctrl Pts',(105.828633711985,1075.53968325811,419.372823013811));
#118314=CARTESIAN_POINT('Ctrl Pts',(105.854469043342,1075.53762287042,419.515167045892));
#118315=CARTESIAN_POINT('Ctrl Pts',(105.850010428383,1075.53957190013,419.801536839165));
#118316=CARTESIAN_POINT('Ctrl Pts',(105.81987321488,1075.54354935951,419.942695662963));
#118317=CARTESIAN_POINT('Ctrl Pts',(105.707147584058,1075.55701077624,420.205849421708));
#118318=CARTESIAN_POINT('Ctrl Pts',(105.625507553164,1075.56637704818,420.325183367221));
#118319=CARTESIAN_POINT('Ctrl Pts',(105.420671355516,1075.58923218899,420.526316245184));
#118320=CARTESIAN_POINT('Ctrl Pts',(105.299193802991,1075.60252338783,420.605936850527));
#118321=CARTESIAN_POINT('Ctrl Pts',(105.100901594778,1075.62380745086,420.686230699525));
#118322=CARTESIAN_POINT('Ctrl Pts',(105.03348467881,1075.63098393756,420.706274568668));
#118323=CARTESIAN_POINT('Ctrl Pts',(104.895171228648,1075.64558403776,420.733349890659));
#118324=CARTESIAN_POINT('Ctrl Pts',(104.824558764112,1075.65297656371,420.740203883603));
#118325=CARTESIAN_POINT('Ctrl Pts',(104.753780331061,1075.66032526247,420.740219393541));
#118326=CARTESIAN_POINT('Origin',(104.753539540173,1067.7251047501,419.641388283931));
#118327=CARTESIAN_POINT('',(104.753539540173,1075.65786345153,420.140219419923));
#118328=CARTESIAN_POINT('',(104.753539540173,1075.6529321444,419.142557147938));
#118329=CARTESIAN_POINT('Ctrl Pts',(104.753539540173,1075.65786345153,420.140219419923));
#118330=CARTESIAN_POINT('Ctrl Pts',(104.687308095507,1075.66474562987,420.140219419923));
#118331=CARTESIAN_POINT('Ctrl Pts',(104.6217006974,1075.67147329423,420.127028753312));
#118332=CARTESIAN_POINT('Ctrl Pts',(104.499402998231,1075.68384521078,420.075722277205));
#118333=CARTESIAN_POINT('Ctrl Pts',(104.443910813031,1075.68936866123,420.038097664375));
#118334=CARTESIAN_POINT('Ctrl Pts',(104.351273826184,1075.69841656153,419.94363288491));
#118335=CARTESIAN_POINT('Ctrl Pts',(104.314888857087,1075.70186926393,419.887903677498));
#118336=CARTESIAN_POINT('Ctrl Pts',(104.266247826669,1075.70625322989,419.766304749997));
#118337=CARTESIAN_POINT('Ctrl Pts',(104.254127516133,1075.70717766645,419.70179843261));
#118338=CARTESIAN_POINT('Ctrl Pts',(104.2553322653,1075.70642279515,419.571718340932));
#118339=CARTESIAN_POINT('Ctrl Pts',(104.268652931906,1075.70475016815,419.507442009579));
#118340=CARTESIAN_POINT('Ctrl Pts',(104.319266761738,1075.69898536685,419.387422063991));
#118341=CARTESIAN_POINT('Ctrl Pts',(104.356155572995,1075.69494004472,419.332905003089));
#118342=CARTESIAN_POINT('Ctrl Pts',(104.449605432924,1075.68488233212,419.240305082476));
#118343=CARTESIAN_POINT('Ctrl Pts',(104.5056018145,1075.67893304666,419.203489809737));
#118344=CARTESIAN_POINT('Ctrl Pts',(104.59652450694,1075.66935129237,419.166851252507));
#118345=CARTESIAN_POINT('Ctrl Pts',(104.62700921512,1075.66614981598,419.15783042343));
#118346=CARTESIAN_POINT('Ctrl Pts',(104.689569604725,1075.65959990815,419.14564039129));
#118347=CARTESIAN_POINT('Ctrl Pts',(104.721518529795,1075.6562649377,419.142557147938));
#118348=CARTESIAN_POINT('Ctrl Pts',(104.753539540173,1075.6529321444,419.142557147938));
#118349=CARTESIAN_POINT('',(104.753539540173,1082.7251047501,419.142557147938));
#118350=CARTESIAN_POINT('',(104.753539540173,1067.7251047501,419.142557147938));
#118351=CARTESIAN_POINT('Origin',(104.753539540173,1082.7251047501,419.641388283931));
#118352=CARTESIAN_POINT('Ctrl Pts',(104.753539540173,1075.6529321444,419.142557147938));
#118353=CARTESIAN_POINT('Ctrl Pts',(104.753554883302,1075.65293054746,419.142557147938));
#118354=CARTESIAN_POINT('Ctrl Pts',(104.753570226448,1075.65292895053,419.14255714865));
#118355=CARTESIAN_POINT('Ctrl Pts',(104.753585569611,1075.65292735359,419.142557150066));
#118356=CARTESIAN_POINT('Ctrl Pts',(104.820236507847,1075.64599024648,419.142563300253));
#118357=CARTESIAN_POINT('Ctrl Pts',(104.886245227159,1075.63916129711,419.155927665713));
#118358=CARTESIAN_POINT('Ctrl Pts',(105.008600799258,1075.62659969549,419.207627952597));
#118359=CARTESIAN_POINT('Ctrl Pts',(105.063844999928,1075.62097982271,419.2452423481));
#118360=CARTESIAN_POINT('Ctrl Pts',(105.15578253575,1075.61176696558,419.339246517142));
#118361=CARTESIAN_POINT('Ctrl Pts',(105.191850127128,1075.60823474515,419.394430821737));
#118362=CARTESIAN_POINT('Ctrl Pts',(105.240552991933,1075.60369561211,419.515377191944));
#118363=CARTESIAN_POINT('Ctrl Pts',(105.252822055778,1075.60272146629,419.579884890652));
#118364=CARTESIAN_POINT('Ctrl Pts',(105.251894482801,1075.60347331626,419.709928517852));
#118365=CARTESIAN_POINT('Ctrl Pts',(105.238738326434,1075.60518842731,419.774163933337));
#118366=CARTESIAN_POINT('Ctrl Pts',(105.188503374222,1075.61109544875,419.894139303052));
#118367=CARTESIAN_POINT('Ctrl Pts',(105.15183985976,1075.61523693659,419.948662143914));
#118368=CARTESIAN_POINT('Ctrl Pts',(105.059485096615,1075.62541254168,420.040774108678));
#118369=CARTESIAN_POINT('Ctrl Pts',(105.004574740326,1075.63135882211,420.077368044466));
#118370=CARTESIAN_POINT('Ctrl Pts',(104.914082025973,1075.64101053315,420.114804766002));
#118371=CARTESIAN_POINT('Ctrl Pts',(104.88278861588,1075.64432587833,420.124286571065));
#118372=CARTESIAN_POINT('Ctrl Pts',(104.818882512722,1075.65105180129,420.136990864592));
#118373=CARTESIAN_POINT('Ctrl Pts',(104.78641959614,1075.65444670141,420.140197247639));
#118374=CARTESIAN_POINT('Ctrl Pts',(104.753764951171,1075.65784002859,420.140219381712));
#118375=CARTESIAN_POINT('Ctrl Pts',(104.753652244768,1075.65785174028,420.140219419923));
#118376=CARTESIAN_POINT('Ctrl Pts',(104.753539540173,1075.65786345153,420.140219419923));
#118377=CARTESIAN_POINT('Origin',(111.756957497769,1067.7251047501,431.748662623815));
#118378=CARTESIAN_POINT('',(111.756957497785,1076.82908683398,430.658121875088));
#118379=CARTESIAN_POINT('Ctrl Pts',(111.75727025721,1076.81040039708,432.839203327695));
#118380=CARTESIAN_POINT('Ctrl Pts',(111.902381742046,1076.79092321827,432.839161710737));
#118381=CARTESIAN_POINT('Ctrl Pts',(112.046147905152,1076.77177761504,432.810156830667));
#118382=CARTESIAN_POINT('Ctrl Pts',(112.308989063476,1076.73713110618,432.69950342034));
#118383=CARTESIAN_POINT('Ctrl Pts',(112.426451522639,1076.72183019829,432.620864925895));
#118384=CARTESIAN_POINT('Ctrl Pts',(112.610205488221,1076.69835402504,432.438136469508));
#118385=CARTESIAN_POINT('Ctrl Pts',(112.680329885432,1076.68960723474,432.34099987065));
#118386=CARTESIAN_POINT('Ctrl Pts',(112.775480883036,1076.67824727762,432.149686176776));
#118387=CARTESIAN_POINT('Ctrl Pts',(112.806413414772,1076.67479002866,432.059908091913));
#118388=CARTESIAN_POINT('Ctrl Pts',(112.830928519096,1076.67247594805,431.940060959275));
#118389=CARTESIAN_POINT('Ctrl Pts',(112.835445613322,1076.67209561867,431.912707390979));
#118390=CARTESIAN_POINT('Ctrl Pts',(112.840971520463,1076.67172067452,431.868921685871));
#118391=CARTESIAN_POINT('Ctrl Pts',(112.842659079724,1076.67163207462,431.852589222748));
#118392=CARTESIAN_POINT('Ctrl Pts',(112.845117214313,1076.6715618758,431.822073228129));
#118393=CARTESIAN_POINT('Ctrl Pts',(112.845980687728,1076.6715674332,431.807900935848));
#118394=CARTESIAN_POINT('Ctrl Pts',(112.84728008644,1076.67166416966,431.776475037786));
#118395=CARTESIAN_POINT('Ctrl Pts',(112.847583645854,1076.67177352059,431.759220087844));
#118396=CARTESIAN_POINT('Ctrl Pts',(112.847279913083,1076.6722479771,431.709761661606));
#118397=CARTESIAN_POINT('Ctrl Pts',(112.845655753014,1076.67275233942,431.677585353316));
#118398=CARTESIAN_POINT('Ctrl Pts',(112.828979890943,1076.6765753079,431.502040475541));
#118399=CARTESIAN_POINT('Ctrl Pts',(112.78705630706,1076.6835436819,431.362841729849));
#118400=CARTESIAN_POINT('Ctrl Pts',(112.665394732555,1076.70217029938,431.134469564144));
#118401=CARTESIAN_POINT('Ctrl Pts',(112.595729305969,1076.71248370333,431.042347247913));
#118402=CARTESIAN_POINT('Ctrl Pts',(112.422010651828,1076.73757576167,430.875178388979));
#118403=CARTESIAN_POINT('Ctrl Pts',(112.316453851464,1076.75251609532,430.804123561165));
#118404=CARTESIAN_POINT('Ctrl Pts',(112.07657617303,1076.78585597769,430.69711021615));
#118405=CARTESIAN_POINT('Ctrl Pts',(111.942611320986,1076.8041585093,430.665418413196));
#118406=CARTESIAN_POINT('Ctrl Pts',(111.661168067832,1076.84196882221,430.652659141278));
#118407=CARTESIAN_POINT('Ctrl Pts',(111.5160160997,1076.86112237415,430.675158454265));
#118408=CARTESIAN_POINT('Ctrl Pts',(111.247033082611,1076.8959726345,430.774403056583));
#118409=CARTESIAN_POINT('Ctrl Pts',(111.125137220351,1076.91144094223,430.84859073697));
#118410=CARTESIAN_POINT('Ctrl Pts',(110.936862817124,1076.93477697119,431.020901325329));
#118411=CARTESIAN_POINT('Ctrl Pts',(110.865437059576,1076.94339940202,431.110347351822));
#118412=CARTESIAN_POINT('Ctrl Pts',(110.754005580943,1076.95636331188,431.306192426863));
#118413=CARTESIAN_POINT('Ctrl Pts',(110.714031538733,1076.96071523188,431.410974238829));
#118414=CARTESIAN_POINT('Ctrl Pts',(110.684999757307,1076.96338113125,431.546398510142));
#118415=CARTESIAN_POINT('Ctrl Pts',(110.680332206982,1076.96376999925,431.572928853762));
#118416=CARTESIAN_POINT('Ctrl Pts',(110.674247574482,1076.96419759711,431.617028146599));
#118417=CARTESIAN_POINT('Ctrl Pts',(110.672265543499,1076.96431093093,431.634505692611));
#118418=CARTESIAN_POINT('Ctrl Pts',(110.669456605958,1076.96441482982,431.666079052284));
#118419=CARTESIAN_POINT('Ctrl Pts',(110.668479088377,1076.96442522452,431.68015721576));
#118420=CARTESIAN_POINT('Ctrl Pts',(110.666980413094,1076.96437101206,431.710156565671));
#118421=CARTESIAN_POINT('Ctrl Pts',(110.666534329686,1076.96429659172,431.726078025884));
#118422=CARTESIAN_POINT('Ctrl Pts',(110.666274409588,1076.96397574151,431.768642355027));
#118423=CARTESIAN_POINT('Ctrl Pts',(110.667087901174,1076.96364739238,431.795276875441));
#118424=CARTESIAN_POINT('Ctrl Pts',(110.67523109658,1076.96157361978,431.916336904323));
#118425=CARTESIAN_POINT('Ctrl Pts',(110.693862561181,1076.95836105401,432.009539071371));
#118426=CARTESIAN_POINT('Ctrl Pts',(110.75862031329,1076.94828780795,432.200363156414));
#118427=CARTESIAN_POINT('Ctrl Pts',(110.807642981491,1076.94106358344,432.295895149266));
#118428=CARTESIAN_POINT('Ctrl Pts',(110.939756315756,1076.92214738207,432.480777916079));
#118429=CARTESIAN_POINT('Ctrl Pts',(111.025516972836,1076.91012897666,432.566419021153));
#118430=CARTESIAN_POINT('Ctrl Pts',(111.218727770251,1076.88340794796,432.704338833626));
#118431=CARTESIAN_POINT('Ctrl Pts',(111.324343496112,1076.86895036648,432.756530884704));
#118432=CARTESIAN_POINT('Ctrl Pts',(111.54017868944,1076.83962445961,432.822973548804));
#118433=CARTESIAN_POINT('Ctrl Pts',(111.648436672709,1076.82500827728,432.839234540405));
#118434=CARTESIAN_POINT('Ctrl Pts',(111.75727025721,1076.81040039708,432.839203327695));
#118435=CARTESIAN_POINT('',(111.756957497753,1074.81089668524,430.658121875087));
#118436=CARTESIAN_POINT('',(111.756957497769,1067.7251047501,430.658121875087));
#118437=CARTESIAN_POINT('Ctrl Pts',(111.756676799939,1074.79213585482,432.839203336419));
#118438=CARTESIAN_POINT('Ctrl Pts',(111.685336789338,1074.80179067849,432.839184973981));
#118439=CARTESIAN_POINT('Ctrl Pts',(111.61416304056,1074.81146046818,432.832166367726));
#118440=CARTESIAN_POINT('Ctrl Pts',(111.402102858394,1074.84038596573,432.789980057988));
#118441=CARTESIAN_POINT('Ctrl Pts',(111.26691656466,1074.85898197916,432.733657466272));
#118442=CARTESIAN_POINT('Ctrl Pts',(111.026953109172,1074.89238584326,432.571596577775));
#118443=CARTESIAN_POINT('Ctrl Pts',(110.924330817354,1074.90689346776,432.46768798791));
#118444=CARTESIAN_POINT('Ctrl Pts',(110.765555579852,1074.92997212448,432.225478463408));
#118445=CARTESIAN_POINT('Ctrl Pts',(110.710988485895,1074.9383146646,432.089670289979));
#118446=CARTESIAN_POINT('Ctrl Pts',(110.658843592089,1074.94756386189,431.807701263431));
#118447=CARTESIAN_POINT('Ctrl Pts',(110.660460841978,1074.94855131792,431.664709323906));
#118448=CARTESIAN_POINT('Ctrl Pts',(110.718360677713,1074.94325334289,431.387091065484));
#118449=CARTESIAN_POINT('Ctrl Pts',(110.774139435225,1074.93700976715,431.255300249266));
#118450=CARTESIAN_POINT('Ctrl Pts',(110.934594932809,1074.91779174939,431.01791303319));
#118451=CARTESIAN_POINT('Ctrl Pts',(111.038708429017,1074.90486215894,430.915441976632));
#118452=CARTESIAN_POINT('Ctrl Pts',(111.2808515148,1074.87396993153,430.756881120247));
#118453=CARTESIAN_POINT('Ctrl Pts',(111.41662418256,1074.85628999999,430.702541711662));
#118454=CARTESIAN_POINT('Ctrl Pts',(111.628661045039,1074.82814366381,430.663370031491));
#118455=CARTESIAN_POINT('Ctrl Pts',(111.699550933579,1074.81865134874,430.657324632177));
#118456=CARTESIAN_POINT('Ctrl Pts',(111.841732594009,1074.79944746737,430.659090819334));
#118457=CARTESIAN_POINT('Ctrl Pts',(111.912707084578,1074.78977810564,430.666952673787));
#118458=CARTESIAN_POINT('Ctrl Pts',(112.125858871651,1074.76048623674,430.711991224333));
#118459=CARTESIAN_POINT('Ctrl Pts',(112.261882570826,1074.74143505668,430.770953595469));
#118460=CARTESIAN_POINT('Ctrl Pts',(112.499774167161,1074.70743783601,430.937442051952));
#118461=CARTESIAN_POINT('Ctrl Pts',(112.600121881773,1074.69272932387,431.042214961932));
#118462=CARTESIAN_POINT('Ctrl Pts',(112.753729407214,1074.66945233698,431.283891616949));
#118463=CARTESIAN_POINT('Ctrl Pts',(112.805948745228,1074.6610538322,431.418070304207));
#118464=CARTESIAN_POINT('Ctrl Pts',(112.855496719518,1074.65173543934,431.698163389931));
#118465=CARTESIAN_POINT('Ctrl Pts',(112.852768146603,1074.65085045777,431.841129578785));
#118466=CARTESIAN_POINT('Ctrl Pts',(112.792797957082,1074.65670190277,432.117909946033));
#118467=CARTESIAN_POINT('Ctrl Pts',(112.736226830982,1074.66336973984,432.248915791649));
#118468=CARTESIAN_POINT('Ctrl Pts',(112.575953438042,1074.68341185282,432.482653942603));
#118469=CARTESIAN_POINT('Ctrl Pts',(112.473527027896,1074.6966302517,432.582863203708));
#118470=CARTESIAN_POINT('Ctrl Pts',(112.2352762265,1074.72791877231,432.739115643008));
#118471=CARTESIAN_POINT('Ctrl Pts',(112.101390509769,1074.74573701192,432.79319551915));
#118472=CARTESIAN_POINT('Ctrl Pts',(111.893683261218,1074.77362868244,432.832771180604));
#118473=CARTESIAN_POINT('Ctrl Pts',(111.825247851777,1074.78285576909,432.839220986145));
#118474=CARTESIAN_POINT('Ctrl Pts',(111.756676799939,1074.79213585482,432.839203336419));
#118475=CARTESIAN_POINT('Origin',(111.756957497769,1067.7251047501,431.748662623815));
#118476=CARTESIAN_POINT('',(111.756957497769,1074.79784893105,432.239203372544));
#118477=CARTESIAN_POINT('',(111.756957497769,1074.80630411877,431.258121875087));
#118478=CARTESIAN_POINT('Ctrl Pts',(111.756957497769,1074.79784893105,432.239203372544));
#118479=CARTESIAN_POINT('Ctrl Pts',(111.725374838794,1074.80211913335,432.239203372544));
#118480=CARTESIAN_POINT('Ctrl Pts',(111.693862381834,1074.80640164172,432.236153273107));
#118481=CARTESIAN_POINT('Ctrl Pts',(111.598702625693,1074.81940105083,432.217553834054));
#118482=CARTESIAN_POINT('Ctrl Pts',(111.537627148781,1074.82783931817,432.192301833779));
#118483=CARTESIAN_POINT('Ctrl Pts',(111.429107335121,1074.84304638832,432.119341812944));
#118484=CARTESIAN_POINT('Ctrl Pts',(111.382666546665,1074.84967409467,432.072427251562));
#118485=CARTESIAN_POINT('Ctrl Pts',(111.31136320506,1074.86015249039,431.963702187915));
#118486=CARTESIAN_POINT('Ctrl Pts',(111.286918958097,1074.86393667771,431.903199231883));
#118487=CARTESIAN_POINT('Ctrl Pts',(111.263109129291,1074.86819548905,431.777002839856));
#118488=CARTESIAN_POINT('Ctrl Pts',(111.263604197717,1074.86867731751,431.712678298726));
#118489=CARTESIAN_POINT('Ctrl Pts',(111.289189338445,1074.86632293511,431.58775498063));
#118490=CARTESIAN_POINT('Ctrl Pts',(111.314036076062,1074.86350825481,431.528429468777));
#118491=CARTESIAN_POINT('Ctrl Pts',(111.385170426667,1074.85489419562,431.422296119667));
#118492=CARTESIAN_POINT('Ctrl Pts',(111.430897821905,1074.84915945784,431.376642252814));
#118493=CARTESIAN_POINT('Ctrl Pts',(111.538405098834,1074.83534679618,431.304643113215));
#118494=CARTESIAN_POINT('Ctrl Pts',(111.599484517994,1074.82735137497,431.279516718815));
#118495=CARTESIAN_POINT('Ctrl Pts',(111.694308950933,1074.81473253188,431.261134356665));
#118496=CARTESIAN_POINT('Ctrl Pts',(111.725507307599,1074.81055040783,431.258133896878));
#118497=CARTESIAN_POINT('Ctrl Pts',(111.756769426889,1074.80632951177,431.258121911136));
#118498=CARTESIAN_POINT('Ctrl Pts',(111.756832117468,1074.80632104752,431.258121887101));
#118499=CARTESIAN_POINT('Ctrl Pts',(111.756894807763,1074.80631258319,431.258121875087));
#118500=CARTESIAN_POINT('Ctrl Pts',(111.756957497769,1074.80630411877,431.258121875087));
#118501=CARTESIAN_POINT('',(111.756957497769,1082.7251047501,431.258121875087));
#118502=CARTESIAN_POINT('',(111.756957497769,1067.7251047501,431.258121875087));
#118503=CARTESIAN_POINT('Origin',(111.756957497769,1082.7251047501,431.748662623815));
#118504=CARTESIAN_POINT('Ctrl Pts',(111.756957497769,1074.80630411877,431.258121875087));
#118505=CARTESIAN_POINT('Ctrl Pts',(111.78894086001,1074.80198571955,431.258121875087));
#118506=CARTESIAN_POINT('Ctrl Pts',(111.82084916161,1074.79764588071,431.261249858237));
#118507=CARTESIAN_POINT('Ctrl Pts',(111.916695267811,1074.78451351391,431.280225632813));
#118508=CARTESIAN_POINT('Ctrl Pts',(111.978012474172,1074.77597625463,431.305828974978));
#118509=CARTESIAN_POINT('Ctrl Pts',(112.086225850602,1074.76063819376,431.379298041251));
#118510=CARTESIAN_POINT('Ctrl Pts',(112.132271420881,1074.75396260125,431.426148010146));
#118511=CARTESIAN_POINT('Ctrl Pts',(112.202836977189,1074.74340516081,431.534368544303));
#118512=CARTESIAN_POINT('Ctrl Pts',(112.227019608748,1074.73958151596,431.594410285604));
#118513=CARTESIAN_POINT('Ctrl Pts',(112.250793234647,1074.73524139378,431.720097888902));
#118514=CARTESIAN_POINT('Ctrl Pts',(112.250327396791,1074.73474438414,431.784424990654));
#118515=CARTESIAN_POINT('Ctrl Pts',(112.224812517838,1074.73714097658,431.90928651105));
#118516=CARTESIAN_POINT('Ctrl Pts',(112.20003784051,1074.74000803974,431.96855198485));
#118517=CARTESIAN_POINT('Ctrl Pts',(112.12910604374,1074.74875875828,432.074596453481));
#118518=CARTESIAN_POINT('Ctrl Pts',(112.083512174581,1074.75457511682,432.120230132115));
#118519=CARTESIAN_POINT('Ctrl Pts',(111.97706736352,1074.76843142764,432.191760203727));
#118520=CARTESIAN_POINT('Ctrl Pts',(111.917087983988,1074.77635989495,432.216765724299));
#118521=CARTESIAN_POINT('Ctrl Pts',(111.822579290969,1074.78900032703,432.235855343108));
#118522=CARTESIAN_POINT('Ctrl Pts',(111.790538507449,1074.79330923836,432.239105481057));
#118523=CARTESIAN_POINT('Ctrl Pts',(111.757932,1074.79771717655,432.239202646579));
#118524=CARTESIAN_POINT('Ctrl Pts',(111.757444740529,1074.79778305233,432.239203372544));
#118525=CARTESIAN_POINT('Ctrl Pts',(111.756957497769,1074.79784893105,432.239203372544));
#118526=CARTESIAN_POINT('Origin',(79.4772023228649,1067.7251047501,383.340094328387));
#118527=CARTESIAN_POINT('',(79.4772023228812,1078.65448750233,381.861791196193));
#118528=CARTESIAN_POINT('Ctrl Pts',(79.4773064989971,1078.68961796465,384.81839745691));
#118529=CARTESIAN_POINT('Ctrl Pts',(79.6578339946104,1078.68607426205,384.818384735123));
#118530=CARTESIAN_POINT('Ctrl Pts',(79.836830601856,1078.68200456401,384.785303885374));
#118531=CARTESIAN_POINT('Ctrl Pts',(80.1867059151628,1078.67273509248,384.651451899359));
#118532=CARTESIAN_POINT('Ctrl Pts',(80.3525634585585,1078.66756101805,384.547071048555));
#118533=CARTESIAN_POINT('Ctrl Pts',(80.6340875241951,1078.65714773939,384.280556940427));
#118534=CARTESIAN_POINT('Ctrl Pts',(80.7471708722345,1078.65201364776,384.121143869101));
#118535=CARTESIAN_POINT('Ctrl Pts',(80.8991655963413,1078.64310803231,383.781853449734));
#118536=CARTESIAN_POINT('Ctrl Pts',(80.9420212089376,1078.63933893738,383.60738718419));
#118537=CARTESIAN_POINT('Ctrl Pts',(80.9635643432908,1078.63342109524,383.25183193677));
#118538=CARTESIAN_POINT('Ctrl Pts',(80.9421538036005,1078.63132275943,383.073660644745));
#118539=CARTESIAN_POINT('Ctrl Pts',(80.876512373027,1078.63000398959,382.861269826507));
#118540=CARTESIAN_POINT('Ctrl Pts',(80.861540351744,1078.62980609948,382.819565948513));
#118541=CARTESIAN_POINT('Ctrl Pts',(80.8337123673341,1078.62958784562,382.751791404895));
#118542=CARTESIAN_POINT('Ctrl Pts',(80.8219202799108,1078.62952980079,382.725315137572));
#118543=CARTESIAN_POINT('Ctrl Pts',(80.7992811203725,1078.62947641101,382.6782574625));
#118544=CARTESIAN_POINT('Ctrl Pts',(80.7887120002637,1078.62947093756,382.657552937272));
#118545=CARTESIAN_POINT('Ctrl Pts',(80.7652055631167,1078.62949821313,382.614068408584));
#118546=CARTESIAN_POINT('Ctrl Pts',(80.7521420397551,1078.62953588972,382.591365607003));
#118547=CARTESIAN_POINT('Ctrl Pts',(80.7157428543219,1078.6296979789,382.531825721137));
#118548=CARTESIAN_POINT('Ctrl Pts',(80.6913691662945,1078.62986333655,382.495653907294));
#118549=CARTESIAN_POINT('Ctrl Pts',(80.5758348535649,1078.6308813964,382.339560419491));
#118550=CARTESIAN_POINT('Ctrl Pts',(80.4682669407166,1078.63242196648,382.232913962992));
#118551=CARTESIAN_POINT('Ctrl Pts',(80.2243706001013,1078.63681483155,382.055608510863));
#118552=CARTESIAN_POINT('Ctrl Pts',(80.0894106673181,1078.63964278792,381.986078311478));
#118553=CARTESIAN_POINT('Ctrl Pts',(79.7880964850754,1078.64655843017,381.885257431442));
#118554=CARTESIAN_POINT('Ctrl Pts',(79.6220920608436,1078.6506949489,381.859484017786));
#118555=CARTESIAN_POINT('Ctrl Pts',(79.2756447960113,1078.65976047334,381.864613338933));
#118556=CARTESIAN_POINT('Ctrl Pts',(79.0979539302923,1078.66464635616,381.900011030537));
#118557=CARTESIAN_POINT('Ctrl Pts',(78.7518267241186,1078.67449913495,382.037642641232));
#118558=CARTESIAN_POINT('Ctrl Pts',(78.5883205091446,1078.67934851276,382.143245868681));
#118559=CARTESIAN_POINT('Ctrl Pts',(78.3103492235038,1078.68806918596,382.411977945481));
#118560=CARTESIAN_POINT('Ctrl Pts',(78.1988380884844,1078.69185427754,382.572800338836));
#118561=CARTESIAN_POINT('Ctrl Pts',(78.0504301882596,1078.69784731183,382.914073895328));
#118562=CARTESIAN_POINT('Ctrl Pts',(78.0094874103787,1078.70011438911,383.089115733394));
#118563=CARTESIAN_POINT('Ctrl Pts',(77.9921229956226,1078.70345252035,383.440919095969));
#118564=CARTESIAN_POINT('Ctrl Pts',(78.0142688186805,1078.70453002803,383.614783512436));
#118565=CARTESIAN_POINT('Ctrl Pts',(78.0791043739633,1078.70520849499,383.82238078746));
#118566=CARTESIAN_POINT('Ctrl Pts',(78.0939237557013,1078.70531014815,383.863371046404));
#118567=CARTESIAN_POINT('Ctrl Pts',(78.1214133705135,1078.70542214587,383.930036077492));
#118568=CARTESIAN_POINT('Ctrl Pts',(78.1330571157045,1078.7054518573,383.956104567591));
#118569=CARTESIAN_POINT('Ctrl Pts',(78.15539559675,1078.70547912024,384.002462978809));
#118570=CARTESIAN_POINT('Ctrl Pts',(78.165821570848,1078.70548185375,384.022872311212));
#118571=CARTESIAN_POINT('Ctrl Pts',(78.1890011987403,1078.70546766206,384.06575632791));
#118572=CARTESIAN_POINT('Ctrl Pts',(78.2018782188641,1078.70544819287,384.088155758255));
#118573=CARTESIAN_POINT('Ctrl Pts',(78.2377454160883,1078.70536440756,384.146925951444));
#118574=CARTESIAN_POINT('Ctrl Pts',(78.2617473919494,1078.70527893162,384.182649959848));
#118575=CARTESIAN_POINT('Ctrl Pts',(78.3753391430794,1078.70475016454,384.33674133563));
#118576=CARTESIAN_POINT('Ctrl Pts',(78.4808951230963,1078.70394945669,384.442264202522));
#118577=CARTESIAN_POINT('Ctrl Pts',(78.7219575096514,1078.70150403823,384.619854943717));
#118578=CARTESIAN_POINT('Ctrl Pts',(78.8565358187346,1078.69985736615,384.690261845773));
#118579=CARTESIAN_POINT('Ctrl Pts',(79.1532792153285,1078.69553142343,384.791605819647));
#118580=CARTESIAN_POINT('Ctrl Pts',(79.3147437498588,1078.69280902447,384.818408912719));
#118581=CARTESIAN_POINT('Ctrl Pts',(79.4773064989971,1078.68961796465,384.81839745691));
#118582=CARTESIAN_POINT('',(79.4772023228652,1076.65355727679,381.861791196194));
#118583=CARTESIAN_POINT('',(79.4772023228649,1067.7251047501,381.861791196194));
#118584=CARTESIAN_POINT('',(79.4772023228649,1076.68910595681,384.81839746058));
#118585=CARTESIAN_POINT('Ctrl Pts',(79.4772023228649,1076.68910595681,384.81839746058));
#118586=CARTESIAN_POINT('Ctrl Pts',(79.4323165774695,1076.68999757484,384.81839746058));
#118587=CARTESIAN_POINT('Ctrl Pts',(79.3877738363708,1076.69084832688,384.81635744192));
#118588=CARTESIAN_POINT('Ctrl Pts',(79.3435699272914,1076.69166091905,384.81234516758));
#118589=CARTESIAN_POINT('Ctrl Pts',(79.2989291589977,1076.69248154192,384.808293240661));
#118590=CARTESIAN_POINT('Ctrl Pts',(79.2546330221333,1076.69326324693,384.802229881876));
#118591=CARTESIAN_POINT('Ctrl Pts',(79.2106740020746,1076.69400882121,384.794172319716));
#118592=CARTESIAN_POINT('Ctrl Pts',(79.2034450509487,1076.69413142904,384.792847273731));
#118593=CARTESIAN_POINT('Ctrl Pts',(79.1962252274782,1076.69425305979,384.791468184736));
#118594=CARTESIAN_POINT('Ctrl Pts',(79.189014517095,1076.69437372585,384.790034995883));
#118595=CARTESIAN_POINT('Ctrl Pts',(79.1508933289145,1076.69501165655,384.782458091654));
#118596=CARTESIAN_POINT('Ctrl Pts',(79.1128619636276,1076.6956246815,384.77333184482));
#118597=CARTESIAN_POINT('Ctrl Pts',(79.0751776100142,1076.69621034861,384.762682209999));
#118598=CARTESIAN_POINT('Ctrl Pts',(79.0375295333672,1076.69679545193,384.752042827084));
#118599=CARTESIAN_POINT('Ctrl Pts',(79.0002284001745,1076.69735325007,384.739883108458));
#118600=CARTESIAN_POINT('Ctrl Pts',(78.9635194136748,1076.69788129803,384.726279748689));
#118601=CARTESIAN_POINT('Ctrl Pts',(78.9459072244516,1076.69813464418,384.719753146645));
#118602=CARTESIAN_POINT('Ctrl Pts',(78.9284311173179,1076.69838114221,384.712894976343));
#118603=CARTESIAN_POINT('Ctrl Pts',(78.9111166457398,1076.6986205221,384.705717686713));
#118604=CARTESIAN_POINT('Ctrl Pts',(78.8693868293314,1076.69919745444,384.688419614566));
#118605=CARTESIAN_POINT('Ctrl Pts',(78.8286635630319,1076.69973316404,384.669302084844));
#118606=CARTESIAN_POINT('Ctrl Pts',(78.7889305802416,1076.70022999697,384.648399399446));
#118607=CARTESIAN_POINT('Ctrl Pts',(78.7491034394834,1076.70072800729,384.627447179524));
#118608=CARTESIAN_POINT('Ctrl Pts',(78.7102704342413,1076.70118695647,384.604700910479));
#118609=CARTESIAN_POINT('Ctrl Pts',(78.6724373642652,1076.70160920733,384.580148162727));
#118610=CARTESIAN_POINT('Ctrl Pts',(78.6670397817217,1076.70166944918,384.57664526215));
#118611=CARTESIAN_POINT('Ctrl Pts',(78.6616626012551,1076.70172894405,384.573105520616));
#118612=CARTESIAN_POINT('Ctrl Pts',(78.6563058918429,1076.70178769882,384.569528832616));
#118613=CARTESIAN_POINT('Ctrl Pts',(78.6261684482637,1076.7021182597,384.54940598769));
#118614=CARTESIAN_POINT('Ctrl Pts',(78.5966145481867,1076.70242534945,384.528065374972));
#118615=CARTESIAN_POINT('Ctrl Pts',(78.5678623889557,1076.7027080878,384.505633274648));
#118616=CARTESIAN_POINT('Ctrl Pts',(78.5391033511076,1076.70299089379,384.483195807706));
#118617=CARTESIAN_POINT('Ctrl Pts',(78.5111469194186,1076.70324933674,384.459666670504));
#118618=CARTESIAN_POINT('Ctrl Pts',(78.4841803351657,1076.70348253576,384.435214176896));
#118619=CARTESIAN_POINT('Ctrl Pts',(78.4662182055165,1076.70363786693,384.418926653926));
#118620=CARTESIAN_POINT('Ctrl Pts',(78.4486945839047,1076.70378199803,384.402230329042));
#118621=CARTESIAN_POINT('Ctrl Pts',(78.4316556816896,1076.70391466873,384.385183976111));
#118622=CARTESIAN_POINT('Ctrl Pts',(78.3965683871994,1076.70418787037,384.350081338761));
#118623=CARTESIAN_POINT('Ctrl Pts',(78.3631689880996,1076.70441584811,384.313125644738));
#118624=CARTESIAN_POINT('Ctrl Pts',(78.3316900422146,1076.70459872642,384.27453628246));
#118625=CARTESIAN_POINT('Ctrl Pts',(78.3002292294129,1076.70478149938,384.235969149139));
#118626=CARTESIAN_POINT('Ctrl Pts',(78.2706870783422,1076.70491922485,384.195770682281));
#118627=CARTESIAN_POINT('Ctrl Pts',(78.2432574468465,1076.70501202707,384.154195178159));
#118628=CARTESIAN_POINT('Ctrl Pts',(78.2158071059045,1076.70510489936,384.112588284419));
#118629=CARTESIAN_POINT('Ctrl Pts',(78.1904728123462,1076.70515278055,384.069602794041));
#118630=CARTESIAN_POINT('Ctrl Pts',(78.1674047872852,1076.70515579517,384.025521615881));
#118631=CARTESIAN_POINT('Ctrl Pts',(78.1469356867591,1076.70515847014,383.986406777716));
#118632=CARTESIAN_POINT('Ctrl Pts',(78.1282504482097,1076.7051258187,383.946429892694));
#118633=CARTESIAN_POINT('Ctrl Pts',(78.1114222681008,1076.70505792785,383.905801843505));
#118634=CARTESIAN_POINT('Ctrl Pts',(78.092545671038,1076.70498177295,383.86022832878));
#118635=CARTESIAN_POINT('Ctrl Pts',(78.0759005429512,1076.7048607265,383.813578976737));
#118636=CARTESIAN_POINT('Ctrl Pts',(78.0616230533806,1076.70469467634,383.766140666781));
#118637=CARTESIAN_POINT('Ctrl Pts',(78.0473559677274,1076.70452874718,383.718736924824));
#118638=CARTESIAN_POINT('Ctrl Pts',(78.0354533023461,1076.70431787986,383.670545949035));
#118639=CARTESIAN_POINT('Ctrl Pts',(78.0260025224258,1076.70406196247,383.621873124356));
#118640=CARTESIAN_POINT('Ctrl Pts',(78.0165466406782,1076.70380590693,383.573174024561));
#118641=CARTESIAN_POINT('Ctrl Pts',(78.0095454198943,1076.70350475266,383.523993164022));
#118642=CARTESIAN_POINT('Ctrl Pts',(78.0050352763836,1076.70315838755,383.474646689596));
#118643=CARTESIAN_POINT('Ctrl Pts',(78.0009506314825,1076.70284469943,383.429955689261));
#118644=CARTESIAN_POINT('Ctrl Pts',(77.9989085705711,1076.7024939287,383.385129306266));
#118645=CARTESIAN_POINT('Ctrl Pts',(77.9988992229576,1076.70210599207,383.340403289638));
#118646=CARTESIAN_POINT('Ctrl Pts',(77.9988916155266,1076.701790275,383.304003615509));
#118647=CARTESIAN_POINT('Ctrl Pts',(78.0002326693678,1076.70144728133,383.267387185696));
#118648=CARTESIAN_POINT('Ctrl Pts',(78.0029444698945,1076.70107842819,383.230806023397));
#118649=CARTESIAN_POINT('Ctrl Pts',(78.005654947569,1076.70070975499,383.194242705874));
#118650=CARTESIAN_POINT('Ctrl Pts',(78.0097348316084,1076.70031524755,383.157715212124));
#118651=CARTESIAN_POINT('Ctrl Pts',(78.0151540721176,1076.69989632095,383.121473507926));
#118652=CARTESIAN_POINT('Ctrl Pts',(78.0186769104227,1076.69962399299,383.097914180087));
#118653=CARTESIAN_POINT('Ctrl Pts',(78.022764660728,1076.69934134599,383.074475563693));
#118654=CARTESIAN_POINT('Ctrl Pts',(78.0273974478024,1076.69904876866,383.051224158765));
#118655=CARTESIAN_POINT('Ctrl Pts',(78.0362211421981,1076.69849152033,383.006939090605));
#118656=CARTESIAN_POINT('Ctrl Pts',(78.0470339763282,1076.69789823608,382.963236436771));
#118657=CARTESIAN_POINT('Ctrl Pts',(78.0598128163726,1076.69726649033,382.920109641121));
#118658=CARTESIAN_POINT('Ctrl Pts',(78.0725773291265,1076.69663545287,382.877031198069));
#118659=CARTESIAN_POINT('Ctrl Pts',(78.0873037191838,1076.69596604009,382.834526420395));
#118660=CARTESIAN_POINT('Ctrl Pts',(78.1040183448495,1076.69525583455,382.792603768492));
#118661=CARTESIAN_POINT('Ctrl Pts',(78.1063929514182,1076.69515493736,382.786647918413));
#118662=CARTESIAN_POINT('Ctrl Pts',(78.1088077641602,1076.69505321684,382.780703855331));
#118663=CARTESIAN_POINT('Ctrl Pts',(78.1112629341433,1076.69495066606,382.774771644434));
#118664=CARTESIAN_POINT('Ctrl Pts',(78.1258989119271,1076.69433933124,382.739408020941));
#118665=CARTESIAN_POINT('Ctrl Pts',(78.1419638050131,1076.69369808852,382.70448981176));
#118666=CARTESIAN_POINT('Ctrl Pts',(78.1593650916418,1076.69303031757,382.670254659022));
#118667=CARTESIAN_POINT('Ctrl Pts',(78.1767815203228,1076.69236196556,382.635989715931));
#118668=CARTESIAN_POINT('Ctrl Pts',(78.1955363984234,1076.69166703914,382.602409562577));
#118669=CARTESIAN_POINT('Ctrl Pts',(78.2154904348338,1076.69094892683,382.569728660503));
#118670=CARTESIAN_POINT('Ctrl Pts',(78.2260517243111,1076.69056884373,382.55243128467));
#118671=CARTESIAN_POINT('Ctrl Pts',(78.2369481848875,1076.69018226538,382.535385372116));
#118672=CARTESIAN_POINT('Ctrl Pts',(78.2481543628143,1076.6897896942,382.51861927548));
#118673=CARTESIAN_POINT('Ctrl Pts',(78.2730325534311,1076.68891816951,382.481397829352));
#118674=CARTESIAN_POINT('Ctrl Pts',(78.299559302157,1076.68801358794,382.445362019445));
#118675=CARTESIAN_POINT('Ctrl Pts',(78.3277429257228,1076.68707374922,382.41051203242));
#118676=CARTESIAN_POINT('Ctrl Pts',(78.3556834593331,1076.68614201682,382.375962634203));
#118677=CARTESIAN_POINT('Ctrl Pts',(78.3852530400077,1076.68517563284,382.342578026162));
#118678=CARTESIAN_POINT('Ctrl Pts',(78.4164955420233,1076.68417245347,382.310394723779));
#118679=CARTESIAN_POINT('Ctrl Pts',(78.4215509809009,1076.68401012614,382.305187051295));
#118680=CARTESIAN_POINT('Ctrl Pts',(78.4266502871599,1076.68384683538,382.300010923153));
#118681=CARTESIAN_POINT('Ctrl Pts',(78.4317937177455,1076.68368257211,382.294866602485));
#118682=CARTESIAN_POINT('Ctrl Pts',(78.4811168907444,1076.68210736162,382.24553489399));
#118683=CARTESIAN_POINT('Ctrl Pts',(78.5336262529255,1076.68046914874,382.19999488545));
#118684=CARTESIAN_POINT('Ctrl Pts',(78.5889038618298,1076.67877789683,382.158440404949));
#118685=CARTESIAN_POINT('Ctrl Pts',(78.646998755554,1076.67700044839,382.114768054132));
#118686=CARTESIAN_POINT('Ctrl Pts',(78.7081529543673,1076.67516441677,382.075495751653));
#118687=CARTESIAN_POINT('Ctrl Pts',(78.7719313713774,1076.6732813677,382.040874163965));
#118688=CARTESIAN_POINT('Ctrl Pts',(78.8172395161129,1076.6719436509,382.016279011255));
#118689=CARTESIAN_POINT('Ctrl Pts',(78.8638732351684,1076.67058220593,381.994031511756));
#118690=CARTESIAN_POINT('Ctrl Pts',(78.9116821341399,1076.66920117927,381.974236697886));
#118691=CARTESIAN_POINT('Ctrl Pts',(78.9534074216605,1076.66799588621,381.956960744707));
#118692=CARTESIAN_POINT('Ctrl Pts',(78.9956969695686,1076.66678565021,381.941686228821));
#118693=CARTESIAN_POINT('Ctrl Pts',(79.0385369690515,1076.66557138359,381.928374505612));
#118694=CARTESIAN_POINT('Ctrl Pts',(79.0815117452,1076.66435329684,381.915020903091));
#118695=CARTESIAN_POINT('Ctrl Pts',(79.1250413371005,1076.66313115407,381.903642156297));
#118696=CARTESIAN_POINT('Ctrl Pts',(79.1691299093578,1076.66190587627,381.894248023039));
#118697=CARTESIAN_POINT('Ctrl Pts',(79.1754387204867,1076.66173054634,381.892903778728));
#118698=CARTESIAN_POINT('Ctrl Pts',(79.1817589940561,1076.66155515221,381.891600256707));
#118699=CARTESIAN_POINT('Ctrl Pts',(79.1880907555688,1076.6613796966,381.890337572131));
#118700=CARTESIAN_POINT('Ctrl Pts',(79.2234843642184,1076.6603989257,381.883279352451));
#118701=CARTESIAN_POINT('Ctrl Pts',(79.259331463925,1076.65941372101,381.877482778857));
#118702=CARTESIAN_POINT('Ctrl Pts',(79.295388881851,1076.65843163133,381.873014227193));
#118703=CARTESIAN_POINT('Ctrl Pts',(79.3314500263962,1076.65744944014,381.868545213694));
#118704=CARTESIAN_POINT('Ctrl Pts',(79.3677209539181,1076.65647036461,381.865404600017));
#118705=CARTESIAN_POINT('Ctrl Pts',(79.4039505509298,1076.6555019559,381.863607170108));
#118706=CARTESIAN_POINT('Ctrl Pts',(79.4284125670731,1076.65484809189,381.862393555742));
#118707=CARTESIAN_POINT('Ctrl Pts',(79.4528555850251,1076.65419909074,381.861791196194));
#118708=CARTESIAN_POINT('Ctrl Pts',(79.4772023228649,1076.65355727679,381.861791196194));
#118709=CARTESIAN_POINT('Ctrl Pts',(79.4772023228652,1076.65355727679,381.861791196194));
#118710=CARTESIAN_POINT('Ctrl Pts',(79.6729707687277,1076.64839654768,381.861791196194));
#118711=CARTESIAN_POINT('Ctrl Pts',(79.866806416513,1076.64358157986,381.900676359504));
#118712=CARTESIAN_POINT('Ctrl Pts',(80.2255548712202,1076.63559755373,382.050669534883));
#118713=CARTESIAN_POINT('Ctrl Pts',(80.3873767252618,1076.632490266,382.159314096149));
#118714=CARTESIAN_POINT('Ctrl Pts',(80.660352144368,1076.62860861734,382.432929539083));
#118715=CARTESIAN_POINT('Ctrl Pts',(80.7687708768473,1076.62787984994,382.595349081387));
#118716=CARTESIAN_POINT('Ctrl Pts',(80.9170871154754,1076.62900365002,382.953166720926));
#118717=CARTESIAN_POINT('Ctrl Pts',(80.955367665541,1076.63085058817,383.145157575024));
#118718=CARTESIAN_POINT('Ctrl Pts',(80.9556418926109,1076.63671612003,383.532075796931));
#118719=CARTESIAN_POINT('Ctrl Pts',(80.9179706056803,1076.64066296239,383.723259023923));
#118720=CARTESIAN_POINT('Ctrl Pts',(80.7712549670908,1076.64983688938,384.080439810865));
#118721=CARTESIAN_POINT('Ctrl Pts',(80.6635672715775,1076.65496970436,384.242987364763));
#118722=CARTESIAN_POINT('Ctrl Pts',(80.4597270928463,1076.66283262355,384.448856776867));
#118723=CARTESIAN_POINT('Ctrl Pts',(80.3852058085155,1076.66546317263,384.510666375708));
#118724=CARTESIAN_POINT('Ctrl Pts',(80.178978583346,1076.67214380466,384.650094652687));
#118725=CARTESIAN_POINT('Ctrl Pts',(80.0403270719585,1076.67609393888,384.715406827373));
#118726=CARTESIAN_POINT('Ctrl Pts',(79.7587501365082,1076.68317131549,384.798185252103));
#118727=CARTESIAN_POINT('Ctrl Pts',(79.6183469796841,1076.6863022355,384.81839746058));
#118728=CARTESIAN_POINT('Ctrl Pts',(79.4772023228649,1076.68910595681,384.81839746058));
#118729=CARTESIAN_POINT('Origin',(79.4772023228649,1067.7251047501,383.340094328387));
#118730=CARTESIAN_POINT('',(79.4772023228649,1076.68289265596,384.21839746058));
#118731=CARTESIAN_POINT('',(79.4772023229628,1076.66179580958,382.461791196194));
#118732=CARTESIAN_POINT('Ctrl Pts',(79.4772023228649,1076.68289265596,384.21839746058));
#118733=CARTESIAN_POINT('Ctrl Pts',(79.3652526559606,1076.68526371833,384.21839746058));
#118734=CARTESIAN_POINT('Ctrl Pts',(79.2542783682972,1076.68729633286,384.196992809842));
#118735=CARTESIAN_POINT('Ctrl Pts',(79.0420083774302,1076.69064094287,384.111866380992));
#118736=CARTESIAN_POINT('Ctrl Pts',(78.9434550090199,1076.69188875241,384.047301429353));
#118737=CARTESIAN_POINT('Ctrl Pts',(78.7771243994947,1076.69343485552,383.883223559309));
#118738=CARTESIAN_POINT('Ctrl Pts',(78.7110935093777,1076.69371708435,383.785264270313));
#118739=CARTESIAN_POINT('Ctrl Pts',(78.6213255463339,1076.69329477762,383.569333997618));
#118740=CARTESIAN_POINT('Ctrl Pts',(78.598450481321,1076.69259474931,383.453539462766));
#118741=CARTESIAN_POINT('Ctrl Pts',(78.5993599252962,1076.69023161065,383.220140723507));
#118742=CARTESIAN_POINT('Ctrl Pts',(78.6230011791956,1076.688592191,383.104862932747));
#118743=CARTESIAN_POINT('Ctrl Pts',(78.7139033442099,1076.68445895829,382.890227975624));
#118744=CARTESIAN_POINT('Ctrl Pts',(78.7802792285221,1076.68200293971,382.793011066017));
#118745=CARTESIAN_POINT('Ctrl Pts',(78.9045559895815,1076.67790004802,382.671697262365));
#118746=CARTESIAN_POINT('Ctrl Pts',(78.9492196479396,1076.67648948421,382.635883802985));
#118747=CARTESIAN_POINT('Ctrl Pts',(79.0456063271205,1076.67355785249,382.572953389854));
#118748=CARTESIAN_POINT('Ctrl Pts',(79.0971921818112,1076.67204256838,382.546134345015));
#118749=CARTESIAN_POINT('Ctrl Pts',(79.2548033101116,1076.6675615439,382.483097553544));
#118750=CARTESIAN_POINT('Ctrl Pts',(79.3655095007989,1076.66459268337,382.461791196169));
#118751=CARTESIAN_POINT('Ctrl Pts',(79.4772023230607,1076.66179580958,382.461791196194));
#118752=CARTESIAN_POINT('',(79.4772023228649,1082.7251047501,382.461791196194));
#118753=CARTESIAN_POINT('',(79.4772023228649,1067.7251047501,382.461791196194));
#118754=CARTESIAN_POINT('Origin',(79.4772023228649,1082.7251047501,383.340094328387));
#118755=CARTESIAN_POINT('Ctrl Pts',(79.4772023230607,1076.66179580958,382.461791196194));
#118756=CARTESIAN_POINT('Ctrl Pts',(79.4806295203402,1076.66170998994,382.461791196194));
#118757=CARTESIAN_POINT('Ctrl Pts',(79.4840576466145,1076.66162433483,382.461811255905));
#118758=CARTESIAN_POINT('Ctrl Pts',(79.6026910282681,1076.65866671775,382.46320045041));
#118759=CARTESIAN_POINT('Ctrl Pts',(79.7165197423068,1076.65604185539,382.487204617594));
#118760=CARTESIAN_POINT('Ctrl Pts',(79.9283760477523,1076.65170526073,382.577778928352));
#118761=CARTESIAN_POINT('Ctrl Pts',(80.0243554599845,1076.65003774835,382.643452765418));
#118762=CARTESIAN_POINT('Ctrl Pts',(80.1853883939126,1076.64799329725,382.808001150205));
#118763=CARTESIAN_POINT('Ctrl Pts',(80.2489203113362,1076.64763587441,382.90523468599));
#118764=CARTESIAN_POINT('Ctrl Pts',(80.3321322595537,1076.64829141853,383.111827764756));
#118765=CARTESIAN_POINT('Ctrl Pts',(80.353651967693,1076.64921177656,383.218254704458));
#118766=CARTESIAN_POINT('Ctrl Pts',(80.3553908959406,1076.65066400983,383.325909049407));
#118767=CARTESIAN_POINT('Ctrl Pts',(80.3572452836985,1076.65221266695,383.440711313171));
#118768=CARTESIAN_POINT('Ctrl Pts',(80.3365703578649,1076.65433562453,383.554761917856));
#118769=CARTESIAN_POINT('Ctrl Pts',(80.2525014000806,1076.65937701402,383.768488947881));
#118770=CARTESIAN_POINT('Ctrl Pts',(80.1898930480443,1076.66224474932,383.866098161961));
#118771=CARTESIAN_POINT('Ctrl Pts',(80.070492135499,1076.6667429314,383.990262667662));
#118772=CARTESIAN_POINT('Ctrl Pts',(80.0267418154695,1076.66826425098,384.027639208293));
#118773=CARTESIAN_POINT('Ctrl Pts',(79.9325698297907,1076.671300918,384.093322675064));
#118774=CARTESIAN_POINT('Ctrl Pts',(79.8823730763377,1076.67280895582,384.121470869562));
#118775=CARTESIAN_POINT('Ctrl Pts',(79.7227328060416,1076.67728776372,384.191442760892));
#118776=CARTESIAN_POINT('Ctrl Pts',(79.6073729687394,1076.68010796009,384.216528949717));
#118777=CARTESIAN_POINT('Ctrl Pts',(79.4860569412789,1076.68270462264,384.2183639967));
#118778=CARTESIAN_POINT('Ctrl Pts',(79.4816288695732,1076.68279890295,384.21839746058));
#118779=CARTESIAN_POINT('Ctrl Pts',(79.4772023228649,1076.68289265596,384.21839746058));
#118780=CARTESIAN_POINT('Origin',(90.2477595453611,1067.7251047501,389.798048628597));
#118781=CARTESIAN_POINT('',(90.247759545381,1078.31906551735,388.522604507461));
#118782=CARTESIAN_POINT('Ctrl Pts',(90.2479786339883,1078.37784002205,391.073492730917));
#118783=CARTESIAN_POINT('Ctrl Pts',(90.4072924505591,1078.36862711137,391.073465364884));
#118784=CARTESIAN_POINT('Ctrl Pts',(90.5651682441571,1078.35867651224,391.04358936537));
#118785=CARTESIAN_POINT('Ctrl Pts',(90.8708245606265,1078.33764550322,390.923717765228));
#118786=CARTESIAN_POINT('Ctrl Pts',(91.0144009896261,1078.32673821539,390.831301921722));
#118787=CARTESIAN_POINT('Ctrl Pts',(91.2543335457832,1078.30637295623,390.598576482715));
#118788=CARTESIAN_POINT('Ctrl Pts',(91.349470918864,1078.29708085559,390.461603592906));
#118789=CARTESIAN_POINT('Ctrl Pts',(91.4710866406911,1078.28258950731,390.184252922138));
#118790=CARTESIAN_POINT('Ctrl Pts',(91.5056040894251,1078.27706243863,390.050110186705));
#118791=CARTESIAN_POINT('Ctrl Pts',(91.5295394970062,1078.26895950706,389.785640309555));
#118792=CARTESIAN_POINT('Ctrl Pts',(91.5218465334233,1078.26624929792,389.657232693508));
#118793=CARTESIAN_POINT('Ctrl Pts',(91.4874399942531,1078.26444461193,389.495849786554));
#118794=CARTESIAN_POINT('Ctrl Pts',(91.4781338812537,1078.2641499748,389.459949707738));
#118795=CARTESIAN_POINT('Ctrl Pts',(91.4609077209896,1078.2638600006,389.403710981464));
#118796=CARTESIAN_POINT('Ctrl Pts',(91.4540075087571,1078.26379133505,389.383082922125));
#118797=CARTESIAN_POINT('Ctrl Pts',(91.4402753035378,1078.2637358018,389.345273516858));
#118798=CARTESIAN_POINT('Ctrl Pts',(91.433590732954,1078.26373819292,389.328044873608));
#118799=CARTESIAN_POINT('Ctrl Pts',(91.4179825826874,1078.2638051891,389.29027191666));
#118800=CARTESIAN_POINT('Ctrl Pts',(91.4088874543157,1078.26388285747,389.269805206658));
#118801=CARTESIAN_POINT('Ctrl Pts',(91.3816603437648,1078.26421798979,389.212641533564));
#118802=CARTESIAN_POINT('Ctrl Pts',(91.3622948430431,1078.26457087267,389.176563819338));
#118803=CARTESIAN_POINT('Ctrl Pts',(91.2535722341533,1078.26708713355,388.995493658735));
#118804=CARTESIAN_POINT('Ctrl Pts',(91.1375907889607,1078.27142677805,388.868575846934));
#118805=CARTESIAN_POINT('Ctrl Pts',(90.8906327389324,1078.28278379058,388.688149139343));
#118806=CARTESIAN_POINT('Ctrl Pts',(90.7690566330834,1078.28900378146,388.626132389191));
#118807=CARTESIAN_POINT('Ctrl Pts',(90.4989402363623,1078.30389328142,388.538818864234));
#118808=CARTESIAN_POINT('Ctrl Pts',(90.3509870841868,1078.31262280569,388.518176868577));
#118809=CARTESIAN_POINT('Ctrl Pts',(90.0435750160734,1078.33176483397,388.52900630582));
#118810=CARTESIAN_POINT('Ctrl Pts',(89.8867552869763,1078.34208576919,388.564423401423));
#118811=CARTESIAN_POINT('Ctrl Pts',(89.5854871661062,1078.36301604762,388.695003523307));
#118812=CARTESIAN_POINT('Ctrl Pts',(89.4452958580764,1078.37340027826,388.792369144175));
#118813=CARTESIAN_POINT('Ctrl Pts',(89.2139757836579,1078.39203626485,389.033065941907));
#118814=CARTESIAN_POINT('Ctrl Pts',(89.1238577013517,1078.40016459864,389.172916564038));
#118815=CARTESIAN_POINT('Ctrl Pts',(89.0106452550058,1078.41260133766,389.45715746681));
#118816=CARTESIAN_POINT('Ctrl Pts',(88.980534804604,1078.41720851734,389.5960066182));
#118817=CARTESIAN_POINT('Ctrl Pts',(88.9683368003032,1078.42325841467,389.850514311394));
#118818=CARTESIAN_POINT('Ctrl Pts',(88.9780938792126,1078.42511565541,389.964272834517));
#118819=CARTESIAN_POINT('Ctrl Pts',(89.0105033558247,1078.42640768506,390.109835672536));
#118820=CARTESIAN_POINT('Ctrl Pts',(89.0196454770702,1078.42662929179,390.144097686916));
#118821=CARTESIAN_POINT('Ctrl Pts',(89.0364608738141,1078.42684554273,390.197991983752));
#118822=CARTESIAN_POINT('Ctrl Pts',(89.0432135346738,1078.42689582628,390.217891543741));
#118823=CARTESIAN_POINT('Ctrl Pts',(89.0567634727298,1078.42693336289,390.254799274328));
#118824=CARTESIAN_POINT('Ctrl Pts',(89.0634414568015,1078.42692789351,390.271845486051));
#118825=CARTESIAN_POINT('Ctrl Pts',(89.079238194387,1078.42686416128,390.309745144983));
#118826=CARTESIAN_POINT('Ctrl Pts',(89.0885528293671,1078.42679340296,390.330510131756));
#118827=CARTESIAN_POINT('Ctrl Pts',(89.1171692155467,1078.42648547983,390.389989377509));
#118828=CARTESIAN_POINT('Ctrl Pts',(89.1378904746825,1078.42615605807,390.427984199798));
#118829=CARTESIAN_POINT('Ctrl Pts',(89.2494796056993,1078.42390412141,390.609936239275));
#118830=CARTESIAN_POINT('Ctrl Pts',(89.3665830158952,1078.42017199153,390.73571927123));
#118831=CARTESIAN_POINT('Ctrl Pts',(89.6158695138219,1078.41020970893,390.914346516717));
#118832=CARTESIAN_POINT('Ctrl Pts',(89.7388957093978,1078.4046794162,390.975521365935));
#118833=CARTESIAN_POINT('Ctrl Pts',(89.9918960393226,1078.3921179301,391.054150890187));
#118834=CARTESIAN_POINT('Ctrl Pts',(90.1195896616231,1078.38526458923,391.073514784854));
#118835=CARTESIAN_POINT('Ctrl Pts',(90.2479786339883,1078.37784002205,391.073492730917));
#118836=CARTESIAN_POINT('',(90.2477595453332,1076.31447289884,388.522604507461));
#118837=CARTESIAN_POINT('',(90.2477595453611,1067.7251047501,388.522604507461));
#118838=CARTESIAN_POINT('Ctrl Pts',(90.2473924269198,1076.37389480859,391.073492696899));
#118839=CARTESIAN_POINT('Ctrl Pts',(90.0786678211981,1076.38375238938,391.07344413192));
#118840=CARTESIAN_POINT('Ctrl Pts',(89.9115576809659,1076.39258810219,391.039916041364));
#118841=CARTESIAN_POINT('Ctrl Pts',(89.6001222777372,1076.40737676698,390.909708654403));
#118842=CARTESIAN_POINT('Ctrl Pts',(89.4588627501205,1076.41319074441,390.814365881412));
#118843=CARTESIAN_POINT('Ctrl Pts',(89.2212821771998,1076.4212058014,390.573782629421));
#118844=CARTESIAN_POINT('Ctrl Pts',(89.1274746485026,1076.42332030174,390.430817231719));
#118845=CARTESIAN_POINT('Ctrl Pts',(89.0011623088369,1076.42359751866,390.116542235314));
#118846=CARTESIAN_POINT('Ctrl Pts',(88.9699388158943,1076.4217570164,389.9483936573));
#118847=CARTESIAN_POINT('Ctrl Pts',(88.974966989438,1076.41426223305,389.610248087243));
#118848=CARTESIAN_POINT('Ctrl Pts',(89.0109791987585,1076.40868962099,389.443635792331));
#118849=CARTESIAN_POINT('Ctrl Pts',(89.1457249137492,1076.39432665083,389.134141610723));
#118850=CARTESIAN_POINT('Ctrl Pts',(89.2431414882275,1076.38567244326,388.994335807397));
#118851=CARTESIAN_POINT('Ctrl Pts',(89.4875261158289,1076.36615484006,388.759933106992));
#118852=CARTESIAN_POINT('Ctrl Pts',(89.632428630942,1076.35546600574,388.668012091641));
#118853=CARTESIAN_POINT('Ctrl Pts',(89.9490985165273,1076.33352043879,388.546562565143));
#118854=CARTESIAN_POINT('Ctrl Pts',(90.1176726428313,1076.3224810292,388.51800816092));
#118855=CARTESIAN_POINT('Ctrl Pts',(90.454422931293,1076.30172067755,388.528349923876));
#118856=CARTESIAN_POINT('Ctrl Pts',(90.6193498029185,1076.2921906145,388.566462382039));
#118857=CARTESIAN_POINT('Ctrl Pts',(90.9247820613952,1076.27603432292,388.70424411318));
#118858=CARTESIAN_POINT('Ctrl Pts',(91.0623730244936,1076.26956346593,388.802450032287));
#118859=CARTESIAN_POINT('Ctrl Pts',(91.291415537799,1076.26077000566,389.046115902754));
#118860=CARTESIAN_POINT('Ctrl Pts',(91.3807791954783,1076.25852248664,389.18902839898));
#118861=CARTESIAN_POINT('Ctrl Pts',(91.4992089951027,1076.25864459449,389.500791779399));
#118862=CARTESIAN_POINT('Ctrl Pts',(91.5272777349046,1076.26100037752,389.666514235576));
#118863=CARTESIAN_POINT('Ctrl Pts',(91.5181766731156,1076.26995313121,389.999301759715));
#118864=CARTESIAN_POINT('Ctrl Pts',(91.4811032128848,1076.27645944988,390.163127478227));
#118865=CARTESIAN_POINT('Ctrl Pts',(91.3460764523357,1076.29262394204,390.467566296283));
#118866=CARTESIAN_POINT('Ctrl Pts',(91.2492760870129,1076.30212968719,390.60519176657));
#118867=CARTESIAN_POINT('Ctrl Pts',(91.0080112746451,1076.32272303391,390.83568287336));
#118868=CARTESIAN_POINT('Ctrl Pts',(90.8657207867423,1076.33361480845,390.926224837942));
#118869=CARTESIAN_POINT('Ctrl Pts',(90.5625742841719,1076.3546622751,391.044116987762));
#118870=CARTESIAN_POINT('Ctrl Pts',(90.4056823246697,1076.36464686607,391.073538258395));
#118871=CARTESIAN_POINT('Ctrl Pts',(90.2473924269198,1076.37389480859,391.073492696899));
#118872=CARTESIAN_POINT('Origin',(90.2477595453611,1067.7251047501,389.798048628597));
#118873=CARTESIAN_POINT('',(90.2477595453611,1076.3606248843,390.473492749734));
#118874=CARTESIAN_POINT('',(90.2477595453612,1076.32917837425,389.122604507461));
#118875=CARTESIAN_POINT('Ctrl Pts',(90.2477595453611,1076.3606248843,390.473492749734));
#118876=CARTESIAN_POINT('Ctrl Pts',(90.2043920721301,1076.36319732881,390.473492749734));
#118877=CARTESIAN_POINT('Ctrl Pts',(90.1610125495164,1076.36566376778,390.469316146937));
#118878=CARTESIAN_POINT('Ctrl Pts',(90.0301266378503,1076.37278298611,390.443741260242));
#118879=CARTESIAN_POINT('Ctrl Pts',(89.9463009289524,1076.3768891315,390.409127887364));
#118880=CARTESIAN_POINT('Ctrl Pts',(89.7970259838005,1076.38330872468,390.309068283425));
#118881=CARTESIAN_POINT('Ctrl Pts',(89.7330857382475,1076.38555825709,390.244614648894));
#118882=CARTESIAN_POINT('Ctrl Pts',(89.6341405527321,1076.38791588244,390.094351645691));
#118883=CARTESIAN_POINT('Ctrl Pts',(89.6001639605402,1076.3879988915,390.010048714635));
#118884=CARTESIAN_POINT('Ctrl Pts',(89.5672600607563,1076.38596507471,389.833156887381));
#118885=CARTESIAN_POINT('Ctrl Pts',(89.5686397960403,1076.38386995074,389.742366687895));
#118886=CARTESIAN_POINT('Ctrl Pts',(89.6068257228187,1076.37772919497,389.566750407836));
#118887=CARTESIAN_POINT('Ctrl Pts',(89.6432272718938,1076.37374505058,389.483686272504));
#118888=CARTESIAN_POINT('Ctrl Pts',(89.7464541356269,1076.36434306899,389.336510143142));
#118889=CARTESIAN_POINT('Ctrl Pts',(89.8123271951584,1076.35901407682,389.27391686985));
#118890=CARTESIAN_POINT('Ctrl Pts',(89.9650841166153,1076.34766646312,389.177968647693));
#118891=CARTESIAN_POINT('Ctrl Pts',(90.0505569705632,1076.34175694847,389.145733736912));
#118892=CARTESIAN_POINT('Ctrl Pts',(90.1754297270574,1076.33367615497,389.125520878135));
#118893=CARTESIAN_POINT('Ctrl Pts',(90.2114348409469,1076.33140664045,389.122618319795));
#118894=CARTESIAN_POINT('Ctrl Pts',(90.2475017958103,1076.32919418435,389.12260455664));
#118895=CARTESIAN_POINT('Ctrl Pts',(90.2475877131029,1076.32918891392,389.122604523854));
#118896=CARTESIAN_POINT('Ctrl Pts',(90.2476736296214,1076.32918364389,389.122604507461));
#118897=CARTESIAN_POINT('Ctrl Pts',(90.2477595453612,1076.32917837425,389.122604507461));
#118898=CARTESIAN_POINT('',(90.2477595453611,1082.7251047501,389.122604507461));
#118899=CARTESIAN_POINT('',(90.2477595453611,1067.7251047501,389.122604507461));
#118900=CARTESIAN_POINT('Origin',(90.2477595453611,1082.7251047501,389.798048628597));
#118901=CARTESIAN_POINT('Ctrl Pts',(90.2477595453612,1076.32917837425,389.122604507461));
#118902=CARTESIAN_POINT('Ctrl Pts',(90.3363441354781,1076.32374504016,389.122604507461));
#118903=CARTESIAN_POINT('Ctrl Pts',(90.4241007966864,1076.31872897983,389.140031364471));
#118904=CARTESIAN_POINT('Ctrl Pts',(90.587837013375,1076.31016472553,389.207782768556));
#118905=CARTESIAN_POINT('Ctrl Pts',(90.6622418995852,1076.30669931367,389.257416805097));
#118906=CARTESIAN_POINT('Ctrl Pts',(90.7875044729904,1076.30185856023,389.382464264245));
#118907=CARTESIAN_POINT('Ctrl Pts',(90.8372022803927,1076.3005257356,389.456584447126));
#118908=CARTESIAN_POINT('Ctrl Pts',(90.9051620205711,1076.30020727945,389.619631964433));
#118909=CARTESIAN_POINT('Ctrl Pts',(90.9228181857498,1076.30122032886,389.706932955501));
#118910=CARTESIAN_POINT('Ctrl Pts',(90.9235767550121,1076.30545578206,389.883377994996));
#118911=CARTESIAN_POINT('Ctrl Pts',(90.9066640330344,1076.30863653759,389.970801489982));
#118912=CARTESIAN_POINT('Ctrl Pts',(90.8401661034984,1076.31671697932,390.134333828792));
#118913=CARTESIAN_POINT('Ctrl Pts',(90.7911515887479,1076.32154108136,390.208837027244));
#118914=CARTESIAN_POINT('Ctrl Pts',(90.6671338231893,1076.33215574363,390.334878350438));
#118915=CARTESIAN_POINT('Ctrl Pts',(90.593254242526,1076.33784599028,390.385151674791));
#118916=CARTESIAN_POINT('Ctrl Pts',(90.471117276196,1076.34643557514,390.437024038278));
#118917=CARTESIAN_POINT('Ctrl Pts',(90.4288363024025,1076.3492860713,390.450267765535));
#118918=CARTESIAN_POINT('Ctrl Pts',(90.3401321550213,1076.35502446918,390.468754036599));
#118919=CARTESIAN_POINT('Ctrl Pts',(90.2939526865699,1076.35788482859,390.473492749734));
#118920=CARTESIAN_POINT('Ctrl Pts',(90.2477595453611,1076.3606248843,390.473492749734));
#118921=CARTESIAN_POINT('Origin',(101.429261354593,1067.7251047501,397.970702670951));
#118922=CARTESIAN_POINT('',(101.429261354616,1077.63689261564,396.871871534958));
#118923=CARTESIAN_POINT('Ctrl Pts',(101.429493570798,1077.6944933282,399.069533782406));
#118924=CARTESIAN_POINT('Ctrl Pts',(101.570114169588,1077.68059568689,399.069504065026));
#118925=CARTESIAN_POINT('Ctrl Pts',(101.709401215988,1077.66602446619,399.042481726076));
#118926=CARTESIAN_POINT('Ctrl Pts',(101.974745505556,1077.63660140021,398.935609334865));
#118927=CARTESIAN_POINT('Ctrl Pts',(102.097645727388,1077.62203792686,398.85495706354));
#118928=CARTESIAN_POINT('Ctrl Pts',(102.300390061509,1077.59607657363,398.654778498191));
#118929=CARTESIAN_POINT('Ctrl Pts',(102.38008642834,1077.58480050336,398.538884121675));
#118930=CARTESIAN_POINT('Ctrl Pts',(102.486863479351,1077.56724256247,398.294764832151));
#118931=CARTESIAN_POINT('Ctrl Pts',(102.517235416251,1077.56073649119,398.170454293728));
#118932=CARTESIAN_POINT('Ctrl Pts',(102.530485929281,1077.5539583423,397.971211786179));
#118933=CARTESIAN_POINT('Ctrl Pts',(102.528118025575,1077.55222622028,397.898488200265));
#118934=CARTESIAN_POINT('Ctrl Pts',(102.515183338414,1077.5509077762,397.800768043311));
#118935=CARTESIAN_POINT('Ctrl Pts',(102.510863688064,1077.55065819879,397.775150056597));
#118936=CARTESIAN_POINT('Ctrl Pts',(102.502325967931,1077.55041101339,397.733566093651));
#118937=CARTESIAN_POINT('Ctrl Pts',(102.498649030552,1077.55035468184,397.717500322744));
#118938=CARTESIAN_POINT('Ctrl Pts',(102.490877245652,1077.5503226105,397.686741376454));
#118939=CARTESIAN_POINT('Ctrl Pts',(102.486835124766,1077.55034116017,397.672038920362));
#118940=CARTESIAN_POINT('Ctrl Pts',(102.476813549706,1077.55046219606,397.638346744497));
#118941=CARTESIAN_POINT('Ctrl Pts',(102.47062145392,1077.55058857402,397.61942617132));
#118942=CARTESIAN_POINT('Ctrl Pts',(102.449874079969,1077.55115830721,397.561411632438));
#118943=CARTESIAN_POINT('Ctrl Pts',(102.433605780676,1077.5517967795,397.522973810068));
#118944=CARTESIAN_POINT('Ctrl Pts',(102.350770301885,1077.55579018709,397.354632119186));
#118945=CARTESIAN_POINT('Ctrl Pts',(102.260963329105,1077.56190750512,397.237947552194));
#118946=CARTESIAN_POINT('Ctrl Pts',(102.062286967439,1077.5776687232,397.064839397336));
#118947=CARTESIAN_POINT('Ctrl Pts',(101.961669014374,1077.58630768889,397.002299025535));
#118948=CARTESIAN_POINT('Ctrl Pts',(101.734340889773,1077.60696342372,396.907245255332));
#118949=CARTESIAN_POINT('Ctrl Pts',(101.607799466399,1077.61906353407,396.878872319039));
#118950=CARTESIAN_POINT('Ctrl Pts',(101.340870322989,1077.64568030702,396.866697678955));
#118951=CARTESIAN_POINT('Ctrl Pts',(101.202482023023,1077.66007960346,396.886636115246));
#118952=CARTESIAN_POINT('Ctrl Pts',(100.933620267909,1077.6892557907,396.979225792778));
#118953=CARTESIAN_POINT('Ctrl Pts',(100.806507605167,1077.70373406477,397.053689947072));
#118954=CARTESIAN_POINT('Ctrl Pts',(100.592365051029,1077.72965371775,397.244801758827));
#118955=CARTESIAN_POINT('Ctrl Pts',(100.506089086297,1077.74094623503,397.358204768748));
#118956=CARTESIAN_POINT('Ctrl Pts',(100.38954102776,1077.75825520151,397.594700476585));
#118957=CARTESIAN_POINT('Ctrl Pts',(100.354127119112,1077.76465594977,397.712778277675));
#118958=CARTESIAN_POINT('Ctrl Pts',(100.327844372379,1077.7724947124,397.922933852471));
#118959=CARTESIAN_POINT('Ctrl Pts',(100.327600168607,1077.77477782493,398.012573491737));
#118960=CARTESIAN_POINT('Ctrl Pts',(100.34157339482,1077.77638028477,398.129331870532));
#118961=CARTESIAN_POINT('Ctrl Pts',(100.346012245204,1077.77665805758,398.15724974196));
#118962=CARTESIAN_POINT('Ctrl Pts',(100.354818878955,1077.77692965227,398.201546788563));
#118963=CARTESIAN_POINT('Ctrl Pts',(100.358497412579,1077.77699268152,398.218049050297));
#118964=CARTESIAN_POINT('Ctrl Pts',(100.365790839327,1077.7770364592,398.247545643728));
#118965=CARTESIAN_POINT('Ctrl Pts',(100.369266953818,1077.77703128813,398.260570639017));
#118966=CARTESIAN_POINT('Ctrl Pts',(100.377936098852,1077.77696183636,398.290809289014));
#118967=CARTESIAN_POINT('Ctrl Pts',(100.383313660878,1077.77687842146,398.307965845557));
#118968=CARTESIAN_POINT('Ctrl Pts',(100.39975632701,1077.77651792379,398.356240863478));
#118969=CARTESIAN_POINT('Ctrl Pts',(100.411806143182,1077.77613738196,398.387001811308));
#118970=CARTESIAN_POINT('Ctrl Pts',(100.484498084542,1077.77328380231,398.550474620684));
#118971=CARTESIAN_POINT('Ctrl Pts',(100.569691975595,1077.76813744088,398.670561399635));
#118972=CARTESIAN_POINT('Ctrl Pts',(100.760535136054,1077.75427983179,398.850364712881));
#118973=CARTESIAN_POINT('Ctrl Pts',(100.857419397221,1077.74657847039,398.916194746146));
#118974=CARTESIAN_POINT('Ctrl Pts',(101.039521930982,1077.73103980715,399.001589257506));
#118975=CARTESIAN_POINT('Ctrl Pts',(101.120183985121,1077.72385589326,399.028568136013));
#118976=CARTESIAN_POINT('Ctrl Pts',(101.27757129444,1077.70927321966,399.061671103831));
#118977=CARTESIAN_POINT('Ctrl Pts',(101.353445151774,1077.70200925161,399.069549853735));
#118978=CARTESIAN_POINT('Ctrl Pts',(101.429493570798,1077.6944933282,399.069533782406));
#118979=CARTESIAN_POINT('',(101.429261354572,1075.62570687173,396.871871534959));
#118980=CARTESIAN_POINT('',(101.429261354593,1067.7251047501,396.871871534959));
#118981=CARTESIAN_POINT('Ctrl Pts',(101.428824109534,1075.68390181721,399.06953371995));
#118982=CARTESIAN_POINT('Ctrl Pts',(101.283118147846,1075.69843181531,399.069475740871));
#118983=CARTESIAN_POINT('Ctrl Pts',(101.13874912924,1075.71195732163,399.040437274791));
#118984=CARTESIAN_POINT('Ctrl Pts',(100.869966130838,1075.73547780411,398.927676464783));
#118985=CARTESIAN_POINT('Ctrl Pts',(100.748147277168,1075.74525357799,398.845216604272));
#118986=CARTESIAN_POINT('Ctrl Pts',(100.543500785851,1075.75984986348,398.637170030997));
#118987=CARTESIAN_POINT('Ctrl Pts',(100.462816124142,1075.76451724927,398.513641006511));
#118988=CARTESIAN_POINT('Ctrl Pts',(100.355577104622,1075.76806198767,398.244832180365));
#118989=CARTESIAN_POINT('Ctrl Pts',(100.329030698117,1075.7670195189,398.102712524122));
#118990=CARTESIAN_POINT('Ctrl Pts',(100.331972350312,1075.75936870649,397.813495563413));
#118991=CARTESIAN_POINT('Ctrl Pts',(100.36255146929,1075.75272765045,397.669334337659));
#118992=CARTESIAN_POINT('Ctrl Pts',(100.478051834914,1075.73458193086,397.401599442797));
#118993=CARTESIAN_POINT('Ctrl Pts',(100.561787929872,1075.72325879679,397.280713035585));
#118994=CARTESIAN_POINT('Ctrl Pts',(100.771752308137,1075.69725319785,397.07824217027));
#118995=CARTESIAN_POINT('Ctrl Pts',(100.896119724191,1075.68280793521,396.998843706387));
#118996=CARTESIAN_POINT('Ctrl Pts',(101.099118750661,1075.66037880992,396.92019080175));
#118997=CARTESIAN_POINT('Ctrl Pts',(101.168337372211,1075.65290133642,396.900895733485));
#118998=CARTESIAN_POINT('Ctrl Pts',(101.382892660413,1075.63022365326,396.863162951671));
#118999=CARTESIAN_POINT('Ctrl Pts',(101.530533126309,1075.61528668515,396.866810028771));
#119000=CARTESIAN_POINT('Ctrl Pts',(101.814062762848,1075.58797342294,396.931360455569));
#119001=CARTESIAN_POINT('Ctrl Pts',(101.947377545443,1075.57582990881,396.990936590587));
#119002=CARTESIAN_POINT('Ctrl Pts',(102.182729390908,1075.55599730865,397.158041962838));
#119003=CARTESIAN_POINT('Ctrl Pts',(102.282654681582,1075.54847789514,397.263649463309));
#119004=CARTESIAN_POINT('Ctrl Pts',(102.435678626395,1075.53918627221,397.506933630482));
#119005=CARTESIAN_POINT('Ctrl Pts',(102.487527926722,1075.53747427039,397.641995746359));
#119006=CARTESIAN_POINT('Ctrl Pts',(102.536384974375,1075.5401145013,397.924169840587));
#119007=CARTESIAN_POINT('Ctrl Pts',(102.533023360652,1075.54442675161,398.06843602517));
#119008=CARTESIAN_POINT('Ctrl Pts',(102.471234631415,1075.55849440184,398.347879580521));
#119009=CARTESIAN_POINT('Ctrl Pts',(102.413246441751,1075.5681258234,398.480273664585));
#119010=CARTESIAN_POINT('Ctrl Pts',(102.249486945095,1075.59140627521,398.715940073188));
#119011=CARTESIAN_POINT('Ctrl Pts',(102.14499270199,1075.60485359843,398.816758062767));
#119012=CARTESIAN_POINT('Ctrl Pts',(101.963519900669,1075.62647206832,398.933615686175));
#119013=CARTESIAN_POINT('Ctrl Pts',(101.89918202132,1075.63388506018,398.966596438669));
#119014=CARTESIAN_POINT('Ctrl Pts',(101.768280558606,1075.64849837418,399.018175774439));
#119015=CARTESIAN_POINT('Ctrl Pts',(101.702254414096,1075.6556606865,399.037290202223));
#119016=CARTESIAN_POINT('Ctrl Pts',(101.56697018122,1075.66992994431,399.063060186457));
#119017=CARTESIAN_POINT('Ctrl Pts',(101.497979788506,1075.67700551817,399.069561238265));
#119018=CARTESIAN_POINT('Ctrl Pts',(101.428824109533,1075.68390181721,399.06953371995));
#119019=CARTESIAN_POINT('Origin',(101.429261354593,1067.7251047501,397.970702670951));
#119020=CARTESIAN_POINT('',(101.429261354593,1075.66856733728,398.469533806944));
#119021=CARTESIAN_POINT('',(101.429261354593,1075.64217240143,397.471871534959));
#119022=CARTESIAN_POINT('Ctrl Pts',(101.429261354593,1075.66856733728,398.469533806944));
#119023=CARTESIAN_POINT('Ctrl Pts',(101.396725259188,1075.67182918461,398.469533806944));
#119024=CARTESIAN_POINT('Ctrl Pts',(101.364178506132,1075.67500282734,398.466350650069));
#119025=CARTESIAN_POINT('Ctrl Pts',(101.266977566166,1075.68420943944,398.447046565021));
#119026=CARTESIAN_POINT('Ctrl Pts',(101.205032551033,1075.6897021991,398.421233424481));
#119027=CARTESIAN_POINT('Ctrl Pts',(101.094874904145,1075.69870538601,398.346778844227));
#119028=CARTESIAN_POINT('Ctrl Pts',(101.047762299093,1075.70212737812,398.298911441355));
#119029=CARTESIAN_POINT('Ctrl Pts',(100.975899018794,1075.70637630619,398.188697938427));
#119030=CARTESIAN_POINT('Ctrl Pts',(100.951367518801,1075.70721976277,398.127804081999));
#119031=CARTESIAN_POINT('Ctrl Pts',(100.927061625673,1075.70630237684,398.00000569481));
#119032=CARTESIAN_POINT('Ctrl Pts',(100.927528876131,1075.70455067681,397.934375840882));
#119033=CARTESIAN_POINT('Ctrl Pts',(100.953630317649,1075.69864101878,397.806803050874));
#119034=CARTESIAN_POINT('Ctrl Pts',(100.979102284652,1075.69453192855,397.746138789854));
#119035=CARTESIAN_POINT('Ctrl Pts',(101.052616408138,1075.68435848275,397.636941267692));
#119036=CARTESIAN_POINT('Ctrl Pts',(101.100398225715,1075.67835508124,397.589793552283));
#119037=CARTESIAN_POINT('Ctrl Pts',(101.183162262418,1075.66864061709,397.535586954051));
#119038=CARTESIAN_POINT('Ctrl Pts',(101.212043073601,1075.66534555193,397.520474218651));
#119039=CARTESIAN_POINT('Ctrl Pts',(101.271649811749,1075.65871997472,397.496359259037));
#119040=CARTESIAN_POINT('Ctrl Pts',(101.302189757706,1075.65540641244,397.487281858555));
#119041=CARTESIAN_POINT('Ctrl Pts',(101.364879120949,1075.64876173334,397.475003708015));
#119042=CARTESIAN_POINT('Ctrl Pts',(101.396901311918,1075.64544559241,397.471888121455));
#119043=CARTESIAN_POINT('Ctrl Pts',(101.429004655058,1075.64219836474,397.471871601006));
#119044=CARTESIAN_POINT('Ctrl Pts',(101.429090222574,1075.64218970965,397.471871556973));
#119045=CARTESIAN_POINT('Ctrl Pts',(101.429175789089,1075.64218105522,397.471871534959));
#119046=CARTESIAN_POINT('Ctrl Pts',(101.429261354593,1075.64217240143,397.471871534959));
#119047=CARTESIAN_POINT('',(101.429261354593,1082.7251047501,397.471871534959));
#119048=CARTESIAN_POINT('',(101.429261354593,1067.7251047501,397.471871534959));
#119049=CARTESIAN_POINT('Origin',(101.429261354593,1082.7251047501,397.970702670951));
#119050=CARTESIAN_POINT('Ctrl Pts',(101.429261354593,1075.64217240143,397.471871534959));
#119051=CARTESIAN_POINT('Ctrl Pts',(101.495421950748,1075.63548115745,397.471871534959));
#119052=CARTESIAN_POINT('Ctrl Pts',(101.560978599971,1075.62917816881,397.485034008547));
#119053=CARTESIAN_POINT('Ctrl Pts',(101.682419981123,1075.61818275567,397.535935948996));
#119054=CARTESIAN_POINT('Ctrl Pts',(101.737249774835,1075.61357707225,397.572869047254));
#119055=CARTESIAN_POINT('Ctrl Pts',(101.829287030385,1075.60666323584,397.665652088365));
#119056=CARTESIAN_POINT('Ctrl Pts',(101.865692713758,1075.60440995756,397.720473476261));
#119057=CARTESIAN_POINT('Ctrl Pts',(101.915264791931,1075.60257310897,397.840873822758));
#119058=CARTESIAN_POINT('Ctrl Pts',(101.928023384354,1075.60299801806,397.905210534623));
#119059=CARTESIAN_POINT('Ctrl Pts',(101.928161096421,1075.60647968227,398.035194002776));
#119060=CARTESIAN_POINT('Ctrl Pts',(101.915517978015,1075.60950367989,398.099548383412));
#119061=CARTESIAN_POINT('Ctrl Pts',(101.866221262996,1075.61776614351,398.220012152439));
#119062=CARTESIAN_POINT('Ctrl Pts',(101.829930797645,1075.62293418494,398.274900719215));
#119063=CARTESIAN_POINT('Ctrl Pts',(101.73814313638,1075.63473796658,398.367837084625));
#119064=CARTESIAN_POINT('Ctrl Pts',(101.683408510518,1075.64126910735,398.404894731071));
#119065=CARTESIAN_POINT('Ctrl Pts',(101.593043672638,1075.65140156573,398.443009268326));
#119066=CARTESIAN_POINT('Ctrl Pts',(101.561793158021,1075.65480771647,398.452712395339));
#119067=CARTESIAN_POINT('Ctrl Pts',(101.496660735388,1075.66171451687,398.466117623723));
#119068=CARTESIAN_POINT('Ctrl Pts',(101.46296676434,1075.66518826246,398.469533806944));
#119069=CARTESIAN_POINT('Ctrl Pts',(101.429261354593,1075.66856733728,398.469533806944));
#119070=CARTESIAN_POINT('Origin',(110.796881705952,1067.7251047501,408.357311548868));
#119071=CARTESIAN_POINT('',(110.79688170597,1076.79846644782,407.266770800141));
#119072=CARTESIAN_POINT('Ctrl Pts',(110.797596068878,1076.84090759235,409.447852063623));
#119073=CARTESIAN_POINT('Ctrl Pts',(110.940798490479,1076.82194611934,409.447758258304));
#119074=CARTESIAN_POINT('Ctrl Pts',(111.082602685119,1076.80252747935,409.419458867192));
#119075=CARTESIAN_POINT('Ctrl Pts',(111.347547647025,1076.76496011306,409.309506201558));
#119076=CARTESIAN_POINT('Ctrl Pts',(111.468196495587,1076.7471620535,409.228716494913));
#119077=CARTESIAN_POINT('Ctrl Pts',(111.663174628467,1076.71701008936,409.032843373741));
#119078=CARTESIAN_POINT('Ctrl Pts',(111.738859542695,1076.7045810305,408.922638121687));
#119079=CARTESIAN_POINT('Ctrl Pts',(111.850538649928,1076.68446048781,408.672117681504));
#119080=CARTESIAN_POINT('Ctrl Pts',(111.882517354936,1076.67733136566,408.532763321516));
#119081=CARTESIAN_POINT('Ctrl Pts',(111.887907789629,1076.67312014269,408.35848053537));
#119082=CARTESIAN_POINT('Ctrl Pts',(111.887456463124,1076.67253121684,408.325903660198));
#119083=CARTESIAN_POINT('Ctrl Pts',(111.884521713249,1076.6719325176,408.275919304519));
#119084=CARTESIAN_POINT('Ctrl Pts',(111.883075271443,1076.67178095054,408.258472999811));
#119085=CARTESIAN_POINT('Ctrl Pts',(111.879652867879,1076.67160909169,408.226548432727));
#119086=CARTESIAN_POINT('Ctrl Pts',(111.877804756182,1076.67157122571,408.212060906793));
#119087=CARTESIAN_POINT('Ctrl Pts',(111.873479467553,1076.67157620347,408.18284269891));
#119088=CARTESIAN_POINT('Ctrl Pts',(111.870989531762,1076.67162088662,408.168117223433));
#119089=CARTESIAN_POINT('Ctrl Pts',(111.864156962088,1076.67183338189,408.132211687618));
#119090=CARTESIAN_POINT('Ctrl Pts',(111.859485544345,1076.67204730599,408.111101412548));
#119091=CARTESIAN_POINT('Ctrl Pts',(111.840716041769,1076.6731171682,408.036821405501));
#119092=CARTESIAN_POINT('Ctrl Pts',(111.823230749441,1076.67445279373,407.984606899442));
#119093=CARTESIAN_POINT('Ctrl Pts',(111.745848355034,1076.68130575353,407.800912492653));
#119094=CARTESIAN_POINT('Ctrl Pts',(111.664032941405,1076.6900207055,407.680514225089));
#119095=CARTESIAN_POINT('Ctrl Pts',(111.47660366712,1076.7117353652,407.496275756476));
#119096=CARTESIAN_POINT('Ctrl Pts',(111.378919935215,1076.72357163678,407.427495958239));
#119097=CARTESIAN_POINT('Ctrl Pts',(111.155543420406,1076.75151197595,407.319304807177));
#119098=CARTESIAN_POINT('Ctrl Pts',(111.029813890956,1076.76769471878,407.284107570939));
#119099=CARTESIAN_POINT('Ctrl Pts',(110.761934560225,1076.80298809342,407.258414106273));
#119100=CARTESIAN_POINT('Ctrl Pts',(110.62160256584,1076.8219212525,407.271923152553));
#119101=CARTESIAN_POINT('Ctrl Pts',(110.348934538908,1076.8595917202,407.352549191111));
#119102=CARTESIAN_POINT('Ctrl Pts',(110.219603083,1076.87794711436,407.420804922885));
#119103=CARTESIAN_POINT('Ctrl Pts',(110.000530428149,1076.91013053916,407.599619671674));
#119104=CARTESIAN_POINT('Ctrl Pts',(109.911078128603,1076.92385613248,407.706355951291));
#119105=CARTESIAN_POINT('Ctrl Pts',(109.782567297638,1076.9450121476,407.937372447147));
#119106=CARTESIAN_POINT('Ctrl Pts',(109.740768013442,1076.95272737992,408.057510368056));
#119107=CARTESIAN_POINT('Ctrl Pts',(109.709490002801,1076.9604471158,408.249856803403));
#119108=CARTESIAN_POINT('Ctrl Pts',(109.704885749696,1076.96234661771,408.318346506131));
#119109=CARTESIAN_POINT('Ctrl Pts',(109.707401418855,1076.96378737287,408.411231851096));
#119110=CARTESIAN_POINT('Ctrl Pts',(109.708880866583,1076.96405911113,408.435599411419));
#119111=CARTESIAN_POINT('Ctrl Pts',(109.712631138036,1076.96432803011,408.475289733741));
#119112=CARTESIAN_POINT('Ctrl Pts',(109.714412642405,1076.96438930685,408.490649034774));
#119113=CARTESIAN_POINT('Ctrl Pts',(109.718468114861,1076.96442438148,408.520122708937));
#119114=CARTESIAN_POINT('Ctrl Pts',(109.720694191577,1076.96440444519,408.534240291552));
#119115=CARTESIAN_POINT('Ctrl Pts',(109.72646223583,1076.96427375415,408.566664952867));
#119116=CARTESIAN_POINT('Ctrl Pts',(109.730197472961,1076.96413721157,408.584932737935));
#119117=CARTESIAN_POINT('Ctrl Pts',(109.743198805031,1076.9635215027,408.641135341062));
#119118=CARTESIAN_POINT('Ctrl Pts',(109.75403409151,1076.96283139683,408.678670724879));
#119119=CARTESIAN_POINT('Ctrl Pts',(109.814372691947,1076.95831109599,408.852164245958));
#119120=CARTESIAN_POINT('Ctrl Pts',(109.888540162546,1076.95108732914,408.977816204453));
#119121=CARTESIAN_POINT('Ctrl Pts',(110.062727173184,1076.93213260548,409.172108767722));
#119122=CARTESIAN_POINT('Ctrl Pts',(110.153883205898,1076.92165881263,409.245769799526));
#119123=CARTESIAN_POINT('Ctrl Pts',(110.341538697821,1076.89917000054,409.353270798214));
#119124=CARTESIAN_POINT('Ctrl Pts',(110.434606194538,1076.88768352365,409.390746166895));
#119125=CARTESIAN_POINT('Ctrl Pts',(110.618468559949,1076.86437474434,409.43690112176));
#119126=CARTESIAN_POINT('Ctrl Pts',(110.707891313523,1076.85278542428,409.447910825082));
#119127=CARTESIAN_POINT('Ctrl Pts',(110.797596068878,1076.84090759235,409.447852063623));
#119128=CARTESIAN_POINT('',(110.796881705933,1074.78002293647,407.26677080014));
#119129=CARTESIAN_POINT('',(110.796881705952,1067.7251047501,407.26677080014));
#119130=CARTESIAN_POINT('Ctrl Pts',(110.797104296965,1074.82288111126,409.44785227488));
#119131=CARTESIAN_POINT('Ctrl Pts',(110.652438844663,1074.84219373867,409.447881802644));
#119132=CARTESIAN_POINT('Ctrl Pts',(110.509041163128,1074.86067712467,409.41912529087));
#119133=CARTESIAN_POINT('Ctrl Pts',(110.242179317219,1074.89380419229,409.307272717847));
#119134=CARTESIAN_POINT('Ctrl Pts',(110.121210562518,1074.90814599874,409.225486400346));
#119135=CARTESIAN_POINT('Ctrl Pts',(109.918968855179,1074.93074023296,409.019984542716));
#119136=CARTESIAN_POINT('Ctrl Pts',(109.83936521802,1074.93882396886,408.898726784053));
#119137=CARTESIAN_POINT('Ctrl Pts',(109.732560159946,1074.9477078735,408.63399921831));
#119138=CARTESIAN_POINT('Ctrl Pts',(109.705652335196,1074.94852919444,408.49356864231));
#119139=CARTESIAN_POINT('Ctrl Pts',(109.707057740186,1074.94290529174,408.209967554164));
#119140=CARTESIAN_POINT('Ctrl Pts',(109.735462484341,1074.93650257059,408.069675734858));
#119141=CARTESIAN_POINT('Ctrl Pts',(109.84542065414,1074.91699009266,407.805042530233));
#119142=CARTESIAN_POINT('Ctrl Pts',(109.927041106778,1074.90392926951,407.683873081696));
#119143=CARTESIAN_POINT('Ctrl Pts',(110.132663885017,1074.87283895158,407.480336697443));
#119144=CARTESIAN_POINT('Ctrl Pts',(110.254768731147,1074.85509826984,407.400089688862));
#119145=CARTESIAN_POINT('Ctrl Pts',(110.454534828223,1074.82691355067,407.319473955404));
#119146=CARTESIAN_POINT('Ctrl Pts',(110.522711679009,1074.81741858841,407.29942049743));
#119147=CARTESIAN_POINT('Ctrl Pts',(110.662207018169,1074.79822716727,407.27278280803));
#119148=CARTESIAN_POINT('Ctrl Pts',(110.733225327124,1074.78857285774,407.266307963273));
#119149=CARTESIAN_POINT('Ctrl Pts',(110.950836314104,1074.75934327395,407.267802286347));
#119150=CARTESIAN_POINT('Ctrl Pts',(111.095764470464,1074.74036228006,407.298306539936));
#119151=CARTESIAN_POINT('Ctrl Pts',(111.36201243672,1074.70654289296,407.413666149387));
#119152=CARTESIAN_POINT('Ctrl Pts',(111.481279983993,1074.69194134382,407.496162584562));
#119153=CARTESIAN_POINT('Ctrl Pts',(111.680159312817,1074.66891163819,407.702046636736));
#119154=CARTESIAN_POINT('Ctrl Pts',(111.758204460931,1074.66065081163,407.822974454505));
#119155=CARTESIAN_POINT('Ctrl Pts',(111.862928670743,1074.65161706806,408.087354033574));
#119156=CARTESIAN_POINT('Ctrl Pts',(111.88894651253,1074.65087800413,408.227935717224));
#119157=CARTESIAN_POINT('Ctrl Pts',(111.885761555839,1074.65701288816,408.51111919239));
#119158=CARTESIAN_POINT('Ctrl Pts',(111.856631937355,1074.66381808078,408.650835991852));
#119159=CARTESIAN_POINT('Ctrl Pts',(111.746500202022,1074.68411125413,408.912052886199));
#119160=CARTESIAN_POINT('Ctrl Pts',(111.666228687497,1074.69744235606,409.030820038809));
#119161=CARTESIAN_POINT('Ctrl Pts',(111.464078426709,1074.72891417179,409.231754012385));
#119162=CARTESIAN_POINT('Ctrl Pts',(111.343705581201,1074.74680083847,409.311608728508));
#119163=CARTESIAN_POINT('Ctrl Pts',(111.14622773306,1074.77501547182,409.392793530291));
#119164=CARTESIAN_POINT('Ctrl Pts',(111.078476928241,1074.78452761695,409.413230826971));
#119165=CARTESIAN_POINT('Ctrl Pts',(110.939390232132,1074.80372666124,409.440843814289));
#119166=CARTESIAN_POINT('Ctrl Pts',(110.86833802526,1074.81337151217,409.447837735315));
#119167=CARTESIAN_POINT('Ctrl Pts',(110.797104296965,1074.82288111126,409.44785227488));
#119168=CARTESIAN_POINT('Origin',(110.796881705952,1067.7251047501,408.357311548868));
#119169=CARTESIAN_POINT('',(110.796881705952,1074.81171529132,408.847852297596));
#119170=CARTESIAN_POINT('',(110.796881705952,1074.79242545665,407.86677080014));
#119171=CARTESIAN_POINT('Ctrl Pts',(110.796881705952,1074.81171529132,408.847852297596));
#119172=CARTESIAN_POINT('Ctrl Pts',(110.732230902365,1074.82036176743,408.847852297596));
#119173=CARTESIAN_POINT('Ctrl Pts',(110.668137201305,1074.82866376,408.835071239047));
#119174=CARTESIAN_POINT('Ctrl Pts',(110.548079367316,1074.84367802719,408.785079045369));
#119175=CARTESIAN_POINT('Ctrl Pts',(110.493348101575,1074.85023254509,408.748186842145));
#119176=CARTESIAN_POINT('Ctrl Pts',(110.402117569826,1074.86054008216,408.655567616644));
#119177=CARTESIAN_POINT('Ctrl Pts',(110.366286408721,1074.8642284773,408.601041247894));
#119178=CARTESIAN_POINT('Ctrl Pts',(110.318190424013,1074.86828640209,408.481983554045));
#119179=CARTESIAN_POINT('Ctrl Pts',(110.306058615111,1074.86866517485,408.418821584829));
#119180=CARTESIAN_POINT('Ctrl Pts',(110.306633608904,1074.86610898353,408.291303235435));
#119181=CARTESIAN_POINT('Ctrl Pts',(110.319362355406,1074.8631961676,408.228242712091));
#119182=CARTESIAN_POINT('Ctrl Pts',(110.368313422293,1074.85440131949,408.110180529535));
#119183=CARTESIAN_POINT('Ctrl Pts',(110.404219439568,1074.84858498955,408.056422718336));
#119184=CARTESIAN_POINT('Ctrl Pts',(110.495510813699,1074.83464611687,407.964773307526));
#119185=CARTESIAN_POINT('Ctrl Pts',(110.550425655568,1074.82661064083,407.928187191488));
#119186=CARTESIAN_POINT('Ctrl Pts',(110.640080283218,1074.81391187333,407.891430867615));
#119187=CARTESIAN_POINT('Ctrl Pts',(110.670443074312,1074.80967184199,407.882291851998));
#119188=CARTESIAN_POINT('Ctrl Pts',(110.73280598265,1074.801079668,407.869925255115));
#119189=CARTESIAN_POINT('Ctrl Pts',(110.764681141398,1074.79674591179,407.866786851268));
#119190=CARTESIAN_POINT('Ctrl Pts',(110.796636258659,1074.792458388,407.866770861555));
#119191=CARTESIAN_POINT('Ctrl Pts',(110.796718075338,1074.79244741039,407.866770820616));
#119192=CARTESIAN_POINT('Ctrl Pts',(110.796799891105,1074.79243643327,407.86677080014));
#119193=CARTESIAN_POINT('Ctrl Pts',(110.796881705952,1074.79242545665,407.86677080014));
#119194=CARTESIAN_POINT('',(110.796881705952,1082.7251047501,407.86677080014));
#119195=CARTESIAN_POINT('',(110.796881705952,1067.7251047501,407.86677080014));
#119196=CARTESIAN_POINT('Origin',(110.796881705952,1082.7251047501,408.357311548868));
#119197=CARTESIAN_POINT('Ctrl Pts',(110.796881705952,1074.79242545665,407.86677080014));
#119198=CARTESIAN_POINT('Ctrl Pts',(110.862448424036,1074.78362875217,407.86677080014));
#119199=CARTESIAN_POINT('Ctrl Pts',(110.927424711471,1074.77515064853,407.87991650284));
#119200=CARTESIAN_POINT('Ctrl Pts',(111.047742741636,1074.75994924986,407.930797048961));
#119201=CARTESIAN_POINT('Ctrl Pts',(111.102033244182,1074.75335292131,407.967751717849));
#119202=CARTESIAN_POINT('Ctrl Pts',(111.192335164697,1074.7429825256,408.060085497495));
#119203=CARTESIAN_POINT('Ctrl Pts',(111.227759642654,1074.73926380156,408.114222684894));
#119204=CARTESIAN_POINT('Ctrl Pts',(111.27561552072,1074.73514222284,408.232803372901));
#119205=CARTESIAN_POINT('Ctrl Pts',(111.287725651519,1074.73475766369,408.295968305641));
#119206=CARTESIAN_POINT('Ctrl Pts',(111.287107750214,1074.7373736331,408.423406605835));
#119207=CARTESIAN_POINT('Ctrl Pts',(111.274389220315,1074.74034695761,408.486382547684));
#119208=CARTESIAN_POINT('Ctrl Pts',(111.225528705733,1074.74929199442,408.60427926035));
#119209=CARTESIAN_POINT('Ctrl Pts',(111.189707559974,1074.75519534922,408.6579641971));
#119210=CARTESIAN_POINT('Ctrl Pts',(111.099232079229,1074.76919354963,408.748938714261));
#119211=CARTESIAN_POINT('Ctrl Pts',(111.045258313269,1074.77717531092,408.785184830353));
#119212=CARTESIAN_POINT('Ctrl Pts',(110.956297730916,1074.78985619173,408.822334846439));
#119213=CARTESIAN_POINT('Ctrl Pts',(110.925549031485,1074.79416760951,408.83176266743));
#119214=CARTESIAN_POINT('Ctrl Pts',(110.862723959561,1074.80283806631,408.844466863021));
#119215=CARTESIAN_POINT('Ctrl Pts',(110.830790115671,1074.80717767322,408.84772577844));
#119216=CARTESIAN_POINT('Ctrl Pts',(110.798136690445,1074.81154742282,408.847851093668));
#119217=CARTESIAN_POINT('Ctrl Pts',(110.797509171956,1074.81163137327,408.847852297596));
#119218=CARTESIAN_POINT('Ctrl Pts',(110.796881705952,1074.81171529132,408.847852297596));
#119219=CARTESIAN_POINT('Origin',(69.1578093449752,1067.7251047501,367.717925093334));
#119220=CARTESIAN_POINT('',(69.1578093449994,1078.64674583663,366.23962196114));
#119221=CARTESIAN_POINT('',(69.1578093449753,1078.69514019783,369.196228225527));
#119222=CARTESIAN_POINT('Ctrl Pts',(69.1578093449994,1078.64674583663,366.23962196114));
#119223=CARTESIAN_POINT('Ctrl Pts',(69.0296449594974,1078.64978215304,366.239621961138));
#119224=CARTESIAN_POINT('Ctrl Pts',(68.9020372739768,1078.65305477435,366.256287402465));
#119225=CARTESIAN_POINT('Ctrl Pts',(68.6682202561937,1078.65943950329,366.318415431848));
#119226=CARTESIAN_POINT('Ctrl Pts',(68.5620016043582,1078.66250668231,366.360229385106));
#119227=CARTESIAN_POINT('Ctrl Pts',(68.2929599044742,1078.67068017121,366.503851637143));
#119228=CARTESIAN_POINT('Ctrl Pts',(68.1433397887672,1078.67566912136,366.62577319367));
#119229=CARTESIAN_POINT('Ctrl Pts',(67.9073232828472,1078.68448653439,366.909636845607));
#119230=CARTESIAN_POINT('Ctrl Pts',(67.8191858166255,1078.68830218495,367.065897950557));
#119231=CARTESIAN_POINT('Ctrl Pts',(67.70719855906,1078.69461389355,367.389196055409));
#119232=CARTESIAN_POINT('Ctrl Pts',(67.6796760452616,1078.69714927108,367.552210845489));
#119233=CARTESIAN_POINT('Ctrl Pts',(67.6793262989304,1078.70137772082,367.891909047171));
#119234=CARTESIAN_POINT('Ctrl Pts',(67.7104015479753,1078.70297179684,368.066058318319));
#119235=CARTESIAN_POINT('Ctrl Pts',(67.8049247097742,1078.70459182585,368.321657185957));
#119236=CARTESIAN_POINT('Ctrl Pts',(67.8474429188161,1078.70499568347,368.409104794057));
#119237=CARTESIAN_POINT('Ctrl Pts',(67.9185829621773,1078.70532619632,368.52490184275));
#119238=CARTESIAN_POINT('Ctrl Pts',(67.9402469233516,1078.70539357062,368.557231508571));
#119239=CARTESIAN_POINT('Ctrl Pts',(67.9784442733099,1078.70546072103,368.609637745062));
#119240=CARTESIAN_POINT('Ctrl Pts',(67.9942772144347,1078.70547551981,368.630200494422));
#119241=CARTESIAN_POINT('Ctrl Pts',(68.0263437354676,1078.70548089504,368.669652666604));
#119242=CARTESIAN_POINT('Ctrl Pts',(68.0425297450801,1078.70547243057,368.688569834165));
#119243=CARTESIAN_POINT('Ctrl Pts',(68.0817827631551,1078.70542631421,368.732167417706));
#119244=CARTESIAN_POINT('Ctrl Pts',(68.1052332637385,1078.70537934681,368.756483847911));
#119245=CARTESIAN_POINT('Ctrl Pts',(68.183526721153,1078.70516165467,368.832290230457));
#119246=CARTESIAN_POINT('Ctrl Pts',(68.24147084426,1078.70491031437,368.880405174778));
#119247=CARTESIAN_POINT('Ctrl Pts',(68.463348284611,1078.70362891227,369.037706880796));
#119248=CARTESIAN_POINT('Ctrl Pts',(68.6449874630025,1078.7020157938,369.118321248062));
#119249=CARTESIAN_POINT('Ctrl Pts',(68.9423791004867,1078.69836935129,369.18442071346));
#119250=CARTESIAN_POINT('Ctrl Pts',(69.049929047363,1078.69686402144,369.196228225527));
#119251=CARTESIAN_POINT('Ctrl Pts',(69.1578093449753,1078.69514019783,369.196228225527));
#119252=CARTESIAN_POINT('',(69.1578093449571,1076.64572521568,366.239621961141));
#119253=CARTESIAN_POINT('',(69.1578093449752,1067.7251047501,366.23962196114));
#119254=CARTESIAN_POINT('',(69.1578093449752,1076.6946925711,369.196228225527));
#119255=CARTESIAN_POINT('Ctrl Pts',(69.1578093449752,1076.6946925711,369.196228225527));
#119256=CARTESIAN_POINT('Ctrl Pts',(69.1129243695232,1076.69541844176,369.196228225527));
#119257=CARTESIAN_POINT('Ctrl Pts',(69.0683825043262,1076.6961017847,369.19418827694));
#119258=CARTESIAN_POINT('Ctrl Pts',(69.0241795694995,1076.69674557598,369.190176170344));
#119259=CARTESIAN_POINT('Ctrl Pts',(68.9795394951775,1076.69739573396,369.186124386513));
#119260=CARTESIAN_POINT('Ctrl Pts',(68.9352441571163,1076.69800555415,369.18006124436));
#119261=CARTESIAN_POINT('Ctrl Pts',(68.8912860273357,1076.69857810177,369.172004001718));
#119262=CARTESIAN_POINT('Ctrl Pts',(68.8840484801668,1076.69867236966,369.170677405842));
#119263=CARTESIAN_POINT('Ctrl Pts',(68.8768200852097,1076.69876562716,369.169296638954));
#119264=CARTESIAN_POINT('Ctrl Pts',(68.8696008277746,1076.69885788794,369.167861644106));
#119265=CARTESIAN_POINT('Ctrl Pts',(68.8314853405077,1076.69934499682,369.160285307016));
#119266=CARTESIAN_POINT('Ctrl Pts',(68.793459694709,1076.69980569616,369.151160086375));
#119267=CARTESIAN_POINT('Ctrl Pts',(68.7557810565234,1076.70023844489,369.140511964473));
#119268=CARTESIAN_POINT('Ctrl Pts',(68.7181385859787,1076.70067077823,369.129874063679));
#119269=CARTESIAN_POINT('Ctrl Pts',(68.6808430566933,1076.7010752146,369.117716304634));
#119270=CARTESIAN_POINT('Ctrl Pts',(68.6441396458052,1076.70145021738,369.104115408841));
#119271=CARTESIAN_POINT('Ctrl Pts',(68.6265107180164,1076.70163033407,369.097582795006));
#119272=CARTESIAN_POINT('Ctrl Pts',(68.6090181661426,1076.70180366057,369.090717997316));
#119273=CARTESIAN_POINT('Ctrl Pts',(68.5916876243133,1076.70197002661,369.083533510138));
#119274=CARTESIAN_POINT('Ctrl Pts',(68.5499591554298,1076.70237060267,369.066234705946));
#119275=CARTESIAN_POINT('Ctrl Pts',(68.5092372895722,1076.70273123869,369.04711656848));
#119276=CARTESIAN_POINT('Ctrl Pts',(68.4695057440446,1076.7030537665,369.026213403913));
#119277=CARTESIAN_POINT('Ctrl Pts',(68.4296799567572,1076.70337705933,369.005260657811));
#119278=CARTESIAN_POINT('Ctrl Pts',(68.3908483463713,1076.70366206297,368.982513983927));
#119279=CARTESIAN_POINT('Ctrl Pts',(68.3530166957146,1076.7039106223,368.957960956665));
#119280=CARTESIAN_POINT('Ctrl Pts',(68.347613722873,1076.7039461206,368.954454386448));
#119281=CARTESIAN_POINT('Ctrl Pts',(68.3422311949065,1076.70398087557,368.950910901442));
#119282=CARTESIAN_POINT('Ctrl Pts',(68.336869180964,1076.70401489258,368.947330395814));
#119283=CARTESIAN_POINT('Ctrl Pts',(68.3067288594723,1076.70420610496,368.927204079115));
#119284=CARTESIAN_POINT('Ctrl Pts',(68.277172490896,1076.70437365221,368.905859877632));
#119285=CARTESIAN_POINT('Ctrl Pts',(68.2484182459181,1076.70451718386,368.883424119334));
#119286=CARTESIAN_POINT('Ctrl Pts',(68.2196569893529,1076.7046607505,368.860982890183));
#119287=CARTESIAN_POINT('Ctrl Pts',(68.1916987292402,1076.70478028982,368.837449911598));
#119288=CARTESIAN_POINT('Ctrl Pts',(68.1647306760372,1076.70487545108,368.812993542314));
#119289=CARTESIAN_POINT('Ctrl Pts',(68.1467730472035,1076.70493881757,368.796708406754));
#119290=CARTESIAN_POINT('Ctrl Pts',(68.1292538177756,1076.70499137475,368.780014703662));
#119291=CARTESIAN_POINT('Ctrl Pts',(68.1122191473878,1076.70503301906,368.762971163783));
#119292=CARTESIAN_POINT('Ctrl Pts',(68.0771355036054,1076.70511878734,368.727869252899));
#119293=CARTESIAN_POINT('Ctrl Pts',(68.0437396734568,1076.70515964597,368.690914637454));
#119294=CARTESIAN_POINT('Ctrl Pts',(68.0122641653214,1076.70515559111,368.652326715777));
#119295=CARTESIAN_POINT('Ctrl Pts',(67.9808067613756,1076.70515153857,368.613760989232));
#119296=CARTESIAN_POINT('Ctrl Pts',(67.9512678913311,1076.7051026242,368.573564288066));
#119297=CARTESIAN_POINT('Ctrl Pts',(67.9238413581347,1076.70500884412,368.531990912605));
#119298=CARTESIAN_POINT('Ctrl Pts',(67.8963940645984,1076.70491499307,368.490386068442));
#119299=CARTESIAN_POINT('Ctrl Pts',(67.8710626435722,1076.70477620837,368.447402985898));
#119300=CARTESIAN_POINT('Ctrl Pts',(67.8479972570152,1076.70459248618,368.403324571658));
#119301=CARTESIAN_POINT('Ctrl Pts',(67.8275232175205,1076.70442940478,368.364198273393));
#119302=CARTESIAN_POINT('Ctrl Pts',(67.8088341266088,1076.70423091595,368.324209594824));
#119303=CARTESIAN_POINT('Ctrl Pts',(67.7920032094858,1076.70399701699,368.283569638001));
#119304=CARTESIAN_POINT('Ctrl Pts',(67.7731266905889,1076.70373469034,368.237990368177));
#119305=CARTESIAN_POINT('Ctrl Pts',(67.756482261278,1076.70342600895,368.191335359111));
#119306=CARTESIAN_POINT('Ctrl Pts',(67.7422060389957,1076.70307117226,368.143891560033));
#119307=CARTESIAN_POINT('Ctrl Pts',(67.727940201487,1076.70271659368,368.096482272405));
#119308=CARTESIAN_POINT('Ctrl Pts',(67.7160393578063,1076.70231592693,368.048285916623));
#119309=CARTESIAN_POINT('Ctrl Pts',(67.7065909166684,1076.70186937099,367.999607936253));
#119310=CARTESIAN_POINT('Ctrl Pts',(67.6971373622955,1076.70142257339,367.950903612707));
#119311=CARTESIAN_POINT('Ctrl Pts',(67.690138992944,1076.70092983692,367.901717751667));
#119312=CARTESIAN_POINT('Ctrl Pts',(67.6856321660866,1076.70039136092,367.852366547552));
#119313=CARTESIAN_POINT('Ctrl Pts',(67.6815524693982,1076.69990391845,367.807692556212));
#119314=CARTESIAN_POINT('Ctrl Pts',(67.6795137893469,1076.69937899545,367.762883532693));
#119315=CARTESIAN_POINT('Ctrl Pts',(67.6795062338911,1076.69881673977,367.71817491663));
#119316=CARTESIAN_POINT('Ctrl Pts',(67.6795000833663,1076.69835903508,367.681779832221));
#119317=CARTESIAN_POINT('Ctrl Pts',(67.6808422638254,1076.69787293693,367.6451681948));
#119318=CARTESIAN_POINT('Ctrl Pts',(67.6835548113673,1076.69736076001,367.608592020619));
#119319=CARTESIAN_POINT('Ctrl Pts',(67.6862660494103,1076.69684883035,367.57203350381));
#119320=CARTESIAN_POINT('Ctrl Pts',(67.6903463283445,1076.69631084708,367.535511006626));
#119321=CARTESIAN_POINT('Ctrl Pts',(67.6957655489489,1076.69574912154,367.499274483562));
#119322=CARTESIAN_POINT('Ctrl Pts',(67.6992897940453,1076.69538381837,367.475709030512));
#119323=CARTESIAN_POINT('Ctrl Pts',(67.7033792317309,1076.69500847411,367.452264464278));
#119324=CARTESIAN_POINT('Ctrl Pts',(67.708013947672,1076.69462372445,367.429007360041));
#119325=CARTESIAN_POINT('Ctrl Pts',(67.7168391423511,1076.69389110337,367.384722343402));
#119326=CARTESIAN_POINT('Ctrl Pts',(67.7276535011892,1076.69312395991,367.341019701624));
#119327=CARTESIAN_POINT('Ctrl Pts',(67.7404339194266,1076.69232010618,367.297892887779));
#119328=CARTESIAN_POINT('Ctrl Pts',(67.7531999187991,1076.69151715936,367.254814729595));
#119329=CARTESIAN_POINT('Ctrl Pts',(67.7679278213293,1076.69067758506,367.212310198549));
#119330=CARTESIAN_POINT('Ctrl Pts',(67.7846440120623,1076.68979920278,367.170387771191));
#119331=CARTESIAN_POINT('Ctrl Pts',(67.7870168346456,1076.68967451856,367.164436984677));
#119332=CARTESIAN_POINT('Ctrl Pts',(67.789429796553,1076.68954905239,367.15849796482));
#119333=CARTESIAN_POINT('Ctrl Pts',(67.7918830485335,1076.68942279803,367.152570776695));
#119334=CARTESIAN_POINT('Ctrl Pts',(67.8065254954997,1076.68866923799,367.117193840911));
#119335=CARTESIAN_POINT('Ctrl Pts',(67.8225977706757,1076.68788737807,367.082263123204));
#119336=CARTESIAN_POINT('Ctrl Pts',(67.8400072677222,1076.68708182782,367.048016266821));
#119337=CARTESIAN_POINT('Ctrl Pts',(67.8574319591611,1076.68627557453,367.013739520994));
#119338=CARTESIAN_POINT('Ctrl Pts',(67.8761959365134,1076.68544558954,366.980148374759));
#119339=CARTESIAN_POINT('Ctrl Pts',(67.8961598287834,1076.68459649448,366.947457281582));
#119340=CARTESIAN_POINT('Ctrl Pts',(67.9067045072196,1076.68414801309,366.930190254661));
#119341=CARTESIAN_POINT('Ctrl Pts',(67.9175831835706,1076.68369420032,366.913173875774));
#119342=CARTESIAN_POINT('Ctrl Pts',(67.9287705538774,1076.68323573722,366.896436322486));
#119343=CARTESIAN_POINT('Ctrl Pts',(67.9536480055309,1076.68221624886,366.859216881161));
#119344=CARTESIAN_POINT('Ctrl Pts',(67.9801739456007,1076.68116933278,366.823182839392));
#119345=CARTESIAN_POINT('Ctrl Pts',(68.008356743339,1076.68009372025,366.788334394561));
#119346=CARTESIAN_POINT('Ctrl Pts',(68.0362961581857,1076.67902739656,366.753786896263));
#119347=CARTESIAN_POINT('Ctrl Pts',(68.0658645682457,1076.67793286991,366.720403941188));
#119348=CARTESIAN_POINT('Ctrl Pts',(68.0971058920654,1076.67680890415,366.688222060592));
#119349=CARTESIAN_POINT('Ctrl Pts',(68.1021604648095,1076.67662705633,366.683015313994));
#119350=CARTESIAN_POINT('Ctrl Pts',(68.1072588930011,1076.67644443789,366.677840097268));
#119351=CARTESIAN_POINT('Ctrl Pts',(68.1124014336536,1076.67626104361,366.672696673514));
#119352=CARTESIAN_POINT('Ctrl Pts',(68.1616662374676,1076.67450415265,366.623423409718));
#119353=CARTESIAN_POINT('Ctrl Pts',(68.2141095020647,1076.67270591134,366.577933034726));
#119354=CARTESIAN_POINT('Ctrl Pts',(68.2693151663366,1076.67088010323,366.53641832434));
#119355=CARTESIAN_POINT('Ctrl Pts',(68.3272964798804,1076.66896249652,366.492816323145));
#119356=CARTESIAN_POINT('Ctrl Pts',(68.3883266438417,1076.66701448131,366.45359774211));
#119357=CARTESIAN_POINT('Ctrl Pts',(68.451973582526,1076.66505202649,366.41901169087));
#119358=CARTESIAN_POINT('Ctrl Pts',(68.497452943878,1076.66364974079,366.394297988144));
#119359=CARTESIAN_POINT('Ctrl Pts',(68.5442696367321,1076.66224008235,366.371950199882));
#119360=CARTESIAN_POINT('Ctrl Pts',(68.5922717248266,1076.66082887737,366.352074680276));
#119361=CARTESIAN_POINT('Ctrl Pts',(68.6339957019783,1076.65960224147,366.334798645861));
#119362=CARTESIAN_POINT('Ctrl Pts',(68.67628421805,1076.65838450843,366.319523819645));
#119363=CARTESIAN_POINT('Ctrl Pts',(68.7191235128161,1076.65717723202,366.306211633982));
#119364=CARTESIAN_POINT('Ctrl Pts',(68.7620966106071,1076.65596618483,366.29285786942));
#119365=CARTESIAN_POINT('Ctrl Pts',(68.805624828294,1076.6547656597,366.281478718402));
#119366=CARTESIAN_POINT('Ctrl Pts',(68.8497123649171,1076.65357722502,366.2720840227));
#119367=CARTESIAN_POINT('Ctrl Pts',(68.8560243419479,1076.65340707778,366.2707389917));
#119368=CARTESIAN_POINT('Ctrl Pts',(68.8623478003799,1076.65323717837,366.269434722546));
#119369=CARTESIAN_POINT('Ctrl Pts',(68.868682765832,1076.65306753139,366.268171330833));
#119370=CARTESIAN_POINT('Ctrl Pts',(68.9040718768512,1076.65211982992,366.261113627054));
#119371=CARTESIAN_POINT('Ctrl Pts',(68.9399147782392,1076.65117790773,366.255317170565));
#119372=CARTESIAN_POINT('Ctrl Pts',(68.9759683148074,1076.65024912806,366.250848411493));
#119373=CARTESIAN_POINT('Ctrl Pts',(69.0120253008042,1076.64932025953,366.246379224872));
#119374=CARTESIAN_POINT('Ctrl Pts',(69.0482923836453,1076.64840453604,366.243238093264));
#119375=CARTESIAN_POINT('Ctrl Pts',(69.0845184620344,1076.64750932295,366.241439875958));
#119376=CARTESIAN_POINT('Ctrl Pts',(69.1089934386633,1076.64690450123,366.240224968672));
#119377=CARTESIAN_POINT('Ctrl Pts',(69.1334495417676,1076.64630904166,366.239621961141));
#119378=CARTESIAN_POINT('Ctrl Pts',(69.1578093449571,1076.64572521568,366.23962196114));
#119379=CARTESIAN_POINT('Ctrl Pts',(69.1578093449571,1076.64572521568,366.23962196114));
#119380=CARTESIAN_POINT('Ctrl Pts',(69.352931273687,1076.64104877185,366.239621961138));
#119381=CARTESIAN_POINT('Ctrl Pts',(69.5461424200158,1076.63700733176,366.278250654702));
#119382=CARTESIAN_POINT('Ctrl Pts',(69.904617273348,1076.63102126722,366.427584991751));
#119383=CARTESIAN_POINT('Ctrl Pts',(70.0666751927357,1076.62911941045,366.536116840485));
#119384=CARTESIAN_POINT('Ctrl Pts',(70.3402320110238,1076.62785827307,366.809749322705));
#119385=CARTESIAN_POINT('Ctrl Pts',(70.4489338813008,1076.62851936261,366.972337429951));
#119386=CARTESIAN_POINT('Ctrl Pts',(70.5976113015266,1076.63229212897,367.330569118657));
#119387=CARTESIAN_POINT('Ctrl Pts',(70.635978789656,1076.63536880311,367.522789870244));
#119388=CARTESIAN_POINT('Ctrl Pts',(70.6362446921766,1076.64325078239,367.909901156615));
#119389=CARTESIAN_POINT('Ctrl Pts',(70.5985838608918,1076.64796333925,368.101050258007));
#119390=CARTESIAN_POINT('Ctrl Pts',(70.4518734837467,1076.65810199654,368.458266969645));
#119391=CARTESIAN_POINT('Ctrl Pts',(70.3441445489206,1076.66342525502,368.62087363203));
#119392=CARTESIAN_POINT('Ctrl Pts',(70.1402224447557,1076.67118325305,368.826787579702));
#119393=CARTESIAN_POINT('Ctrl Pts',(70.0656838951687,1076.67371436516,368.888598425619));
#119394=CARTESIAN_POINT('Ctrl Pts',(69.8595005831698,1076.67999687825,369.027960622456));
#119395=CARTESIAN_POINT('Ctrl Pts',(69.7209274126418,1076.68357129267,369.093230903822));
#119396=CARTESIAN_POINT('Ctrl Pts',(69.4394106335367,1076.68976760015,369.176008313024));
#119397=CARTESIAN_POINT('Ctrl Pts',(69.2989808746828,1076.69240957396,369.196228225527));
#119398=CARTESIAN_POINT('Ctrl Pts',(69.1578093449752,1076.6946925711,369.196228225527));
#119399=CARTESIAN_POINT('Ctrl Pts',(69.1578093449753,1078.69514019783,369.196228225527));
#119400=CARTESIAN_POINT('Ctrl Pts',(69.2026895040078,1078.69442305597,369.196228225527));
#119401=CARTESIAN_POINT('Ctrl Pts',(69.2472253980492,1078.69367481439,369.194188714804));
#119402=CARTESIAN_POINT('Ctrl Pts',(69.2914212403612,1078.69289411521,369.190177793132));
#119403=CARTESIAN_POINT('Ctrl Pts',(69.336057578074,1078.69210563488,369.186126895018));
#119404=CARTESIAN_POINT('Ctrl Pts',(69.380347982333,1078.69128404672,369.180065092482));
#119405=CARTESIAN_POINT('Ctrl Pts',(69.4243000771816,1078.69042795185,369.172009974041));
#119406=CARTESIAN_POINT('Ctrl Pts',(69.4315466965742,1078.69028680286,369.170681883134));
#119407=CARTESIAN_POINT('Ctrl Pts',(69.4387841084827,1078.69014471585,369.169299491733));
#119408=CARTESIAN_POINT('Ctrl Pts',(69.4460123282472,1078.69000168453,369.167862744092));
#119409=CARTESIAN_POINT('Ctrl Pts',(69.4841481969199,1078.68924705566,369.160282507028));
#119410=CARTESIAN_POINT('Ctrl Pts',(69.5221930517588,1078.68846212262,369.151151951091));
#119411=CARTESIAN_POINT('Ctrl Pts',(69.5598897116961,1078.68765110172,369.140497245933));
#119412=CARTESIAN_POINT('Ctrl Pts',(69.5975507316531,1078.68684084759,369.129852614174));
#119413=CARTESIAN_POINT('Ctrl Pts',(69.6348636152083,1078.68600455491,369.117686835009));
#119414=CARTESIAN_POINT('Ctrl Pts',(69.6715831858082,1078.68514642804,369.104076813431));
#119415=CARTESIAN_POINT('Ctrl Pts',(69.6891632639869,1078.68473558616,369.097560799233));
#119416=CARTESIAN_POINT('Ctrl Pts',(69.7066075675586,1078.68431973951,369.090714478063));
#119417=CARTESIAN_POINT('Ctrl Pts',(69.7238907087858,1078.6838993495,369.083550239631));
#119418=CARTESIAN_POINT('Ctrl Pts',(69.7656195477865,1078.68288434957,369.066252727092));
#119419=CARTESIAN_POINT('Ctrl Pts',(69.8063408444482,1078.68184536983,369.047136277935));
#119420=CARTESIAN_POINT('Ctrl Pts',(69.8460709945219,1078.680781756,369.026235474098));
#119421=CARTESIAN_POINT('Ctrl Pts',(69.8858984397647,1078.67971553749,369.00528348628));
#119422=CARTESIAN_POINT('Ctrl Pts',(69.9247307253615,1078.67862456408,368.982537971681));
#119423=CARTESIAN_POINT('Ctrl Pts',(69.9625622349569,1078.67750817665,368.957986759832));
#119424=CARTESIAN_POINT('Ctrl Pts',(69.9679489099638,1078.67734921878,368.954491012486));
#119425=CARTESIAN_POINT('Ctrl Pts',(69.9733152466221,1078.67718974567,368.950958585688));
#119426=CARTESIAN_POINT('Ctrl Pts',(69.9786611769871,1078.67702975542,368.947389375261));
#119427=CARTESIAN_POINT('Ctrl Pts',(70.0088029708973,1078.67612768734,368.927265206454));
#119428=CARTESIAN_POINT('Ctrl Pts',(70.0383607050039,1078.6752067494,368.905923237811));
#119429=CARTESIAN_POINT('Ctrl Pts',(70.0671162296579,1078.6742734662,368.883489823463));
#119430=CARTESIAN_POINT('Ctrl Pts',(70.0958788993767,1078.6733399511,368.861050834944));
#119431=CARTESIAN_POINT('Ctrl Pts',(70.123838479359,1078.6723940846,368.837520198105));
#119432=CARTESIAN_POINT('Ctrl Pts',(70.1508077805883,1078.67144239617,368.81306629771));
#119433=CARTESIAN_POINT('Ctrl Pts',(70.1687464501386,1078.67080937924,368.796800750647));
#119434=CARTESIAN_POINT('Ctrl Pts',(70.1862476557113,1078.67017378653,368.78012759345));
#119435=CARTESIAN_POINT('Ctrl Pts',(70.2032653927109,1078.66953753953,368.763105366256));
#119436=CARTESIAN_POINT('Ctrl Pts',(70.2383773093518,1078.66822480028,368.727984185201));
#119437=CARTESIAN_POINT('Ctrl Pts',(70.2717988799081,1078.66689541973,368.691008063464));
#119438=CARTESIAN_POINT('Ctrl Pts',(70.303297459044,1078.66555961571,368.652396671917));
#119439=CARTESIAN_POINT('Ctrl Pts',(70.3347779802083,1078.66422457749,368.61380741608));
#119440=CARTESIAN_POINT('Ctrl Pts',(70.3643372941782,1078.66288312317,368.573585218041));
#119441=CARTESIAN_POINT('Ctrl Pts',(70.3917814682312,1078.66154545297,368.531984642556));
#119442=CARTESIAN_POINT('Ctrl Pts',(70.4192463413744,1078.66020677388,368.490352690864));
#119443=CARTESIAN_POINT('Ctrl Pts',(70.4445925464701,1078.65887188463,368.447340802391));
#119444=CARTESIAN_POINT('Ctrl Pts',(70.4676697967241,1078.65755100857,368.403232139552));
#119445=CARTESIAN_POINT('Ctrl Pts',(70.4880669909355,1078.65638353129,368.364245997251));
#119446=CARTESIAN_POINT('Ctrl Pts',(70.5066921717936,1078.65522700137,368.324403695189));
#119447=CARTESIAN_POINT('Ctrl Pts',(70.5234728961012,1078.65408847797,368.283913799739));
#119448=CARTESIAN_POINT('Ctrl Pts',(70.5423509878215,1078.65280765429,368.238363205733));
#119449=CARTESIAN_POINT('Ctrl Pts',(70.5590001328656,1078.65154335145,368.191736150675));
#119450=CARTESIAN_POINT('Ctrl Pts',(70.5732838951057,1078.6503058413,368.144319216869));
#119451=CARTESIAN_POINT('Ctrl Pts',(70.5875571559638,1078.64906924097,368.09693714386));
#119452=CARTESIAN_POINT('Ctrl Pts',(70.5994682789034,1078.64785939396,368.048766927578));
#119453=CARTESIAN_POINT('Ctrl Pts',(70.608929510515,1078.64668654949,368.00011371078));
#119454=CARTESIAN_POINT('Ctrl Pts',(70.618395766857,1078.64551308214,367.951434654926));
#119455=CARTESIAN_POINT('Ctrl Pts',(70.6254094006007,1078.64437665664,367.902272693871));
#119456=CARTESIAN_POINT('Ctrl Pts',(70.6299336955014,1078.64328753856,367.852943785523));
#119457=CARTESIAN_POINT('Ctrl Pts',(70.6340334740229,1078.64230061286,367.808243428147));
#119458=CARTESIAN_POINT('Ctrl Pts',(70.6360897811352,1078.64135253334,367.763406441123));
#119459=CARTESIAN_POINT('Ctrl Pts',(70.636112290058,1078.64045093853,367.718668875577));
#119460=CARTESIAN_POINT('Ctrl Pts',(70.6361306194975,1078.63971675292,367.682238233956));
#119461=CARTESIAN_POINT('Ctrl Pts',(70.6347980636925,1078.63900781863,367.64558925659));
#119462=CARTESIAN_POINT('Ctrl Pts',(70.6320921581352,1078.63832976351,367.608974014984));
#119463=CARTESIAN_POINT('Ctrl Pts',(70.6293876811409,1078.63765206636,367.572378104124));
#119464=CARTESIAN_POINT('Ctrl Pts',(70.625311306697,1078.63700521579,367.535816484357));
#119465=CARTESIAN_POINT('Ctrl Pts',(70.6198927054709,1078.63639483075,367.499539201815));
#119466=CARTESIAN_POINT('Ctrl Pts',(70.6163845710028,1078.6359996526,367.476052405134));
#119467=CARTESIAN_POINT('Ctrl Pts',(70.6123149010517,1078.63561975927,367.452684733468));
#119468=CARTESIAN_POINT('Ctrl Pts',(70.6077032114111,1078.63525667561,367.429501920333));
#119469=CARTESIAN_POINT('Ctrl Pts',(70.5988938480721,1078.63456310423,367.385217538674));
#119470=CARTESIAN_POINT('Ctrl Pts',(70.588095576243,1078.63392774252,367.341515392521));
#119471=CARTESIAN_POINT('Ctrl Pts',(70.5753316548135,1078.63335222651,367.298388859185));
#119472=CARTESIAN_POINT('Ctrl Pts',(70.5625816171825,1078.63277733651,367.255309236206));
#119473=CARTESIAN_POINT('Ctrl Pts',(70.5478699270497,1078.63226216208,367.21280307215));
#119474=CARTESIAN_POINT('Ctrl Pts',(70.5311703381008,1078.63180833392,367.170878721247));
#119475=CARTESIAN_POINT('Ctrl Pts',(70.5287932953106,1078.63174373539,367.164911150646));
#119476=CARTESIAN_POINT('Ctrl Pts',(70.5263758980182,1078.63168037979,367.158955406119));
#119477=CARTESIAN_POINT('Ctrl Pts',(70.5239179945542,1078.63161827185,367.153011552871));
#119478=CARTESIAN_POINT('Ctrl Pts',(70.5093450285995,1078.6312500324,367.117770310779));
#119479=CARTESIAN_POINT('Ctrl Pts',(70.4933514000306,1078.63092718475,367.082966502713));
#119480=CARTESIAN_POINT('Ctrl Pts',(70.4760287367767,1078.63065157815,367.048837815222));
#119481=CARTESIAN_POINT('Ctrl Pts',(70.4586916236253,1078.63037574165,367.014680658896));
#119482=CARTESIAN_POINT('Ctrl Pts',(70.4400235261928,1078.63014722503,366.981200293855));
#119483=CARTESIAN_POINT('Ctrl Pts',(70.420162889289,1078.62996788219,366.948611321319));
#119484=CARTESIAN_POINT('Ctrl Pts',(70.4094681278935,1078.6298713078,366.931062473964));
#119485=CARTESIAN_POINT('Ctrl Pts',(70.3984283410797,1078.62978899241,366.913771648191));
#119486=CARTESIAN_POINT('Ctrl Pts',(70.3870702416581,1078.62972122551,366.896768714476));
#119487=CARTESIAN_POINT('Ctrl Pts',(70.3622003491434,1078.62957284193,366.859538794378));
#119488=CARTESIAN_POINT('Ctrl Pts',(70.3356819388416,1078.62949150588,366.823495001307));
#119489=CARTESIAN_POINT('Ctrl Pts',(70.3075069097702,1078.62947843671,366.78863737677));
#119490=CARTESIAN_POINT('Ctrl Pts',(70.2795732684654,1078.62946547951,366.754078392709));
#119491=CARTESIAN_POINT('Ctrl Pts',(70.2500106423273,1078.62951962446,366.72068467377));
#119492=CARTESIAN_POINT('Ctrl Pts',(70.2187753212431,1078.62964205983,366.688492556518));
#119493=CARTESIAN_POINT('Ctrl Pts',(70.2137096637967,1078.62966191606,366.683271728532));
#119494=CARTESIAN_POINT('Ctrl Pts',(70.20859994706,1078.62968356842,366.678082594804));
#119495=CARTESIAN_POINT('Ctrl Pts',(70.2034459129137,1078.62970702199,366.672925419438));
#119496=CARTESIAN_POINT('Ctrl Pts',(70.153642759543,1078.62993365258,366.62309191263));
#119497=CARTESIAN_POINT('Ctrl Pts',(70.1005834878078,1078.63032599499,366.577120035045));
#119498=CARTESIAN_POINT('Ctrl Pts',(70.0446997169128,1078.63087440028,366.535213962577));
#119499=CARTESIAN_POINT('Ctrl Pts',(69.9858388820021,1078.63145202045,366.491075451989));
#119500=CARTESIAN_POINT('Ctrl Pts',(69.9238428387631,1078.63220277408,366.451445317227));
#119501=CARTESIAN_POINT('Ctrl Pts',(69.8591657617108,1078.63311538654,366.41658757856));
#119502=CARTESIAN_POINT('Ctrl Pts',(69.8151253679448,1078.63373680937,366.392851989282));
#119503=CARTESIAN_POINT('Ctrl Pts',(69.7698407589187,1078.63443328001,366.371329815705));
#119504=CARTESIAN_POINT('Ctrl Pts',(69.7234507243797,1078.63520123882,366.352117646964));
#119505=CARTESIAN_POINT('Ctrl Pts',(69.6817292201314,1078.63589191295,366.334838923469));
#119506=CARTESIAN_POINT('Ctrl Pts',(69.6394448286438,1078.63663436471,366.319561988434));
#119507=CARTESIAN_POINT('Ctrl Pts',(69.5966115042897,1078.63742637666,366.306247787561));
#119508=CARTESIAN_POINT('Ctrl Pts',(69.5536388323326,1078.63822096521,366.292890272236));
#119509=CARTESIAN_POINT('Ctrl Pts',(69.5101127552433,1078.63906543694,366.281507975003));
#119510=CARTESIAN_POINT('Ctrl Pts',(69.4660291753488,1078.63995755266,366.27211020656));
#119511=CARTESIAN_POINT('Ctrl Pts',(69.4596877970459,1078.6400858826,366.270758347091));
#119512=CARTESIAN_POINT('Ctrl Pts',(69.4533348654621,1078.64021519842,366.269447638946));
#119513=CARTESIAN_POINT('Ctrl Pts',(69.4469703547381,1078.64034549345,366.268178197808));
#119514=CARTESIAN_POINT('Ctrl Pts',(69.4115753791297,1078.64107010364,366.261118450401));
#119515=CARTESIAN_POINT('Ctrl Pts',(69.3757272816245,1078.64182781151,366.255320538375));
#119516=CARTESIAN_POINT('Ctrl Pts',(69.3396692499277,1078.64261197157,366.250850751106));
#119517=CARTESIAN_POINT('Ctrl Pts',(69.3036070482776,1078.64339622231,366.246380446926));
#119518=CARTESIAN_POINT('Ctrl Pts',(69.2673354426477,1078.64420693137,366.24323867791));
#119519=CARTESIAN_POINT('Ctrl Pts',(69.23110555833,1078.64503745094,366.241440140562));
#119520=CARTESIAN_POINT('Ctrl Pts',(69.2066284800311,1078.64559855383,366.240225040368));
#119521=CARTESIAN_POINT('Ctrl Pts',(69.1821706012387,1078.64616869906,366.239621961141));
#119522=CARTESIAN_POINT('Ctrl Pts',(69.1578093449994,1078.64674583663,366.23962196114));
#119523=CARTESIAN_POINT('Origin',(69.1578093449752,1067.7251047501,367.717925093334));
#119524=CARTESIAN_POINT('',(69.1578093449752,1076.68648464657,368.596228225527));
#119525=CARTESIAN_POINT('',(69.1578093460768,1076.65741108276,366.83962196114));
#119526=CARTESIAN_POINT('Ctrl Pts',(69.1578093449752,1076.68648464657,368.596228225527));
#119527=CARTESIAN_POINT('Ctrl Pts',(69.1033913216514,1076.68745213356,368.596228225527));
#119528=CARTESIAN_POINT('Ctrl Pts',(69.0489568302921,1076.68833127394,368.591170819637));
#119529=CARTESIAN_POINT('Ctrl Pts',(68.8806783358555,1076.690788854,368.559470806678));
#119530=CARTESIAN_POINT('Ctrl Pts',(68.7715682797969,1076.69200219795,368.515308799181));
#119531=CARTESIAN_POINT('Ctrl Pts',(68.5767947391705,1076.69347843089,368.386857203596));
#119532=CARTESIAN_POINT('Ctrl Pts',(68.4931144571871,1076.69372679574,368.303782852469));
#119533=CARTESIAN_POINT('Ctrl Pts',(68.3631859945438,1076.6932401161,368.109848421111));
#119534=CARTESIAN_POINT('Ctrl Pts',(68.3182074810282,1076.692509962,368.000940182514));
#119535=CARTESIAN_POINT('Ctrl Pts',(68.2734740550392,1076.69009005642,367.772113640544));
#119536=CARTESIAN_POINT('Ctrl Pts',(68.2740910388,1076.68842327646,367.654486218947));
#119537=CARTESIAN_POINT('Ctrl Pts',(68.3212194444405,1076.68423805352,367.426110114958));
#119538=CARTESIAN_POINT('Ctrl Pts',(68.3673558816376,1076.68175664377,367.317651689982));
#119539=CARTESIAN_POINT('Ctrl Pts',(68.4656778165328,1076.67762249391,367.174193405861));
#119540=CARTESIAN_POINT('Ctrl Pts',(68.5025586164138,1076.67620237088,367.130271796045));
#119541=CARTESIAN_POINT('Ctrl Pts',(68.5848923080706,1076.67325751785,367.049684240538));
#119542=CARTESIAN_POINT('Ctrl Pts',(68.6302535863163,1076.67173882008,367.013322693962));
#119543=CARTESIAN_POINT('Ctrl Pts',(68.7754303711597,1076.66716266438,366.918879626459));
#119544=CARTESIAN_POINT('Ctrl Pts',(68.8834192681614,1076.66410705643,366.875667143876));
#119545=CARTESIAN_POINT('Ctrl Pts',(69.0499335363381,1076.65990656262,366.844589377721));
#119546=CARTESIAN_POINT('Ctrl Pts',(69.1038777531703,1076.65861970931,366.839621961005));
#119547=CARTESIAN_POINT('Ctrl Pts',(69.1578093471783,1076.65741108276,366.839621961141));
#119548=CARTESIAN_POINT('',(69.1578093449752,1082.7251047501,366.83962196114));
#119549=CARTESIAN_POINT('',(69.1578093449752,1067.7251047501,366.83962196114));
#119550=CARTESIAN_POINT('Origin',(69.1578093449752,1082.7251047501,367.717925093334));
#119551=CARTESIAN_POINT('Ctrl Pts',(69.1578093471783,1076.65741108276,366.839621961141));
#119552=CARTESIAN_POINT('Ctrl Pts',(69.2185893566547,1076.65604898073,366.839621961293));
#119553=CARTESIAN_POINT('Ctrl Pts',(69.2793533349976,1076.65478627884,366.845931115126));
#119554=CARTESIAN_POINT('Ctrl Pts',(69.4518434428587,1076.65151826913,366.882320930328));
#119555=CARTESIAN_POINT('Ctrl Pts',(69.5588086901154,1076.64989055328,366.928055881927));
#119556=CARTESIAN_POINT('Ctrl Pts',(69.7488354249485,1076.64793522068,367.058121529201));
#119557=CARTESIAN_POINT('Ctrl Pts',(69.8300894466683,1076.64762590062,367.141129793432));
#119558=CARTESIAN_POINT('Ctrl Pts',(69.9558650303434,1076.64839705208,367.333586542729));
#119559=CARTESIAN_POINT('Ctrl Pts',(69.9992304916355,1076.64946717695,367.441127444555));
#119560=CARTESIAN_POINT('Ctrl Pts',(70.0300594458653,1076.65185531037,367.603360484574));
#119561=CARTESIAN_POINT('Ctrl Pts',(70.0351869866777,1076.65269087043,367.653477995551));
#119562=CARTESIAN_POINT('Ctrl Pts',(70.0359981836434,1076.65362084856,367.703756266315));
#119563=CARTESIAN_POINT('Ctrl Pts',(70.0378500058754,1076.65574382761,367.818532853905));
#119564=CARTESIAN_POINT('Ctrl Pts',(70.0171825981728,1076.6583288395,367.932558929511));
#119565=CARTESIAN_POINT('Ctrl Pts',(69.9331307082613,1076.66401532473,368.146283551002));
#119566=CARTESIAN_POINT('Ctrl Pts',(69.8705162180584,1076.667060243,368.243911836661));
#119567=CARTESIAN_POINT('Ctrl Pts',(69.7510970754531,1076.67161375661,368.36809574681));
#119568=CARTESIAN_POINT('Ctrl Pts',(69.7073423318817,1076.67311852531,368.405475708202));
#119569=CARTESIAN_POINT('Ctrl Pts',(69.5642433266447,1076.67758605903,368.505281356192));
#119570=CARTESIAN_POINT('Ctrl Pts',(69.4558031000024,1076.68039187618,368.552383553611));
#119571=CARTESIAN_POINT('Ctrl Pts',(69.280854745882,1076.68418363178,368.589761703587));
#119572=CARTESIAN_POINT('Ctrl Pts',(69.2193425741478,1076.68539065977,368.596228225527));
#119573=CARTESIAN_POINT('Ctrl Pts',(69.1578093449752,1076.68648464657,368.596228225527));
#119574=CARTESIAN_POINT('Origin',(81.0356882485065,1067.7251047501,371.795432834555));
#119575=CARTESIAN_POINT('',(81.0356882485327,1078.30327084026,370.519988713418));
#119576=CARTESIAN_POINT('Ctrl Pts',(81.0358308103573,1078.39242989444,373.070876947723));
#119577=CARTESIAN_POINT('Ctrl Pts',(81.1884057339834,1078.38464480654,373.070859893771));
#119578=CARTESIAN_POINT('Ctrl Pts',(81.3397012484411,1078.37589925079,373.043466129561));
#119579=CARTESIAN_POINT('Ctrl Pts',(81.6362004968986,1078.35649977253,372.932561804349));
#119580=CARTESIAN_POINT('Ctrl Pts',(81.7773347281252,1078.34592815118,372.84597014097));
#119581=CARTESIAN_POINT('Ctrl Pts',(82.0221333562771,1078.32463994517,372.621261163093));
#119582=CARTESIAN_POINT('Ctrl Pts',(82.1223789098522,1078.31413379904,372.484049947285));
#119583=CARTESIAN_POINT('Ctrl Pts',(82.2604701861183,1078.29547983935,372.18579151591));
#119584=CARTESIAN_POINT('Ctrl Pts',(82.2998253150436,1078.28741255873,372.028814535696));
#119585=CARTESIAN_POINT('Ctrl Pts',(82.3180263290313,1078.27452947834,371.712080372361));
#119586=CARTESIAN_POINT('Ctrl Pts',(82.2980863433854,1078.26975656345,371.555181212364));
#119587=CARTESIAN_POINT('Ctrl Pts',(82.230290382327,1078.26569525718,371.343864336666));
#119588=CARTESIAN_POINT('Ctrl Pts',(82.2057103902217,1078.26483747344,371.283536647818));
#119589=CARTESIAN_POINT('Ctrl Pts',(82.1637902669127,1078.26409447237,371.199639910996));
#119590=CARTESIAN_POINT('Ctrl Pts',(82.1500816406033,1078.26393383565,371.174376650431));
#119591=CARTESIAN_POINT('Ctrl Pts',(82.1253259030924,1078.26377515,371.132218174737));
#119592=CARTESIAN_POINT('Ctrl Pts',(82.1147099969581,1078.26374289513,371.11508294322));
#119593=CARTESIAN_POINT('Ctrl Pts',(82.092485921406,1078.26374479798,371.081040332632));
#119594=CARTESIAN_POINT('Ctrl Pts',(82.0808671468127,1078.26378010454,371.064146957027));
#119595=CARTESIAN_POINT('Ctrl Pts',(82.0515881305638,1078.26394965979,371.023700129456));
#119596=CARTESIAN_POINT('Ctrl Pts',(82.0335101567194,1078.26412026554,371.000464073211));
#119597=CARTESIAN_POINT('Ctrl Pts',(81.9677303517599,1078.26496011535,370.921698343161));
#119598=CARTESIAN_POINT('Ctrl Pts',(81.916071287035,1078.26599219976,370.869669134888));
#119599=CARTESIAN_POINT('Ctrl Pts',(81.7305123881603,1078.27081199972,370.712431814371));
#119600=CARTESIAN_POINT('Ctrl Pts',(81.5801518157617,1078.2763930109,370.629589776234));
#119601=CARTESIAN_POINT('Ctrl Pts',(81.2836407110295,1078.28987780946,370.536414934771));
#119602=CARTESIAN_POINT('Ctrl Pts',(81.1432081065826,1078.29712579653,370.516753914293));
#119603=CARTESIAN_POINT('Ctrl Pts',(80.8499294205669,1078.31384887624,370.524396367248));
#119604=CARTESIAN_POINT('Ctrl Pts',(80.6993718381563,1078.32332341751,370.555709947107));
#119605=CARTESIAN_POINT('Ctrl Pts',(80.4061269803256,1078.34352829353,370.674173509885));
#119606=CARTESIAN_POINT('Ctrl Pts',(80.2675152898507,1078.35411256255,370.764177743707));
#119607=CARTESIAN_POINT('Ctrl Pts',(80.0287193674031,1078.3746344643,370.994770384816));
#119608=CARTESIAN_POINT('Ctrl Pts',(79.9319894839163,1078.38434908772,371.134426379589));
#119609=CARTESIAN_POINT('Ctrl Pts',(79.8016793128289,1078.40100311338,371.435544837902));
#119610=CARTESIAN_POINT('Ctrl Pts',(79.7663144653885,1078.40791454577,371.592892921503));
#119611=CARTESIAN_POINT('Ctrl Pts',(79.7555594008279,1078.41884473075,371.9138956309));
#119612=CARTESIAN_POINT('Ctrl Pts',(79.7807739763514,1078.42274345753,372.074677947513));
#119613=CARTESIAN_POINT('Ctrl Pts',(79.8544181503619,1078.42567992686,372.279743248795));
#119614=CARTESIAN_POINT('Ctrl Pts',(79.8770507726827,1078.426226461,372.331637364107));
#119615=CARTESIAN_POINT('Ctrl Pts',(79.9149836863006,1078.42670601796,372.40490167505));
#119616=CARTESIAN_POINT('Ctrl Pts',(79.9276143978122,1078.42681086608,372.427574705602));
#119617=CARTESIAN_POINT('Ctrl Pts',(79.9510629483887,1078.42691439707,372.466801468702));
#119618=CARTESIAN_POINT('Ctrl Pts',(79.9615904440653,1078.42693243513,372.483518435096));
#119619=CARTESIAN_POINT('Ctrl Pts',(79.9840364482984,1078.42691457718,372.517390040069));
#119620=CARTESIAN_POINT('Ctrl Pts',(79.9959966323434,1078.42687554582,372.534509998901));
#119621=CARTESIAN_POINT('Ctrl Pts',(80.0272844313338,1078.4267014353,372.577032364982));
#119622=CARTESIAN_POINT('Ctrl Pts',(80.0471550020037,1078.42652657543,372.602017026243));
#119623=CARTESIAN_POINT('Ctrl Pts',(80.1267268383092,1078.42559156516,372.694705612336));
#119624=CARTESIAN_POINT('Ctrl Pts',(80.1926097137023,1078.42434897808,372.756743560868));
#119625=CARTESIAN_POINT('Ctrl Pts',(80.3621654348938,1078.42014608295,372.885463580501));
#119626=CARTESIAN_POINT('Ctrl Pts',(80.4700191567871,1078.41675140564,372.945131146269));
#119627=CARTESIAN_POINT('Ctrl Pts',(80.7289068154651,1078.40704746284,373.042994997205));
#119628=CARTESIAN_POINT('Ctrl Pts',(80.8817622928742,1078.4002911925,373.070894168621));
#119629=CARTESIAN_POINT('Ctrl Pts',(81.0358308103573,1078.39242989444,373.070876947723));
#119630=CARTESIAN_POINT('',(81.0356882484902,1076.29851503552,370.519988713418));
#119631=CARTESIAN_POINT('',(81.0356882485065,1067.7251047501,370.519988713418));
#119632=CARTESIAN_POINT('Ctrl Pts',(81.0350565731442,1076.38864406689,373.070876799269));
#119633=CARTESIAN_POINT('Ctrl Pts',(80.8664862906615,1076.39733226541,373.070793313285));
#119634=CARTESIAN_POINT('Ctrl Pts',(80.6995315644439,1076.40467581067,373.037291772264));
#119635=CARTESIAN_POINT('Ctrl Pts',(80.3878190702641,1076.41605389929,372.907023308189));
#119636=CARTESIAN_POINT('Ctrl Pts',(80.2462379881508,1076.41997082751,372.811387209307));
#119637=CARTESIAN_POINT('Ctrl Pts',(80.0083555405032,1076.42395235266,372.570101428271));
#119638=CARTESIAN_POINT('Ctrl Pts',(79.9145584601887,1076.42397030439,372.426774287735));
#119639=CARTESIAN_POINT('Ctrl Pts',(79.7886672873119,1076.42005915076,372.112191055772));
#119640=CARTESIAN_POINT('Ctrl Pts',(79.7577013174188,1076.41617589414,371.944158949024));
#119641=CARTESIAN_POINT('Ctrl Pts',(79.7631060572532,1076.40485953809,371.606355933519));
#119642=CARTESIAN_POINT('Ctrl Pts',(79.7992394641575,1076.39754357679,371.439949186657));
#119643=CARTESIAN_POINT('Ctrl Pts',(79.9342772081048,1076.38018301084,371.130405535808));
#119644=CARTESIAN_POINT('Ctrl Pts',(80.0320561229994,1076.37029650381,370.990413983824));
#119645=CARTESIAN_POINT('Ctrl Pts',(80.2142332201473,1076.35452936383,370.816218435966));
#119646=CARTESIAN_POINT('Ctrl Pts',(80.2796872431149,1076.34920883116,370.764845732684));
#119647=CARTESIAN_POINT('Ctrl Pts',(80.4923704658847,1076.33287422385,370.629148188538));
#119648=CARTESIAN_POINT('Ctrl Pts',(80.6518029340403,1076.32184527168,370.5674030045));
#119649=CARTESIAN_POINT('Ctrl Pts',(80.9837668752778,1076.30114301383,370.510077213482));
#119650=CARTESIAN_POINT('Ctrl Pts',(81.1529565440444,1076.29165948219,370.514369669047));
#119651=CARTESIAN_POINT('Ctrl Pts',(81.479741220954,1076.27562556121,370.588133207905));
#119652=CARTESIAN_POINT('Ctrl Pts',(81.6341893472203,1076.26922910276,370.656751372915));
#119653=CARTESIAN_POINT('Ctrl Pts',(81.9073817641115,1076.26059966692,370.849513871025));
#119654=CARTESIAN_POINT('Ctrl Pts',(82.0235678754709,1076.25844036517,370.971585818619));
#119655=CARTESIAN_POINT('Ctrl Pts',(82.2021010434889,1076.25873859831,371.253243552757));
#119656=CARTESIAN_POINT('Ctrl Pts',(82.2628343095997,1076.26118130393,371.409971277465));
#119657=CARTESIAN_POINT('Ctrl Pts',(82.3206615205412,1076.27029388232,371.737851187403));
#119658=CARTESIAN_POINT('Ctrl Pts',(82.3171892246466,1076.27687221552,371.905812334753));
#119659=CARTESIAN_POINT('Ctrl Pts',(82.2459237164212,1076.29315510069,372.231203944968));
#119660=CARTESIAN_POINT('Ctrl Pts',(82.1786575957118,1076.30270616538,372.385474573604));
#119661=CARTESIAN_POINT('Ctrl Pts',(81.9884413495885,1076.32335627142,372.659687639345));
#119662=CARTESIAN_POINT('Ctrl Pts',(81.8671613616621,1076.33425872348,372.776920528879));
#119663=CARTESIAN_POINT('Ctrl Pts',(81.5841304790166,1076.35603408549,372.959375490447));
#119664=CARTESIAN_POINT('Ctrl Pts',(81.4245552059327,1076.36668916406,373.021955669117));
#119665=CARTESIAN_POINT('Ctrl Pts',(81.1839937467045,1076.3807211026,373.064415325453));
#119666=CARTESIAN_POINT('Ctrl Pts',(81.1096012482494,1076.38480199623,373.070913718206));
#119667=CARTESIAN_POINT('Ctrl Pts',(81.0350565731442,1076.38864406688,373.070876799269));
#119668=CARTESIAN_POINT('Origin',(81.0356882485065,1067.7251047501,371.795432834555));
#119669=CARTESIAN_POINT('',(81.0356882485065,1076.36858155369,372.470876955691));
#119670=CARTESIAN_POINT('',(81.0356882485072,1076.32087957987,371.119988713418));
#119671=CARTESIAN_POINT('Ctrl Pts',(81.0356882485065,1076.36858155369,372.470876955691));
#119672=CARTESIAN_POINT('Ctrl Pts',(80.9466770371988,1076.37328023044,372.470876955691));
#119673=CARTESIAN_POINT('Ctrl Pts',(80.858496420118,1076.37729165449,372.453281738094));
#119674=CARTESIAN_POINT('Ctrl Pts',(80.6931986193752,1076.38356420663,372.384512535967));
#119675=CARTESIAN_POINT('Ctrl Pts',(80.6178670477176,1076.38574621753,372.333715093343));
#119676=CARTESIAN_POINT('Ctrl Pts',(80.4914463209232,1076.38795918467,372.205482579773));
#119677=CARTESIAN_POINT('Ctrl Pts',(80.441669457937,1076.38796586462,372.129321688419));
#119678=CARTESIAN_POINT('Ctrl Pts',(80.3749629387847,1076.38577894784,371.962060009786));
#119679=CARTESIAN_POINT('Ctrl Pts',(80.3586739916778,1076.3836093465,371.872672515698));
#119680=CARTESIAN_POINT('Ctrl Pts',(80.3620505018149,1076.37733324501,371.692930128103));
#119681=CARTESIAN_POINT('Ctrl Pts',(80.3816374802864,1076.37329081345,371.604382799259));
#119682=CARTESIAN_POINT('Ctrl Pts',(80.4543124070447,1076.36379836162,371.440021372384));
#119683=CARTESIAN_POINT('Ctrl Pts',(80.5067431586288,1076.35843882412,371.365871375587));
#119684=CARTESIAN_POINT('Ctrl Pts',(80.6041627856006,1076.34998549194,371.273943714408));
#119685=CARTESIAN_POINT('Ctrl Pts',(80.6390795219818,1076.34715044972,371.246920070266));
#119686=CARTESIAN_POINT('Ctrl Pts',(80.75227468855,1076.33850025317,371.175807294144));
#119687=CARTESIAN_POINT('Ctrl Pts',(80.8369215519361,1076.33272090615,371.143700506065));
#119688=CARTESIAN_POINT('Ctrl Pts',(80.9618312322459,1076.32508481194,371.123022719963));
#119689=CARTESIAN_POINT('Ctrl Pts',(80.9987260469959,1076.32293230681,371.119988713418));
#119690=CARTESIAN_POINT('Ctrl Pts',(81.0356882485079,1076.32087957987,371.119988713418));
#119691=CARTESIAN_POINT('',(81.0356882485065,1082.7251047501,371.119988713418));
#119692=CARTESIAN_POINT('',(81.0356882485065,1067.7251047501,371.119988713418));
#119693=CARTESIAN_POINT('Origin',(81.0356882485065,1082.7251047501,371.795432834555));
#119694=CARTESIAN_POINT('Ctrl Pts',(81.0356882485079,1076.32087957987,371.119988713418));
#119695=CARTESIAN_POINT('Ctrl Pts',(81.0357054443659,1076.32087862488,371.119988713418));
#119696=CARTESIAN_POINT('Ctrl Pts',(81.0357226402371,1076.32087766989,371.119988713433));
#119697=CARTESIAN_POINT('Ctrl Pts',(81.0357398361243,1076.32087671495,371.119988714746));
#119698=CARTESIAN_POINT('Ctrl Pts',(81.1243435443242,1076.31595626447,371.119995482045));
#119699=CARTESIAN_POINT('Ctrl Pts',(81.2121212293695,1076.31167662248,371.1374365346));
#119700=CARTESIAN_POINT('Ctrl Pts',(81.3757717600072,1076.30495878294,371.20518644674));
#119701=CARTESIAN_POINT('Ctrl Pts',(81.4500812808145,1076.30258252459,371.254752409407));
#119702=CARTESIAN_POINT('Ctrl Pts',(81.5752349561495,1076.30010567544,371.379610221861));
#119703=CARTESIAN_POINT('Ctrl Pts',(81.624909378144,1076.30002439202,371.453617243076));
#119704=CARTESIAN_POINT('Ctrl Pts',(81.6929459822121,1076.30218324274,371.616489854028));
#119705=CARTESIAN_POINT('Ctrl Pts',(81.7106653117081,1076.30440012159,371.703751217166));
#119706=CARTESIAN_POINT('Ctrl Pts',(81.711581903132,1076.31082095477,371.880232247626));
#119707=CARTESIAN_POINT('Ctrl Pts',(81.6947185259169,1076.31496437524,371.967740683178));
#119708=CARTESIAN_POINT('Ctrl Pts',(81.6282500105839,1076.32459376466,372.131471779847));
#119709=CARTESIAN_POINT('Ctrl Pts',(81.5791991967838,1076.32998936313,372.206089947184));
#119710=CARTESIAN_POINT('Ctrl Pts',(81.4861691653524,1076.33845164833,372.300653578167));
#119711=CARTESIAN_POINT('Ctrl Pts',(81.4521293101644,1076.34131459263,372.329059735823));
#119712=CARTESIAN_POINT('Ctrl Pts',(81.3790581437592,1076.34703343511,372.378759987772));
#119713=CARTESIAN_POINT('Ctrl Pts',(81.3402091740787,1076.3498758091,372.39994986762));
#119714=CARTESIAN_POINT('Ctrl Pts',(81.2168163045953,1076.35834006927,372.452318629312));
#119715=CARTESIAN_POINT('Ctrl Pts',(81.1278547392712,1076.36370538279,372.470577877855));
#119716=CARTESIAN_POINT('Ctrl Pts',(81.0371671841974,1076.36850344002,372.470875741445));
#119717=CARTESIAN_POINT('Ctrl Pts',(81.0364276876917,1076.36854252056,372.470876955691));
#119718=CARTESIAN_POINT('Ctrl Pts',(81.0356882485065,1076.36858155369,372.470876955691));
#119719=CARTESIAN_POINT('Origin',(93.672037736222,1067.7251047501,377.464729830671));
#119720=CARTESIAN_POINT('',(93.6720377362532,1077.61442735557,376.365898694678));
#119721=CARTESIAN_POINT('Ctrl Pts',(93.6722192570493,1077.71636978598,378.563560951671));
#119722=CARTESIAN_POINT('Ctrl Pts',(93.8069726126999,1077.70416449936,378.563538691161));
#119723=CARTESIAN_POINT('Ctrl Pts',(93.940501286018,1077.69085765877,378.538730121288));
#119724=CARTESIAN_POINT('Ctrl Pts',(94.2016485877809,1077.66224246217,378.43838866533));
#119725=CARTESIAN_POINT('Ctrl Pts',(94.3255105403184,1077.64712923762,378.359985369633));
#119726=CARTESIAN_POINT('Ctrl Pts',(94.5347285823885,1077.61827030834,378.160376146465));
#119727=CARTESIAN_POINT('Ctrl Pts',(94.6184400607495,1077.60478587765,378.04139872997));
#119728=CARTESIAN_POINT('Ctrl Pts',(94.7296608502277,1077.58235612848,377.790162862338));
#119729=CARTESIAN_POINT('Ctrl Pts',(94.7608616898128,1077.5732810015,377.66220907866));
#119730=CARTESIAN_POINT('Ctrl Pts',(94.7768578192544,1077.55920490251,377.400090184243));
#119731=CARTESIAN_POINT('Ctrl Pts',(94.761151718272,1077.5543550064,377.268059088689));
#119732=CARTESIAN_POINT('Ctrl Pts',(94.7132900568707,1077.55143784041,377.112337778839));
#119733=CARTESIAN_POINT('Ctrl Pts',(94.7029581550161,1077.55102180196,377.08316740982));
#119734=CARTESIAN_POINT('Ctrl Pts',(94.6839831446964,1077.55056687306,377.03602026585));
#119735=CARTESIAN_POINT('Ctrl Pts',(94.6760580635762,1077.55044644325,377.017775007529));
#119736=CARTESIAN_POINT('Ctrl Pts',(94.6609820194468,1077.5503341694,376.985494206524));
#119737=CARTESIAN_POINT('Ctrl Pts',(94.6540163884814,1077.55032075154,376.971378526587));
#119738=CARTESIAN_POINT('Ctrl Pts',(94.638659320679,1077.5503688821,376.941872610019));
#119739=CARTESIAN_POINT('Ctrl Pts',(94.6301980774744,1077.55043909865,376.9265238189));
#119740=CARTESIAN_POINT('Ctrl Pts',(94.6069027087987,1077.5507426925,376.886557620365));
#119741=CARTESIAN_POINT('Ctrl Pts',(94.591464265452,1077.55105160028,376.862309430856));
#119742=CARTESIAN_POINT('Ctrl Pts',(94.5201593218287,1077.55291754057,376.759451893077));
#119743=CARTESIAN_POINT('Ctrl Pts',(94.4550541510353,1077.55569270544,376.687813708108));
#119744=CARTESIAN_POINT('Ctrl Pts',(94.2985320845842,1077.56426327506,376.555481884181));
#119745=CARTESIAN_POINT('Ctrl Pts',(94.2057097935229,1077.57034920252,376.498092424018));
#119746=CARTESIAN_POINT('Ctrl Pts',(93.9942661857174,1077.58605697478,376.407181231617));
#119747=CARTESIAN_POINT('Ctrl Pts',(93.875350856341,1077.59590936187,376.378058458468));
#119748=CARTESIAN_POINT('Ctrl Pts',(93.6225289033882,1077.61876654283,376.35910222023));
#119749=CARTESIAN_POINT('Ctrl Pts',(93.4902316494238,1077.63178686478,376.373046808699));
#119750=CARTESIAN_POINT('Ctrl Pts',(93.2274118087518,1077.65976644178,376.449898376105));
#119751=CARTESIAN_POINT('Ctrl Pts',(93.1001687450403,1077.67454334546,376.515757354355));
#119752=CARTESIAN_POINT('Ctrl Pts',(92.875384414685,1077.70331172652,376.694145559379));
#119753=CARTESIAN_POINT('Ctrl Pts',(92.7806737081482,1077.71700711364,376.80595132329));
#119754=CARTESIAN_POINT('Ctrl Pts',(92.6442788952363,1077.74049955449,377.052639481322));
#119755=CARTESIAN_POINT('Ctrl Pts',(92.6009804713983,1077.75027787408,377.183641342492));
#119756=CARTESIAN_POINT('Ctrl Pts',(92.5645515134517,1077.76578290103,377.456560579428));
#119757=CARTESIAN_POINT('Ctrl Pts',(92.5723172959504,1077.77132429832,377.596096035243));
#119758=CARTESIAN_POINT('Ctrl Pts',(92.617145577569,1077.77537339781,377.775874390503));
#119759=CARTESIAN_POINT('Ctrl Pts',(92.631313516235,1077.77610400737,377.820401539368));
#119760=CARTESIAN_POINT('Ctrl Pts',(92.6552155756255,1077.77672037922,377.881704528439));
#119761=CARTESIAN_POINT('Ctrl Pts',(92.6626225706082,1077.77685015094,377.899328791607));
#119762=CARTESIAN_POINT('Ctrl Pts',(92.6770338023038,1077.77699746021,377.931260024202));
#119763=CARTESIAN_POINT('Ctrl Pts',(92.683896484605,1077.77703011922,377.94562495789));
#119764=CARTESIAN_POINT('Ctrl Pts',(92.6983841906382,1077.77702681335,377.974329900841));
#119765=CARTESIAN_POINT('Ctrl Pts',(92.7060198356745,1077.77698946814,377.988660046438));
#119766=CARTESIAN_POINT('Ctrl Pts',(92.7254306868201,1077.77681124326,378.023221273012));
#119767=CARTESIAN_POINT('Ctrl Pts',(92.7375399568977,1077.77663198026,378.043255067068));
#119768=CARTESIAN_POINT('Ctrl Pts',(92.7822988664053,1077.7757428724,378.112228474618));
#119769=CARTESIAN_POINT('Ctrl Pts',(92.8182241127524,1077.77464221183,378.158912856635));
#119770=CARTESIAN_POINT('Ctrl Pts',(92.955485621408,1077.7692326222,378.310420338624));
#119771=CARTESIAN_POINT('Ctrl Pts',(93.0736737001234,1077.76264378489,378.39775559986));
#119772=CARTESIAN_POINT('Ctrl Pts',(93.2844673200733,1077.74825829438,378.496651028051));
#119773=CARTESIAN_POINT('Ctrl Pts',(93.3677105903819,1077.74204282004,378.524182025668));
#119774=CARTESIAN_POINT('Ctrl Pts',(93.5253735340906,1077.72931031049,378.556211222365));
#119775=CARTESIAN_POINT('Ctrl Pts',(93.5987219805113,1077.72302680259,378.563573093014));
#119776=CARTESIAN_POINT('Ctrl Pts',(93.6722192570494,1077.71636978598,378.563560951671));
#119777=CARTESIAN_POINT('',(93.6720377362221,1075.60303707734,376.365898694679));
#119778=CARTESIAN_POINT('',(93.672037736222,1067.7251047501,376.365898694679));
#119779=CARTESIAN_POINT('Ctrl Pts',(93.6718533219435,1075.70594646218,378.563560951189));
#119780=CARTESIAN_POINT('Ctrl Pts',(93.5264011728922,1075.71923995543,378.563536540292));
#119781=CARTESIAN_POINT('Ctrl Pts',(93.3822507739243,1075.73099086691,378.534632194512));
#119782=CARTESIAN_POINT('Ctrl Pts',(93.1132797204475,1075.75015626527,378.422064723482));
#119783=CARTESIAN_POINT('Ctrl Pts',(92.9911786947583,1075.75737768,378.339487097749));
#119784=CARTESIAN_POINT('Ctrl Pts',(92.7871558505531,1075.76630049765,378.132106267149));
#119785=CARTESIAN_POINT('Ctrl Pts',(92.7069670767,1075.767959732,378.009765079275));
#119786=CARTESIAN_POINT('Ctrl Pts',(92.5992293667541,1075.76555675552,377.742355363055));
#119787=CARTESIAN_POINT('Ctrl Pts',(92.5722187985566,1075.76157684131,377.600200246242));
#119788=CARTESIAN_POINT('Ctrl Pts',(92.5742681550686,1075.74832304881,377.311065603305));
#119789=CARTESIAN_POINT('Ctrl Pts',(92.6043371897209,1075.73908663897,377.166993298332));
#119790=CARTESIAN_POINT('Ctrl Pts',(92.7188044499007,1075.71647031607,376.899016341679));
#119791=CARTESIAN_POINT('Ctrl Pts',(92.80213277933,1075.70330675867,376.777796144562));
#119792=CARTESIAN_POINT('Ctrl Pts',(92.957757529143,1075.68200378671,376.626679273154));
#119793=CARTESIAN_POINT('Ctrl Pts',(93.0136780383686,1075.67477205783,376.58207328005));
#119794=CARTESIAN_POINT('Ctrl Pts',(93.1335681882368,1075.66003685109,376.504204542886));
#119795=CARTESIAN_POINT('Ctrl Pts',(93.1972919032829,1075.65256627695,376.471163708906));
#119796=CARTESIAN_POINT('Ctrl Pts',(93.3994687805416,1075.62990018571,376.390253784415));
#119797=CARTESIAN_POINT('Ctrl Pts',(93.5447127617592,1075.61497447705,376.363538608292));
#119798=CARTESIAN_POINT('Ctrl Pts',(93.8354181602545,1075.58770264304,376.368553787696));
#119799=CARTESIAN_POINT('Ctrl Pts',(93.978088294476,1075.57558818508,376.399502214301));
#119800=CARTESIAN_POINT('Ctrl Pts',(94.2426651545265,1075.55582408963,376.51472645125));
#119801=CARTESIAN_POINT('Ctrl Pts',(94.3621119467305,1075.54834330311,376.597554918917));
#119802=CARTESIAN_POINT('Ctrl Pts',(94.5617904319835,1075.5391317027,376.804204799827));
#119803=CARTESIAN_POINT('Ctrl Pts',(94.6402580869334,1075.53746098628,376.925729772193));
#119804=CARTESIAN_POINT('Ctrl Pts',(94.7460161189048,1075.54018185347,377.191853128827));
#119805=CARTESIAN_POINT('Ctrl Pts',(94.7723507116371,1075.54453380114,377.333746448445));
#119806=CARTESIAN_POINT('Ctrl Pts',(94.7692532755111,1075.55867537877,377.619964173259));
#119807=CARTESIAN_POINT('Ctrl Pts',(94.7396711864189,1075.56834103044,377.761473666155));
#119808=CARTESIAN_POINT('Ctrl Pts',(94.6277405914666,1075.59167914103,378.025791613268));
#119809=CARTESIAN_POINT('Ctrl Pts',(94.5461379024299,1075.60514926797,378.145934458013));
#119810=CARTESIAN_POINT('Ctrl Pts',(94.3924695673108,1075.62678943036,378.297563876846));
#119811=CARTESIAN_POINT('Ctrl Pts',(94.3362606254359,1075.63420691134,378.343045695243));
#119812=CARTESIAN_POINT('Ctrl Pts',(94.2159504354054,1075.64916839968,378.422204779237));
#119813=CARTESIAN_POINT('Ctrl Pts',(94.1521513402626,1075.65667739653,378.455734718383));
#119814=CARTESIAN_POINT('Ctrl Pts',(93.9542201423241,1075.67878305921,378.536126584217));
#119815=CARTESIAN_POINT('Ctrl Pts',(93.813744660885,1075.69297840658,378.563584764483));
#119816=CARTESIAN_POINT('Ctrl Pts',(93.6718533219435,1075.70594646218,378.563560951189));
#119817=CARTESIAN_POINT('Origin',(93.672037736222,1067.7251047501,377.464729830671));
#119818=CARTESIAN_POINT('',(93.6720377362219,1075.67866049267,377.963560966664));
#119819=CARTESIAN_POINT('',(93.672037736222,1075.63195590694,376.965898694679));
#119820=CARTESIAN_POINT('Ctrl Pts',(93.6720377362219,1075.67866049267,377.963560966664));
#119821=CARTESIAN_POINT('Ctrl Pts',(93.6058998860328,1075.684763007,377.963560966664));
#119822=CARTESIAN_POINT('Ctrl Pts',(93.5403511446652,1075.69018085178,377.950407548697));
#119823=CARTESIAN_POINT('Ctrl Pts',(93.4179092189567,1075.69904625754,377.899093828582));
#119824=CARTESIAN_POINT('Ctrl Pts',(93.3622879773617,1075.70239783057,377.861369755518));
#119825=CARTESIAN_POINT('Ctrl Pts',(93.2701945710849,1075.70649147921,377.767352417574));
#119826=CARTESIAN_POINT('Ctrl Pts',(93.234208934487,1075.70725376,377.712455394587));
#119827=CARTESIAN_POINT('Ctrl Pts',(93.1853227757369,1075.70617538341,377.591902707691));
#119828=CARTESIAN_POINT('Ctrl Pts',(93.1729159538782,1075.70434469343,377.52744659807));
#119829=CARTESIAN_POINT('Ctrl Pts',(93.1735087932216,1075.69828795475,377.397205779866));
#119830=CARTESIAN_POINT('Ctrl Pts',(93.1866054048728,1075.69411175676,377.332706721366));
#119831=CARTESIAN_POINT('Ctrl Pts',(93.2372996771602,1075.68382886917,377.21124250193));
#119832=CARTESIAN_POINT('Ctrl Pts',(93.274893086152,1075.67778614536,377.155676442994));
#119833=CARTESIAN_POINT('Ctrl Pts',(93.3453758446788,1075.66803744424,377.086337562461));
#119834=CARTESIAN_POINT('Ctrl Pts',(93.3707100698784,1075.66473559238,377.065869730989));
#119835=CARTESIAN_POINT('Ctrl Pts',(93.4250289965021,1075.65802442011,377.030128954924));
#119836=CARTESIAN_POINT('Ctrl Pts',(93.4538948022533,1075.65463035487,377.014946826748));
#119837=CARTESIAN_POINT('Ctrl Pts',(93.5437056075,1075.64455376019,376.978402820946));
#119838=CARTESIAN_POINT('Ctrl Pts',(93.6075511765563,1075.63799913074,376.965898694679));
#119839=CARTESIAN_POINT('Ctrl Pts',(93.672037736222,1075.63195590694,376.965898694679));
#119840=CARTESIAN_POINT('',(93.672037736222,1082.7251047501,376.965898694679));
#119841=CARTESIAN_POINT('',(93.672037736222,1067.7251047501,376.965898694679));
#119842=CARTESIAN_POINT('Origin',(93.672037736222,1082.7251047501,377.464729830671));
#119843=CARTESIAN_POINT('Ctrl Pts',(93.672037736222,1075.63195590694,376.965898694679));
#119844=CARTESIAN_POINT('Ctrl Pts',(93.6720484915353,1075.63195489903,376.965898694679));
#119845=CARTESIAN_POINT('Ctrl Pts',(93.6720592468665,1075.63195389113,376.965898695025));
#119846=CARTESIAN_POINT('Ctrl Pts',(93.6720700022155,1075.63195288325,376.965898695721));
#119847=CARTESIAN_POINT('Ctrl Pts',(93.7381764088161,1075.62575805452,376.965902971695));
#119848=CARTESIAN_POINT('Ctrl Pts',(93.8036919268756,1075.62021962966,376.979048112777));
#119849=CARTESIAN_POINT('Ctrl Pts',(93.9249685551116,1075.61120428251,377.029854466407));
#119850=CARTESIAN_POINT('Ctrl Pts',(93.979678677085,1075.60778648756,377.066656469242));
#119851=CARTESIAN_POINT('Ctrl Pts',(94.0716200681311,1075.603496699,377.159123318087));
#119852=CARTESIAN_POINT('Ctrl Pts',(94.1080262747016,1075.60265471042,377.213772593599));
#119853=CARTESIAN_POINT('Ctrl Pts',(94.1577777270919,1075.6036696957,377.333919423654));
#119854=CARTESIAN_POINT('Ctrl Pts',(94.1706559676332,1075.60551295254,377.3982030184));
#119855=CARTESIAN_POINT('Ctrl Pts',(94.1710772677511,1075.61165428562,377.528248779548));
#119856=CARTESIAN_POINT('Ctrl Pts',(94.1585298528844,1075.61589956251,377.592730355597));
#119857=CARTESIAN_POINT('Ctrl Pts',(94.1093259777868,1075.6262445344,377.713505120068));
#119858=CARTESIAN_POINT('Ctrl Pts',(94.0730001144866,1075.63225474547,377.768580069253));
#119859=CARTESIAN_POINT('Ctrl Pts',(94.0041977852763,1075.64197104994,377.838320117501));
#119860=CARTESIAN_POINT('Ctrl Pts',(93.9790269289867,1075.64530535397,377.859263394115));
#119861=CARTESIAN_POINT('Ctrl Pts',(93.9250115168889,1075.65205820513,377.895890811382));
#119862=CARTESIAN_POINT('Ctrl Pts',(93.8962977328366,1075.65546102669,377.91149925783));
#119863=CARTESIAN_POINT('Ctrl Pts',(93.8050509164328,1075.66574049287,377.950072140307));
#119864=CARTESIAN_POINT('Ctrl Pts',(93.7392424435488,1075.67245522381,377.963470859681));
#119865=CARTESIAN_POINT('Ctrl Pts',(93.6724858533722,1075.67861913784,377.963560815709));
#119866=CARTESIAN_POINT('Ctrl Pts',(93.6722617914164,1075.67863981918,377.963560966664));
#119867=CARTESIAN_POINT('Ctrl Pts',(93.6720377362219,1075.67866049267,377.963560966664));
#119868=CARTESIAN_POINT('Origin',(104.994450521159,1067.7251047501,385.676728598176));
#119869=CARTESIAN_POINT('',(104.994450521181,1076.76862933859,384.586187849449));
#119870=CARTESIAN_POINT('Ctrl Pts',(104.994633285524,1076.87046141638,386.76726933159));
#119871=CARTESIAN_POINT('Ctrl Pts',(105.131833259839,1076.85333286283,386.767246338165));
#119872=CARTESIAN_POINT('Ctrl Pts',(105.267718545062,1076.83509138601,386.741333633219));
#119873=CARTESIAN_POINT('Ctrl Pts',(105.530325094078,1076.79716254288,386.63757987829));
#119874=CARTESIAN_POINT('Ctrl Pts',(105.653538059104,1076.77780942427,386.557668010356));
#119875=CARTESIAN_POINT('Ctrl Pts',(105.858143402187,1076.74234604782,386.357287723099));
#119876=CARTESIAN_POINT('Ctrl Pts',(105.938900147509,1076.72647291626,386.239988648573));
#119877=CARTESIAN_POINT('Ctrl Pts',(106.043387948015,1076.70163546465,385.998859661691));
#119878=CARTESIAN_POINT('Ctrl Pts',(106.072793049309,1076.69219014714,385.87994369037));
#119879=CARTESIAN_POINT('Ctrl Pts',(106.089667233352,1076.6793090253,385.655445393521));
#119880=CARTESIAN_POINT('Ctrl Pts',(106.082737437329,1076.67524695972,385.55177151307));
#119881=CARTESIAN_POINT('Ctrl Pts',(106.055200125584,1076.67258699994,385.421877171064));
#119882=CARTESIAN_POINT('Ctrl Pts',(106.047963832544,1076.67216051198,385.393446127906));
#119883=CARTESIAN_POINT('Ctrl Pts',(106.034704465905,1076.67174196399,385.348942751733));
#119884=CARTESIAN_POINT('Ctrl Pts',(106.029434046577,1076.67164299811,385.332663259662));
#119885=CARTESIAN_POINT('Ctrl Pts',(106.01899629093,1076.67156241664,385.302836808276));
#119886=CARTESIAN_POINT('Ctrl Pts',(106.013937755519,1076.67156516685,385.289256166582));
#119887=CARTESIAN_POINT('Ctrl Pts',(106.002169479634,1076.67165893655,385.259489458096));
#119888=CARTESIAN_POINT('Ctrl Pts',(105.995337394395,1076.67176826091,385.243356421428));
#119889=CARTESIAN_POINT('Ctrl Pts',(105.974960017513,1076.67224037247,385.198293275171));
#119890=CARTESIAN_POINT('Ctrl Pts',(105.960529291255,1076.67273749297,385.169786125775));
#119891=CARTESIAN_POINT('Ctrl Pts',(105.874194892632,1076.67652888274,385.016349175557));
#119892=CARTESIAN_POINT('Ctrl Pts',(105.779405815304,1076.68347640333,384.906142161435));
#119893=CARTESIAN_POINT('Ctrl Pts',(105.575566594723,1076.70206856823,384.746786035878));
#119894=CARTESIAN_POINT('Ctrl Pts',(105.474525489599,1076.71236791538,384.690855692307));
#119895=CARTESIAN_POINT('Ctrl Pts',(105.247953699509,1076.73743328187,384.608552052302));
#119896=CARTESIAN_POINT('Ctrl Pts',(105.122669325942,1076.75236128811,384.586432904679));
#119897=CARTESIAN_POINT('Ctrl Pts',(104.860053917182,1076.78568102768,384.58592683987));
#119898=CARTESIAN_POINT('Ctrl Pts',(104.72477820044,1076.80397641313,384.611292371405));
#119899=CARTESIAN_POINT('Ctrl Pts',(104.462369570083,1076.84178556993,384.713769297562));
#119900=CARTESIAN_POINT('Ctrl Pts',(104.338813916159,1076.86094567878,384.793209576895));
#119901=CARTESIAN_POINT('Ctrl Pts',(104.133173658214,1076.89582103737,384.99304978521));
#119902=CARTESIAN_POINT('Ctrl Pts',(104.051829332693,1076.91130668487,385.110335141414));
#119903=CARTESIAN_POINT('Ctrl Pts',(103.9493959124,1076.93472860304,385.344783563755));
#119904=CARTESIAN_POINT('Ctrl Pts',(103.920335107035,1076.94340083518,385.456122569877));
#119905=CARTESIAN_POINT('Ctrl Pts',(103.898341977279,1076.95632730457,385.679937638596));
#119906=CARTESIAN_POINT('Ctrl Pts',(103.904281400433,1076.96065170195,385.79087886747));
#119907=CARTESIAN_POINT('Ctrl Pts',(103.932945111882,1076.96340025134,385.928496425229));
#119908=CARTESIAN_POINT('Ctrl Pts',(103.940279985098,1076.96382644933,385.957629889771));
#119909=CARTESIAN_POINT('Ctrl Pts',(103.953690200165,1076.9642419062,386.00290731595));
#119910=CARTESIAN_POINT('Ctrl Pts',(103.958960841991,1076.96434001242,386.019271660269));
#119911=CARTESIAN_POINT('Ctrl Pts',(103.968910185781,1076.9644190025,386.047830336804));
#119912=CARTESIAN_POINT('Ctrl Pts',(103.97342510192,1076.96442241269,386.060077753699));
#119913=CARTESIAN_POINT('Ctrl Pts',(103.984192208757,1076.96436037941,386.087744436638));
#119914=CARTESIAN_POINT('Ctrl Pts',(103.990579517295,1076.96427578225,386.103107385609));
#119915=CARTESIAN_POINT('Ctrl Pts',(104.008814937133,1076.96391202882,386.144284037777));
#119916=CARTESIAN_POINT('Ctrl Pts',(104.021323346397,1076.9635377495,386.169789331306));
#119917=CARTESIAN_POINT('Ctrl Pts',(104.085327406492,1076.96107813431,386.288351459443));
#119918=CARTESIAN_POINT('Ctrl Pts',(104.149224725981,1076.95713113042,386.373974107909));
#119919=CARTESIAN_POINT('Ctrl Pts',(104.301834591077,1076.94529580539,386.526146918114));
#119920=CARTESIAN_POINT('Ctrl Pts',(104.390313940337,1076.93736524954,386.59116430131));
#119921=CARTESIAN_POINT('Ctrl Pts',(104.571110202303,1076.91937906314,386.686247035992));
#119922=CARTESIAN_POINT('Ctrl Pts',(104.660724526256,1076.90979923496,386.719288662887));
#119923=CARTESIAN_POINT('Ctrl Pts',(104.832603767784,1076.89024419292,386.758248009956));
#119924=CARTESIAN_POINT('Ctrl Pts',(104.913525354245,1076.88058723128,386.767282924516));
#119925=CARTESIAN_POINT('Ctrl Pts',(104.994633285524,1076.87046141638,386.76726933159));
#119926=CARTESIAN_POINT('',(104.994450521159,1074.74993967683,384.586187849448));
#119927=CARTESIAN_POINT('',(104.994450521159,1067.7251047501,384.586187849448));
#119928=CARTESIAN_POINT('Ctrl Pts',(104.993488433118,1074.85275892785,386.767268922521));
#119929=CARTESIAN_POINT('Ctrl Pts',(104.848894050105,1074.87095330795,386.767141359584));
#119930=CARTESIAN_POINT('Ctrl Pts',(104.705538610491,1074.88756311335,386.738257385749));
#119931=CARTESIAN_POINT('Ctrl Pts',(104.438687030779,1074.91567748798,386.626080293747));
#119932=CARTESIAN_POINT('Ctrl Pts',(104.317764632415,1074.92692549908,386.544119650505));
#119933=CARTESIAN_POINT('Ctrl Pts',(104.115898398542,1074.94251123594,386.338505252222));
#119934=CARTESIAN_POINT('Ctrl Pts',(104.036584485142,1074.94676743849,386.217424362304));
#119935=CARTESIAN_POINT('Ctrl Pts',(103.929993585147,1074.94781847454,385.952935140033));
#119936=CARTESIAN_POINT('Ctrl Pts',(103.903175231259,1074.94469329364,385.812505239435));
#119937=CARTESIAN_POINT('Ctrl Pts',(103.904692652719,1074.93132865139,385.526049797475));
#119938=CARTESIAN_POINT('Ctrl Pts',(103.93432703878,1074.92106172641,385.382974201478));
#119939=CARTESIAN_POINT('Ctrl Pts',(104.047585187939,1074.89462196658,385.116602069858));
#119940=CARTESIAN_POINT('Ctrl Pts',(104.130245107814,1074.8786936825,384.996058232639));
#119941=CARTESIAN_POINT('Ctrl Pts',(104.338162169601,1074.84312401658,384.793680168606));
#119942=CARTESIAN_POINT('Ctrl Pts',(104.461731642368,1074.82379728769,384.714110364067));
#119943=CARTESIAN_POINT('Ctrl Pts',(104.73363518047,1074.784287512,384.607741245521));
#119944=CARTESIAN_POINT('Ctrl Pts',(104.879567783969,1074.76447519522,384.582376661305));
#119945=CARTESIAN_POINT('Ctrl Pts',(105.169986449437,1074.72767768233,384.590840635096));
#119946=CARTESIAN_POINT('Ctrl Pts',(105.311734870644,1074.71098974609,384.623437323337));
#119947=CARTESIAN_POINT('Ctrl Pts',(105.573464807664,1074.68286566589,384.741611689425));
#119948=CARTESIAN_POINT('Ctrl Pts',(105.6910983992,1074.67165698388,384.825544961858));
#119949=CARTESIAN_POINT('Ctrl Pts',(105.886435982201,1074.65632244418,385.03346829857));
#119950=CARTESIAN_POINT('Ctrl Pts',(105.962559155349,1074.65228317652,385.154959248906));
#119951=CARTESIAN_POINT('Ctrl Pts',(106.06371306275,1074.65190767947,385.419886601982));
#119952=CARTESIAN_POINT('Ctrl Pts',(106.087946901198,1074.65553960046,385.560513977255));
#119953=CARTESIAN_POINT('Ctrl Pts',(106.081449055933,1074.67000160222,385.843526770489));
#119954=CARTESIAN_POINT('Ctrl Pts',(106.050584602473,1074.68071050683,385.983067765841));
#119955=CARTESIAN_POINT('Ctrl Pts',(105.937020596228,1074.7078463793,386.243487413592));
#119956=CARTESIAN_POINT('Ctrl Pts',(105.85492648638,1074.72406183403,386.361644029438));
#119957=CARTESIAN_POINT('Ctrl Pts',(105.649393385778,1074.7598564498,386.560450824642));
#119958=CARTESIAN_POINT('Ctrl Pts',(105.527488624727,1074.77913013045,386.638879168424));
#119959=CARTESIAN_POINT('Ctrl Pts',(105.330629273114,1074.80778502169,386.716392154147));
#119960=CARTESIAN_POINT('Ctrl Pts',(105.265058168699,1074.81698560129,386.735355511107));
#119961=CARTESIAN_POINT('Ctrl Pts',(105.130707495125,1074.83517037925,386.760898443258));
#119962=CARTESIAN_POINT('Ctrl Pts',(105.062187610499,1074.84411447763,386.767329529778));
#119963=CARTESIAN_POINT('Ctrl Pts',(104.993488433118,1074.85275892785,386.767268922522));
#119964=CARTESIAN_POINT('Origin',(104.994450521159,1067.7251047501,385.676728598176));
#119965=CARTESIAN_POINT('',(104.994450521159,1074.82513013623,386.167269346904));
#119966=CARTESIAN_POINT('',(104.994450521159,1074.77893852154,385.186187849448));
#119967=CARTESIAN_POINT('Ctrl Pts',(104.994450521159,1074.82513013623,386.167269346904));
#119968=CARTESIAN_POINT('Ctrl Pts',(104.961419275554,1074.82930714217,386.167269346904));
#119969=CARTESIAN_POINT('Ctrl Pts',(104.928372056375,1074.83332530481,386.163933201317));
#119970=CARTESIAN_POINT('Ctrl Pts',(104.831883977299,1074.84457534412,386.144127822702));
#119971=CARTESIAN_POINT('Ctrl Pts',(104.771100254234,1074.85102591974,386.118354154493));
#119972=CARTESIAN_POINT('Ctrl Pts',(104.663869618342,1074.86108560777,386.04484503087));
#119973=CARTESIAN_POINT('Ctrl Pts',(104.618302621517,1074.86463432453,385.99817313082));
#119974=CARTESIAN_POINT('Ctrl Pts',(104.548366762419,1074.86840152833,385.890500793405));
#119975=CARTESIAN_POINT('Ctrl Pts',(104.524399009584,1074.86863103434,385.830813769502));
#119976=CARTESIAN_POINT('Ctrl Pts',(104.500619619116,1074.86578258252,385.705541217366));
#119977=CARTESIAN_POINT('Ctrl Pts',(104.501073431236,1074.86273014935,385.641222927864));
#119978=CARTESIAN_POINT('Ctrl Pts',(104.526837632459,1074.85358833337,385.514693139946));
#119979=CARTESIAN_POINT('Ctrl Pts',(104.552589963409,1074.84750928077,385.453910247323));
#119980=CARTESIAN_POINT('Ctrl Pts',(104.626388233192,1074.8331465811,385.345880995702));
#119981=CARTESIAN_POINT('Ctrl Pts',(104.673807640141,1074.82499455012,385.299771707557));
#119982=CARTESIAN_POINT('Ctrl Pts',(104.784046408763,1074.80769812398,385.228755129994));
#119983=CARTESIAN_POINT('Ctrl Pts',(104.845888373133,1074.7987138235,385.204629265908));
#119984=CARTESIAN_POINT('Ctrl Pts',(104.938305311029,1074.78620333812,385.188603019807));
#119985=CARTESIAN_POINT('Ctrl Pts',(104.966346558262,1074.78251941681,385.186187849448));
#119986=CARTESIAN_POINT('Ctrl Pts',(104.994450521159,1074.77893852154,385.186187849448));
#119987=CARTESIAN_POINT('',(104.994450521159,1082.7251047501,385.186187849448));
#119988=CARTESIAN_POINT('',(104.994450521159,1067.7251047501,385.186187849448));
#119989=CARTESIAN_POINT('Origin',(104.994450521159,1082.7251047501,385.676728598176));
#119990=CARTESIAN_POINT('Ctrl Pts',(104.994450521159,1074.77893852154,385.186187849448));
#119991=CARTESIAN_POINT('Ctrl Pts',(104.994464257439,1074.77893677132,385.186187849448));
#119992=CARTESIAN_POINT('Ctrl Pts',(104.994477993734,1074.77893502112,385.186187850023));
#119993=CARTESIAN_POINT('Ctrl Pts',(104.994491730044,1074.77893327095,385.186187851177));
#119994=CARTESIAN_POINT('Ctrl Pts',(105.059640385892,1074.77063253974,385.186193324124));
#119995=CARTESIAN_POINT('Ctrl Pts',(105.124238028413,1074.76299834931,385.199177344179));
#119996=CARTESIAN_POINT('Ctrl Pts',(105.243714845829,1074.75010145091,385.249381071327));
#119997=CARTESIAN_POINT('Ctrl Pts',(105.297582269794,1074.74492664549,385.285709133516));
#119998=CARTESIAN_POINT('Ctrl Pts',(105.387874370596,1074.73768627985,385.376856186067));
#119999=CARTESIAN_POINT('Ctrl Pts',(105.423554179795,1074.73566461898,385.430581951871));
#120000=CARTESIAN_POINT('Ctrl Pts',(105.472206670697,1074.73503589283,385.548540810414));
#120001=CARTESIAN_POINT('Ctrl Pts',(105.484780053331,1074.73642066584,385.611525372796));
#120002=CARTESIAN_POINT('Ctrl Pts',(105.485197961527,1074.74242685904,385.738943318982));
#120003=CARTESIAN_POINT('Ctrl Pts',(105.472950987099,1074.74699876339,385.802095233921));
#120004=CARTESIAN_POINT('Ctrl Pts',(105.424901815903,1074.75876995799,385.920588122722));
#120005=CARTESIAN_POINT('Ctrl Pts',(105.389351189106,1074.76587783325,385.974693766438));
#120006=CARTESIAN_POINT('Ctrl Pts',(105.298329439124,1074.78187046461,386.067408110274));
#120007=CARTESIAN_POINT('Ctrl Pts',(105.24319545496,1074.79064456718,386.104614012243));
#120008=CARTESIAN_POINT('Ctrl Pts',(105.152746248563,1074.80389813393,386.142136541162));
#120009=CARTESIAN_POINT('Ctrl Pts',(105.121934370952,1074.80824743372,386.151502715335));
#120010=CARTESIAN_POINT('Ctrl Pts',(105.05876146013,1074.81684508775,386.164106074168));
#120011=CARTESIAN_POINT('Ctrl Pts',(105.026613563918,1074.82106291994,386.167269346904));
#120012=CARTESIAN_POINT('Ctrl Pts',(104.994450521159,1074.82513013623,386.167269346904));
#120013=CARTESIAN_POINT('Origin',(55.815888242722,1067.7251047501,354.582660180055));
#120014=CARTESIAN_POINT('',(55.8158882427517,1078.63997504936,353.104357047861));
#120015=CARTESIAN_POINT('Ctrl Pts',(57.2939968241464,1078.64787169026,354.606642927438));
#120016=CARTESIAN_POINT('Ctrl Pts',(57.2969184316135,1078.64352236629,354.426577941565));
#120017=CARTESIAN_POINT('Ctrl Pts',(57.266912218914,1078.63966729243,354.247472367867));
#120018=CARTESIAN_POINT('Ctrl Pts',(57.145828661031,1078.63368068486,353.913962040012));
#120019=CARTESIAN_POINT('Ctrl Pts',(57.0575700354636,1078.63155159986,353.761604601839));
#120020=CARTESIAN_POINT('Ctrl Pts',(56.9104943662943,1078.63007661884,353.587655299811));
#120021=CARTESIAN_POINT('Ctrl Pts',(56.8740669522224,1078.62982565291,353.548999118833));
#120022=CARTESIAN_POINT('Ctrl Pts',(56.8129432314803,1078.62957717498,353.490760801996));
#120023=CARTESIAN_POINT('Ctrl Pts',(56.789564844328,1078.62951801421,353.469863349694));
#120024=CARTESIAN_POINT('Ctrl Pts',(56.7450898180418,1078.62947008869,353.432583392865));
#120025=CARTESIAN_POINT('Ctrl Pts',(56.7241795261188,1078.62947216577,353.415998648908));
#120026=CARTESIAN_POINT('Ctrl Pts',(56.676976352036,1078.62953006807,353.380598655119));
#120027=CARTESIAN_POINT('Ctrl Pts',(56.6504920054245,1078.62959713719,353.362061477982));
#120028=CARTESIAN_POINT('Ctrl Pts',(56.5742373535414,1078.62988507737,353.312331596955));
#120029=CARTESIAN_POINT('Ctrl Pts',(56.5231862823401,1078.63018663483,353.283215133532));
#120030=CARTESIAN_POINT('Ctrl Pts',(56.2939538201222,1078.63199098522,353.169994991084));
#120031=CARTESIAN_POINT('Ctrl Pts',(56.1017200431752,1078.63463960227,353.118946086318));
#120032=CARTESIAN_POINT('Ctrl Pts',(55.745589600636,1078.64121184432,353.097401602526));
#120033=CARTESIAN_POINT('Ctrl Pts',(55.585518832982,1078.64475387938,353.113695084757));
#120034=CARTESIAN_POINT('Ctrl Pts',(55.2635527974551,1078.652906188,353.200470502829));
#120035=CARTESIAN_POINT('Ctrl Pts',(55.1051858181154,1078.65751512975,353.274829427366));
#120036=CARTESIAN_POINT('Ctrl Pts',(54.8113020715414,1078.66717696182,353.482283652066));
#120037=CARTESIAN_POINT('Ctrl Pts',(54.6808733268301,1078.67214756829,353.617379678643));
#120038=CARTESIAN_POINT('Ctrl Pts',(54.4719245610859,1078.6816697907,353.936645493797));
#120039=CARTESIAN_POINT('Ctrl Pts',(54.3983791070371,1078.68609408375,354.119788496336));
#120040=CARTESIAN_POINT('Ctrl Pts',(54.3278338269869,1078.69359342704,354.498491252392));
#120041=CARTESIAN_POINT('Ctrl Pts',(54.3293240155054,1078.69664048303,354.690013471633));
#120042=CARTESIAN_POINT('Ctrl Pts',(54.4021872456954,1078.70126943562,355.04988143644));
#120043=CARTESIAN_POINT('Ctrl Pts',(54.4683972021584,1078.70290214987,355.215998798835));
#120044=CARTESIAN_POINT('Ctrl Pts',(54.613838310897,1078.70455694528,355.44860008299));
#120045=CARTESIAN_POINT('Ctrl Pts',(54.6731883621541,1078.70496900646,355.525535153428));
#120046=CARTESIAN_POINT('Ctrl Pts',(54.767589425649,1078.70531607425,355.625786162928));
#120047=CARTESIAN_POINT('Ctrl Pts',(54.7967540417351,1078.70538890873,355.654298045532));
#120048=CARTESIAN_POINT('Ctrl Pts',(54.84576976925,1078.70545858904,355.698403792387));
#120049=CARTESIAN_POINT('Ctrl Pts',(54.8649067311524,1078.70547382994,355.714759038956));
#120050=CARTESIAN_POINT('Ctrl Pts',(54.9054491574829,1078.70548191424,355.747654584633));
#120051=CARTESIAN_POINT('Ctrl Pts',(54.9269098935684,1078.70547300861,355.76411216166));
#120052=CARTESIAN_POINT('Ctrl Pts',(54.978011082835,1078.70542165694,355.801119013134));
#120053=CARTESIAN_POINT('Ctrl Pts',(55.0079761274488,1078.70536904224,355.821190790078));
#120054=CARTESIAN_POINT('Ctrl Pts',(55.1046488053296,1078.70512954056,355.880943465592));
#120055=CARTESIAN_POINT('Ctrl Pts',(55.1737621594419,1078.70485839347,355.916479883787));
#120056=CARTESIAN_POINT('Ctrl Pts',(55.4267538566271,1078.7035121241,356.022321300206));
#120057=CARTESIAN_POINT('Ctrl Pts',(55.6214916457768,1078.70186102409,356.061259217013));
#120058=CARTESIAN_POINT('Ctrl Pts',(55.981739897164,1078.6974773684,356.060713995291));
#120059=CARTESIAN_POINT('Ctrl Pts',(56.1441760343487,1078.69499804822,356.033305645742));
#120060=CARTESIAN_POINT('Ctrl Pts',(56.4664743251616,1078.68880333957,355.921910257738));
#120061=CARTESIAN_POINT('Ctrl Pts',(56.6223443169839,1078.68504706121,355.834249011311));
#120062=CARTESIAN_POINT('Ctrl Pts',(56.9057054315686,1078.67633804477,355.599516228649));
#120063=CARTESIAN_POINT('Ctrl Pts',(57.0275736034234,1078.67139544533,355.450710142807));
#120064=CARTESIAN_POINT('Ctrl Pts',(57.1705702404536,1078.66331797367,355.184833116585));
#120065=CARTESIAN_POINT('Ctrl Pts',(57.2120608397622,1078.66031418798,355.081135640913));
#120066=CARTESIAN_POINT('Ctrl Pts',(57.2743500699509,1078.65407101206,354.854084693676));
#120067=CARTESIAN_POINT('Ctrl Pts',(57.2919833333689,1078.65086912363,354.730738718023));
#120068=CARTESIAN_POINT('Ctrl Pts',(57.2939968241464,1078.64787169026,354.606642927438));
#120069=CARTESIAN_POINT('',(55.8158882427049,1076.63887570959,353.104357047862));
#120070=CARTESIAN_POINT('',(55.815888242722,1067.7251047501,353.104357047862));
#120071=CARTESIAN_POINT('Ctrl Pts',(55.8159488750934,1076.69909976501,356.060963311005));
#120072=CARTESIAN_POINT('Ctrl Pts',(55.6205302673948,1076.70150112669,356.060971326069));
#120073=CARTESIAN_POINT('Ctrl Pts',(55.4270293164456,1076.7031613472,356.022230223064));
#120074=CARTESIAN_POINT('Ctrl Pts',(55.0656195798272,1076.70511406965,355.871443026767));
#120075=CARTESIAN_POINT('Ctrl Pts',(54.9014037352093,1076.70538694798,355.760617365159));
#120076=CARTESIAN_POINT('Ctrl Pts',(54.6260845612497,1076.70455121485,355.481597781454));
#120077=CARTESIAN_POINT('Ctrl Pts',(54.5176090973004,1076.70345118471,355.316274419462));
#120078=CARTESIAN_POINT('Ctrl Pts',(54.3717074783901,1076.69979801304,354.953778924329));
#120079=CARTESIAN_POINT('Ctrl Pts',(54.335408016863,1076.69727930961,354.760307636342));
#120080=CARTESIAN_POINT('Ctrl Pts',(54.3399685391359,1076.6907742897,354.370081298712));
#120081=CARTESIAN_POINT('Ctrl Pts',(54.3809338631428,1076.68684116129,354.177166361784));
#120082=CARTESIAN_POINT('Ctrl Pts',(54.4961456775211,1076.68009878215,353.90971080636));
#120083=CARTESIAN_POINT('Ctrl Pts',(54.5425784356717,1076.67775331901,353.825519238522));
#120084=CARTESIAN_POINT('Ctrl Pts',(54.652036610934,1076.67282477512,353.665953010365));
#120085=CARTESIAN_POINT('Ctrl Pts',(54.7150682705674,1076.67025030537,353.591147526017));
#120086=CARTESIAN_POINT('Ctrl Pts',(54.924069295383,1076.66241063477,353.387803372566));
#120087=CARTESIAN_POINT('Ctrl Pts',(55.088417322061,1076.65707067033,353.281195099306));
#120088=CARTESIAN_POINT('Ctrl Pts',(55.4490082435505,1076.64696688877,353.13750612433));
#120089=CARTESIAN_POINT('Ctrl Pts',(55.6417743015555,1076.64230806022,353.101861096665));
#120090=CARTESIAN_POINT('Ctrl Pts',(56.0299605837615,1076.63464889073,353.107123027127));
#120091=CARTESIAN_POINT('Ctrl Pts',(56.2216071052081,1076.6317288412,353.147933582595));
#120092=CARTESIAN_POINT('Ctrl Pts',(56.5778045152464,1076.62830445861,353.301111942892));
#120093=CARTESIAN_POINT('Ctrl Pts',(56.7389539407118,1076.62783146734,353.411833886296));
#120094=CARTESIAN_POINT('Ctrl Pts',(57.0090681159595,1076.62945740592,353.688776930316));
#120095=CARTESIAN_POINT('Ctrl Pts',(57.1155430882697,1076.63153277978,353.85218504));
#120096=CARTESIAN_POINT('Ctrl Pts',(57.2595455391089,1076.63778079007,354.210520645505));
#120097=CARTESIAN_POINT('Ctrl Pts',(57.295744328831,1076.64188570826,354.401971590899));
#120098=CARTESIAN_POINT('Ctrl Pts',(57.2925349242128,1076.65127643338,354.788087702466));
#120099=CARTESIAN_POINT('Ctrl Pts',(57.2530932340981,1076.65646600966,354.97904706042));
#120100=CARTESIAN_POINT('Ctrl Pts',(57.1405307400976,1076.66434065629,355.246009099696));
#120101=CARTESIAN_POINT('Ctrl Pts',(57.0943714723888,1076.66696296708,355.331118890569));
#120102=CARTESIAN_POINT('Ctrl Pts',(56.9861041145873,1076.67210986742,355.491124314132));
#120103=CARTESIAN_POINT('Ctrl Pts',(56.9242534152109,1076.67462204577,355.565635106593));
#120104=CARTESIAN_POINT('Ctrl Pts',(56.7162992535386,1076.68193309578,355.771366953678));
#120105=CARTESIAN_POINT('Ctrl Pts',(56.5510024355483,1076.68634792033,355.880111642091));
#120106=CARTESIAN_POINT('Ctrl Pts',(56.1934713067884,1076.69377697856,356.024454103851));
#120107=CARTESIAN_POINT('Ctrl Pts',(56.0055962117159,1076.69676932242,356.060955532649));
#120108=CARTESIAN_POINT('Ctrl Pts',(55.8159488750934,1076.69909976501,356.060963311005));
#120109=CARTESIAN_POINT('Origin',(55.815888242722,1067.7251047501,354.582660180055));
#120110=CARTESIAN_POINT('',(55.815888242722,1076.68940454296,355.460963312248));
#120111=CARTESIAN_POINT('',(55.8158882427295,1076.65362934538,353.704357047862));
#120112=CARTESIAN_POINT('Ctrl Pts',(55.815888242722,1076.68940454296,355.460963312248));
#120113=CARTESIAN_POINT('Ctrl Pts',(55.7020152112483,1076.69098784474,355.460963312248));
#120114=CARTESIAN_POINT('Ctrl Pts',(55.5891889227174,1076.69213028676,355.438817072165));
#120115=CARTESIAN_POINT('Ctrl Pts',(55.3754742486306,1076.69352199293,355.351506169293));
#120116=CARTESIAN_POINT('Ctrl Pts',(55.2771422558615,1076.6937347303,355.28611011008));
#120117=CARTESIAN_POINT('Ctrl Pts',(55.1119513573992,1076.69317380385,355.120743520564));
#120118=CARTESIAN_POINT('Ctrl Pts',(55.0467101966484,1076.69240603686,355.022460759002));
#120119=CARTESIAN_POINT('Ctrl Pts',(54.9586126127917,1076.68991215862,354.806421275002));
#120120=CARTESIAN_POINT('Ctrl Pts',(54.9365246902861,1076.68821059589,354.690861218791));
#120121=CARTESIAN_POINT('Ctrl Pts',(54.9387250458333,1076.68396437041,354.457744922806));
#120122=CARTESIAN_POINT('Ctrl Pts',(54.9630448406274,1076.68145810191,354.342505892462));
#120123=CARTESIAN_POINT('Ctrl Pts',(55.0317542656464,1076.67729810155,354.182888163623));
#120124=CARTESIAN_POINT('Ctrl Pts',(55.0594259513635,1076.6758715647,354.132717645012));
#120125=CARTESIAN_POINT('Ctrl Pts',(55.1245972640669,1076.67291653756,354.037777734949));
#120126=CARTESIAN_POINT('Ctrl Pts',(55.1620755956594,1076.67139407967,353.993330914934));
#120127=CARTESIAN_POINT('Ctrl Pts',(55.2862506747189,1076.66681439603,353.8726119167));
#120128=CARTESIAN_POINT('Ctrl Pts',(55.3838375411703,1076.66376624872,353.809344060017));
#120129=CARTESIAN_POINT('Ctrl Pts',(55.594289888278,1076.65818353779,353.725509099961));
#120130=CARTESIAN_POINT('Ctrl Pts',(55.7046005627282,1076.65568877212,353.70435704786));
#120131=CARTESIAN_POINT('Ctrl Pts',(55.815888242737,1076.65362934538,353.704357047862));
#120132=CARTESIAN_POINT('',(55.815888242722,1082.7251047501,353.704357047862));
#120133=CARTESIAN_POINT('',(55.815888242722,1067.7251047501,353.704357047862));
#120134=CARTESIAN_POINT('Origin',(55.815888242722,1082.7251047501,354.582660180055));
#120135=CARTESIAN_POINT('Ctrl Pts',(55.815888242737,1076.65362934538,353.704357047862));
#120136=CARTESIAN_POINT('Ctrl Pts',(55.8197649584117,1076.65355760507,353.704357047862));
#120137=CARTESIAN_POINT('Ctrl Pts',(55.8236428596713,1076.65348639333,353.704382714809));
#120138=CARTESIAN_POINT('Ctrl Pts',(55.94269192059,1076.6513172319,353.705959702638));
#120139=CARTESIAN_POINT('Ctrl Pts',(56.0564524851715,1076.64973468531,353.730125629126));
#120140=CARTESIAN_POINT('Ctrl Pts',(56.2680142300927,1076.64787775109,353.820931480909));
#120141=CARTESIAN_POINT('Ctrl Pts',(56.3637850202993,1076.64762079416,353.886629799102));
#120142=CARTESIAN_POINT('Ctrl Pts',(56.524435932203,1076.64849385808,354.051086024939));
#120143=CARTESIAN_POINT('Ctrl Pts',(56.5878053142086,1076.64961279919,354.148203815499));
#120144=CARTESIAN_POINT('Ctrl Pts',(56.6708758297469,1076.65291270086,354.354622230776));
#120145=CARTESIAN_POINT('Ctrl Pts',(56.692362346411,1076.65499271175,354.461025189534));
#120146=CARTESIAN_POINT('Ctrl Pts',(56.6940795884859,1076.65740429285,354.568647605487));
#120147=CARTESIAN_POINT('Ctrl Pts',(56.695912136676,1076.65997780223,354.683496447389));
#120148=CARTESIAN_POINT('Ctrl Pts',(56.675197332517,1076.66287848519,354.797591719143));
#120149=CARTESIAN_POINT('Ctrl Pts',(56.6120843920517,1076.66739708317,354.957871277574));
#120150=CARTESIAN_POINT('Ctrl Pts',(56.5858662871713,1076.66892038143,355.009093597327));
#120151=CARTESIAN_POINT('Ctrl Pts',(56.5238073760246,1076.6719520213,355.105692665344));
#120152=CARTESIAN_POINT('Ctrl Pts',(56.488114175994,1076.67345306842,355.150837026364));
#120153=CARTESIAN_POINT('Ctrl Pts',(56.3671601182725,1076.67789849534,355.276329231394));
#120154=CARTESIAN_POINT('Ctrl Pts',(56.2700564020598,1076.68068038924,355.343456793896));
#120155=CARTESIAN_POINT('Ctrl Pts',(56.0556557242177,1076.68557767416,355.435591881462));
#120156=CARTESIAN_POINT('Ctrl Pts',(55.9405592226238,1076.6876493049,355.45983816675));
#120157=CARTESIAN_POINT('Ctrl Pts',(55.8213514717962,1076.68932833524,355.460950571655));
#120158=CARTESIAN_POINT('Ctrl Pts',(55.8186195561669,1076.68936656651,355.460963312248));
#120159=CARTESIAN_POINT('Ctrl Pts',(55.815888242722,1076.68940454296,355.460963312248));
#120160=CARTESIAN_POINT('Origin',(68.2819685228176,1067.7251047501,356.101514707942));
#120161=CARTESIAN_POINT('',(68.2819685228382,1078.28930526318,354.826070586805));
#120162=CARTESIAN_POINT('Ctrl Pts',(68.282008024927,1078.40494025576,357.376958828466));
#120163=CARTESIAN_POINT('Ctrl Pts',(68.4272802061516,1078.39879186158,357.376954329204));
#120164=CARTESIAN_POINT('Ctrl Pts',(68.5714409895716,1078.39156248641,357.352130990053));
#120165=CARTESIAN_POINT('Ctrl Pts',(68.8561106303347,1078.37478862654,357.251176962716));
#120166=CARTESIAN_POINT('Ctrl Pts',(68.9929803058314,1078.36524410491,357.171936387957));
#120167=CARTESIAN_POINT('Ctrl Pts',(69.2401787937585,1078.34460608442,356.960049394559));
#120168=CARTESIAN_POINT('Ctrl Pts',(69.3452663176645,1078.33364968231,356.825841584997));
#120169=CARTESIAN_POINT('Ctrl Pts',(69.4961240041268,1078.31268843434,356.526205651141));
#120170=CARTESIAN_POINT('Ctrl Pts',(69.541194980926,1078.30287538035,356.364037485814));
#120171=CARTESIAN_POINT('Ctrl Pts',(69.5651287858941,1078.2865830692,356.047718379383));
#120172=CARTESIAN_POINT('Ctrl Pts',(69.5498492769712,1078.28000210315,355.896805757738));
#120173=CARTESIAN_POINT('Ctrl Pts',(69.4699812033245,1078.27021904016,355.616505019617));
#120174=CARTESIAN_POINT('Ctrl Pts',(69.4091767994855,1078.26689651899,355.48830280211));
#120175=CARTESIAN_POINT('Ctrl Pts',(69.3047154976682,1078.26463988305,355.338300271891));
#120176=CARTESIAN_POINT('Ctrl Pts',(69.2791342029159,1078.26426398515,355.305167754843));
#120177=CARTESIAN_POINT('Ctrl Pts',(69.2359820433617,1078.26389295801,355.254624979299));
#120178=CARTESIAN_POINT('Ctrl Pts',(69.219454788941,1078.26380487357,355.236365282305));
#120179=CARTESIAN_POINT('Ctrl Pts',(69.1879157711236,1078.26373353825,355.203485953658));
#120180=CARTESIAN_POINT('Ctrl Pts',(69.1730524688451,1078.26373657647,355.188735730667));
#120181=CARTESIAN_POINT('Ctrl Pts',(69.1393978101969,1078.26382249366,355.156942920723));
#120182=CARTESIAN_POINT('Ctrl Pts',(69.120447626172,1078.26392208629,355.140081602065));
#120183=CARTESIAN_POINT('Ctrl Pts',(69.0655988363193,1078.26435079336,355.094134514308));
#120184=CARTESIAN_POINT('Ctrl Pts',(69.0286061874164,1078.26480094747,355.06641895646));
#120185=CARTESIAN_POINT('Ctrl Pts',(68.8491710423865,1078.26770141377,354.946615701958));
#120186=CARTESIAN_POINT('Ctrl Pts',(68.6908265634068,1078.27225783199,354.881551543092));
#120187=CARTESIAN_POINT('Ctrl Pts',(68.3900923339753,1078.28398741261,354.823313845346));
#120188=CARTESIAN_POINT('Ctrl Pts',(68.2524605328724,1078.29040904682,354.819098072872));
#120189=CARTESIAN_POINT('Ctrl Pts',(67.9689162741077,1078.30566702941,354.856118564548));
#120190=CARTESIAN_POINT('Ctrl Pts',(67.8255586356722,1078.31455037641,354.901231276389));
#120191=CARTESIAN_POINT('Ctrl Pts',(67.551168832755,1078.33392323053,355.043992272885));
#120192=CARTESIAN_POINT('Ctrl Pts',(67.424251565182,1078.34431063248,355.144048758361));
#120193=CARTESIAN_POINT('Ctrl Pts',(67.2084156789855,1078.36520467754,355.392456335813));
#120194=CARTESIAN_POINT('Ctrl Pts',(67.1240363732813,1078.3754831245,355.540711432959));
#120195=CARTESIAN_POINT('Ctrl Pts',(67.0194583715021,1078.39379384599,355.857015045418));
#120196=CARTESIAN_POINT('Ctrl Pts',(66.9984817094128,1078.40171497849,356.021443183465));
#120197=CARTESIAN_POINT('Ctrl Pts',(67.0189659068121,1078.41399803443,356.332295928338));
#120198=CARTESIAN_POINT('Ctrl Pts',(67.0540164470797,1078.41855445889,356.476470869262));
#120199=CARTESIAN_POINT('Ctrl Pts',(67.1516738658537,1078.4238111331,356.700335628744));
#120200=CARTESIAN_POINT('Ctrl Pts',(67.2004345792778,1078.42527979935,356.784479161516));
#120201=CARTESIAN_POINT('Ctrl Pts',(67.279503240532,1078.42641945879,356.890874824266));
#120202=CARTESIAN_POINT('Ctrl Pts',(67.301934253527,1078.42663933128,356.918557511908));
#120203=CARTESIAN_POINT('Ctrl Pts',(67.3405656922861,1078.42685775384,356.962350020648));
#120204=CARTESIAN_POINT('Ctrl Pts',(67.3560918682947,1078.42690746137,356.979027758045));
#120205=CARTESIAN_POINT('Ctrl Pts',(67.3868844889647,1078.42693479388,357.010376653845));
#120206=CARTESIAN_POINT('Ctrl Pts',(67.4020859106746,1078.42691729389,357.025101223384));
#120207=CARTESIAN_POINT('Ctrl Pts',(67.4380042430564,1078.42680614552,357.058200851031));
#120208=CARTESIAN_POINT('Ctrl Pts',(67.4589671476937,1078.42669071757,357.076293039177));
#120209=CARTESIAN_POINT('Ctrl Pts',(67.5255308873736,1078.42617220858,357.130062458145));
#120210=CARTESIAN_POINT('Ctrl Pts',(67.5729821404391,1078.42559337644,357.163327385636));
#120211=CARTESIAN_POINT('Ctrl Pts',(67.6866109848778,1078.42374837165,357.231962589286));
#120212=CARTESIAN_POINT('Ctrl Pts',(67.7539742470069,1078.42233401632,357.264950568641));
#120213=CARTESIAN_POINT('Ctrl Pts',(67.9700757138016,1078.41683452277,357.348124314899));
#120214=CARTESIAN_POINT('Ctrl Pts',(68.1254001479995,1078.41156841368,357.376963678809));
#120215=CARTESIAN_POINT('Ctrl Pts',(68.282008024927,1078.40494025576,357.376958828466));
#120216=CARTESIAN_POINT('',(68.2819685228178,1076.28440570417,354.826070586806));
#120217=CARTESIAN_POINT('',(68.2819685228176,1067.7251047501,354.826070586806));
#120218=CARTESIAN_POINT('Ctrl Pts',(68.2828783104664,1076.40120959841,357.376958504597));
#120219=CARTESIAN_POINT('Ctrl Pts',(68.1139567583433,1076.40843995203,357.37707899814));
#120220=CARTESIAN_POINT('Ctrl Pts',(67.9466278649383,1076.41406505978,357.343639921872));
#120221=CARTESIAN_POINT('Ctrl Pts',(67.6339827215819,1076.42166979259,357.213131289088));
#120222=CARTESIAN_POINT('Ctrl Pts',(67.4919227930535,1076.4235606558,357.117102529378));
#120223=CARTESIAN_POINT('Ctrl Pts',(67.2537522745128,1076.42336444091,356.875047956837));
#120224=CARTESIAN_POINT('Ctrl Pts',(67.1600452959416,1076.42127982381,356.731479350378));
#120225=CARTESIAN_POINT('Ctrl Pts',(67.0346165639685,1076.4133081298,356.416836516397));
#120226=CARTESIAN_POINT('Ctrl Pts',(67.003877767371,1076.40751346596,356.24903397595));
#120227=CARTESIAN_POINT('Ctrl Pts',(67.0095239001937,1076.39276767705,355.911567035652));
#120228=CARTESIAN_POINT('Ctrl Pts',(67.0457543452616,1076.38396179721,355.745243186752));
#120229=CARTESIAN_POINT('Ctrl Pts',(67.1462960048837,1076.369313427,355.515147547741));
#120230=CARTESIAN_POINT('Ctrl Pts',(67.1866324669658,1076.36428440595,355.442869201086));
#120231=CARTESIAN_POINT('Ctrl Pts',(67.2808780688924,1076.35391284183,355.306878818267));
#120232=CARTESIAN_POINT('Ctrl Pts',(67.3346184608261,1076.34859344092,355.243520334193));
#120233=CARTESIAN_POINT('Ctrl Pts',(67.5156475588365,1076.33225853127,355.067994680925));
#120234=CARTESIAN_POINT('Ctrl Pts',(67.6594388532063,1076.3212403891,354.975512882304));
#120235=CARTESIAN_POINT('Ctrl Pts',(67.9730905331906,1076.30059636382,354.852750475746));
#120236=CARTESIAN_POINT('Ctrl Pts',(68.1396460975408,1076.29115894958,354.822999083903));
#120237=CARTESIAN_POINT('Ctrl Pts',(68.4744759275764,1076.27524404749,354.829635769033));
#120238=CARTESIAN_POINT('Ctrl Pts',(68.6394985229903,1076.2689190114,354.865816191403));
#120239=CARTESIAN_POINT('Ctrl Pts',(68.9457644325333,1076.26044482447,354.99970932176));
#120240=CARTESIAN_POINT('Ctrl Pts',(69.0840834178632,1076.25836832752,355.095915883548));
#120241=CARTESIAN_POINT('Ctrl Pts',(69.3155747813728,1076.25883093411,355.335910886107));
#120242=CARTESIAN_POINT('Ctrl Pts',(69.4065789781513,1076.26135484848,355.477237605242));
#120243=CARTESIAN_POINT('Ctrl Pts',(69.5291562007942,1076.27061731939,355.786853877496));
#120244=CARTESIAN_POINT('Ctrl Pts',(69.5595173346668,1076.27726386798,355.952136508149));
#120245=CARTESIAN_POINT('Ctrl Pts',(69.5550756438495,1076.29365984583,356.285321351552));
#120246=CARTESIAN_POINT('Ctrl Pts',(69.5201498404082,1076.30325476694,356.450019900906));
#120247=CARTESIAN_POINT('Ctrl Pts',(69.3888204583184,1076.32396004204,356.756926860179));
#120248=CARTESIAN_POINT('Ctrl Pts',(69.2935198658765,1076.33487293518,356.896147746133));
#120249=CARTESIAN_POINT('Ctrl Pts',(69.0530584958274,1076.35661504826,357.131498335221));
#120250=CARTESIAN_POINT('Ctrl Pts',(68.9095899511603,1076.36722761946,357.2247075545));
#120251=CARTESIAN_POINT('Ctrl Pts',(68.602778087315,1076.3861212556,357.346356448884));
#120252=CARTESIAN_POINT('Ctrl Pts',(68.4435885401786,1076.39433071424,357.376843868278));
#120253=CARTESIAN_POINT('Ctrl Pts',(68.2828783104664,1076.40120959841,357.376958504597));
#120254=CARTESIAN_POINT('Origin',(68.2819685228176,1067.7251047501,356.101514707942));
#120255=CARTESIAN_POINT('',(68.2819685228176,1076.37545952532,356.776958829078));
#120256=CARTESIAN_POINT('',(68.2819685228177,1076.31358867648,355.426070586806));
#120257=CARTESIAN_POINT('Ctrl Pts',(68.2819685228176,1076.37545952532,356.776958829078));
#120258=CARTESIAN_POINT('Ctrl Pts',(68.2814488826747,1076.37548245635,356.776958829078));
#120259=CARTESIAN_POINT('Ctrl Pts',(68.2809292117553,1076.37550536127,356.776958229415));
#120260=CARTESIAN_POINT('Ctrl Pts',(68.1905059800451,1076.3794860582,356.776749520431));
#120261=CARTESIAN_POINT('Ctrl Pts',(68.1015116578338,1076.38258242533,356.758594310527));
#120262=CARTESIAN_POINT('Ctrl Pts',(67.9364242674877,1076.38672767774,356.688710918134));
#120263=CARTESIAN_POINT('Ctrl Pts',(67.8618880002053,1076.38775102954,356.637925606172));
#120264=CARTESIAN_POINT('Ctrl Pts',(67.7375745412074,1076.38761756947,356.510983791035));
#120265=CARTESIAN_POINT('Ctrl Pts',(67.6887506463528,1076.38648584552,356.436354826076));
#120266=CARTESIAN_POINT('Ctrl Pts',(67.6219904881311,1076.38215781662,356.271057086154));
#120267=CARTESIAN_POINT('Ctrl Pts',(67.6053146123236,1076.37896661029,356.181789805928));
#120268=CARTESIAN_POINT('Ctrl Pts',(67.6078691598746,1076.37089386361,356.002143801593));
#120269=CARTESIAN_POINT('Ctrl Pts',(67.627028665527,1076.36609359528,355.913560241435));
#120270=CARTESIAN_POINT('Ctrl Pts',(67.680475129787,1076.35818119408,355.791098857711));
#120271=CARTESIAN_POINT('Ctrl Pts',(67.7019159684127,1076.35547748858,355.752673156844));
#120272=CARTESIAN_POINT('Ctrl Pts',(67.7519892924917,1076.34993029553,355.68046763933));
#120273=CARTESIAN_POINT('Ctrl Pts',(67.7805173901468,1076.34709959059,355.646866496652));
#120274=CARTESIAN_POINT('Ctrl Pts',(67.8770853906298,1076.33840108898,355.553358074326));
#120275=CARTESIAN_POINT('Ctrl Pts',(67.954054961846,1076.33257086589,355.504117765021));
#120276=CARTESIAN_POINT('Ctrl Pts',(68.1160982976483,1076.32211248113,355.441482222345));
#120277=CARTESIAN_POINT('Ctrl Pts',(68.1986617481032,1076.31751514527,355.426070586806));
#120278=CARTESIAN_POINT('Ctrl Pts',(68.2819685228178,1076.31358867648,355.426070586806));
#120279=CARTESIAN_POINT('',(68.2819685228176,1082.7251047501,355.426070586806));
#120280=CARTESIAN_POINT('',(68.2819685228176,1067.7251047501,355.426070586806));
#120281=CARTESIAN_POINT('Origin',(68.2819685228176,1082.7251047501,356.101514707942));
#120282=CARTESIAN_POINT('Ctrl Pts',(68.2819685228178,1076.31358867648,355.426070586806));
#120283=CARTESIAN_POINT('Ctrl Pts',(68.2820960517956,1076.3135826657,355.426070586806));
#120284=CARTESIAN_POINT('Ctrl Pts',(68.2822235825154,1076.3135766565,355.426070622914));
#120285=CARTESIAN_POINT('Ctrl Pts',(68.2823511149623,1076.31357064887,355.426070695152));
#120286=CARTESIAN_POINT('Ctrl Pts',(68.3708482950225,1076.30940184007,355.426120822646));
#120287=CARTESIAN_POINT('Ctrl Pts',(68.4585121162839,1076.30607015087,355.443562902922));
#120288=CARTESIAN_POINT('Ctrl Pts',(68.6219598404336,1076.30152420804,355.51123144722));
#120289=CARTESIAN_POINT('Ctrl Pts',(68.6961761521499,1076.30034993916,355.560713989813));
#120290=CARTESIAN_POINT('Ctrl Pts',(68.8212687860782,1076.30035029981,355.685381908252));
#120291=CARTESIAN_POINT('Ctrl Pts',(68.8709521077544,1076.30152159786,355.759309061297));
#120292=CARTESIAN_POINT('Ctrl Pts',(68.9391073604367,1076.30605164107,355.92210943135));
#120293=CARTESIAN_POINT('Ctrl Pts',(68.9568921450285,1076.30936685706,356.009404789735));
#120294=CARTESIAN_POINT('Ctrl Pts',(68.957911846463,1076.31767337057,356.186036349548));
#120295=CARTESIAN_POINT('Ctrl Pts',(68.9410550673682,1076.3225870389,356.273669451315));
#120296=CARTESIAN_POINT('Ctrl Pts',(68.8745184277081,1076.33332184607,356.437597389258));
#120297=CARTESIAN_POINT('Ctrl Pts',(68.8254035959997,1076.33904115829,356.512296353457));
#120298=CARTESIAN_POINT('Ctrl Pts',(68.7001941369294,1076.35058538137,356.639474188949));
#120299=CARTESIAN_POINT('Ctrl Pts',(68.6249180721111,1076.35629672746,356.690330819141));
#120300=CARTESIAN_POINT('Ctrl Pts',(68.4595535166777,1076.36681187013,356.759271270782));
#120301=CARTESIAN_POINT('Ctrl Pts',(68.3712149398878,1076.37152119931,356.776958829078));
#120302=CARTESIAN_POINT('Ctrl Pts',(68.2819685228176,1076.37545952532,356.776958829078));
#120303=CARTESIAN_POINT('Origin',(81.8208965804709,1067.7251047501,359.019679174786));
#120304=CARTESIAN_POINT('',(81.8208965804941,1077.59408165984,357.920848038793));
#120305=CARTESIAN_POINT('Ctrl Pts',(81.8210035103925,1077.7359053691,360.118510305575));
#120306=CARTESIAN_POINT('Ctrl Pts',(81.9496451149812,1077.72579923846,360.118497787149));
#120307=CARTESIAN_POINT('Ctrl Pts',(82.0771867011425,1077.71429950911,360.095896627786));
#120308=CARTESIAN_POINT('Ctrl Pts',(82.3281251504515,1077.68850385192,360.004253756816));
#120309=CARTESIAN_POINT('Ctrl Pts',(82.4481865036554,1077.67428181328,359.932450106309));
#120310=CARTESIAN_POINT('Ctrl Pts',(82.6606388749049,1077.64490797405,359.743242171231));
#120311=CARTESIAN_POINT('Ctrl Pts',(82.7492199475112,1077.63002722378,359.625452369551));
#120312=CARTESIAN_POINT('Ctrl Pts',(82.8731938158463,1077.60287609857,359.366210021708));
#120313=CARTESIAN_POINT('Ctrl Pts',(82.9090582715662,1077.59078693907,359.227983574739));
#120314=CARTESIAN_POINT('Ctrl Pts',(82.9251667013517,1077.5719472468,358.964074781048));
#120315=CARTESIAN_POINT('Ctrl Pts',(82.9120606293678,1077.56483506721,358.841034095682));
#120316=CARTESIAN_POINT('Ctrl Pts',(82.853763293938,1077.55582794555,358.633407710144));
#120317=CARTESIAN_POINT('Ctrl Pts',(82.8175121955166,1077.55311661812,358.547673633375));
#120318=CARTESIAN_POINT('Ctrl Pts',(82.7555063823544,1077.55115313016,358.440996830497));
#120319=CARTESIAN_POINT('Ctrl Pts',(82.7390063568056,1077.55080121932,358.415160050793));
#120320=CARTESIAN_POINT('Ctrl Pts',(82.7107543559653,1077.55045507672,358.374751864592));
#120321=CARTESIAN_POINT('Ctrl Pts',(82.6996735929003,1077.55037484604,358.359732907036));
#120322=CARTESIAN_POINT('Ctrl Pts',(82.6779419959406,1077.5503191592,358.33179619459));
#120323=CARTESIAN_POINT('Ctrl Pts',(82.6673680872842,1077.55033373728,358.318825534113));
#120324=CARTESIAN_POINT('Ctrl Pts',(82.6428038034306,1077.55045913375,358.290060551153));
#120325=CARTESIAN_POINT('Ctrl Pts',(82.6286466693954,1077.55059402165,358.27441775756));
#120326=CARTESIAN_POINT('Ctrl Pts',(82.5852591569209,1077.55118740004,358.229166628975));
#120327=CARTESIAN_POINT('Ctrl Pts',(82.5547908274227,1077.55183251712,358.20080260558));
#120328=CARTESIAN_POINT('Ctrl Pts',(82.4106550737012,1077.55585407554,358.08113972463));
#120329=CARTESIAN_POINT('Ctrl Pts',(82.2812029852015,1077.56198574477,358.011350846977));
#120330=CARTESIAN_POINT('Ctrl Pts',(82.0291910157458,1077.57777641674,357.934338306733));
#120331=CARTESIAN_POINT('Ctrl Pts',(81.9116317904677,1077.5864420575,357.918283630983));
#120332=CARTESIAN_POINT('Ctrl Pts',(81.6650306041736,1077.60714755689,357.924349784796));
#120333=CARTESIAN_POINT('Ctrl Pts',(81.5378381430728,1077.61926818079,357.950159267881));
#120334=CARTESIAN_POINT('Ctrl Pts',(81.2890745397625,1077.64591669128,358.048172727042));
#120335=CARTESIAN_POINT('Ctrl Pts',(81.1708569576794,1077.66032572816,358.122964382053));
#120336=CARTESIAN_POINT('Ctrl Pts',(80.9632831192145,1077.68950104246,358.317409025053));
#120337=CARTESIAN_POINT('Ctrl Pts',(80.8777158067086,1077.70396833387,358.437319646737));
#120338=CARTESIAN_POINT('Ctrl Pts',(80.7603979468685,1077.72985602794,358.699258395091));
#120339=CARTESIAN_POINT('Ctrl Pts',(80.7280108804241,1077.74112813057,358.838017680069));
#120340=CARTESIAN_POINT('Ctrl Pts',(80.7182084206833,1077.75856839595,359.10417984325));
#120341=CARTESIAN_POINT('Ctrl Pts',(80.7349613879902,1077.7650481351,359.229086414236));
#120342=CARTESIAN_POINT('Ctrl Pts',(80.7976633685545,1077.77261700745,359.428981992576));
#120343=CARTESIAN_POINT('Ctrl Pts',(80.8320695343832,1077.77474977431,359.506263043289));
#120344=CARTESIAN_POINT('Ctrl Pts',(80.8898797516962,1077.77634355938,359.60405389632));
#120345=CARTESIAN_POINT('Ctrl Pts',(80.9057719866548,1077.77663908646,359.628639984643));
#120346=CARTESIAN_POINT('Ctrl Pts',(80.9331332808851,1077.77693110665,359.667474600064));
#120347=CARTESIAN_POINT('Ctrl Pts',(80.9440090002506,1077.77699826099,359.682122209562));
#120348=CARTESIAN_POINT('Ctrl Pts',(80.9654900791558,1077.77704056504,359.709596764533));
#120349=CARTESIAN_POINT('Ctrl Pts',(80.9760319875259,1077.77702329249,359.722466753914));
#120350=CARTESIAN_POINT('Ctrl Pts',(81.0007632700304,1077.77689835445,359.751298684624));
#120351=CARTESIAN_POINT('Ctrl Pts',(81.0151337479807,1077.77676647162,359.767096047392));
#120352=CARTESIAN_POINT('Ctrl Pts',(81.0600518878109,1077.77618036699,359.813672225824));
#120353=CARTESIAN_POINT('Ctrl Pts',(81.0919668509945,1077.77553457729,359.843068768853));
#120354=CARTESIAN_POINT('Ctrl Pts',(81.1684310725808,1077.77349360069,359.905561940639));
#120355=CARTESIAN_POINT('Ctrl Pts',(81.2139123191459,1077.77194299733,359.937321360241));
#120356=CARTESIAN_POINT('Ctrl Pts',(81.3532701792501,1077.76625859978,360.019729940068));
#120357=CARTESIAN_POINT('Ctrl Pts',(81.4522984247743,1077.76109302637,360.060296548066));
#120358=CARTESIAN_POINT('Ctrl Pts',(81.6424277467173,1077.74921977244,360.107610906314));
#120359=CARTESIAN_POINT('Ctrl Pts',(81.7315768295082,1077.74293076125,360.118519007902));
#120360=CARTESIAN_POINT('Ctrl Pts',(81.8210035103925,1077.7359053691,360.118510305575));
#120361=CARTESIAN_POINT('',(81.8208965804711,1075.58250670589,357.920848038793));
#120362=CARTESIAN_POINT('',(81.8208965804709,1067.7251047501,357.920848038793));
#120363=CARTESIAN_POINT('Ctrl Pts',(81.8203364796409,1075.72568197611,360.11851016803));
#120364=CARTESIAN_POINT('Ctrl Pts',(81.6748513000131,1075.73721127236,360.118436010702));
#120365=CARTESIAN_POINT('Ctrl Pts',(81.5306805462196,1075.74672849855,360.089469144153));
#120366=CARTESIAN_POINT('Ctrl Pts',(81.2618461305948,1075.76073707659,359.976824306072));
#120367=CARTESIAN_POINT('Ctrl Pts',(81.1399103591242,1075.7650899466,359.894302916234));
#120368=CARTESIAN_POINT('Ctrl Pts',(80.9352730099284,1075.768047685,359.686305972091));
#120369=CARTESIAN_POINT('Ctrl Pts',(80.8546944157296,1075.76662105825,359.562964091174));
#120370=CARTESIAN_POINT('Ctrl Pts',(80.7464431802241,1075.75810450695,359.292141971266));
#120371=CARTESIAN_POINT('Ctrl Pts',(80.7198546155749,1075.75110285212,359.147451758713));
#120372=CARTESIAN_POINT('Ctrl Pts',(80.7245685152145,1075.73231752799,358.856066705015));
#120373=CARTESIAN_POINT('Ctrl Pts',(80.7559361766191,1075.72071042844,358.71230042189));
#120374=CARTESIAN_POINT('Ctrl Pts',(80.873125219009,1075.69423688013,358.444657028142));
#120375=CARTESIAN_POINT('Ctrl Pts',(80.9581686919438,1075.67960707372,358.32356797675));
#120376=CARTESIAN_POINT('Ctrl Pts',(81.1165287884067,1075.65702132493,358.173233928333));
#120377=CARTESIAN_POINT('Ctrl Pts',(81.1734298595951,1075.64951009384,358.128954821535));
#120378=CARTESIAN_POINT('Ctrl Pts',(81.3578182002398,1075.62685045887,358.012531732351));
#120379=CARTESIAN_POINT('Ctrl Pts',(81.4957887389163,1075.61203371471,357.959897319903));
#120380=CARTESIAN_POINT('Ctrl Pts',(81.7826337015554,1075.58512819763,357.912046817121));
#120381=CARTESIAN_POINT('Ctrl Pts',(81.9286185636597,1075.57326760528,357.91659604885));
#120382=CARTESIAN_POINT('Ctrl Pts',(82.2098166212493,1075.5541349373,357.981952412458));
#120383=CARTESIAN_POINT('Ctrl Pts',(82.3423401505379,1075.54702471785,358.041772051681));
#120384=CARTESIAN_POINT('Ctrl Pts',(82.5761994330248,1075.53861721898,358.20883287706));
#120385=CARTESIAN_POINT('Ctrl Pts',(82.6753882754589,1075.53737025829,358.314121354662));
#120386=CARTESIAN_POINT('Ctrl Pts',(82.8276040985836,1075.54092604795,358.55662369521));
#120387=CARTESIAN_POINT('Ctrl Pts',(82.879210882916,1075.54567967013,358.691347940956));
#120388=CARTESIAN_POINT('Ctrl Pts',(82.9280594719914,1075.56054356659,358.973272901754));
#120389=CARTESIAN_POINT('Ctrl Pts',(82.9246469618963,1075.57052259812,359.117740886092));
#120390=CARTESIAN_POINT('Ctrl Pts',(82.8625822165472,1075.59435807866,359.397878520871));
#120391=CARTESIAN_POINT('Ctrl Pts',(82.8041739820782,1075.60800756338,359.530800078522));
#120392=CARTESIAN_POINT('Ctrl Pts',(82.6806331736267,1075.62980163666,359.707782908721));
#120393=CARTESIAN_POINT('Ctrl Pts',(82.6336243995114,1075.63725178508,359.762716196854));
#120394=CARTESIAN_POINT('Ctrl Pts',(82.5295312429813,1075.65226318573,359.862572687651));
#120395=CARTESIAN_POINT('Ctrl Pts',(82.4726866690676,1075.65978957021,359.907261992778));
#120396=CARTESIAN_POINT('Ctrl Pts',(82.2884884512699,1075.68231542504,360.02476940505));
#120397=CARTESIAN_POINT('Ctrl Pts',(82.1505373258723,1075.69681693572,360.078092773233));
#120398=CARTESIAN_POINT('Ctrl Pts',(81.9447607738923,1075.71547192738,360.11327867515));
#120399=CARTESIAN_POINT('Ctrl Pts',(81.8826168770904,1075.72074642765,360.11854191386));
#120400=CARTESIAN_POINT('Ctrl Pts',(81.8203364796409,1075.72568197611,360.11851016803));
#120401=CARTESIAN_POINT('Origin',(81.8208965804709,1067.7251047501,359.019679174786));
#120402=CARTESIAN_POINT('',(81.8208965804709,1075.68770968364,359.518510310778));
#120403=CARTESIAN_POINT('',(81.8208965804708,1075.62273721903,358.520848038793));
#120404=CARTESIAN_POINT('Ctrl Pts',(81.8208965804709,1075.68770968364,359.518510310778));
#120405=CARTESIAN_POINT('Ctrl Pts',(81.7879945785618,1075.6903532399,359.518510310778));
#120406=CARTESIAN_POINT('Ctrl Pts',(81.7550763799472,1075.69278479065,359.515255218438));
#120407=CARTESIAN_POINT('Ctrl Pts',(81.6575716992867,1075.69934037109,359.495663082824));
#120408=CARTESIAN_POINT('Ctrl Pts',(81.5957192253617,1075.70262161683,359.46972951162));
#120409=CARTESIAN_POINT('Ctrl Pts',(81.4863399484057,1075.70660325775,359.395478948915));
#120410=CARTESIAN_POINT('Ctrl Pts',(81.4397720828946,1075.70729150202,359.348162169015));
#120411=CARTESIAN_POINT('Ctrl Pts',(81.3680599741735,1075.70601502793,359.238772116286));
#120412=CARTESIAN_POINT('Ctrl Pts',(81.343401036283,1075.70409193481,359.177956954028));
#120413=CARTESIAN_POINT('Ctrl Pts',(81.3185003947358,1075.69780607712,359.048870127068));
#120414=CARTESIAN_POINT('Ctrl Pts',(81.3190988368862,1075.69345140553,358.981783870762));
#120415=CARTESIAN_POINT('Ctrl Pts',(81.3465173653583,1075.68286651085,358.85164093288));
#120416=CARTESIAN_POINT('Ctrl Pts',(81.3731663997571,1075.67673446555,358.7899068656));
#120417=CARTESIAN_POINT('Ctrl Pts',(81.4296859052742,1075.66688857504,358.708472190585));
#120418=CARTESIAN_POINT('Ctrl Pts',(81.4508538977159,1075.66355900733,358.683579325378));
#120419=CARTESIAN_POINT('Ctrl Pts',(81.4977877577823,1075.65680419623,358.638233899828));
#120420=CARTESIAN_POINT('Ctrl Pts',(81.5234558602621,1075.65339438285,358.61789717551));
#120421=CARTESIAN_POINT('Ctrl Pts',(81.6067070831681,1075.64312404903,358.564315958701));
#120422=CARTESIAN_POINT('Ctrl Pts',(81.6691226552038,1075.63642650157,358.539880240271));
#120423=CARTESIAN_POINT('Ctrl Pts',(81.7629342065803,1075.62766038669,358.523388114674));
#120424=CARTESIAN_POINT('Ctrl Pts',(81.7917338964536,1075.62513259164,358.520865178427));
#120425=CARTESIAN_POINT('Ctrl Pts',(81.8206019166418,1075.62276141663,358.520848125837));
#120426=CARTESIAN_POINT('Ctrl Pts',(81.8207001391889,1075.62275334878,358.520848067817));
#120427=CARTESIAN_POINT('Ctrl Pts',(81.8207983604694,1075.62274528291,358.520848038793));
#120428=CARTESIAN_POINT('Ctrl Pts',(81.8208965804707,1075.62273721903,358.520848038793));
#120429=CARTESIAN_POINT('',(81.8208965804709,1082.7251047501,358.520848038793));
#120430=CARTESIAN_POINT('',(81.8208965804709,1067.7251047501,358.520848038793));
#120431=CARTESIAN_POINT('Origin',(81.8208965804709,1082.7251047501,359.019679174786));
#120432=CARTESIAN_POINT('Ctrl Pts',(81.8208965804707,1075.62273721903,358.520848038793));
#120433=CARTESIAN_POINT('Ctrl Pts',(81.886228206205,1075.61737347788,358.520848038793));
#120434=CARTESIAN_POINT('Ctrl Pts',(81.9509939035222,1075.61288729907,358.533682714537));
#120435=CARTESIAN_POINT('Ctrl Pts',(82.0717020651763,1075.60623432872,358.583589329763));
#120436=CARTESIAN_POINT('Ctrl Pts',(82.1264928596674,1075.60412300937,358.620056055585));
#120437=CARTESIAN_POINT('Ctrl Pts',(82.2187957612182,1075.60258075092,358.711895613239));
#120438=CARTESIAN_POINT('Ctrl Pts',(82.255453124008,1075.60315492614,358.766277803405));
#120439=CARTESIAN_POINT('Ctrl Pts',(82.3058747440072,1075.60692094092,358.886058668206));
#120440=CARTESIAN_POINT('Ctrl Pts',(82.3191209577567,1075.61007699176,358.950275056747));
#120441=CARTESIAN_POINT('Ctrl Pts',(82.3202966963971,1075.61856836367,359.080395035986));
#120442=CARTESIAN_POINT('Ctrl Pts',(82.308088585028,1075.6238310256,359.145035623558));
#120443=CARTESIAN_POINT('Ctrl Pts',(82.2594537562011,1075.63577470265,359.266234841303));
#120444=CARTESIAN_POINT('Ctrl Pts',(82.2233441044727,1075.64234981651,359.321587259796));
#120445=CARTESIAN_POINT('Ctrl Pts',(82.154738941984,1075.65251450466,359.391771376562));
#120446=CARTESIAN_POINT('Ctrl Pts',(82.1296175665403,1075.65593017312,359.412864444856));
#120447=CARTESIAN_POINT('Ctrl Pts',(82.0475879396677,1075.66623581512,359.468999918754));
#120448=CARTESIAN_POINT('Ctrl Pts',(81.9855377649109,1075.67295302678,359.495264246264));
#120449=CARTESIAN_POINT('Ctrl Pts',(81.8873987449316,1075.68214848607,359.515183930342));
#120450=CARTESIAN_POINT('Ctrl Pts',(81.8541559389162,1075.68503741509,359.518510310778));
#120451=CARTESIAN_POINT('Ctrl Pts',(81.8208965804709,1075.68770968364,359.518510310778));
#120452=CARTESIAN_POINT('Origin',(94.6032580293201,1067.7251047501,364.698164080197));
#120453=CARTESIAN_POINT('',(94.603258029345,1076.74090351967,363.607623331469));
#120454=CARTESIAN_POINT('Ctrl Pts',(94.6034039085428,1076.89760555679,365.788704819168));
#120455=CARTESIAN_POINT('Ctrl Pts',(94.7345715164352,1076.88291957311,365.788687273167));
#120456=CARTESIAN_POINT('Ctrl Pts',(94.8645131843872,1076.86663458984,365.765007633727));
#120457=CARTESIAN_POINT('Ctrl Pts',(95.1194451714134,1076.8310043412,365.669165482204));
#120458=CARTESIAN_POINT('Ctrl Pts',(95.2409065605302,1076.81183546033,365.594092782859));
#120459=CARTESIAN_POINT('Ctrl Pts',(95.4504462837096,1076.77394048259,365.399853698011));
#120460=CARTESIAN_POINT('Ctrl Pts',(95.5358649587737,1076.75558261267,365.281629155982));
#120461=CARTESIAN_POINT('Ctrl Pts',(95.6520812154778,1076.72364186116,365.026360743801));
#120462=CARTESIAN_POINT('Ctrl Pts',(95.6848675699349,1076.71011204164,364.893053069973));
#120463=CARTESIAN_POINT('Ctrl Pts',(95.6993864053341,1076.68872730221,364.62404129982));
#120464=CARTESIAN_POINT('Ctrl Pts',(95.6821801915352,1076.68093172327,364.490785253847));
#120465=CARTESIAN_POINT('Ctrl Pts',(95.625009822732,1076.67452023046,364.313305550669));
#120466=CARTESIAN_POINT('Ctrl Pts',(95.6050800208169,1076.67321231869,364.264057828994));
#120467=CARTESIAN_POINT('Ctrl Pts',(95.5715298011371,1076.67209630214,364.195916599161));
#120468=CARTESIAN_POINT('Ctrl Pts',(95.560777705991,1076.67185854829,364.175709371293));
#120469=CARTESIAN_POINT('Ctrl Pts',(95.5422287287133,1076.67163221522,364.143347936837));
#120470=CARTESIAN_POINT('Ctrl Pts',(95.5348128341495,1076.67158400599,364.130984582994));
#120471=CARTESIAN_POINT('Ctrl Pts',(95.5187805069463,1076.67156534444,364.105419519539));
#120472=CARTESIAN_POINT('Ctrl Pts',(95.5101186477741,1076.67160256858,364.092250443705));
#120473=CARTESIAN_POINT('Ctrl Pts',(95.4889328370921,1076.67180192759,364.06151302807));
#120474=CARTESIAN_POINT('Ctrl Pts',(95.4761673802746,1076.67200500754,364.044120026008));
#120475=CARTESIAN_POINT('Ctrl Pts',(95.4326666278011,1076.67295764359,363.988393840474));
#120476=CARTESIAN_POINT('Ctrl Pts',(95.3998624117891,1076.67407276017,363.951764783842));
#120477=CARTESIAN_POINT('Ctrl Pts',(95.2610071374953,1076.68023247673,363.816330678941));
#120478=CARTESIAN_POINT('Ctrl Pts',(95.1383344063074,1076.68863564959,363.736994062286));
#120479=CARTESIAN_POINT('Ctrl Pts',(94.8940154330133,1076.70981701248,363.640471722811));
#120480=CARTESIAN_POINT('Ctrl Pts',(94.7779025299033,1076.72137604043,363.615263249293));
#120481=CARTESIAN_POINT('Ctrl Pts',(94.5312467376063,1076.74880671727,363.602370560171));
#120482=CARTESIAN_POINT('Ctrl Pts',(94.4022859908853,1076.76477130994,363.618587666129));
#120483=CARTESIAN_POINT('Ctrl Pts',(94.1464455761988,1076.79973329141,363.69818720285));
#120484=CARTESIAN_POINT('Ctrl Pts',(94.0227620182876,1076.81856805543,363.764545231607));
#120485=CARTESIAN_POINT('Ctrl Pts',(93.8025779388021,1076.85631439853,363.94373611102));
#120486=CARTESIAN_POINT('Ctrl Pts',(93.7094662193629,1076.87484481459,364.05670241198));
#120487=CARTESIAN_POINT('Ctrl Pts',(93.5758711658185,1076.90758767687,364.307041190962));
#120488=CARTESIAN_POINT('Ctrl Pts',(93.5344142658805,1076.92166706804,364.440881622791));
#120489=CARTESIAN_POINT('Ctrl Pts',(93.5055131619185,1076.94342908994,364.704071881101));
#120490=CARTESIAN_POINT('Ctrl Pts',(93.5134809992833,1076.95143159331,364.830604631922));
#120491=CARTESIAN_POINT('Ctrl Pts',(93.5600296450457,1076.95985923957,365.02420022273));
#120492=CARTESIAN_POINT('Ctrl Pts',(93.5842352256024,1076.96203225347,365.093417911572));
#120493=CARTESIAN_POINT('Ctrl Pts',(93.6263102562109,1076.96368941769,365.183489651022));
#120494=CARTESIAN_POINT('Ctrl Pts',(93.6382727170041,1076.96400364626,365.206859832407));
#120495=CARTESIAN_POINT('Ctrl Pts',(93.6591888633484,1076.96431490137,365.244323484867));
#120496=CARTESIAN_POINT('Ctrl Pts',(93.6676426918722,1076.96438582107,365.258682270905));
#120497=CARTESIAN_POINT('Ctrl Pts',(93.6845445728684,1076.96442611252,365.285941486676));
#120498=CARTESIAN_POINT('Ctrl Pts',(93.6929436471067,1076.96440268446,365.298867349726));
#120499=CARTESIAN_POINT('Ctrl Pts',(93.7129282675081,1076.96425008642,365.328240751172));
#120500=CARTESIAN_POINT('Ctrl Pts',(93.7247003152812,1076.96409087818,365.344554052353));
#120501=CARTESIAN_POINT('Ctrl Pts',(93.7624725316358,1076.96337400637,365.393958078733));
#120502=CARTESIAN_POINT('Ctrl Pts',(93.7899381971193,1076.96257174082,365.4258724012));
#120503=CARTESIAN_POINT('Ctrl Pts',(93.9196394980028,1076.95762238231,365.5600453961));
#120504=CARTESIAN_POINT('Ctrl Pts',(94.0396461207868,1076.95014294675,365.642843885717));
#120505=CARTESIAN_POINT('Ctrl Pts',(94.2465145052762,1076.93342147644,365.73188247013));
#120506=CARTESIAN_POINT('Ctrl Pts',(94.32417754157,1076.92644267633,365.755485767671));
#120507=CARTESIAN_POINT('Ctrl Pts',(94.4695833862916,1076.91213653877,365.782556602382));
#120508=CARTESIAN_POINT('Ctrl Pts',(94.5364491625008,1076.9051020441,365.788713775556));
#120509=CARTESIAN_POINT('Ctrl Pts',(94.6034039085428,1076.89760555679,365.788704819168));
#120510=CARTESIAN_POINT('',(94.6032580293202,1074.72198576327,363.607623331468));
#120511=CARTESIAN_POINT('',(94.6032580293201,1067.7251047501,363.607623331468));
#120512=CARTESIAN_POINT('Ctrl Pts',(94.6024843825279,1074.88008894717,365.788704554506));
#120513=CARTESIAN_POINT('Ctrl Pts',(94.4580905763941,1074.89638168322,365.788602119239));
#120514=CARTESIAN_POINT('Ctrl Pts',(94.3149041808003,1074.91041844163,365.759822716901));
#120515=CARTESIAN_POINT('Ctrl Pts',(94.0478148968823,1074.93239665398,365.647754598289));
#120516=CARTESIAN_POINT('Ctrl Pts',(93.9266353324091,1074.94011908936,365.565643651049));
#120517=CARTESIAN_POINT('Ctrl Pts',(93.7257672460261,1074.94807140394,365.360998186142));
#120518=CARTESIAN_POINT('Ctrl Pts',(93.6471830436114,1074.94839699918,365.24154621693));
#120519=CARTESIAN_POINT('Ctrl Pts',(93.5399736185817,1074.94180138391,364.978981084259));
#120520=CARTESIAN_POINT('Ctrl Pts',(93.5125448378681,1074.93493078036,364.83848532818));
#120521=CARTESIAN_POINT('Ctrl Pts',(93.5128953027451,1074.9145632267,364.551947282319));
#120522=CARTESIAN_POINT('Ctrl Pts',(93.5419373637495,1074.90112683102,364.408801334487));
#120523=CARTESIAN_POINT('Ctrl Pts',(93.6540884616984,1074.86941262532,364.14192291546));
#120524=CARTESIAN_POINT('Ctrl Pts',(93.7363418777446,1074.85142241365,364.020906732474));
#120525=CARTESIAN_POINT('Ctrl Pts',(93.943818278137,1074.81314300848,363.81742414112));
#120526=CARTESIAN_POINT('Ctrl Pts',(94.0674115956666,1074.7931995908,363.737215533729));
#120527=CARTESIAN_POINT('Ctrl Pts',(94.3382107013227,1074.75430992866,363.630397256631));
#120528=CARTESIAN_POINT('Ctrl Pts',(94.4827771833473,1074.73572547102,363.604566296967));
#120529=CARTESIAN_POINT('Ctrl Pts',(94.771631845205,1074.70273517309,363.611205121975));
#120530=CARTESIAN_POINT('Ctrl Pts',(94.9131470606423,1074.68858566121,363.642731415956));
#120531=CARTESIAN_POINT('Ctrl Pts',(95.1748321497686,1074.66662099108,363.75856755272));
#120532=CARTESIAN_POINT('Ctrl Pts',(95.2926172799575,1074.65896115871,363.841179675866));
#120533=CARTESIAN_POINT('Ctrl Pts',(95.4891311884377,1074.65118912929,364.046586066743));
#120534=CARTESIAN_POINT('Ctrl Pts',(95.5661545114112,1074.65109939044,364.166979738535));
#120535=CARTESIAN_POINT('Ctrl Pts',(95.6698641777838,1074.65849322358,364.430451950522));
#120536=CARTESIAN_POINT('Ctrl Pts',(95.6955094012144,1074.66589885394,364.57084618374));
#120537=CARTESIAN_POINT('Ctrl Pts',(95.6918976183761,1074.68726700068,364.854330615544));
#120538=CARTESIAN_POINT('Ctrl Pts',(95.6622668743928,1074.70106418117,364.994624476514));
#120539=CARTESIAN_POINT('Ctrl Pts',(95.5506493052697,1074.73326922215,365.256968123332));
#120540=CARTESIAN_POINT('Ctrl Pts',(95.4691819321429,1074.75141521818,365.37631789352));
#120541=CARTESIAN_POINT('Ctrl Pts',(95.3160734736272,1074.77995980457,365.526594003809));
#120542=CARTESIAN_POINT('Ctrl Pts',(95.2601887561047,1074.7896376246,365.57157168583));
#120543=CARTESIAN_POINT('Ctrl Pts',(95.1406646726612,1074.80898201746,365.649770123526));
#120544=CARTESIAN_POINT('Ctrl Pts',(95.0773227458251,1074.81860525188,365.682860159408));
#120545=CARTESIAN_POINT('Ctrl Pts',(94.8814544432978,1074.84661074313,365.761863484231));
#120546=CARTESIAN_POINT('Ctrl Pts',(94.7427005524783,1074.86426759646,365.788804026092));
#120547=CARTESIAN_POINT('Ctrl Pts',(94.602484382528,1074.88008894717,365.788704554506));
#120548=CARTESIAN_POINT('Origin',(94.6032580293201,1067.7251047501,364.698164080197));
#120549=CARTESIAN_POINT('',(94.6032580293201,1074.83751173097,365.188704828925));
#120550=CARTESIAN_POINT('',(94.6032580293198,1074.76643751182,364.207623331468));
#120551=CARTESIAN_POINT('Ctrl Pts',(94.6032580293201,1074.83751173097,365.188704828925));
#120552=CARTESIAN_POINT('Ctrl Pts',(94.5389061106776,1074.84482891857,365.188704828925));
#120553=CARTESIAN_POINT('Ctrl Pts',(94.4750626242078,1074.85116271567,365.176041667615));
#120554=CARTESIAN_POINT('Ctrl Pts',(94.355799041386,1074.86113145739,365.126600282273));
#120555=CARTESIAN_POINT('Ctrl Pts',(94.301577574366,1074.86466829042,365.090341076152));
#120556=CARTESIAN_POINT('Ctrl Pts',(94.2109220617968,1074.86841034894,364.999429988502));
#120557=CARTESIAN_POINT('Ctrl Pts',(94.1751501476945,1074.86862713673,364.945981842153));
#120558=CARTESIAN_POINT('Ctrl Pts',(94.1260143351309,1074.86575397584,364.82831382425));
#120559=CARTESIAN_POINT('Ctrl Pts',(94.113177601997,1074.86268898348,364.765276774419));
#120560=CARTESIAN_POINT('Ctrl Pts',(94.1122778758208,1074.85361851103,364.637475867034));
#120561=CARTESIAN_POINT('Ctrl Pts',(94.124409879171,1074.8476812996,364.573978135957));
#120562=CARTESIAN_POINT('Ctrl Pts',(94.1728220578349,1074.833538774,364.453940275409));
#120563=CARTESIAN_POINT('Ctrl Pts',(94.2092053512491,1074.82542114712,364.398796248784));
#120564=CARTESIAN_POINT('Ctrl Pts',(94.2778158189421,1074.81260148508,364.329731172231));
#120565=CARTESIAN_POINT('Ctrl Pts',(94.3025463005061,1074.80829768802,364.309284998983));
#120566=CARTESIAN_POINT('Ctrl Pts',(94.355671400612,1074.79963006164,364.273477049086));
#120567=CARTESIAN_POINT('Ctrl Pts',(94.3839538127132,1074.79528551796,364.258204655916));
#120568=CARTESIAN_POINT('Ctrl Pts',(94.4734209271869,1074.78231080277,364.220680126695));
#120569=CARTESIAN_POINT('Ctrl Pts',(94.5377780281442,1074.77397382395,364.207675108751));
#120570=CARTESIAN_POINT('Ctrl Pts',(94.6028689869237,1074.766482277,364.207623485824));
#120571=CARTESIAN_POINT('Ctrl Pts',(94.6029986698093,1074.76646735134,364.207623382974));
#120572=CARTESIAN_POINT('Ctrl Pts',(94.6031283506174,1074.76645242961,364.207623331468));
#120573=CARTESIAN_POINT('Ctrl Pts',(94.6032580293194,1074.76643751182,364.207623331468));
#120574=CARTESIAN_POINT('',(94.6032580293201,1082.7251047501,364.207623331468));
#120575=CARTESIAN_POINT('',(94.6032580293201,1067.7251047501,364.207623331468));
#120576=CARTESIAN_POINT('Origin',(94.6032580293201,1082.7251047501,364.698164080197));
#120577=CARTESIAN_POINT('Ctrl Pts',(94.6032580293194,1074.76643751182,364.207623331468));
#120578=CARTESIAN_POINT('Ctrl Pts',(94.6680332572963,1074.75898599329,364.207623331468));
#120579=CARTESIAN_POINT('Ctrl Pts',(94.732282812711,1074.75251641632,364.22045357071));
#120580=CARTESIAN_POINT('Ctrl Pts',(94.8513221203709,1074.74241360936,364.270156160834));
#120581=CARTESIAN_POINT('Ctrl Pts',(94.9050646308186,1074.73883903866,364.306169283017));
#120582=CARTESIAN_POINT('Ctrl Pts',(94.9954062537941,1074.73502183265,364.396654863073));
#120583=CARTESIAN_POINT('Ctrl Pts',(95.0312087567533,1074.73479450522,364.450076096674));
#120584=CARTESIAN_POINT('Ctrl Pts',(95.0803863796765,1074.73771692571,364.567632508475));
#120585=CARTESIAN_POINT('Ctrl Pts',(95.0932612525265,1074.74083680898,364.6305720752));
#120586=CARTESIAN_POINT('Ctrl Pts',(95.0943071710892,1074.75004537671,364.75818118997));
#120587=CARTESIAN_POINT('Ctrl Pts',(95.0822883095453,1074.7560633823,364.821590601207));
#120588=CARTESIAN_POINT('Ctrl Pts',(95.0345111409291,1074.77024359054,364.940668529626));
#120589=CARTESIAN_POINT('Ctrl Pts',(94.9989705004992,1074.77829084204,364.995113303414));
#120590=CARTESIAN_POINT('Ctrl Pts',(94.9315400724301,1074.7910311435,365.064078933143));
#120591=CARTESIAN_POINT('Ctrl Pts',(94.9068770365164,1074.79535855075,365.08478716013));
#120592=CARTESIAN_POINT('Ctrl Pts',(94.853912051573,1074.80404676007,365.121048452993));
#120593=CARTESIAN_POINT('Ctrl Pts',(94.8257343886553,1074.80838806796,365.136528568761));
#120594=CARTESIAN_POINT('Ctrl Pts',(94.7361499980262,1074.82138885907,365.17486371948));
#120595=CARTESIAN_POINT('Ctrl Pts',(94.6714494675528,1074.82973127462,365.188339619355));
#120596=CARTESIAN_POINT('Ctrl Pts',(94.6050444588179,1074.83730842527,365.18870238954));
#120597=CARTESIAN_POINT('Ctrl Pts',(94.6041511950963,1074.83741017283,365.188704828925));
#120598=CARTESIAN_POINT('Ctrl Pts',(94.6032580293201,1074.83751173097,365.188704828925));
#120599=CARTESIAN_POINT('Origin',(40.0345449899143,1067.7251047501,344.508373695255));
#120600=CARTESIAN_POINT('',(40.0345449899354,1078.63462185218,343.030070563061));
#120601=CARTESIAN_POINT('Ctrl Pts',(40.0345298081687,1078.70265697563,345.98667682737));
#120602=CARTESIAN_POINT('Ctrl Pts',(40.1870769959575,1078.70139267951,345.986678393986));
#120603=CARTESIAN_POINT('Ctrl Pts',(40.3387045132084,1078.69970637529,345.963067796558));
#120604=CARTESIAN_POINT('Ctrl Pts',(40.6443100614649,1078.69522348719,345.865531202951));
#120605=CARTESIAN_POINT('Ctrl Pts',(40.7946868828938,1078.69235957377,345.787384514896));
#120606=CARTESIAN_POINT('Ctrl Pts',(41.0731536536299,1078.68537357539,345.575890364103));
#120607=CARTESIAN_POINT('Ctrl Pts',(41.1962041796893,1078.68122519747,345.440489855969));
#120608=CARTESIAN_POINT('Ctrl Pts',(41.3942627051156,1078.67182114612,345.120395956006));
#120609=CARTESIAN_POINT('Ctrl Pts',(41.4630461188509,1078.66659597651,344.935906577345));
#120610=CARTESIAN_POINT('Ctrl Pts',(41.5247801004033,1078.65617516795,344.552542153899));
#120611=CARTESIAN_POINT('Ctrl Pts',(41.5177816248192,1078.65108473326,344.35748835509));
#120612=CARTESIAN_POINT('Ctrl Pts',(41.4327450684474,1078.64233694907,343.996615763979));
#120613=CARTESIAN_POINT('Ctrl Pts',(41.3612884748127,1078.63867249004,343.832636670864));
#120614=CARTESIAN_POINT('Ctrl Pts',(41.1751693589469,1078.63331757418,343.554987476488));
#120615=CARTESIAN_POINT('Ctrl Pts',(41.0676812309894,1078.63148296546,343.439447183941));
#120616=CARTESIAN_POINT('Ctrl Pts',(40.900837799776,1078.63009065238,343.309240123584));
#120617=CARTESIAN_POINT('Ctrl Pts',(40.8557842742147,1078.62982884019,343.277946656458));
#120618=CARTESIAN_POINT('Ctrl Pts',(40.7803487871408,1078.62956909741,343.231543233202));
#120619=CARTESIAN_POINT('Ctrl Pts',(40.7510034224305,1078.62950848805,343.214848799138));
#120620=CARTESIAN_POINT('Ctrl Pts',(40.6942129493864,1078.62946662967,343.185066887409));
#120621=CARTESIAN_POINT('Ctrl Pts',(40.6668851573709,1078.6294780536,343.171792745258));
#120622=CARTESIAN_POINT('Ctrl Pts',(40.6042326255494,1078.62957444674,343.143711907255));
#120623=CARTESIAN_POINT('Ctrl Pts',(40.5687023967708,1078.62967776305,343.129416972725));
#120624=CARTESIAN_POINT('Ctrl Pts',(40.4622711798401,1078.63012789365,343.091327746049));
#120625=CARTESIAN_POINT('Ctrl Pts',(40.3900764676671,1078.63061242729,343.071513947266));
#120626=CARTESIAN_POINT('Ctrl Pts',(40.1235794022449,1078.63302242121,343.019697593838));
#120627=CARTESIAN_POINT('Ctrl Pts',(39.9249134544416,1078.63599068713,343.021076484672));
#120628=CARTESIAN_POINT('Ctrl Pts',(39.5729307101086,1078.64308306182,343.094577439807));
#120629=CARTESIAN_POINT('Ctrl Pts',(39.4200998508842,1078.64686751981,343.153988802032));
#120630=CARTESIAN_POINT('Ctrl Pts',(39.1286721787148,1078.65540846637,343.326949504323));
#120631=CARTESIAN_POINT('Ctrl Pts',(38.9945511780422,1078.66014661647,343.443113584532));
#120632=CARTESIAN_POINT('Ctrl Pts',(38.7656111355713,1078.669929276,343.726871526025));
#120633=CARTESIAN_POINT('Ctrl Pts',(38.676366399166,1078.67487810754,343.894945216506));
#120634=CARTESIAN_POINT('Ctrl Pts',(38.5639733887957,1078.68414479644,344.261723965494));
#120635=CARTESIAN_POINT('Ctrl Pts',(38.5442910887746,1078.68834557585,344.457684168192));
#120636=CARTESIAN_POINT('Ctrl Pts',(38.5813876113478,1078.69532059509,344.838189453119));
#120637=CARTESIAN_POINT('Ctrl Pts',(38.634805416616,1078.69808858127,345.019432170996));
#120638=CARTESIAN_POINT('Ctrl Pts',(38.8090992727656,1078.70241362814,345.357446072826));
#120639=CARTESIAN_POINT('Ctrl Pts',(38.9303211481427,1078.7038969122,345.510039693333));
#120640=CARTESIAN_POINT('Ctrl Pts',(39.1226285262451,1078.70497375118,345.67340753571));
#120641=CARTESIAN_POINT('Ctrl Pts',(39.1700835710925,1078.70516294444,345.709041005679));
#120642=CARTESIAN_POINT('Ctrl Pts',(39.2513688025827,1078.70537039742,345.762753910481));
#120643=CARTESIAN_POINT('Ctrl Pts',(39.2839893481535,1078.70542545781,345.782540442394));
#120644=CARTESIAN_POINT('Ctrl Pts',(39.3435674557254,1078.70547731213,345.815595916527));
#120645=CARTESIAN_POINT('Ctrl Pts',(39.3702333284403,1078.70548401993,345.829346785688));
#120646=CARTESIAN_POINT('Ctrl Pts',(39.4271176663775,1078.70546425427,345.856522157912));
#120647=CARTESIAN_POINT('Ctrl Pts',(39.4574055970158,1078.70543434374,345.869763554872));
#120648=CARTESIAN_POINT('Ctrl Pts',(39.5373721782761,1078.7053054182,345.901575027128));
#120649=CARTESIAN_POINT('Ctrl Pts',(39.587651027545,1078.70517570101,345.918507205525));
#120650=CARTESIAN_POINT('Ctrl Pts',(39.7676148496473,1078.70453971941,345.968518380772));
#120651=CARTESIAN_POINT('Ctrl Pts',(39.9007648912784,1078.70376560612,345.986675453643));
#120652=CARTESIAN_POINT('Ctrl Pts',(40.0345298081687,1078.70265697563,345.98667682737));
#120653=CARTESIAN_POINT('',(40.0345449898976,1076.63346048996,343.030070563062));
#120654=CARTESIAN_POINT('',(40.0345449899143,1067.7251047501,343.030070563062));
#120655=CARTESIAN_POINT('Ctrl Pts',(40.0345647694422,1076.70230005615,345.986676827316));
#120656=CARTESIAN_POINT('Ctrl Pts',(39.8381690817314,1076.70394762921,345.986679455068));
#120657=CARTESIAN_POINT('Ctrl Pts',(39.6437235768841,1076.70486623863,345.947544487483));
#120658=CARTESIAN_POINT('Ctrl Pts',(39.2812618398217,1076.70533123689,345.795472409541));
#120659=CARTESIAN_POINT('Ctrl Pts',(39.1169027655019,1076.70487241795,345.683954438994));
#120660=CARTESIAN_POINT('Ctrl Pts',(38.8422407547009,1076.70253132886,345.403939431545));
#120661=CARTESIAN_POINT('Ctrl Pts',(38.7343551487054,1076.70067430054,345.238530258621));
#120662=CARTESIAN_POINT('Ctrl Pts',(38.5895216200697,1076.6954824908,344.876090383321));
#120663=CARTESIAN_POINT('Ctrl Pts',(38.5537025844545,1076.69219612885,344.682744773146));
#120664=CARTESIAN_POINT('Ctrl Pts',(38.5590755428721,1076.68424813219,344.292265910432));
#120665=CARTESIAN_POINT('Ctrl Pts',(38.6006335398305,1076.67965161652,344.098981965935));
#120666=CARTESIAN_POINT('Ctrl Pts',(38.7175062361582,1076.67212935267,343.829909392309));
#120667=CARTESIAN_POINT('Ctrl Pts',(38.7651558928275,1076.66954215796,343.74446561809));
#120668=CARTESIAN_POINT('Ctrl Pts',(38.931623387017,1076.66168215188,343.505094156789));
#120669=CARTESIAN_POINT('Ctrl Pts',(39.0726414234504,1076.65635074054,343.369185675713));
#120670=CARTESIAN_POINT('Ctrl Pts',(39.3991621772117,1076.64631592817,343.159551097859));
#120671=CARTESIAN_POINT('Ctrl Pts',(39.5815172535644,1076.64171670725,343.08787721764));
#120672=CARTESIAN_POINT('Ctrl Pts',(39.9633978584457,1076.6342187386,343.019100194819));
#120673=CARTESIAN_POINT('Ctrl Pts',(40.159205054712,1076.63139847529,343.022618519874));
#120674=CARTESIAN_POINT('Ctrl Pts',(40.5379335556789,1076.62819188702,343.104998264033));
#120675=CARTESIAN_POINT('Ctrl Pts',(40.7172015103969,1076.6278351644,343.182913632582));
#120676=CARTESIAN_POINT('Ctrl Pts',(41.0351944871715,1076.62968477286,343.403195653141));
#120677=CARTESIAN_POINT('Ctrl Pts',(41.1709204276943,1076.63186629871,343.543303964137));
#120678=CARTESIAN_POINT('Ctrl Pts',(41.3807213749652,1076.63829496575,343.867685954405));
#120679=CARTESIAN_POINT('Ctrl Pts',(41.4528055038673,1076.64247319015,344.048811916474));
#120680=CARTESIAN_POINT('Ctrl Pts',(41.5232926801648,1076.65196438147,344.428654534693));
#120681=CARTESIAN_POINT('Ctrl Pts',(41.5209540579369,1076.65718006625,344.623734821265));
#120682=CARTESIAN_POINT('Ctrl Pts',(41.461261755044,1076.66505854813,344.907362481619));
#120683=CARTESIAN_POINT('Ctrl Pts',(41.4321470439931,1076.66767583019,344.99972042017));
#120684=CARTESIAN_POINT('Ctrl Pts',(41.3563368966256,1076.67280097439,345.177379111665));
#120685=CARTESIAN_POINT('Ctrl Pts',(41.3098333686639,1076.67529657552,345.262258612636));
#120686=CARTESIAN_POINT('Ctrl Pts',(41.1452079246329,1076.68253558073,345.50335243865));
#120687=CARTESIAN_POINT('Ctrl Pts',(41.0041200277274,1076.68688658498,345.641285195669));
#120688=CARTESIAN_POINT('Ctrl Pts',(40.6769876094355,1076.69429247959,345.853953686285));
#120689=CARTESIAN_POINT('Ctrl Pts',(40.4942945461983,1076.69728591065,345.926808178478));
#120690=CARTESIAN_POINT('Ctrl Pts',(40.2142754775636,1076.70064097964,345.978464690868));
#120691=CARTESIAN_POINT('Ctrl Pts',(40.1245146495462,1076.7015454622,345.986675623797));
#120692=CARTESIAN_POINT('Ctrl Pts',(40.0345647694422,1076.70230005615,345.986676827316));
#120693=CARTESIAN_POINT('Origin',(40.0345449899143,1067.7251047501,344.508373695255));
#120694=CARTESIAN_POINT('',(40.0345449899143,1076.69158153387,345.386676827448));
#120695=CARTESIAN_POINT('',(40.034544986754,1076.65067043015,343.630070563062));
#120696=CARTESIAN_POINT('Ctrl Pts',(40.0345449899143,1076.69158153387,345.386676827448));
#120697=CARTESIAN_POINT('Ctrl Pts',(39.9786335213035,1076.69212537235,345.386676827448));
#120698=CARTESIAN_POINT('Ctrl Pts',(39.9227111060459,1076.69256032714,345.38133799963));
#120699=CARTESIAN_POINT('Ctrl Pts',(39.7524248425115,1076.69355902828,345.348358848986));
#120700=CARTESIAN_POINT('Ctrl Pts',(39.6429228985649,1076.69373899373,345.303231742983));
#120701=CARTESIAN_POINT('Ctrl Pts',(39.448278352782,1076.69310701969,345.172761769052));
#120702=CARTESIAN_POINT('Ctrl Pts',(39.3650471625921,1076.69230229399,345.088797046905));
#120703=CARTESIAN_POINT('Ctrl Pts',(39.2366872348667,1076.68973511117,344.893628048601));
#120704=CARTESIAN_POINT('Ctrl Pts',(39.1926679333464,1076.687999699,344.784486146156));
#120705=CARTESIAN_POINT('Ctrl Pts',(39.1498113885486,1076.68369650378,344.55549678087));
#120706=CARTESIAN_POINT('Ctrl Pts',(39.1513641080747,1076.68116920148,344.437928321518));
#120707=CARTESIAN_POINT('Ctrl Pts',(39.1877575310469,1076.67698995566,344.268331674107));
#120708=CARTESIAN_POINT('Ctrl Pts',(39.205126676018,1076.67555954236,344.213867043996));
#120709=CARTESIAN_POINT('Ctrl Pts',(39.2502520250954,1076.67261762342,344.10890519359));
#120710=CARTESIAN_POINT('Ctrl Pts',(39.2779349695538,1076.67111286994,344.058671909614));
#120711=CARTESIAN_POINT('Ctrl Pts',(39.3761497672044,1076.6665198648,343.915517746365));
#120712=CARTESIAN_POINT('Ctrl Pts',(39.4604198919524,1076.6634462406,343.833581805168));
#120713=CARTESIAN_POINT('Ctrl Pts',(39.6549650142604,1076.65777816535,343.707999929808));
#120714=CARTESIAN_POINT('Ctrl Pts',(39.763074061024,1076.65523628195,343.665173713736));
#120715=CARTESIAN_POINT('Ctrl Pts',(39.9286757203146,1076.6522249091,343.634854570039));
#120716=CARTESIAN_POINT('Ctrl Pts',(39.9816183328414,1076.65138505455,343.630070563443));
#120717=CARTESIAN_POINT('Ctrl Pts',(40.0345449835937,1076.65067043015,343.630070563062));
#120718=CARTESIAN_POINT('',(40.0345449899143,1082.7251047501,343.630070563062));
#120719=CARTESIAN_POINT('',(40.0345449899143,1067.7251047501,343.630070563062));
#120720=CARTESIAN_POINT('Origin',(40.0345449899143,1082.7251047501,344.508373695255));
#120721=CARTESIAN_POINT('Ctrl Pts',(40.0345449835937,1076.65067043015,343.630070563062));
#120722=CARTESIAN_POINT('Ctrl Pts',(40.0962035459098,1076.64983790604,343.630070562618));
#120723=CARTESIAN_POINT('Ctrl Pts',(40.1578404465244,1076.64917544013,343.636563440191));
#120724=CARTESIAN_POINT('Ctrl Pts',(40.3308810453299,1076.64782522135,343.673611547947));
#120725=CARTESIAN_POINT('Ctrl Pts',(40.4375233994829,1076.64762160324,343.719544297305));
#120726=CARTESIAN_POINT('Ctrl Pts',(40.6269430771155,1076.64859800546,343.849829191404));
#120727=CARTESIAN_POINT('Ctrl Pts',(40.7079102894806,1076.6497664633,343.932880149146));
#120728=CARTESIAN_POINT('Ctrl Pts',(40.8332649402529,1076.65325914728,344.125415059333));
#120729=CARTESIAN_POINT('Ctrl Pts',(40.8764455468128,1076.6555473135,344.233036523614));
#120730=CARTESIAN_POINT('Ctrl Pts',(40.9068968632132,1076.65933360956,344.394815192062));
#120731=CARTESIAN_POINT('Ctrl Pts',(40.9119290308596,1076.66053770417,344.444418012714));
#120732=CARTESIAN_POINT('Ctrl Pts',(40.9127333929343,1076.66178363424,344.494177892296));
#120733=CARTESIAN_POINT('Ctrl Pts',(40.9145913478028,1076.66466154447,344.609115696348));
#120734=CARTESIAN_POINT('Ctrl Pts',(40.8938666841488,1076.66772012843,344.723306089928));
#120735=CARTESIAN_POINT('Ctrl Pts',(40.8307220192165,1076.67226453346,344.883616932722));
#120736=CARTESIAN_POINT('Ctrl Pts',(40.8045283503295,1076.67376017027,344.934790321281));
#120737=CARTESIAN_POINT('Ctrl Pts',(40.7105285925089,1076.67817941879,345.081133380678));
#120738=CARTESIAN_POINT('Ctrl Pts',(40.6286166916474,1076.68093604389,345.165708538019));
#120739=CARTESIAN_POINT('Ctrl Pts',(40.4366974478299,1076.68578220386,345.297829447687));
#120740=CARTESIAN_POINT('Ctrl Pts',(40.3286359851419,1076.68782722287,345.344125209233));
#120741=CARTESIAN_POINT('Ctrl Pts',(40.1553017976055,1076.69027980393,345.380449449774));
#120742=CARTESIAN_POINT('Ctrl Pts',(40.0949297780623,1076.69099418439,345.386676827448));
#120743=CARTESIAN_POINT('Ctrl Pts',(40.0345449899143,1076.69158153387,345.386676827448));
#120744=CARTESIAN_POINT('Origin',(52.543999119444,1067.7251047501,343.402193778667));
#120745=CARTESIAN_POINT('',(52.5439991194616,1078.27787179661,342.12674965753));
#120746=CARTESIAN_POINT('Ctrl Pts',(52.5439470409818,1078.414918165,344.67763789874));
#120747=CARTESIAN_POINT('Ctrl Pts',(52.6806287622999,1078.41052452383,344.677643479677));
#120748=CARTESIAN_POINT('Ctrl Pts',(52.8163853250807,1078.40503088569,344.65567846108));
#120749=CARTESIAN_POINT('Ctrl Pts',(53.0877764056428,1078.39154679656,344.5655398441));
#120750=CARTESIAN_POINT('Ctrl Pts',(53.2201162054865,1078.3834727294,344.493938536534));
#120751=CARTESIAN_POINT('Ctrl Pts',(53.4629019934239,1078.36520134234,344.301195872381));
#120752=CARTESIAN_POINT('Ctrl Pts',(53.5687394638358,1078.35504826614,344.178388505717));
#120753=CARTESIAN_POINT('Ctrl Pts',(53.7333383278594,1078.33388013324,343.892865438981));
#120754=CARTESIAN_POINT('Ctrl Pts',(53.7878043824023,1078.32305394832,343.731206514432));
#120755=CARTESIAN_POINT('Ctrl Pts',(53.8299759183017,1078.30309729252,343.400679940482));
#120756=CARTESIAN_POINT('Ctrl Pts',(53.8191019530346,1078.29411629439,343.235191379999));
#120757=CARTESIAN_POINT('Ctrl Pts',(53.7391934951799,1078.27978612663,342.932863065434));
#120758=CARTESIAN_POINT('Ctrl Pts',(53.6765468888482,1078.27428018031,342.797109888813));
#120759=CARTESIAN_POINT('Ctrl Pts',(53.5357022654691,1078.26778955493,342.594101148773));
#120760=CARTESIAN_POINT('Ctrl Pts',(53.4702493947951,1078.26592976164,342.519836287121));
#120761=CARTESIAN_POINT('Ctrl Pts',(53.3684220975573,1078.26443171191,342.428258731446));
#120762=CARTESIAN_POINT('Ctrl Pts',(53.3388244100163,1078.26413114032,342.403957521689));
#120763=CARTESIAN_POINT('Ctrl Pts',(53.2880554917141,1078.26383087659,342.365965283963));
#120764=CARTESIAN_POINT('Ctrl Pts',(53.2674921492526,1078.26376336979,342.351504848028));
#120765=CARTESIAN_POINT('Ctrl Pts',(53.2266567979879,1078.26373244668,342.324556416679));
#120766=CARTESIAN_POINT('Ctrl Pts',(53.2064359306392,1078.26376367514,342.31200973171));
#120767=CARTESIAN_POINT('Ctrl Pts',(53.1584316695823,1078.26394450058,342.284052910683));
#120768=CARTESIAN_POINT('Ctrl Pts',(53.1304003051289,1078.26413017116,342.26910068918));
#120769=CARTESIAN_POINT('Ctrl Pts',(53.0402284246735,1078.26497458922,342.225245110275));
#120770=CARTESIAN_POINT('Ctrl Pts',(52.9763066088944,1078.26593088975,342.200295062625));
#120771=CARTESIAN_POINT('Ctrl Pts',(52.7478690818006,1078.2705386644,342.131722806857));
#120772=CARTESIAN_POINT('Ctrl Pts',(52.5769645665709,1078.27604053758,342.115907675524));
#120773=CARTESIAN_POINT('Ctrl Pts',(52.268016297067,1078.28940144417,342.149027699748));
#120774=CARTESIAN_POINT('Ctrl Pts',(52.131482905164,1078.29660142415,342.18712348529));
#120775=CARTESIAN_POINT('Ctrl Pts',(51.865880749568,1078.31324185179,342.311253696498));
#120776=CARTESIAN_POINT('Ctrl Pts',(51.7404935650894,1078.3226834259,342.400018787585));
#120777=CARTESIAN_POINT('Ctrl Pts',(51.5192208871175,1078.34284470951,342.625455281768));
#120778=CARTESIAN_POINT('Ctrl Pts',(51.4281787326337,1078.35342112333,342.763097396756));
#120779=CARTESIAN_POINT('Ctrl Pts',(51.3012247989589,1078.37398239285,343.069650137752));
#120780=CARTESIAN_POINT('Ctrl Pts',(51.2682200221517,1078.38374276718,343.236379318044));
#120781=CARTESIAN_POINT('Ctrl Pts',(51.2688793490305,1078.40054058862,343.56526497517));
#120782=CARTESIAN_POINT('Ctrl Pts',(51.2994994186301,1078.40753814576,343.724340385699));
#120783=CARTESIAN_POINT('Ctrl Pts',(51.4200335928109,1078.41874857271,344.027373443867));
#120784=CARTESIAN_POINT('Ctrl Pts',(51.5105682129547,1078.42276773402,344.167827510623));
#120785=CARTESIAN_POINT('Ctrl Pts',(51.6632745076855,1078.42569550122,344.326344748451));
#120786=CARTESIAN_POINT('Ctrl Pts',(51.7035848423353,1078.42622028533,344.363149096999));
#120787=CARTESIAN_POINT('Ctrl Pts',(51.7684815765133,1078.42671193573,344.41518498354));
#120788=CARTESIAN_POINT('Ctrl Pts',(51.7914328720423,1078.42682522576,344.432350422273));
#120789=CARTESIAN_POINT('Ctrl Pts',(51.8339428942365,1078.42692850034,344.461964535543));
#120790=CARTESIAN_POINT('Ctrl Pts',(51.8532998285876,1078.42693794926,344.474680791104));
#120791=CARTESIAN_POINT('Ctrl Pts',(51.8952905869465,1078.42687980587,344.500657456102));
#120792=CARTESIAN_POINT('Ctrl Pts',(51.9180089549087,1078.42680186758,344.513760920601));
#120793=CARTESIAN_POINT('Ctrl Pts',(51.9797073234866,1078.42646826494,344.546855462759));
#120794=CARTESIAN_POINT('Ctrl Pts',(52.0193394914607,1078.42612873875,344.565554300254));
#120795=CARTESIAN_POINT('Ctrl Pts',(52.1978811024911,1078.4240594286,344.638809653504));
#120796=CARTESIAN_POINT('Ctrl Pts',(52.3447533564488,1078.42096974804,344.67077594215));
#120797=CARTESIAN_POINT('Ctrl Pts',(52.5104912914418,1078.41597667431,344.677307423537));
#120798=CARTESIAN_POINT('Ctrl Pts',(52.5272186158717,1078.41545590111,344.677637215691));
#120799=CARTESIAN_POINT('Ctrl Pts',(52.5439470409818,1078.414918165,344.677637898739));
#120800=CARTESIAN_POINT('',(52.5439991194251,1076.27285491302,342.12674965753));
#120801=CARTESIAN_POINT('',(52.543999119444,1067.7251047501,342.126749657531));
#120802=CARTESIAN_POINT('Ctrl Pts',(52.5448741578425,1076.41130048726,344.677637599636));
#120803=CARTESIAN_POINT('Ctrl Pts',(52.3760585255815,1076.4167911207,344.67775341827));
#120804=CARTESIAN_POINT('Ctrl Pts',(52.2088482972886,1076.42049246151,344.644351612941));
#120805=CARTESIAN_POINT('Ctrl Pts',(51.8969113527991,1076.42404043833,344.514231820045));
#120806=CARTESIAN_POINT('Ctrl Pts',(51.7553423336663,1076.42384876801,344.418741966092));
#120807=CARTESIAN_POINT('Ctrl Pts',(51.5178702888806,1076.41954871692,344.178292808864));
#120808=CARTESIAN_POINT('Ctrl Pts',(51.4242785122984,1076.41548646548,344.035808714357));
#120809=CARTESIAN_POINT('Ctrl Pts',(51.2980352713163,1076.40384472051,343.722815650814));
#120810=CARTESIAN_POINT('Ctrl Pts',(51.2666181326482,1076.3963770296,343.555427530059));
#120811=CARTESIAN_POINT('Ctrl Pts',(51.2706886250048,1076.37874428829,343.217261708239));
#120812=CARTESIAN_POINT('Ctrl Pts',(51.3065307289596,1076.36873442188,343.049834047307));
#120813=CARTESIAN_POINT('Ctrl Pts',(51.407604560614,1076.35276810011,342.816974900379));
#120814=CARTESIAN_POINT('Ctrl Pts',(51.4487844347974,1076.34734114316,342.743121125799));
#120815=CARTESIAN_POINT('Ctrl Pts',(51.5926665317801,1076.33100148369,342.536271250745));
#120816=CARTESIAN_POINT('Ctrl Pts',(51.7145906311547,1076.32011487132,342.418857721563));
#120817=CARTESIAN_POINT('Ctrl Pts',(51.9968842888048,1076.2996593575,342.237923173106));
#120818=CARTESIAN_POINT('Ctrl Pts',(52.1545332014154,1076.29029077785,342.176135972092));
#120819=CARTESIAN_POINT('Ctrl Pts',(52.4844665501504,1076.27456705509,342.117189794759));
#120820=CARTESIAN_POINT('Ctrl Pts',(52.6535123759482,1076.26836276017,342.120464788608));
#120821=CARTESIAN_POINT('Ctrl Pts',(52.980196402225,1076.26016733156,342.192089869105));
#120822=CARTESIAN_POINT('Ctrl Pts',(53.1346721618463,1076.25824420501,342.259503616586));
#120823=CARTESIAN_POINT('Ctrl Pts',(53.4085097230585,1076.25901715282,342.449777353806));
#120824=CARTESIAN_POINT('Ctrl Pts',(53.525287599844,1076.26169208717,342.570612864856));
#120825=CARTESIAN_POINT('Ctrl Pts',(53.7058022611237,1076.27122502918,342.8502324545));
#120826=CARTESIAN_POINT('Ctrl Pts',(53.7677911877719,1076.2779866748,343.006293756194));
#120827=CARTESIAN_POINT('Ctrl Pts',(53.8284633256784,1076.2945610217,343.333678621171));
#120828=CARTESIAN_POINT('Ctrl Pts',(53.8264053467256,1076.30421755588,343.501892394966));
#120829=CARTESIAN_POINT('Ctrl Pts',(53.7576888084343,1076.32499206789,343.828362276718));
#120830=CARTESIAN_POINT('Ctrl Pts',(53.691504005586,1076.33591258319,343.983474542858));
#120831=CARTESIAN_POINT('Ctrl Pts',(53.503066844489,1076.35747764861,344.259447919595));
#120832=CARTESIAN_POINT('Ctrl Pts',(53.382571470997,1076.36791606443,344.377650827589));
#120833=CARTESIAN_POINT('Ctrl Pts',(53.1014708282764,1076.38707781672,344.561706105059));
#120834=CARTESIAN_POINT('Ctrl Pts',(52.9432602796086,1076.39559959136,344.62525367013));
#120835=CARTESIAN_POINT('Ctrl Pts',(52.7005954176518,1076.40586432971,344.670384508208));
#120836=CARTESIAN_POINT('Ctrl Pts',(52.6228257610832,1076.40876515523,344.677584119706));
#120837=CARTESIAN_POINT('Ctrl Pts',(52.5448741578425,1076.41130048726,344.677637599636));
#120838=CARTESIAN_POINT('Origin',(52.543999119444,1067.7251047501,343.402193778667));
#120839=CARTESIAN_POINT('',(52.543999119444,1076.38098512892,344.077637899803));
#120840=CARTESIAN_POINT('',(52.5439991194442,1076.3076507295,342.726749657531));
#120841=CARTESIAN_POINT('Ctrl Pts',(52.543999119444,1076.38098512892,344.077637899803));
#120842=CARTESIAN_POINT('Ctrl Pts',(52.5433807264998,1076.38100599235,344.077637899803));
#120843=CARTESIAN_POINT('Ctrl Pts',(52.542762289986,1076.3810268122,344.077637050562));
#120844=CARTESIAN_POINT('Ctrl Pts',(52.4523875817405,1076.38406271807,344.077388808654));
#120845=CARTESIAN_POINT('Ctrl Pts',(52.3635521603753,1076.38609930809,344.059253661504));
#120846=CARTESIAN_POINT('Ctrl Pts',(52.1981297309606,1076.3880170916,343.989276229176));
#120847=CARTESIAN_POINT('Ctrl Pts',(52.1232170008691,1076.38787904209,343.938135262467));
#120848=CARTESIAN_POINT('Ctrl Pts',(51.9977994361851,1076.38542237209,343.809568380947));
#120849=CARTESIAN_POINT('Ctrl Pts',(51.9485567483193,1076.38312830049,343.733445801916));
#120850=CARTESIAN_POINT('Ctrl Pts',(51.8826782488512,1076.37662930272,343.566366025876));
#120851=CARTESIAN_POINT('Ctrl Pts',(51.8667406204239,1076.37248613241,343.477071121541));
#120852=CARTESIAN_POINT('Ctrl Pts',(51.8707060407776,1076.36282170416,343.297156301785));
#120853=CARTESIAN_POINT('Ctrl Pts',(51.890726046444,1076.35738996094,343.20833338735));
#120854=CARTESIAN_POINT('Ctrl Pts',(51.9458353864727,1076.3488351946,343.08529995842));
#120855=CARTESIAN_POINT('Ctrl Pts',(51.9681033615599,1076.34595007169,343.046433614101));
#120856=CARTESIAN_POINT('Ctrl Pts',(52.0455468991329,1076.33731465088,342.937823430901));
#120857=CARTESIAN_POINT('Ctrl Pts',(52.110786128562,1076.33162386015,342.876431855099));
#120858=CARTESIAN_POINT('Ctrl Pts',(52.2612458989706,1076.32103007045,342.782402809608));
#120859=CARTESIAN_POINT('Ctrl Pts',(52.3450082375807,1076.31622956707,342.750653784727));
#120860=CARTESIAN_POINT('Ctrl Pts',(52.4693696608681,1076.3105451118,342.729847663679));
#120861=CARTESIAN_POINT('Ctrl Pts',(52.5066490854813,1076.30901319594,342.726749657531));
#120862=CARTESIAN_POINT('Ctrl Pts',(52.5439991194443,1076.3076507295,342.726749657531));
#120863=CARTESIAN_POINT('',(52.543999119444,1082.7251047501,342.72674965753));
#120864=CARTESIAN_POINT('',(52.543999119444,1067.7251047501,342.72674965753));
#120865=CARTESIAN_POINT('Origin',(52.543999119444,1082.7251047501,343.402193778667));
#120866=CARTESIAN_POINT('Ctrl Pts',(52.5439991194443,1076.3076507295,342.726749657531));
#120867=CARTESIAN_POINT('Ctrl Pts',(52.5441477900375,1076.30764530625,342.726749657531));
#120868=CARTESIAN_POINT('Ctrl Pts',(52.5442964617491,1076.30763988567,342.726749706442));
#120869=CARTESIAN_POINT('Ctrl Pts',(52.5444451345556,1076.30763446778,342.726749804615));
#120870=CARTESIAN_POINT('Ctrl Pts',(52.6329197611313,1076.30441030596,342.726808226946));
#120871=CARTESIAN_POINT('Ctrl Pts',(52.7205517733353,1076.30218341099,342.744249612993));
#120872=CARTESIAN_POINT('Ctrl Pts',(52.8839167860554,1076.3000238337,342.811876149376));
#120873=CARTESIAN_POINT('Ctrl Pts',(52.9580808165592,1076.30010657371,342.861310328468));
#120874=CARTESIAN_POINT('Ctrl Pts',(53.0831251884017,1076.30258187268,342.985844757017));
#120875=CARTESIAN_POINT('Ctrl Pts',(53.1328063450898,1076.30494745181,343.059702544723));
#120876=CARTESIAN_POINT('Ctrl Pts',(53.2010284385821,1076.3116279873,343.222391644339));
#120877=CARTESIAN_POINT('Ctrl Pts',(53.2188641763637,1076.31587973779,343.309666606089));
#120878=CARTESIAN_POINT('Ctrl Pts',(53.2199960970929,1076.32567177348,343.486302900883));
#120879=CARTESIAN_POINT('Ctrl Pts',(53.2031883434355,1076.33112027135,343.573973116125));
#120880=CARTESIAN_POINT('Ctrl Pts',(53.1367204121467,1076.34245755723,343.737976388051));
#120881=CARTESIAN_POINT('Ctrl Pts',(53.0876321814311,1076.34823836342,343.812721321394));
#120882=CARTESIAN_POINT('Ctrl Pts',(52.9623579357704,1076.35944707001,343.940071688636));
#120883=CARTESIAN_POINT('Ctrl Pts',(52.8869687016715,1076.36475686067,343.991021635442));
#120884=CARTESIAN_POINT('Ctrl Pts',(52.7214919960114,1076.37405943928,344.059968834246));
#120885=CARTESIAN_POINT('Ctrl Pts',(52.6331988197174,1076.37797569543,344.077637899803));
#120886=CARTESIAN_POINT('Ctrl Pts',(52.543999119444,1076.38098512892,344.077637899803));
#120887=CARTESIAN_POINT('Origin',(66.3937896239309,1067.7251047501,343.44168792613));
#120888=CARTESIAN_POINT('',(66.3937896239499,1077.5767973048,342.342856790137));
#120889=CARTESIAN_POINT('Ctrl Pts',(66.393844446936,1077.75229507912,344.540519060755));
#120890=CARTESIAN_POINT('Ctrl Pts',(66.5156047808145,1077.74457990434,344.540512985874));
#120891=CARTESIAN_POINT('Ctrl Pts',(66.6364164896922,1077.73532362626,344.520270125798));
#120892=CARTESIAN_POINT('Ctrl Pts',(66.8764648242798,1077.71349668689,344.437659106797));
#120893=CARTESIAN_POINT('Ctrl Pts',(66.9926823993953,1077.70088000448,344.372395271678));
#120894=CARTESIAN_POINT('Ctrl Pts',(67.2041742539876,1077.67328602451,344.197326472306));
#120895=CARTESIAN_POINT('Ctrl Pts',(67.2951792475751,1077.65845261111,344.086051003281));
#120896=CARTESIAN_POINT('Ctrl Pts',(67.4308913778546,1077.62913740611,343.832688323854));
#120897=CARTESIAN_POINT('Ctrl Pts',(67.4734312399676,1077.61494537538,343.692466422285));
#120898=CARTESIAN_POINT('Ctrl Pts',(67.5007105882041,1077.59022872158,343.411663502516));
#120899=CARTESIAN_POINT('Ctrl Pts',(67.4883765111924,1077.57975612923,343.273978206053));
#120900=CARTESIAN_POINT('Ctrl Pts',(67.4125482135635,1077.5628407334,343.006484785892));
#120901=CARTESIAN_POINT('Ctrl Pts',(67.3484012867948,1077.55667540388,342.879507191737));
#120902=CARTESIAN_POINT('Ctrl Pts',(67.2363297287251,1077.55230747336,342.735077440396));
#120903=CARTESIAN_POINT('Ctrl Pts',(67.2088793297651,1077.55155832973,342.703581066852));
#120904=CARTESIAN_POINT('Ctrl Pts',(67.1640309920068,1077.55079498211,342.657684895358));
#120905=CARTESIAN_POINT('Ctrl Pts',(67.1478742767711,1077.55060127544,342.642132478529));
#120906=CARTESIAN_POINT('Ctrl Pts',(67.1174314726128,1077.55038077762,342.614572503704));
#120907=CARTESIAN_POINT('Ctrl Pts',(67.103294019441,1077.55033139913,342.602413851488));
#120908=CARTESIAN_POINT('Ctrl Pts',(67.0741661943938,1077.55033423748,342.578625234909));
#120909=CARTESIAN_POINT('Ctrl Pts',(67.0591704618174,1077.55038821109,342.567012089965));
#120910=CARTESIAN_POINT('Ctrl Pts',(67.0219534853485,1077.55064734677,342.539701329928));
#120911=CARTESIAN_POINT('Ctrl Pts',(66.9994360342243,1077.55090789771,342.524430069476));
#120912=CARTESIAN_POINT('Ctrl Pts',(66.919336635988,1077.55218540012,342.474343177823));
#120913=CARTESIAN_POINT('Ctrl Pts',(66.8591547614701,1077.55374852366,342.443997143634));
#120914=CARTESIAN_POINT('Ctrl Pts',(66.660270835929,1077.56072099858,342.365636889656));
#120915=CARTESIAN_POINT('Ctrl Pts',(66.5147068104391,1077.56842132315,342.339779830423));
#120916=CARTESIAN_POINT('Ctrl Pts',(66.2463109020279,1077.58696107329,342.345962596173));
#120917=CARTESIAN_POINT('Ctrl Pts',(66.1255671040911,1077.59694354704,342.369134434207));
#120918=CARTESIAN_POINT('Ctrl Pts',(65.8870664179928,1077.62003066478,342.457718359591));
#120919=CARTESIAN_POINT('Ctrl Pts',(65.7723544065373,1077.6331425326,342.525857453649));
#120920=CARTESIAN_POINT('Ctrl Pts',(65.5652017859656,1077.66124856549,342.70607871717));
#120921=CARTESIAN_POINT('Ctrl Pts',(65.4769899780966,1077.67605320035,342.819460488795));
#120922=CARTESIAN_POINT('Ctrl Pts',(65.3475510385666,1077.70475009774,343.075883486354));
#120923=CARTESIAN_POINT('Ctrl Pts',(65.3084313242539,1077.71834953237,343.216990505056));
#120924=CARTESIAN_POINT('Ctrl Pts',(65.2879561572984,1077.7415744366,343.497635090311));
#120925=CARTESIAN_POINT('Ctrl Pts',(65.3033975496496,1077.75119426144,343.634327110823));
#120926=CARTESIAN_POINT('Ctrl Pts',(65.3860847421763,1077.76673889436,343.903094257173));
#120927=CARTESIAN_POINT('Ctrl Pts',(65.455557862181,1077.77225539152,344.031721937204));
#120928=CARTESIAN_POINT('Ctrl Pts',(65.5706513000055,1077.77568245297,344.170471871437));
#120929=CARTESIAN_POINT('Ctrl Pts',(65.594554333178,1077.77618819588,344.196609138093));
#120930=CARTESIAN_POINT('Ctrl Pts',(65.6358849765145,1077.7767426396,344.237635048401));
#120931=CARTESIAN_POINT('Ctrl Pts',(65.652588831005,1077.77688970836,344.253212852171));
#120932=CARTESIAN_POINT('Ctrl Pts',(65.683366751852,1077.77702686598,344.280172335808));
#120933=CARTESIAN_POINT('Ctrl Pts',(65.6972592660129,1077.77704324397,344.29174805819));
#120934=CARTESIAN_POINT('Ctrl Pts',(65.7271922708986,1077.77698438626,344.315462593795));
#120935=CARTESIAN_POINT('Ctrl Pts',(65.74329306933,1077.77689868224,344.327514329823));
#120936=CARTESIAN_POINT('Ctrl Pts',(65.7865323385124,1077.77652918998,344.358064821957));
#120937=CARTESIAN_POINT('Ctrl Pts',(65.814183915158,1077.77615455756,344.375799824849));
#120938=CARTESIAN_POINT('Ctrl Pts',(65.9355059909989,1077.77393712333,344.446149514732));
#120939=CARTESIAN_POINT('Ctrl Pts',(66.0357869149437,1077.77070578318,344.486093316765));
#120940=CARTESIAN_POINT('Ctrl Pts',(66.2233615474464,1077.76231076593,344.530580163756));
#120941=CARTESIAN_POINT('Ctrl Pts',(66.3084805240333,1077.75770404577,344.540523319741));
#120942=CARTESIAN_POINT('Ctrl Pts',(66.393844446936,1077.75229507912,344.540519060755));
#120943=CARTESIAN_POINT('',(66.3937896239311,1075.56506587574,342.342856790137));
#120944=CARTESIAN_POINT('',(66.3937896239309,1067.7251047501,342.342856790137));
#120945=CARTESIAN_POINT('Ctrl Pts',(66.3932272216318,1075.74221012263,344.540518918198));
#120946=CARTESIAN_POINT('Ctrl Pts',(66.2474802543578,1075.75152431216,344.540444322168));
#120947=CARTESIAN_POINT('Ctrl Pts',(66.103078919897,1075.75843983839,344.511372802697));
#120948=CARTESIAN_POINT('Ctrl Pts',(65.8336989264172,1075.76676134646,344.398294360709));
#120949=CARTESIAN_POINT('Ctrl Pts',(65.7115269763156,1075.76807547437,344.315375098008));
#120950=CARTESIAN_POINT('Ctrl Pts',(65.5068551547325,1075.76487056035,344.106616976573));
#120951=CARTESIAN_POINT('Ctrl Pts',(65.4264460255889,1075.76038790145,343.982967587889));
#120952=CARTESIAN_POINT('Ctrl Pts',(65.3187398076029,1075.74613160246,343.7117951189));
#120953=CARTESIAN_POINT('Ctrl Pts',(65.2924759146155,1075.73650629327,343.567057759706));
#120954=CARTESIAN_POINT('Ctrl Pts',(65.2978182202965,1075.71323086363,343.275602151053));
#120955=CARTESIAN_POINT('Ctrl Pts',(65.3295437562049,1075.69979682563,343.131771747123));
#120956=CARTESIAN_POINT('Ctrl Pts',(65.4171797226662,1075.67821918432,342.932986273977));
#120957=CARTESIAN_POINT('Ctrl Pts',(65.452341935033,1075.67091610097,342.870534494126));
#120958=CARTESIAN_POINT('Ctrl Pts',(65.5344480859605,1075.65608241569,342.75312801349));
#120959=CARTESIAN_POINT('Ctrl Pts',(65.5812512531236,1075.64858516863,342.69847617303));
#120960=CARTESIAN_POINT('Ctrl Pts',(65.7384930843161,1075.62595622194,342.54761293775));
#120961=CARTESIAN_POINT('Ctrl Pts',(65.8631256982616,1075.61117448687,342.468432654874));
#120962=CARTESIAN_POINT('Ctrl Pts',(66.1345163634118,1075.58438902696,342.364157470795));
#120963=CARTESIAN_POINT('Ctrl Pts',(66.2783887558511,1075.57261072206,342.339390174486));
#120964=CARTESIAN_POINT('Ctrl Pts',(66.566849366719,1075.55367179737,342.347079732253));
#120965=CARTESIAN_POINT('Ctrl Pts',(66.7086065581168,1075.5466708528,342.379107852499));
#120966=CARTESIAN_POINT('Ctrl Pts',(66.9711281072818,1075.53849079615,342.495841035501));
#120967=CARTESIAN_POINT('Ctrl Pts',(67.0893930388519,1075.53736121238,342.57907879815));
#120968=CARTESIAN_POINT('Ctrl Pts',(67.287157616269,1075.54114581463,342.786110836944));
#120969=CARTESIAN_POINT('Ctrl Pts',(67.3647506911734,1075.54601098546,342.90776706945));
#120970=CARTESIAN_POINT('Ctrl Pts',(67.4691769431824,1075.56107977074,343.174248689843));
#120971=CARTESIAN_POINT('Ctrl Pts',(67.4948053120897,1075.57115155937,343.316533160801));
#120972=CARTESIAN_POINT('Ctrl Pts',(67.4901297386214,1075.59513940164,343.603554794462));
#120973=CARTESIAN_POINT('Ctrl Pts',(67.4595134358805,1075.60884679079,343.745548817247));
#120974=CARTESIAN_POINT('Ctrl Pts',(67.3738733608471,1075.63069259695,343.943754995825));
#120975=CARTESIAN_POINT('Ctrl Pts',(67.3388066801131,1075.63815275872,344.006997741652));
#120976=CARTESIAN_POINT('Ctrl Pts',(67.2568961660437,1075.6531536218,344.125541247711));
#120977=CARTESIAN_POINT('Ctrl Pts',(67.210269256498,1075.66065939707,344.180586074322));
#120978=CARTESIAN_POINT('Ctrl Pts',(67.053711728565,1075.68311375052,344.332344363354));
#120979=CARTESIAN_POINT('Ctrl Pts',(66.9295361570051,1075.69755011896,344.412149796458));
#120980=CARTESIAN_POINT('Ctrl Pts',(66.6659000552012,1075.72273875493,344.515040382875));
#120981=CARTESIAN_POINT('Ctrl Pts',(66.5302251879546,1075.73345505178,344.540589036325));
#120982=CARTESIAN_POINT('Ctrl Pts',(66.3932272216318,1075.74221012263,344.540518918198));
#120983=CARTESIAN_POINT('Origin',(66.3937896239309,1067.7251047501,343.44168792613));
#120984=CARTESIAN_POINT('',(66.3937896239309,1075.69533039084,343.940519062122));
#120985=CARTESIAN_POINT('',(66.3937896239307,1075.61493016275,342.942856790137));
#120986=CARTESIAN_POINT('Ctrl Pts',(66.3937896239309,1075.69533039084,343.940519062122));
#120987=CARTESIAN_POINT('Ctrl Pts',(66.3936857389102,1075.69533714603,343.940519062122));
#120988=CARTESIAN_POINT('Ctrl Pts',(66.3935818520956,1075.69534389873,343.94051902967));
#120989=CARTESIAN_POINT('Ctrl Pts',(66.3270401237183,1075.69966748105,343.940477455626));
#120990=CARTESIAN_POINT('Ctrl Pts',(66.2612210191196,1075.70287960374,343.927163298428));
#120991=CARTESIAN_POINT('Ctrl Pts',(66.1400081066437,1075.70668362999,343.876030984594));
#120992=CARTESIAN_POINT('Ctrl Pts',(66.0856109827812,1075.70729671465,343.839290514662));
#120993=CARTESIAN_POINT('Ctrl Pts',(65.9939584714249,1075.70592219778,343.746973765016));
#120994=CARTESIAN_POINT('Ctrl Pts',(65.9576216472256,1075.70394746083,343.692312800562));
#120995=CARTESIAN_POINT('Ctrl Pts',(65.9073820050535,1075.69756411103,343.570782221173));
#120996=CARTESIAN_POINT('Ctrl Pts',(65.8945458337568,1075.69316420124,343.504904016412));
#120997=CARTESIAN_POINT('Ctrl Pts',(65.8953923813694,1075.68251179053,343.37195999464));
#120998=CARTESIAN_POINT('Ctrl Pts',(65.9091289550251,1075.67636087266,343.306221376174));
#120999=CARTESIAN_POINT('Ctrl Pts',(65.9481307274171,1075.66650499341,343.215236903949));
#121000=CARTESIAN_POINT('Ctrl Pts',(65.9638492653669,1075.66317600945,343.186653888216));
#121001=CARTESIAN_POINT('Ctrl Pts',(66.0006561980104,1075.65642883476,343.132913877559));
#121002=CARTESIAN_POINT('Ctrl Pts',(66.0216703849935,1075.65302603371,343.107887747318));
#121003=CARTESIAN_POINT('Ctrl Pts',(66.0927979615361,1075.64271090725,343.038312395468));
#121004=CARTESIAN_POINT('Ctrl Pts',(66.1495729191216,1075.63597265537,343.001601506029));
#121005=CARTESIAN_POINT('Ctrl Pts',(66.2697411886632,1075.62416188221,342.954555511029));
#121006=CARTESIAN_POINT('Ctrl Pts',(66.3313197546715,1075.61910513006,342.94289143163));
#121007=CARTESIAN_POINT('Ctrl Pts',(66.3935123918432,1075.61494868444,342.942856867238));
#121008=CARTESIAN_POINT('Ctrl Pts',(66.3936048036805,1075.61494250839,342.942856815879));
#121009=CARTESIAN_POINT('Ctrl Pts',(66.3936972143795,1075.61493633449,342.942856790137));
#121010=CARTESIAN_POINT('Ctrl Pts',(66.3937896239304,1075.61493016275,342.942856790137));
#121011=CARTESIAN_POINT('',(66.3937896239309,1082.7251047501,342.942856790137));
#121012=CARTESIAN_POINT('',(66.3937896239309,1067.7251047501,342.942856790137));
#121013=CARTESIAN_POINT('Origin',(66.3937896239309,1082.7251047501,343.44168792613));
#121014=CARTESIAN_POINT('Ctrl Pts',(66.3937896239304,1075.61493016275,342.942856790137));
#121015=CARTESIAN_POINT('Ctrl Pts',(66.4589533147248,1075.61057808795,342.942856790137));
#121016=CARTESIAN_POINT('Ctrl Pts',(66.5235459705353,1075.60729823447,342.955625539973));
#121017=CARTESIAN_POINT('Ctrl Pts',(66.6440165015387,1075.60329532221,343.005284692942));
#121018=CARTESIAN_POINT('Ctrl Pts',(66.6987277318149,1075.60260290825,343.041591128476));
#121019=CARTESIAN_POINT('Ctrl Pts',(66.7910831321971,1075.60391406314,343.133123469872));
#121020=CARTESIAN_POINT('Ctrl Pts',(66.8278269578003,1075.60590102542,343.187411743355));
#121021=CARTESIAN_POINT('Ctrl Pts',(66.8785310374756,1075.61230429113,343.307150947806));
#121022=CARTESIAN_POINT('Ctrl Pts',(66.8919118393908,1075.61666534876,343.371458683115));
#121023=CARTESIAN_POINT('Ctrl Pts',(66.8932790056263,1075.62719848133,343.501853998062));
#121024=CARTESIAN_POINT('Ctrl Pts',(66.8810979459664,1075.63327925175,343.56669291016));
#121025=CARTESIAN_POINT('Ctrl Pts',(66.8446327996808,1075.64306395291,343.657657305404));
#121026=CARTESIAN_POINT('Ctrl Pts',(66.8295081670838,1075.64641669883,343.686740724506));
#121027=CARTESIAN_POINT('Ctrl Pts',(66.7938191334769,1075.65319311943,343.74147932882));
#121028=CARTESIAN_POINT('Ctrl Pts',(66.7733449568916,1075.65660102139,343.767012808854));
#121029=CARTESIAN_POINT('Ctrl Pts',(66.7040105152463,1075.66687236542,343.837949850398));
#121030=CARTESIAN_POINT('Ctrl Pts',(66.6484158564627,1075.67355077613,343.875780188069));
#121031=CARTESIAN_POINT('Ctrl Pts',(66.5258839728004,1075.68567659138,343.927257184211));
#121032=CARTESIAN_POINT('Ctrl Pts',(66.4602034002325,1075.69101179288,343.940519062122));
#121033=CARTESIAN_POINT('Ctrl Pts',(66.3937896239309,1075.69533039084,343.940519062122));
#121034=CARTESIAN_POINT('Origin',(80.0774492048022,1067.7251047501,346.338481930687));
#121035=CARTESIAN_POINT('',(80.0774492048332,1076.71653899679,345.247941181959));
#121036=CARTESIAN_POINT('Ctrl Pts',(80.0774862161661,1076.9212633053,347.429022678787));
#121037=CARTESIAN_POINT('Ctrl Pts',(80.2021222418157,1076.90950098152,347.429018448822));
#121038=CARTESIAN_POINT('Ctrl Pts',(80.3256605239218,1076.89583373553,347.407650156297));
#121039=CARTESIAN_POINT('Ctrl Pts',(80.5699985990722,1076.86454049355,347.320777825101));
#121040=CARTESIAN_POINT('Ctrl Pts',(80.6876112503,1076.84693371904,347.252349941046));
#121041=CARTESIAN_POINT('Ctrl Pts',(80.8999983458895,1076.80940010752,347.069172492099));
#121042=CARTESIAN_POINT('Ctrl Pts',(80.9901724003361,1076.78975347167,346.952862829086));
#121043=CARTESIAN_POINT('Ctrl Pts',(81.1180192331078,1076.75293679588,346.694550975318));
#121044=CARTESIAN_POINT('Ctrl Pts',(81.1556736200037,1076.73605787768,346.555548346587));
#121045=CARTESIAN_POINT('Ctrl Pts',(81.1740311378466,1076.70871655558,346.287633171766));
#121046=CARTESIAN_POINT('Ctrl Pts',(81.1608924211059,1076.69793181172,346.161504102804));
#121047=CARTESIAN_POINT('Ctrl Pts',(81.0937106174324,1076.68187202188,345.925206689725));
#121048=CARTESIAN_POINT('Ctrl Pts',(81.0422696197197,1076.67645739526,345.816220218082));
#121049=CARTESIAN_POINT('Ctrl Pts',(80.954871778068,1076.67291909723,345.689987089237));
#121050=CARTESIAN_POINT('Ctrl Pts',(80.9344018195415,1076.67235413996,345.663168199325));
#121051=CARTESIAN_POINT('Ctrl Pts',(80.9001939403582,1076.67180071413,345.622416442801));
#121052=CARTESIAN_POINT('Ctrl Pts',(80.8872702293781,1076.67166965193,345.607832472062));
#121053=CARTESIAN_POINT('Ctrl Pts',(80.8638040799272,1076.6715650625,345.58273969905));
#121054=CARTESIAN_POINT('Ctrl Pts',(80.8534245708629,1076.67156160475,345.572086116607));
#121055=CARTESIAN_POINT('Ctrl Pts',(80.829272568673,1076.67164906389,345.548290179324));
#121056=CARTESIAN_POINT('Ctrl Pts',(80.8153676395287,1076.67176663643,345.535289719132));
#121057=CARTESIAN_POINT('Ctrl Pts',(80.7767076367494,1076.67227144132,345.500996081948));
#121058=CARTESIAN_POINT('Ctrl Pts',(80.7513272062193,1076.67279113894,345.480441759747));
#121059=CARTESIAN_POINT('Ctrl Pts',(80.6266659516045,1076.67620264786,345.388430654137));
#121060=CARTESIAN_POINT('Ctrl Pts',(80.5168429989352,1076.68166430112,345.332939718575));
#121061=CARTESIAN_POINT('Ctrl Pts',(80.2926834941226,1076.69698303526,345.263478914974));
#121062=CARTESIAN_POINT('Ctrl Pts',(80.1807647002479,1076.70636891199,345.247053057343));
#121063=CARTESIAN_POINT('Ctrl Pts',(79.9439600129226,1076.72967133889,345.249003870407));
#121064=CARTESIAN_POINT('Ctrl Pts',(79.8207213725019,1076.74379757481,345.271340812334));
#121065=CARTESIAN_POINT('Ctrl Pts',(79.5775385247131,1076.77578286523,345.359963177364));
#121066=CARTESIAN_POINT('Ctrl Pts',(79.4607415971847,1076.7935925419,345.429067615163));
#121067=CARTESIAN_POINT('Ctrl Pts',(79.2503495668522,1076.83111960669,345.613072547751));
#121068=CARTESIAN_POINT('Ctrl Pts',(79.1612564043964,1076.85052630989,345.729426103173));
#121069=CARTESIAN_POINT('Ctrl Pts',(79.0349882716665,1076.88662159092,345.987954979939));
#121070=CARTESIAN_POINT('Ctrl Pts',(78.9980559790793,1076.9030227927,346.127241921194));
#121071=CARTESIAN_POINT('Ctrl Pts',(78.981157704172,1076.92937822644,346.395425618788));
#121072=CARTESIAN_POINT('Ctrl Pts',(78.995011499467,1076.93967409601,346.52155125629));
#121073=CARTESIAN_POINT('Ctrl Pts',(79.063141240306,1076.95481244733,346.756110474455));
#121074=CARTESIAN_POINT('Ctrl Pts',(79.1143343080273,1076.95985541406,346.863543473075));
#121075=CARTESIAN_POINT('Ctrl Pts',(79.2009074300033,1076.96315645615,346.988150699005));
#121076=CARTESIAN_POINT('Ctrl Pts',(79.2212195178538,1076.96368449461,347.014696499386));
#121077=CARTESIAN_POINT('Ctrl Pts',(79.2551481772751,1076.96420162873,347.055052310515));
#121078=CARTESIAN_POINT('Ctrl Pts',(79.2679668532749,1076.96432402151,347.06950207222));
#121079=CARTESIAN_POINT('Ctrl Pts',(79.2912376489969,1076.96442142945,347.094370770387));
#121080=CARTESIAN_POINT('Ctrl Pts',(79.301529867698,1076.96442444433,347.104932015753));
#121081=CARTESIAN_POINT('Ctrl Pts',(79.325475171283,1076.96434204236,347.128526422866));
#121082=CARTESIAN_POINT('Ctrl Pts',(79.3392585456271,1076.96423166111,347.141420142427));
#121083=CARTESIAN_POINT('Ctrl Pts',(79.3775700528827,1076.96375815884,347.175438165737));
#121084=CARTESIAN_POINT('Ctrl Pts',(79.4027134025562,1076.96327100895,347.195837054384));
#121085=CARTESIAN_POINT('Ctrl Pts',(79.5260322643498,1076.96007646042,347.28709834934));
#121086=CARTESIAN_POINT('Ctrl Pts',(79.6345701952546,1076.95496847895,347.342346363548));
#121087=CARTESIAN_POINT('Ctrl Pts',(79.8559841104131,1076.94057462712,347.412081134828));
#121088=CARTESIAN_POINT('Ctrl Pts',(79.9664798597703,1076.93173935103,347.429026446181));
#121089=CARTESIAN_POINT('Ctrl Pts',(80.0774862161661,1076.9212633053,347.429022678787));
#121090=CARTESIAN_POINT('',(80.0774492048021,1074.69742129942,345.247941181958));
#121091=CARTESIAN_POINT('',(80.0774492048022,1067.7251047501,345.247941181958));
#121092=CARTESIAN_POINT('Ctrl Pts',(80.0781137458199,1074.9037808193,347.42902247694));
#121093=CARTESIAN_POINT('Ctrl Pts',(79.9334466289482,1074.91755562924,347.429110632519));
#121094=CARTESIAN_POINT('Ctrl Pts',(79.7899751621157,1074.9284898498,347.400411437874));
#121095=CARTESIAN_POINT('Ctrl Pts',(79.5254490843108,1074.94327057592,347.289612618674));
#121096=CARTESIAN_POINT('Ctrl Pts',(79.4065916812818,1074.94713161862,347.209891653313));
#121097=CARTESIAN_POINT('Ctrl Pts',(79.2060658521217,1074.94755442777,347.009346371445));
#121098=CARTESIAN_POINT('Ctrl Pts',(79.1264022916102,1074.9441185709,346.890598141408));
#121099=CARTESIAN_POINT('Ctrl Pts',(79.0166350565131,1074.93028306558,346.628703085767));
#121100=CARTESIAN_POINT('Ctrl Pts',(78.9879263739783,1074.91998207438,346.488070119579));
#121101=CARTESIAN_POINT('Ctrl Pts',(78.9859242803638,1074.89351348247,346.201340752291));
#121102=CARTESIAN_POINT('Ctrl Pts',(79.0137424215749,1074.87749855487,346.058069531191));
#121103=CARTESIAN_POINT('Ctrl Pts',(79.1235861989138,1074.84186845908,345.790323711697));
#121104=CARTESIAN_POINT('Ctrl Pts',(79.2048518700485,1074.82257431892,345.668524335293));
#121105=CARTESIAN_POINT('Ctrl Pts',(79.4108424343549,1074.78319878757,345.46313421656));
#121106=CARTESIAN_POINT('Ctrl Pts',(79.5339549215185,1074.76348460309,345.381790061626));
#121107=CARTESIAN_POINT('Ctrl Pts',(79.8037781608253,1074.72672636237,345.272957371469));
#121108=CARTESIAN_POINT('Ctrl Pts',(79.947699847112,1074.71000823119,345.245992427068));
#121109=CARTESIAN_POINT('Ctrl Pts',(80.2356656514258,1074.68204977285,345.250074345777));
#121110=CARTESIAN_POINT('Ctrl Pts',(80.3768755282356,1074.67099564023,345.280116708461));
#121111=CARTESIAN_POINT('Ctrl Pts',(80.6387431159376,1074.65598367746,345.392781516202));
#121112=CARTESIAN_POINT('Ctrl Pts',(80.7569490114497,1074.65211172391,345.473765989537));
#121113=CARTESIAN_POINT('Ctrl Pts',(80.9553827767437,1074.65206476887,345.676266937325));
#121114=CARTESIAN_POINT('Ctrl Pts',(81.0337311360745,1074.655860176,345.795555777806));
#121115=CARTESIAN_POINT('Ctrl Pts',(81.1407526310339,1074.67063283288,346.057762614982));
#121116=CARTESIAN_POINT('Ctrl Pts',(81.168134940995,1074.68149026881,346.198137657933));
#121117=CARTESIAN_POINT('Ctrl Pts',(81.1678423651269,1074.70888881994,346.482476047229));
#121118=CARTESIAN_POINT('Ctrl Pts',(81.1396252966577,1074.72521645264,346.623698286506));
#121119=CARTESIAN_POINT('Ctrl Pts',(81.0292947954484,1074.76148410104,346.890431916308));
#121120=CARTESIAN_POINT('Ctrl Pts',(80.9468371392338,1074.78115616437,347.01285012048));
#121121=CARTESIAN_POINT('Ctrl Pts',(80.7395671019805,1074.82055590851,347.217048915134));
#121122=CARTESIAN_POINT('Ctrl Pts',(80.6170155088918,1074.83991514004,347.297235108876));
#121123=CARTESIAN_POINT('Ctrl Pts',(80.3539046017529,1074.87501442923,347.402418178793));
#121124=CARTESIAN_POINT('Ctrl Pts',(80.2167606810137,1074.89057923471,347.42893798987));
#121125=CARTESIAN_POINT('Ctrl Pts',(80.0781137458199,1074.9037808193,347.42902247694));
#121126=CARTESIAN_POINT('Origin',(80.0774492048022,1067.7251047501,346.338481930687));
#121127=CARTESIAN_POINT('',(80.0774492048022,1074.84832662855,346.829022679415));
#121128=CARTESIAN_POINT('',(80.0774492048022,1074.75547652073,345.847941181958));
#121129=CARTESIAN_POINT('Ctrl Pts',(80.0774492048022,1074.84832662855,346.829022679415));
#121130=CARTESIAN_POINT('Ctrl Pts',(80.0448262837344,1074.85146078003,346.829022679415));
#121131=CARTESIAN_POINT('Ctrl Pts',(80.0121774599946,1074.85428931932,346.82576858999));
#121132=CARTESIAN_POINT('Ctrl Pts',(79.9173773701227,1074.86158169795,346.806551318557));
#121133=CARTESIAN_POINT('Ctrl Pts',(79.8577669540331,1074.86496734547,346.78173228012));
#121134=CARTESIAN_POINT('Ctrl Pts',(79.7516219069293,1074.86847995328,346.710670330104));
#121135=CARTESIAN_POINT('Ctrl Pts',(79.7060940777251,1074.86858860055,346.665259594229));
#121136=CARTESIAN_POINT('Ctrl Pts',(79.6348796406192,1074.86550463963,346.559470199017));
#121137=CARTESIAN_POINT('Ctrl Pts',(79.6099534868352,1074.86233716934,346.500139824643));
#121138=CARTESIAN_POINT('Ctrl Pts',(79.5840705163992,1074.85307807046,346.374918800676));
#121139=CARTESIAN_POINT('Ctrl Pts',(79.5835615662606,1074.84705566208,346.310230045752));
#121140=CARTESIAN_POINT('Ctrl Pts',(79.6075899148517,1074.83278916591,346.183118039608));
#121141=CARTESIAN_POINT('Ctrl Pts',(79.6324412816207,1074.82463920019,346.122027803914));
#121142=CARTESIAN_POINT('Ctrl Pts',(79.7045910480179,1074.80738198665,346.013072575906));
#121143=CARTESIAN_POINT('Ctrl Pts',(79.7512860855446,1074.79843440899,345.966284796809));
#121144=CARTESIAN_POINT('Ctrl Pts',(79.8604184380882,1074.78096377653,345.893695992609));
#121145=CARTESIAN_POINT('Ctrl Pts',(79.9218656775853,1074.77260759018,345.868640899455));
#121146=CARTESIAN_POINT('Ctrl Pts',(80.0164631193384,1074.76169513746,345.850792958124));
#121147=CARTESIAN_POINT('Ctrl Pts',(80.0469102527727,1074.75845540067,345.847941181958));
#121148=CARTESIAN_POINT('Ctrl Pts',(80.0774492048022,1074.75547652073,345.847941181958));
#121149=CARTESIAN_POINT('',(80.0774492048022,1082.7251047501,345.847941181958));
#121150=CARTESIAN_POINT('',(80.0774492048022,1067.7251047501,345.847941181958));
#121151=CARTESIAN_POINT('Origin',(80.0774492048022,1082.7251047501,346.338481930687));
#121152=CARTESIAN_POINT('Ctrl Pts',(80.0774492048022,1074.75547652073,345.847941181958));
#121153=CARTESIAN_POINT('Ctrl Pts',(80.0775388926569,1074.75546777226,345.847941181958));
#121154=CARTESIAN_POINT('Ctrl Pts',(80.0776285813035,1074.75545902603,345.847941206553));
#121155=CARTESIAN_POINT('Ctrl Pts',(80.077718270732,1074.75545028205,345.847941255749));
#121156=CARTESIAN_POINT('Ctrl Pts',(80.141896953241,1074.74919339174,345.847976458328));
#121157=CARTESIAN_POINT('Ctrl Pts',(80.2055508752481,1074.74417955805,345.860606346322));
#121158=CARTESIAN_POINT('Ctrl Pts',(80.3239842080001,1074.73728505508,345.90962237699));
#121159=CARTESIAN_POINT('Ctrl Pts',(80.3776497106477,1074.73544608304,345.945301405553));
#121160=CARTESIAN_POINT('Ctrl Pts',(80.4681858369132,1074.73518183834,346.0351519956));
#121161=CARTESIAN_POINT('Ctrl Pts',(80.5041882971281,1074.73674795505,346.088345403766));
#121162=CARTESIAN_POINT('Ctrl Pts',(80.5539774203366,1074.74309711386,346.205696589049));
#121163=CARTESIAN_POINT('Ctrl Pts',(80.567162622304,1074.74782998118,346.26871759626));
#121164=CARTESIAN_POINT('Ctrl Pts',(80.5687495278745,1074.75988222632,346.396699556429));
#121165=CARTESIAN_POINT('Ctrl Pts',(80.5568964923362,1074.76710791374,346.460424134477));
#121166=CARTESIAN_POINT('Ctrl Pts',(80.5088924221565,1074.78323359995,346.580959464777));
#121167=CARTESIAN_POINT('Ctrl Pts',(80.4726313521396,1074.7920133588,346.636404740842));
#121168=CARTESIAN_POINT('Ctrl Pts',(80.4041238268715,1074.80521790094,346.705819008354));
#121169=CARTESIAN_POINT('Ctrl Pts',(80.3794855574961,1074.80954079106,346.726331785911));
#121170=CARTESIAN_POINT('Ctrl Pts',(80.2990547436627,1074.82247169893,346.780948487007));
#121171=CARTESIAN_POINT('Ctrl Pts',(80.2382523658034,1074.83074194295,346.80650742751));
#121172=CARTESIAN_POINT('Ctrl Pts',(80.1422619523651,1074.84179563017,346.825808794145));
#121173=CARTESIAN_POINT('Ctrl Pts',(80.1098683705286,1074.84521205226,346.829022679415));
#121174=CARTESIAN_POINT('Ctrl Pts',(80.0774492048022,1074.84832662855,346.829022679415));
#121175=CARTESIAN_POINT('Origin',(22.5035000139866,1067.7251047501,337.93536030011));
#121176=CARTESIAN_POINT('',(22.5035000140068,1078.63105472707,336.457057167916));
#121177=CARTESIAN_POINT('Ctrl Pts',(22.5033438253408,1078.70463574344,339.413663424052));
#121178=CARTESIAN_POINT('Ctrl Pts',(22.6998393579387,1078.70375115027,339.413684184592));
#121179=CARTESIAN_POINT('Ctrl Pts',(22.8943758673387,1078.7021830175,339.374527560636));
#121180=CARTESIAN_POINT('Ctrl Pts',(23.2260457576551,1078.69795923647,339.235338949005));
#121181=CARTESIAN_POINT('Ctrl Pts',(23.3650392043164,1078.69555654171,339.147697921552));
#121182=CARTESIAN_POINT('Ctrl Pts',(23.6188702233219,1078.68952231744,338.921552645424));
#121183=CARTESIAN_POINT('Ctrl Pts',(23.7286905091169,1078.68584933042,338.781248797633));
#121184=CARTESIAN_POINT('Ctrl Pts',(23.8996139680247,1078.67729456531,338.457116205948));
#121185=CARTESIAN_POINT('Ctrl Pts',(23.9549739161666,1078.67241988861,338.273858498662));
#121186=CARTESIAN_POINT('Ctrl Pts',(23.993946068272,1078.66216121608,337.891234536368));
#121187=CARTESIAN_POINT('Ctrl Pts',(23.9751491699249,1078.65686956334,337.695303155037));
#121188=CARTESIAN_POINT('Ctrl Pts',(23.8647860477522,1078.64713360485,337.329217038423));
#121189=CARTESIAN_POINT('Ctrl Pts',(23.7770464117301,1078.64275882396,337.161668900629));
#121190=CARTESIAN_POINT('Ctrl Pts',(23.5377313979699,1078.63538889654,336.860870933825));
#121191=CARTESIAN_POINT('Ctrl Pts',(23.3855479512426,1078.63255547997,336.732794403445));
#121192=CARTESIAN_POINT('Ctrl Pts',(23.1537881881404,1078.63041906278,336.606067547748));
#121193=CARTESIAN_POINT('Ctrl Pts',(23.0927109542506,1078.63002173119,336.577890361605));
#121194=CARTESIAN_POINT('Ctrl Pts',(22.9925613722135,1078.62962914115,336.539724871977));
#121195=CARTESIAN_POINT('Ctrl Pts',(22.9546313787496,1078.6295363605,336.527006732112));
#121196=CARTESIAN_POINT('Ctrl Pts',(22.8826391492461,1078.62946389862,336.506074612261));
#121197=CARTESIAN_POINT('Ctrl Pts',(22.8487097479939,1078.62947153563,336.497502761961));
#121198=CARTESIAN_POINT('Ctrl Pts',(22.7727872377825,1078.6295804406,336.481164371475));
#121199=CARTESIAN_POINT('Ctrl Pts',(22.7306971316394,1078.62970188202,336.473996947489));
#121200=CARTESIAN_POINT('Ctrl Pts',(22.6102597817211,1078.63022070365,336.45881756648));
#121201=CARTESIAN_POINT('Ctrl Pts',(22.5315032163279,1078.63076385718,336.455228048553));
#121202=CARTESIAN_POINT('Ctrl Pts',(22.2564445706053,1078.63335212975,336.464659975376));
#121203=CARTESIAN_POINT('Ctrl Pts',(22.0633677201798,1078.63640804246,336.510485687278));
#121204=CARTESIAN_POINT('Ctrl Pts',(21.735934141379,1078.6436481339,336.661339136317));
#121205=CARTESIAN_POINT('Ctrl Pts',(21.5994184030165,1078.64750785798,336.754294071997));
#121206=CARTESIAN_POINT('Ctrl Pts',(21.3532341336299,1078.65616651653,336.990081719004));
#121207=CARTESIAN_POINT('Ctrl Pts',(21.2484887016351,1078.66094145711,337.134356113793));
#121208=CARTESIAN_POINT('Ctrl Pts',(21.0895331219666,1078.67075352981,337.464267130856));
#121209=CARTESIAN_POINT('Ctrl Pts',(21.0408757487221,1078.67569103634,337.649062160451));
#121210=CARTESIAN_POINT('Ctrl Pts',(21.0155710478685,1078.68487172237,338.032484083151));
#121211=CARTESIAN_POINT('Ctrl Pts',(21.0413204969999,1078.68900202211,338.227603192364));
#121212=CARTESIAN_POINT('Ctrl Pts',(21.1643989648315,1078.69582054318,338.588852624159));
#121213=CARTESIAN_POINT('Ctrl Pts',(21.2575618128547,1078.69850742647,338.7526047337));
#121214=CARTESIAN_POINT('Ctrl Pts',(21.498624319817,1078.70259042803,339.035239076157));
#121215=CARTESIAN_POINT('Ctrl Pts',(21.6438028711614,1078.70397036597,339.152090625918));
#121216=CARTESIAN_POINT('Ctrl Pts',(21.8639160723917,1078.70501767913,339.269719614016));
#121217=CARTESIAN_POINT('Ctrl Pts',(21.9230370295853,1078.70521343792,339.296479391541));
#121218=CARTESIAN_POINT('Ctrl Pts',(22.0203369658017,1078.70540677569,339.333023816273));
#121219=CARTESIAN_POINT('Ctrl Pts',(22.0574822187452,1078.70545205528,339.345317025429));
#121220=CARTESIAN_POINT('Ctrl Pts',(22.1279356211446,1078.7054856114,339.365570378957));
#121221=CARTESIAN_POINT('Ctrl Pts',(22.1611180321196,1078.70548032346,339.37387483295));
#121222=CARTESIAN_POINT('Ctrl Pts',(22.2359580776211,1078.70542160349,339.389868348979));
#121223=CARTESIAN_POINT('Ctrl Pts',(22.2777185955029,1078.70535704877,339.396933115691));
#121224=CARTESIAN_POINT('Ctrl Pts',(22.3806336989986,1078.70511991689,339.409827045523));
#121225=CARTESIAN_POINT('Ctrl Pts',(22.4419589121447,1078.70491208904,339.41365693849));
#121226=CARTESIAN_POINT('Ctrl Pts',(22.5033438253408,1078.70463574344,339.413663424052));
#121227=CARTESIAN_POINT('',(22.5035000139672,1076.62985213807,336.457057167916));
#121228=CARTESIAN_POINT('',(22.5035000139866,1067.7251047501,336.457057167916));
#121229=CARTESIAN_POINT('Ctrl Pts',(22.5035260490889,1076.70430235654,339.413663432074));
#121230=CARTESIAN_POINT('Ctrl Pts',(22.3076788371628,1076.70519520394,339.413666881233));
#121231=CARTESIAN_POINT('Ctrl Pts',(22.1137677330167,1076.70538754263,339.374750988217));
#121232=CARTESIAN_POINT('Ctrl Pts',(21.7527313031503,1076.70439216947,339.223748601578));
#121233=CARTESIAN_POINT('Ctrl Pts',(21.5891218480039,1076.70321411592,339.11328534297));
#121234=CARTESIAN_POINT('Ctrl Pts',(21.3147874457625,1076.69940261299,338.835542643899));
#121235=CARTESIAN_POINT('Ctrl Pts',(21.206597453164,1076.69680306849,338.671160869024));
#121236=CARTESIAN_POINT('Ctrl Pts',(21.0599426673985,1076.69013715911,338.30924466156));
#121237=CARTESIAN_POINT('Ctrl Pts',(21.0231932299689,1076.68612319168,338.115164727295));
#121238=CARTESIAN_POINT('Ctrl Pts',(21.0273720866854,1076.67693757734,337.723704893172));
#121239=CARTESIAN_POINT('Ctrl Pts',(21.0683744972371,1076.67185192883,337.530194015843));
#121240=CARTESIAN_POINT('Ctrl Pts',(21.2226910821344,1076.66132785084,337.172098605117));
#121241=CARTESIAN_POINT('Ctrl Pts',(21.3338390723428,1076.65599830827,337.010733148387));
#121242=CARTESIAN_POINT('Ctrl Pts',(21.6122223415557,1076.64599102733,336.740069375323));
#121243=CARTESIAN_POINT('Ctrl Pts',(21.7767966931952,1076.64141768865,336.633435040405));
#121244=CARTESIAN_POINT('Ctrl Pts',(22.1376408798258,1076.63399700659,336.489954508475));
#121245=CARTESIAN_POINT('Ctrl Pts',(22.3303783413942,1076.63122725497,336.45445156041));
#121246=CARTESIAN_POINT('Ctrl Pts',(22.7180943579612,1076.62813692179,336.459953621801));
#121247=CARTESIAN_POINT('Ctrl Pts',(22.9092997859577,1076.62784337958,336.500716264339));
#121248=CARTESIAN_POINT('Ctrl Pts',(23.2646560876052,1076.62981478918,336.653437586307));
#121249=CARTESIAN_POINT('Ctrl Pts',(23.4254392124878,1076.63205207791,336.763736146618));
#121250=CARTESIAN_POINT('Ctrl Pts',(23.6953603606003,1076.63857096145,337.039770842792));
#121251=CARTESIAN_POINT('Ctrl Pts',(23.801945903119,1076.64278211273,337.202804356312));
#121252=CARTESIAN_POINT('Ctrl Pts',(23.9465274573639,1076.65231326441,337.560737575826));
#121253=CARTESIAN_POINT('Ctrl Pts',(23.9830708203088,1076.65753584508,337.752231578144));
#121254=CARTESIAN_POINT('Ctrl Pts',(23.9811187188208,1076.66540907678,338.041903382089));
#121255=CARTESIAN_POINT('Ctrl Pts',(23.9710044060804,1076.6680227192,338.138189482373));
#121256=CARTESIAN_POINT('Ctrl Pts',(23.9321348193541,1076.67313785636,338.327424681259));
#121257=CARTESIAN_POINT('Ctrl Pts',(23.9034696544849,1076.67562702131,338.419919623396));
#121258=CARTESIAN_POINT('Ctrl Pts',(23.7899135097339,1076.68285475593,338.689654095926));
#121259=CARTESIAN_POINT('Ctrl Pts',(23.678644083091,1076.68719199501,338.853436943178));
#121260=CARTESIAN_POINT('Ctrl Pts',(23.3995246799656,1076.69454406291,339.127208323104));
#121261=CARTESIAN_POINT('Ctrl Pts',(23.2347606929472,1076.69750180075,339.234832374726));
#121262=CARTESIAN_POINT('Ctrl Pts',(22.878880550176,1076.70194543775,339.377585959403));
#121263=CARTESIAN_POINT('Ctrl Pts',(22.6920707453321,1076.70344280057,339.413660111523));
#121264=CARTESIAN_POINT('Ctrl Pts',(22.5035260490889,1076.70430235654,339.413663432074));
#121265=CARTESIAN_POINT('Origin',(22.5035000139866,1067.7251047501,337.93536030011));
#121266=CARTESIAN_POINT('',(22.5035000139866,1076.69297254634,338.813663432303));
#121267=CARTESIAN_POINT('',(22.5035000139359,1076.64871264505,337.057057167916));
#121268=CARTESIAN_POINT('Ctrl Pts',(22.5035000139866,1076.69297254634,338.813663432303));
#121269=CARTESIAN_POINT('Ctrl Pts',(22.3878767363282,1076.69359423243,338.813663432303));
#121270=CARTESIAN_POINT('Ctrl Pts',(22.2733708709006,1076.69373416697,338.790831450123));
#121271=CARTESIAN_POINT('Ctrl Pts',(22.0588653938933,1076.6930455795,338.701727736787));
#121272=CARTESIAN_POINT('Ctrl Pts',(21.9611437701684,1076.69221489214,338.635979444957));
#121273=CARTESIAN_POINT('Ctrl Pts',(21.7972022392667,1076.68960067082,338.47026886885));
#121274=CARTESIAN_POINT('Ctrl Pts',(21.7325714022931,1076.68784156337,338.37199507179));
#121275=CARTESIAN_POINT('Ctrl Pts',(21.6452933652732,1076.68348938718,338.15567604397));
#121276=CARTESIAN_POINT('Ctrl Pts',(21.6236359871019,1076.68093454894,338.039733910526));
#121277=CARTESIAN_POINT('Ctrl Pts',(21.6269271605318,1076.67528671955,337.806589730332));
#121278=CARTESIAN_POINT('Ctrl Pts',(21.651684659901,1076.67225026564,337.691698814802));
#121279=CARTESIAN_POINT('Ctrl Pts',(21.7440712650905,1076.66612043095,337.479336588598));
#121280=CARTESIAN_POINT('Ctrl Pts',(21.810373419722,1076.66308830352,337.383756695907));
#121281=CARTESIAN_POINT('Ctrl Pts',(21.9761262991321,1076.65748436421,337.223617330552));
#121282=CARTESIAN_POINT('Ctrl Pts',(22.0739834480995,1076.65496945098,337.160621496983));
#121283=CARTESIAN_POINT('Ctrl Pts',(22.2838754306421,1076.65100816475,337.077829047932));
#121284=CARTESIAN_POINT('Ctrl Pts',(22.3932172379869,1076.64955887,337.057057167929));
#121285=CARTESIAN_POINT('Ctrl Pts',(22.5035000138852,1076.64871264505,337.057057167917));
#121286=CARTESIAN_POINT('',(22.5035000139866,1082.7251047501,337.057057167916));
#121287=CARTESIAN_POINT('',(22.5035000139866,1067.7251047501,337.057057167916));
#121288=CARTESIAN_POINT('Origin',(22.5035000139866,1082.7251047501,337.93536030011));
#121289=CARTESIAN_POINT('Ctrl Pts',(22.5035000138852,1076.64871264505,337.057057167916));
#121290=CARTESIAN_POINT('Ctrl Pts',(22.5083455647385,1076.64867546403,337.057057167916));
#121291=CARTESIAN_POINT('Ctrl Pts',(22.5131929321026,1076.64863944285,337.057097266808));
#121292=CARTESIAN_POINT('Ctrl Pts',(22.633052817737,1076.64777788057,337.059081997554));
#121293=CARTESIAN_POINT('Ctrl Pts',(22.746577983698,1076.64762843378,337.08356157286));
#121294=CARTESIAN_POINT('Ctrl Pts',(22.9575589611612,1076.64870989134,337.174811135971));
#121295=CARTESIAN_POINT('Ctrl Pts',(23.0529995289714,1076.64992730021,337.240628668182));
#121296=CARTESIAN_POINT('Ctrl Pts',(23.2130964306104,1076.65350239392,337.405207037073));
#121297=CARTESIAN_POINT('Ctrl Pts',(23.2762234220587,1076.65582284456,337.502365674146));
#121298=CARTESIAN_POINT('Ctrl Pts',(23.3586278483235,1076.6609686024,337.708182993632));
#121299=CARTESIAN_POINT('Ctrl Pts',(23.3799111548858,1076.66370395421,337.813890257395));
#121300=CARTESIAN_POINT('Ctrl Pts',(23.381682622606,1076.66651885184,337.920810456847));
#121301=CARTESIAN_POINT('Ctrl Pts',(23.3826335120876,1076.66802983425,337.978203144207));
#121302=CARTESIAN_POINT('Ctrl Pts',(23.3779558593717,1076.66955366055,338.035551066894));
#121303=CARTESIAN_POINT('Ctrl Pts',(23.3574760532041,1076.67257789149,338.14852043641));
#121304=CARTESIAN_POINT('Ctrl Pts',(23.3417211491484,1076.67407102164,338.203870679632));
#121305=CARTESIAN_POINT('Ctrl Pts',(23.2777947269055,1076.67848416595,338.366141427581));
#121306=CARTESIAN_POINT('Ctrl Pts',(23.2135880123276,1076.68123002284,338.46534386836));
#121307=CARTESIAN_POINT('Ctrl Pts',(23.0504339278554,1076.68603251116,338.632390075667));
#121308=CARTESIAN_POINT('Ctrl Pts',(22.9532592893986,1076.68804699463,338.698712717894));
#121309=CARTESIAN_POINT('Ctrl Pts',(22.7386428959933,1076.69120466253,338.789590833938));
#121310=CARTESIAN_POINT('Ctrl Pts',(22.623326353342,1076.69231903148,338.813224537003));
#121311=CARTESIAN_POINT('Ctrl Pts',(22.5056741696389,1076.69296081386,338.813661414268));
#121312=CARTESIAN_POINT('Ctrl Pts',(22.5045870424311,1076.69296670158,338.813663432303));
#121313=CARTESIAN_POINT('Ctrl Pts',(22.5035000139866,1076.69297254634,338.813663432303));
#121314=CARTESIAN_POINT('Origin',(34.5096048204692,1067.7251047501,334.252491309441));
#121315=CARTESIAN_POINT('',(34.5096048204916,1078.26956110846,332.977047188305));
#121316=CARTESIAN_POINT('Ctrl Pts',(34.5096147511975,1078.42202229817,335.527935430539));
#121317=CARTESIAN_POINT('Ctrl Pts',(34.6788900809127,1078.41848212202,335.527934112545));
#121318=CARTESIAN_POINT('Ctrl Pts',(34.8464284900048,1078.4131107714,335.494234862051));
#121319=CARTESIAN_POINT('Ctrl Pts',(35.1359547877757,1078.40014346458,335.372934139495));
#121320=CARTESIAN_POINT('Ctrl Pts',(35.2589154610803,1078.39307233246,335.294707124768));
#121321=CARTESIAN_POINT('Ctrl Pts',(35.4818542978442,1078.37658785593,335.092666420833));
#121322=CARTESIAN_POINT('Ctrl Pts',(35.5773303002289,1078.36716823394,334.967405662373));
#121323=CARTESIAN_POINT('Ctrl Pts',(35.7235798016571,1078.34671690063,334.678196417761));
#121324=CARTESIAN_POINT('Ctrl Pts',(35.7690250311635,1078.33581296784,334.514829661878));
#121325=CARTESIAN_POINT('Ctrl Pts',(35.7939442785044,1078.31474731809,334.180726523008));
#121326=CARTESIAN_POINT('Ctrl Pts',(35.7735107608398,1078.30478590551,334.013217513336));
#121327=CARTESIAN_POINT('Ctrl Pts',(35.6732223167888,1078.28795050828,333.70797182205));
#121328=CARTESIAN_POINT('Ctrl Pts',(35.5989622077366,1078.28103732217,333.5714310054));
#121329=CARTESIAN_POINT('Ctrl Pts',(35.4155791059637,1078.27094007561,333.344226731133));
#121330=CARTESIAN_POINT('Ctrl Pts',(35.3122412652377,1078.26750497797,333.25172802105));
#121331=CARTESIAN_POINT('Ctrl Pts',(35.1553934425796,1078.26489491942,333.151561732247));
#121332=CARTESIAN_POINT('Ctrl Pts',(35.1132568748934,1078.26440402831,333.127905410159));
#121333=CARTESIAN_POINT('Ctrl Pts',(35.0431913814379,1078.26391702572,333.093644634156));
#121334=CARTESIAN_POINT('Ctrl Pts',(35.0160556824621,1078.26380335544,333.081531108159));
#121335=CARTESIAN_POINT('Ctrl Pts',(34.9637699943256,1078.26372442065,333.060348324321));
#121336=CARTESIAN_POINT('Ctrl Pts',(34.9387096191683,1078.2637453383,333.051100461356));
#121337=CARTESIAN_POINT('Ctrl Pts',(34.8814984999493,1078.26392411984,333.032006872119));
#121338=CARTESIAN_POINT('Ctrl Pts',(34.8492119449382,1078.26411591185,333.022631926122));
#121339=CARTESIAN_POINT('Ctrl Pts',(34.7531149081119,1078.26495074532,332.998801609938));
#121340=CARTESIAN_POINT('Ctrl Pts',(34.6885241418035,1078.26584788466,332.987967011555));
#121341=CARTESIAN_POINT('Ctrl Pts',(34.4540959154272,1078.27028355316,332.966968894671));
#121342=CARTESIAN_POINT('Ctrl Pts',(34.2835286720398,1078.27571016965,332.985803391606));
#121343=CARTESIAN_POINT('Ctrl Pts',(33.9875839019163,1078.28895387294,333.080280780492));
#121344=CARTESIAN_POINT('Ctrl Pts',(33.8615088215039,1078.29610909007,333.145003815832));
#121345=CARTESIAN_POINT('Ctrl Pts',(33.6263666062539,1078.31267232065,333.319836449441));
#121346=CARTESIAN_POINT('Ctrl Pts',(33.5214296212414,1078.32208286624,333.431854167036));
#121347=CARTESIAN_POINT('Ctrl Pts',(33.3500320209256,1078.34220280928,333.696781295865));
#121348=CARTESIAN_POINT('Ctrl Pts',(33.2884764937801,1078.35277145748,333.849659006327));
#121349=CARTESIAN_POINT('Ctrl Pts',(33.2254191467029,1078.37336833541,334.175263302984));
#121350=CARTESIAN_POINT('Ctrl Pts',(33.2264379303475,1078.38317088678,334.345296792578));
#121351=CARTESIAN_POINT('Ctrl Pts',(33.2930446394784,1078.40010063959,334.668064508785));
#121352=CARTESIAN_POINT('Ctrl Pts',(33.3552300229392,1078.40717753,334.818330797793));
#121353=CARTESIAN_POINT('Ctrl Pts',(33.5370927722223,1078.41866703403,335.095004549569));
#121354=CARTESIAN_POINT('Ctrl Pts',(33.6578343919329,1078.42280636336,335.216920579092));
#121355=CARTESIAN_POINT('Ctrl Pts',(33.8427374050399,1078.42572190528,335.34098853853));
#121356=CARTESIAN_POINT('Ctrl Pts',(33.8883070459096,1078.42622474696,335.367627096213));
#121357=CARTESIAN_POINT('Ctrl Pts',(33.9629561123523,1078.4267216759,335.405264287277));
#121358=CARTESIAN_POINT('Ctrl Pts',(33.9910117492956,1078.42684008769,335.418154900283));
#121359=CARTESIAN_POINT('Ctrl Pts',(34.0413320849543,1078.42693406491,335.439098731677));
#121360=CARTESIAN_POINT('Ctrl Pts',(34.0634049784836,1078.42693656199,335.447573830197));
#121361=CARTESIAN_POINT('Ctrl Pts',(34.1142066581152,1078.42685506576,335.465475852172));
#121362=CARTESIAN_POINT('Ctrl Pts',(34.1430605655501,1078.42674681612,335.474504603571));
#121363=CARTESIAN_POINT('Ctrl Pts',(34.2217440071173,1078.42628615239,335.49608784527));
#121364=CARTESIAN_POINT('Ctrl Pts',(34.2720544852055,1078.42581637568,335.506670602497));
#121365=CARTESIAN_POINT('Ctrl Pts',(34.3846975793669,1078.42437984733,335.523342615151));
#121366=CARTESIAN_POINT('Ctrl Pts',(34.4471161568302,1078.42332937601,335.527935917159));
#121367=CARTESIAN_POINT('Ctrl Pts',(34.5096147511975,1078.42202229817,335.527935430539));
#121368=CARTESIAN_POINT('',(34.5096048204403,1076.26445914773,332.977047188305));
#121369=CARTESIAN_POINT('',(34.5096048204692,1067.7251047501,332.977047188305));
#121370=CARTESIAN_POINT('Ctrl Pts',(34.5102109201886,1076.41849772182,335.527935286566));
#121371=CARTESIAN_POINT('Ctrl Pts',(34.340802513415,1076.42208285403,335.528015790602));
#121372=CARTESIAN_POINT('Ctrl Pts',(34.1730438365003,1076.42374639349,335.49434307368));
#121373=CARTESIAN_POINT('Ctrl Pts',(33.8605337398837,1076.42310943455,335.36341668331));
#121374=CARTESIAN_POINT('Ctrl Pts',(33.7189220406696,1076.42081641364,335.267504925686));
#121375=CARTESIAN_POINT('Ctrl Pts',(33.4818233026479,1076.41246193248,335.026393198278));
#121376=CARTESIAN_POINT('Ctrl Pts',(33.388563752612,1076.40649108723,334.883750708962));
#121377=CARTESIAN_POINT('Ctrl Pts',(33.2629400687953,1076.39142866753,334.5704421047));
#121378=CARTESIAN_POINT('Ctrl Pts',(33.2318666463486,1076.38247877826,334.402859557023));
#121379=CARTESIAN_POINT('Ctrl Pts',(33.2354824664854,1076.36766235584,334.151400656831));
#121380=CARTESIAN_POINT('Ctrl Pts',(33.2447238528446,1076.36258362599,334.068970626844));
#121381=CARTESIAN_POINT('Ctrl Pts',(33.2791157729686,1076.35212829543,333.906711076648));
#121382=CARTESIAN_POINT('Ctrl Pts',(33.3042586837665,1076.34677504228,333.827277996471));
#121383=CARTESIAN_POINT('Ctrl Pts',(33.4035232894238,1076.33040323854,333.59522743218));
#121384=CARTESIAN_POINT('Ctrl Pts',(33.5004296136776,1076.31941991101,333.454373892106));
#121385=CARTESIAN_POINT('Ctrl Pts',(33.7423609597917,1076.29894476336,333.21993421309));
#121386=CARTESIAN_POINT('Ctrl Pts',(33.8845533658297,1076.28963946483,333.12812963202));
#121387=CARTESIAN_POINT('Ctrl Pts',(34.1960783506563,1076.2740769255,333.004912336979));
#121388=CARTESIAN_POINT('Ctrl Pts',(34.3623240049718,1076.26796854383,332.9745620649));
#121389=CARTESIAN_POINT('Ctrl Pts',(34.6965963480527,1076.2599801983,332.979841362785));
#121390=CARTESIAN_POINT('Ctrl Pts',(34.8613404043709,1076.25816692957,333.015195519091));
#121391=CARTESIAN_POINT('Ctrl Pts',(35.1675090936512,1076.25915691969,333.147211945058));
#121392=CARTESIAN_POINT('Ctrl Pts',(35.3059899336232,1076.26193861752,333.242427561267));
#121393=CARTESIAN_POINT('Ctrl Pts',(35.5385438700153,1076.27166771401,333.480639647995));
#121394=CARTESIAN_POINT('Ctrl Pts',(35.6303460932242,1076.27851813776,333.621329378398));
#121395=CARTESIAN_POINT('Ctrl Pts',(35.7548949936911,1076.29523851775,333.930277026068));
#121396=CARTESIAN_POINT('Ctrl Pts',(35.7862914377388,1076.30495095122,334.095633422479));
#121397=CARTESIAN_POINT('Ctrl Pts',(35.7837278835445,1076.32579386364,334.429373808202));
#121398=CARTESIAN_POINT('Ctrl Pts',(35.7496234062969,1076.33672577133,334.594579542738));
#121399=CARTESIAN_POINT('Ctrl Pts',(35.6186724076319,1076.35843100728,334.904803232953));
#121400=CARTESIAN_POINT('Ctrl Pts',(35.5221498569416,1076.3689855776,335.046418752925));
#121401=CARTESIAN_POINT('Ctrl Pts',(35.2800739986142,1076.38812047267,335.282815051021));
#121402=CARTESIAN_POINT('Ctrl Pts',(35.1372193674678,1076.39652954069,335.37558137405));
#121403=CARTESIAN_POINT('Ctrl Pts',(34.8308026336779,1076.41000443043,335.497279305095));
#121404=CARTESIAN_POINT('Ctrl Pts',(34.6712631505156,1076.41508942852,335.527858753442));
#121405=CARTESIAN_POINT('Ctrl Pts',(34.5102109201886,1076.41849772182,335.527935286566));
#121406=CARTESIAN_POINT('Origin',(34.5096048204692,1067.7251047501,334.252491309441));
#121407=CARTESIAN_POINT('',(34.5096048204692,1076.38494400861,334.927935430577));
#121408=CARTESIAN_POINT('',(34.5096048204691,1076.30335139737,333.577047188305));
#121409=CARTESIAN_POINT('Ctrl Pts',(34.5096048204692,1076.38494400861,334.927935430577));
#121410=CARTESIAN_POINT('Ctrl Pts',(34.5076204863166,1076.38498777139,334.927935430577));
#121411=CARTESIAN_POINT('Ctrl Pts',(34.505635719696,1076.38503103526,334.927926686154));
#121412=CARTESIAN_POINT('Ctrl Pts',(34.4136515499107,1076.38701252793,334.927115786453));
#121413=CARTESIAN_POINT('Ctrl Pts',(34.3247019053225,1076.38788513909,334.908341647077));
#121414=CARTESIAN_POINT('Ctrl Pts',(34.1594034672164,1076.38741377614,334.837029001987));
#121415=CARTESIAN_POINT('Ctrl Pts',(34.0847309499407,1076.3860749365,334.785222161754));
#121416=CARTESIAN_POINT('Ctrl Pts',(33.960171830601,1076.38132376325,334.655508926247));
#121417=CARTESIAN_POINT('Ctrl Pts',(33.911510309296,1076.37796080277,334.578944121455));
#121418=CARTESIAN_POINT('Ctrl Pts',(33.846960452068,1076.36959080339,334.411256518578));
#121419=CARTESIAN_POINT('Ctrl Pts',(33.8317482226124,1076.3646644461,334.321796648458));
#121420=CARTESIAN_POINT('Ctrl Pts',(33.83580476543,1076.35661574422,334.188042091632));
#121421=CARTESIAN_POINT('Ctrl Pts',(33.8414312719777,1076.3538746385,334.144308576499));
#121422=CARTESIAN_POINT('Ctrl Pts',(33.8611295966575,1076.34827017143,334.058457123008));
#121423=CARTESIAN_POINT('Ctrl Pts',(33.8751765830277,1076.34541975035,334.016546567831));
#121424=CARTESIAN_POINT('Ctrl Pts',(33.9298550244792,1076.3367634241,333.894513470876));
#121425=CARTESIAN_POINT('Ctrl Pts',(33.9824256775183,1076.33102829037,333.820814073603));
#121426=CARTESIAN_POINT('Ctrl Pts',(34.1125602101747,1076.32045290633,333.698922122255));
#121427=CARTESIAN_POINT('Ctrl Pts',(34.1885855586371,1076.31570608637,333.651623978921));
#121428=CARTESIAN_POINT('Ctrl Pts',(34.347662912495,1076.30816746905,333.591731499172));
#121429=CARTESIAN_POINT('Ctrl Pts',(34.4282875005316,1076.30530761802,333.577047188305));
#121430=CARTESIAN_POINT('Ctrl Pts',(34.509604820469,1076.30335139737,333.577047188305));
#121431=CARTESIAN_POINT('',(34.5096048204692,1082.7251047501,333.577047188305));
#121432=CARTESIAN_POINT('',(34.5096048204692,1067.7251047501,333.577047188305));
#121433=CARTESIAN_POINT('Origin',(34.5096048204692,1082.7251047501,334.252491309441));
#121434=CARTESIAN_POINT('Ctrl Pts',(34.509604820469,1076.30335139737,333.577047188305));
#121435=CARTESIAN_POINT('Ctrl Pts',(34.5097104357425,1076.30334885662,333.577047188305));
#121436=CARTESIAN_POINT('Ctrl Pts',(34.5098160521846,1076.3033463174,333.577047213136));
#121437=CARTESIAN_POINT('Ctrl Pts',(34.5099216697866,1076.3033437797,333.577047262681));
#121438=CARTESIAN_POINT('Ctrl Pts',(34.5982697152156,1076.3012210189,333.577088706532));
#121439=CARTESIAN_POINT('Ctrl Pts',(34.6857691725621,1076.30020595607,333.594463525176));
#121440=CARTESIAN_POINT('Ctrl Pts',(34.8489964149025,1076.30052704744,333.66187938198));
#121441=CARTESIAN_POINT('Ctrl Pts',(34.9231439920578,1076.30185616366,333.711206804535));
#121442=CARTESIAN_POINT('Ctrl Pts',(35.0483053469897,1076.30667596252,333.835580321072));
#121443=CARTESIAN_POINT('Ctrl Pts',(35.0980858579031,1076.31012002537,333.909429616361));
#121444=CARTESIAN_POINT('Ctrl Pts',(35.1665194890139,1076.31863717469,334.072209307536));
#121445=CARTESIAN_POINT('Ctrl Pts',(35.1844379846351,1076.32363062344,334.159603982343));
#121446=CARTESIAN_POINT('Ctrl Pts',(35.1856305787911,1076.33446701535,334.336475996902));
#121447=CARTESIAN_POINT('Ctrl Pts',(35.1688126803986,1076.3402072694,334.424264869087));
#121448=CARTESIAN_POINT('Ctrl Pts',(35.1016905359036,1076.35174522374,334.589801169872));
#121449=CARTESIAN_POINT('Ctrl Pts',(35.051457375514,1076.35742799787,334.665705040811));
#121450=CARTESIAN_POINT('Ctrl Pts',(34.9243861831326,1076.36785261679,334.7930861097));
#121451=CARTESIAN_POINT('Ctrl Pts',(34.8489091855288,1076.37249601905,334.843397942504));
#121452=CARTESIAN_POINT('Ctrl Pts',(34.684486155862,1076.38009119671,334.9107908759));
#121453=CARTESIAN_POINT('Ctrl Pts',(34.5974694356268,1076.3830062301,334.927935430577));
#121454=CARTESIAN_POINT('Ctrl Pts',(34.5096048204692,1076.38494400861,334.927935430577));
#121455=CARTESIAN_POINT('Origin',(48.0649554680753,1067.7251047501,331.411589053766));
#121456=CARTESIAN_POINT('',(48.0649554680963,1077.56338652908,330.312757917773));
#121457=CARTESIAN_POINT('Ctrl Pts',(48.0649716197798,1077.7648831442,332.510420189639));
#121458=CARTESIAN_POINT('Ctrl Pts',(48.178352154084,1077.75970685431,332.51041852306));
#121459=CARTESIAN_POINT('Ctrl Pts',(48.2909673304275,1077.75299736048,332.492869337076));
#121460=CARTESIAN_POINT('Ctrl Pts',(48.5182099272391,1077.73608180198,332.420395537207));
#121461=CARTESIAN_POINT('Ctrl Pts',(48.6300971783606,1077.72570234581,332.362217480017));
#121462=CARTESIAN_POINT('Ctrl Pts',(48.8375449886251,1077.70183999985,332.204606627412));
#121463=CARTESIAN_POINT('Ctrl Pts',(48.9292536117016,1077.68837022053,332.103487055596));
#121464=CARTESIAN_POINT('Ctrl Pts',(49.076808191232,1077.6595310852,331.864194664782));
#121465=CARTESIAN_POINT('Ctrl Pts',(49.1278923488863,1077.64437043363,331.726036229211));
#121466=CARTESIAN_POINT('Ctrl Pts',(49.1727821420296,1077.61567136738,331.439938839538));
#121467=CARTESIAN_POINT('Ctrl Pts',(49.1670087823169,1077.6023817782,331.294844533771));
#121468=CARTESIAN_POINT('Ctrl Pts',(49.1030881065632,1077.58048206346,331.028806169293));
#121469=CARTESIAN_POINT('Ctrl Pts',(49.0506916953905,1077.5717112608,330.908968998611));
#121470=CARTESIAN_POINT('Ctrl Pts',(48.9137468474225,1077.55899518548,330.704082580428));
#121471=CARTESIAN_POINT('Ctrl Pts',(48.8339446140538,1077.55472994776,330.618054006717));
#121472=CARTESIAN_POINT('Ctrl Pts',(48.7118554226231,1077.55163429195,330.522533033387));
#121473=CARTESIAN_POINT('Ctrl Pts',(48.6804372721054,1077.55107968466,330.500500263895));
#121474=CARTESIAN_POINT('Ctrl Pts',(48.6284098270173,1077.5505342769,330.467936946777));
#121475=CARTESIAN_POINT('Ctrl Pts',(48.6085110774363,1077.55040687991,330.456336492958));
#121476=CARTESIAN_POINT('Ctrl Pts',(48.5721328957578,1077.55031714434,330.436633984257));
#121477=CARTESIAN_POINT('Ctrl Pts',(48.5557874136468,1077.55032651203,330.428303575575));
#121478=CARTESIAN_POINT('Ctrl Pts',(48.5172560827631,1077.55046276867,330.409866525129));
#121479=CARTESIAN_POINT('Ctrl Pts',(48.4949276757087,1077.55062723603,330.400081408223));
#121480=CARTESIAN_POINT('Ctrl Pts',(48.4312248328205,1077.55133327342,330.374655159362));
#121481=CARTESIAN_POINT('Ctrl Pts',(48.3892090526295,1077.55207222191,330.360758931861));
#121482=CARTESIAN_POINT('Ctrl Pts',(48.2053273015861,1077.5564524783,330.312021908459));
#121483=CARTESIAN_POINT('Ctrl Pts',(48.0582476593478,1077.5628157921,330.303147962668));
#121484=CARTESIAN_POINT('Ctrl Pts',(47.7960385763287,1077.57903617972,330.33955486139));
#121485=CARTESIAN_POINT('Ctrl Pts',(47.6817784495743,1077.58792245681,330.374910895428));
#121486=CARTESIAN_POINT('Ctrl Pts',(47.4595029378342,1077.60903606065,330.485501826043));
#121487=CARTESIAN_POINT('Ctrl Pts',(47.3547201557304,1077.62132926004,330.56321930683));
#121488=CARTESIAN_POINT('Ctrl Pts',(47.1703253790053,1077.6482429037,330.758551376419));
#121489=CARTESIAN_POINT('Ctrl Pts',(47.0948590130962,1077.66273278756,330.877055188268));
#121490=CARTESIAN_POINT('Ctrl Pts',(46.9898151758799,1077.69187966943,331.141904072517));
#121491=CARTESIAN_POINT('Ctrl Pts',(46.9635360839081,1077.70623475282,331.286757043586));
#121492=CARTESIAN_POINT('Ctrl Pts',(46.9690147760831,1077.73177127797,331.573235184765));
#121493=CARTESIAN_POINT('Ctrl Pts',(46.9986860515326,1077.74281768748,331.712185253558));
#121494=CARTESIAN_POINT('Ctrl Pts',(47.1056810555825,1077.7602775885,331.963615565543));
#121495=CARTESIAN_POINT('Ctrl Pts',(47.1791061162971,1077.76678995776,332.075112078044));
#121496=CARTESIAN_POINT('Ctrl Pts',(47.3189767550015,1077.7733420861,332.221422522343));
#121497=CARTESIAN_POINT('Ctrl Pts',(47.3719924400894,1077.77497059055,332.267229676188));
#121498=CARTESIAN_POINT('Ctrl Pts',(47.4536558318971,1077.77636730149,332.325184020711));
#121499=CARTESIAN_POINT('Ctrl Pts',(47.479011047914,1077.77666611122,332.341649425967));
#121500=CARTESIAN_POINT('Ctrl Pts',(47.5213221343044,1077.77695163752,332.366707850815));
#121501=CARTESIAN_POINT('Ctrl Pts',(47.5378779011577,1077.77701312378,332.375942915218));
#121502=CARTESIAN_POINT('Ctrl Pts',(47.5729061019401,1077.77703996846,332.394310551927));
#121503=CARTESIAN_POINT('Ctrl Pts',(47.5914130828635,1077.77699652618,332.403361065396));
#121504=CARTESIAN_POINT('Ctrl Pts',(47.6355333725391,1077.77675929222,332.423420667363));
#121505=CARTESIAN_POINT('Ctrl Pts',(47.6613322255803,1077.77651792696,332.433985616383));
#121506=CARTESIAN_POINT('Ctrl Pts',(47.7452564333032,1077.77540886323,332.464681620272));
#121507=CARTESIAN_POINT('Ctrl Pts',(47.8046708492155,1077.77413896231,332.480916341996));
#121508=CARTESIAN_POINT('Ctrl Pts',(47.9310591630673,1077.77044888337,332.504291375912));
#121509=CARTESIAN_POINT('Ctrl Pts',(47.9979557989091,1077.76794269333,332.510421174704));
#121510=CARTESIAN_POINT('Ctrl Pts',(48.0649716197798,1077.7648831442,332.510420189639));
#121511=CARTESIAN_POINT('',(48.0649554680754,1075.55153395083,330.312757917773));
#121512=CARTESIAN_POINT('',(48.0649554680753,1067.7251047501,330.312757917773));
#121513=CARTESIAN_POINT('Ctrl Pts',(48.0649874847738,1075.75487488712,332.510420189292));
#121514=CARTESIAN_POINT('Ctrl Pts',(47.9186934725305,1075.76161608273,332.510424451868));
#121515=CARTESIAN_POINT('Ctrl Pts',(47.77378732338,1075.76566123828,332.481212826068));
#121516=CARTESIAN_POINT('Ctrl Pts',(47.5067627381033,1075.76791600253,332.36886332233));
#121517=CARTESIAN_POINT('Ctrl Pts',(47.3868749072479,1075.76622817133,332.288026427572));
#121518=CARTESIAN_POINT('Ctrl Pts',(47.1828382832594,1075.75732351336,332.082895532957));
#121519=CARTESIAN_POINT('Ctrl Pts',(47.1015698117973,1075.75008447038,331.95986121963));
#121520=CARTESIAN_POINT('Ctrl Pts',(46.9919493351637,1075.73088939794,331.689650946595));
#121521=CARTESIAN_POINT('Ctrl Pts',(46.9646269580503,1075.71912894922,331.545217250679));
#121522=CARTESIAN_POINT('Ctrl Pts',(46.9677551381208,1075.69247091493,331.253735442318));
#121523=CARTESIAN_POINT('Ctrl Pts',(46.998428562372,1075.67781839374,331.109531855694));
#121524=CARTESIAN_POINT('Ctrl Pts',(47.0847385615665,1075.65527800369,330.909857236068));
#121525=CARTESIAN_POINT('Ctrl Pts',(47.119517409326,1075.64779663082,330.847047921984));
#121526=CARTESIAN_POINT('Ctrl Pts',(47.2430714473924,1075.62519853705,330.667756621868));
#121527=CARTESIAN_POINT('Ctrl Pts',(47.3492014365594,1075.61044739057,330.565111949947));
#121528=CARTESIAN_POINT('Ctrl Pts',(47.5939727676699,1075.58376638424,330.408369154433));
#121529=CARTESIAN_POINT('Ctrl Pts',(47.7298416619558,1075.57205931713,330.355153140756));
#121530=CARTESIAN_POINT('Ctrl Pts',(48.0138021853828,1075.55328624887,330.304574479363));
#121531=CARTESIAN_POINT('Ctrl Pts',(48.1590369585093,1075.54637812743,330.307363022654));
#121532=CARTESIAN_POINT('Ctrl Pts',(48.4396166961066,1075.53838981627,330.368723946942));
#121533=CARTESIAN_POINT('Ctrl Pts',(48.5722161574972,1075.53735884485,330.426380120262));
#121534=CARTESIAN_POINT('Ctrl Pts',(48.8076871283584,1075.54133536622,330.589247538962));
#121535=CARTESIAN_POINT('Ctrl Pts',(48.9082472702065,1075.54629435517,330.692768456006));
#121536=CARTESIAN_POINT('Ctrl Pts',(49.064329507079,1075.56153603297,330.93278602151));
#121537=CARTESIAN_POINT('Ctrl Pts',(49.1181445935129,1075.57168658861,331.067044682633));
#121538=CARTESIAN_POINT('Ctrl Pts',(49.1714343129085,1075.5958042192,331.349249458987));
#121539=CARTESIAN_POINT('Ctrl Pts',(49.170049411285,1075.60956112074,331.494569515375));
#121540=CARTESIAN_POINT('Ctrl Pts',(49.1260696578948,1075.63144476061,331.705978096679));
#121541=CARTESIAN_POINT('Ctrl Pts',(49.1044752427592,1075.63890669277,331.774940051196));
#121542=CARTESIAN_POINT('Ctrl Pts',(49.0482183160794,1075.65388793986,331.907348066901));
#121543=CARTESIAN_POINT('Ctrl Pts',(49.0137391194163,1075.66137241396,331.970510972076));
#121544=CARTESIAN_POINT('Ctrl Pts',(48.8913182184056,1075.68375750389,332.150376217104));
#121545=CARTESIAN_POINT('Ctrl Pts',(48.7860710315865,1075.69813484908,332.253449521655));
#121546=CARTESIAN_POINT('Ctrl Pts',(48.5417130443118,1075.72398963666,332.412232229124));
#121547=CARTESIAN_POINT('Ctrl Pts',(48.4051043623622,1075.73522779827,332.466560848604));
#121548=CARTESIAN_POINT('Ctrl Pts',(48.1968430398588,1075.74826246404,332.504468511868));
#121549=CARTESIAN_POINT('Ctrl Pts',(48.1309961998813,1075.75183322017,332.510418265992));
#121550=CARTESIAN_POINT('Ctrl Pts',(48.0649874847738,1075.75487488712,332.510420189292));
#121551=CARTESIAN_POINT('Origin',(48.0649554680753,1067.7251047501,331.411589053766));
#121552=CARTESIAN_POINT('',(48.0649554680753,1075.70120171291,331.910420189758));
#121553=CARTESIAN_POINT('',(48.0649554680763,1075.60888786087,330.912757917773));
#121554=CARTESIAN_POINT('Ctrl Pts',(48.0649554680753,1075.70120171291,331.910420189758));
#121555=CARTESIAN_POINT('Ctrl Pts',(48.0306710331432,1075.7028123358,331.910420189758));
#121556=CARTESIAN_POINT('Ctrl Pts',(47.9963809644694,1075.70409991635,331.906885757966));
#121557=CARTESIAN_POINT('Ctrl Pts',(47.899017501197,1075.7068113055,331.886480708058));
#121558=CARTESIAN_POINT('Ctrl Pts',(47.838605396802,1075.70731189829,331.860839012816));
#121559=CARTESIAN_POINT('Ctrl Pts',(47.7309687707835,1075.70571568726,331.787780017816));
#121560=CARTESIAN_POINT('Ctrl Pts',(47.6848282042222,1075.70363260956,331.741074234883));
#121561=CARTESIAN_POINT('Ctrl Pts',(47.6129305960903,1075.6971102356,331.63242461102));
#121562=CARTESIAN_POINT('Ctrl Pts',(47.5879750129836,1075.6927246489,331.571489610806));
#121563=CARTESIAN_POINT('Ctrl Pts',(47.5626553064818,1075.68209624682,331.442322121797));
#121564=CARTESIAN_POINT('Ctrl Pts',(47.5630437078385,1075.67592344304,331.375255516538));
#121565=CARTESIAN_POINT('Ctrl Pts',(47.5831174809899,1075.66605577145,331.278472134671));
#121566=CARTESIAN_POINT('Ctrl Pts',(47.5928059226919,1075.66272723371,331.247388089204));
#121567=CARTESIAN_POINT('Ctrl Pts',(47.6181011662297,1075.65598822601,331.187509268941));
#121568=CARTESIAN_POINT('Ctrl Pts',(47.6336593298329,1075.65259309782,331.158855648727));
#121569=CARTESIAN_POINT('Ctrl Pts',(47.6893341221625,1075.64230630239,331.076625907071));
#121570=CARTESIAN_POINT('Ctrl Pts',(47.7375191470671,1075.63559657088,331.029375263062));
#121571=CARTESIAN_POINT('Ctrl Pts',(47.8485629393243,1075.62353502493,330.957392611238));
#121572=CARTESIAN_POINT('Ctrl Pts',(47.9100422347544,1075.61827364809,330.932904458574));
#121573=CARTESIAN_POINT('Ctrl Pts',(48.0043710097193,1075.61208154299,330.915523963248));
#121574=CARTESIAN_POINT('Ctrl Pts',(48.0346206392831,1075.61035734689,330.912757917773));
#121575=CARTESIAN_POINT('Ctrl Pts',(48.0649554680778,1075.60888786087,330.912757917773));
#121576=CARTESIAN_POINT('',(48.0649554680753,1082.7251047501,330.912757917773));
#121577=CARTESIAN_POINT('',(48.0649554680753,1067.7251047501,330.912757917773));
#121578=CARTESIAN_POINT('Origin',(48.0649554680753,1082.7251047501,331.411589053766));
#121579=CARTESIAN_POINT('Ctrl Pts',(48.0649636762499,1075.60888746326,330.912757917841));
#121580=CARTESIAN_POINT('Ctrl Pts',(48.1300654628176,1075.60573388934,330.912758989078));
#121581=CARTESIAN_POINT('Ctrl Pts',(48.1945770351577,1075.60380209979,330.925504507233));
#121582=CARTESIAN_POINT('Ctrl Pts',(48.3149247369696,1075.60262406827,330.975046456933));
#121583=CARTESIAN_POINT('Ctrl Pts',(48.3695851031577,1075.60338155543,331.011275263444));
#121584=CARTESIAN_POINT('Ctrl Pts',(48.462007986295,1075.60749709355,331.102697530493));
#121585=CARTESIAN_POINT('Ctrl Pts',(48.4988235568122,1075.61081819815,331.157013265499));
#121586=CARTESIAN_POINT('Ctrl Pts',(48.54968213026,1075.61960069567,331.276917082956));
#121587=CARTESIAN_POINT('Ctrl Pts',(48.5631047536,1075.624987281,331.34139428124));
#121588=CARTESIAN_POINT('Ctrl Pts',(48.5644345106547,1075.63723543239,331.473389224999));
#121589=CARTESIAN_POINT('Ctrl Pts',(48.5516724214059,1075.64400915804,331.539635813471));
#121590=CARTESIAN_POINT('Ctrl Pts',(48.5138825399483,1075.65432757827,331.631492619645));
#121591=CARTESIAN_POINT('Ctrl Pts',(48.4985721202037,1075.65772548985,331.660325500007));
#121592=CARTESIAN_POINT('Ctrl Pts',(48.4438364840096,1075.66794837201,331.742785713353));
#121593=CARTESIAN_POINT('Ctrl Pts',(48.396409921061,1075.67456732752,331.790258573698));
#121594=CARTESIAN_POINT('Ctrl Pts',(48.2857635303348,1075.68654875824,331.863784226594));
#121595=CARTESIAN_POINT('Ctrl Pts',(48.2236579472687,1075.69179636756,331.889153178431));
#121596=CARTESIAN_POINT('Ctrl Pts',(48.1274943987379,1075.69799473505,331.907479517654));
#121597=CARTESIAN_POINT('Ctrl Pts',(48.0962272775363,1075.69973261789,331.910420189758));
#121598=CARTESIAN_POINT('Ctrl Pts',(48.0649554680753,1075.70120171291,331.910420189758));
#121599=CARTESIAN_POINT('Origin',(62.0518715958009,1067.7251047501,331.400088359109));
#121600=CARTESIAN_POINT('',(62.0518715958319,1076.69664647652,330.309547610381));
#121601=CARTESIAN_POINT('Ctrl Pts',(62.051916276496,1076.94042940536,332.490629106922));
#121602=CARTESIAN_POINT('Ctrl Pts',(62.1689467597441,1076.9319000034,332.49062431205));
#121603=CARTESIAN_POINT('Ctrl Pts',(62.2850515643844,1076.92135625036,332.471782941714));
#121604=CARTESIAN_POINT('Ctrl Pts',(62.5175406903148,1076.89581200022,332.394515759891));
#121605=CARTESIAN_POINT('Ctrl Pts',(62.6310201944877,1076.88066974096,332.33295422707));
#121606=CARTESIAN_POINT('Ctrl Pts',(62.8394604484178,1076.846863144,332.167003639001));
#121607=CARTESIAN_POINT('Ctrl Pts',(62.930330983206,1076.82830242782,332.06094370315));
#121608=CARTESIAN_POINT('Ctrl Pts',(63.0708677040734,1076.79026494312,331.814790810824));
#121609=CARTESIAN_POINT('Ctrl Pts',(63.1169988033058,1076.77114287074,331.675589569795));
#121610=CARTESIAN_POINT('Ctrl Pts',(63.1513190413059,1076.73657033434,331.392472888326));
#121611=CARTESIAN_POINT('Ctrl Pts',(63.1413081417149,1076.72131894172,331.251450726646));
#121612=CARTESIAN_POINT('Ctrl Pts',(63.0720818267986,1076.69736837096,330.994895270063));
#121613=CARTESIAN_POINT('Ctrl Pts',(63.0187160747209,1076.68832780491,330.88017768393));
#121614=CARTESIAN_POINT('Ctrl Pts',(62.899835283627,1076.67786000366,330.709430009114));
#121615=CARTESIAN_POINT('Ctrl Pts',(62.8452953736487,1076.67491669758,330.647397028657));
#121616=CARTESIAN_POINT('Ctrl Pts',(62.7615123585332,1076.67260892928,330.571456052561));
#121617=CARTESIAN_POINT('Ctrl Pts',(62.7379046939632,1076.67215873912,330.551807495784));
#121618=CARTESIAN_POINT('Ctrl Pts',(62.6977604198812,1076.67171059519,330.521169333621));
#121619=CARTESIAN_POINT('Ctrl Pts',(62.6816990465148,1076.67160888888,330.50958937468));
#121620=CARTESIAN_POINT('Ctrl Pts',(62.6500336421708,1076.67155548727,330.488044703156));
#121621=CARTESIAN_POINT('Ctrl Pts',(62.6344739316891,1076.67159442429,330.478027637488));
#121622=CARTESIAN_POINT('Ctrl Pts',(62.5978413736133,1076.67183458392,330.455741838846));
#121623=CARTESIAN_POINT('Ctrl Pts',(62.5765977291325,1076.67208333596,330.443774746252));
#121624=CARTESIAN_POINT('Ctrl Pts',(62.5091956281057,1076.67320688124,330.408727739606));
#121625=CARTESIAN_POINT('Ctrl Pts',(62.4617984909764,1076.67446909744,330.388209592741));
#121626=CARTESIAN_POINT('Ctrl Pts',(62.2769377920682,1076.68111883128,330.323305189534));
#121627=CARTESIAN_POINT('Ctrl Pts',(62.1327875076142,1076.6897742696,330.303065934061));
#121628=CARTESIAN_POINT('Ctrl Pts',(61.8702586788995,1076.71140682714,330.318211972485));
#121629=CARTESIAN_POINT('Ctrl Pts',(61.7535533797444,1076.72322357857,330.344452723208));
#121630=CARTESIAN_POINT('Ctrl Pts',(61.5232586626982,1076.75112863505,330.437451679091));
#121631=CARTESIAN_POINT('Ctrl Pts',(61.4127560950302,1076.76729379384,330.507026288529));
#121632=CARTESIAN_POINT('Ctrl Pts',(61.2139210672944,1076.80255994862,330.688314858694));
#121633=CARTESIAN_POINT('Ctrl Pts',(61.1297600389307,1076.82148441762,330.801351381263));
#121634=CARTESIAN_POINT('Ctrl Pts',(61.0064643877677,1076.85917076983,331.057543244206));
#121635=CARTESIAN_POINT('Ctrl Pts',(60.9702207203452,1076.87755070318,331.199251640443));
#121636=CARTESIAN_POINT('Ctrl Pts',(60.9556738464336,1076.90983274036,331.482017924519));
#121637=CARTESIAN_POINT('Ctrl Pts',(60.9748427048558,1076.92362227454,331.620293430687));
#121638=CARTESIAN_POINT('Ctrl Pts',(61.0621953451036,1076.94537653608,331.876936286487));
#121639=CARTESIAN_POINT('Ctrl Pts',(61.1274646747224,1076.95338504239,331.9937210282));
#121640=CARTESIAN_POINT('Ctrl Pts',(61.2509721729956,1076.96067487758,332.142734368523));
#121641=CARTESIAN_POINT('Ctrl Pts',(61.2935487614635,1076.96232006156,332.186163227701));
#121642=CARTESIAN_POINT('Ctrl Pts',(61.3597305078431,1076.96374168654,332.24325583806));
#121643=CARTESIAN_POINT('Ctrl Pts',(61.3805621655427,1076.96404818618,332.259933980456));
#121644=CARTESIAN_POINT('Ctrl Pts',(61.4155782452409,1076.96433999831,332.285919270919));
#121645=CARTESIAN_POINT('Ctrl Pts',(61.4294040470271,1076.96440171869,332.295688603362));
#121646=CARTESIAN_POINT('Ctrl Pts',(61.4588680779628,1076.96442293528,332.315495929317));
#121647=CARTESIAN_POINT('Ctrl Pts',(61.4745465235254,1076.96437188357,332.325463927271));
#121648=CARTESIAN_POINT('Ctrl Pts',(61.5123307337301,1076.96410340793,332.348152111356));
#121649=CARTESIAN_POINT('Ctrl Pts',(61.534642267143,1076.96383117136,332.360506455053));
#121650=CARTESIAN_POINT('Ctrl Pts',(61.6090517280108,1076.96255840619,332.398363215552));
#121651=CARTESIAN_POINT('Ctrl Pts',(61.662740225478,1076.9610741055,332.420488006479));
#121652=CARTESIAN_POINT('Ctrl Pts',(61.8259551604238,1076.95494829649,332.472991398032));
#121653=CARTESIAN_POINT('Ctrl Pts',(61.9386477587942,1076.94868462819,332.490633747662));
#121654=CARTESIAN_POINT('Ctrl Pts',(62.051916276496,1076.94042940536,332.490629106922));
#121655=CARTESIAN_POINT('',(62.0518715958011,1074.67736588017,330.309547610381));
#121656=CARTESIAN_POINT('',(62.0518715958009,1067.7251047501,330.309547610381));
#121657=CARTESIAN_POINT('Ctrl Pts',(62.0518920858522,1074.9231689021,332.490629107645));
#121658=CARTESIAN_POINT('Ctrl Pts',(61.9072766880482,1074.9337967205,332.490631824808));
#121659=CARTESIAN_POINT('Ctrl Pts',(61.7639282422094,1074.94112803438,332.461868316459));
#121660=CARTESIAN_POINT('Ctrl Pts',(61.4996256396725,1074.94829122717,332.35107001861));
#121661=CARTESIAN_POINT('Ctrl Pts',(61.3809087112088,1074.9482181156,332.271380194124));
#121662=CARTESIAN_POINT('Ctrl Pts',(61.1803663694778,1074.94084440522,332.070843453706));
#121663=CARTESIAN_POINT('Ctrl Pts',(61.100660326611,1074.93360139843,331.951939984251));
#121664=CARTESIAN_POINT('Ctrl Pts',(60.9899959889945,1074.91255576933,331.687646155658));
#121665=CARTESIAN_POINT('Ctrl Pts',(60.9613228924259,1074.89882163901,331.544430066913));
#121666=CARTESIAN_POINT('Ctrl Pts',(60.9613388548559,1074.86660946104,331.254722168143));
#121667=CARTESIAN_POINT('Ctrl Pts',(60.9903839082085,1074.84841713424,331.111065437832));
#121668=CARTESIAN_POINT('Ctrl Pts',(61.0741556946148,1074.8198039495,330.911805339064));
#121669=CARTESIAN_POINT('Ctrl Pts',(61.1081062745881,1074.81020402191,330.849042381779));
#121670=CARTESIAN_POINT('Ctrl Pts',(61.2299476471322,1074.78070840419,330.668499216895));
#121671=CARTESIAN_POINT('Ctrl Pts',(61.3357050178387,1074.76096641421,330.564660631712));
#121672=CARTESIAN_POINT('Ctrl Pts',(61.5795997859539,1074.72451459745,330.406653089535));
#121673=CARTESIAN_POINT('Ctrl Pts',(61.7147457076355,1074.70809339683,330.352983008506));
#121674=CARTESIAN_POINT('Ctrl Pts',(61.9971928860336,1074.68064821233,330.301591792456));
#121675=CARTESIAN_POINT('Ctrl Pts',(62.1416183696132,1074.66984339509,330.303841104559));
#121676=CARTESIAN_POINT('Ctrl Pts',(62.4203883616412,1074.65539081775,330.363939536672));
#121677=CARTESIAN_POINT('Ctrl Pts',(62.5520072922979,1074.65182117772,330.42063815083));
#121678=CARTESIAN_POINT('Ctrl Pts',(62.7857347125334,1074.65238493327,330.581104864286));
#121679=CARTESIAN_POINT('Ctrl Pts',(62.8855793518802,1074.65648012115,330.683035833256));
#121680=CARTESIAN_POINT('Ctrl Pts',(63.0410814226853,1074.67180421789,330.919606615128));
#121681=CARTESIAN_POINT('Ctrl Pts',(63.0949950473784,1074.68290651985,331.052000355747));
#121682=CARTESIAN_POINT('Ctrl Pts',(63.1495440183203,1074.71070786131,331.330909671221));
#121683=CARTESIAN_POINT('Ctrl Pts',(63.149121740666,1074.72718943165,331.474850097114));
#121684=CARTESIAN_POINT('Ctrl Pts',(63.092896486172,1074.76334686442,331.755324436365));
#121685=CARTESIAN_POINT('Ctrl Pts',(63.0371047486052,1074.78271234783,331.889164603409));
#121686=CARTESIAN_POINT('Ctrl Pts',(62.8759167863411,1074.82184081789,332.129056530396));
#121687=CARTESIAN_POINT('Ctrl Pts',(62.7713671965666,1074.84123833865,332.232454513835));
#121688=CARTESIAN_POINT('Ctrl Pts',(62.5285877224576,1074.87703484017,332.391508195153));
#121689=CARTESIAN_POINT('Ctrl Pts',(62.3929410695632,1074.89311730865,332.446020732886));
#121690=CARTESIAN_POINT('Ctrl Pts',(62.1849547481319,1074.91270964417,332.484520659806));
#121691=CARTESIAN_POINT('Ctrl Pts',(62.1185199715278,1074.91827240366,332.490627855781));
#121692=CARTESIAN_POINT('Ctrl Pts',(62.0518920858522,1074.9231689021,332.490629107645));
#121693=CARTESIAN_POINT('Origin',(62.0518715958009,1067.7251047501,331.400088359109));
#121694=CARTESIAN_POINT('',(62.0518715958009,1074.85711166046,331.890629107838));
#121695=CARTESIAN_POINT('',(62.0518715957995,1074.74654397689,330.909547610381));
#121696=CARTESIAN_POINT('Ctrl Pts',(62.051871595801,1074.85711166046,331.890629107838));
#121697=CARTESIAN_POINT('Ctrl Pts',(62.0508414461873,1074.85718823713,331.890629107838));
#121698=CARTESIAN_POINT('Ctrl Pts',(62.0498111098117,1074.8572644638,331.890625862824));
#121699=CARTESIAN_POINT('Ctrl Pts',(61.9842804536085,1074.8620894158,331.890212932986));
#121700=CARTESIAN_POINT('Ctrl Pts',(61.9204148249089,1074.86536582664,331.877088205641));
#121701=CARTESIAN_POINT('Ctrl Pts',(61.8021903547936,1074.86856750923,331.827110421472));
#121702=CARTESIAN_POINT('Ctrl Pts',(61.7489041167558,1074.86850855109,331.791111240611));
#121703=CARTESIAN_POINT('Ctrl Pts',(61.659006187408,1074.86509854825,331.700684959973));
#121704=CARTESIAN_POINT('Ctrl Pts',(61.6233336316729,1074.86177673475,331.64714692349));
#121705=CARTESIAN_POINT('Ctrl Pts',(61.5737682166001,1074.85214402318,331.527897368748));
#121706=CARTESIAN_POINT('Ctrl Pts',(61.561038995203,1074.84584993916,331.46311795312));
#121707=CARTESIAN_POINT('Ctrl Pts',(61.5616343725284,1074.83114636991,331.33226118111));
#121708=CARTESIAN_POINT('Ctrl Pts',(61.5750848572269,1074.82287118521,331.267471907523));
#121709=CARTESIAN_POINT('Ctrl Pts',(61.6134133509576,1074.80991482127,331.177795982349));
#121710=CARTESIAN_POINT('Ctrl Pts',(61.6288841399801,1074.80558139531,331.149607902732));
#121711=CARTESIAN_POINT('Ctrl Pts',(61.684147017624,1074.79232851443,331.068818318877));
#121712=CARTESIAN_POINT('Ctrl Pts',(61.7318809974185,1074.78350501292,331.022492357096));
#121713=CARTESIAN_POINT('Ctrl Pts',(61.8421902947146,1074.76719952519,330.951870066679));
#121714=CARTESIAN_POINT('Ctrl Pts',(61.9035280093915,1074.75985750452,330.927979432424));
#121715=CARTESIAN_POINT('Ctrl Pts',(61.9955737695265,1074.75108054626,330.911977110688));
#121716=CARTESIAN_POINT('Ctrl Pts',(62.0236815926941,1074.74867782624,330.909548068142));
#121717=CARTESIAN_POINT('Ctrl Pts',(62.0518636290663,1074.74654457992,330.909547610446));
#121718=CARTESIAN_POINT('',(62.0518715958009,1082.7251047501,330.909547610381));
#121719=CARTESIAN_POINT('',(62.0518715958009,1067.7251047501,330.909547610381));
#121720=CARTESIAN_POINT('Origin',(62.0518715958009,1082.7251047501,331.400088359109));
#121721=CARTESIAN_POINT('Ctrl Pts',(62.0518715957962,1074.74654397689,330.909547610381));
#121722=CARTESIAN_POINT('Ctrl Pts',(62.115868350468,1074.74169984421,330.90954761038));
#121723=CARTESIAN_POINT('Ctrl Pts',(62.179320075241,1074.73831573489,330.92206916904));
#121724=CARTESIAN_POINT('Ctrl Pts',(62.2975373009314,1074.73489722521,330.970744933648));
#121725=CARTESIAN_POINT('Ctrl Pts',(62.3511527164464,1074.73487485355,331.00623768826));
#121726=CARTESIAN_POINT('Ctrl Pts',(62.4418284087802,1074.73819498118,331.095747096567));
#121727=CARTESIAN_POINT('Ctrl Pts',(62.4779637585687,1074.74150435431,331.148858725687));
#121728=CARTESIAN_POINT('Ctrl Pts',(62.5281132346037,1074.7510522655,331.266201330322));
#121729=CARTESIAN_POINT('Ctrl Pts',(62.5414636331938,1074.7572172371,331.329347871775));
#121730=CARTESIAN_POINT('Ctrl Pts',(62.5432727372191,1074.77162897249,331.457648809979));
#121731=CARTESIAN_POINT('Ctrl Pts',(62.5314601012918,1074.77975838652,331.521593733552));
#121732=CARTESIAN_POINT('Ctrl Pts',(62.4833880269776,1074.79702613393,331.64246581233));
#121733=CARTESIAN_POINT('Ctrl Pts',(62.4470523632795,1074.80601828966,331.698057412042));
#121734=CARTESIAN_POINT('Ctrl Pts',(62.3548570296498,1074.82341668373,331.791383377283));
#121735=CARTESIAN_POINT('Ctrl Pts',(62.2999617822409,1074.83166156739,331.828321795356));
#121736=CARTESIAN_POINT('Ctrl Pts',(62.1799911633698,1074.84616489195,331.877939340832));
#121737=CARTESIAN_POINT('Ctrl Pts',(62.116296600872,1074.85232259687,331.890629107838));
#121738=CARTESIAN_POINT('Ctrl Pts',(62.051871595801,1074.85711166046,331.890629107838));
#121739=CARTESIAN_POINT('Origin',(3.98894410367401,1067.7251047501,335.150892220804));
#121740=CARTESIAN_POINT('',(3.98894410369655,1078.62952598896,333.672589088611));
#121741=CARTESIAN_POINT('Ctrl Pts',(3.98892918962189,1078.70545283844,336.629195352922));
#121742=CARTESIAN_POINT('Ctrl Pts',(4.03786747477723,1078.70541435023,336.629195846643));
#121743=CARTESIAN_POINT('Ctrl Pts',(4.08677555468786,1078.70533301832,336.626766232996));
#121744=CARTESIAN_POINT('Ctrl Pts',(4.22075614699632,1078.70499063064,336.613420428748));
#121745=CARTESIAN_POINT('Ctrl Pts',(4.30513902806456,1078.704641378,336.597524920551));
#121746=CARTESIAN_POINT('Ctrl Pts',(4.57794731394422,1078.70304196814,336.52111207434));
#121747=CARTESIAN_POINT('Ctrl Pts',(4.75561762870029,1078.70123172322,336.430202147003));
#121748=CARTESIAN_POINT('Ctrl Pts',(5.04060446999527,1078.69650897887,336.203133442749));
#121749=CARTESIAN_POINT('Ctrl Pts',(5.15252223361214,1078.69384077107,336.077866790619));
#121750=CARTESIAN_POINT('Ctrl Pts',(5.3366583079901,1078.68725393482,335.784397588403));
#121751=CARTESIAN_POINT('Ctrl Pts',(5.40360494039046,1078.68330483038,335.616069770505));
#121752=CARTESIAN_POINT('Ctrl Pts',(5.47638562696601,1078.67425120324,335.250950368245));
#121753=CARTESIAN_POINT('Ctrl Pts',(5.47675254686655,1078.66916769866,335.056472056768));
#121754=CARTESIAN_POINT('Ctrl Pts',(5.40256039196515,1078.65877688197,334.676754766409));
#121755=CARTESIAN_POINT('Ctrl Pts',(5.32808988340935,1078.65357279211,334.495293135256));
#121756=CARTESIAN_POINT('Ctrl Pts',(5.11867226978488,1078.64429345339,334.179752629101));
#121757=CARTESIAN_POINT('Ctrl Pts',(4.98881021210526,1078.64026181465,334.046503035112));
#121758=CARTESIAN_POINT('Ctrl Pts',(4.7067037902564,1078.63429626432,333.848649819207));
#121759=CARTESIAN_POINT('Ctrl Pts',(4.56154612480652,1078.63219749884,333.778614155116));
#121760=CARTESIAN_POINT('Ctrl Pts',(4.34326559247139,1078.63038211411,333.714093153353));
#121761=CARTESIAN_POINT('Ctrl Pts',(4.27730718287703,1078.62999143848,333.699416335752));
#121762=CARTESIAN_POINT('Ctrl Pts',(4.1661353663951,1078.62959503315,333.682558523943));
#121763=CARTESIAN_POINT('Ctrl Pts',(4.12140975412106,1078.6295044828,333.677849972551));
#121764=CARTESIAN_POINT('Ctrl Pts',(4.03402577116883,1078.62946143129,333.672663026376));
#121765=CARTESIAN_POINT('Ctrl Pts',(3.99142324262148,1078.62950194538,333.671977837842));
#121766=CARTESIAN_POINT('Ctrl Pts',(3.89258045832872,1078.62973820764,333.674659556288));
#121767=CARTESIAN_POINT('Ctrl Pts',(3.83644371024871,1078.62997954585,333.679398978925));
#121768=CARTESIAN_POINT('Ctrl Pts',(3.66586755016836,1078.63103848406,333.703667783558));
#121769=CARTESIAN_POINT('Ctrl Pts',(3.55334610772653,1078.63219297376,333.733468664245));
#121770=CARTESIAN_POINT('Ctrl Pts',(3.26184166844232,1078.63638726145,333.848704653796));
#121771=CARTESIAN_POINT('Ctrl Pts',(3.09461816678822,1078.64014081387,333.957351726536));
#121772=CARTESIAN_POINT('Ctrl Pts',(2.83228962003559,1078.64848060665,334.214702922275));
#121773=CARTESIAN_POINT('Ctrl Pts',(2.73235499249032,1078.65281241297,334.353848566448));
#121774=CARTESIAN_POINT('Ctrl Pts',(2.57893055794889,1078.66214975565,334.670869898601));
#121775=CARTESIAN_POINT('Ctrl Pts',(2.5305635037259,1078.66709716785,334.848094398121));
#121776=CARTESIAN_POINT('Ctrl Pts',(2.49961085669172,1078.67693717591,335.224181933052));
#121777=CARTESIAN_POINT('Ctrl Pts',(2.52228959250107,1078.68170139175,335.419997076885));
#121778=CARTESIAN_POINT('Ctrl Pts',(2.64179380622852,1078.690076523,335.789546881013));
#121779=CARTESIAN_POINT('Ctrl Pts',(2.73668484288976,1078.69362319307,335.959934329484));
#121780=CARTESIAN_POINT('Ctrl Pts',(2.97658100153028,1078.69914702624,336.242704702269));
#121781=CARTESIAN_POINT('Ctrl Pts',(3.11498027446472,1078.70118871564,336.356348738234));
#121782=CARTESIAN_POINT('Ctrl Pts',(3.38118618246868,1078.70371203262,336.504456515524));
#121783=CARTESIAN_POINT('Ctrl Pts',(3.49965089958669,1078.70446244868,336.55164167264));
#121784=CARTESIAN_POINT('Ctrl Pts',(3.68054300568547,1078.70514283027,336.59790144199));
#121785=CARTESIAN_POINT('Ctrl Pts',(3.73924715800365,1078.70529591923,336.60917833755));
#121786=CARTESIAN_POINT('Ctrl Pts',(3.84050345373653,1078.70544857856,336.622334362943));
#121787=CARTESIAN_POINT('Ctrl Pts',(3.88275021557812,1078.70547971821,336.625985257367));
#121788=CARTESIAN_POINT('Ctrl Pts',(3.94636085655102,1078.70547819981,336.628735205219));
#121789=CARTESIAN_POINT('Ctrl Pts',(3.967643781809,1078.70546957865,336.629195138182));
#121790=CARTESIAN_POINT('Ctrl Pts',(3.98892918962189,1078.70545283844,336.629195352922));
#121791=CARTESIAN_POINT('',(3.98894410365689,1076.62830575618,333.672589088611));
#121792=CARTESIAN_POINT('',(3.98894410367401,1067.7251047501,333.672589088611));
#121793=CARTESIAN_POINT('Ctrl Pts',(3.98878836967398,1076.70513034802,336.629195344795));
#121794=CARTESIAN_POINT('Ctrl Pts',(3.7930202123859,1076.70528585575,336.629174721312));
#121795=CARTESIAN_POINT('Ctrl Pts',(3.59919331969724,1076.70475707765,336.590266460707));
#121796=CARTESIAN_POINT('Ctrl Pts',(3.23859265166785,1076.70228199228,336.439463716588));
#121797=CARTESIAN_POINT('Ctrl Pts',(3.075274785619,1076.70035886093,336.329300839745));
#121798=CARTESIAN_POINT('Ctrl Pts',(2.80088043015867,1076.69503122865,336.051964074437));
#121799=CARTESIAN_POINT('Ctrl Pts',(2.69249236033706,1076.6916707662,335.887526388395));
#121800=CARTESIAN_POINT('Ctrl Pts',(2.54517248907245,1076.68357204508,335.524528027989));
#121801=CARTESIAN_POINT('Ctrl Pts',(2.50832320045053,1076.67889691296,335.329310069862));
#121802=CARTESIAN_POINT('Ctrl Pts',(2.51315100918465,1076.66880288985,334.938648120785));
#121803=CARTESIAN_POINT('Ctrl Pts',(2.55370690269806,1076.66349351796,334.747030171959));
#121804=CARTESIAN_POINT('Ctrl Pts',(2.70656038072564,1076.65300750955,334.390255602793));
#121805=CARTESIAN_POINT('Ctrl Pts',(2.81743887061719,1076.64793808138,334.228580517299));
#121806=CARTESIAN_POINT('Ctrl Pts',(3.095369869255,1076.63903923649,333.95731938209));
#121807=CARTESIAN_POINT('Ctrl Pts',(3.25972780495756,1076.63530369453,333.850374268239));
#121808=CARTESIAN_POINT('Ctrl Pts',(3.62009120867445,1076.63000627701,333.706275428726));
#121809=CARTESIAN_POINT('Ctrl Pts',(3.8125361211168,1076.62849720654,333.6704000379));
#121810=CARTESIAN_POINT('Ctrl Pts',(4.19976287471065,1076.62806931342,333.674978342989));
#121811=CARTESIAN_POINT('Ctrl Pts',(4.39078290107999,1076.62914776945,333.715173933314));
#121812=CARTESIAN_POINT('Ctrl Pts',(4.74617483270904,1076.63365995214,333.866669597516));
#121813=CARTESIAN_POINT('Ctrl Pts',(4.90716816144421,1076.63704150804,333.976380078437));
#121814=CARTESIAN_POINT('Ctrl Pts',(5.1779123931955,1076.64538915298,334.251456192178));
#121815=CARTESIAN_POINT('Ctrl Pts',(5.28505196529667,1076.65026846074,334.414192486284));
#121816=CARTESIAN_POINT('Ctrl Pts',(5.43083042257437,1076.6605739556,334.771837263306));
#121817=CARTESIAN_POINT('Ctrl Pts',(5.4679805068262,1076.66589594301,334.963353327041));
#121818=CARTESIAN_POINT('Ctrl Pts',(5.46686421438338,1076.67354941954,335.253186362826));
#121819=CARTESIAN_POINT('Ctrl Pts',(5.45702436219599,1076.67602885489,335.349520432207));
#121820=CARTESIAN_POINT('Ctrl Pts',(5.39896579566468,1076.68321919339,335.636318864411));
#121821=CARTESIAN_POINT('Ctrl Pts',(5.32224942252514,1076.6875225925,335.818804368267));
#121822=CARTESIAN_POINT('Ctrl Pts',(5.10273419738406,1076.6948015051,336.142270875995));
#121823=CARTESIAN_POINT('Ctrl Pts',(4.96247867826358,1076.69772050267,336.280316098033));
#121824=CARTESIAN_POINT('Ctrl Pts',(4.63614714833236,1076.70216533599,336.494266421958));
#121825=CARTESIAN_POINT('Ctrl Pts',(4.45319269068329,1076.70365284641,336.567932575272));
#121826=CARTESIAN_POINT('Ctrl Pts',(4.1713828408152,1076.70483439467,336.620738883684));
#121827=CARTESIAN_POINT('Ctrl Pts',(4.08018360826906,1076.70505774854,336.629204972959));
#121828=CARTESIAN_POINT('Ctrl Pts',(3.98878836967398,1076.70513034802,336.629195344795));
#121829=CARTESIAN_POINT('Origin',(3.98894410367401,1067.7251047501,335.150892220804));
#121830=CARTESIAN_POINT('',(3.98894410367403,1076.69355479191,336.029195352998));
#121831=CARTESIAN_POINT('',(3.98894410317932,1076.64787682225,334.272589088611));
#121832=CARTESIAN_POINT('Ctrl Pts',(3.98894410367403,1076.69355479191,336.029195352998));
#121833=CARTESIAN_POINT('Ctrl Pts',(3.93091475126699,1076.69360970332,336.029195352998));
#121834=CARTESIAN_POINT('Ctrl Pts',(3.87288505415834,1076.69354277828,336.023444360572));
#121835=CARTESIAN_POINT('Ctrl Pts',(3.70138881123196,1076.69297135146,335.988942426484));
#121836=CARTESIAN_POINT('Ctrl Pts',(3.59278219407908,1076.69210617214,335.943401124292));
#121837=CARTESIAN_POINT('Ctrl Pts',(3.39982045431152,1076.68942545344,335.812645313259));
#121838=CARTESIAN_POINT('Ctrl Pts',(3.31735426483233,1076.68763485745,335.728774569024));
#121839=CARTESIAN_POINT('Ctrl Pts',(3.18975861923189,1076.68322620786,335.533471034364));
#121840=CARTESIAN_POINT('Ctrl Pts',(3.14601743550809,1076.68064682687,335.423904157034));
#121841=CARTESIAN_POINT('Ctrl Pts',(3.10403796131332,1076.67496401598,335.19451813196));
#121842=CARTESIAN_POINT('Ctrl Pts',(3.10605029308206,1076.67191761824,335.0770058293));
#121843=CARTESIAN_POINT('Ctrl Pts',(3.15551202014162,1076.66578701744,334.850756746851));
#121844=CARTESIAN_POINT('Ctrl Pts',(3.20202687940525,1076.66276395548,334.744132968252));
#121845=CARTESIAN_POINT('Ctrl Pts',(3.33359160165528,1076.65719862283,334.554893473413));
#121846=CARTESIAN_POINT('Ctrl Pts',(3.41738042736138,1076.65471290943,334.47412045959));
#121847=CARTESIAN_POINT('Ctrl Pts',(3.61131803505323,1076.65074150661,334.349589423035));
#121848=CARTESIAN_POINT('Ctrl Pts',(3.71956672676871,1076.64929614901,334.307016244285));
#121849=CARTESIAN_POINT('Ctrl Pts',(3.88455002691543,1076.64816214277,334.277240351956));
#121850=CARTESIAN_POINT('Ctrl Pts',(3.93675683209862,1076.64794813166,334.27258908867));
#121851=CARTESIAN_POINT('Ctrl Pts',(3.98894410268463,1076.64787682225,334.272589088611));
#121852=CARTESIAN_POINT('',(3.98894410367401,1082.7251047501,334.272589088611));
#121853=CARTESIAN_POINT('',(3.98894410367401,1067.7251047501,334.272589088611));
#121854=CARTESIAN_POINT('Origin',(3.98894410367401,1082.7251047501,335.150892220804));
#121855=CARTESIAN_POINT('Ctrl Pts',(3.98894410268463,1076.64787682225,334.272589088611));
#121856=CARTESIAN_POINT('Ctrl Pts',(4.05123528120277,1076.64779170673,334.272589088541));
#121857=CARTESIAN_POINT('Ctrl Pts',(4.11349862889648,1076.64791000709,334.27921590747));
#121858=CARTESIAN_POINT('Ctrl Pts',(4.28690692430041,1076.6488211043,334.316733106288));
#121859=CARTESIAN_POINT('Ctrl Pts',(4.39329327861196,1076.65008504048,334.362791891777));
#121860=CARTESIAN_POINT('Ctrl Pts',(4.5822611944483,1076.65373968478,334.493196024519));
#121861=CARTESIAN_POINT('Ctrl Pts',(4.66303086930762,1076.65609242238,334.576268200363));
#121862=CARTESIAN_POINT('Ctrl Pts',(4.78808835047346,1076.66146718022,334.768826134735));
#121863=CARTESIAN_POINT('Ctrl Pts',(4.83114447161027,1076.66443548735,334.876478862489));
#121864=CARTESIAN_POINT('Ctrl Pts',(4.86138277028479,1076.66877929985,335.038087607017));
#121865=CARTESIAN_POINT('Ctrl Pts',(4.86635837388089,1076.67009391629,335.087501981756));
#121866=CARTESIAN_POINT('Ctrl Pts',(4.86713848754261,1076.67139771689,335.137071361129));
#121867=CARTESIAN_POINT('Ctrl Pts',(4.86804189137142,1076.67290757181,335.194474749012));
#121868=CARTESIAN_POINT('Ctrl Pts',(4.86331485679127,1076.67439610009,335.251829481203));
#121869=CARTESIAN_POINT('Ctrl Pts',(4.83205951683594,1076.67878878755,335.423390817771));
#121870=CARTESIAN_POINT('Ctrl Pts',(4.78831343977695,1076.68151307608,335.533136456035));
#121871=CARTESIAN_POINT('Ctrl Pts',(4.66066562184075,1076.68626326664,335.728625856977));
#121872=CARTESIAN_POINT('Ctrl Pts',(4.57820143998906,1076.68824752279,335.81253020833));
#121873=CARTESIAN_POINT('Ctrl Pts',(4.38528525337268,1076.69134030004,335.943304162282));
#121874=CARTESIAN_POINT('Ctrl Pts',(4.27673716279811,1076.69242055267,335.988854081877));
#121875=CARTESIAN_POINT('Ctrl Pts',(4.10520212664494,1076.69332251958,336.023424552889));
#121876=CARTESIAN_POINT('Ctrl Pts',(4.04707328810597,1076.69349978603,336.029195352998));
#121877=CARTESIAN_POINT('Ctrl Pts',(3.98894410367403,1076.69355479191,336.029195352998));
#121878=CARTESIAN_POINT('Origin',(14.9669751953833,1067.7251047501,329.052293203314));
#121879=CARTESIAN_POINT('',(14.9669751953994,1078.26481065249,327.776849082177));
#121880=CARTESIAN_POINT('Ctrl Pts',(14.9670414268982,1078.42603035398,330.327737322731));
#121881=CARTESIAN_POINT('Ctrl Pts',(15.0508755418035,1078.42527386653,330.327732969376));
#121882=CARTESIAN_POINT('Ctrl Pts',(15.1344986130066,1078.42404243283,330.319463080818));
#121883=CARTESIAN_POINT('Ctrl Pts',(15.3828386223669,1078.41892060072,330.269880459933));
#121884=CARTESIAN_POINT('Ctrl Pts',(15.5406646352344,1078.41365256733,330.203947377001));
#121885=CARTESIAN_POINT('Ctrl Pts',(15.800795671808,1078.40085954674,330.028209766681));
#121886=CARTESIAN_POINT('Ctrl Pts',(15.9059480870898,1078.39386610398,329.927492297754));
#121887=CARTESIAN_POINT('Ctrl Pts',(16.0847682905068,1078.37752469092,329.686025913971));
#121888=CARTESIAN_POINT('Ctrl Pts',(16.1537883367907,1078.36816846601,329.544766148022));
#121889=CARTESIAN_POINT('Ctrl Pts',(16.2405793382962,1078.34781444111,329.233253811105));
#121890=CARTESIAN_POINT('Ctrl Pts',(16.2533118075247,1078.33694000721,329.064612431137));
#121891=CARTESIAN_POINT('Ctrl Pts',(16.2128969673545,1078.31582579914,328.732243032528));
#121892=CARTESIAN_POINT('Ctrl Pts',(16.1602070366504,1078.30578990794,328.5716870269));
#121893=CARTESIAN_POINT('Ctrl Pts',(16.0013166061144,1078.28866933711,328.28988839172));
#121894=CARTESIAN_POINT('Ctrl Pts',(15.9003079684194,1078.28157845807,328.169088801628));
#121895=CARTESIAN_POINT('Ctrl Pts',(15.6764154780689,1078.27138138027,327.983881540676));
#121896=CARTESIAN_POINT('Ctrl Pts',(15.559980959649,1078.26792199564,327.915116530907));
#121897=CARTESIAN_POINT('Ctrl Pts',(15.385990907775,1078.26508680129,327.846494022059));
#121898=CARTESIAN_POINT('Ctrl Pts',(15.3358973241739,1078.26450956568,327.830236409693));
#121899=CARTESIAN_POINT('Ctrl Pts',(15.2520136569127,1078.26392919189,327.808642599197));
#121900=CARTESIAN_POINT('Ctrl Pts',(15.2187604003336,1078.2637954118,327.801486259334));
#121901=CARTESIAN_POINT('Ctrl Pts',(15.1541280676858,1078.26371955065,327.790259133371));
#121902=CARTESIAN_POINT('Ctrl Pts',(15.1228053640728,1078.26376461733,327.786010006042));
#121903=CARTESIAN_POINT('Ctrl Pts',(15.0504839633303,1078.26405564935,327.77892339476));
#121904=CARTESIAN_POINT('Ctrl Pts',(15.0094419579447,1078.26435761509,327.776894914863));
#121905=CARTESIAN_POINT('Ctrl Pts',(14.8849931185867,1078.26568508702,327.776758351789));
#121906=CARTESIAN_POINT('Ctrl Pts',(14.8018126880519,1078.26713253849,327.784843607977));
#121907=CARTESIAN_POINT('Ctrl Pts',(14.5537424610274,1078.27313282264,327.83380074425));
#121908=CARTESIAN_POINT('Ctrl Pts',(14.3957239243208,1078.27929053976,327.899421225175));
#121909=CARTESIAN_POINT('Ctrl Pts',(14.1357208939644,1078.29378738404,328.07428420265));
#121910=CARTESIAN_POINT('Ctrl Pts',(14.0307570734049,1078.30155384578,328.174253138317));
#121911=CARTESIAN_POINT('Ctrl Pts',(13.8520496664264,1078.31915947966,328.413770259329));
#121912=CARTESIAN_POINT('Ctrl Pts',(13.7828031126072,1078.32896464567,328.553803466007));
#121913=CARTESIAN_POINT('Ctrl Pts',(13.6948406554323,1078.34958137226,328.862514498121));
#121914=CARTESIAN_POINT('Ctrl Pts',(13.6809575238583,1078.36021843774,329.02962463015));
#121915=CARTESIAN_POINT('Ctrl Pts',(13.7182230595974,1078.38034586136,329.361274643958));
#121916=CARTESIAN_POINT('Ctrl Pts',(13.7695958184114,1078.38963305736,329.522580854854));
#121917=CARTESIAN_POINT('Ctrl Pts',(13.9268499640947,1078.4051665969,329.807041172956));
#121918=CARTESIAN_POINT('Ctrl Pts',(14.0278029367714,1078.41143660226,329.929500549406));
#121919=CARTESIAN_POINT('Ctrl Pts',(14.2531259830977,1078.42038043295,330.118020163101));
#121920=CARTESIAN_POINT('Ctrl Pts',(14.3710980251748,1078.42336651719,330.188206407939));
#121921=CARTESIAN_POINT('Ctrl Pts',(14.5470803108169,1078.42579036702,330.257795593266));
#121922=CARTESIAN_POINT('Ctrl Pts',(14.5973608879206,1078.4262785311,330.274149724578));
#121923=CARTESIAN_POINT('Ctrl Pts',(14.6812541583739,1078.42676739415,330.295782058203));
#121924=CARTESIAN_POINT('Ctrl Pts',(14.7143194977419,1078.42688008699,330.302919517373));
#121925=CARTESIAN_POINT('Ctrl Pts',(14.7783391756695,1078.42694625575,330.314095875837));
#121926=CARTESIAN_POINT('Ctrl Pts',(14.8092350207692,1078.42691145009,330.318329364288));
#121927=CARTESIAN_POINT('Ctrl Pts',(14.8801998610739,1078.426679681,330.325415061572));
#121928=CARTESIAN_POINT('Ctrl Pts',(14.9203103683575,1078.42643908147,330.327515346321));
#121929=CARTESIAN_POINT('Ctrl Pts',(14.9626486368974,1078.42606966526,330.327731877347));
#121930=CARTESIAN_POINT('Ctrl Pts',(14.9648450320519,1078.42605017341,330.327737436785));
#121931=CARTESIAN_POINT('Ctrl Pts',(14.9670414268982,1078.42603035398,330.327737322731));
#121932=CARTESIAN_POINT('',(14.9669751953554,1076.25966013686,327.776849082178));
#121933=CARTESIAN_POINT('',(14.9669751953833,1067.7251047501,327.776849082178));
#121934=CARTESIAN_POINT('Ctrl Pts',(14.9669818897757,1076.42256163736,330.327737324433));
#121935=CARTESIAN_POINT('Ctrl Pts',(14.7973915322079,1076.42410781104,330.327738214557));
#121936=CARTESIAN_POINT('Ctrl Pts',(14.6294952652309,1076.42367255477,330.293914196354));
#121937=CARTESIAN_POINT('Ctrl Pts',(14.3171888818399,1076.41887675521,330.162764125605));
#121938=CARTESIAN_POINT('Ctrl Pts',(14.1758534955704,1076.4145717933,330.06691872567));
#121939=CARTESIAN_POINT('Ctrl Pts',(13.9391054826949,1076.40248529862,329.826047172991));
#121940=CARTESIAN_POINT('Ctrl Pts',(13.8459413763126,1076.39482645647,329.683524440797));
#121941=CARTESIAN_POINT('Ctrl Pts',(13.7201763700816,1076.37689844833,329.369956021304));
#121942=CARTESIAN_POINT('Ctrl Pts',(13.6890849546996,1076.36679130366,329.201895792141));
#121943=CARTESIAN_POINT('Ctrl Pts',(13.6929566703232,1076.35082650684,328.949614980448));
#121944=CARTESIAN_POINT('Ctrl Pts',(13.7023526050109,1076.34546178853,328.866836214588));
#121945=CARTESIAN_POINT('Ctrl Pts',(13.7551310672895,1076.32908051219,328.620038786145));
#121946=CARTESIAN_POINT('Ctrl Pts',(13.8231346388622,1076.31812610706,328.463180210707));
#121947=CARTESIAN_POINT('Ctrl Pts',(14.0154443533977,1076.29778257473,328.186602895354));
#121948=CARTESIAN_POINT('Ctrl Pts',(14.1373073185298,1076.28857790361,328.069173828211));
#121949=CARTESIAN_POINT('Ctrl Pts',(14.4192675079826,1076.27327608476,327.88835237167));
#121950=CARTESIAN_POINT('Ctrl Pts',(14.5765366991904,1076.26732491336,327.826592684308));
#121951=CARTESIAN_POINT('Ctrl Pts',(14.9055193028814,1076.25968212144,327.767451429315));
#121952=CARTESIAN_POINT('Ctrl Pts',(15.0739592792332,1076.25805376913,327.770433937849));
#121953=CARTESIAN_POINT('Ctrl Pts',(15.3997830801189,1076.25941081277,327.841030809865));
#121954=CARTESIAN_POINT('Ctrl Pts',(15.5539987330769,1076.26237164526,327.907802579917));
#121955=CARTESIAN_POINT('Ctrl Pts',(15.8280758297298,1076.27242547397,328.09679163355));
#121956=CARTESIAN_POINT('Ctrl Pts',(15.9452593815558,1076.27941898224,328.217192535579));
#121957=CARTESIAN_POINT('Ctrl Pts',(16.126974089001,1076.29636844751,328.496431438403));
#121958=CARTESIAN_POINT('Ctrl Pts',(16.1896186643221,1076.30616474413,328.652684640968));
#121959=CARTESIAN_POINT('Ctrl Pts',(16.2358663161956,1076.32185850349,328.898537767218));
#121960=CARTESIAN_POINT('Ctrl Pts',(16.2432063861972,1076.32722385042,328.981883410289));
#121961=CARTESIAN_POINT('Ctrl Pts',(16.2414983319426,1076.33804693771,329.14884085682));
#121962=CARTESIAN_POINT('Ctrl Pts',(16.2324459257184,1076.34347900151,329.232056830215));
#121963=CARTESIAN_POINT('Ctrl Pts',(16.1805702870738,1076.35975331527,329.479704078509));
#121964=CARTESIAN_POINT('Ctrl Pts',(16.1130768669453,1076.37024051315,329.637076535622));
#121965=CARTESIAN_POINT('Ctrl Pts',(15.9210142141033,1076.38919409139,329.915419032512));
#121966=CARTESIAN_POINT('Ctrl Pts',(15.7986708492355,1076.39749028877,330.033873879393));
#121967=CARTESIAN_POINT('Ctrl Pts',(15.5147036387591,1076.41103039056,330.216457158506));
#121968=CARTESIAN_POINT('Ctrl Pts',(15.3558558765118,1076.4161414139,330.278706558088));
#121969=CARTESIAN_POINT('Ctrl Pts',(15.1160129447032,1076.42082132936,330.321193333598));
#121970=CARTESIAN_POINT('Ctrl Pts',(15.0415718435788,1076.42188159266,330.327736932934));
#121971=CARTESIAN_POINT('Ctrl Pts',(14.9669818897757,1076.42256163736,330.327737324433));
#121972=CARTESIAN_POINT('Origin',(14.9669751953833,1067.7251047501,329.052293203314));
#121973=CARTESIAN_POINT('',(14.9669751953833,1076.38718569293,329.72773732445));
#121974=CARTESIAN_POINT('',(14.9669751953839,1076.30090002967,328.376849082178));
#121975=CARTESIAN_POINT('Ctrl Pts',(14.9669751953833,1076.38718569293,329.72773732445));
#121976=CARTESIAN_POINT('Ctrl Pts',(14.9194354684686,1076.38763918504,329.72773732445));
#121977=CARTESIAN_POINT('Ctrl Pts',(14.8719081858183,1076.3877866468,329.722718311536));
#121978=CARTESIAN_POINT('Ctrl Pts',(14.7371605195918,1076.38731020095,329.69378916954));
#121979=CARTESIAN_POINT('Ctrl Pts',(14.6538046338945,1076.38589623523,329.65747948583));
#121980=CARTESIAN_POINT('Ctrl Pts',(14.5063694136426,1076.38100410945,329.554432181541));
#121981=CARTESIAN_POINT('Ctrl Pts',(14.4437471384081,1076.37757731989,329.488781690384));
#121982=CARTESIAN_POINT('Ctrl Pts',(14.3478389426105,1076.36910032337,329.33684759343));
#121983=CARTESIAN_POINT('Ctrl Pts',(14.3155307410438,1076.3641322677,329.252068096327));
#121984=CARTESIAN_POINT('Ctrl Pts',(14.2935059757345,1076.35604253381,329.120104927158));
#121985=CARTESIAN_POINT('Ctrl Pts',(14.2905207933502,1076.35329154602,329.076123350273));
#121986=CARTESIAN_POINT('Ctrl Pts',(14.2931443375162,1076.34767485741,328.988105006611));
#121987=CARTESIAN_POINT('Ctrl Pts',(14.2987684474515,1076.34482214203,328.944276252203));
#121988=CARTESIAN_POINT('Ctrl Pts',(14.3286558647562,1076.33616895413,328.813953637626));
#121989=CARTESIAN_POINT('Ctrl Pts',(14.365881272224,1076.33045126678,328.731436764397));
#121990=CARTESIAN_POINT('Ctrl Pts',(14.4698049177082,1076.31994204415,328.586564729992));
#121991=CARTESIAN_POINT('Ctrl Pts',(14.5351649459538,1076.31524289661,328.525384325979));
#121992=CARTESIAN_POINT('Ctrl Pts',(14.6856790386531,1076.30750211623,328.431866759496));
#121993=CARTESIAN_POINT('Ctrl Pts',(14.7693259695929,1076.30453310428,328.400371241936));
#121994=CARTESIAN_POINT('Ctrl Pts',(14.8931461334107,1076.30187437154,328.379880400079));
#121995=CARTESIAN_POINT('Ctrl Pts',(14.9300237741418,1076.30128645698,328.376849082178));
#121996=CARTESIAN_POINT('Ctrl Pts',(14.966975195385,1076.30090002967,328.376849082178));
#121997=CARTESIAN_POINT('',(14.9669751953833,1082.7251047501,328.376849082178));
#121998=CARTESIAN_POINT('',(14.9669751953833,1067.7251047501,328.376849082178));
#121999=CARTESIAN_POINT('Origin',(14.9669751953833,1082.7251047501,329.052293203314));
#122000=CARTESIAN_POINT('Ctrl Pts',(14.9669835900019,1076.30089994188,328.37684908223));
#122001=CARTESIAN_POINT('Ctrl Pts',(15.0552529225584,1076.29997691983,328.376850179267));
#122002=CARTESIAN_POINT('Ctrl Pts',(15.1426683856137,1076.3002189197,328.394154081871));
#122003=CARTESIAN_POINT('Ctrl Pts',(15.3058514613236,1076.30299993899,328.461385760682));
#122004=CARTESIAN_POINT('Ctrl Pts',(15.3800287689552,1076.30551021201,328.510642195034));
#122005=CARTESIAN_POINT('Ctrl Pts',(15.5053418329324,1076.31244578406,328.634935009798));
#122006=CARTESIAN_POINT('Ctrl Pts',(15.5552218458248,1076.31680594787,328.708810684804));
#122007=CARTESIAN_POINT('Ctrl Pts',(15.6238180723971,1076.3267621582,328.871704004732));
#122008=CARTESIAN_POINT('Ctrl Pts',(15.6417942447796,1076.33226457382,328.959195813127));
#122009=CARTESIAN_POINT('Ctrl Pts',(15.6427078900658,1076.34079539611,329.091873747251));
#122010=CARTESIAN_POINT('Ctrl Pts',(15.638666851738,1076.34366543975,329.136028245512));
#122011=CARTESIAN_POINT('Ctrl Pts',(15.6133842956322,1076.35233006512,329.267904706217));
#122012=CARTESIAN_POINT('Ctrl Pts',(15.5789119379269,1076.35798780034,329.352081595718));
#122013=CARTESIAN_POINT('Ctrl Pts',(15.4791310258456,1076.36833895204,329.501714414155));
#122014=CARTESIAN_POINT('Ctrl Pts',(15.4149168999795,1076.37293438836,329.565755076838));
#122015=CARTESIAN_POINT('Ctrl Pts',(15.2651186974525,1076.38050188352,329.665000015237));
#122016=CARTESIAN_POINT('Ctrl Pts',(15.1810292835317,1076.38339912944,329.699201532241));
#122017=CARTESIAN_POINT('Ctrl Pts',(15.0511420367375,1076.38614310924,329.723805255119));
#122018=CARTESIAN_POINT('Ctrl Pts',(15.0090537415224,1076.38678429624,329.72773732445));
#122019=CARTESIAN_POINT('Ctrl Pts',(14.9669751953833,1076.38718569293,329.72773732445));
#122020=CARTESIAN_POINT('Origin',(27.6354521170193,1067.7251047501,323.455155605234));
#122021=CARTESIAN_POINT('',(27.635452117036,1077.55448697719,322.356324469241));
#122022=CARTESIAN_POINT('Ctrl Pts',(27.6354554833944,1077.77317479141,324.553986741222));
#122023=CARTESIAN_POINT('Ctrl Pts',(27.78209499346,1077.76933775153,324.553986291977));
#122024=CARTESIAN_POINT('Ctrl Pts',(27.9271434753266,1077.76272537266,324.524634563112));
#122025=CARTESIAN_POINT('Ctrl Pts',(28.1739870805,1077.74618397533,324.420638081256));
#122026=CARTESIAN_POINT('Ctrl Pts',(28.2772138623149,1077.73712735143,324.355305784982));
#122027=CARTESIAN_POINT('Ctrl Pts',(28.465932012245,1077.71567121148,324.186672230339));
#122028=CARTESIAN_POINT('Ctrl Pts',(28.5475671410015,1077.70321917219,324.081903618919));
#122029=CARTESIAN_POINT('Ctrl Pts',(28.6745324689479,1077.67588242266,323.839673648655));
#122030=CARTESIAN_POINT('Ctrl Pts',(28.7154272804537,1077.6611311179,323.702514468041));
#122031=CARTESIAN_POINT('Ctrl Pts',(28.7431770865928,1077.6317537095,323.416840957285));
#122032=CARTESIAN_POINT('Ctrl Pts',(28.7284304245995,1077.61741873458,323.270839115508));
#122033=CARTESIAN_POINT('Ctrl Pts',(28.6449444884221,1077.59219529833,322.999639008381));
#122034=CARTESIAN_POINT('Ctrl Pts',(28.579593209094,1077.58139708564,322.876155530717));
#122035=CARTESIAN_POINT('Ctrl Pts',(28.4015541037616,1077.5636020172,322.653994853476));
#122036=CARTESIAN_POINT('Ctrl Pts',(28.2883036486213,1077.55702439445,322.559263112266));
#122037=CARTESIAN_POINT('Ctrl Pts',(28.1185711617126,1077.55230238832,322.46711842826));
#122038=CARTESIAN_POINT('Ctrl Pts',(28.0760381468249,1077.55146969942,322.447432193482));
#122039=CARTESIAN_POINT('Ctrl Pts',(28.0069992603195,1077.55065580183,322.420688068669));
#122040=CARTESIAN_POINT('Ctrl Pts',(27.9812674154294,1077.55046431554,322.41180416452));
#122041=CARTESIAN_POINT('Ctrl Pts',(27.9327826170647,1077.55030907866,322.397055880877));
#122042=CARTESIAN_POINT('Ctrl Pts',(27.9101206603123,1077.55031762918,322.390948086064));
#122043=CARTESIAN_POINT('Ctrl Pts',(27.8597731958885,1077.55051373314,322.37909402679));
#122044=CARTESIAN_POINT('Ctrl Pts',(27.8320270728602,1077.55073743386,322.373681308994));
#122045=CARTESIAN_POINT('Ctrl Pts',(27.7533536848727,1077.55169445846,322.361461484103));
#122046=CARTESIAN_POINT('Ctrl Pts',(27.7021202585493,1077.5526937123,322.357147642689));
#122047=CARTESIAN_POINT('Ctrl Pts',(27.504547116373,1077.55797550645,322.354391246003));
#122048=CARTESIAN_POINT('Ctrl Pts',(27.3594979330312,1077.56486021906,322.381564525387));
#122049=CARTESIAN_POINT('Ctrl Pts',(27.1123086761813,1077.58201058351,322.481355677257));
#122050=CARTESIAN_POINT('Ctrl Pts',(27.0087976084889,1077.59135801052,322.544540131769));
#122051=CARTESIAN_POINT('Ctrl Pts',(26.8186156075235,1077.61331288489,322.708616137735));
#122052=CARTESIAN_POINT('Ctrl Pts',(26.7356818667534,1077.62595896572,322.811017313524));
#122053=CARTESIAN_POINT('Ctrl Pts',(26.604985371743,1077.65340077059,323.048579265206));
#122054=CARTESIAN_POINT('Ctrl Pts',(26.5614979401041,1077.66804161175,323.183517000024));
#122055=CARTESIAN_POINT('Ctrl Pts',(26.5271042354151,1077.69706815676,323.467368269408));
#122056=CARTESIAN_POINT('Ctrl Pts',(26.5384377477433,1077.71115022112,323.613901157408));
#122057=CARTESIAN_POINT('Ctrl Pts',(26.6160006262472,1077.73585151202,323.888296295945));
#122058=CARTESIAN_POINT('Ctrl Pts',(26.6792043795877,1077.74637213626,324.014221197783));
#122059=CARTESIAN_POINT('Ctrl Pts',(26.8506198362845,1077.76335470198,324.237120432146));
#122060=CARTESIAN_POINT('Ctrl Pts',(26.9577336417413,1077.76960833789,324.331617522846));
#122061=CARTESIAN_POINT('Ctrl Pts',(27.1261596779175,1077.77465431793,324.430308089278));
#122062=CARTESIAN_POINT('Ctrl Pts',(27.1743178349814,1077.77566096828,324.453983851187));
#122063=CARTESIAN_POINT('Ctrl Pts',(27.2505559288919,1077.77661378816,324.484769082922));
#122064=CARTESIAN_POINT('Ctrl Pts',(27.2775036728934,1077.77683515168,324.494444786114));
#122065=CARTESIAN_POINT('Ctrl Pts',(27.3270076596723,1077.77703575534,324.510065177338));
#122066=CARTESIAN_POINT('Ctrl Pts',(27.3494333768748,1077.77705237694,324.516365045468));
#122067=CARTESIAN_POINT('Ctrl Pts',(27.3977436051221,1077.77693106367,324.528293693508));
#122068=CARTESIAN_POINT('Ctrl Pts',(27.423665293593,1077.77677172099,324.533708792302));
#122069=CARTESIAN_POINT('Ctrl Pts',(27.4933860815695,1077.77609332228,324.545663100758));
#122070=CARTESIAN_POINT('Ctrl Pts',(27.5374238124978,1077.77540513588,324.550499888846));
#122071=CARTESIAN_POINT('Ctrl Pts',(27.5995585848569,1077.77407183489,324.553547051538));
#122072=CARTESIAN_POINT('Ctrl Pts',(27.6175061940963,1077.77364446114,324.553986796211));
#122073=CARTESIAN_POINT('Ctrl Pts',(27.6354554833944,1077.77317479141,324.553986741221));
#122074=CARTESIAN_POINT('',(27.635452116996,1075.54255412639,322.356324469242));
#122075=CARTESIAN_POINT('',(27.6354521170193,1067.7251047501,322.356324469242));
#122076=CARTESIAN_POINT('Ctrl Pts',(27.6354637578243,1075.7632441652,324.553986741165));
#122077=CARTESIAN_POINT('Ctrl Pts',(27.4893848818429,1075.76710221568,324.553988288697));
#122078=CARTESIAN_POINT('Ctrl Pts',(27.3447413669374,1075.76810235755,324.524859733852));
#122079=CARTESIAN_POINT('Ctrl Pts',(27.0753847867248,1075.76428525466,324.411752571686));
#122080=CARTESIAN_POINT('Ctrl Pts',(26.9534410681139,1075.75951030705,324.328977880892));
#122081=CARTESIAN_POINT('Ctrl Pts',(26.7491438613275,1075.74472243282,324.120844299191));
#122082=CARTESIAN_POINT('Ctrl Pts',(26.6688433354455,1075.7348596376,323.997622254667));
#122083=CARTESIAN_POINT('Ctrl Pts',(26.5607566653673,1075.71118587656,323.726812293878));
#122084=CARTESIAN_POINT('Ctrl Pts',(26.5342459186675,1075.69759180768,323.581819681718));
#122085=CARTESIAN_POINT('Ctrl Pts',(26.5380357036236,1075.67585756518,323.364425471326));
#122086=CARTESIAN_POINT('Ctrl Pts',(26.546275071122,1075.66851545085,323.293154931303));
#122087=CARTESIAN_POINT('Ctrl Pts',(26.576551672069,1075.6536322625,323.152955190422));
#122088=CARTESIAN_POINT('Ctrl Pts',(26.5985785079818,1075.64612482737,323.084361186689));
#122089=CARTESIAN_POINT('Ctrl Pts',(26.6852172837086,1075.62353484456,322.884339423397));
#122090=CARTESIAN_POINT('Ctrl Pts',(26.7694851961867,1075.60885159091,322.763109239036));
#122091=CARTESIAN_POINT('Ctrl Pts',(26.979357587787,1075.58238452567,322.561941176326));
#122092=CARTESIAN_POINT('Ctrl Pts',(27.1024258318607,1075.57082202732,322.483425754171));
#122093=CARTESIAN_POINT('Ctrl Pts',(27.3713583443627,1075.55240563357,322.378881570527));
#122094=CARTESIAN_POINT('Ctrl Pts',(27.5144402415721,1075.54570557635,322.353550160154));
#122095=CARTESIAN_POINT('Ctrl Pts',(27.8016371369334,1075.53816692316,322.359562940599));
#122096=CARTESIAN_POINT('Ctrl Pts',(27.9428784569236,1075.53737148428,322.390524849676));
#122097=CARTESIAN_POINT('Ctrl Pts',(28.2053399882139,1075.54180882458,322.504832444295));
#122098=CARTESIAN_POINT('Ctrl Pts',(28.3239729793978,1075.54698711339,322.586955359263));
#122099=CARTESIAN_POINT('Ctrl Pts',(28.5234273573164,1075.56261813331,322.792219089591));
#122100=CARTESIAN_POINT('Ctrl Pts',(28.6021500792818,1075.57293440965,322.913494049916));
#122101=CARTESIAN_POINT('Ctrl Pts',(28.7089690590344,1075.59730911865,323.179967444967));
#122102=CARTESIAN_POINT('Ctrl Pts',(28.7357146877056,1075.61115506102,323.322762436554));
#122103=CARTESIAN_POINT('Ctrl Pts',(28.7334763005315,1075.63311520331,323.538696203443));
#122104=CARTESIAN_POINT('Ctrl Pts',(28.7256236824297,1075.64059723465,323.610588873429));
#122105=CARTESIAN_POINT('Ctrl Pts',(28.6959788472949,1075.65561155148,323.751625342745));
#122106=CARTESIAN_POINT('Ctrl Pts',(28.6742851296499,1075.6631089484,323.820448464849));
#122107=CARTESIAN_POINT('Ctrl Pts',(28.5886406650049,1075.68548973464,324.021024212218));
#122108=CARTESIAN_POINT('Ctrl Pts',(28.5050027746342,1075.6998135266,324.142697999747));
#122109=CARTESIAN_POINT('Ctrl Pts',(28.2953907973526,1075.72544481533,324.345707774317));
#122110=CARTESIAN_POINT('Ctrl Pts',(28.1716927693333,1075.7365204612,324.425274518019));
#122111=CARTESIAN_POINT('Ctrl Pts',(27.9084124987656,1075.75354880344,324.528316300412));
#122112=CARTESIAN_POINT('Ctrl Pts',(27.7725918425639,1075.75962251169,324.553985288457));
#122113=CARTESIAN_POINT('Ctrl Pts',(27.6354637578243,1075.7632441652,324.553986741165));
#122114=CARTESIAN_POINT('Origin',(27.6354521170193,1067.7251047501,323.455155605234));
#122115=CARTESIAN_POINT('',(27.6354521170193,1075.70507826342,323.953986741227));
#122116=CARTESIAN_POINT('',(27.6354521170193,1075.60488526556,322.956324469242));
#122117=CARTESIAN_POINT('Ctrl Pts',(27.6354521170193,1075.70507826342,323.953986741227));
#122118=CARTESIAN_POINT('Ctrl Pts',(27.634044503031,1075.70511623235,323.953986741227));
#122119=CARTESIAN_POINT('Ctrl Pts',(27.6326365788117,1075.70515362057,323.953980783171));
#122120=CARTESIAN_POINT('Ctrl Pts',(27.5662202751841,1075.70688953137,323.953418398493));
#122121=CARTESIAN_POINT('Ctrl Pts',(27.501934139173,1075.70731419297,323.940164730451));
#122122=CARTESIAN_POINT('Ctrl Pts',(27.382030109535,1075.70556779413,323.889715649661));
#122123=CARTESIAN_POINT('Ctrl Pts',(27.3276115070596,1075.70341274803,323.853011731308));
#122124=CARTESIAN_POINT('Ctrl Pts',(27.234877522119,1075.69669649567,323.759780973222));
#122125=CARTESIAN_POINT('Ctrl Pts',(27.197921958113,1075.6921483109,323.703765212779));
#122126=CARTESIAN_POINT('Ctrl Pts',(27.1480534878934,1075.68125181367,323.580493573235));
#122127=CARTESIAN_POINT('Ctrl Pts',(27.135713339052,1075.67500623829,323.514435177438));
#122128=CARTESIAN_POINT('Ctrl Pts',(27.1371431232632,1075.66506192422,323.415382620928));
#122129=CARTESIAN_POINT('Ctrl Pts',(27.1408029297177,1075.66171215883,323.382939317489));
#122130=CARTESIAN_POINT('Ctrl Pts',(27.1544047637778,1075.65494142215,323.319174211982));
#122131=CARTESIAN_POINT('Ctrl Pts',(27.1643286318015,1075.65153595021,323.288002183825));
#122132=CARTESIAN_POINT('Ctrl Pts',(27.2036824476216,1075.64124433757,323.196526028818));
#122133=CARTESIAN_POINT('Ctrl Pts',(27.2422663137376,1075.63456288874,323.140942034853));
#122134=CARTESIAN_POINT('Ctrl Pts',(27.3380542535881,1075.62263149001,323.049350748552));
#122135=CARTESIAN_POINT('Ctrl Pts',(27.3939003959041,1075.61746697062,323.013802116999));
#122136=CARTESIAN_POINT('Ctrl Pts',(27.5125646838575,1075.6094812346,322.967784142417));
#122137=CARTESIAN_POINT('Ctrl Pts',(27.5737163233485,1075.60660692522,322.956324469242));
#122138=CARTESIAN_POINT('Ctrl Pts',(27.6354521170193,1075.60488526556,322.956324469242));
#122139=CARTESIAN_POINT('',(27.6354521170193,1082.7251047501,322.956324469242));
#122140=CARTESIAN_POINT('',(27.6354521170193,1067.7251047501,322.956324469242));
#122141=CARTESIAN_POINT('Origin',(27.6354521170193,1082.7251047501,323.455155605234));
#122142=CARTESIAN_POINT('Ctrl Pts',(27.6354526343093,1075.60488525113,322.956324469242));
#122143=CARTESIAN_POINT('Ctrl Pts',(27.7004736444753,1075.60307198173,322.956324536669));
#122144=CARTESIAN_POINT('Ctrl Pts',(27.7648809908801,1075.60257292419,322.969037435341));
#122145=CARTESIAN_POINT('Ctrl Pts',(27.8851394872723,1075.60426457263,323.018451535124));
#122146=CARTESIAN_POINT('Ctrl Pts',(27.9397996373544,1075.60643549965,323.054635109211));
#122147=CARTESIAN_POINT('Ctrl Pts',(28.0323199462946,1075.6131730729,323.146009206826));
#122148=CARTESIAN_POINT('Ctrl Pts',(28.0692064098541,1075.61768166637,323.200369259097));
#122149=CARTESIAN_POINT('Ctrl Pts',(28.1201754896558,1075.62845341682,323.320417951284));
#122150=CARTESIAN_POINT('Ctrl Pts',(28.1336271886545,1075.63462291697,323.385018683961));
#122151=CARTESIAN_POINT('Ctrl Pts',(28.1345768312166,1075.64448793891,323.483043289621));
#122152=CARTESIAN_POINT('Ctrl Pts',(28.1316735317111,1075.64785881459,323.515709779067));
#122153=CARTESIAN_POINT('Ctrl Pts',(28.1195251090723,1075.65465299698,323.579946749933));
#122154=CARTESIAN_POINT('Ctrl Pts',(28.1103170093908,1075.65806050761,323.611370153617));
#122155=CARTESIAN_POINT('Ctrl Pts',(28.0732135116152,1075.66830142562,323.703406689827));
#122156=CARTESIAN_POINT('Ctrl Pts',(28.0362007253373,1075.67492087552,323.759581440303));
#122157=CARTESIAN_POINT('Ctrl Pts',(27.9424006803349,1075.68686729279,323.853933002792));
#122158=CARTESIAN_POINT('Ctrl Pts',(27.8866104873441,1075.69208213468,323.891249257643));
#122159=CARTESIAN_POINT('Ctrl Pts',(27.7649500282382,1075.70032657103,323.941251252787));
#122160=CARTESIAN_POINT('Ctrl Pts',(27.7005326457111,1075.70332278349,323.953986741227));
#122161=CARTESIAN_POINT('Ctrl Pts',(27.6354521170193,1075.70507826342,323.953986741227));
#122162=CARTESIAN_POINT('Origin',(41.3143294401475,1067.7251047501,320.535862846908));
#122163=CARTESIAN_POINT('',(41.3143294401746,1076.68214102844,319.44532209818));
#122164=CARTESIAN_POINT('Ctrl Pts',(41.3143428194402,1076.95432942362,321.626403595554));
#122165=CARTESIAN_POINT('Ctrl Pts',(41.4218166275092,1076.94912750026,321.626402277012));
#122166=CARTESIAN_POINT('Ctrl Pts',(41.5285827596115,1076.9420159031,321.610514544172));
#122167=CARTESIAN_POINT('Ctrl Pts',(41.7465386926837,1076.92332534773,321.544328843047));
#122168=CARTESIAN_POINT('Ctrl Pts',(41.8551072169579,1076.91143255922,321.49047694153));
#122169=CARTESIAN_POINT('Ctrl Pts',(42.0589629662026,1076.88334386355,321.34333706984));
#122170=CARTESIAN_POINT('Ctrl Pts',(42.1505005855932,1076.86707680082,321.248068199629));
#122171=CARTESIAN_POINT('Ctrl Pts',(42.3011116436337,1076.83147654984,321.021183105947));
#122172=CARTESIAN_POINT('Ctrl Pts',(42.355651873213,1076.81231902425,320.889292817876));
#122173=CARTESIAN_POINT('Ctrl Pts',(42.4119342200797,1076.77440537764,320.609182994267));
#122174=CARTESIAN_POINT('Ctrl Pts',(42.41202397689,1076.75601805803,320.463273429836));
#122175=CARTESIAN_POINT('Ctrl Pts',(42.3567504731207,1076.72393887002,320.187633286867));
#122176=CARTESIAN_POINT('Ctrl Pts',(42.3049909651277,1076.71031809491,320.059822407833));
#122177=CARTESIAN_POINT('Ctrl Pts',(42.154338259021,1076.68820754652,319.826247547805));
#122178=CARTESIAN_POINT('Ctrl Pts',(42.0555296045438,1076.6801007609,319.723525029405));
#122179=CARTESIAN_POINT('Ctrl Pts',(41.9050007143757,1076.67427562563,319.618159098336));
#122180=CARTESIAN_POINT('Ctrl Pts',(41.8689131970497,1076.67326327875,319.595910218023));
#122181=CARTESIAN_POINT('Ctrl Pts',(41.8079915436222,1076.67215899292,319.563084875167));
#122182=CARTESIAN_POINT('Ctrl Pts',(41.7839041937303,1076.67186608549,319.551231457372));
#122183=CARTESIAN_POINT('Ctrl Pts',(41.7403350435942,1076.67158708966,319.531753994512));
#122184=CARTESIAN_POINT('Ctrl Pts',(41.7210262273562,1076.67154742382,319.523779301169));
#122185=CARTESIAN_POINT('Ctrl Pts',(41.6801633928604,1076.67163704969,319.508260998845));
#122186=CARTESIAN_POINT('Ctrl Pts',(41.6585780577322,1076.67178232638,319.500830056112));
#122187=CARTESIAN_POINT('Ctrl Pts',(41.6020992464047,1076.67241313776,319.483349027432));
#122188=CARTESIAN_POINT('Ctrl Pts',(41.5669122236252,1076.67304852764,319.474355366001));
#122189=CARTESIAN_POINT('Ctrl Pts',(41.4234207721387,1076.67660184293,319.445217862265));
#122190=CARTESIAN_POINT('Ctrl Pts',(41.3128898742779,1076.68151244776,319.439794759528));
#122191=CARTESIAN_POINT('Ctrl Pts',(41.0916870010979,1076.69558248906,319.46238955167));
#122192=CARTESIAN_POINT('Ctrl Pts',(40.9824491401439,1076.70474597225,319.491016072199));
#122193=CARTESIAN_POINT('Ctrl Pts',(40.7657586636322,1076.72761581736,319.585197821066));
#122194=CARTESIAN_POINT('Ctrl Pts',(40.6613385128956,1076.74153617064,319.653698614563));
#122195=CARTESIAN_POINT('Ctrl Pts',(40.4725764169351,1076.77317112897,319.829642607107));
#122196=CARTESIAN_POINT('Ctrl Pts',(40.3921978359933,1076.79084654215,319.938436490654));
#122197=CARTESIAN_POINT('Ctrl Pts',(40.2704151628547,1076.8282082524,320.188890633183));
#122198=CARTESIAN_POINT('Ctrl Pts',(40.233653008625,1076.84759758869,320.330131809515));
#122199=CARTESIAN_POINT('Ctrl Pts',(40.2174761305333,1076.88394167024,320.617160634091));
#122200=CARTESIAN_POINT('Ctrl Pts',(40.23754079299,1076.90058842704,320.760227311747));
#122201=CARTESIAN_POINT('Ctrl Pts',(40.3273217429563,1076.92777313096,321.017237138234));
#122202=CARTESIAN_POINT('Ctrl Pts',(40.3911610969451,1076.93854377822,321.130641097368));
#122203=CARTESIAN_POINT('Ctrl Pts',(40.5462268939571,1076.95395216355,321.31838197958));
#122204=CARTESIAN_POINT('Ctrl Pts',(40.6323826063517,1076.95906139893,321.394530103112));
#122205=CARTESIAN_POINT('Ctrl Pts',(40.7612065228253,1076.96281648845,321.476502172275));
#122206=CARTESIAN_POINT('Ctrl Pts',(40.7945994162274,1076.96349816862,321.495356845758));
#122207=CARTESIAN_POINT('Ctrl Pts',(40.849669187214,1076.96416938875,321.522730056165));
#122208=CARTESIAN_POINT('Ctrl Pts',(40.8707427482178,1076.96432584328,321.532380259352));
#122209=CARTESIAN_POINT('Ctrl Pts',(40.9091990554738,1076.96443342747,321.548528681394));
#122210=CARTESIAN_POINT('Ctrl Pts',(40.9264699651473,1076.96441935669,321.555268433267));
#122211=CARTESIAN_POINT('Ctrl Pts',(40.9671501679068,1076.96424215797,321.569959809575));
#122212=CARTESIAN_POINT('Ctrl Pts',(40.9906739658815,1076.96403096218,321.577561951523));
#122213=CARTESIAN_POINT('Ctrl Pts',(41.0577482813037,1076.96312542355,321.596746803453));
#122214=CARTESIAN_POINT('Ctrl Pts',(41.1017807062377,1076.9621774666,321.606437629254));
#122215=CARTESIAN_POINT('Ctrl Pts',(41.201900545872,1076.95923915612,321.622052494203));
#122216=CARTESIAN_POINT('Ctrl Pts',(41.2580901248877,1076.95705215404,321.62640428569));
#122217=CARTESIAN_POINT('Ctrl Pts',(41.3143428194403,1076.95432942362,321.626403595554));
#122218=CARTESIAN_POINT('',(41.3143294401476,1074.66274184067,319.445322098179));
#122219=CARTESIAN_POINT('',(41.3143294401475,1067.7251047501,319.445322098179));
#122220=CARTESIAN_POINT('Ctrl Pts',(41.314812718535,1074.93716077403,321.626403488553));
#122221=CARTESIAN_POINT('Ctrl Pts',(41.1715706204318,1074.94415975441,321.626466966985));
#122222=CARTESIAN_POINT('Ctrl Pts',(41.0296257881001,1074.94761527766,321.598307263943));
#122223=CARTESIAN_POINT('Ctrl Pts',(40.7661667853346,1074.94706138158,321.489219256244));
#122224=CARTESIAN_POINT('Ctrl Pts',(40.6471136149637,1074.94314345929,321.410015151242));
#122225=CARTESIAN_POINT('Ctrl Pts',(40.4436327271655,1074.9282686863,321.208304548177));
#122226=CARTESIAN_POINT('Ctrl Pts',(40.3622271759297,1074.91729988569,321.086920184947));
#122227=CARTESIAN_POINT('Ctrl Pts',(40.2514001287905,1074.88966635459,320.819529671462));
#122228=CARTESIAN_POINT('Ctrl Pts',(40.22323779074,1074.87325991693,320.676134756145));
#122229=CARTESIAN_POINT('Ctrl Pts',(40.2240712253127,1074.84635165742,320.460731515587));
#122230=CARTESIAN_POINT('Ctrl Pts',(40.2312612710062,1074.83715955598,320.390050263008));
#122231=CARTESIAN_POINT('Ctrl Pts',(40.2592825923277,1074.81832765418,320.250884592581));
#122232=CARTESIAN_POINT('Ctrl Pts',(40.2801031120063,1074.8087284771,320.182721629814));
#122233=CARTESIAN_POINT('Ctrl Pts',(40.3636445847771,1074.77926437491,319.981852006162));
#122234=CARTESIAN_POINT('Ctrl Pts',(40.4465935118131,1074.7595824578,319.85923951023));
#122235=CARTESIAN_POINT('Ctrl Pts',(40.6540803439798,1074.72330166367,319.656084325281));
#122236=CARTESIAN_POINT('Ctrl Pts',(40.7758210107337,1074.70699060038,319.576655842871));
#122237=CARTESIAN_POINT('Ctrl Pts',(41.0423110224472,1074.67981823942,319.47018350843));
#122238=CARTESIAN_POINT('Ctrl Pts',(41.1842336149242,1074.669172538,319.443677603048));
#122239=CARTESIAN_POINT('Ctrl Pts',(41.4692836080394,1074.65506020246,319.447107815698));
#122240=CARTESIAN_POINT('Ctrl Pts',(41.6095117397283,1074.65166939933,319.476470135398));
#122241=CARTESIAN_POINT('Ctrl Pts',(41.8704724359342,1074.65258759188,319.587181347956));
#122242=CARTESIAN_POINT('Ctrl Pts',(41.9886136753546,1074.65685765158,319.66720053904));
#122243=CARTESIAN_POINT('Ctrl Pts',(42.1881325358432,1074.67250856062,319.868119441079));
#122244=CARTESIAN_POINT('Ctrl Pts',(42.2673412716932,1074.68376186316,319.987179146882));
#122245=CARTESIAN_POINT('Ctrl Pts',(42.3763256559622,1074.7118212103,320.249764494128));
#122246=CARTESIAN_POINT('Ctrl Pts',(42.4045472972949,1074.72840748582,320.390979483382));
#122247=CARTESIAN_POINT('Ctrl Pts',(42.4051904739248,1074.7647076447,320.677135393134));
#122248=CARTESIAN_POINT('Ctrl Pts',(42.3770995356429,1074.78410874865,320.819433855955));
#122249=CARTESIAN_POINT('Ctrl Pts',(42.2668478998924,1074.82320033299,321.086396971585));
#122250=CARTESIAN_POINT('Ctrl Pts',(42.1850879715168,1074.84252574672,321.208338340571));
#122251=CARTESIAN_POINT('Ctrl Pts',(41.9790840161114,1074.87814078714,321.41236025411));
#122252=CARTESIAN_POINT('Ctrl Pts',(41.8571019468562,1074.89411356443,321.492772676195));
#122253=CARTESIAN_POINT('Ctrl Pts',(41.5932926861952,1074.92022809525,321.599323040952));
#122254=CARTESIAN_POINT('Ctrl Pts',(41.4548180418782,1074.93031994633,321.626341444513));
#122255=CARTESIAN_POINT('Ctrl Pts',(41.314812718535,1074.93716077403,321.626403488553));
#122256=CARTESIAN_POINT('Origin',(41.3143294401475,1067.7251047501,320.535862846908));
#122257=CARTESIAN_POINT('',(41.3143294401474,1074.86349252611,321.026403595636));
#122258=CARTESIAN_POINT('',(41.3143294401486,1074.74003968768,320.045322098179));
#122259=CARTESIAN_POINT('Ctrl Pts',(41.3143294401475,1074.86349252611,321.026403595636));
#122260=CARTESIAN_POINT('Ctrl Pts',(41.3128461441749,1074.86356585894,321.026403595636));
#122261=CARTESIAN_POINT('Ctrl Pts',(41.311362475265,1074.86363837087,321.026396867861));
#122262=CARTESIAN_POINT('Ctrl Pts',(41.2461231309153,1074.86678989609,321.025804888836));
#122263=CARTESIAN_POINT('Ctrl Pts',(41.1830517971698,1074.86828664131,321.012801589578));
#122264=CARTESIAN_POINT('Ctrl Pts',(41.0654668578589,1074.8679427817,320.96336554765));
#122265=CARTESIAN_POINT('Ctrl Pts',(41.0121363364488,1074.86611110015,320.927474302055));
#122266=CARTESIAN_POINT('Ctrl Pts',(40.9219662375796,1074.8593183105,320.837152945459));
#122267=CARTESIAN_POINT('Ctrl Pts',(40.8861257096163,1074.85440853092,320.783534500662));
#122268=CARTESIAN_POINT('Ctrl Pts',(40.8363689843546,1074.84197415737,320.66421014995));
#122269=CARTESIAN_POINT('Ctrl Pts',(40.8235619957307,1074.83450870245,320.599426216224));
#122270=CARTESIAN_POINT('Ctrl Pts',(40.8239043346288,1074.82229754514,320.502134287703));
#122271=CARTESIAN_POINT('Ctrl Pts',(40.8271483246973,1074.81813395482,320.47023476108));
#122272=CARTESIAN_POINT('Ctrl Pts',(40.8398022570964,1074.80962223017,320.407485629597));
#122273=CARTESIAN_POINT('Ctrl Pts',(40.8491966197144,1074.80529284422,320.376779305835));
#122274=CARTESIAN_POINT('Ctrl Pts',(40.8867898432869,1074.7920577392,320.28654447439));
#122275=CARTESIAN_POINT('Ctrl Pts',(40.9240193757248,1074.78325330532,320.231528258088));
#122276=CARTESIAN_POINT('Ctrl Pts',(41.017513513941,1074.76698530552,320.139926546507));
#122277=CARTESIAN_POINT('Ctrl Pts',(41.0726737877535,1074.75966276451,320.104012551252));
#122278=CARTESIAN_POINT('Ctrl Pts',(41.1908666812368,1074.74776277432,320.057097400236));
#122279=CARTESIAN_POINT('Ctrl Pts',(41.2522651499211,1074.7431707449,320.045322098179));
#122280=CARTESIAN_POINT('Ctrl Pts',(41.3143294401506,1074.74003968768,320.045322098179));
#122281=CARTESIAN_POINT('',(41.3143294401475,1082.7251047501,320.045322098179));
#122282=CARTESIAN_POINT('',(41.3143294401475,1067.7251047501,320.045322098179));
#122283=CARTESIAN_POINT('Origin',(41.3143294401475,1082.7251047501,320.535862846908));
#122284=CARTESIAN_POINT('Ctrl Pts',(41.3143357717175,1074.74003936826,320.04532209822));
#122285=CARTESIAN_POINT('Ctrl Pts',(41.3781299766579,1074.73682114373,320.045322921633));
#122286=CARTESIAN_POINT('Ctrl Pts',(41.4413545263827,1074.73521147509,320.057768195823));
#122287=CARTESIAN_POINT('Ctrl Pts',(41.5593563747643,1074.73540889194,320.106158929656));
#122288=CARTESIAN_POINT('Ctrl Pts',(41.6129569156641,1074.73720296111,320.141535103922));
#122289=CARTESIAN_POINT('Ctrl Pts',(41.7038314946861,1074.74397664506,320.230906139878));
#122290=CARTESIAN_POINT('Ctrl Pts',(41.7401150978535,1074.74890226474,320.284085696526));
#122291=CARTESIAN_POINT('Ctrl Pts',(41.7905321071453,1074.76127962073,320.40171467661));
#122292=CARTESIAN_POINT('Ctrl Pts',(41.8039575734674,1074.76863453191,320.465124426693));
#122293=CARTESIAN_POINT('Ctrl Pts',(41.8057157905573,1074.78495844504,320.595010761301));
#122294=CARTESIAN_POINT('Ctrl Pts',(41.793362062695,1074.79380651393,320.660267504426));
#122295=CARTESIAN_POINT('Ctrl Pts',(41.7438144368007,1074.81156672865,320.781750903608));
#122296=CARTESIAN_POINT('Ctrl Pts',(41.7071739584895,1074.82031168915,320.836867395503));
#122297=CARTESIAN_POINT('Ctrl Pts',(41.6145238676394,1074.83649756601,320.929277488738));
#122298=CARTESIAN_POINT('Ctrl Pts',(41.5594893696512,1074.84378943367,320.965764438528));
#122299=CARTESIAN_POINT('Ctrl Pts',(41.4402856454316,1074.85573639902,321.014145779283));
#122300=CARTESIAN_POINT('Ctrl Pts',(41.3776473147849,1074.86036214679,321.026403595636));
#122301=CARTESIAN_POINT('Ctrl Pts',(41.3143294401475,1074.86349252611,321.026403595636));
#122302=CARTESIAN_POINT('Origin',(-14.6999478050467,1067.7251047501,336.276664073765));
#122303=CARTESIAN_POINT('',(-14.6999478050671,1076.62893223815,334.798360941572));
#122304=CARTESIAN_POINT('',(-14.6999478050467,1067.7251047501,334.798360941572));
#122305=CARTESIAN_POINT('Ctrl Pts',(-14.7001323799959,1076.70479648561,
337.754967194436));
#122306=CARTESIAN_POINT('Ctrl Pts',(-14.8957174153601,1076.70421870621,
337.754942774479));
#122307=CARTESIAN_POINT('Ctrl Pts',(-15.0893628551477,1076.70295890393,
337.716103585662));
#122308=CARTESIAN_POINT('Ctrl Pts',(-15.4496590785385,1076.69897902633,
337.565577962594));
#122309=CARTESIAN_POINT('Ctrl Pts',(-15.6128648691738,1076.69629503056,
337.45562172281));
#122310=CARTESIAN_POINT('Ctrl Pts',(-15.8877068483204,1076.68946791284,
337.178254670474));
#122311=CARTESIAN_POINT('Ctrl Pts',(-15.9964363629675,1076.68537915515,
337.013376391187));
#122312=CARTESIAN_POINT('Ctrl Pts',(-16.143526651107,1076.6760751074,336.650605313986));
#122313=CARTESIAN_POINT('Ctrl Pts',(-16.1803177063381,1076.67094723356,
336.456248500635));
#122314=CARTESIAN_POINT('Ctrl Pts',(-16.1760250080137,1076.66039506669,
336.066348106327));
#122315=CARTESIAN_POINT('Ctrl Pts',(-16.135702478106,1076.65507972852,335.874609375946));
#122316=CARTESIAN_POINT('Ctrl Pts',(-15.9832429731908,1076.64516680223,
335.517560480363));
#122317=CARTESIAN_POINT('Ctrl Pts',(-15.8725418398901,1076.64067274634,
335.35573025354));
#122318=CARTESIAN_POINT('Ctrl Pts',(-15.5950090525183,1076.63346531469,
335.084230376839));
#122319=CARTESIAN_POINT('Ctrl Pts',(-15.4309223292167,1076.6308271039,334.977156605108));
#122320=CARTESIAN_POINT('Ctrl Pts',(-15.0711758210652,1076.62802354181,
334.832693752177));
#122321=CARTESIAN_POINT('Ctrl Pts',(-14.8790874762117,1076.62788220176,
334.796539023342));
#122322=CARTESIAN_POINT('Ctrl Pts',(-14.492366869078,1076.63014395414,334.800319623269));
#122323=CARTESIAN_POINT('Ctrl Pts',(-14.3014805265477,1076.63251681089,
334.840037186407));
#122324=CARTESIAN_POINT('Ctrl Pts',(-13.9459269105799,1076.63926185274,
334.9905549053));
#122325=CARTESIAN_POINT('Ctrl Pts',(-13.7846630300826,1076.64356169163,
335.099860498032));
#122326=CARTESIAN_POINT('Ctrl Pts',(-13.5131316530228,1076.65320905303,
335.374359106864));
#122327=CARTESIAN_POINT('Ctrl Pts',(-13.405521946531,1076.65845805784,335.536971833433));
#122328=CARTESIAN_POINT('Ctrl Pts',(-13.2955725337978,1076.66632703601,
335.805028646334));
#122329=CARTESIAN_POINT('Ctrl Pts',(-13.2677636227205,1076.66893183358,
335.897772577147));
#122330=CARTESIAN_POINT('Ctrl Pts',(-13.2306355304937,1076.6740168994,336.08736641753));
#122331=CARTESIAN_POINT('Ctrl Pts',(-13.2214072090968,1076.67648492476,
336.183762191161));
#122332=CARTESIAN_POINT('Ctrl Pts',(-13.2221400186975,1076.68362806364,
336.476172445074));
#122333=CARTESIAN_POINT('Ctrl Pts',(-13.2615276495364,1076.68788966242,
336.66995329469));
#122334=CARTESIAN_POINT('Ctrl Pts',(-13.4131658664563,1076.69508381343,
337.030019992103));
#122335=CARTESIAN_POINT('Ctrl Pts',(-13.5235705203483,1076.69795956421,
337.192904836477));
#122336=CARTESIAN_POINT('Ctrl Pts',(-13.8016209096952,1076.70232020223,
337.466871387134));
#122337=CARTESIAN_POINT('Ctrl Pts',(-13.9666897463278,1076.70376629342,
337.575094380905));
#122338=CARTESIAN_POINT('Ctrl Pts',(-14.323521881502,1076.7052676937,337.718701187015));
#122339=CARTESIAN_POINT('Ctrl Pts',(-14.5109563147374,1076.70535533222,
337.754990814194));
#122340=CARTESIAN_POINT('Ctrl Pts',(-14.7001323799959,1076.70479648561,
337.754967194436));
#122341=CARTESIAN_POINT('Origin',(-14.6999478050467,1067.7251047501,336.276664073765));
#122342=CARTESIAN_POINT('',(-14.6999478050467,1076.69331989119,337.154967205958));
#122343=CARTESIAN_POINT('',(-14.6999478049914,1076.64821521145,335.398360941572));
#122344=CARTESIAN_POINT('Ctrl Pts',(-14.6999478050467,1076.69331989119,
337.154967205958));
#122345=CARTESIAN_POINT('Ctrl Pts',(-14.7009690133301,1076.69331631968,
337.154967205958));
#122346=CARTESIAN_POINT('Ctrl Pts',(-14.7019903090399,1076.6933127102,337.154965424911));
#122347=CARTESIAN_POINT('Ctrl Pts',(-14.8197051797538,1076.69289233503,
337.154554784525));
#122348=CARTESIAN_POINT('Ctrl Pts',(-14.9351523343786,1076.69199137635,
337.130895378293));
#122349=CARTESIAN_POINT('Ctrl Pts',(-15.149848331648,1076.68924131929,337.03992980832));
#122350=CARTESIAN_POINT('Ctrl Pts',(-15.2469926280456,1076.68741838492,
336.973603155994));
#122351=CARTESIAN_POINT('Ctrl Pts',(-15.4099403752669,1076.68295357097,
336.806722403128));
#122352=CARTESIAN_POINT('Ctrl Pts',(-15.4740387894439,1076.68035136175,
336.707745689171));
#122353=CARTESIAN_POINT('Ctrl Pts',(-15.5596391832146,1076.67463626738,
336.490889282691));
#122354=CARTESIAN_POINT('Ctrl Pts',(-15.5804295691151,1076.67158052066,
336.375214774509));
#122355=CARTESIAN_POINT('Ctrl Pts',(-15.5757351879597,1076.665450948,336.143680355862));
#122356=CARTESIAN_POINT('Ctrl Pts',(-15.5507610283096,1076.66243812165,
336.030074047769));
#122357=CARTESIAN_POINT('Ctrl Pts',(-15.4583672024248,1076.65691398668,
335.818955908892));
#122358=CARTESIAN_POINT('Ctrl Pts',(-15.3918314957487,1076.6544588038,335.723493769938));
#122359=CARTESIAN_POINT('Ctrl Pts',(-15.2257389425843,1076.65056444469,
335.563764242563));
#122360=CARTESIAN_POINT('Ctrl Pts',(-15.1278164029263,1076.64916478105,
335.50102621267));
#122361=CARTESIAN_POINT('Ctrl Pts',(-14.9183826869667,1076.64773857793,
335.41890461113));
#122362=CARTESIAN_POINT('Ctrl Pts',(-14.8096227972511,1076.64766396979,
335.398360941558));
#122363=CARTESIAN_POINT('Ctrl Pts',(-14.6999478049361,1076.64821521145,
335.398360941572));
#122364=CARTESIAN_POINT('',(-14.6999478050467,1082.7251047501,335.398360941572));
#122365=CARTESIAN_POINT('',(-14.6999478050467,1067.7251047501,335.398360941572));
#122366=CARTESIAN_POINT('Origin',(-14.6999478050467,1082.7251047501,336.276664073765));
#122367=CARTESIAN_POINT('Ctrl Pts',(-14.6999478049361,1076.64821521145,
335.398360941572));
#122368=CARTESIAN_POINT('Ctrl Pts',(-14.6947111011966,1076.64824153184,
335.398360941572));
#122369=CARTESIAN_POINT('Ctrl Pts',(-14.6894723111497,1076.6482692717,335.398407775651));
#122370=CARTESIAN_POINT('Ctrl Pts',(-14.569409954258,1076.64893731845,335.40055643325));
#122371=CARTESIAN_POINT('Ctrl Pts',(-14.4561050216884,1076.65024750165,
335.42511110646));
#122372=CARTESIAN_POINT('Ctrl Pts',(-14.2454119130326,1076.65398123313,
335.516406631954));
#122373=CARTESIAN_POINT('Ctrl Pts',(-14.1500509251862,1076.65636615552,
335.582254989699));
#122374=CARTESIAN_POINT('Ctrl Pts',(-13.9900092290904,1076.66178631504,
335.746948899337));
#122375=CARTESIAN_POINT('Ctrl Pts',(-13.9268930265349,1076.66476739208,
335.844234325778));
#122376=CARTESIAN_POINT('Ctrl Pts',(-13.8645400063229,1076.66921265106,
336.000356130546));
#122377=CARTESIAN_POINT('Ctrl Pts',(-13.8493270604945,1076.67062404865,
336.051504898227));
#122378=CARTESIAN_POINT('Ctrl Pts',(-13.8282750640927,1076.67342571959,
336.156322335976));
#122379=CARTESIAN_POINT('Ctrl Pts',(-13.8225521104539,1076.67480987164,
336.209787600263));
#122380=CARTESIAN_POINT('Ctrl Pts',(-13.8217442258762,1076.67615522911,
336.263440399819));
#122381=CARTESIAN_POINT('Ctrl Pts',(-13.8199848288176,1076.67908512532,
336.380284538617));
#122382=CARTESIAN_POINT('Ctrl Pts',(-13.8415618709421,1076.68178577728,
336.496319632915));
#122383=CARTESIAN_POINT('Ctrl Pts',(-13.9287208200021,1076.68648279568,
336.712773304373));
#122384=CARTESIAN_POINT('Ctrl Pts',(-13.9932886641846,1076.6884375335,336.811096708633));
#122385=CARTESIAN_POINT('Ctrl Pts',(-14.1571383012838,1076.69146843165,
336.976935330054));
#122386=CARTESIAN_POINT('Ctrl Pts',(-14.2548352530162,1076.692516146,337.042757206605));
#122387=CARTESIAN_POINT('Ctrl Pts',(-14.4694686493758,1076.69364587763,
337.132064727983));
#122388=CARTESIAN_POINT('Ctrl Pts',(-14.5841461198548,1076.69372488816,
337.154967205958));
#122389=CARTESIAN_POINT('Ctrl Pts',(-14.6999478050467,1076.69331989119,
337.154967205958));
#122390=CARTESIAN_POINT('Origin',(-5.22978306525612,1067.7251047501,328.028873070842));
#122391=CARTESIAN_POINT('',(-5.22978306527338,1076.25871334817,326.753428949706));
#122392=CARTESIAN_POINT('',(-5.22978306525612,1067.7251047501,326.753428949706));
#122393=CARTESIAN_POINT('Ctrl Pts',(-5.22980002134218,1076.42335631864,
329.304317191865));
#122394=CARTESIAN_POINT('Ctrl Pts',(-5.39871008864912,1076.42281868721,
329.304314946331));
#122395=CARTESIAN_POINT('Ctrl Pts',(-5.5659217275966,1076.42032080269,329.27075924164));
#122396=CARTESIAN_POINT('Ctrl Pts',(-5.87732970737173,1076.41159226847,
329.140578640962));
#122397=CARTESIAN_POINT('Ctrl Pts',(-6.01845082508294,1076.40544851869,
329.045323293699));
#122398=CARTESIAN_POINT('Ctrl Pts',(-6.25583188549957,1076.39007218768,
328.805140032806));
#122399=CARTESIAN_POINT('Ctrl Pts',(-6.34957526252597,1076.38097658469,
328.662428174666));
#122400=CARTESIAN_POINT('Ctrl Pts',(-6.4437826020366,1076.36598863353,328.428685660021));
#122401=CARTESIAN_POINT('Ctrl Pts',(-6.46721545286191,1076.36085853699,
328.348877497224));
#122402=CARTESIAN_POINT('Ctrl Pts',(-6.49850324657515,1076.35025697929,
328.18450719843));
#122403=CARTESIAN_POINT('Ctrl Pts',(-6.50601640248389,1076.34480694621,
328.100286993975));
#122404=CARTESIAN_POINT('Ctrl Pts',(-6.5034629094911,1076.32844751407,327.848318943459));
#122405=CARTESIAN_POINT('Ctrl Pts',(-6.46873196795216,1076.31761440162,
327.682634354775));
#122406=CARTESIAN_POINT('Ctrl Pts',(-6.33715013572135,1076.29740617211,
327.374196116182));
#122407=CARTESIAN_POINT('Ctrl Pts',(-6.24157877707444,1076.2882291901,327.234407631844));
#122408=CARTESIAN_POINT('Ctrl Pts',(-6.0019832135847,1076.27300620447,327.000047598259));
#122409=CARTESIAN_POINT('Ctrl Pts',(-5.8604023862094,1076.26710555059,326.907652267113));
#122410=CARTESIAN_POINT('Ctrl Pts',(-5.5500800430281,1076.25958131043,326.783072665468));
#122411=CARTESIAN_POINT('Ctrl Pts',(-5.38448313634122,1076.25801833975,
326.751888435179));
#122412=CARTESIAN_POINT('Ctrl Pts',(-5.05111387272699,1076.25950720414,
326.75508203554));
#122413=CARTESIAN_POINT('Ctrl Pts',(-4.88661425568984,1076.26253097892,
326.789245222799));
#122414=CARTESIAN_POINT('Ctrl Pts',(-4.58007283918707,1076.27269469094,
326.918772839875));
#122415=CARTESIAN_POINT('Ctrl Pts',(-4.44100867108024,1076.27973281541,
327.01288271623));
#122416=CARTESIAN_POINT('Ctrl Pts',(-4.20660263042861,1076.29674796525,
327.249354942443));
#122417=CARTESIAN_POINT('Ctrl Pts',(-4.11362655130575,1076.30656481447,
327.389571834589));
#122418=CARTESIAN_POINT('Ctrl Pts',(-4.01849713856952,1076.32227319417,
327.620818220311));
#122419=CARTESIAN_POINT('Ctrl Pts',(-3.99440092444456,1076.3276417906,327.700922507677));
#122420=CARTESIAN_POINT('Ctrl Pts',(-3.96219290797154,1076.33846635749,
327.864725572457));
#122421=CARTESIAN_POINT('Ctrl Pts',(-3.95416735250404,1076.34389666082,
327.948038155783));
#122422=CARTESIAN_POINT('Ctrl Pts',(-3.9546907780537,1076.36000641825,328.198680620265));
#122423=CARTESIAN_POINT('Ctrl Pts',(-3.98789229642846,1076.37033621946,
328.364177170258));
#122424=CARTESIAN_POINT('Ctrl Pts',(-4.11689228092931,1076.38917183608,
328.674403822433));
#122425=CARTESIAN_POINT('Ctrl Pts',(-4.21199517874441,1076.39747873865,
328.815883529567));
#122426=CARTESIAN_POINT('Ctrl Pts',(-4.45169695792621,1076.41101550019,
329.05345514243));
#122427=CARTESIAN_POINT('Ctrl Pts',(-4.59384341222352,1076.41612139346,
329.14726512928));
#122428=CARTESIAN_POINT('Ctrl Pts',(-4.90250109010282,1076.42253561259,
329.272525358247));
#122429=CARTESIAN_POINT('Ctrl Pts',(-5.06537340948472,1076.42387967949,
329.304319377796));
#122430=CARTESIAN_POINT('Ctrl Pts',(-5.22980002134219,1076.42335631864,
329.304317191866));
#122431=CARTESIAN_POINT('Origin',(-5.22978306525612,1067.7251047501,328.028873070842));
#122432=CARTESIAN_POINT('',(-5.22978306525612,1076.38762615333,328.704317191978));
#122433=CARTESIAN_POINT('',(-5.22978306525612,1076.30041692086,327.353428949706));
#122434=CARTESIAN_POINT('Ctrl Pts',(-5.22978306525612,1076.38762615333,
328.704317191978));
#122435=CARTESIAN_POINT('Ctrl Pts',(-5.23150159288228,1076.38762042817,
328.704317191978));
#122436=CARTESIAN_POINT('Ctrl Pts',(-5.23322043819156,1076.38761429833,
328.704310633325));
#122437=CARTESIAN_POINT('Ctrl Pts',(-5.32469806735429,1076.38726656726,
328.703612251232));
#122438=CARTESIAN_POINT('Ctrl Pts',(-5.41340925249523,1076.38583007508,
328.685041934543));
#122439=CARTESIAN_POINT('Ctrl Pts',(-5.57840986133551,1076.38090364662,
328.61431840182));
#122440=CARTESIAN_POINT('Ctrl Pts',(-5.65303014191035,1076.37746078315,
328.562855613516));
#122441=CARTESIAN_POINT('Ctrl Pts',(-5.77797587655441,1076.36894858366,
328.433615026693));
#122442=CARTESIAN_POINT('Ctrl Pts',(-5.82696387717909,1076.36395756775,
328.357042943192));
#122443=CARTESIAN_POINT('Ctrl Pts',(-5.87545701961128,1076.35583555273,
328.232036422869));
#122444=CARTESIAN_POINT('Ctrl Pts',(-5.8873412449498,1076.35307295674,328.189455342913));
#122445=CARTESIAN_POINT('Ctrl Pts',(-5.90273979728353,1076.3474050146,328.10202024457));
#122446=CARTESIAN_POINT('Ctrl Pts',(-5.90610384351652,1076.34451200176,
328.057355719052));
#122447=CARTESIAN_POINT('Ctrl Pts',(-5.90290750237631,1076.33588076271,
327.923997444573));
#122448=CARTESIAN_POINT('Ctrl Pts',(-5.88332825018665,1076.33023000309,
327.836572457998));
#122449=CARTESIAN_POINT('Ctrl Pts',(-5.81149381182939,1076.31979054399,
327.674326511174));
#122450=CARTESIAN_POINT('Ctrl Pts',(-5.75995094481466,1076.31510288466,
327.601059445507));
#122451=CARTESIAN_POINT('Ctrl Pts',(-5.63157738022333,1076.3073944345,327.478757479008));
#122452=CARTESIAN_POINT('Ctrl Pts',(-5.55605322117435,1076.30444602716,
327.430855883987));
#122453=CARTESIAN_POINT('Ctrl Pts',(-5.3957101543754,1076.30085281192,327.368848489771));
#122454=CARTESIAN_POINT('Ctrl Pts',(-5.31311406372096,1076.30011236494,
327.353430235009));
#122455=CARTESIAN_POINT('Ctrl Pts',(-5.2297934839294,1076.30041688277,327.353428949791));
#122456=CARTESIAN_POINT('Ctrl Pts',(-5.22979001103696,1076.30041689547,
327.353428949737));
#122457=CARTESIAN_POINT('Ctrl Pts',(-5.22978653814587,1076.30041690816,
327.353428949706));
#122458=CARTESIAN_POINT('Ctrl Pts',(-5.22978306525612,1076.30041692086,
327.353428949706));
#122459=CARTESIAN_POINT('',(-5.22978306525612,1082.7251047501,327.353428949706));
#122460=CARTESIAN_POINT('',(-5.22978306525612,1067.7251047501,327.353428949706));
#122461=CARTESIAN_POINT('Origin',(-5.22978306525612,1082.7251047501,328.028873070842));
#122462=CARTESIAN_POINT('Ctrl Pts',(-5.22978306525612,1076.30041692086,
327.353428949706));
#122463=CARTESIAN_POINT('Ctrl Pts',(-5.14157676647768,1076.30073938674,
327.353428949706));
#122464=CARTESIAN_POINT('Ctrl Pts',(-5.05423792967729,1076.30222686055,
327.370706767218));
#122465=CARTESIAN_POINT('Ctrl Pts',(-4.89112798246151,1076.30733494484,
327.43784075922));
#122466=CARTESIAN_POINT('Ctrl Pts',(-4.81694914848848,1076.31090587175,
327.487058810574));
#122467=CARTESIAN_POINT('Ctrl Pts',(-4.69157712628812,1076.31962785362,
327.611300922366));
#122468=CARTESIAN_POINT('Ctrl Pts',(-4.64164741770922,1076.32469737144,
327.685189581609));
#122469=CARTESIAN_POINT('Ctrl Pts',(-4.59018686609572,1076.33288805052,
327.807297470601));
#122470=CARTESIAN_POINT('Ctrl Pts',(-4.57706081607156,1076.33569860303,
327.849618819418));
#122471=CARTESIAN_POINT('Ctrl Pts',(-4.55926121635584,1076.34139282905,
327.936237453764));
#122472=CARTESIAN_POINT('Ctrl Pts',(-4.554635302571,1076.34426301577,327.980330348298));
#122473=CARTESIAN_POINT('Ctrl Pts',(-4.55378680854414,1076.35282244118,
328.113133712064));
#122474=CARTESIAN_POINT('Ctrl Pts',(-4.57065005764883,1076.35836941536,
328.200980577174));
#122475=CARTESIAN_POINT('Ctrl Pts',(-4.63782053446517,1076.36860395823,
328.366334551107));
#122476=CARTESIAN_POINT('Ctrl Pts',(-4.68792980095587,1076.37317792213,
328.44203993191));
#122477=CARTESIAN_POINT('Ctrl Pts',(-4.81475200576151,1076.38067821524,
328.569263487384));
#122478=CARTESIAN_POINT('Ctrl Pts',(-4.89013394019629,1076.38353503896,
328.619568660416));
#122479=CARTESIAN_POINT('Ctrl Pts',(-5.05459613291234,1076.38715314282,
328.687115392195));
#122480=CARTESIAN_POINT('Ctrl Pts',(-5.14177299919702,1076.38791935332,
328.704317191978));
#122481=CARTESIAN_POINT('Ctrl Pts',(-5.22978306525612,1076.38762615333,
328.704317191978));
#122482=CARTESIAN_POINT('Origin',(5.99814689883732,1067.7251047501,319.92012190144));
#122483=CARTESIAN_POINT('',(5.99814689885421,1077.55052528867,318.821290765448));
#122484=CARTESIAN_POINT('Ctrl Pts',(5.99813818557661,1077.77685023714,321.018953037398));
#122485=CARTESIAN_POINT('Ctrl Pts',(6.03402897129008,1077.77664671849,321.018953321997));
#122486=CARTESIAN_POINT('Ctrl Pts',(6.06989643802268,1077.77626924974,321.017195170753));
#122487=CARTESIAN_POINT('Ctrl Pts',(6.17620552639777,1077.77463143461,321.00674815849));
#122488=CARTESIAN_POINT('Ctrl Pts',(6.24594597955941,1077.77287303179,320.992993074577));
#122489=CARTESIAN_POINT('Ctrl Pts',(6.45377180865714,1077.76550514219,320.930652940034));
#122490=CARTESIAN_POINT('Ctrl Pts',(6.58379753294961,1077.7578662106,320.86124351676));
#122491=CARTESIAN_POINT('Ctrl Pts',(6.79256249897359,1077.73947535801,320.689435887432));
#122492=CARTESIAN_POINT('Ctrl Pts',(6.87449189597205,1077.72947345924,320.594591294463));
#122493=CARTESIAN_POINT('Ctrl Pts',(7.00828522979832,1077.70628616274,320.373040185438));
#122494=CARTESIAN_POINT('Ctrl Pts',(7.05604257103551,1077.69309841382,320.246205023341));
#122495=CARTESIAN_POINT('Ctrl Pts',(7.10524446530176,1077.66466058666,319.971700421772));
#122496=CARTESIAN_POINT('Ctrl Pts',(7.10242385109399,1077.64959635674,319.825760756618));
#122497=CARTESIAN_POINT('Ctrl Pts',(7.04047630273029,1077.62059346521,319.543525880911));
#122498=CARTESIAN_POINT('Ctrl Pts',(6.98200714074261,1077.60692740777,319.409869716104));
#122499=CARTESIAN_POINT('Ctrl Pts',(6.82220397605965,1077.58375388275,319.180872799465));
#122500=CARTESIAN_POINT('Ctrl Pts',(6.72543431367814,1077.57422145046,319.085448010837));
#122501=CARTESIAN_POINT('Ctrl Pts',(6.51859700134971,1077.56060975366,318.945576404004));
#122502=CARTESIAN_POINT('Ctrl Pts',(6.41395855628505,1077.55601580324,318.896530792454));
#122503=CARTESIAN_POINT('Ctrl Pts',(6.25908125103286,1077.55217888507,318.851717900121));
#122504=CARTESIAN_POINT('Ctrl Pts',(6.21382852968329,1077.55138256315,318.841671041601));
#122505=CARTESIAN_POINT('Ctrl Pts',(6.13810911774021,1077.55057980112,318.829819094664));
#122506=CARTESIAN_POINT('Ctrl Pts',(6.10796415248247,1077.55039594371,318.826371517131));
#122507=CARTESIAN_POINT('Ctrl Pts',(6.04934396738986,1077.55030002877,318.822115593108));
#122508=CARTESIAN_POINT('Ctrl Pts',(6.02090449053742,1077.55037183287,318.821158275126));
#122509=CARTESIAN_POINT('Ctrl Pts',(5.95516186915943,1077.55081059801,318.821498507502));
#122510=CARTESIAN_POINT('Ctrl Pts',(5.91789992129018,1077.55126218835,318.823590490068));
#122511=CARTESIAN_POINT('Ctrl Pts',(5.80468741502161,1077.55325336375,318.835748275193));
#122512=CARTESIAN_POINT('Ctrl Pts',(5.72964185224664,1077.55543241902,318.851856583078));
#122513=CARTESIAN_POINT('Ctrl Pts',(5.5180690553479,1077.56409248179,318.920978794798));
#122514=CARTESIAN_POINT('Ctrl Pts',(5.38980380252459,1077.57259517038,318.993514882065));
#122515=CARTESIAN_POINT('Ctrl Pts',(5.18501286018711,1077.59256525408,319.170555573244));
#122516=CARTESIAN_POINT('Ctrl Pts',(5.10520765179409,1077.60328663014,319.26770684178));
#122517=CARTESIAN_POINT('Ctrl Pts',(4.97682703080281,1077.62765395393,319.492986858509));
#122518=CARTESIAN_POINT('Ctrl Pts',(4.93226986812911,1077.64126162121,319.621100347007));
#122519=CARTESIAN_POINT('Ctrl Pts',(4.89011008043779,1077.67001296525,319.896780935986));
#122520=CARTESIAN_POINT('Ctrl Pts',(4.89663199986748,1077.68492539953,320.042505340985));
#122521=CARTESIAN_POINT('Ctrl Pts',(4.96566438556969,1077.71307929742,320.322880898688));
#122522=CARTESIAN_POINT('Ctrl Pts',(5.027419178452,1077.7260593628,320.454904094474));
#122523=CARTESIAN_POINT('Ctrl Pts',(5.19233780381988,1077.7476326199,320.679074630057));
#122524=CARTESIAN_POINT('Ctrl Pts',(5.29073536817695,1077.75630093277,320.771572677047));
#122525=CARTESIAN_POINT('Ctrl Pts',(5.49533855247392,1077.76823964554,320.90325598723));
#122526=CARTESIAN_POINT('Ctrl Pts',(5.59557219190474,1077.77214426792,320.94838508845));
#122527=CARTESIAN_POINT('Ctrl Pts',(5.74421632212992,1077.77543953415,320.990157912074));
#122528=CARTESIAN_POINT('Ctrl Pts',(5.7882815736842,1077.77613099893,320.999665830365));
#122529=CARTESIAN_POINT('Ctrl Pts',(5.86233075455628,1077.77682681649,321.010936056465));
#122530=CARTESIAN_POINT('Ctrl Pts',(5.89202334245002,1077.77698389273,321.014224004991));
#122531=CARTESIAN_POINT('Ctrl Pts',(5.94721680696162,1077.77705135174,321.018067459556));
#122532=CARTESIAN_POINT('Ctrl Pts',(5.97267374842211,1077.77699463319,321.018952835476));
#122533=CARTESIAN_POINT('Ctrl Pts',(5.99813818557661,1077.77685023714,321.018953037398));
#122534=CARTESIAN_POINT('',(5.99814689882034,1075.53855673557,318.821290765448));
#122535=CARTESIAN_POINT('',(5.99814689883732,1067.7251047501,318.821290765448));
#122536=CARTESIAN_POINT('Ctrl Pts',(5.99814215972078,1075.76695402288,321.018953037423));
#122537=CARTESIAN_POINT('Ctrl Pts',(5.8520632422525,1075.76779012951,321.018952407403));
#122538=CARTESIAN_POINT('Ctrl Pts',(5.70748007846799,1075.76571137799,320.989822594062));
#122539=CARTESIAN_POINT('Ctrl Pts',(5.43836269523627,1075.75594245909,320.876859596151));
#122540=CARTESIAN_POINT('Ctrl Pts',(5.31656708136263,1075.74835604039,320.794240606573));
#122541=CARTESIAN_POINT('Ctrl Pts',(5.11225111323726,1075.72854766061,320.586373200309));
#122542=CARTESIAN_POINT('Ctrl Pts',(5.03184052795361,1075.71651409246,320.463144520239));
#122543=CARTESIAN_POINT('Ctrl Pts',(4.92340990019868,1075.68940727686,320.191876799852));
#122544=CARTESIAN_POINT('Ctrl Pts',(4.89681414578907,1075.67457833951,320.046343626292));
#122545=CARTESIAN_POINT('Ctrl Pts',(4.90082033537793,1075.65189539804,319.828060324323));
#122546=CARTESIAN_POINT('Ctrl Pts',(4.90919448778044,1075.64438522352,319.75646364717));
#122547=CARTESIAN_POINT('Ctrl Pts',(4.95560403582249,1075.62183169916,319.543456432126));
#122548=CARTESIAN_POINT('Ctrl Pts',(5.01488014313486,1075.60722242713,319.408252145682));
#122549=CARTESIAN_POINT('Ctrl Pts',(5.1819575818043,1075.58098895896,319.170373367996));
#122550=CARTESIAN_POINT('Ctrl Pts',(5.28754186240645,1075.56958294292,319.069585267379));
#122551=CARTESIAN_POINT('Ctrl Pts',(5.53119986459102,1075.55154162309,318.915101627791));
#122552=CARTESIAN_POINT('Ctrl Pts',(5.66667436248557,1075.54505598575,318.86262643622));
#122553=CARTESIAN_POINT('Ctrl Pts',(5.94958340526732,1075.53797150875,318.813063661307));
#122554=CARTESIAN_POINT('Ctrl Pts',(6.09412503465963,1075.53741155264,318.81616050575));
#122555=CARTESIAN_POINT('Ctrl Pts',(6.37370239329595,1075.54230703978,318.877603496269));
#122556=CARTESIAN_POINT('Ctrl Pts',(6.50596325036728,1075.54770443986,318.935259734272));
#122557=CARTESIAN_POINT('Ctrl Pts',(6.74132532924915,1075.56372765755,319.098127177709));
#122558=CARTESIAN_POINT('Ctrl Pts',(6.84200443907265,1075.57421391683,319.201921968478));
#122559=CARTESIAN_POINT('Ctrl Pts',(6.99830220519505,1075.59885591519,319.442773031183));
#122560=CARTESIAN_POINT('Ctrl Pts',(7.05213167518135,1075.61279646497,319.577734835983));
#122561=CARTESIAN_POINT('Ctrl Pts',(7.09163764881545,1075.63483204805,319.790065273794));
#122562=CARTESIAN_POINT('Ctrl Pts',(7.0978154874518,1075.64232752601,319.862126551262));
#122563=CARTESIAN_POINT('Ctrl Pts',(7.09596075417271,1075.65734489128,320.006231284631));
#122564=CARTESIAN_POINT('Ctrl Pts',(7.0879657580583,1075.66483193062,320.077941104531));
#122565=CARTESIAN_POINT('Ctrl Pts',(7.04266969368658,1075.68714864385,320.291260197174));
#122566=CARTESIAN_POINT('Ctrl Pts',(6.98410971497628,1075.70138589349,320.426785277514));
#122567=CARTESIAN_POINT('Ctrl Pts',(6.81765790554724,1075.72677144719,320.666448688881));
#122568=CARTESIAN_POINT('Ctrl Pts',(6.71165676234959,1075.73769031499,320.768407327162));
#122569=CARTESIAN_POINT('Ctrl Pts',(6.46581951217859,1075.75488418721,320.925084279348));
#122570=CARTESIAN_POINT('Ctrl Pts',(6.3284757494544,1075.76099042824,320.978238176426));
#122571=CARTESIAN_POINT('Ctrl Pts',(6.12305966386463,1075.76570599713,321.013617894088));
#122572=CARTESIAN_POINT('Ctrl Pts',(6.06066155676042,1075.76659618286,321.018953307061));
#122573=CARTESIAN_POINT('Ctrl Pts',(5.99814215972077,1075.76695402288,321.018953037423));
#122574=CARTESIAN_POINT('Origin',(5.99814689883732,1067.7251047501,319.92012190144));
#122575=CARTESIAN_POINT('',(5.99814689883734,1075.70679891916,320.418953037433));
#122576=CARTESIAN_POINT('',(5.99814689883732,1075.60310529675,319.421290765448));
#122577=CARTESIAN_POINT('Ctrl Pts',(5.99814689883733,1075.70679891916,320.418953037433));
#122578=CARTESIAN_POINT('Ctrl Pts',(5.96441846974092,1075.70699626532,320.418953037433));
#122579=CARTESIAN_POINT('Ctrl Pts',(5.93069536794872,1075.70684424762,320.415532205603));
#122580=CARTESIAN_POINT('Ctrl Pts',(5.83377706009526,1075.70537201006,320.395567176941));
#122581=CARTESIAN_POINT('Ctrl Pts',(5.77327328762252,1075.70312564208,320.37010782257));
#122582=CARTESIAN_POINT('Ctrl Pts',(5.66422493924436,1075.69624140982,320.296622433145));
#122583=CARTESIAN_POINT('Ctrl Pts',(5.61711214887369,1075.69161867454,320.248834122477));
#122584=CARTESIAN_POINT('Ctrl Pts',(5.54428472231775,1075.68060086452,320.137557262403));
#122585=CARTESIAN_POINT('Ctrl Pts',(5.51936898699363,1075.6743093303,320.075128000783));
#122586=CARTESIAN_POINT('Ctrl Pts',(5.50157357306298,1075.66432386098,319.977648817592));
#122587=CARTESIAN_POINT('Ctrl Pts',(5.49887761981519,1075.6609649492,319.94510039372));
#122588=CARTESIAN_POINT('Ctrl Pts',(5.49987058814139,1075.65418528476,319.879885292506));
#122589=CARTESIAN_POINT('Ctrl Pts',(5.50357083567267,1075.65078007968,319.84736919866));
#122590=CARTESIAN_POINT('Ctrl Pts',(5.52447286235389,1075.6405052714,319.749977334952));
#122591=CARTESIAN_POINT('Ctrl Pts',(5.55157271801686,1075.6338558112,319.687960042484));
#122592=CARTESIAN_POINT('Ctrl Pts',(5.62782968782083,1075.62202739303,319.579552702453));
#122593=CARTESIAN_POINT('Ctrl Pts',(5.67573429197332,1075.61693167691,319.53387141516));
#122594=CARTESIAN_POINT('Ctrl Pts',(5.78626645296075,1075.60888384346,319.463839833566));
#122595=CARTESIAN_POINT('Ctrl Pts',(5.8477201001261,1075.60599824989,319.440047475464));
#122596=CARTESIAN_POINT('Ctrl Pts',(5.94048365436939,1075.60371931919,319.423795457181));
#122597=CARTESIAN_POINT('Ctrl Pts',(5.96928596170959,1075.6032800873,319.421290779236));
#122598=CARTESIAN_POINT('Ctrl Pts',(5.99814666053062,1075.6031052982,319.421290765448));
#122599=CARTESIAN_POINT('',(5.99814689883732,1082.7251047501,319.421290765448));
#122600=CARTESIAN_POINT('',(5.99814689883732,1067.7251047501,319.421290765448));
#122601=CARTESIAN_POINT('Origin',(5.99814689883732,1082.7251047501,319.92012190144));
#122602=CARTESIAN_POINT('Ctrl Pts',(5.99814689883732,1075.60310529675,319.421290765448));
#122603=CARTESIAN_POINT('Ctrl Pts',(6.06311539178196,1075.60271183123,319.421290765448));
#122604=CARTESIAN_POINT('Ctrl Pts',(6.12744245729569,1075.60366470266,319.433982617426));
#122605=CARTESIAN_POINT('Ctrl Pts',(6.24768404791999,1075.60814847313,319.483322509358));
#122606=CARTESIAN_POINT('Ctrl Pts',(6.30239155130446,1075.6116386024,319.519518727233));
#122607=CARTESIAN_POINT('Ctrl Pts',(6.39505069803708,1075.62070993086,319.61099203887));
#122608=CARTESIAN_POINT('Ctrl Pts',(6.43200846161313,1075.62621351316,319.665481246679));
#122609=CARTESIAN_POINT('Ctrl Pts',(6.48300583552815,1075.63851005159,319.785811662801));
#122610=CARTESIAN_POINT('Ctrl Pts',(6.49642641021656,1075.64519299541,319.850573521958));
#122611=CARTESIAN_POINT('Ctrl Pts',(6.49722829744655,1075.65540057616,319.948712305593));
#122612=CARTESIAN_POINT('Ctrl Pts',(6.49428573182464,1075.65880628682,319.981327562342));
#122613=CARTESIAN_POINT('Ctrl Pts',(6.47572426394299,1075.66902696246,320.078815924131));
#122614=CARTESIAN_POINT('Ctrl Pts',(6.45030022400967,1075.67561331809,320.141102859008));
#122615=CARTESIAN_POINT('Ctrl Pts',(6.37656230478856,1075.68745878926,320.251848514706));
#122616=CARTESIAN_POINT('Ctrl Pts',(6.32906250043543,1075.69260689519,320.299269679326));
#122617=CARTESIAN_POINT('Ctrl Pts',(6.21823285328952,1075.70078131365,320.372675577079));
#122618=CARTESIAN_POINT('Ctrl Pts',(6.15605483786203,1075.70372887614,320.397951468107));
#122619=CARTESIAN_POINT('Ctrl Pts',(6.06011541117237,1075.70614157331,320.416066641399));
#122620=CARTESIAN_POINT('Ctrl Pts',(6.0291289075029,1075.70661764241,320.418953037433));
#122621=CARTESIAN_POINT('Ctrl Pts',(5.99814689883733,1075.70679891916,320.418953037433));
#122622=CARTESIAN_POINT('Origin',(18.7711528398115,1067.7251047501,314.220624181303));
#122623=CARTESIAN_POINT('',(18.7711528398304,1076.67369445817,313.130083432575));
#122624=CARTESIAN_POINT('Ctrl Pts',(18.7711740718832,1076.96239192968,315.311164929825));
#122625=CARTESIAN_POINT('Ctrl Pts',(18.8565499206275,1076.96051699849,315.311163267617));
#122626=CARTESIAN_POINT('Ctrl Pts',(18.9415846564319,1076.95735423103,315.301135976198));
#122627=CARTESIAN_POINT('Ctrl Pts',(19.1311831022978,1076.94732452807,315.255843937261));
#122628=CARTESIAN_POINT('Ctrl Pts',(19.2332557852884,1076.93971748319,315.214459674833));
#122629=CARTESIAN_POINT('Ctrl Pts',(19.4322313852995,1076.91999789434,315.096477580774));
#122630=CARTESIAN_POINT('Ctrl Pts',(19.5257834587689,1076.90760984435,315.01723865809));
#122631=CARTESIAN_POINT('Ctrl Pts',(19.6896281664456,1076.87860994378,314.823276719968));
#122632=CARTESIAN_POINT('Ctrl Pts',(19.7558161700798,1076.8619549548,314.707608257872));
#122633=CARTESIAN_POINT('Ctrl Pts',(19.8470622156246,1076.82577039875,314.448668701238));
#122634=CARTESIAN_POINT('Ctrl Pts',(19.8676238443435,1076.80644410249,314.30628029851));
#122635=CARTESIAN_POINT('Ctrl Pts',(19.8527409615674,1076.76870378821,314.02017626805));
#122636=CARTESIAN_POINT('Ctrl Pts',(19.8168462631533,1076.75065099957,313.879104658375));
#122637=CARTESIAN_POINT('Ctrl Pts',(19.6959591480312,1076.71958386177,313.627087015878));
#122638=CARTESIAN_POINT('Ctrl Pts',(19.6152440639234,1076.70658793918,313.516934170119));
#122639=CARTESIAN_POINT('Ctrl Pts',(19.4206920631347,1076.68647743287,313.334909402774));
#122640=CARTESIAN_POINT('Ctrl Pts',(19.3097508668743,1076.67934092959,313.26334533726));
#122641=CARTESIAN_POINT('Ctrl Pts',(19.1467556238646,1076.67394628016,313.195804475051));
#122642=CARTESIAN_POINT('Ctrl Pts',(19.1038406874721,1076.67293970615,313.181079460163));
#122643=CARTESIAN_POINT('Ctrl Pts',(19.0336632541015,1076.67194328844,313.161794376889));
#122644=CARTESIAN_POINT('Ctrl Pts',(19.006934431174,1076.67170933742,313.155523503489));
#122645=CARTESIAN_POINT('Ctrl Pts',(18.958493776337,1076.67154464163,313.146071967829));
#122646=CARTESIAN_POINT('Ctrl Pts',(18.9368697139823,1076.67156228046,313.142525390757));
#122647=CARTESIAN_POINT('Ctrl Pts',(18.8863227687454,1076.67181449815,313.135791946905));
#122648=CARTESIAN_POINT('Ctrl Pts',(18.8573514578252,1076.67211815113,313.133106501733));
#122649=CARTESIAN_POINT('Ctrl Pts',(18.7760127610326,1076.6734137555,313.128837595686));
#122650=CARTESIAN_POINT('Ctrl Pts',(18.7235995544648,1076.67476037677,313.129864090982));
#122651=CARTESIAN_POINT('Ctrl Pts',(18.5272316905924,1076.68172290723,313.14788783336));
#122652=CARTESIAN_POINT('Ctrl Pts',(18.387274609478,1076.69060574131,313.189709918569));
#122653=CARTESIAN_POINT('Ctrl Pts',(18.1537486489474,1076.71268883386,313.3137173955));
#122654=CARTESIAN_POINT('Ctrl Pts',(18.0579679195659,1076.72474532902,313.386985085639));
#122655=CARTESIAN_POINT('Ctrl Pts',(17.8869006773265,1076.75308924173,313.569195688427));
#122656=CARTESIAN_POINT('Ctrl Pts',(17.8155509647045,1076.76943533832,313.679315750208));
#122657=CARTESIAN_POINT('Ctrl Pts',(17.7111546376568,1076.80497054691,313.92852096586));
#122658=CARTESIAN_POINT('Ctrl Pts',(17.6824280302455,1076.82397007963,314.06701414303));
#122659=CARTESIAN_POINT('Ctrl Pts',(17.6789078331298,1076.86159801367,314.351718371588));
#122660=CARTESIAN_POINT('Ctrl Pts',(17.7058887326829,1076.8798450509,314.495380783429));
#122661=CARTESIAN_POINT('Ctrl Pts',(17.8120190855963,1076.91175911336,314.757641847138));
#122662=CARTESIAN_POINT('Ctrl Pts',(17.8876879721164,1076.92532286863,314.874791524117));
#122663=CARTESIAN_POINT('Ctrl Pts',(18.0817104693889,1076.94733857193,315.077447522578));
#122664=CARTESIAN_POINT('Ctrl Pts',(18.1992413928995,1076.95543054713,315.160035366346));
#122665=CARTESIAN_POINT('Ctrl Pts',(18.3746981532943,1076.96161699663,315.237750606446));
#122666=CARTESIAN_POINT('Ctrl Pts',(18.4212117517483,1076.96278147958,315.254677246983));
#122667=CARTESIAN_POINT('Ctrl Pts',(18.4961788547779,1076.96392961285,315.27631592709));
#122668=CARTESIAN_POINT('Ctrl Pts',(18.5239370633942,1076.96420373902,315.28315901993));
#122669=CARTESIAN_POINT('Ctrl Pts',(18.575504662916,1076.96443793567,315.293741098617));
#122670=CARTESIAN_POINT('Ctrl Pts',(18.5992296758164,1076.96444072701,315.297796665258));
#122671=CARTESIAN_POINT('Ctrl Pts',(18.6510687077741,1076.96422007506,315.304901642252));
#122672=CARTESIAN_POINT('Ctrl Pts',(18.6792053473891,1076.96395716417,315.307649170701));
#122673=CARTESIAN_POINT('Ctrl Pts',(18.7286471402936,1076.96324547549,315.310543772322));
#122674=CARTESIAN_POINT('Ctrl Pts',(18.7499090730405,1076.96285892837,315.31116534384));
#122675=CARTESIAN_POINT('Ctrl Pts',(18.7711740718832,1076.96239192968,315.311164929825));
#122676=CARTESIAN_POINT('',(18.7711528397839,1074.65422628875,313.130083432575));
#122677=CARTESIAN_POINT('',(18.7711528398115,1067.7251047501,313.130083432575));
#122678=CARTESIAN_POINT('Ctrl Pts',(18.7711532049613,1074.94531438668,315.311164930032));
#122679=CARTESIAN_POINT('Ctrl Pts',(18.6295126016433,1074.94845071869,315.311164977458));
#122680=CARTESIAN_POINT('Ctrl Pts',(18.489229947793,1074.94796418247,315.283570179508));
#122681=CARTESIAN_POINT('Ctrl Pts',(18.2267237729283,1074.93978639499,315.176157584916));
#122682=CARTESIAN_POINT('Ctrl Pts',(18.1072149318836,1074.93215740244,315.097287744657));
#122683=CARTESIAN_POINT('Ctrl Pts',(17.9029672783477,1074.91041133747,314.896289324538));
#122684=CARTESIAN_POINT('Ctrl Pts',(17.8211634545652,1074.89637264129,314.77528758755));
#122685=CARTESIAN_POINT('Ctrl Pts',(17.7092090647952,1074.86368561375,314.50812596384));
#122686=CARTESIAN_POINT('Ctrl Pts',(17.6804647626921,1074.845328699,314.364440658711));
#122687=CARTESIAN_POINT('Ctrl Pts',(17.6806852961651,1074.81659288248,314.148331197341));
#122688=CARTESIAN_POINT('Ctrl Pts',(17.6877266598991,1074.8069732511,314.077340547243));
#122689=CARTESIAN_POINT('Ctrl Pts',(17.7302684298483,1074.77748284186,313.863797989307));
#122690=CARTESIAN_POINT('Ctrl Pts',(17.7876191912421,1074.7578316948,313.72718186224));
#122691=CARTESIAN_POINT('Ctrl Pts',(17.9513659157638,1074.72172657867,313.487216582186));
#122692=CARTESIAN_POINT('Ctrl Pts',(18.0551863687773,1074.70555474421,313.385482955735));
#122693=CARTESIAN_POINT('Ctrl Pts',(18.29564469102,1074.67873327706,313.228880973402));
#122694=CARTESIAN_POINT('Ctrl Pts',(18.4296096178777,1074.66829510334,313.175092557974));
#122695=CARTESIAN_POINT('Ctrl Pts',(18.7097753803758,1074.65463487909,313.122613565655));
#122696=CARTESIAN_POINT('Ctrl Pts',(18.8530190433782,1074.65148405588,313.123930813235));
#122697=CARTESIAN_POINT('Ctrl Pts',(19.1305877934054,1074.65288064726,313.181347029997));
#122698=CARTESIAN_POINT('Ctrl Pts',(19.2621108319926,1074.65738529076,313.236657969319));
#122699=CARTESIAN_POINT('Ctrl Pts',(19.4971345229847,1074.67346948716,313.394569742299));
#122700=CARTESIAN_POINT('Ctrl Pts',(19.5981458415991,1074.68491825309,313.49580068736));
#122701=CARTESIAN_POINT('Ctrl Pts',(19.7564893702803,1074.71330363923,313.731948520451));
#122702=CARTESIAN_POINT('Ctrl Pts',(19.8118442657399,1074.73001744375,313.86490971987));
#122703=CARTESIAN_POINT('Ctrl Pts',(19.8542934928333,1074.75731680167,314.074892457734));
#122704=CARTESIAN_POINT('Ctrl Pts',(19.861529504772,1074.76676550202,314.146451478113));
#122705=CARTESIAN_POINT('Ctrl Pts',(19.8618518685598,1074.78596641096,314.289763692645));
#122706=CARTESIAN_POINT('Ctrl Pts',(19.8549625708726,1074.79567461623,314.361192331446));
#122707=CARTESIAN_POINT('Ctrl Pts',(19.8130360169185,1074.8250147734,314.574003122828));
#122708=CARTESIAN_POINT('Ctrl Pts',(19.7567052206923,1074.84428996541,314.70965518479));
#122709=CARTESIAN_POINT('Ctrl Pts',(19.5945503301769,1074.87970950716,314.950124265562));
#122710=CARTESIAN_POINT('Ctrl Pts',(19.4906374493414,1074.89553987892,315.052867407687));
#122711=CARTESIAN_POINT('Ctrl Pts',(19.2486324127144,1074.92175013034,315.211672874505));
#122712=CARTESIAN_POINT('Ctrl Pts',(19.1130654563246,1074.93188496957,315.266273233153));
#122713=CARTESIAN_POINT('Ctrl Pts',(18.9048291638458,1074.94155174826,315.305004789759));
#122714=CARTESIAN_POINT('Ctrl Pts',(18.8380754588461,1074.94383253471,315.311164907624));
#122715=CARTESIAN_POINT('Ctrl Pts',(18.7711532049613,1074.94531438668,315.311164930032));
#122716=CARTESIAN_POINT('Origin',(18.7711528398115,1067.7251047501,314.220624181303));
#122717=CARTESIAN_POINT('',(18.7711528398116,1074.86719845859,314.711164930032));
#122718=CARTESIAN_POINT('',(18.771152839812,1074.73625576269,313.730083432575));
#122719=CARTESIAN_POINT('Ctrl Pts',(18.7711528398116,1074.86719845859,314.711164930032));
#122720=CARTESIAN_POINT('Ctrl Pts',(18.7385480853299,1074.86793038454,314.711164930032));
#122721=CARTESIAN_POINT('Ctrl Pts',(18.7059390521038,1074.86823314263,314.70791427713));
#122722=CARTESIAN_POINT('Ctrl Pts',(18.6113554544388,1074.86782827932,314.688765320027));
#122723=CARTESIAN_POINT('Ctrl Pts',(18.5520019098276,1074.86590240622,314.664079613653));
#122724=CARTESIAN_POINT('Ctrl Pts',(18.445809349119,1074.85893388317,314.593285686387));
#122725=CARTESIAN_POINT('Ctrl Pts',(18.4001099060201,1074.8539440585,314.547773970777));
#122726=CARTESIAN_POINT('Ctrl Pts',(18.3278152053011,1074.84137102067,314.440565017267));
#122727=CARTESIAN_POINT('Ctrl Pts',(18.3024956026649,1074.83384807965,314.379547469962));
#122728=CARTESIAN_POINT('Ctrl Pts',(18.283676651615,1074.82157631196,314.284047924447));
#122729=CARTESIAN_POINT('Ctrl Pts',(18.2805795723888,1074.81739646137,314.252114230671));
#122730=CARTESIAN_POINT('Ctrl Pts',(18.2806451986833,1074.80886056661,314.188056780906));
#122731=CARTESIAN_POINT('Ctrl Pts',(18.2838218962225,1074.80452333255,314.156076775462));
#122732=CARTESIAN_POINT('Ctrl Pts',(18.302963549083,1074.791280049,314.060141259098));
#122733=CARTESIAN_POINT('Ctrl Pts',(18.3286834286998,1074.78249115736,313.998837836215));
#122734=CARTESIAN_POINT('Ctrl Pts',(18.4024071876352,1074.76630381678,313.890639135883));
#122735=CARTESIAN_POINT('Ctrl Pts',(18.4494365092931,1074.75904405019,313.844606638804));
#122736=CARTESIAN_POINT('Ctrl Pts',(18.5580244506283,1074.74708388726,313.774167856831));
#122737=CARTESIAN_POINT('Ctrl Pts',(18.6182659084927,1074.74245928634,313.750095322647));
#122738=CARTESIAN_POINT('Ctrl Pts',(18.7110831417207,1074.73800637966,313.732848716439));
#122739=CARTESIAN_POINT('Ctrl Pts',(18.7410768438834,1074.73694555396,313.730083432575));
#122740=CARTESIAN_POINT('Ctrl Pts',(18.7711528398128,1074.73625576269,313.730083432575));
#122741=CARTESIAN_POINT('',(18.7711528398115,1082.7251047501,313.730083432575));
#122742=CARTESIAN_POINT('',(18.7711528398115,1067.7251047501,313.730083432575));
#122743=CARTESIAN_POINT('Origin',(18.7711528398115,1082.7251047501,314.220624181303));
#122744=CARTESIAN_POINT('Ctrl Pts',(18.7711586301647,1074.7362556299,313.730083432609));
#122745=CARTESIAN_POINT('Ctrl Pts',(18.8348430630451,1074.7347951324,313.730084184342));
#122746=CARTESIAN_POINT('Ctrl Pts',(18.8979158494026,1074.73502164797,313.742486465278));
#122747=CARTESIAN_POINT('Ctrl Pts',(19.0158429155388,1074.73882248562,313.790718113182));
#122748=CARTESIAN_POINT('Ctrl Pts',(19.0694925402283,1074.74236107298,313.826079148332));
#122749=CARTESIAN_POINT('Ctrl Pts',(19.1605784364352,1074.7523200418,313.915526407697));
#122750=CARTESIAN_POINT('Ctrl Pts',(19.1969823754605,1074.75866387993,313.968872448428));
#122751=CARTESIAN_POINT('Ctrl Pts',(19.2475053338174,1074.77335681989,314.086903594016));
#122752=CARTESIAN_POINT('Ctrl Pts',(19.2609156300818,1074.78158534014,314.150575152938));
#122753=CARTESIAN_POINT('Ctrl Pts',(19.2620328545287,1074.79446778855,314.247095450945));
#122754=CARTESIAN_POINT('Ctrl Pts',(19.2592433843294,1074.79881998562,314.279199203387));
#122755=CARTESIAN_POINT('Ctrl Pts',(19.2412905284059,1074.81203868588,314.375201128204));
#122756=CARTESIAN_POINT('Ctrl Pts',(19.2164540477036,1074.82077499339,314.436593985981));
#122757=CARTESIAN_POINT('Ctrl Pts',(19.1442117511555,1074.83691514523,314.545771484838));
#122758=CARTESIAN_POINT('Ctrl Pts',(19.0976099832201,1074.84417083407,314.592573906919));
#122759=CARTESIAN_POINT('Ctrl Pts',(18.9887695707287,1074.85622054663,314.665071771415));
#122760=CARTESIAN_POINT('Ctrl Pts',(18.927683439345,1074.86090184323,314.690107358892));
#122761=CARTESIAN_POINT('Ctrl Pts',(18.8329207682236,1074.86542665211,314.708247913804));
#122762=CARTESIAN_POINT('Ctrl Pts',(18.8020387239465,1074.86650511861,314.711164930032));
#122763=CARTESIAN_POINT('Ctrl Pts',(18.7711528398116,1074.86719845859,314.711164930032));
#122764=CARTESIAN_POINT('Origin',(-32.7463814565112,1067.7251047501,341.263474226965));
#122765=CARTESIAN_POINT('',(-32.7463814565318,1076.63168654751,339.785171094771));
#122766=CARTESIAN_POINT('',(-32.7463814565112,1067.7251047501,339.785171094771));
#122767=CARTESIAN_POINT('Ctrl Pts',(-32.7470870485927,1076.70329236998,
342.741777190769));
#122768=CARTESIAN_POINT('Ctrl Pts',(-32.9423914885626,1076.70197251887,
342.741683972214));
#122769=CARTESIAN_POINT('Ctrl Pts',(-33.1357477776511,1076.69996211391,
342.702888100506));
#122770=CARTESIAN_POINT('Ctrl Pts',(-33.4957903882059,1076.69446217964,
342.55256025233));
#122771=CARTESIAN_POINT('Ctrl Pts',(-33.6589997362473,1076.69102122284,
342.44265849417));
#122772=CARTESIAN_POINT('Ctrl Pts',(-33.9343950040687,1076.68278802472,
342.164883295513));
#122773=CARTESIAN_POINT('Ctrl Pts',(-34.0434534885546,1076.67806211271,
341.99934777928));
#122774=CARTESIAN_POINT('Ctrl Pts',(-34.1904010961292,1076.66785445784,
341.635723945508));
#122775=CARTESIAN_POINT('Ctrl Pts',(-34.226969885446,1076.66247571627,341.441290303896));
#122776=CARTESIAN_POINT('Ctrl Pts',(-34.2222006804835,1076.65197963566,
341.051339442137));
#122777=CARTESIAN_POINT('Ctrl Pts',(-34.1816369203232,1076.64696787535,
340.859626242509));
#122778=CARTESIAN_POINT('Ctrl Pts',(-34.0287522855682,1076.63825541818,
340.502836086486));
#122779=CARTESIAN_POINT('Ctrl Pts',(-33.9179210750424,1076.6346464259,340.341220182126));
#122780=CARTESIAN_POINT('Ctrl Pts',(-33.6403510676973,1076.6296453929,340.070263234071));
#122781=CARTESIAN_POINT('Ctrl Pts',(-33.4764013116883,1076.62830318012,
339.96346991672));
#122782=CARTESIAN_POINT('Ctrl Pts',(-33.1170599009339,1076.62821181225,
339.819396893368));
#122783=CARTESIAN_POINT('Ctrl Pts',(-32.925226969539,1076.62945743532,339.783349057752));
#122784=CARTESIAN_POINT('Ctrl Pts',(-32.5388448250334,1076.63426868405,
339.787132334209));
#122785=CARTESIAN_POINT('Ctrl Pts',(-32.3480268118459,1076.63778014823,
339.826825916564));
#122786=CARTESIAN_POINT('Ctrl Pts',(-31.9923956996128,1076.64632548213,
339.977323938767));
#122787=CARTESIAN_POINT('Ctrl Pts',(-31.8310124580455,1076.65127082582,
340.086712346266));
#122788=CARTESIAN_POINT('Ctrl Pts',(-31.5593083828433,1076.66163684506,
340.361472537787));
#122789=CARTESIAN_POINT('Ctrl Pts',(-31.4516537547339,1076.66695266425,
340.524264482069));
#122790=CARTESIAN_POINT('Ctrl Pts',(-31.3039330523849,1076.67717046794,
340.884919591891));
#122791=CARTESIAN_POINT('Ctrl Pts',(-31.2664474452449,1076.68196158429,
341.079721979092));
#122792=CARTESIAN_POINT('Ctrl Pts',(-31.269804627352,1076.69034599917,341.47103163766));
#122793=CARTESIAN_POINT('Ctrl Pts',(-31.3099952016447,1076.69387164049,
341.663677597622));
#122794=CARTESIAN_POINT('Ctrl Pts',(-31.4629309126439,1076.69954362996,
342.0225846597));
#122795=CARTESIAN_POINT('Ctrl Pts',(-31.5742902131587,1076.70164036403,
342.18526696593));
#122796=CARTESIAN_POINT('Ctrl Pts',(-31.8545217810664,1076.70445798862,
342.45866714017));
#122797=CARTESIAN_POINT('Ctrl Pts',(-32.0209035674124,1076.70515030379,
342.566387699169));
#122798=CARTESIAN_POINT('Ctrl Pts',(-32.3765474074373,1076.70516218888,
342.706815634382));
#122799=CARTESIAN_POINT('Ctrl Pts',(-32.5609957573799,1076.70454995941,
342.7418660119));
#122800=CARTESIAN_POINT('Ctrl Pts',(-32.7470870485927,1076.70329236998,
342.741777190769));
#122801=CARTESIAN_POINT('Origin',(-32.7463814565112,1067.7251047501,341.263474226965));
#122802=CARTESIAN_POINT('',(-32.7463814565112,1076.69227114041,342.141777359158));
#122803=CARTESIAN_POINT('',(-32.7463814563977,1076.64970661189,340.385171094772));
#122804=CARTESIAN_POINT('Ctrl Pts',(-32.7463814565112,1076.69227114041,
342.141777359158));
#122805=CARTESIAN_POINT('Ctrl Pts',(-32.7476268445788,1076.69226131304,
342.141777359158));
#122806=CARTESIAN_POINT('Ctrl Pts',(-32.7488723621132,1076.69225142971,
342.141774710315));
#122807=CARTESIAN_POINT('Ctrl Pts',(-32.8667671123006,1076.69131071209,
342.141273148912));
#122808=CARTESIAN_POINT('Ctrl Pts',(-32.9821514820699,1076.68990936895,
342.117543144741));
#122809=CARTESIAN_POINT('Ctrl Pts',(-33.1967235692852,1076.68621385391,
342.026475417372));
#122810=CARTESIAN_POINT('Ctrl Pts',(-33.2938069723275,1076.68395473799,
341.960109667909));
#122811=CARTESIAN_POINT('Ctrl Pts',(-33.45676683502,1076.67874629255,341.793043322698));
#122812=CARTESIAN_POINT('Ctrl Pts',(-33.5208812683237,1076.67584407161,
341.693867602432));
#122813=CARTESIAN_POINT('Ctrl Pts',(-33.6063087830092,1076.66976369463,
341.476752963199));
#122814=CARTESIAN_POINT('Ctrl Pts',(-33.6269735772364,1076.66664714384,
341.361047467887));
#122815=CARTESIAN_POINT('Ctrl Pts',(-33.6220192032145,1076.66069232682,
341.129518889262));
#122816=CARTESIAN_POINT('Ctrl Pts',(-33.5969222871173,1076.65791120844,
341.015949009934));
#122817=CARTESIAN_POINT('Ctrl Pts',(-33.5043246500839,1076.653140776,340.804993273576));
#122818=CARTESIAN_POINT('Ctrl Pts',(-33.4377304794073,1076.65120014331,
340.709648472046));
#122819=CARTESIAN_POINT('Ctrl Pts',(-33.2716177131071,1076.64853964147,
340.550182843906));
#122820=CARTESIAN_POINT('Ctrl Pts',(-33.1737465768415,1076.64784604426,
340.487575726962));
#122821=CARTESIAN_POINT('Ctrl Pts',(-32.9645139181643,1076.64785395915,
340.405656643403));
#122822=CARTESIAN_POINT('Ctrl Pts',(-32.8559011532274,1076.64849047604,
340.385171094743));
#122823=CARTESIAN_POINT('Ctrl Pts',(-32.7463814562842,1076.64970661189,
340.385171094771));
#122824=CARTESIAN_POINT('',(-32.7463814565112,1082.7251047501,340.385171094771));
#122825=CARTESIAN_POINT('',(-32.7463814565112,1067.7251047501,340.385171094771));
#122826=CARTESIAN_POINT('Origin',(-32.7463814565112,1082.7251047501,341.263474226965));
#122827=CARTESIAN_POINT('Ctrl Pts',(-32.7463814562842,1076.64970661189,
340.385171094771));
#122828=CARTESIAN_POINT('Ctrl Pts',(-32.7410877836287,1076.64976539424,
340.385171094773));
#122829=CARTESIAN_POINT('Ctrl Pts',(-32.7357919920265,1076.6498255239,340.385218953388));
#122830=CARTESIAN_POINT('Ctrl Pts',(-32.6156783143586,1076.65121930985,
340.387391924009));
#122831=CARTESIAN_POINT('Ctrl Pts',(-32.5023849415872,1076.65315679928,
340.4119664611));
#122832=CARTESIAN_POINT('Ctrl Pts',(-32.2916472160877,1076.65791509622,
340.50332418109));
#122833=CARTESIAN_POINT('Ctrl Pts',(-32.19624116946,1076.66068784022,340.56924510938));
#122834=CARTESIAN_POINT('Ctrl Pts',(-32.0361639662629,1076.66659587187,
340.734116874935));
#122835=CARTESIAN_POINT('Ctrl Pts',(-31.9730575347923,1076.66967254534,
340.831504332081));
#122836=CARTESIAN_POINT('Ctrl Pts',(-31.890930205726,1076.67545878808,341.037551927229));
#122837=CARTESIAN_POINT('Ctrl Pts',(-31.8698088465635,1076.67813105007,
341.143224669835));
#122838=CARTESIAN_POINT('Ctrl Pts',(-31.8681802914946,1076.68057177695,
341.250091186051));
#122839=CARTESIAN_POINT('Ctrl Pts',(-31.8664057517647,1076.68323129207,
341.366537281396));
#122840=CARTESIAN_POINT('Ctrl Pts',(-31.8878091293091,1076.68556652517,
341.4821886438));
#122841=CARTESIAN_POINT('Ctrl Pts',(-31.9745374154931,1076.68943079159,
341.69852433212));
#122842=CARTESIAN_POINT('Ctrl Pts',(-32.0390473530326,1076.6909235103,341.797040381191));
#122843=CARTESIAN_POINT('Ctrl Pts',(-32.2030559898266,1076.69297894973,
341.96340568665));
#122844=CARTESIAN_POINT('Ctrl Pts',(-32.3010287740737,1076.69352027147,
342.029482453987));
#122845=CARTESIAN_POINT('Ctrl Pts',(-32.5159752164315,1076.69361847209,
342.118890353154));
#122846=CARTESIAN_POINT('Ctrl Pts',(-32.6306190082936,1076.69318462243,
342.141777359158));
#122847=CARTESIAN_POINT('Ctrl Pts',(-32.7463814565112,1076.69227114041,
342.141777359158));
#122848=CARTESIAN_POINT('Origin',(-25.1979747106603,1067.7251047501,331.226959282729));
#122849=CARTESIAN_POINT('',(-25.1979747106792,1076.26166943286,329.951515161593));
#122850=CARTESIAN_POINT('',(-25.1979747106603,1067.7251047501,329.951515161593));
#122851=CARTESIAN_POINT('Ctrl Pts',(-25.1980032377211,1076.42086980393,
332.502403403546));
#122852=CARTESIAN_POINT('Ctrl Pts',(-25.36705969148,1076.41826882087,332.502399622366));
#122853=CARTESIAN_POINT('Ctrl Pts',(-25.5343921697909,1076.41376902618,
332.468784797302));
#122854=CARTESIAN_POINT('Ctrl Pts',(-25.8458881365049,1076.40132876238,
332.338455592051));
#122855=CARTESIAN_POINT('Ctrl Pts',(-25.9869961492942,1076.39351219026,
332.243138053092));
#122856=CARTESIAN_POINT('Ctrl Pts',(-26.2245078606825,1076.37532289726,
332.002649118291));
#122857=CARTESIAN_POINT('Ctrl Pts',(-26.3183251064285,1076.3651134342,331.859611292541));
#122858=CARTESIAN_POINT('Ctrl Pts',(-26.4129107652612,1076.34898533397,
331.624205262477));
#122859=CARTESIAN_POINT('Ctrl Pts',(-26.4365172614667,1076.34352500537,
331.543005334542));
#122860=CARTESIAN_POINT('Ctrl Pts',(-26.4825679162042,1076.32716353809,
331.295293385328));
#122861=CARTESIAN_POINT('Ctrl Pts',(-26.4804270245162,1076.31636411902,
331.126052751354));
#122862=CARTESIAN_POINT('Ctrl Pts',(-26.4108043557608,1076.29629617508,
330.798150060569));
#122863=CARTESIAN_POINT('Ctrl Pts',(-26.3440301995677,1076.28722377961,
330.64263696166));
#122864=CARTESIAN_POINT('Ctrl Pts',(-26.1542812502165,1076.27226345453,
330.366600016229));
#122865=CARTESIAN_POINT('Ctrl Pts',(-26.0332861584661,1076.26651779982,
330.248677000342));
#122866=CARTESIAN_POINT('Ctrl Pts',(-25.7530239795191,1076.25932675635,
330.0665671552));
#122867=CARTESIAN_POINT('Ctrl Pts',(-25.5966355803637,1076.25793970918,
330.003983116595));
#122868=CARTESIAN_POINT('Ctrl Pts',(-25.2689795137375,1076.25977446275,
329.942657018773));
#122869=CARTESIAN_POINT('Ctrl Pts',(-25.1009567331692,1076.26296704667,
329.944369712011));
#122870=CARTESIAN_POINT('Ctrl Pts',(-24.7750493429435,1076.27343781723,
330.012212322424));
#122871=CARTESIAN_POINT('Ctrl Pts',(-24.6203360176324,1076.2806128095,330.07771394198));
#122872=CARTESIAN_POINT('Ctrl Pts',(-24.3445146671539,1076.29784880489,
330.264573161085));
#122873=CARTESIAN_POINT('Ctrl Pts',(-24.2261483303946,1076.30774747809,
330.384284884773));
#122874=CARTESIAN_POINT('Ctrl Pts',(-24.0881316782512,1076.32352699544,
330.592944913446));
#122875=CARTESIAN_POINT('Ctrl Pts',(-24.049028858082,1076.32890941553,330.666916761111));
#122876=CARTESIAN_POINT('Ctrl Pts',(-23.9858266572107,1076.33974392426,
330.821462373265));
#122877=CARTESIAN_POINT('Ctrl Pts',(-23.9618841178172,1076.34517029959,
330.901672657433));
#122878=CARTESIAN_POINT('Ctrl Pts',(-23.9136159982493,1076.36139485872,
331.150048110655));
#122879=CARTESIAN_POINT('Ctrl Pts',(-23.9147658066077,1076.37180532051,
331.321279810547));
#122880=CARTESIAN_POINT('Ctrl Pts',(-23.9837983035842,1076.39053694666,
331.652348720763));
#122881=CARTESIAN_POINT('Ctrl Pts',(-24.0506083409084,1076.39869042679,
331.80900113857));
#122882=CARTESIAN_POINT('Ctrl Pts',(-24.2415044822947,1076.4118984853,332.087450762062));
#122883=CARTESIAN_POINT('Ctrl Pts',(-24.363752916489,1076.41682377266,332.206442664842));
#122884=CARTESIAN_POINT('Ctrl Pts',(-24.6479982924025,1076.42293360066,
332.39014394625));
#122885=CARTESIAN_POINT('Ctrl Pts',(-24.8072436045823,1076.42404946741,
332.452850820141));
#122886=CARTESIAN_POINT('Ctrl Pts',(-25.0480040306134,1076.42279725656,
332.495778924567));
#122887=CARTESIAN_POINT('Ctrl Pts',(-25.1229325560726,1076.42202478836,
332.502405082605));
#122888=CARTESIAN_POINT('Ctrl Pts',(-25.1980032377211,1076.42086980393,
332.502403403546));
#122889=CARTESIAN_POINT('Origin',(-25.1979747106603,1067.7251047501,331.226959282729));
#122890=CARTESIAN_POINT('',(-25.1979747106603,1076.38624898044,331.902403403865));
#122891=CARTESIAN_POINT('',(-25.1979747106602,1076.3019258569,330.551515161593));
#122892=CARTESIAN_POINT('Ctrl Pts',(-25.1979747106603,1076.38624898044,
331.902403403865));
#122893=CARTESIAN_POINT('Ctrl Pts',(-25.2471812358611,1076.38545783245,
331.902403403865));
#122894=CARTESIAN_POINT('Ctrl Pts',(-25.2963568705416,1076.38434577168,
331.897026203571));
#122895=CARTESIAN_POINT('Ctrl Pts',(-25.4323214908925,1076.3803418051,331.866786924668));
#122896=CARTESIAN_POINT('Ctrl Pts',(-25.5152270241464,1076.37679013501,
331.82998264202));
#122897=CARTESIAN_POINT('Ctrl Pts',(-25.6618430249056,1076.36810176254,
331.726092728421));
#122898=CARTESIAN_POINT('Ctrl Pts',(-25.7240629546574,1076.36304832444,
331.660004822544));
#122899=CARTESIAN_POINT('Ctrl Pts',(-25.7947649861978,1076.35487229256,
331.546338881351));
#122900=CARTESIAN_POINT('Ctrl Pts',(-25.8143011508075,1076.35209936297,
331.506785957527));
#122901=CARTESIAN_POINT('Ctrl Pts',(-25.8454405672376,1076.34645311229,
331.424341249773));
#122902=CARTESIAN_POINT('Ctrl Pts',(-25.8569487026477,1076.34359288809,
331.381635759692));
#122903=CARTESIAN_POINT('Ctrl Pts',(-25.8789581544592,1076.33494671822,
331.249717581615));
#122904=CARTESIAN_POINT('Ctrl Pts',(-25.875969789591,1076.32926836339,331.159245492184));
#122905=CARTESIAN_POINT('Ctrl Pts',(-25.8350622871002,1076.31890066796,
330.985710803517));
#122906=CARTESIAN_POINT('Ctrl Pts',(-25.7979324441916,1076.31430177259,
330.904245617303));
#122907=CARTESIAN_POINT('Ctrl Pts',(-25.6943862091979,1076.30681073806,
330.760449535376));
#122908=CARTESIAN_POINT('Ctrl Pts',(-25.6290457199438,1076.30398861186,
330.699470787555));
#122909=CARTESIAN_POINT('Ctrl Pts',(-25.4787036906503,1076.30056020518,
330.606301500901));
#122910=CARTESIAN_POINT('Ctrl Pts',(-25.3952258217971,1076.29998235526,
330.574947530313));
#122911=CARTESIAN_POINT('Ctrl Pts',(-25.2716845042923,1076.30082579969,
330.554536759418));
#122912=CARTESIAN_POINT('Ctrl Pts',(-25.2348649592348,1076.3012770248,330.551515771758));
#122913=CARTESIAN_POINT('Ctrl Pts',(-25.1979858830973,1076.30192566039,
330.551515161756));
#122914=CARTESIAN_POINT('Ctrl Pts',(-25.1979821589501,1076.30192572589,
330.551515161694));
#122915=CARTESIAN_POINT('Ctrl Pts',(-25.1979784348043,1076.30192579139,
330.551515161593));
#122916=CARTESIAN_POINT('Ctrl Pts',(-25.1979747106602,1076.3019258569,330.551515161593));
#122917=CARTESIAN_POINT('',(-25.1979747106603,1082.7251047501,330.551515161593));
#122918=CARTESIAN_POINT('',(-25.1979747106603,1067.7251047501,330.551515161593));
#122919=CARTESIAN_POINT('Origin',(-25.1979747106603,1082.7251047501,331.226959282729));
#122920=CARTESIAN_POINT('Ctrl Pts',(-25.1979747106602,1076.3019258569,330.551515161593));
#122921=CARTESIAN_POINT('Ctrl Pts',(-25.109754694076,1076.30347758071,330.551515161593));
#122922=CARTESIAN_POINT('Ctrl Pts',(-25.0224144977182,1076.30613837089,
330.568798147374));
#122923=CARTESIAN_POINT('Ctrl Pts',(-24.8592059024046,1076.31333459836,
330.635974818503));
#122924=CARTESIAN_POINT('Ctrl Pts',(-24.784940815646,1076.31780258741,330.685278616937));
#122925=CARTESIAN_POINT('Ctrl Pts',(-24.6594569177532,1076.32791710315,
330.809761185901));
#122926=CARTESIAN_POINT('Ctrl Pts',(-24.609502878529,1076.33346843719,330.88381207894));
#122927=CARTESIAN_POINT('Ctrl Pts',(-24.5581135217446,1076.34202464141,
331.006144925782));
#122928=CARTESIAN_POINT('Ctrl Pts',(-24.5450295698096,1076.34489499932,
331.048510411215));
#122929=CARTESIAN_POINT('Ctrl Pts',(-24.5181676135318,1076.35353733772,
331.180085689814));
#122930=CARTESIAN_POINT('Ctrl Pts',(-24.5179767652101,1076.35914812453,
331.271059263526));
#122931=CARTESIAN_POINT('Ctrl Pts',(-24.5532474129041,1076.36934944255,
331.447438544772));
#122932=CARTESIAN_POINT('Ctrl Pts',(-24.5882335394392,1076.37384368879,
331.531117263122));
#122933=CARTESIAN_POINT('Ctrl Pts',(-24.6889438876951,1076.38116825472,
331.679932907919));
#122934=CARTESIAN_POINT('Ctrl Pts',(-24.7536613715196,1076.3839264696,331.743576301247));
#122935=CARTESIAN_POINT('Ctrl Pts',(-24.9043545433581,1076.38736353833,
331.841869194931));
#122936=CARTESIAN_POINT('Ctrl Pts',(-24.9888282224768,1076.3880059005,331.875486363782));
#122937=CARTESIAN_POINT('Ctrl Pts',(-25.1172929206417,1076.38733026166,
331.898791292979));
#122938=CARTESIAN_POINT('Ctrl Pts',(-25.1576441914772,1076.38689741901,
331.902403403865));
#122939=CARTESIAN_POINT('Ctrl Pts',(-25.1979747106603,1076.38624898044,
331.902403403865));
#122940=CARTESIAN_POINT('Origin',(-15.9013061211259,1067.7251047501,320.960985878213));
#122941=CARTESIAN_POINT('',(-15.901306121144,1075.53973422622,319.862154742221));
#122942=CARTESIAN_POINT('',(-15.9013061211259,1067.7251047501,319.862154742221));
#122943=CARTESIAN_POINT('Ctrl Pts',(-15.9013183816517,1075.76586210742,
322.059817014137));
#122944=CARTESIAN_POINT('Ctrl Pts',(-16.0472269922218,1075.76364690165,
322.05981538612));
#122945=CARTESIAN_POINT('Ctrl Pts',(-16.1915897472063,1075.75858015459,
322.030753759462));
#122946=CARTESIAN_POINT('Ctrl Pts',(-16.4604451299536,1075.74326344712,
321.918087664903));
#122947=CARTESIAN_POINT('Ctrl Pts',(-16.58220670375,1075.73316467281,321.835613218183));
#122948=CARTESIAN_POINT('Ctrl Pts',(-16.7868653598449,1075.70909583708,
321.627761662381));
#122949=CARTESIAN_POINT('Ctrl Pts',(-16.8675413122869,1075.69534327377,
321.504242453182));
#122950=CARTESIAN_POINT('Ctrl Pts',(-16.9482963891639,1075.67345610172,
321.302129034095));
#122951=CARTESIAN_POINT('Ctrl Pts',(-16.9683097655656,1075.66607632406,
321.233138440417));
#122952=CARTESIAN_POINT('Ctrl Pts',(-16.9948448527741,1075.65105120479,
321.091049237343));
#122953=CARTESIAN_POINT('Ctrl Pts',(-17.0010635249007,1075.64343914419,
321.018237504974));
#122954=CARTESIAN_POINT('Ctrl Pts',(-16.9979651957292,1075.62094467287,
320.800574562154));
#122955=CARTESIAN_POINT('Ctrl Pts',(-16.9673098121961,1075.60650474725,
320.657538248775));
#122956=CARTESIAN_POINT('Ctrl Pts',(-16.852353782415,1075.58047494831,320.391952227302));
#122957=CARTESIAN_POINT('Ctrl Pts',(-16.7693475035747,1075.56912651833,
320.271870856426));
#122958=CARTESIAN_POINT('Ctrl Pts',(-16.5619837108859,1075.55122442585,
320.071259986371));
#122959=CARTESIAN_POINT('Ctrl Pts',(-16.439927446826,1075.54481883454,319.992451446599));
#122960=CARTESIAN_POINT('Ctrl Pts',(-16.1728997908162,1075.5379049811,319.886661577952));
#122961=CARTESIAN_POINT('Ctrl Pts',(-16.0307255945619,1075.53743358193,
319.860444336545));
#122962=CARTESIAN_POINT('Ctrl Pts',(-15.7445118197114,1075.54250111157,
319.864035640628));
#122963=CARTESIAN_POINT('Ctrl Pts',(-15.6033283901581,1075.54798015182,
319.893728990274));
#122964=CARTESIAN_POINT('Ctrl Pts',(-15.3398915156939,1075.56414806262,
320.00558002081));
#122965=CARTESIAN_POINT('Ctrl Pts',(-15.2202951230251,1075.57469598467,
320.086841748472));
#122966=CARTESIAN_POINT('Ctrl Pts',(-15.018490373626,1075.59943336025,320.291055452454));
#122967=CARTESIAN_POINT('Ctrl Pts',(-14.9384574793007,1075.6134067287,320.412320353851));
#122968=CARTESIAN_POINT('Ctrl Pts',(-14.8567867324523,1075.63546720063,
320.612251183191));
#122969=CARTESIAN_POINT('Ctrl Pts',(-14.8361484273098,1075.64296696986,
320.681569384525));
#122970=CARTESIAN_POINT('Ctrl Pts',(-14.8087834485469,1075.6579890958,320.823107614848));
#122971=CARTESIAN_POINT('Ctrl Pts',(-14.802095746972,1075.66547659229,320.894994585311));
#122972=CARTESIAN_POINT('Ctrl Pts',(-14.8032947200149,1075.687779544,321.113173425508));
#122973=CARTESIAN_POINT('Ctrl Pts',(-14.8332484575461,1075.7019896304,321.257806786604));
#122974=CARTESIAN_POINT('Ctrl Pts',(-14.9478420172994,1075.72728452876,
321.526238004055));
#122975=CARTESIAN_POINT('Ctrl Pts',(-15.031047423577,1075.73814208654,321.647525124861));
#122976=CARTESIAN_POINT('Ctrl Pts',(-15.2400991870558,1075.75518944082,
321.850623175349));
#122977=CARTESIAN_POINT('Ctrl Pts',(-15.3638024185795,1075.76121419415,
321.930417864329));
#122978=CARTESIAN_POINT('Ctrl Pts',(-15.6275412594093,1075.76746576582,
322.034011522529));
#122979=CARTESIAN_POINT('Ctrl Pts',(-15.7638192353197,1075.76794963948,
322.059818548324));
#122980=CARTESIAN_POINT('Ctrl Pts',(-15.9013183816517,1075.76586210742,
322.059817014137));
#122981=CARTESIAN_POINT('Origin',(-15.9013061211259,1067.7251047501,320.960985878213));
#122982=CARTESIAN_POINT('',(-15.9013061211259,1075.70629239322,321.459817014206));
#122983=CARTESIAN_POINT('',(-15.9013061211256,1075.60362949862,320.462154742221));
#122984=CARTESIAN_POINT('Ctrl Pts',(-15.9013061211259,1075.70629239322,
321.459817014206));
#122985=CARTESIAN_POINT('Ctrl Pts',(-15.9027535012539,1075.70626993847,
321.459817014206));
#122986=CARTESIAN_POINT('Ctrl Pts',(-15.9042011776659,1075.70624684176,
321.459810714755));
#122987=CARTESIAN_POINT('Ctrl Pts',(-15.9707105043603,1075.70515642044,
321.459231640583));
#122988=CARTESIAN_POINT('Ctrl Pts',(-16.0349930669914,1075.70281517994,
321.445942636561));
#122989=CARTESIAN_POINT('Ctrl Pts',(-16.156182577991,1075.69575713627,321.394914764689));
#122990=CARTESIAN_POINT('Ctrl Pts',(-16.2116400238405,1075.69105759309,
321.35713204646));
#122991=CARTESIAN_POINT('Ctrl Pts',(-16.304622580305,1075.6799136683,321.262000551855));
#122992=CARTESIAN_POINT('Ctrl Pts',(-16.3411480830573,1075.67357315667,
321.205525304293));
#122993=CARTESIAN_POINT('Ctrl Pts',(-16.3774474234298,1075.6635429136,321.113253709203));
#122994=CARTESIAN_POINT('Ctrl Pts',(-16.3863796690735,1075.66017364307,
321.081812503107));
#122995=CARTESIAN_POINT('Ctrl Pts',(-16.3979926987541,1075.6533829733,321.017577036737));
#122996=CARTESIAN_POINT('Ctrl Pts',(-16.4006327713848,1075.64997719005,
320.984928600088));
#122997=CARTESIAN_POINT('Ctrl Pts',(-16.3989004958387,1075.63979069932,
320.885965480553));
#122998=CARTESIAN_POINT('Ctrl Pts',(-16.3845348923151,1075.63324025375,
320.820523772531));
#122999=CARTESIAN_POINT('Ctrl Pts',(-16.3313385075833,1075.62155424489,
320.699845122897));
#123000=CARTESIAN_POINT('Ctrl Pts',(-16.2933462146483,1075.61651332255,
320.645638342996));
#123001=CARTESIAN_POINT('Ctrl Pts',(-16.198733867935,1075.60859541564,320.555247933136));
#123002=CARTESIAN_POINT('Ctrl Pts',(-16.1431566091223,1075.60578355299,
320.519842299189));
#123003=CARTESIAN_POINT('Ctrl Pts',(-16.024595193168,1075.60285688101,320.473681964203));
#123004=CARTESIAN_POINT('Ctrl Pts',(-15.9632237991125,1075.6026355528,320.462154742221));
#123005=CARTESIAN_POINT('Ctrl Pts',(-15.9013061211248,1075.60362949862,
320.462154742221));
#123006=CARTESIAN_POINT('',(-15.9013061211259,1082.7251047501,320.462154742221));
#123007=CARTESIAN_POINT('',(-15.9013061211259,1067.7251047501,320.462154742221));
#123008=CARTESIAN_POINT('Origin',(-15.9013061211259,1082.7251047501,320.960985878213));
#123009=CARTESIAN_POINT('Ctrl Pts',(-15.9013021674381,1075.60362956209,
320.462154742237));
#123010=CARTESIAN_POINT('Ctrl Pts',(-15.8363273247354,1075.60467263752,
320.462155257221));
#123011=CARTESIAN_POINT('Ctrl Pts',(-15.7720200532064,1075.60703351656,
320.474849655884));
#123012=CARTESIAN_POINT('Ctrl Pts',(-15.6517121538532,1075.61411388871,
320.524202822739));
#123013=CARTESIAN_POINT('Ctrl Pts',(-15.5969274629695,1075.61877242025,
320.560469438888));
#123014=CARTESIAN_POINT('Ctrl Pts',(-15.5041480528897,1075.62978368196,
320.652153043733));
#123015=CARTESIAN_POINT('Ctrl Pts',(-15.46714933412,1075.63604037615,320.706806078424));
#123016=CARTESIAN_POINT('Ctrl Pts',(-15.429011929669,1075.64598127082,320.797148681718));
#123017=CARTESIAN_POINT('Ctrl Pts',(-15.4192811049715,1075.64936875669,
320.828487821771));
#123018=CARTESIAN_POINT('Ctrl Pts',(-15.4061097386104,1075.65617680393,
320.892565172555));
#123019=CARTESIAN_POINT('Ctrl Pts',(-15.4026908943796,1075.65958154805,
320.925153009441));
#123020=CARTESIAN_POINT('Ctrl Pts',(-15.4020652237601,1075.66978294967,
321.024436226829));
#123021=CARTESIAN_POINT('Ctrl Pts',(-15.4149851501882,1075.67633558523,
321.090488908085));
#123022=CARTESIAN_POINT('Ctrl Pts',(-15.4659668956417,1075.68807447895,
321.213415530183));
#123023=CARTESIAN_POINT('Ctrl Pts',(-15.503419072807,1075.69315134413,321.269116239206));
#123024=CARTESIAN_POINT('Ctrl Pts',(-15.5979744807591,1075.7011562374,321.362519086056));
#123025=CARTESIAN_POINT('Ctrl Pts',(-15.6540756517758,1075.70400819849,
321.39931121727));
#123026=CARTESIAN_POINT('Ctrl Pts',(-15.7747893415874,1075.70702747658,
321.447674869886));
#123027=CARTESIAN_POINT('Ctrl Pts',(-15.8377621891094,1075.70727821804,
321.459817014206));
#123028=CARTESIAN_POINT('Ctrl Pts',(-15.9013061211259,1075.70629239322,
321.459817014206));
#123029=CARTESIAN_POINT('Origin',(-4.59241321360898,1067.7251047501,312.73037859586));
#123030=CARTESIAN_POINT('',(-4.5924132136256,1074.6522152412,311.639837847132));
#123031=CARTESIAN_POINT('',(-4.59241321360898,1067.7251047501,311.639837847132));
#123032=CARTESIAN_POINT('Ctrl Pts',(-4.59242154314923,1074.94723110711,
313.820919344557));
#123033=CARTESIAN_POINT('Ctrl Pts',(-4.73417441665283,1074.94646331085,
313.82091826185));
#123034=CARTESIAN_POINT('Ctrl Pts',(-4.87446768389953,1074.94206003125,
313.793280638671));
#123035=CARTESIAN_POINT('Ctrl Pts',(-5.13950864065852,1074.9262762585,313.684810857126));
#123036=CARTESIAN_POINT('Ctrl Pts',(-5.2610613528356,1074.91489969795,313.60389685957));
#123037=CARTESIAN_POINT('Ctrl Pts',(-5.46586598942681,1074.88655943134,
313.399274617924));
#123038=CARTESIAN_POINT('Ctrl Pts',(-5.54686784141405,1074.86984878477,
313.277399654976));
#123039=CARTESIAN_POINT('Ctrl Pts',(-5.62860101239182,1074.84260840697,
313.077717779237));
#123040=CARTESIAN_POINT('Ctrl Pts',(-5.64901645007429,1074.83332330149,
313.009502701119));
#123041=CARTESIAN_POINT('Ctrl Pts',(-5.67635023549569,1074.81434541568,
312.869828260613));
#123042=CARTESIAN_POINT('Ctrl Pts',(-5.68314655426807,1074.80469370511,
312.798670210033));
#123043=CARTESIAN_POINT('Ctrl Pts',(-5.68254464419452,1074.77515502237,
312.580535231193));
#123044=CARTESIAN_POINT('Ctrl Pts',(-5.65248779637873,1074.75553601166,
312.435175883673));
#123045=CARTESIAN_POINT('Ctrl Pts',(-5.53774437308449,1074.71965851928,
312.167982761174));
#123046=CARTESIAN_POINT('Ctrl Pts',(-5.45537699260935,1074.70367302368,
312.048200548254));
#123047=CARTESIAN_POINT('Ctrl Pts',(-5.24943671602821,1074.6773203616,311.848345273121));
#123048=CARTESIAN_POINT('Ctrl Pts',(-5.12828913258207,1074.66715917283,
311.769845770818));
#123049=CARTESIAN_POINT('Ctrl Pts',(-4.86342142412553,1074.65410276184,
311.664570774242));
#123050=CARTESIAN_POINT('Ctrl Pts',(-4.72260569605938,1074.65127210857,
311.6383706536));
#123051=CARTESIAN_POINT('Ctrl Pts',(-4.43921361249575,1074.65330593362,
311.641426329821));
#123052=CARTESIAN_POINT('Ctrl Pts',(-4.29953671467465,1074.65812173189,
311.670451496656));
#123053=CARTESIAN_POINT('Ctrl Pts',(-4.03859143543839,1074.67477760158,
311.7802760977));
#123054=CARTESIAN_POINT('Ctrl Pts',(-3.920026596784,1074.68648206998,311.860217895112));
#123055=CARTESIAN_POINT('Ctrl Pts',(-3.71928348622794,1074.71529000323,
312.06154683786));
#123056=CARTESIAN_POINT('Ctrl Pts',(-3.63941913700345,1074.7321666632,312.181401833915));
#123057=CARTESIAN_POINT('Ctrl Pts',(-3.5574261244455,1074.75962418542,312.379331949081));
#123058=CARTESIAN_POINT('Ctrl Pts',(-3.53657934187177,1074.76911108084,
312.448175008495));
#123059=CARTESIAN_POINT('Ctrl Pts',(-3.50871996467179,1074.78836976263,
312.588860340566));
#123060=CARTESIAN_POINT('Ctrl Pts',(-3.50176299797697,1074.79809774018,
312.660382283191));
#123061=CARTESIAN_POINT('Ctrl Pts',(-3.50209860283686,1074.82744712561,
312.877561022191));
#123062=CARTESIAN_POINT('Ctrl Pts',(-3.53143919505767,1074.84666254094,
313.021677024456));
#123063=CARTESIAN_POINT('Ctrl Pts',(-3.64469868835762,1074.88182214959,
313.288955618368));
#123064=CARTESIAN_POINT('Ctrl Pts',(-3.72708461848955,1074.89745764829,
313.409725430513));
#123065=CARTESIAN_POINT('Ctrl Pts',(-3.93424897340151,1074.92317009665,
313.611828490723));
#123066=CARTESIAN_POINT('Ctrl Pts',(-4.05677723349741,1074.93301348281,
313.691288427238));
#123067=CARTESIAN_POINT('Ctrl Pts',(-4.31905539402455,1074.94529213272,
313.79498192967));
#123068=CARTESIAN_POINT('Ctrl Pts',(-4.45509219391934,1074.9479749436,313.820920393477));
#123069=CARTESIAN_POINT('Ctrl Pts',(-4.59242154314923,1074.94723110711,
313.820919344557));
#123070=CARTESIAN_POINT('Origin',(-4.59241321360898,1067.7251047501,312.73037859586));
#123071=CARTESIAN_POINT('',(-4.59241321360898,1074.8680726283,313.220919344589));
#123072=CARTESIAN_POINT('',(-4.59241321360906,1074.73536251872,312.239837847132));
#123073=CARTESIAN_POINT('Ctrl Pts',(-4.59241321360898,1074.8680726283,313.220919344589));
#123074=CARTESIAN_POINT('Ctrl Pts',(-4.59343259811277,1074.86806703061,
313.220919344589));
#123075=CARTESIAN_POINT('Ctrl Pts',(-4.59445214105991,1074.86806100691,
313.220916167041));
#123076=CARTESIAN_POINT('Ctrl Pts',(-4.65919666386597,1074.86765146619,
313.220512464842));
#123077=CARTESIAN_POINT('Ctrl Pts',(-4.72218589708467,1074.86559231559,
313.207702474031));
#123078=CARTESIAN_POINT('Ctrl Pts',(-4.84000296423593,1074.85837634849,
313.158658728959));
#123079=CARTESIAN_POINT('Ctrl Pts',(-4.89359922392605,1074.85327469048,
313.122789291614));
#123080=CARTESIAN_POINT('Ctrl Pts',(-4.98520338088352,1074.84050617101,
313.031452684482));
#123081=CARTESIAN_POINT('Ctrl Pts',(-5.02181171024764,1074.83290009585,
312.976388746648));
#123082=CARTESIAN_POINT('Ctrl Pts',(-5.05865719923982,1074.82053899349,
312.886182966118));
#123083=CARTESIAN_POINT('Ctrl Pts',(-5.06783727646721,1074.8163344332,312.855393246639));
#123084=CARTESIAN_POINT('Ctrl Pts',(-5.08007526073578,1074.80776045823,
312.792409544954));
#123085=CARTESIAN_POINT('Ctrl Pts',(-5.08308941819944,1074.80340996283,
312.760354062892));
#123086=CARTESIAN_POINT('Ctrl Pts',(-5.08266187334577,1074.79015019368,
312.66236355755));
#123087=CARTESIAN_POINT('Ctrl Pts',(-5.06910752841617,1074.78138135226,
312.597165597613));
#123088=CARTESIAN_POINT('Ctrl Pts',(-5.01733907562667,1074.76531240295,
312.47680634019));
#123089=CARTESIAN_POINT('Ctrl Pts',(-4.97996812233148,1074.75814666573,
312.422662009554));
#123090=CARTESIAN_POINT('Ctrl Pts',(-4.88683250062607,1074.74641467959,
312.332805671349));
#123091=CARTESIAN_POINT('Ctrl Pts',(-4.83229404821456,1074.74192219264,
312.297679426263));
#123092=CARTESIAN_POINT('Ctrl Pts',(-4.71513682801718,1074.73626345487,
312.251460229922));
#123093=CARTESIAN_POINT('Ctrl Pts',(-4.6540664253156,1074.73501655744,312.239838061364));
#123094=CARTESIAN_POINT('Ctrl Pts',(-4.59241491815632,1074.73536250915,
312.239837847135));
#123095=CARTESIAN_POINT('',(-4.59241321360898,1082.7251047501,312.239837847132));
#123096=CARTESIAN_POINT('',(-4.59241321360898,1067.7251047501,312.239837847132));
#123097=CARTESIAN_POINT('Origin',(-4.59241321360898,1082.7251047501,312.73037859586));
#123098=CARTESIAN_POINT('Ctrl Pts',(-4.59241321360922,1074.73536251872,
312.239837847132));
#123099=CARTESIAN_POINT('Ctrl Pts',(-4.52875064557946,1074.73571978555,
312.239837847132));
#123100=CARTESIAN_POINT('Ctrl Pts',(-4.46574735051964,1074.73776821706,
312.252229509161));
#123101=CARTESIAN_POINT('Ctrl Pts',(-4.34776850179519,1074.7450132071,312.300425563072));
#123102=CARTESIAN_POINT('Ctrl Pts',(-4.29401920231488,1074.75015182552,
312.335858802838));
#123103=CARTESIAN_POINT('Ctrl Pts',(-4.20273370102847,1074.76288605867,
312.425558610257));
#123104=CARTESIAN_POINT('Ctrl Pts',(-4.16624547770014,1074.77038146574,
312.479137556319));
#123105=CARTESIAN_POINT('Ctrl Pts',(-4.128484121288,1074.78262864972,312.56777786159));
#123106=CARTESIAN_POINT('Ctrl Pts',(-4.11881011052542,1074.78686288898,
312.598592580366));
#123107=CARTESIAN_POINT('Ctrl Pts',(-4.10564643941886,1074.79547983249,
312.661638793863));
#123108=CARTESIAN_POINT('Ctrl Pts',(-4.10218535791044,1074.79984300773,
312.693727376496));
#123109=CARTESIAN_POINT('Ctrl Pts',(-4.10129632511921,1074.81307368021,
312.791531019133));
#123110=CARTESIAN_POINT('Ctrl Pts',(-4.11386954858357,1074.82178992049,
312.856651742813));
#123111=CARTESIAN_POINT('Ctrl Pts',(-4.16383161852702,1074.83782658645,
312.977796257153));
#123112=CARTESIAN_POINT('Ctrl Pts',(-4.20059282629724,1074.84500106704,
313.032706154599));
#123113=CARTESIAN_POINT('Ctrl Pts',(-4.29347628013839,1074.85683857716,
313.124739868));
#123114=CARTESIAN_POINT('Ctrl Pts',(-4.34856892267024,1074.86139424134,
313.161016716072));
#123115=CARTESIAN_POINT('Ctrl Pts',(-4.4674544550444,1074.86714703548,313.208867730578));
#123116=CARTESIAN_POINT('Ctrl Pts',(-4.52963335727786,1074.86841736828,
313.220919344589));
#123117=CARTESIAN_POINT('Ctrl Pts',(-4.59241321360898,1074.8680726283,313.220919344589));
#123118=CARTESIAN_POINT('Origin',(-49.3616411037539,1067.7251047501,349.893375147338));
#123119=CARTESIAN_POINT('',(-49.3616411037758,1076.63637248492,348.415072015145));
#123120=CARTESIAN_POINT('',(-49.3616411037539,1067.7251047501,348.415072015145));
#123121=CARTESIAN_POINT('Ctrl Pts',(-49.3624372582816,1076.70060106622,
351.371678065143));
#123122=CARTESIAN_POINT('Ctrl Pts',(-49.5573261371424,1076.6985286974,351.371573105827));
#123123=CARTESIAN_POINT('Ctrl Pts',(-49.7502737386378,1076.69575821467,
351.332930288383));
#123124=CARTESIAN_POINT('Ctrl Pts',(-50.1107340574847,1076.68876623073,
351.182757831355));
#123125=CARTESIAN_POINT('Ctrl Pts',(-50.2745829485658,1076.68460066891,
351.072432238936));
#123126=CARTESIAN_POINT('Ctrl Pts',(-50.5500125666934,1076.67517733427,
350.794222637883));
#123127=CARTESIAN_POINT('Ctrl Pts',(-50.6587901775009,1076.67000872495,
350.629005017809));
#123128=CARTESIAN_POINT('Ctrl Pts',(-50.8049247452241,1076.65943419735,
350.267498610164));
#123129=CARTESIAN_POINT('Ctrl Pts',(-50.8415216207758,1076.65413721465,
350.075015038867));
#123130=CARTESIAN_POINT('Ctrl Pts',(-50.838261778393,1076.64432889098,349.686809038781));
#123131=CARTESIAN_POINT('Ctrl Pts',(-50.7983972091676,1076.63992013039,
349.494851033114));
#123132=CARTESIAN_POINT('Ctrl Pts',(-50.6468018068872,1076.63293865188,
349.137477534985));
#123133=CARTESIAN_POINT('Ctrl Pts',(-50.5366114824806,1076.63043852341,
348.975511260837));
#123134=CARTESIAN_POINT('Ctrl Pts',(-50.2602807225132,1076.62793377259,
348.703713849592));
#123135=CARTESIAN_POINT('Ctrl Pts',(-50.0969595379003,1076.62794991829,
348.596396391019));
#123136=CARTESIAN_POINT('Ctrl Pts',(-49.7386548966553,1076.63050995024,
348.450967511084));
#123137=CARTESIAN_POINT('Ctrl Pts',(-49.5472065995713,1076.63302082595,
348.414106937213));
#123138=CARTESIAN_POINT('Ctrl Pts',(-49.1610999938002,1076.63999363883,
348.416075018567));
#123139=CARTESIAN_POINT('Ctrl Pts',(-48.970157576568,1076.64438124009,348.454847472195));
#123140=CARTESIAN_POINT('Ctrl Pts',(-48.6138111271898,1076.65414039512,
348.603627656267));
#123141=CARTESIAN_POINT('Ctrl Pts',(-48.4518556663351,1076.65941239181,
348.712280146129));
#123142=CARTESIAN_POINT('Ctrl Pts',(-48.178794140413,1076.66989527097,348.985831772015));
#123143=CARTESIAN_POINT('Ctrl Pts',(-48.0703593694701,1076.6750017051,349.148150999423));
#123144=CARTESIAN_POINT('Ctrl Pts',(-47.9212624073684,1076.68439492229,
349.507424230142));
#123145=CARTESIAN_POINT('Ctrl Pts',(-47.8828801681462,1076.68858075922,
349.701217613954));
#123146=CARTESIAN_POINT('Ctrl Pts',(-47.8838021698197,1076.69561581394,
350.091731480461));
#123147=CARTESIAN_POINT('Ctrl Pts',(-47.9227879557564,1076.69840881142,
350.284606960883));
#123148=CARTESIAN_POINT('Ctrl Pts',(-48.0736060068292,1076.70260581189,
350.644772576739));
#123149=CARTESIAN_POINT('Ctrl Pts',(-48.1842076763103,1076.7039716175,350.80840891566));
#123150=CARTESIAN_POINT('Ctrl Pts',(-48.4630809225606,1076.70533906345,
351.083518673881));
#123151=CARTESIAN_POINT('Ctrl Pts',(-48.6287430128023,1076.70532690411,
351.19211005852));
#123152=CARTESIAN_POINT('Ctrl Pts',(-48.9861537457672,1076.70393342627,
351.335635161093));
#123153=CARTESIAN_POINT('Ctrl Pts',(-49.1734369125114,1076.70261081877,
351.371779853132));
#123154=CARTESIAN_POINT('Ctrl Pts',(-49.3624372582816,1076.70060106622,
351.371678065143));
#123155=CARTESIAN_POINT('Origin',(-49.3616411037539,1067.7251047501,349.893375147338));
#123156=CARTESIAN_POINT('',(-49.3616411037539,1076.69042463418,350.771678279532));
#123157=CARTESIAN_POINT('',(-49.3616411037048,1076.65225835227,349.015072015145));
#123158=CARTESIAN_POINT('Ctrl Pts',(-49.3616411037539,1076.69042463418,
350.771678279532));
#123159=CARTESIAN_POINT('Ctrl Pts',(-49.3625704187744,1076.69041333812,
350.771678279532));
#123160=CARTESIAN_POINT('Ctrl Pts',(-49.3634998059874,1076.69040201185,
350.771676804597));
#123161=CARTESIAN_POINT('Ctrl Pts',(-49.4809116296106,1076.6889674243,350.771304080901));
#123162=CARTESIAN_POINT('Ctrl Pts',(-49.5961581176758,1076.6870980418,350.747765838718));
#123163=CARTESIAN_POINT('Ctrl Pts',(-49.8110004431342,1076.68255175518,
350.657001385538));
#123164=CARTESIAN_POINT('Ctrl Pts',(-49.9084153153564,1076.67991546678,
350.590572237286));
#123165=CARTESIAN_POINT('Ctrl Pts',(-50.0713045452949,1076.67415320759,
350.423789609162));
#123166=CARTESIAN_POINT('Ctrl Pts',(-50.1352663641717,1076.67108484349,
350.325190465426));
#123167=CARTESIAN_POINT('Ctrl Pts',(-50.2205951676991,1076.66495902319,
350.109905191831));
#123168=CARTESIAN_POINT('Ctrl Pts',(-50.2415618915099,1076.66196233688,
349.995495063625));
#123169=CARTESIAN_POINT('Ctrl Pts',(-50.2381316140452,1076.65650070811,
349.765084242071));
#123170=CARTESIAN_POINT('Ctrl Pts',(-50.2137590463193,1076.65409128658,
349.651315422922));
#123171=CARTESIAN_POINT('Ctrl Pts',(-50.1224986918316,1076.6503118739,349.439751385887));
#123172=CARTESIAN_POINT('Ctrl Pts',(-50.0565270679309,1076.64898016664,
349.343997948549));
#123173=CARTESIAN_POINT('Ctrl Pts',(-49.891513023805,1076.64766604219,349.1835328555));
#123174=CARTESIAN_POINT('Ctrl Pts',(-49.7941231829853,1076.64769517389,
349.120329542137));
#123175=CARTESIAN_POINT('Ctrl Pts',(-49.583695091253,1076.64909847968,349.036310411531));
#123176=CARTESIAN_POINT('Ctrl Pts',(-49.4731558007671,1076.65041868008,
349.015072015133));
#123177=CARTESIAN_POINT('Ctrl Pts',(-49.3616411036557,1076.65225835227,
349.015072015145));
#123178=CARTESIAN_POINT('',(-49.3616411037539,1082.7251047501,349.015072015145));
#123179=CARTESIAN_POINT('',(-49.3616411037539,1067.7251047501,349.015072015145));
#123180=CARTESIAN_POINT('Origin',(-49.3616411037539,1082.7251047501,349.893375147338));
#123181=CARTESIAN_POINT('Ctrl Pts',(-49.3616411036557,1076.65225835227,
349.015072015145));
#123182=CARTESIAN_POINT('Ctrl Pts',(-49.358388971609,1076.65231200311,349.015072015146));
#123183=CARTESIAN_POINT('Ctrl Pts',(-49.3551360099501,1076.65236609375,
349.015090077852));
#123184=CARTESIAN_POINT('Ctrl Pts',(-49.237082057938,1076.65434454469,349.016401844435));
#123185=CARTESIAN_POINT('Ctrl Pts',(-49.1236465415889,1076.65677534514,
349.040174079882));
#123186=CARTESIAN_POINT('Ctrl Pts',(-48.9122815362571,1076.6622589491,349.130033646003));
#123187=CARTESIAN_POINT('Ctrl Pts',(-48.8163994673081,1076.66525699316,
349.195289044838));
#123188=CARTESIAN_POINT('Ctrl Pts',(-48.6551513088489,1076.67133890587,
349.359051416487));
#123189=CARTESIAN_POINT('Ctrl Pts',(-48.5913579463045,1076.67436309738,
349.456002597264));
#123190=CARTESIAN_POINT('Ctrl Pts',(-48.5070154856061,1076.67988048972,
349.663384664));
#123191=CARTESIAN_POINT('Ctrl Pts',(-48.4851032457939,1076.68234651501,
349.771045990123));
#123192=CARTESIAN_POINT('Ctrl Pts',(-48.4834403150115,1076.68450315177,
349.879967437887));
#123193=CARTESIAN_POINT('Ctrl Pts',(-48.48166237498,1076.68680894276,349.996421955609));
#123194=CARTESIAN_POINT('Ctrl Pts',(-48.5030657737506,1076.68871900412,
350.112081873623));
#123195=CARTESIAN_POINT('Ctrl Pts',(-48.5898341393267,1076.69165504541,
350.328517937336));
#123196=CARTESIAN_POINT('Ctrl Pts',(-48.6544168509016,1076.69265298522,
350.427108128113));
#123197=CARTESIAN_POINT('Ctrl Pts',(-48.8184786592588,1076.69368492031,
350.593416341232));
#123198=CARTESIAN_POINT('Ctrl Pts',(-48.9163750845321,1076.69370826272,
350.659417789244));
#123199=CARTESIAN_POINT('Ctrl Pts',(-49.1312263548964,1076.69277304321,
350.748789351629));
#123200=CARTESIAN_POINT('Ctrl Pts',(-49.2458735547687,1076.69183181851,
350.771678279532));
#123201=CARTESIAN_POINT('Ctrl Pts',(-49.3616411037539,1076.69042463418,
350.771678279532));
#123202=CARTESIAN_POINT('Origin',(-44.0648939479107,1067.7251047501,338.506780125395));
#123203=CARTESIAN_POINT('',(-44.0648939479323,1076.26837051893,337.231336004259));
#123204=CARTESIAN_POINT('',(-44.0648939479107,1067.7251047501,337.231336004259));
#123205=CARTESIAN_POINT('Ctrl Pts',(-44.0649261075141,1076.4151789643,339.782224246126));
#123206=CARTESIAN_POINT('Ctrl Pts',(-44.2336598940819,1076.41060464631,
339.782219991599));
#123207=CARTESIAN_POINT('Ctrl Pts',(-44.4006651244362,1076.40426367171,
339.748733322867));
#123208=CARTESIAN_POINT('Ctrl Pts',(-44.7122484929901,1076.38855220908,
339.618652496492));
#123209=CARTESIAN_POINT('Ctrl Pts',(-44.8536809853667,1076.37932519515,
339.52319728587));
#123210=CARTESIAN_POINT('Ctrl Pts',(-45.0306315424271,1076.36420574997,
339.344027076611));
#123211=CARTESIAN_POINT('Ctrl Pts',(-45.0829933660694,1076.35904397866,
339.279503945446));
#123212=CARTESIAN_POINT('Ctrl Pts',(-45.1752520753158,1076.34839634336,
339.140008453564));
#123213=CARTESIAN_POINT('Ctrl Pts',(-45.2146887254062,1076.34293216348,
339.065210168011));
#123214=CARTESIAN_POINT('Ctrl Pts',(-45.309571491767,1076.32656966431,338.831790783897));
#123215=CARTESIAN_POINT('Ctrl Pts',(-45.3414761794732,1076.31578487138,
338.665554696912));
#123216=CARTESIAN_POINT('Ctrl Pts',(-45.3391385409566,1076.29577801926,
338.330304067015));
#123217=CARTESIAN_POINT('Ctrl Pts',(-45.3049515910949,1076.28675174734,
338.164518416843));
#123218=CARTESIAN_POINT('Ctrl Pts',(-45.1744747321936,1076.2719115661,337.855950572801));
#123219=CARTESIAN_POINT('Ctrl Pts',(-45.079605021859,1076.26623866432,337.716115255821));
#123220=CARTESIAN_POINT('Ctrl Pts',(-44.8415852495467,1076.259208809,337.481430483732));
#123221=CARTESIAN_POINT('Ctrl Pts',(-44.7009398145652,1076.25790804247,
337.38872474482));
#123222=CARTESIAN_POINT('Ctrl Pts',(-44.3922760685759,1076.25991350823,
337.262879219626));
#123223=CARTESIAN_POINT('Ctrl Pts',(-44.227347641951,1076.26318826141,337.230829011179));
#123224=CARTESIAN_POINT('Ctrl Pts',(-43.8945015931953,1076.27380526315,
337.231855349343));
#123225=CARTESIAN_POINT('Ctrl Pts',(-43.7298146663088,1076.28104267337,
337.264949285428));
#123226=CARTESIAN_POINT('Ctrl Pts',(-43.4221342121765,1076.29837523064,
337.39258424967));
#123227=CARTESIAN_POINT('Ctrl Pts',(-43.2821552025762,1076.30830719036,
337.486065369304));
#123228=CARTESIAN_POINT('Ctrl Pts',(-43.1050532123365,1076.32411306166,
337.662723940361));
#123229=CARTESIAN_POINT('Ctrl Pts',(-43.0518889994096,1076.32950057698,
337.727328676111));
#123230=CARTESIAN_POINT('Ctrl Pts',(-42.9589294291105,1076.34033751772,
337.866020596402));
#123231=CARTESIAN_POINT('Ctrl Pts',(-42.9193609705127,1076.34576122432,
337.939783417094));
#123232=CARTESIAN_POINT('Ctrl Pts',(-42.8221237512356,1076.36197546012,
338.173521564673));
#123233=CARTESIAN_POINT('Ctrl Pts',(-42.7888468807461,1076.37236605329,
338.341636945681));
#123234=CARTESIAN_POINT('Ctrl Pts',(-42.7900653299466,1076.39102444614,
338.680003284053));
#123235=CARTESIAN_POINT('Ctrl Pts',(-42.8241096351059,1076.39912655215,
338.846913054497));
#123236=CARTESIAN_POINT('Ctrl Pts',(-42.9552802592578,1076.4122089099,339.157939313282));
#123237=CARTESIAN_POINT('Ctrl Pts',(-43.0511214816866,1076.41706360979,
339.298959797462));
#123238=CARTESIAN_POINT('Ctrl Pts',(-43.2925182921174,1076.42302688752,
339.535782995973));
#123239=CARTESIAN_POINT('Ctrl Pts',(-43.4357602165995,1076.42407033161,
339.629103391144));
#123240=CARTESIAN_POINT('Ctrl Pts',(-43.7432075571928,1076.42224124413,
339.751529034989));
#123241=CARTESIAN_POINT('Ctrl Pts',(-43.9033505103276,1076.41955922611,
339.782228320163));
#123242=CARTESIAN_POINT('Ctrl Pts',(-44.064926107514,1076.4151789643,339.782224246126));
#123243=CARTESIAN_POINT('Origin',(-44.0648939479107,1067.7251047501,338.506780125395));
#123244=CARTESIAN_POINT('',(-44.0648939479107,1076.38310559156,339.182224246531));
#123245=CARTESIAN_POINT('',(-44.0648939479116,1076.3053526307,337.831336004259));
#123246=CARTESIAN_POINT('Ctrl Pts',(-44.0648939479107,1076.38310559156,
339.182224246531));
#123247=CARTESIAN_POINT('Ctrl Pts',(-44.0701053267806,1076.38295851287,
339.182224246531));
#123248=CARTESIAN_POINT('Ctrl Pts',(-44.07531929434,1076.382807996,339.182163934248));
#123249=CARTESIAN_POINT('Ctrl Pts',(-44.1703403507942,1076.3800033562,339.179962995578));
#123250=CARTESIAN_POINT('Ctrl Pts',(-44.2587997309686,1076.37639117361,
339.159989869285));
#123251=CARTESIAN_POINT('Ctrl Pts',(-44.422867070002,1076.36759865339,339.086586505214));
#123252=CARTESIAN_POINT('Ctrl Pts',(-44.4968037028826,1076.36250120841,
339.033812918612));
#123253=CARTESIAN_POINT('Ctrl Pts',(-44.5883168675794,1076.35427915154,
338.935959179585));
#123254=CARTESIAN_POINT('Ctrl Pts',(-44.6151895017533,1076.35149386377,
338.900912515337));
#123255=CARTESIAN_POINT('Ctrl Pts',(-44.6620541643205,1076.34579761963,
338.825560558424));
#123256=CARTESIAN_POINT('Ctrl Pts',(-44.6818289598925,1076.34289924136,
338.785370116022));
#123257=CARTESIAN_POINT('Ctrl Pts',(-44.7285808174976,1076.33428482065,
338.660445497062));
#123258=CARTESIAN_POINT('Ctrl Pts',(-44.743010021877,1076.32868756283,338.572034526306));
#123259=CARTESIAN_POINT('Ctrl Pts',(-44.7368560300366,1076.31843825193,
338.394749413042));
#123260=CARTESIAN_POINT('Ctrl Pts',(-44.7163664259211,1076.31388509559,
338.307582723559));
#123261=CARTESIAN_POINT('Ctrl Pts',(-44.6429157475108,1076.30650787739,
338.14629644736));
#123262=CARTESIAN_POINT('Ctrl Pts',(-44.5907474285419,1076.30375264393,
338.073714035702));
#123263=CARTESIAN_POINT('Ctrl Pts',(-44.461504086302,1076.30046952909,337.952952110373));
#123264=CARTESIAN_POINT('Ctrl Pts',(-44.3857627848415,1076.29996838611,
337.905888769468));
#123265=CARTESIAN_POINT('Ctrl Pts',(-44.2269518232933,1076.30125692338,
337.846034014573));
#123266=CARTESIAN_POINT('Ctrl Pts',(-44.1462502246026,1076.30285836369,
337.831336791843));
#123267=CARTESIAN_POINT('Ctrl Pts',(-44.0649004869312,1076.30535243022,
337.831336004291));
#123268=CARTESIAN_POINT('',(-44.0648939479107,1082.7251047501,337.831336004259));
#123269=CARTESIAN_POINT('',(-44.0648939479107,1067.7251047501,337.831336004259));
#123270=CARTESIAN_POINT('Origin',(-44.0648939479107,1082.7251047501,338.506780125395));
#123271=CARTESIAN_POINT('Ctrl Pts',(-44.0648939479131,1076.3053526307,337.831336004259));
#123272=CARTESIAN_POINT('Ctrl Pts',(-43.9766448134179,1076.30805827353,
337.831336004259));
#123273=CARTESIAN_POINT('Ctrl Pts',(-43.889288750267,1076.31176270499,337.848628616159));
#123274=CARTESIAN_POINT('Ctrl Pts',(-43.7260036952492,1076.32070212658,
337.915854565925));
#123275=CARTESIAN_POINT('Ctrl Pts',(-43.6516833975952,1076.3258532554,337.965220516065));
#123276=CARTESIAN_POINT('Ctrl Pts',(-43.5576135704436,1076.33411829575,
338.058621136685));
#123277=CARTESIAN_POINT('Ctrl Pts',(-43.5293733861181,1076.33694500713,
338.092778854888));
#123278=CARTESIAN_POINT('Ctrl Pts',(-43.4799654418549,1076.34265482929,
338.166133842445));
#123279=CARTESIAN_POINT('Ctrl Pts',(-43.4589184628472,1076.34552439997,
338.205159436198));
#123280=CARTESIAN_POINT('Ctrl Pts',(-43.4070362814347,1076.35415686086,
338.32909816132));
#123281=CARTESIAN_POINT('Ctrl Pts',(-43.3892155291544,1076.35974582471,
338.41838465554));
#123282=CARTESIAN_POINT('Ctrl Pts',(-43.3896877983555,1076.36987042931,
338.598348130609));
#123283=CARTESIAN_POINT('Ctrl Pts',(-43.4078277279341,1076.37431118753,
338.68723528674));
#123284=CARTESIAN_POINT('Ctrl Pts',(-43.4778407350897,1076.38150504704,
338.852695445679));
#123285=CARTESIAN_POINT('Ctrl Pts',(-43.5289898388636,1076.38418867834,
338.927619124806));
#123286=CARTESIAN_POINT('Ctrl Pts',(-43.6576940453655,1076.38746799743,
339.053129768485));
#123287=CARTESIAN_POINT('Ctrl Pts',(-43.733965202815,1076.38802990554,339.102429483049));
#123288=CARTESIAN_POINT('Ctrl Pts',(-43.8964582207888,1076.38697465127,
339.16634457229));
#123289=CARTESIAN_POINT('Ctrl Pts',(-43.980335296259,1076.38549205715,339.182224246531));
#123290=CARTESIAN_POINT('Ctrl Pts',(-44.0648939479107,1076.38310559156,
339.182224246531));
#123291=CARTESIAN_POINT('Origin',(-37.1057957606635,1067.7251047501,326.532256785149));
#123292=CARTESIAN_POINT('',(-37.1057957606863,1075.54602985383,325.433425649156));
#123293=CARTESIAN_POINT('',(-37.1057957606635,1067.7251047501,325.433425649156));
#123294=CARTESIAN_POINT('Ctrl Pts',(-37.1058073123272,1075.76001085596,
327.63108792108));
#123295=CARTESIAN_POINT('Ctrl Pts',(-37.2518284405106,1075.75482651318,
327.631086386007));
#123296=CARTESIAN_POINT('Ctrl Pts',(-37.3962598046139,1075.74695417433,
327.601981034185));
#123297=CARTESIAN_POINT('Ctrl Pts',(-37.6650853491754,1075.72665806207,
327.489263457504));
#123298=CARTESIAN_POINT('Ctrl Pts',(-37.7867990112802,1075.71443564425,
327.406797640552));
#123299=CARTESIAN_POINT('Ctrl Pts',(-37.9914435144782,1075.68708110747,
327.198924779726));
#123300=CARTESIAN_POINT('Ctrl Pts',(-38.0721596202323,1075.67219889787,
327.075320147664));
#123301=CARTESIAN_POINT('Ctrl Pts',(-38.180945642096,1075.64166922648,326.802791977858));
#123302=CARTESIAN_POINT('Ctrl Pts',(-38.2075079548967,1075.62631399735,
326.656321017783));
#123303=CARTESIAN_POINT('Ctrl Pts',(-38.2013114880832,1075.59771489936,
326.364408113399));
#123304=CARTESIAN_POINT('Ctrl Pts',(-38.169749465209,1075.58470882455,326.221764156176));
#123305=CARTESIAN_POINT('Ctrl Pts',(-38.0532988666014,1075.56269452548,
325.957446292491));
#123306=CARTESIAN_POINT('Ctrl Pts',(-37.9698350118053,1075.55388054548,
325.838221115935));
#123307=CARTESIAN_POINT('Ctrl Pts',(-37.7620152173118,1075.54176321282,
325.639303563615));
#123308=CARTESIAN_POINT('Ctrl Pts',(-37.6399766875971,1075.53854797351,
325.561342179345));
#123309=CARTESIAN_POINT('Ctrl Pts',(-37.3731357590198,1075.53819317261,
325.456886005567));
#123310=CARTESIAN_POINT('Ctrl Pts',(-37.2310757442444,1075.54103782532,
325.431272211773));
#123311=CARTESIAN_POINT('Ctrl Pts',(-36.9449401196969,1075.55240702316,
325.435867034869));
#123312=CARTESIAN_POINT('Ctrl Pts',(-36.8036954486044,1075.56082839968,
325.466140682772));
#123313=CARTESIAN_POINT('Ctrl Pts',(-36.5401773185045,1075.58211239206,
325.579268049508));
#123314=CARTESIAN_POINT('Ctrl Pts',(-36.4205720923164,1075.59479213284,
325.661335190783));
#123315=CARTESIAN_POINT('Ctrl Pts',(-36.2192627347873,1075.62267128543,
325.867176742192));
#123316=CARTESIAN_POINT('Ctrl Pts',(-36.1396820771978,1075.63761886704,
325.989239640643));
#123317=CARTESIAN_POINT('Ctrl Pts',(-36.0592605433807,1075.66012338436,
326.189708769316));
#123318=CARTESIAN_POINT('Ctrl Pts',(-36.0391332125001,1075.66756631343,
326.258745241083));
#123319=CARTESIAN_POINT('Ctrl Pts',(-35.9989565568231,1075.68971399939,
326.472477529121));
#123320=CARTESIAN_POINT('Ctrl Pts',(-36.0007730411933,1075.70377809693,
326.61973599735));
#123321=CARTESIAN_POINT('Ctrl Pts',(-36.0618194981078,1075.72874992371,
326.904693915371));
#123322=CARTESIAN_POINT('Ctrl Pts',(-36.1202761882012,1075.73942548664,
327.039631897666));
#123323=CARTESIAN_POINT('Ctrl Pts',(-36.2867996883745,1075.75607775343,
327.279251163207));
#123324=CARTESIAN_POINT('Ctrl Pts',(-36.393269326976,1075.76187977416,327.3814441553));
#123325=CARTESIAN_POINT('Ctrl Pts',(-36.6375840605244,1075.76775699067,
327.536602841777));
#123326=CARTESIAN_POINT('Ctrl Pts',(-36.7723094344706,1075.76789137202,
327.589007226966));
#123327=CARTESIAN_POINT('Ctrl Pts',(-36.9768529295806,1075.76405293402,
327.625404456655));
#123328=CARTESIAN_POINT('Ctrl Pts',(-37.0412749341261,1075.76230201733,
327.631088599489));
#123329=CARTESIAN_POINT('Ctrl Pts',(-37.1058073123272,1075.76001085596,
327.63108792108));
#123330=CARTESIAN_POINT('Origin',(-37.1057957606635,1067.7251047501,326.532256785149));
#123331=CARTESIAN_POINT('',(-37.1057957606635,1075.70357965628,327.031087921141));
#123332=CARTESIAN_POINT('',(-37.1057957606635,1075.60643384366,326.033425649156));
#123333=CARTESIAN_POINT('Ctrl Pts',(-37.1057957606635,1075.70357965628,
327.031087921141));
#123334=CARTESIAN_POINT('Ctrl Pts',(-37.140106488576,1075.7023363494,327.031087921141));
#123335=CARTESIAN_POINT('Ctrl Pts',(-37.1743956888152,1075.70075395455,
327.027547901333));
#123336=CARTESIAN_POINT('Ctrl Pts',(-37.273219899766,1075.69517982228,327.006837474669));
#123337=CARTESIAN_POINT('Ctrl Pts',(-37.3348755442173,1075.69039082338,
326.980322296078));
#123338=CARTESIAN_POINT('Ctrl Pts',(-37.444177405344,1075.67911765527,326.904750563201));
#123339=CARTESIAN_POINT('Ctrl Pts',(-37.4907178407904,1075.67274226759,
326.856410606957));
#123340=CARTESIAN_POINT('Ctrl Pts',(-37.5622347215614,1075.65923254556,
326.74423882876));
#123341=CARTESIAN_POINT('Ctrl Pts',(-37.5864371812949,1075.65222653652,
326.681440921334));
#123342=CARTESIAN_POINT('Ctrl Pts',(-37.6087771550836,1075.63854469637,
326.549854573336));
#123343=CARTESIAN_POINT('Ctrl Pts',(-37.6066148687186,1075.63200363463,
326.482331093145));
#123344=CARTESIAN_POINT('Ctrl Pts',(-37.5760845179854,1075.62047616974,
326.35353043989));
#123345=CARTESIAN_POINT('Ctrl Pts',(-37.5485935844269,1075.61556928953,
326.293380523485));
#123346=CARTESIAN_POINT('Ctrl Pts',(-37.4720539903056,1075.60796033873,
326.187387836821));
#123347=CARTESIAN_POINT('Ctrl Pts',(-37.4238868403951,1075.60532031765,
326.142500625099));
#123348=CARTESIAN_POINT('Ctrl Pts',(-37.3131435041877,1075.60267900704,
326.073930327446));
#123349=CARTESIAN_POINT('Ctrl Pts',(-37.2517311074801,1075.60269334399,
326.050843199775));
#123350=CARTESIAN_POINT('Ctrl Pts',(-37.1605723102931,1075.60460678886,
326.035684601278));
#123351=CARTESIAN_POINT('Ctrl Pts',(-37.1332046641734,1075.60540804463,
326.033425719712));
#123352=CARTESIAN_POINT('Ctrl Pts',(-37.1057970447751,1075.6064337956,326.033425649158));
#123353=CARTESIAN_POINT('',(-37.1057957606635,1082.7251047501,326.033425649156));
#123354=CARTESIAN_POINT('',(-37.1057957606635,1067.7251047501,326.033425649156));
#123355=CARTESIAN_POINT('Origin',(-37.1057957606635,1082.7251047501,326.532256785149));
#123356=CARTESIAN_POINT('Ctrl Pts',(-37.1057957606636,1075.60643384366,
326.033425649156));
#123357=CARTESIAN_POINT('Ctrl Pts',(-37.0407169455499,1075.6088694843,326.033425649156));
#123358=CARTESIAN_POINT('Ctrl Pts',(-36.9763277968887,1075.61253673435,
326.046159525286));
#123359=CARTESIAN_POINT('Ctrl Pts',(-36.8558063188034,1075.6219137584,326.095671962726));
#123360=CARTESIAN_POINT('Ctrl Pts',(-36.8008960338681,1075.62754321943,
326.132105180252));
#123361=CARTESIAN_POINT('Ctrl Pts',(-36.7071388769123,1075.64013808892,
326.225060758133));
#123362=CARTESIAN_POINT('Ctrl Pts',(-36.6696435445463,1075.64700825431,
326.281138031886));
#123363=CARTESIAN_POINT('Ctrl Pts',(-36.6319410649877,1075.65734999268,
326.373025779382));
#123364=CARTESIAN_POINT('Ctrl Pts',(-36.622558756964,1075.6607360617,326.404291296112));
#123365=CARTESIAN_POINT('Ctrl Pts',(-36.6035095940503,1075.67086637644,
326.501416618221));
#123366=CARTESIAN_POINT('Ctrl Pts',(-36.6038605143582,1075.67734593208,
326.568529010141));
#123367=CARTESIAN_POINT('Ctrl Pts',(-36.6308674213977,1075.68891197812,
326.698635881763));
#123368=CARTESIAN_POINT('Ctrl Pts',(-36.6572112485464,1075.69388735971,
326.760353983765));
#123369=CARTESIAN_POINT('Ctrl Pts',(-36.7322444818216,1075.70162342845,
326.869335007153));
#123370=CARTESIAN_POINT('Ctrl Pts',(-36.7799438054035,1075.70433043034,
326.915656103613));
#123371=CARTESIAN_POINT('Ctrl Pts',(-36.8899237168445,1075.70714178724,
326.986631850417));
#123372=CARTESIAN_POINT('Ctrl Pts',(-36.9509059692144,1075.70725318984,
327.010866369372));
#123373=CARTESIAN_POINT('Ctrl Pts',(-37.0449053721231,1075.70551868177,
327.028302317338));
#123374=CARTESIAN_POINT('Ctrl Pts',(-37.0753590365554,1075.70468258213,
327.031087921141));
#123375=CARTESIAN_POINT('Ctrl Pts',(-37.1057957606635,1075.70357965628,
327.031087921141));
#123376=CARTESIAN_POINT('Origin',(-27.7552687727512,1067.7251047501,316.130256973654));
#123377=CARTESIAN_POINT('',(-27.7552687727736,1074.65680240674,315.039716224926));
#123378=CARTESIAN_POINT('',(-27.7552687727512,1067.7251047501,315.039716224926));
#123379=CARTESIAN_POINT('Ctrl Pts',(-27.7552727853641,1074.94285712098,
317.220797722375));
#123380=CARTESIAN_POINT('Ctrl Pts',(-27.8973584452209,1074.93820301204,
317.220797199575));
#123381=CARTESIAN_POINT('Ctrl Pts',(-28.0378937657681,1074.93004129443,
317.193032001366));
#123382=CARTESIAN_POINT('Ctrl Pts',(-28.3030665935802,1074.90733597777,
317.084292366754));
#123383=CARTESIAN_POINT('Ctrl Pts',(-28.4245787743323,1074.89288518666,
317.003270315551));
#123384=CARTESIAN_POINT('Ctrl Pts',(-28.6292838197719,1074.85956610145,
316.798433088887));
#123385=CARTESIAN_POINT('Ctrl Pts',(-28.7102642929308,1074.84099679104,
316.676382741362));
#123386=CARTESIAN_POINT('Ctrl Pts',(-28.7918734176438,1074.81211645738,
316.476365811308));
#123387=CARTESIAN_POINT('Ctrl Pts',(-28.8122365366506,1074.8024781713,316.408029337154));
#123388=CARTESIAN_POINT('Ctrl Pts',(-28.85373449036,1074.77302037737,316.194396321065));
#123389=CARTESIAN_POINT('Ctrl Pts',(-28.8524287703557,1074.75351190795,
316.046308775394));
#123390=CARTESIAN_POINT('Ctrl Pts',(-28.7918689412043,1074.71791835285,
315.762327358554));
#123391=CARTESIAN_POINT('Ctrl Pts',(-28.7343987300333,1074.70210609435,
315.628907896589));
#123392=CARTESIAN_POINT('Ctrl Pts',(-28.5713852237671,1074.67617142822,
315.392974176405));
#123393=CARTESIAN_POINT('Ctrl Pts',(-28.4679187224216,1074.66624974281,
315.29247203694));
#123394=CARTESIAN_POINT('Ctrl Pts',(-28.2287806000093,1074.65369806997,
315.137703554575));
#123395=CARTESIAN_POINT('Ctrl Pts',(-28.0958312668207,1074.65113008374,
315.084585446537));
#123396=CARTESIAN_POINT('Ctrl Pts',(-27.8173253647566,1074.65368051675,
315.032329998061));
#123397=CARTESIAN_POINT('Ctrl Pts',(-27.6746487315551,1074.65875008991,
315.033567962164));
#123398=CARTESIAN_POINT('Ctrl Pts',(-27.3971930839227,1074.67587815065,
315.090438759667));
#123399=CARTESIAN_POINT('Ctrl Pts',(-27.2652386157998,1074.68779999794,
315.145787840477));
#123400=CARTESIAN_POINT('Ctrl Pts',(-27.0289748507789,1074.7169759611,315.304291257733));
#123401=CARTESIAN_POINT('Ctrl Pts',(-26.9272378234838,1074.73399973998,
315.406398978482));
#123402=CARTESIAN_POINT('Ctrl Pts',(-26.8082980716652,1074.76159306632,
315.584664699751));
#123403=CARTESIAN_POINT('Ctrl Pts',(-26.7744856246139,1074.77110284607,
315.648093801851));
#123404=CARTESIAN_POINT('Ctrl Pts',(-26.7198903389802,1074.79035914604,
315.780429150949));
#123405=CARTESIAN_POINT('Ctrl Pts',(-26.6991939337255,1074.80006156145,
315.849021623245));
#123406=CARTESIAN_POINT('Ctrl Pts',(-26.6572695965763,1074.82929992101,
316.061489943875));
#123407=CARTESIAN_POINT('Ctrl Pts',(-26.6578452791933,1074.84839480724,
316.208149109684));
#123408=CARTESIAN_POINT('Ctrl Pts',(-26.7163654965046,1074.88327995893,
316.491938847863));
#123409=CARTESIAN_POINT('Ctrl Pts',(-26.7733835538738,1074.89875909424,
316.626412377309));
#123410=CARTESIAN_POINT('Ctrl Pts',(-26.9368389624288,1074.92413906852,
316.865353924037));
#123411=CARTESIAN_POINT('Ctrl Pts',(-27.0415458977297,1074.93379587298,
316.967462358757));
#123412=CARTESIAN_POINT('Ctrl Pts',(-27.2823376330203,1074.94583858414,
317.123073465832));
#123413=CARTESIAN_POINT('Ctrl Pts',(-27.4152213834633,1074.94826787575,
317.176081451513));
#123414=CARTESIAN_POINT('Ctrl Pts',(-27.6207763410728,1074.946463579,317.214566103836));
#123415=CARTESIAN_POINT('Ctrl Pts',(-27.6879608245359,1074.94506196839,
317.220797970047));
#123416=CARTESIAN_POINT('Ctrl Pts',(-27.7552727853641,1074.94285712098,
317.220797722375));
#123417=CARTESIAN_POINT('Origin',(-27.7552687727512,1067.7251047501,316.130256973654));
#123418=CARTESIAN_POINT('',(-27.7552687727512,1074.86607808781,316.620797722383));
#123419=CARTESIAN_POINT('',(-27.7552687727512,1074.73740020174,315.639716224926));
#123420=CARTESIAN_POINT('Ctrl Pts',(-27.7552687727512,1074.86607808781,
316.620797722383));
#123421=CARTESIAN_POINT('Ctrl Pts',(-27.7884696064037,1074.86497585636,
316.620797722383));
#123422=CARTESIAN_POINT('Ctrl Pts',(-27.8216492971736,1074.86343664612,
316.617427003901));
#123423=CARTESIAN_POINT('Ctrl Pts',(-27.9170085408949,1074.85771584,316.59777272351));
#123424=CARTESIAN_POINT('Ctrl Pts',(-27.9764850729975,1074.85248196319,
316.572714128191));
#123425=CARTESIAN_POINT('Ctrl Pts',(-28.0837233019206,1074.83949904116,
316.500440952334));
#123426=CARTESIAN_POINT('Ctrl Pts',(-28.1300673257111,1074.831818402,316.453397041095));
#123427=CARTESIAN_POINT('Ctrl Pts',(-28.1833214032295,1074.81939504425,
316.371970184342));
#123428=CARTESIAN_POINT('Ctrl Pts',(-28.198167470537,1074.8151797047,316.343548883207));
#123429=CARTESIAN_POINT('Ctrl Pts',(-28.222132474559,1074.8066020564,316.284188817218));
#123430=CARTESIAN_POINT('Ctrl Pts',(-28.2311863850425,1074.8022586878,316.25337819008));
#123431=CARTESIAN_POINT('Ctrl Pts',(-28.2494497329859,1074.78904135798,
316.157349397889));
#123432=CARTESIAN_POINT('Ctrl Pts',(-28.2486406854603,1074.78032991429,
316.090923533509));
#123433=CARTESIAN_POINT('Ctrl Pts',(-28.2209875291239,1074.76440635846,
315.9630313853));
#123434=CARTESIAN_POINT('Ctrl Pts',(-28.1947220220795,1074.75732954294,
315.902733652316));
#123435=CARTESIAN_POINT('Ctrl Pts',(-28.1206277481484,1074.74581605109,
315.796710376851));
#123436=CARTESIAN_POINT('Ctrl Pts',(-28.0739006966746,1074.74144915903,
315.751788809119));
#123437=CARTESIAN_POINT('Ctrl Pts',(-27.9660563149437,1074.73595691929,
315.682749211619));
#123438=CARTESIAN_POINT('Ctrl Pts',(-27.9061520431679,1074.73486034789,
315.659156489425));
#123439=CARTESIAN_POINT('Ctrl Pts',(-27.81430495024,1074.73575206587,315.642385335104));
#123440=CARTESIAN_POINT('Ctrl Pts',(-27.7848132644947,1074.73639847351,
315.639716237778));
#123441=CARTESIAN_POINT('Ctrl Pts',(-27.755268986145,1074.73740019451,315.639716224926));
#123442=CARTESIAN_POINT('',(-27.7552687727512,1082.7251047501,315.639716224926));
#123443=CARTESIAN_POINT('',(-27.7552687727512,1067.7251047501,315.639716224926));
#123444=CARTESIAN_POINT('Origin',(-27.7552687727512,1082.7251047501,316.130256973654));
#123445=CARTESIAN_POINT('Ctrl Pts',(-27.7552687727512,1074.73740020174,
315.639716224926));
#123446=CARTESIAN_POINT('Ctrl Pts',(-27.6915062829793,1074.73956212063,
315.639716224926));
#123447=CARTESIAN_POINT('Ctrl Pts',(-27.6284419276466,1074.74334710473,
315.652146476916));
#123448=CARTESIAN_POINT('Ctrl Pts',(-27.5102192567908,1074.753745222,315.70049679494));
#123449=CARTESIAN_POINT('Ctrl Pts',(-27.4562985012817,1074.76027853999,
315.736134215707));
#123450=CARTESIAN_POINT('Ctrl Pts',(-27.3638940977153,1074.77541819911,
315.827279615052));
#123451=CARTESIAN_POINT('Ctrl Pts',(-27.3268432956719,1074.78393176463,
315.882460540546));
#123452=CARTESIAN_POINT('Ctrl Pts',(-27.2895397096046,1074.79706746359,
315.972911992357));
#123453=CARTESIAN_POINT('Ctrl Pts',(-27.2802430053885,1074.80142252945,
316.003721191227));
#123454=CARTESIAN_POINT('Ctrl Pts',(-27.2613460142679,1074.81459913811,
316.099406401156));
#123455=CARTESIAN_POINT('Ctrl Pts',(-27.2616284401372,1074.82323949055,
316.165544848401));
#123456=CARTESIAN_POINT('Ctrl Pts',(-27.2881526839442,1074.83907391969,
316.29363484863));
#123457=CARTESIAN_POINT('Ctrl Pts',(-27.3140306965928,1074.84612183971,
316.354369608848));
#123458=CARTESIAN_POINT('Ctrl Pts',(-27.3877637173149,1074.85760796943,
316.461532688281));
#123459=CARTESIAN_POINT('Ctrl Pts',(-27.4345898663682,1074.86196601396,
316.50707588247));
#123460=CARTESIAN_POINT('Ctrl Pts',(-27.5425300250943,1074.86743669456,
316.576838097611));
#123461=CARTESIAN_POINT('Ctrl Pts',(-27.6023149030358,1074.86854575969,
316.600686958105));
#123462=CARTESIAN_POINT('Ctrl Pts',(-27.694858086976,1074.86772161904,316.618009572747));
#123463=CARTESIAN_POINT('Ctrl Pts',(-27.7250721744106,1074.86708058192,
316.620797722383));
#123464=CARTESIAN_POINT('Ctrl Pts',(-27.7552687727512,1074.86607808781,
316.620797722383));
#123465=CARTESIAN_POINT('Origin',(-63.8195601713292,1067.7251047501,361.789198753807));
#123466=CARTESIAN_POINT('',(-63.8195601713524,1076.6426633433,360.310895621613));
#123467=CARTESIAN_POINT('',(-63.8195601713292,1067.7251047501,360.310895621613));
#123468=CARTESIAN_POINT('Ctrl Pts',(-63.8201632810582,1076.69670629135,
363.267501762973));
#123469=CARTESIAN_POINT('Ctrl Pts',(-64.015353854477,1076.69386865944,363.267422130224));
#123470=CARTESIAN_POINT('Ctrl Pts',(-64.2085968376498,1076.69033702687,
363.228685102967));
#123471=CARTESIAN_POINT('Ctrl Pts',(-64.5706194753776,1076.68192930682,
363.077661357673));
#123472=CARTESIAN_POINT('Ctrl Pts',(-64.735509565079,1076.67711908905,362.966166911613));
#123473=CARTESIAN_POINT('Ctrl Pts',(-65.0096989131915,1076.66686056675,
362.687302338553));
#123474=CARTESIAN_POINT('Ctrl Pts',(-65.1171648687651,1076.66152410503,
362.523529083437));
#123475=CARTESIAN_POINT('Ctrl Pts',(-65.2627692911948,1076.65111675822,
362.163678711344));
#123476=CARTESIAN_POINT('Ctrl Pts',(-65.2994325087523,1076.64615292214,
361.971061474138));
#123477=CARTESIAN_POINT('Ctrl Pts',(-65.2961912983331,1076.63759819319,
361.582681058723));
#123478=CARTESIAN_POINT('Ctrl Pts',(-65.256325482641,1076.63409755005,361.390693151394));
#123479=CARTESIAN_POINT('Ctrl Pts',(-65.1047862765125,1076.6293551382,361.033458505376));
#123480=CARTESIAN_POINT('Ctrl Pts',(-64.9947309899203,1076.62815957435,
360.871632163452));
#123481=CARTESIAN_POINT('Ctrl Pts',(-64.7188321430135,1076.628364894,360.60005985534));
#123482=CARTESIAN_POINT('Ctrl Pts',(-64.5558209929454,1076.62975614991,
360.492797899789));
#123483=CARTESIAN_POINT('Ctrl Pts',(-64.1980757816965,1076.63482298825,
360.347206975795));
#123484=CARTESIAN_POINT('Ctrl Pts',(-64.00683986861,1076.6384411848,360.310169143266));
#123485=CARTESIAN_POINT('Ctrl Pts',(-63.6208982831683,1076.64714170327,
360.311644008145));
#123486=CARTESIAN_POINT('Ctrl Pts',(-63.4298961045216,1076.65213408422,
360.350175191289));
#123487=CARTESIAN_POINT('Ctrl Pts',(-63.0732830495466,1076.66253495407,
360.498541330444));
#123488=CARTESIAN_POINT('Ctrl Pts',(-62.9111308706323,1076.66783855036,
360.607046398371));
#123489=CARTESIAN_POINT('Ctrl Pts',(-62.6377034902941,1076.67790751942,
360.880364469796));
#123490=CARTESIAN_POINT('Ctrl Pts',(-62.5290851983599,1076.68257505022,
361.042574576914));
#123491=CARTESIAN_POINT('Ctrl Pts',(-62.3797882542706,1076.69080186221,
361.401241248447));
#123492=CARTESIAN_POINT('Ctrl Pts',(-62.3412016120399,1076.69427503924,
361.594470437375));
#123493=CARTESIAN_POINT('Ctrl Pts',(-62.3413125454988,1076.69982894111,
361.984626181701));
#123494=CARTESIAN_POINT('Ctrl Pts',(-62.3799534221957,1076.7018646516,362.177716371857));
#123495=CARTESIAN_POINT('Ctrl Pts',(-62.5302048996037,1076.70456231898,
362.538348616852));
#123496=CARTESIAN_POINT('Ctrl Pts',(-62.6405679067661,1076.70519950057,
362.702238464813));
#123497=CARTESIAN_POINT('Ctrl Pts',(-62.9186743733461,1076.70510896687,
362.977498579521));
#123498=CARTESIAN_POINT('Ctrl Pts',(-63.0836594593772,1076.70438212369,
363.08615667722));
#123499=CARTESIAN_POINT('Ctrl Pts',(-63.4413841836492,1076.70153441586,
363.230923411168));
#123500=CARTESIAN_POINT('Ctrl Pts',(-63.6298963787954,1076.69947234416,
363.267579386992));
#123501=CARTESIAN_POINT('Ctrl Pts',(-63.8201632810582,1076.69670629135,
363.267501762973));
#123502=CARTESIAN_POINT('Origin',(-63.8195601713292,1067.7251047501,361.789198753807));
#123503=CARTESIAN_POINT('',(-63.8195601713292,1076.68781395203,362.667501886));
#123504=CARTESIAN_POINT('',(-63.8195601713159,1076.65571487055,360.910895621613));
#123505=CARTESIAN_POINT('Ctrl Pts',(-63.8195601713292,1076.68781395203,
362.667501886));
#123506=CARTESIAN_POINT('Ctrl Pts',(-63.8199454877377,1076.68780771864,
362.667501886));
#123507=CARTESIAN_POINT('Ctrl Pts',(-63.8203308166387,1076.6878014804,362.667501632439));
#123508=CARTESIAN_POINT('Ctrl Pts',(-63.9373488144158,1076.68590561051,
362.66734761803));
#123509=CARTESIAN_POINT('Ctrl Pts',(-64.0527834853948,1076.68360606599,
362.643963785317));
#123510=CARTESIAN_POINT('Ctrl Pts',(-64.268441678792,1076.67832383068,362.553198415436));
#123511=CARTESIAN_POINT('Ctrl Pts',(-64.3663936634442,1076.67538804155,
362.486451144002));
#123512=CARTESIAN_POINT('Ctrl Pts',(-64.5287569903648,1076.66930624779,
362.319976532879));
#123513=CARTESIAN_POINT('Ctrl Pts',(-64.5921817907566,1076.66622437169,
362.222490044308));
#123514=CARTESIAN_POINT('Ctrl Pts',(-64.6778083774569,1076.6603259619,362.008539966662));
#123515=CARTESIAN_POINT('Ctrl Pts',(-64.6991574664424,1076.65756875994,
361.894137712006));
#123516=CARTESIAN_POINT('Ctrl Pts',(-64.6964480560042,1076.65286913567,
361.663635011196));
#123517=CARTESIAN_POINT('Ctrl Pts',(-64.6724242359687,1076.65097478949,
361.549771841494));
#123518=CARTESIAN_POINT('Ctrl Pts',(-64.5818293995344,1076.64842252704,
361.337966531035));
#123519=CARTESIAN_POINT('Ctrl Pts',(-64.5161979903458,1076.64778936419,
361.242058726776));
#123520=CARTESIAN_POINT('Ctrl Pts',(-64.3518317690396,1076.64791989456,
361.081170561096));
#123521=CARTESIAN_POINT('Ctrl Pts',(-64.2547513026543,1076.64867960996,
361.017691267961));
#123522=CARTESIAN_POINT('Ctrl Pts',(-64.0437424557757,1076.65142648614,
360.932548615098));
#123523=CARTESIAN_POINT('Ctrl Pts',(-63.9321584635616,1076.65336191998,
360.91089562161));
#123524=CARTESIAN_POINT('Ctrl Pts',(-63.8195601713027,1076.65571487055,
360.910895621613));
#123525=CARTESIAN_POINT('',(-63.8195601713292,1082.7251047501,360.910895621613));
#123526=CARTESIAN_POINT('',(-63.8195601713292,1067.7251047501,360.910895621613));
#123527=CARTESIAN_POINT('Origin',(-63.8195601713292,1082.7251047501,361.789198753807));
#123528=CARTESIAN_POINT('Ctrl Pts',(-63.8195601713027,1076.65571487055,
360.910895621613));
#123529=CARTESIAN_POINT('Ctrl Pts',(-63.8174430765292,1076.65575911118,
360.910895621613));
#123530=CARTESIAN_POINT('Ctrl Pts',(-63.8153256231689,1076.65580349898,
360.910903276298));
#123531=CARTESIAN_POINT('Ctrl Pts',(-63.6984101531963,1076.65826207426,
360.911748888507));
#123532=CARTESIAN_POINT('Ctrl Pts',(-63.5848877566488,1076.66105759599,
360.935078370482));
#123533=CARTESIAN_POINT('Ctrl Pts',(-63.3731563508884,1076.66698821698,
361.024121575518));
#123534=CARTESIAN_POINT('Ctrl Pts',(-63.2770008061881,1076.67006465605,
361.08902112782));
#123535=CARTESIAN_POINT('Ctrl Pts',(-63.1151044300733,1076.67604241627,
361.252194543827));
#123536=CARTESIAN_POINT('Ctrl Pts',(-63.0509377109618,1076.67888594666,
361.348911073015));
#123537=CARTESIAN_POINT('Ctrl Pts',(-62.9653862248395,1076.68389356872,
361.557012103622));
#123538=CARTESIAN_POINT('Ctrl Pts',(-62.9430405935998,1076.68603911317,
361.665748668285));
#123539=CARTESIAN_POINT('Ctrl Pts',(-62.941359524766,1076.68781868475,361.775781734884));
#123540=CARTESIAN_POINT('Ctrl Pts',(-62.939580259543,1076.68970220658,361.892242170563));
#123541=CARTESIAN_POINT('Ctrl Pts',(-62.9609847548429,1076.69114215142,
362.007907060518));
#123542=CARTESIAN_POINT('Ctrl Pts',(-63.0477360763869,1076.6930879473,362.224297014507));
#123543=CARTESIAN_POINT('Ctrl Pts',(-63.1122801435149,1076.69357534904,
362.322845446417));
#123544=CARTESIAN_POINT('Ctrl Pts',(-63.2760938107374,1076.69357125405,
362.488961579553));
#123545=CARTESIAN_POINT('Ctrl Pts',(-63.3737312609862,1076.69307979762,
362.554874514465));
#123546=CARTESIAN_POINT('Ctrl Pts',(-63.5885326016093,1076.69112928325,
362.644489116581));
#123547=CARTESIAN_POINT('Ctrl Pts',(-63.7034794771557,1076.68969182472,
362.667501886));
#123548=CARTESIAN_POINT('Ctrl Pts',(-63.8195601713292,1076.68781395203,
362.667501886));
#123549=CARTESIAN_POINT('Origin',(-61.0059658728168,1067.7251047501,349.55017249556));
#123550=CARTESIAN_POINT('',(-61.0059658728379,1076.2784617343,348.274728374424));
#123551=CARTESIAN_POINT('',(-61.0059658728168,1067.7251047501,348.274728374424));
#123552=CARTESIAN_POINT('Ctrl Pts',(-61.0067058992696,1076.40643702417,
350.825616402011));
#123553=CARTESIAN_POINT('Ctrl Pts',(-61.1753054387743,1076.40003226263,
350.825518578721));
#123554=CARTESIAN_POINT('Ctrl Pts',(-61.3421566834799,1076.39205183224,
350.791992768892));
#123555=CARTESIAN_POINT('Ctrl Pts',(-61.6536284043553,1076.37361992364,
350.661873794951));
#123556=CARTESIAN_POINT('Ctrl Pts',(-61.7950931069933,1076.36333748561,
350.566339211117));
#123557=CARTESIAN_POINT('Ctrl Pts',(-61.9720986104835,1076.34724752692,
350.38697296011));
#123558=CARTESIAN_POINT('Ctrl Pts',(-62.0244933194174,1076.34186431443,
350.322343709386));
#123559=CARTESIAN_POINT('Ctrl Pts',(-62.1635103492835,1076.32548494157,
350.111860644301));
#123560=CARTESIAN_POINT('Ctrl Pts',(-62.2277644014619,1076.31462480656,
349.953446951942));
#123561=CARTESIAN_POINT('Ctrl Pts',(-62.2903191259055,1076.29467144139,
349.622542312494));
#123562=CARTESIAN_POINT('Ctrl Pts',(-62.2887286016733,1076.28575627957,
349.453405539597));
#123563=CARTESIAN_POINT('Ctrl Pts',(-62.2202731715604,1076.27118931772,
349.125717544534));
#123564=CARTESIAN_POINT('Ctrl Pts',(-62.1542350328075,1076.26567540096,
348.97032575603));
#123565=CARTESIAN_POINT('Ctrl Pts',(-61.9661507403253,1076.2589831158,348.694243238935));
#123566=CARTESIAN_POINT('Ctrl Pts',(-61.8461220668367,1076.25785922442,
348.576151501845));
#123567=CARTESIAN_POINT('Ctrl Pts',(-61.5676355023932,1076.26021061205,
348.393016521291));
#123568=CARTESIAN_POINT('Ctrl Pts',(-61.4119736280636,1076.26365396946,
348.32967540113));
#123569=CARTESIAN_POINT('Ctrl Pts',(-61.0850425665927,1076.2745774365,348.266328573456));
#123570=CARTESIAN_POINT('Ctrl Pts',(-60.9169365353592,1076.28195160997,
348.266997869564));
#123571=CARTESIAN_POINT('Ctrl Pts',(-60.5901574624181,1076.2995040843,348.332913182217));
#123572=CARTESIAN_POINT('Ctrl Pts',(-60.4346530062398,1076.30951689685,
348.397703227076));
#123573=CARTESIAN_POINT('Ctrl Pts',(-60.2267010518738,1076.32539106199,
348.537021220366));
#123574=CARTESIAN_POINT('Ctrl Pts',(-60.1620682096721,1076.33079084241,
348.590190938777));
#123575=CARTESIAN_POINT('Ctrl Pts',(-60.0442138254672,1076.34162485025,
348.70830501263));
#123576=CARTESIAN_POINT('Ctrl Pts',(-59.9912546462302,1076.34703336414,
348.772953133667));
#123577=CARTESIAN_POINT('Ctrl Pts',(-59.8511883005758,1076.3631541683,348.982891484046));
#123578=CARTESIAN_POINT('Ctrl Pts',(-59.7862395156745,1076.3734464042,349.140762520099));
#123579=CARTESIAN_POINT('Ctrl Pts',(-59.7218127162375,1076.39190480177,
349.472121104942));
#123580=CARTESIAN_POINT('Ctrl Pts',(-59.7227297197432,1076.39990174225,
349.642303386525));
#123581=CARTESIAN_POINT('Ctrl Pts',(-59.7908666233923,1076.41277231975,
349.973164318111));
#123582=CARTESIAN_POINT('Ctrl Pts',(-59.8576467141859,1076.41751133487,
350.130502875937));
#123583=CARTESIAN_POINT('Ctrl Pts',(-60.049186292316,1076.4232156542,350.410533120237));
#123584=CARTESIAN_POINT('Ctrl Pts',(-60.1722347424379,1076.42411128731,
350.530247317855));
#123585=CARTESIAN_POINT('Ctrl Pts',(-60.4577789939867,1076.42191503209,
350.714237017071));
#123586=CARTESIAN_POINT('Ctrl Pts',(-60.6173197527075,1076.41885092961,
350.776747981925));
#123587=CARTESIAN_POINT('Ctrl Pts',(-60.8577860580678,1076.41177372177,
350.819171155113));
#123588=CARTESIAN_POINT('Ctrl Pts',(-60.9321818678592,1076.40926804406,
350.825659641666));
#123589=CARTESIAN_POINT('Ctrl Pts',(-61.0067058992696,1076.40643702417,
350.825616402011));
#123590=CARTESIAN_POINT('Origin',(-61.0059658728168,1067.7251047501,349.55017249556));
#123591=CARTESIAN_POINT('',(-61.0059658728168,1076.37831455598,350.225616616696));
#123592=CARTESIAN_POINT('',(-61.0059658728176,1076.31052966192,348.874728374424));
#123593=CARTESIAN_POINT('Ctrl Pts',(-61.0059658728168,1076.37831455598,
350.225616616696));
#123594=CARTESIAN_POINT('Ctrl Pts',(-61.0542344883888,1076.37641783823,
350.225616616696));
#123595=CARTESIAN_POINT('Ctrl Pts',(-61.1024739458748,1076.37426575044,
350.220442463225));
#123596=CARTESIAN_POINT('Ctrl Pts',(-61.2375448907151,1076.36748370411,
350.190994170549));
#123597=CARTESIAN_POINT('Ctrl Pts',(-61.3205272413257,1076.3623903405,350.154591162086));
#123598=CARTESIAN_POINT('Ctrl Pts',(-61.4298965737918,1076.35418408558,
350.077842621852));
#123599=CARTESIAN_POINT('Ctrl Pts',(-61.4632927026525,1076.35140697668,
350.049176012208));
#123600=CARTESIAN_POINT('Ctrl Pts',(-61.5241091075068,1076.34576283651,
349.985704802513));
#123601=CARTESIAN_POINT('Ctrl Pts',(-61.5513731195263,1076.34290888727,
349.951036121775));
#123602=CARTESIAN_POINT('Ctrl Pts',(-61.6233351775406,1076.33427925253,
349.838460636607));
#123603=CARTESIAN_POINT('Ctrl Pts',(-61.6561045403002,1076.32862479538,
349.754086858265));
#123604=CARTESIAN_POINT('Ctrl Pts',(-61.686605946541,1076.31834160321,349.578482398263));
#123605=CARTESIAN_POINT('Ctrl Pts',(-61.6844541768283,1076.31380158068,
349.489032894533));
#123606=CARTESIAN_POINT('Ctrl Pts',(-61.6457414101539,1076.30645221666,
349.316219681921));
#123607=CARTESIAN_POINT('Ctrl Pts',(-61.6096384270678,1076.30371138074,
349.234520008511));
#123608=CARTESIAN_POINT('Ctrl Pts',(-61.5080577167856,1076.30045505201,
349.089819711671));
#123609=CARTESIAN_POINT('Ctrl Pts',(-61.4436415274147,1076.2999669893,349.028192578388));
#123610=CARTESIAN_POINT('Ctrl Pts',(-61.2947930869919,1076.30133225723,
348.933252667705));
#123611=CARTESIAN_POINT('Ctrl Pts',(-61.2118340721429,1076.30317014007,
348.900848177727));
#123612=CARTESIAN_POINT('Ctrl Pts',(-61.0858364824871,1076.30733713304,
348.878287309241));
#123613=CARTESIAN_POINT('Ctrl Pts',(-61.0461204817631,1076.30883480827,
348.874750038688));
#123614=CARTESIAN_POINT('Ctrl Pts',(-61.0063319687469,1076.31051420464,
348.874728472955));
#123615=CARTESIAN_POINT('Ctrl Pts',(-61.0062099350874,1076.31051935545,
348.874728406812));
#123616=CARTESIAN_POINT('Ctrl Pts',(-61.0060879031079,1076.3105245079,348.874728374424));
#123617=CARTESIAN_POINT('Ctrl Pts',(-61.0059658728184,1076.31052966192,
348.874728374424));
#123618=CARTESIAN_POINT('',(-61.0059658728168,1082.7251047501,348.874728374424));
#123619=CARTESIAN_POINT('',(-61.0059658728168,1067.7251047501,348.874728374424));
#123620=CARTESIAN_POINT('Origin',(-61.0059658728168,1082.7251047501,349.55017249556));
#123621=CARTESIAN_POINT('Ctrl Pts',(-61.0059658728184,1076.31052966192,
348.874728374424));
#123622=CARTESIAN_POINT('Ctrl Pts',(-60.9176998992336,1076.31425762907,
348.874728374424));
#123623=CARTESIAN_POINT('Ctrl Pts',(-60.8303188655872,1076.31882699849,
348.892029359859));
#123624=CARTESIAN_POINT('Ctrl Pts',(-60.6668950091229,1076.3290905237,348.959330175153));
#123625=CARTESIAN_POINT('Ctrl Pts',(-60.5924665285989,1076.33468917506,
349.008807530495));
#123626=CARTESIAN_POINT('Ctrl Pts',(-60.498438361391,1076.34325793899,349.102305160194));
#123627=CARTESIAN_POINT('Ctrl Pts',(-60.470288271324,1076.3461174665,349.136386371444));
#123628=CARTESIAN_POINT('Ctrl Pts',(-60.3955131618802,1076.35470522712,
349.247458253658));
#123629=CARTESIAN_POINT('Ctrl Pts',(-60.3607078687554,1076.36024970119,
349.331224569256));
#123630=CARTESIAN_POINT('Ctrl Pts',(-60.3259345653945,1076.37028351035,
349.507381430532));
#123631=CARTESIAN_POINT('Ctrl Pts',(-60.3262625962687,1076.37467621228,
349.598017605762));
#123632=CARTESIAN_POINT('Ctrl Pts',(-60.3624093399875,1076.38177287548,
349.774140873562));
#123633=CARTESIAN_POINT('Ctrl Pts',(-60.3979554426796,1076.38440248887,
349.857840918896));
#123634=CARTESIAN_POINT('Ctrl Pts',(-60.4993860991622,1076.38754143813,
350.005778792616));
#123635=CARTESIAN_POINT('Ctrl Pts',(-60.5639999398497,1076.38803790272,
350.068697607441));
#123636=CARTESIAN_POINT('Ctrl Pts',(-60.7131856289696,1076.38685709905,
350.165246944526));
#123637=CARTESIAN_POINT('Ctrl Pts',(-60.7960814594361,1076.38521365448,
350.198230481894));
#123638=CARTESIAN_POINT('Ctrl Pts',(-60.9236336325516,1076.38136334764,
350.221855237295));
#123639=CARTESIAN_POINT('Ctrl Pts',(-60.9648103509532,1076.37993176433,
350.225616616696));
#123640=CARTESIAN_POINT('Ctrl Pts',(-61.0059658728168,1076.37831455598,
350.225616616696));
#123641=CARTESIAN_POINT('Origin',(-56.6885840720973,1067.7251047501,336.39044334969));
#123642=CARTESIAN_POINT('',(-56.6885840721218,1075.55714102284,335.291612213697));
#123643=CARTESIAN_POINT('',(-56.6885840720973,1067.7251047501,335.291612213697));
#123644=CARTESIAN_POINT('Ctrl Pts',(-56.6886635173097,1075.7496222582,337.48927448281));
#123645=CARTESIAN_POINT('Ctrl Pts',(-56.8344491670304,1075.74168330395,
337.489263942544));
#123646=CARTESIAN_POINT('Ctrl Pts',(-56.9786320037909,1075.73133837871,
337.460243990801));
#123647=CARTESIAN_POINT('Ctrl Pts',(-57.2475658978346,1075.70688580914,
337.347677049276));
#123648=CARTESIAN_POINT('Ctrl Pts',(-57.3695861217295,1075.69300350249,
337.265045372198));
#123649=CARTESIAN_POINT('Ctrl Pts',(-57.5749594347056,1075.66339060859,
337.056311688249));
#123650=CARTESIAN_POINT('Ctrl Pts',(-57.6559843038123,1075.64793365169,
336.931896070108));
#123651=CARTESIAN_POINT('Ctrl Pts',(-57.7639354792398,1075.61777360276,
336.65947572204));
#123652=CARTESIAN_POINT('Ctrl Pts',(-57.7901696681622,1075.60335669269,
336.514237357354));
#123653=CARTESIAN_POINT('Ctrl Pts',(-57.7842422704277,1075.57771444552,
336.223721630292));
#123654=CARTESIAN_POINT('Ctrl Pts',(-57.7528904562715,1075.56669838166,
336.081251353044));
#123655=CARTESIAN_POINT('Ctrl Pts',(-57.6370095854657,1075.5495764937,335.817234847899));
#123656=CARTESIAN_POINT('Ctrl Pts',(-57.5539600000379,1075.54361036534,
335.698153927165));
#123657=CARTESIAN_POINT('Ctrl Pts',(-57.3470413252792,1075.53761512669,
335.49917586878));
#123658=CARTESIAN_POINT('Ctrl Pts',(-57.2254514661288,1075.53761608331,
335.421063600339));
#123659=CARTESIAN_POINT('Ctrl Pts',(-56.95925442656,1075.54359724004,335.315904740578));
#123660=CARTESIAN_POINT('Ctrl Pts',(-56.8173162673525,1075.54951253567,
335.289869092651));
#123661=CARTESIAN_POINT('Ctrl Pts',(-56.5310162291635,1075.56646030936,
335.293544430829));
#123662=CARTESIAN_POINT('Ctrl Pts',(-56.3894500677497,1075.57734646249,
335.323461203079));
#123663=CARTESIAN_POINT('Ctrl Pts',(-56.1251606816273,1075.60261266604,
335.436110316585));
#123664=CARTESIAN_POINT('Ctrl Pts',(-56.0050879379537,1075.61677082831,
335.518104474796));
#123665=CARTESIAN_POINT('Ctrl Pts',(-55.853772697369,1075.63896636136,335.67230559026));
#123666=CARTESIAN_POINT('Ctrl Pts',(-55.8084513356478,1075.64648240489,
335.72863011673));
#123667=CARTESIAN_POINT('Ctrl Pts',(-55.7296691301273,1075.6614740001,335.849084447118));
#123668=CARTESIAN_POINT('Ctrl Pts',(-55.6963413169535,1075.66891505494,
335.912903460578));
#123669=CARTESIAN_POINT('Ctrl Pts',(-55.614934311832,1075.69102574124,336.114798853958));
#123670=CARTESIAN_POINT('Ctrl Pts',(-55.5878255203469,1075.70502787136,
336.259687746594));
#123671=CARTESIAN_POINT('Ctrl Pts',(-55.5918854306654,1075.72980139543,
336.551226849469));
#123672=CARTESIAN_POINT('Ctrl Pts',(-55.6227885558044,1075.74034514702,
336.695011167313));
#123673=CARTESIAN_POINT('Ctrl Pts',(-55.7391227224178,1075.75668550736,
336.962493602663));
#123674=CARTESIAN_POINT('Ctrl Pts',(-55.8234249357666,1075.76231514086,
337.083461673728));
#123675=CARTESIAN_POINT('Ctrl Pts',(-56.0346902733854,1075.76790695523,
337.285567862994));
#123676=CARTESIAN_POINT('Ctrl Pts',(-56.1595183826974,1075.7678056593,337.364565226893));
#123677=CARTESIAN_POINT('Ctrl Pts',(-56.4215339292318,1075.76206186809,
337.464750987201));
#123678=CARTESIAN_POINT('Ctrl Pts',(-56.554578478896,1075.75692403987,337.489284177124));
#123679=CARTESIAN_POINT('Ctrl Pts',(-56.6886635173097,1075.7496222582,337.48927448281));
#123680=CARTESIAN_POINT('Origin',(-56.6885840720973,1067.7251047501,336.39044334969));
#123681=CARTESIAN_POINT('',(-56.6885840720973,1075.69877322724,336.889274485682));
#123682=CARTESIAN_POINT('',(-56.6885840720972,1075.61138997104,335.891612213697));
#123683=CARTESIAN_POINT('Ctrl Pts',(-56.6885840720972,1075.69877322723,
336.889274485682));
#123684=CARTESIAN_POINT('Ctrl Pts',(-56.6894491464213,1075.69872525547,
336.889274485682));
#123685=CARTESIAN_POINT('Ctrl Pts',(-56.6903143202152,1075.69867708276,
336.889272235361));
#123686=CARTESIAN_POINT('Ctrl Pts',(-56.7576970253416,1075.69490999697,
336.888921625651));
#123687=CARTESIAN_POINT('Ctrl Pts',(-56.8234066897673,1075.69008096533,
336.875275915875));
#123688=CARTESIAN_POINT('Ctrl Pts',(-56.9456757698671,1075.67873876071,
336.82307097793));
#123689=CARTESIAN_POINT('Ctrl Pts',(-57.0009960109743,1075.67233343206,
336.78496672716));
#123690=CARTESIAN_POINT('Ctrl Pts',(-57.0935839815181,1075.65878126756,
336.689209466401));
#123691=CARTESIAN_POINT('Ctrl Pts',(-57.1298751391389,1075.65176327744,
336.632409856439));
#123692=CARTESIAN_POINT('Ctrl Pts',(-57.178022099384,1075.63808674825,336.507744699949));
#123693=CARTESIAN_POINT('Ctrl Pts',(-57.189342428336,1075.63156314422,336.44106872803));
#123694=CARTESIAN_POINT('Ctrl Pts',(-57.1850034196467,1075.62010134744,
336.308688392635));
#123695=CARTESIAN_POINT('Ctrl Pts',(-57.1700042031795,1075.61524035459,
336.244265817626));
#123696=CARTESIAN_POINT('Ctrl Pts',(-57.1160293855711,1075.60773979562,
336.125167635418));
#123697=CARTESIAN_POINT('Ctrl Pts',(-57.0777297314247,1075.60516108071,
336.071604451795));
#123698=CARTESIAN_POINT('Ctrl Pts',(-56.9828002514258,1075.60264920655,
335.982407647644));
#123699=CARTESIAN_POINT('Ctrl Pts',(-56.9271946859133,1075.60273012714,
335.947587982151));
#123700=CARTESIAN_POINT('Ctrl Pts',(-56.8096376474247,1075.6054603161,335.902713493885));
#123701=CARTESIAN_POINT('Ctrl Pts',(-56.7493441376742,1075.60792128284,
335.891612213697));
#123702=CARTESIAN_POINT('Ctrl Pts',(-56.6885840720971,1075.61138997104,
335.891612213697));
#123703=CARTESIAN_POINT('',(-56.6885840720973,1082.7251047501,335.891612213697));
#123704=CARTESIAN_POINT('',(-56.6885840720973,1067.7251047501,335.891612213697));
#123705=CARTESIAN_POINT('Origin',(-56.6885840720973,1082.7251047501,336.39044334969));
#123706=CARTESIAN_POINT('Ctrl Pts',(-56.6885840720971,1075.61138997104,
335.891612213697));
#123707=CARTESIAN_POINT('Ctrl Pts',(-56.6884990384235,1075.61139482547,
335.891612213697));
#123708=CARTESIAN_POINT('Ctrl Pts',(-56.6884140038361,1075.61139968187,
335.891612235446));
#123709=CARTESIAN_POINT('Ctrl Pts',(-56.6883289683429,1075.61140454024,
335.891612278933));
#123710=CARTESIAN_POINT('Ctrl Pts',(-56.6231385591007,1075.61512909418,
335.891645617508));
#123711=CARTESIAN_POINT('Ctrl Pts',(-56.5586528662546,1075.61994219145,
335.904456408237));
#123712=CARTESIAN_POINT('Ctrl Pts',(-56.4379784929127,1075.63119943098,
335.95419283561));
#123713=CARTESIAN_POINT('Ctrl Pts',(-56.3830001270856,1075.63754486953,
335.990788440737));
#123714=CARTESIAN_POINT('Ctrl Pts',(-56.3135139750078,1075.64755079746,
336.059955081574));
#123715=CARTESIAN_POINT('Ctrl Pts',(-56.292680101939,1075.65094353892,336.085222649743));
#123716=CARTESIAN_POINT('Ctrl Pts',(-56.2562895994222,1075.65774040457,
336.139411092992));
#123717=CARTESIAN_POINT('Ctrl Pts',(-56.2408071720882,1075.6611288352,336.168200308803));
#123718=CARTESIAN_POINT('Ctrl Pts',(-56.202639353073,1075.67125571532,336.259641747662));
#123719=CARTESIAN_POINT('Ctrl Pts',(-56.1895345233825,1075.67772119746,
336.325533686445));
#123720=CARTESIAN_POINT('Ctrl Pts',(-56.1899762510962,1075.68923225219,
336.458485848432));
#123721=CARTESIAN_POINT('Ctrl Pts',(-56.2034468466609,1075.69416854804,
336.524230057133));
#123722=CARTESIAN_POINT('Ctrl Pts',(-56.2551726678914,1075.70181310519,
336.646013731805));
#123723=CARTESIAN_POINT('Ctrl Pts',(-56.2926424310386,1075.70446900306,
336.700933185089));
#123724=CARTESIAN_POINT('Ctrl Pts',(-56.3862038139609,1075.70717419258,
336.792468298214));
#123725=CARTESIAN_POINT('Ctrl Pts',(-56.4411098868677,1075.7072312694,336.828409888256));
#123726=CARTESIAN_POINT('Ctrl Pts',(-56.560888664013,1075.70478130846,336.876910908503));
#123727=CARTESIAN_POINT('Ctrl Pts',(-56.6244631064969,1075.70232898642,
336.889274485682));
#123728=CARTESIAN_POINT('Ctrl Pts',(-56.6885840720972,1075.69877322723,
336.889274485682));
#123729=CARTESIAN_POINT('Origin',(-49.705085901968,1067.7251047501,324.271668315149));
#123730=CARTESIAN_POINT('',(-49.7050859019928,1074.6677741402,323.181127566421));
#123731=CARTESIAN_POINT('',(-49.705085901968,1067.7251047501,323.18112756642));
#123732=CARTESIAN_POINT('Ctrl Pts',(-49.7045317577611,1074.93240199134,
325.362208923087));
#123733=CARTESIAN_POINT('Ctrl Pts',(-49.8493940963802,1074.92389728949,
325.362282533024));
#123734=CARTESIAN_POINT('Ctrl Pts',(-49.9925804253556,1074.91204851772,
325.333496298155));
#123735=CARTESIAN_POINT('Ctrl Pts',(-50.2596848576552,1074.88292013809,
325.221803446226));
#123736=CARTESIAN_POINT('Ctrl Pts',(-50.3808423955098,1074.86590266617,
325.139751063587));
#123737=CARTESIAN_POINT('Ctrl Pts',(-50.532177739072,1074.83836158758,324.985984200759));
#123738=CARTESIAN_POINT('Ctrl Pts',(-50.5769308665596,1074.82900398012,
324.930611673339));
#123739=CARTESIAN_POINT('Ctrl Pts',(-50.6551767204814,1074.80993652455,
324.811752310003));
#123740=CARTESIAN_POINT('Ctrl Pts',(-50.6884446502032,1074.80026814903,
324.748498673531));
#123741=CARTESIAN_POINT('Ctrl Pts',(-50.7705871361969,1074.77076949046,
324.546494173401));
#123742=CARTESIAN_POINT('Ctrl Pts',(-50.7979071668757,1074.75129755642,
324.400644472631));
#123743=CARTESIAN_POINT('Ctrl Pts',(-50.7931038296754,1074.71593933622,
324.110008868538));
#123744=CARTESIAN_POINT('Ctrl Pts',(-50.762366670685,1074.70031598856,323.968007650524));
#123745=CARTESIAN_POINT('Ctrl Pts',(-50.6477606925917,1074.67485058289,
323.705101200891));
#123746=CARTESIAN_POINT('Ctrl Pts',(-50.5655508166102,1074.66520380374,
323.586574474836));
#123747=CARTESIAN_POINT('Ctrl Pts',(-50.3606452792527,1074.65324773146,
323.388709663174));
#123748=CARTESIAN_POINT('Ctrl Pts',(-50.2404042163707,1074.65099377426,
323.311022651359));
#123749=CARTESIAN_POINT('Ctrl Pts',(-49.9771820655242,1074.65416583854,
323.206185028552));
#123750=CARTESIAN_POINT('Ctrl Pts',(-49.8369519245457,1074.65953702178,
323.179958494126));
#123751=CARTESIAN_POINT('Ctrl Pts',(-49.5537773989021,1074.67721516714,
323.182383161852));
#123752=CARTESIAN_POINT('Ctrl Pts',(-49.4136533650652,1074.68938063811,
323.211304456397));
#123753=CARTESIAN_POINT('Ctrl Pts',(-49.1513265559742,1074.71895400281,
323.321368276287));
#123754=CARTESIAN_POINT('Ctrl Pts',(-49.0318440509625,1074.73612774369,
323.401983991196));
#123755=CARTESIAN_POINT('Ctrl Pts',(-48.8807642619317,1074.76387098562,
323.554082316392));
#123756=CARTESIAN_POINT('Ctrl Pts',(-48.8353309354415,1074.77342371778,
323.609886543423));
#123757=CARTESIAN_POINT('Ctrl Pts',(-48.7562044287484,1074.79274070763,
323.729424328376));
#123758=CARTESIAN_POINT('Ctrl Pts',(-48.7226624192436,1074.80246079913,
323.792869135357));
#123759=CARTESIAN_POINT('Ctrl Pts',(-48.6406171815644,1074.83170117203,
323.993644130364));
#123760=CARTESIAN_POINT('Ctrl Pts',(-48.6130333909722,1074.85073155292,
324.137910845684));
#123761=CARTESIAN_POINT('Ctrl Pts',(-48.6161728279485,1074.88534490407,
324.427938350528));
#123762=CARTESIAN_POINT('Ctrl Pts',(-48.6464318479754,1074.90062277419,
324.57090020764));
#123763=CARTESIAN_POINT('Ctrl Pts',(-48.7611674737408,1074.92549253054,
324.836623993457));
#123764=CARTESIAN_POINT('Ctrl Pts',(-48.8443224720443,1074.93485329814,
324.95676596895));
#123765=CARTESIAN_POINT('Ctrl Pts',(-49.0518694102871,1074.94634854687,
325.156597439565));
#123766=CARTESIAN_POINT('Ctrl Pts',(-49.1736447811957,1074.94844781702,
325.234679494678));
#123767=CARTESIAN_POINT('Ctrl Pts',(-49.4338131682571,1074.94526662733,
325.336665715075));
#123768=CARTESIAN_POINT('Ctrl Pts',(-49.5686259828435,1074.9403808636,325.362139864312));
#123769=CARTESIAN_POINT('Ctrl Pts',(-49.7045317577611,1074.93240199134,
325.362208923086));
#123770=CARTESIAN_POINT('Origin',(-49.705085901968,1067.7251047501,324.271668315149));
#123771=CARTESIAN_POINT('',(-49.705085901968,1074.86129916363,324.762209063877));
#123772=CARTESIAN_POINT('',(-49.7050859019679,1074.74227702453,323.78112756642));
#123773=CARTESIAN_POINT('Ctrl Pts',(-49.705085901968,1074.86129916363,324.762209063877));
#123774=CARTESIAN_POINT('Ctrl Pts',(-49.7055456137983,1074.86127180977,
324.762209063877));
#123775=CARTESIAN_POINT('Ctrl Pts',(-49.7060053538754,1074.8612443764,324.762208417647));
#123776=CARTESIAN_POINT('Ctrl Pts',(-49.7704871387181,1074.8573857354,324.762027118034));
#123777=CARTESIAN_POINT('Ctrl Pts',(-49.8337492093071,1074.85209112191,
324.749317746845));
#123778=CARTESIAN_POINT('Ctrl Pts',(-49.95328548125,1074.83899921727,324.699832482791));
#123779=CARTESIAN_POINT('Ctrl Pts',(-50.0081234310176,1074.83126901174,
324.662911112905));
#123780=CARTESIAN_POINT('Ctrl Pts',(-50.076586183687,1074.81878982457,324.593608006074));
#123781=CARTESIAN_POINT('Ctrl Pts',(-50.0968144814737,1074.8145579582,324.568661180176));
#123782=CARTESIAN_POINT('Ctrl Pts',(-50.132148608211,1074.80595291254,324.515139825244));
#123783=CARTESIAN_POINT('Ctrl Pts',(-50.1471626873319,1074.80159876538,
324.486677142847));
#123784=CARTESIAN_POINT('Ctrl Pts',(-50.1841533638763,1074.78836440411,
324.395999925204));
#123785=CARTESIAN_POINT('Ctrl Pts',(-50.1965174791759,1074.77966095661,
324.330606792812));
#123786=CARTESIAN_POINT('Ctrl Pts',(-50.1946492706973,1074.76380931707,
324.199665063864));
#123787=CARTESIAN_POINT('Ctrl Pts',(-50.1808066576286,1074.75679257532,
324.135380605636));
#123788=CARTESIAN_POINT('Ctrl Pts',(-50.1291047977023,1074.74542206639,
324.016815791196));
#123789=CARTESIAN_POINT('Ctrl Pts',(-50.0921597962372,1074.74113726211,
323.963546121838));
#123790=CARTESIAN_POINT('Ctrl Pts',(-50.0000569991088,1074.73582341612,
323.87457009062));
#123791=CARTESIAN_POINT('Ctrl Pts',(-49.945987103598,1074.73482100748,323.839617587412));
#123792=CARTESIAN_POINT('Ctrl Pts',(-49.8288825190181,1074.7362099424,323.792939821709));
#123793=CARTESIAN_POINT('Ctrl Pts',(-49.7672384927223,1074.73850603265,
323.78112756642));
#123794=CARTESIAN_POINT('Ctrl Pts',(-49.7050859019678,1074.74227702453,
323.78112756642));
#123795=CARTESIAN_POINT('',(-49.705085901968,1082.7251047501,323.78112756642));
#123796=CARTESIAN_POINT('',(-49.705085901968,1067.7251047501,323.78112756642));
#123797=CARTESIAN_POINT('Origin',(-49.705085901968,1082.7251047501,324.271668315149));
#123798=CARTESIAN_POINT('Ctrl Pts',(-49.7050859019678,1074.74227702453,
323.78112756642));
#123799=CARTESIAN_POINT('Ctrl Pts',(-49.7050040619518,1074.74228199002,
323.78112756642));
#123800=CARTESIAN_POINT('Ctrl Pts',(-49.7049222210541,1074.74228695807,
323.781127586905));
#123801=CARTESIAN_POINT('Ctrl Pts',(-49.704840379282,1074.74229192867,323.781127627868));
#123802=CARTESIAN_POINT('Ctrl Pts',(-49.6409234603641,1074.74617387742,
323.781159619205));
#123803=CARTESIAN_POINT('Ctrl Pts',(-49.5777366215018,1074.75153806376,
323.793681432173));
#123804=CARTESIAN_POINT('Ctrl Pts',(-49.4592687194716,1074.7646501543,323.842313969592));
#123805=CARTESIAN_POINT('Ctrl Pts',(-49.405216469586,1074.77229422411,323.878188920965));
#123806=CARTESIAN_POINT('Ctrl Pts',(-49.3367866694145,1074.78468339727,
323.946056024522));
#123807=CARTESIAN_POINT('Ctrl Pts',(-49.3162152533231,1074.7889476124,323.970926284283));
#123808=CARTESIAN_POINT('Ctrl Pts',(-49.2802643853385,1074.79759568054,
324.024299075212));
#123809=CARTESIAN_POINT('Ctrl Pts',(-49.2649627538341,1074.80195995729,
324.05267901216));
#123810=CARTESIAN_POINT('Ctrl Pts',(-49.2272555687101,1074.81515184372,
324.142812399));
#123811=CARTESIAN_POINT('Ctrl Pts',(-49.2143109374341,1074.82378669253,
324.207788204707));
#123812=CARTESIAN_POINT('Ctrl Pts',(-49.2147844903059,1074.83956781397,
324.338738520539));
#123813=CARTESIAN_POINT('Ctrl Pts',(-49.2280561837372,1074.84657003657,
324.403442530516));
#123814=CARTESIAN_POINT('Ctrl Pts',(-49.2789933276834,1074.85793777556,
324.523158854203));
#123815=CARTESIAN_POINT('Ctrl Pts',(-49.3158103692566,1074.86222611825,
324.577103343054));
#123816=CARTESIAN_POINT('Ctrl Pts',(-49.4076961864532,1074.867549275,324.66695634815));
#123817=CARTESIAN_POINT('Ctrl Pts',(-49.4615405481388,1074.86858127356,
324.702232199905));
#123818=CARTESIAN_POINT('Ctrl Pts',(-49.579287383854,1074.86731575151,324.750008315291));
#123819=CARTESIAN_POINT('Ctrl Pts',(-49.641919981638,1074.86505767464,324.762209063877));
#123820=CARTESIAN_POINT('Ctrl Pts',(-49.705085901968,1074.86129916363,324.762209063877));
#123821=CARTESIAN_POINT('Origin',(-75.4882582191906,1067.7251047501,376.431040472272));
#123822=CARTESIAN_POINT('',(-75.4882582192121,1076.65013582838,374.952737340079));
#123823=CARTESIAN_POINT('',(-75.4882582191906,1067.7251047501,374.952737340079));
#123824=CARTESIAN_POINT('Ctrl Pts',(-75.4874144218056,1076.69163799014,
377.909343363651));
#123825=CARTESIAN_POINT('Ctrl Pts',(-75.6827415468976,1076.68805926486,
377.909454854008));
#123826=CARTESIAN_POINT('Ctrl Pts',(-75.8761542728031,1076.68382657079,
377.870852981114));
#123827=CARTESIAN_POINT('Ctrl Pts',(-76.1450544222639,1076.67673305976,
377.758899442763));
#123828=CARTESIAN_POINT('Ctrl Pts',(-76.2298494272729,1076.67428790979,
377.71347265165));
#123829=CARTESIAN_POINT('Ctrl Pts',(-76.4725288914479,1076.66662134139,
377.551296525591));
#123830=CARTESIAN_POINT('Ctrl Pts',(-76.6121646848941,1076.66122864575,
377.411140205371));
#123831=CARTESIAN_POINT('Ctrl Pts',(-76.8276270320169,1076.65079155497,
377.086116262237));
#123832=CARTESIAN_POINT('Ctrl Pts',(-76.9019628475037,1076.64585154935,
376.904834607344));
#123833=CARTESIAN_POINT('Ctrl Pts',(-76.976343040882,1076.63736503469,376.523937251217));
#123834=CARTESIAN_POINT('Ctrl Pts',(-76.9756806703523,1076.63390778129,
376.328021630331));
#123835=CARTESIAN_POINT('Ctrl Pts',(-76.8987620580907,1076.62926059287,
375.947933113412));
#123836=CARTESIAN_POINT('Ctrl Pts',(-76.8233781015899,1076.62811659682,
375.767433720505));
#123837=CARTESIAN_POINT('Ctrl Pts',(-76.6075137538433,1076.62842293834,
375.446144237223));
#123838=CARTESIAN_POINT('Ctrl Pts',(-76.4692692472796,1076.62986423688,
375.308380913045));
#123839=CARTESIAN_POINT('Ctrl Pts',(-76.1477920876477,1076.63502127057,
375.0939982024));
#123840=CARTESIAN_POINT('Ctrl Pts',(-75.9677090415123,1076.63867986198,
375.019381249661));
#123841=CARTESIAN_POINT('Ctrl Pts',(-75.5889785768878,1076.64744328673,
374.943575341487));
#123842=CARTESIAN_POINT('Ctrl Pts',(-75.393962310733,1076.65245758771,374.943156778212));
#123843=CARTESIAN_POINT('Ctrl Pts',(-75.0146544172071,1076.66287850511,
375.017371038021));
#123844=CARTESIAN_POINT('Ctrl Pts',(-74.8340193331443,1076.66817983416,
375.091363129787));
#123845=CARTESIAN_POINT('Ctrl Pts',(-74.5092349614717,1076.67829380086,
375.306172695358));
#123846=CARTESIAN_POINT('Ctrl Pts',(-74.3688437965922,1076.68299767023,
375.445782028953));
#123847=CARTESIAN_POINT('Ctrl Pts',(-74.1514358922739,1076.6911867403,375.770570104066));
#123848=CARTESIAN_POINT('Ctrl Pts',(-74.0761343683581,1076.6946052898,375.952260659721));
#123849=CARTESIAN_POINT('Ctrl Pts',(-74.0001947561923,1076.70006327117,
376.33498595089));
#123850=CARTESIAN_POINT('Ctrl Pts',(-74.0005382583571,1076.70205315722,
376.53230337495));
#123851=CARTESIAN_POINT('Ctrl Pts',(-74.0781654507825,1076.70465848027,
376.916465918374));
#123852=CARTESIAN_POINT('Ctrl Pts',(-74.155111593748,1076.70524644866,377.099412513354));
#123853=CARTESIAN_POINT('Ctrl Pts',(-74.3759678646567,1076.70504468597,
377.424402041657));
#123854=CARTESIAN_POINT('Ctrl Pts',(-74.5176392126666,1076.70425718784,
377.56323022199));
#123855=CARTESIAN_POINT('Ctrl Pts',(-74.8459572862212,1076.70124211397,
377.776755326571));
#123856=CARTESIAN_POINT('Ctrl Pts',(-75.0290990036184,1076.69904580999,
377.849724978353));
#123857=CARTESIAN_POINT('Ctrl Pts',(-75.3089626614887,1076.69476517686,
377.90114657676));
#123858=CARTESIAN_POINT('Ctrl Pts',(-75.398095676438,1076.69327446153,377.909292381593));
#123859=CARTESIAN_POINT('Ctrl Pts',(-75.4874144218056,1076.69163799014,
377.909343363651));
#123860=CARTESIAN_POINT('Origin',(-75.4882582191906,1067.7251047501,376.431040472272));
#123861=CARTESIAN_POINT('',(-75.4882582191906,1076.68449717364,377.309343604465));
#123862=CARTESIAN_POINT('',(-75.4882582226568,1076.65987181757,375.552737340079));
#123863=CARTESIAN_POINT('Ctrl Pts',(-75.4882582191906,1076.68449717364,
377.309343604465));
#123864=CARTESIAN_POINT('Ctrl Pts',(-75.4897648571436,1076.68446733747,
377.309343604465));
#123865=CARTESIAN_POINT('Ctrl Pts',(-75.4912716819592,1076.68443743529,
377.309339727744));
#123866=CARTESIAN_POINT('Ctrl Pts',(-75.6093360531358,1076.68208961198,
377.308732064741));
#123867=CARTESIAN_POINT('Ctrl Pts',(-75.7246094171306,1076.67942037264,
377.284935973877));
#123868=CARTESIAN_POINT('Ctrl Pts',(-75.8844460862234,1076.67509031527,
377.216989422195));
#123869=CARTESIAN_POINT('Ctrl Pts',(-75.9347184963435,1076.67361999382,
377.189561131168));
#123870=CARTESIAN_POINT('Ctrl Pts',(-76.0782280956566,1076.66907587537,
377.09202303258));
#123871=CARTESIAN_POINT('Ctrl Pts',(-76.1605302317935,1076.66596277885,
377.008113398505));
#123872=CARTESIAN_POINT('Ctrl Pts',(-76.2869658349762,1076.66005765652,
376.814116483053));
#123873=CARTESIAN_POINT('Ctrl Pts',(-76.3302664836154,1076.65732189573,
376.706188177514));
#123874=CARTESIAN_POINT('Ctrl Pts',(-76.3727349171275,1076.65268004244,
376.479798994131));
#123875=CARTESIAN_POINT('Ctrl Pts',(-76.3715039989058,1076.65082128705,
376.363534746148));
#123876=CARTESIAN_POINT('Ctrl Pts',(-76.3242646963916,1076.64834691408,
376.138216821916));
#123877=CARTESIAN_POINT('Ctrl Pts',(-76.2787611106823,1076.64775567246,
376.031341632903));
#123878=CARTESIAN_POINT('Ctrl Pts',(-76.1492160697001,1076.64796899716,
375.841331760484));
#123879=CARTESIAN_POINT('Ctrl Pts',(-76.0664771514959,1076.64876963235,
375.760009501673));
#123880=CARTESIAN_POINT('Ctrl Pts',(-75.8744368915971,1076.65161652036,
375.633874306666));
#123881=CARTESIAN_POINT('Ctrl Pts',(-75.7670035037809,1076.65363282658,
375.590263956964));
#123882=CARTESIAN_POINT('Ctrl Pts',(-75.5994049531778,1076.65725865743,
375.558010997993));
#123883=CARTESIAN_POINT('Ctrl Pts',(-75.5438273738724,1076.65853347143,
375.552737340517));
#123884=CARTESIAN_POINT('Ctrl Pts',(-75.488258226123,1076.65987181757,375.552737340079));
#123885=CARTESIAN_POINT('',(-75.4882582191906,1082.7251047501,375.552737340079));
#123886=CARTESIAN_POINT('',(-75.4882582191906,1067.7251047501,375.552737340079));
#123887=CARTESIAN_POINT('Origin',(-75.4882582191906,1082.7251047501,376.431040472272));
#123888=CARTESIAN_POINT('Ctrl Pts',(-75.488258226123,1076.65987181757,375.552737340079));
#123889=CARTESIAN_POINT('Ctrl Pts',(-75.4294792692097,1076.66128746984,
375.552737339615));
#123890=CARTESIAN_POINT('Ctrl Pts',(-75.3707097446567,1076.66277414839,
375.558637895176));
#123891=CARTESIAN_POINT('Ctrl Pts',(-75.2002026530587,1076.66728030078,
375.593391578033));
#123892=CARTESIAN_POINT('Ctrl Pts',(-75.0931566296768,1076.67035816284,
375.638243891762));
#123893=CARTESIAN_POINT('Ctrl Pts',(-74.9009299959585,1076.67636918568,
375.767643214141));
#123894=CARTESIAN_POINT('Ctrl Pts',(-74.8180309293281,1076.67923939418,
375.851516328865));
#123895=CARTESIAN_POINT('Ctrl Pts',(-74.6900978634223,1076.68436902491,
376.046457031318));
#123896=CARTESIAN_POINT('Ctrl Pts',(-74.6462082735092,1076.68658173662,
376.15550562242));
#123897=CARTESIAN_POINT('Ctrl Pts',(-74.615791802267,1076.6891393847,376.318519839637));
#123898=CARTESIAN_POINT('Ctrl Pts',(-74.6108434045295,1076.68982209035,
376.367779090221));
#123899=CARTESIAN_POINT('Ctrl Pts',(-74.6100642504227,1076.69042296099,
376.417193261711));
#123900=CARTESIAN_POINT('Ctrl Pts',(-74.6082205493547,1076.69184479247,
376.534121299387));
#123901=CARTESIAN_POINT('Ctrl Pts',(-74.629748032955,1076.69279098358,376.650252553386));
#123902=CARTESIAN_POINT('Ctrl Pts',(-74.7171221748697,1076.69371338343,
376.867510329167));
#123903=CARTESIAN_POINT('Ctrl Pts',(-74.7821919157866,1076.69367926517,
376.966416082538));
#123904=CARTESIAN_POINT('Ctrl Pts',(-74.9470930001565,1076.6926210733,377.132628559757));
#123905=CARTESIAN_POINT('Ctrl Pts',(-75.0451835742738,1076.69160880458,
377.198353097151));
#123906=CARTESIAN_POINT('Ctrl Pts',(-75.2595179757525,1076.68866392777,
377.286791042517));
#123907=CARTESIAN_POINT('Ctrl Pts',(-75.3733445800223,1076.68677282525,
377.309343604465));
#123908=CARTESIAN_POINT('Ctrl Pts',(-75.4882582191906,1076.68449717364,
377.309343604465));
#123909=CARTESIAN_POINT('Origin',(-75.2807843499774,1067.7251047501,363.874487154571));
#123910=CARTESIAN_POINT('',(-75.2807843499963,1076.29141677771,362.599043033435));
#123911=CARTESIAN_POINT('',(-75.2807843499774,1067.7251047501,362.599043033435));
#123912=CARTESIAN_POINT('Ctrl Pts',(-75.2808749340257,1076.39500999161,
365.149931272491));
#123913=CARTESIAN_POINT('Ctrl Pts',(-75.4498210414911,1076.38698060872,
365.149919273672));
#123914=CARTESIAN_POINT('Ctrl Pts',(-75.6170307065239,1076.3776224465,365.116340771465));
#123915=CARTESIAN_POINT('Ctrl Pts',(-75.8492390085435,1076.36237274116,
365.019250115279));
#123916=CARTESIAN_POINT('Ctrl Pts',(-75.9223784283126,1076.35717939432,
364.979917908772));
#123917=CARTESIAN_POINT('Ctrl Pts',(-76.061238436746,1076.34648830333,364.886793904917));
#123918=CARTESIAN_POINT('Ctrl Pts',(-76.1264620246764,1076.34101262697,
364.832976554995));
#123919=CARTESIAN_POINT('Ctrl Pts',(-76.3039794736953,1076.32465583089,
364.654179688324));
#123920=CARTESIAN_POINT('Ctrl Pts',(-76.3974933459678,1076.31392645234,
364.513102161657));
#123921=CARTESIAN_POINT('Ctrl Pts',(-76.5245527179282,1076.29413631785,
364.202917882855));
#123922=CARTESIAN_POINT('Ctrl Pts',(-76.5569187050774,1076.28526892554,
364.036817935459));
#123923=CARTESIAN_POINT('Ctrl Pts',(-76.5555176995462,1076.270828232,363.701911407914));
#123924=CARTESIAN_POINT('Ctrl Pts',(-76.5219309210856,1076.26539150449,
363.536371154417));
#123925=CARTESIAN_POINT('Ctrl Pts',(-76.3929024521023,1076.25887218167,
363.228135518878));
#123926=CARTESIAN_POINT('Ctrl Pts',(-76.2989352653415,1076.25784107666,
363.088386334433));
#123927=CARTESIAN_POINT('Ctrl Pts',(-76.0627598804327,1076.26037567887,
362.853220905376));
#123928=CARTESIAN_POINT('Ctrl Pts',(-75.9229653443812,1076.26390607121,
362.760015899581));
#123929=CARTESIAN_POINT('Ctrl Pts',(-75.6154483973887,1076.27498166654,
362.632519442779));
#123930=CARTESIAN_POINT('Ctrl Pts',(-75.4506912723202,1076.2824186827,362.59950854281));
#123931=CARTESIAN_POINT('Ctrl Pts',(-75.1174768044228,1076.30006499764,
362.598586018667));
#123932=CARTESIAN_POINT('Ctrl Pts',(-74.9522100684297,1076.31010806948,
362.630863635212));
#123933=CARTESIAN_POINT('Ctrl Pts',(-74.7206134221463,1076.32600344859,
362.725602622322));
#123934=CARTESIAN_POINT('Ctrl Pts',(-74.6466383907175,1076.33140704741,
362.764719246028));
#123935=CARTESIAN_POINT('Ctrl Pts',(-74.5073775810664,1076.34225027004,
362.856856148271));
#123936=CARTESIAN_POINT('Ctrl Pts',(-74.4424252380534,1076.34766414583,
362.909662853596));
#123937=CARTESIAN_POINT('Ctrl Pts',(-74.2627876179995,1076.3637936282,363.087642402728));
#123938=CARTESIAN_POINT('Ctrl Pts',(-74.1673821801803,1076.37407487544,
363.22965523587));
#123939=CARTESIAN_POINT('Ctrl Pts',(-74.0379745778915,1076.39245960072,
363.541926165913));
#123940=CARTESIAN_POINT('Ctrl Pts',(-74.0049244006597,1076.4003979401,363.708969289003));
#123941=CARTESIAN_POINT('Ctrl Pts',(-74.0057646263549,1076.41311637904,
364.046622539015));
#123942=CARTESIAN_POINT('Ctrl Pts',(-74.0397555211792,1076.41776996181,
364.213875922484));
#123943=CARTESIAN_POINT('Ctrl Pts',(-74.1712035330894,1076.42330258773,
364.525888642469));
#123944=CARTESIAN_POINT('Ctrl Pts',(-74.2675100910345,1076.42411854434,
364.667440380937));
#123945=CARTESIAN_POINT('Ctrl Pts',(-74.5096750297681,1076.42178479807,
364.904445368011));
#123946=CARTESIAN_POINT('Ctrl Pts',(-74.6530304154158,1076.41866250436,
364.997575027204));
#123947=CARTESIAN_POINT('Ctrl Pts',(-74.9601457853265,1076.40897481434,
365.119446518862));
#123948=CARTESIAN_POINT('Ctrl Pts',(-75.1198146387644,1076.40266459105,
365.149942711246));
#123949=CARTESIAN_POINT('Ctrl Pts',(-75.2808749340257,1076.39500999161,
365.149931272491));
#123950=CARTESIAN_POINT('Origin',(-75.2807843499774,1067.7251047501,363.874487154571));
#123951=CARTESIAN_POINT('',(-75.2807843499774,1076.3720597734,364.549931275707));
#123952=CARTESIAN_POINT('',(-75.2807843499778,1076.31720630032,363.199043033435));
#123953=CARTESIAN_POINT('Ctrl Pts',(-75.2807843499774,1076.3720597734,364.549931275707));
#123954=CARTESIAN_POINT('Ctrl Pts',(-75.2877215036647,1076.3717209374,364.549931275707));
#123955=CARTESIAN_POINT('Ctrl Pts',(-75.2946629386578,1076.37137748182,
364.549824404112));
#123956=CARTESIAN_POINT('Ctrl Pts',(-75.3914829118915,1076.366525004,364.546838321674));
#123957=CARTESIAN_POINT('Ctrl Pts',(-75.4798767778265,1076.36134974017,
364.526148301032));
#123958=CARTESIAN_POINT('Ctrl Pts',(-75.6016450178768,1076.35305791868,
364.470483346753));
#123959=CARTESIAN_POINT('Ctrl Pts',(-75.6397969140367,1076.3502576311,364.448309786551));
#123960=CARTESIAN_POINT('Ctrl Pts',(-75.711775200249,1076.34454471581,364.396472028127));
#123961=CARTESIAN_POINT('Ctrl Pts',(-75.7453531963788,1076.34164487273,
364.366825559236));
#123962=CARTESIAN_POINT('Ctrl Pts',(-75.836106514004,1076.33305189152,364.269086326673));
#123963=CARTESIAN_POINT('Ctrl Pts',(-75.8830807748402,1076.3275018733,364.192822000742));
#123964=CARTESIAN_POINT('Ctrl Pts',(-75.9448261000479,1076.3174107107,364.026563492133));
#123965=CARTESIAN_POINT('Ctrl Pts',(-75.9590418127969,1076.31296668752,
363.938187175942));
#123966=CARTESIAN_POINT('Ctrl Pts',(-75.9525027664394,1076.30585423698,
363.761146251404));
#123967=CARTESIAN_POINT('Ctrl Pts',(-75.9318978026455,1076.30325185463,
363.674204671663));
#123968=CARTESIAN_POINT('Ctrl Pts',(-75.8583863822407,1076.30029495885,
363.513380867354));
#123969=CARTESIAN_POINT('Ctrl Pts',(-75.8062816866164,1076.2999643101,363.441040688944));
#123970=CARTESIAN_POINT('Ctrl Pts',(-75.6772478077877,1076.30163836959,
363.320569784331));
#123971=CARTESIAN_POINT('Ctrl Pts',(-75.6016066419786,1076.30362398676,
363.273593808685));
#123972=CARTESIAN_POINT('Ctrl Pts',(-75.4429036913969,1076.30940021779,
363.213749865197));
#123973=CARTESIAN_POINT('Ctrl Pts',(-75.3621640822628,1076.3129924975,363.199043538177));
#123974=CARTESIAN_POINT('Ctrl Pts',(-75.2807885393945,1076.3172060834,363.199043033448));
#123975=CARTESIAN_POINT('',(-75.2807843499774,1082.7251047501,363.199043033435));
#123976=CARTESIAN_POINT('',(-75.2807843499774,1067.7251047501,363.199043033435));
#123977=CARTESIAN_POINT('Origin',(-75.2807843499774,1082.7251047501,363.874487154571));
#123978=CARTESIAN_POINT('Ctrl Pts',(-75.2807843499784,1076.31720630032,
363.199043033435));
#123979=CARTESIAN_POINT('Ctrl Pts',(-75.1923494186631,1076.32178543985,
363.199043033435));
#123980=CARTESIAN_POINT('Ctrl Pts',(-75.1048022879565,1076.3270122528,363.216409353866));
#123981=CARTESIAN_POINT('Ctrl Pts',(-74.9822262069248,1076.33534324347,
363.266997652347));
#123982=CARTESIAN_POINT('Ctrl Pts',(-74.9431054264288,1076.33818342375,
363.287841643676));
#123983=CARTESIAN_POINT('Ctrl Pts',(-74.8695141570817,1076.34390194688,
363.336866565203));
#123984=CARTESIAN_POINT('Ctrl Pts',(-74.8352170575663,1076.34676671064,
363.364929475761));
#123985=CARTESIAN_POINT('Ctrl Pts',(-74.7401777376837,1076.35535527583,
363.459676970117));
#123986=CARTESIAN_POINT('Ctrl Pts',(-74.6897666533623,1076.36088163242,
363.53532779201));
#123987=CARTESIAN_POINT('Ctrl Pts',(-74.6216654575394,1076.3708364867,363.701730874945));
#123988=CARTESIAN_POINT('Ctrl Pts',(-74.60455276562,1076.37517080223,363.790788986676));
#123989=CARTESIAN_POINT('Ctrl Pts',(-74.6061837746983,1076.3821204472,363.970494750931));
#123990=CARTESIAN_POINT('Ctrl Pts',(-74.624931632915,1076.38466645676,364.059338537434));
#123991=CARTESIAN_POINT('Ctrl Pts',(-74.6961917881948,1076.38764967982,
364.224607327379));
#123992=CARTESIAN_POINT('Ctrl Pts',(-74.7480225687572,1076.38805479619,
364.299339070781));
#123993=CARTESIAN_POINT('Ctrl Pts',(-74.8778961562943,1076.38665154554,
364.424036680836));
#123994=CARTESIAN_POINT('Ctrl Pts',(-74.954602951011,1076.38485851261,364.472753221244));
#123995=CARTESIAN_POINT('Ctrl Pts',(-75.1159547584908,1076.37948362869,
364.534734942781));
#123996=CARTESIAN_POINT('Ctrl Pts',(-75.1980651866747,1076.37610008038,
364.549931275707));
#123997=CARTESIAN_POINT('Ctrl Pts',(-75.2807843499774,1076.3720597734,364.549931275707));
#123998=CARTESIAN_POINT('Origin',(-73.7938092375736,1067.7251047501,350.104695514138));
#123999=CARTESIAN_POINT('',(-73.7938092376029,1075.57253700026,349.005864378145));
#124000=CARTESIAN_POINT('',(-73.7938092375736,1067.7251047501,349.005864378145));
#124001=CARTESIAN_POINT('Ctrl Pts',(-73.7943438286108,1075.73507520609,
351.203526520088));
#124002=CARTESIAN_POINT('Ctrl Pts',(-73.9403170085117,1075.72466814698,
351.203455502841));
#124003=CARTESIAN_POINT('Ctrl Pts',(-74.084675960195,1075.71222254048,351.174300992785));
#124004=CARTESIAN_POINT('Ctrl Pts',(-74.2849583459431,1075.69163544522,
351.090248581891));
#124005=CARTESIAN_POINT('Ctrl Pts',(-74.3480101216659,1075.68457833148,
351.056219174524));
#124006=CARTESIAN_POINT('Ctrl Pts',(-74.5296165654477,1075.66239714621,
350.934006536723));
#124007=CARTESIAN_POINT('Ctrl Pts',(-74.6341208385784,1075.64688776811,
350.827910232112));
#124008=CARTESIAN_POINT('Ctrl Pts',(-74.7935894751206,1075.61685947417,
350.583058284819));
#124009=CARTESIAN_POINT('Ctrl Pts',(-74.8479057527387,1075.60261206263,
350.447227919341));
#124010=CARTESIAN_POINT('Ctrl Pts',(-74.9005698938151,1075.57717485605,
350.162682866827));
#124011=CARTESIAN_POINT('Ctrl Pts',(-74.8986315070578,1075.56621986658,
350.016749704869));
#124012=CARTESIAN_POINT('Ctrl Pts',(-74.8384004917684,1075.54924950489,
349.734665488139));
#124013=CARTESIAN_POINT('Ctrl Pts',(-74.7810666738733,1075.54337181776,
349.601231042371));
#124014=CARTESIAN_POINT('Ctrl Pts',(-74.6185071053364,1075.53756791743,
349.364561147917));
#124015=CARTESIAN_POINT('Ctrl Pts',(-74.5151683413827,1075.53766809888,
349.263526373816));
#124016=CARTESIAN_POINT('Ctrl Pts',(-74.2756832064865,1075.54384041196,
349.106856863847));
#124017=CARTESIAN_POINT('Ctrl Pts',(-74.1419546455288,1075.54984400915,
349.052736057625));
#124018=CARTESIAN_POINT('Ctrl Pts',(-73.8609052025502,1075.56694315995,
348.998578412881));
#124019=CARTESIAN_POINT('Ctrl Pts',(-73.7162781603625,1075.57789026887,
348.999298161707));
#124020=CARTESIAN_POINT('Ctrl Pts',(-73.4347958345081,1075.60324547587,
349.056224428512));
#124021=CARTESIAN_POINT('Ctrl Pts',(-73.3006816519036,1075.61743115363,
349.112247540691));
#124022=CARTESIAN_POINT('Ctrl Pts',(-73.0612986408069,1075.64708439173,
349.272991388969));
#124023=CARTESIAN_POINT('Ctrl Pts',(-72.958399197672,1075.66227779007,349.376410086018));
#124024=CARTESIAN_POINT('Ctrl Pts',(-72.797612000534,1075.6917527953,349.618511135587));
#124025=CARTESIAN_POINT('Ctrl Pts',(-72.7417953372785,1075.70573900701,
349.755246162285));
#124026=CARTESIAN_POINT('Ctrl Pts',(-72.6871649626123,1075.73041142659,
350.041937314009));
#124027=CARTESIAN_POINT('Ctrl Pts',(-72.6885603814981,1075.7408770953,350.189001738921));
#124028=CARTESIAN_POINT('Ctrl Pts',(-72.7487463610536,1075.75702253198,
350.4741281338));
#124029=CARTESIAN_POINT('Ctrl Pts',(-72.8068707077791,1075.76254706029,
350.609318738545));
#124030=CARTESIAN_POINT('Ctrl Pts',(-72.9726685012712,1075.76793996582,
350.849299583654));
#124031=CARTESIAN_POINT('Ctrl Pts',(-73.0786544439614,1075.76775184252,
350.951607007295));
#124032=CARTESIAN_POINT('Ctrl Pts',(-73.3243233086004,1075.76162585565,
351.108823140814));
#124033=CARTESIAN_POINT('Ctrl Pts',(-73.4614663626373,1075.75575198615,
351.16213559445));
#124034=CARTESIAN_POINT('Ctrl Pts',(-73.6674877868136,1075.74371243895,
351.198088647224));
#124035=CARTESIAN_POINT('Ctrl Pts',(-73.7308714385672,1075.7396004272,351.20355739997));
#124036=CARTESIAN_POINT('Ctrl Pts',(-73.7943438286108,1075.73507520609,
351.203526520089));
#124037=CARTESIAN_POINT('Origin',(-73.7938092375736,1067.7251047501,350.104695514138));
#124038=CARTESIAN_POINT('',(-73.7938092375736,1075.69207332612,350.60352665013));
#124039=CARTESIAN_POINT('',(-73.7938092375736,1075.61827177418,349.605864378145));
#124040=CARTESIAN_POINT('Ctrl Pts',(-73.7938092375736,1075.69207332612,
350.60352665013));
#124041=CARTESIAN_POINT('Ctrl Pts',(-73.7979495129483,1075.69177375716,
350.60352665013));
#124042=CARTESIAN_POINT('Ctrl Pts',(-73.802091793159,1075.69147023046,350.603475104143));
#124043=CARTESIAN_POINT('Ctrl Pts',(-73.8728178240604,1075.68622244654,
350.60171277064));
#124044=CARTESIAN_POINT('Ctrl Pts',(-73.9383329755696,1075.68037315732,
350.586738379904));
#124045=CARTESIAN_POINT('Ctrl Pts',(-74.0286377306387,1075.67080350965,
350.546000300336));
#124046=CARTESIAN_POINT('Ctrl Pts',(-74.0569482506047,1075.66754082214,
350.529726126065));
#124047=CARTESIAN_POINT('Ctrl Pts',(-74.1100452604125,1075.66086906725,
350.4918561257));
#124048=CARTESIAN_POINT('Ctrl Pts',(-74.134699477728,1075.65747511528,350.470334703564));
#124049=CARTESIAN_POINT('Ctrl Pts',(-74.2029959977506,1075.64709855625,
350.397763736712));
#124050=CARTESIAN_POINT('Ctrl Pts',(-74.238638821479,1075.64019996183,350.340188220393));
#124051=CARTESIAN_POINT('Ctrl Pts',(-74.2845288500381,1075.62754140758,
350.215728271492));
#124052=CARTESIAN_POINT('Ctrl Pts',(-74.2948822435841,1075.62188043308,
350.150258958649));
#124053=CARTESIAN_POINT('Ctrl Pts',(-74.2896041219376,1075.61246458717,
350.019325521818));
#124054=CARTESIAN_POINT('Ctrl Pts',(-74.2741718712292,1075.60879116,349.95513669967));
#124055=CARTESIAN_POINT('Ctrl Pts',(-74.2194898641718,1075.60395376277,
349.836623196663));
#124056=CARTESIAN_POINT('Ctrl Pts',(-74.1809195751678,1075.60282391206,
349.783420087652));
#124057=CARTESIAN_POINT('Ctrl Pts',(-74.0855925349758,1075.60326819831,
349.694921376715));
#124058=CARTESIAN_POINT('Ctrl Pts',(-74.0298308188195,1075.60483147094,
349.660467354418));
#124059=CARTESIAN_POINT('Ctrl Pts',(-73.9130462923001,1075.61022799793,
349.61664313576));
#124060=CARTESIAN_POINT('Ctrl Pts',(-73.8537514928858,1075.61382884438,
349.6058898588));
#124061=CARTESIAN_POINT('Ctrl Pts',(-73.7940216604385,1075.61825602602,
349.605864423372));
#124062=CARTESIAN_POINT('Ctrl Pts',(-73.793950852004,1075.61826127435,349.605864393219));
#124063=CARTESIAN_POINT('Ctrl Pts',(-73.7938800443809,1075.61826652374,
349.605864378145));
#124064=CARTESIAN_POINT('Ctrl Pts',(-73.7938092375737,1075.61827177418,
349.605864378145));
#124065=CARTESIAN_POINT('',(-73.7938092375736,1082.7251047501,349.605864378145));
#124066=CARTESIAN_POINT('',(-73.7938092375736,1067.7251047501,349.605864378145));
#124067=CARTESIAN_POINT('Origin',(-73.7938092375736,1082.7251047501,350.104695514138));
#124068=CARTESIAN_POINT('Ctrl Pts',(-73.7938092375737,1075.61827177418,
349.605864378145));
#124069=CARTESIAN_POINT('Ctrl Pts',(-73.7285772438854,1075.62310883226,
349.605864378145));
#124070=CARTESIAN_POINT('Ctrl Pts',(-73.6640377663185,1075.6288410551,349.618658646094));
#124071=CARTESIAN_POINT('Ctrl Pts',(-73.543216236694,1075.64145773073,349.668423827516));
#124072=CARTESIAN_POINT('Ctrl Pts',(-73.4881375880883,1075.64822967675,
349.705085037028));
#124073=CARTESIAN_POINT('Ctrl Pts',(-73.3944413635905,1075.66200138751,
349.798437137012));
#124074=CARTESIAN_POINT('Ctrl Pts',(-73.3570671295821,1075.66886930196,
349.854590499074));
#124075=CARTESIAN_POINT('Ctrl Pts',(-73.306774695344,1075.68159917132,349.978015673703));
#124076=CARTESIAN_POINT('Ctrl Pts',(-73.2942236093973,1075.68734219416,
350.04402356237));
#124077=CARTESIAN_POINT('Ctrl Pts',(-73.2957998750605,1075.69694028833,
350.176956305832));
#124078=CARTESIAN_POINT('Ctrl Pts',(-73.3098168227983,1075.7007063751,350.242543762047));
#124079=CARTESIAN_POINT('Ctrl Pts',(-73.3627627989532,1075.7057576137,350.364382063199));
#124080=CARTESIAN_POINT('Ctrl Pts',(-73.4011122848796,1075.70699463425,
350.419391136037));
#124081=CARTESIAN_POINT('Ctrl Pts',(-73.4961277294539,1075.70675684485,
350.510214825593));
#124082=CARTESIAN_POINT('Ctrl Pts',(-73.5514432522579,1075.70534097152,
350.54550420152));
#124083=CARTESIAN_POINT('Ctrl Pts',(-73.669974095671,1075.70017464118,350.591913631098));
#124084=CARTESIAN_POINT('Ctrl Pts',(-73.7316658307316,1075.69656970236,
350.60352665013));
#124085=CARTESIAN_POINT('Ctrl Pts',(-73.7938092375736,1075.69207332612,
350.60352665013));
#124086=CARTESIAN_POINT('Origin',(-69.4825522658041,1067.7251047501,336.798793877895));
#124087=CARTESIAN_POINT('',(-69.482552265823,1074.68462093241,335.708253129166));
#124088=CARTESIAN_POINT('',(-69.4825522658041,1067.7251047501,335.708253129166));
#124089=CARTESIAN_POINT('Ctrl Pts',(-69.482044588625,1074.91623532639,337.889334508454));
#124090=CARTESIAN_POINT('Ctrl Pts',(-69.6268448872223,1074.90431233596,
337.889401917045));
#124091=CARTESIAN_POINT('Ctrl Pts',(-69.7699610523262,1074.88948709449,
337.860634556447));
#124092=CARTESIAN_POINT('Ctrl Pts',(-70.0368352563637,1074.85562701002,
337.749084359417));
#124093=CARTESIAN_POINT('Ctrl Pts',(-70.1579277482776,1074.83690116048,
337.66716268673));
#124094=CARTESIAN_POINT('Ctrl Pts',(-70.3092460076959,1074.80795475402,
337.513563586279));
#124095=CARTESIAN_POINT('Ctrl Pts',(-70.3540051655982,1074.79832384645,
337.458253465507));
#124096=CARTESIAN_POINT('Ctrl Pts',(-70.4735436314901,1074.76896404509,
337.27691019806));
#124097=CARTESIAN_POINT('Ctrl Pts',(-70.5287184548299,1074.74962867978,
337.13977603213));
#124098=CARTESIAN_POINT('Ctrl Pts',(-70.5810814878598,1074.71455491498,
336.854557003272));
#124099=CARTESIAN_POINT('Ctrl Pts',(-70.5789216965246,1074.69908367227,
336.70942848117));
#124100=CARTESIAN_POINT('Ctrl Pts',(-70.5184644809355,1074.67397221671,
336.429363436276));
#124101=CARTESIAN_POINT('Ctrl Pts',(-70.4613246199309,1074.66452295267,
336.297081656758));
#124102=CARTESIAN_POINT('Ctrl Pts',(-70.2996719412468,1074.65297235618,
336.062810712616));
#124103=CARTESIAN_POINT('Ctrl Pts',(-70.197208708713,1074.65092631395,335.962940541778));
#124104=CARTESIAN_POINT('Ctrl Pts',(-69.9599373338993,1074.65450377585,
335.808133153499));
#124105=CARTESIAN_POINT('Ctrl Pts',(-69.8276153228959,1074.66007498532,
335.754685532963));
#124106=CARTESIAN_POINT('Ctrl Pts',(-69.5493717095422,1074.67812828618,
335.701064215748));
#124107=CARTESIAN_POINT('Ctrl Pts',(-69.4061566135024,1074.69046942786,
335.701749622818));
#124108=CARTESIAN_POINT('Ctrl Pts',(-69.126998138824,1074.72034296465,335.75795645933));
#124109=CARTESIAN_POINT('Ctrl Pts',(-68.9938302321287,1074.73763799905,
335.813502389317));
#124110=CARTESIAN_POINT('Ctrl Pts',(-68.8158524427427,1074.76546282371,
335.932820391935));
#124111=CARTESIAN_POINT('Ctrl Pts',(-68.7605056092299,1074.77500173065,
335.978403244282));
#124112=CARTESIAN_POINT('Ctrl Pts',(-68.6597463291446,1074.79425731883,
336.079526422682));
#124113=CARTESIAN_POINT('Ctrl Pts',(-68.6145238193859,1074.80393019429,
336.134804249594));
#124114=CARTESIAN_POINT('Ctrl Pts',(-68.4947890010657,1074.83301338696,
336.314503657827));
#124115=CARTESIAN_POINT('Ctrl Pts',(-68.4392432986122,1074.85191119827,
336.449796131516));
#124116=CARTESIAN_POINT('Ctrl Pts',(-68.3844244251128,1074.88628567302,
336.733828681667));
#124117=CARTESIAN_POINT('Ctrl Pts',(-68.3854281483946,1074.90145000531,
336.879787802314));
#124118=CARTESIAN_POINT('Ctrl Pts',(-68.4445847243561,1074.9261138144,337.163333469513));
#124119=CARTESIAN_POINT('Ctrl Pts',(-68.5021762038381,1074.93536178919,
337.298037043689));
#124120=CARTESIAN_POINT('Ctrl Pts',(-68.664979268859,1074.94649842765,337.534260766224));
#124121=CARTESIAN_POINT('Ctrl Pts',(-68.7673286622167,1074.94845439328,
337.634149339983));
#124122=CARTESIAN_POINT('Ctrl Pts',(-69.004712556087,1074.94507002068,337.789285191735));
#124123=CARTESIAN_POINT('Ctrl Pts',(-69.1373636244834,1074.9397565634,337.842910728574));
#124124=CARTESIAN_POINT('Ctrl Pts',(-69.3442431971288,1074.92689252331,
337.882730528295));
#124125=CARTESIAN_POINT('Ctrl Pts',(-69.4130907838078,1074.92191304641,
337.889302408528));
#124126=CARTESIAN_POINT('Ctrl Pts',(-69.482044588625,1074.91623532639,337.889334508454));
#124127=CARTESIAN_POINT('Origin',(-69.4825522658041,1067.7251047501,336.798793877895));
#124128=CARTESIAN_POINT('',(-69.4825522658041,1074.85393827482,337.289334626623));
#124129=CARTESIAN_POINT('',(-69.4825522658041,1074.74977363876,336.308253129166));
#124130=CARTESIAN_POINT('Ctrl Pts',(-69.4825522658041,1074.85393827482,
337.289334626623));
#124131=CARTESIAN_POINT('Ctrl Pts',(-69.5156608898946,1074.85118092534,
337.289334626623));
#124132=CARTESIAN_POINT('Ctrl Pts',(-69.5487365376258,1074.84807154848,
337.285982577554));
#124133=CARTESIAN_POINT('Ctrl Pts',(-69.6453218199865,1074.83792315234,
337.266139960999));
#124134=CARTESIAN_POINT('Ctrl Pts',(-69.7060039722654,1074.830128241,337.240326933441));
#124135=CARTESIAN_POINT('Ctrl Pts',(-69.7861436696537,1074.81760734305,
337.185423455841));
#124136=CARTESIAN_POINT('Ctrl Pts',(-69.8106551502927,1074.81337335087,
337.164850184747));
#124137=CARTESIAN_POINT('Ctrl Pts',(-69.8553503056872,1074.80478387879,
337.119220492057));
#124138=CARTESIAN_POINT('Ctrl Pts',(-69.8754283392612,1074.80044735509,
337.094259376792));
#124139=CARTESIAN_POINT('Ctrl Pts',(-69.9288586827907,1074.7872828606,337.012665023113));
#124140=CARTESIAN_POINT('Ctrl Pts',(-69.95345227519,1074.7786526084,336.951105668282));
#124141=CARTESIAN_POINT('Ctrl Pts',(-69.9768104861118,1074.7629587941,336.82252465352));
#124142=CARTESIAN_POINT('Ctrl Pts',(-69.975622761632,1074.75602992107,336.756795840196));
#124143=CARTESIAN_POINT('Ctrl Pts',(-69.9477765303257,1074.74487453043,
336.630569671525));
#124144=CARTESIAN_POINT('Ctrl Pts',(-69.9218399501277,1074.74071220095,
336.571236267911));
#124145=CARTESIAN_POINT('Ctrl Pts',(-69.8487299623223,1074.73565201654,
336.466220536245));
#124146=CARTESIAN_POINT('Ctrl Pts',(-69.8024632954533,1074.7347802369,336.421496203756));
#124147=CARTESIAN_POINT('Ctrl Pts',(-69.6954251653061,1074.73644059973,
336.352281990104));
#124148=CARTESIAN_POINT('Ctrl Pts',(-69.6357611873031,1074.73895190826,
336.328475021556));
#124149=CARTESIAN_POINT('Ctrl Pts',(-69.5433400443614,1074.74492535713,
336.311081847338));
#124150=CARTESIAN_POINT('Ctrl Pts',(-69.5129674837563,1074.7471970323,336.308253129166));
#124151=CARTESIAN_POINT('Ctrl Pts',(-69.4825522658041,1074.74977363876,
336.308253129166));
#124152=CARTESIAN_POINT('',(-69.4825522658041,1082.7251047501,336.308253129166));
#124153=CARTESIAN_POINT('',(-69.4825522658041,1067.7251047501,336.308253129166));
#124154=CARTESIAN_POINT('Origin',(-69.4825522658041,1082.7251047501,336.798793877895));
#124155=CARTESIAN_POINT('Ctrl Pts',(-69.48255183749,1074.74977367504,336.308253129166));
#124156=CARTESIAN_POINT('Ctrl Pts',(-69.4183527172007,1074.75521226996,
336.308253185222));
#124157=CARTESIAN_POINT('Ctrl Pts',(-69.3548876880576,1074.76193077302,
336.320853926478));
#124158=CARTESIAN_POINT('Ctrl Pts',(-69.234964446525,1074.77733067317,336.370251892038));
#124159=CARTESIAN_POINT('Ctrl Pts',(-69.1799132064186,1074.78590878087,
336.407205839001));
#124160=CARTESIAN_POINT('Ctrl Pts',(-69.1112824361735,1074.79905699663,
336.476592740311));
#124161=CARTESIAN_POINT('Ctrl Pts',(-69.0910539250758,1074.8034013946,336.50149956963));
#124162=CARTESIAN_POINT('Ctrl Pts',(-69.0373963429084,1074.81651113423,
336.582632990236));
#124163=CARTESIAN_POINT('Ctrl Pts',(-69.012584813969,1074.82505786061,336.643759086384));
#124164=CARTESIAN_POINT('Ctrl Pts',(-68.988414035207,1074.84063673182,336.772111408957));
#124165=CARTESIAN_POINT('Ctrl Pts',(-68.9892279760228,1074.84752250316,
336.838084476661));
#124166=CARTESIAN_POINT('Ctrl Pts',(-69.0165987816869,1074.85862426497,
336.965191865952));
#124167=CARTESIAN_POINT('Ctrl Pts',(-69.0425474794926,1074.86276376567,
337.025111727045));
#124168=CARTESIAN_POINT('Ctrl Pts',(-69.1157573489778,1074.86776989741,
337.130684087977));
#124169=CARTESIAN_POINT('Ctrl Pts',(-69.1619316104886,1074.86863787131,
337.175486532404));
#124170=CARTESIAN_POINT('Ctrl Pts',(-69.2688854443816,1074.86704482667,
337.244936442028));
#124171=CARTESIAN_POINT('Ctrl Pts',(-69.3285787197443,1074.86459932949,
337.268873137344));
#124172=CARTESIAN_POINT('Ctrl Pts',(-69.4213566312991,1074.85873207417,
337.286474621064));
#124173=CARTESIAN_POINT('Ctrl Pts',(-69.4519685163185,1074.85648534792,
337.289334626623));
#124174=CARTESIAN_POINT('Ctrl Pts',(-69.4825522658041,1074.85393827482,
337.289334626623));
#124175=CARTESIAN_POINT('Origin',(-83.8577571500213,1067.7251047501,393.178981560286));
#124176=CARTESIAN_POINT('',(-83.857757150042,1076.65831288829,391.700678428093));
#124177=CARTESIAN_POINT('',(-83.8577571500213,1067.7251047501,391.700678428093));
#124178=CARTESIAN_POINT('Ctrl Pts',(-83.8571940935802,1076.6854098979,394.657284585251));
#124179=CARTESIAN_POINT('Ctrl Pts',(-83.9528543621346,1076.68332503261,
394.657321020359));
#124180=CARTESIAN_POINT('Ctrl Pts',(-84.0482896858879,1076.68110226508,
394.648072189946));
#124181=CARTESIAN_POINT('Ctrl Pts',(-84.237925298588,1076.67637636788,394.610895081188));
#124182=CARTESIAN_POINT('Ctrl Pts',(-84.3315968557539,1076.6738799666,394.582683514737));
#124183=CARTESIAN_POINT('Ctrl Pts',(-84.6011130072004,1076.66619665297,
394.471434048908));
#124184=CARTESIAN_POINT('Ctrl Pts',(-84.7641144709483,1076.66085524092,
394.362842571996));
#124185=CARTESIAN_POINT('Ctrl Pts',(-85.038951478879,1076.65048514005,394.088837035227));
#124186=CARTESIAN_POINT('Ctrl Pts',(-85.1480925625414,1076.64556313726,
393.926042650183));
#124187=CARTESIAN_POINT('Ctrl Pts',(-85.29720850228,1076.63713488144,393.567607409226));
#124188=CARTESIAN_POINT('Ctrl Pts',(-85.3357493456625,1076.63371736493,
393.375454127138));
#124189=CARTESIAN_POINT('Ctrl Pts',(-85.3363669002121,1076.62916473982,
392.987575080872));
#124190=CARTESIAN_POINT('Ctrl Pts',(-85.2985786646413,1076.6280741197,392.795625867869));
#124191=CARTESIAN_POINT('Ctrl Pts',(-85.1512839784971,1076.62848785611,
392.437677318038));
#124192=CARTESIAN_POINT('Ctrl Pts',(-85.0433812733427,1076.6299813596,392.27508309293));
#124193=CARTESIAN_POINT('Ctrl Pts',(-84.7713116447634,1076.63522890501,
392.00082100113));
#124194=CARTESIAN_POINT('Ctrl Pts',(-84.6098376407021,1076.63892452082,
391.89173373863));
#124195=CARTESIAN_POINT('Ctrl Pts',(-84.2540359013528,1076.6477403855,391.741749309456));
#124196=CARTESIAN_POINT('Ctrl Pts',(-84.0631087233663,1076.65276963375,
391.702331024677));
#124197=CARTESIAN_POINT('Ctrl Pts',(-83.6767164193077,1076.66319957231,
391.699125773987));
#124198=CARTESIAN_POINT('Ctrl Pts',(-83.484959280491,1076.66849503082,391.735453626999));
#124199=CARTESIAN_POINT('Ctrl Pts',(-83.12350095616,1076.67858982704,391.880984179758));
#124200=CARTESIAN_POINT('Ctrl Pts',(-82.9577796125186,1076.68327916066,
391.989873201615));
#124201=CARTESIAN_POINT('Ctrl Pts',(-82.6796118544,1076.69142377176,392.265014015731));
#124202=CARTESIAN_POINT('Ctrl Pts',(-82.5695033304998,1076.6948139835,392.428132767469));
#124203=CARTESIAN_POINT('Ctrl Pts',(-82.4187788222995,1076.70020865997,
392.7880223399));
#124204=CARTESIAN_POINT('Ctrl Pts',(-82.3797726792368,1076.70216608927,
392.981307429118));
#124205=CARTESIAN_POINT('Ctrl Pts',(-82.379137778424,1076.70470788168,393.372764725265));
#124206=CARTESIAN_POINT('Ctrl Pts',(-82.4178747972533,1076.70526678929,
393.56706340159));
#124207=CARTESIAN_POINT('Ctrl Pts',(-82.5688901593564,1076.70501100144,
393.92907705046));
#124208=CARTESIAN_POINT('Ctrl Pts',(-82.6796238666232,1076.7041989837,394.093214087362));
#124209=CARTESIAN_POINT('Ctrl Pts',(-82.9579861578556,1076.70113667203,
394.368040577126));
#124210=CARTESIAN_POINT('Ctrl Pts',(-83.1225997395357,1076.69891644088,
394.476281318645));
#124211=CARTESIAN_POINT('Ctrl Pts',(-83.4794127948176,1076.69307788233,
394.62059810628));
#124212=CARTESIAN_POINT('Ctrl Pts',(-83.6674202830168,1076.68954591838,
394.657212304152));
#124213=CARTESIAN_POINT('Ctrl Pts',(-83.8571940935802,1076.6854098979,394.657284585251));
#124214=CARTESIAN_POINT('Origin',(-83.8577571500213,1067.7251047501,393.178981560286));
#124215=CARTESIAN_POINT('',(-83.8577571500214,1076.68056431803,394.057284692479));
#124216=CARTESIAN_POINT('',(-83.8577571500214,1076.66449392106,392.300678428093));
#124217=CARTESIAN_POINT('Ctrl Pts',(-83.8577571500213,1076.68056431803,
394.057284692479));
#124218=CARTESIAN_POINT('Ctrl Pts',(-83.8670327327715,1076.68035245333,
394.057284692479));
#124219=CARTESIAN_POINT('Ctrl Pts',(-83.8763143809642,1076.68013857438,
394.057137756963));
#124220=CARTESIAN_POINT('Ctrl Pts',(-83.9426550514218,1076.67859627437,
394.05503375308));
#124221=CARTESIAN_POINT('Ctrl Pts',(-83.9993979702626,1076.67720503007,
394.047666006467));
#124222=CARTESIAN_POINT('Ctrl Pts',(-84.1115404391114,1076.67430293354,
394.021818713267));
#124223=CARTESIAN_POINT('Ctrl Pts',(-84.1666289995102,1076.67279760102,
394.003225708839));
#124224=CARTESIAN_POINT('Ctrl Pts',(-84.3244367217557,1076.66824031985,
393.931904175525));
#124225=CARTESIAN_POINT('Ctrl Pts',(-84.4190457650727,1076.6651682811,393.864282995571));
#124226=CARTESIAN_POINT('Ctrl Pts',(-84.5767883879247,1076.65935515809,
393.696363226682));
#124227=CARTESIAN_POINT('Ctrl Pts',(-84.6383872444461,1076.65667261187,
393.597681479671));
#124228=CARTESIAN_POINT('Ctrl Pts',(-84.7199568441604,1076.65217975208,
393.382194701899));
#124229=CARTESIAN_POINT('Ctrl Pts',(-84.7391506937016,1076.65041529028,
393.267485487742));
#124230=CARTESIAN_POINT('Ctrl Pts',(-84.7321658922115,1076.6481548133,393.037337041536));
#124231=CARTESIAN_POINT('Ctrl Pts',(-84.706112537041,1076.64768065755,392.924132305296));
#124232=CARTESIAN_POINT('Ctrl Pts',(-84.6119096269206,1076.6481273546,392.714362857543));
#124233=CARTESIAN_POINT('Ctrl Pts',(-84.5447339090463,1076.64904152667,
392.619806061394));
#124234=CARTESIAN_POINT('Ctrl Pts',(-84.3778492305326,1076.65208950437,
392.461971183699));
#124235=CARTESIAN_POINT('Ctrl Pts',(-84.2797698970617,1076.65419121897,
392.400199755891));
#124236=CARTESIAN_POINT('Ctrl Pts',(-84.0721098264575,1076.65904314149,
392.320461958781));
#124237=CARTESIAN_POINT('Ctrl Pts',(-83.9653858733157,1076.66170161447,
392.300678428093));
#124238=CARTESIAN_POINT('Ctrl Pts',(-83.8577571500214,1076.66449392106,
392.300678428093));
#124239=CARTESIAN_POINT('',(-83.8577571500213,1082.7251047501,392.300678428093));
#124240=CARTESIAN_POINT('',(-83.8577571500213,1067.7251047501,392.300678428093));
#124241=CARTESIAN_POINT('Origin',(-83.8577571500213,1082.7251047501,393.178981560286));
#124242=CARTESIAN_POINT('Ctrl Pts',(-83.8577571500215,1076.66449392106,
392.300678428093));
#124243=CARTESIAN_POINT('Ctrl Pts',(-83.8576325991735,1076.66449715239,
392.300678428093));
#124244=CARTESIAN_POINT('Ctrl Pts',(-83.8575080471139,1076.66450038391,
392.300678454586));
#124245=CARTESIAN_POINT('Ctrl Pts',(-83.8573834938509,1076.6645036156,392.300678507575));
#124246=CARTESIAN_POINT('Ctrl Pts',(-83.7424453681473,1076.66748583276,
392.300727405663));
#124247=CARTESIAN_POINT('Ctrl Pts',(-83.6286264789588,1076.67056282292,
392.323337722145));
#124248=CARTESIAN_POINT('Ctrl Pts',(-83.4143101513657,1076.67656701639,
392.411878073479));
#124249=CARTESIAN_POINT('Ctrl Pts',(-83.3162179447018,1076.67943066473,
392.477675041555));
#124250=CARTESIAN_POINT('Ctrl Pts',(-83.1519124801383,1076.68453543471,
392.64347795714));
#124251=CARTESIAN_POINT('Ctrl Pts',(-83.0871956578491,1076.68673069361,
392.74169562649));
#124252=CARTESIAN_POINT('Ctrl Pts',(-82.999794699067,1076.69028414284,392.957803100277));
#124253=CARTESIAN_POINT('Ctrl Pts',(-82.9780358079161,1076.69160888867,
393.073567321889));
#124254=CARTESIAN_POINT('Ctrl Pts',(-82.9810196179529,1076.69331446352,
393.307153084358));
#124255=CARTESIAN_POINT('Ctrl Pts',(-83.0058604890839,1076.69367765092,
393.422639927147));
#124256=CARTESIAN_POINT('Ctrl Pts',(-83.0992918588072,1076.69341808685,
393.637035353046));
#124257=CARTESIAN_POINT('Ctrl Pts',(-83.1669243560869,1076.69279811395,
393.733807464251));
#124258=CARTESIAN_POINT('Ctrl Pts',(-83.3358456582448,1076.6905903592,393.894949496057));
#124259=CARTESIAN_POINT('Ctrl Pts',(-83.4353550347065,1076.68902491243,
393.957811127997));
#124260=CARTESIAN_POINT('Ctrl Pts',(-83.6444027165045,1076.68518587222,
394.037700648553));
#124261=CARTESIAN_POINT('Ctrl Pts',(-83.7506757699026,1076.68301017665,
394.057284692479));
#124262=CARTESIAN_POINT('Ctrl Pts',(-83.8577571500213,1076.68056431803,
394.057284692479));
#124263=CARTESIAN_POINT('Origin',(-86.2654713137621,1067.7251047501,380.853682816142));
#124264=CARTESIAN_POINT('',(-86.2654713137811,1076.3065749206,379.578238695006));
#124265=CARTESIAN_POINT('',(-86.2654713137621,1067.7251047501,379.578238695006));
#124266=CARTESIAN_POINT('Ctrl Pts',(-86.2659855827959,1076.38119950511,
382.1291268336));
#124267=CARTESIAN_POINT('Ctrl Pts',(-86.4358682980053,1076.37179008192,
382.129058335556));
#124268=CARTESIAN_POINT('Ctrl Pts',(-86.6039911709605,1076.36136063546,
382.095050328875));
#124269=CARTESIAN_POINT('Ctrl Pts',(-86.838212942953,1076.34506250357,381.996415866367));
#124270=CARTESIAN_POINT('Ctrl Pts',(-86.9125062498822,1076.33958092772,
381.956051590261));
#124271=CARTESIAN_POINT('Ctrl Pts',(-87.120926270196,1076.32323213126,381.814441036432));
#124272=CARTESIAN_POINT('Ctrl Pts',(-87.2396860582528,1076.31254531983,
381.693793545343));
#124273=CARTESIAN_POINT('Ctrl Pts',(-87.4236826281354,1076.29291722146,
381.413497063116));
#124274=CARTESIAN_POINT('Ctrl Pts',(-87.4871785906302,1076.2841681821,381.256573626955));
#124275=CARTESIAN_POINT('Ctrl Pts',(-87.5497217275718,1076.27002873665,
380.927454436253));
#124276=CARTESIAN_POINT('Ctrl Pts',(-87.5483281141395,1076.26477160671,
380.75850570807));
#124277=CARTESIAN_POINT('Ctrl Pts',(-87.4804422415383,1076.25864463005,
380.431281106168));
#124278=CARTESIAN_POINT('Ctrl Pts',(-87.4148505403703,1076.25782123202,
380.276177917597));
#124279=CARTESIAN_POINT('Ctrl Pts',(-87.2278806424649,1076.26076272105,
380.000320821711));
#124280=CARTESIAN_POINT('Ctrl Pts',(-87.1084596581209,1076.2644873009,379.882189185605));
#124281=CARTESIAN_POINT('Ctrl Pts',(-86.8309951438903,1076.27590558092,
379.698412639541));
#124282=CARTESIAN_POINT('Ctrl Pts',(-86.6756168158444,1076.28348750493,
379.634583953848));
#124283=CARTESIAN_POINT('Ctrl Pts',(-86.3488023339255,1076.30135488652,
379.570080743726));
#124284=CARTESIAN_POINT('Ctrl Pts',(-86.1804566596807,1076.31147216406,
379.570203373631));
#124285=CARTESIAN_POINT('Ctrl Pts',(-85.9350741103993,1076.327421904,379.618950564278));
#124286=CARTESIAN_POINT('Ctrl Pts',(-85.8549948440434,1076.33283452927,
379.643214275629));
#124287=CARTESIAN_POINT('Ctrl Pts',(-85.7007056878628,1076.34367716873,
379.707048541646));
#124288=CARTESIAN_POINT('Ctrl Pts',(-85.6268640325357,1076.34908143445,
379.746473557798));
#124289=CARTESIAN_POINT('Ctrl Pts',(-85.416338610646,1076.36517058836,379.886989368421));
#124290=CARTESIAN_POINT('Ctrl Pts',(-85.2954204815106,1076.37539263519,
380.008368862177));
#124291=CARTESIAN_POINT('Ctrl Pts',(-85.1087361966729,1076.39358550485,
380.290517624953));
#124292=CARTESIAN_POINT('Ctrl Pts',(-85.0444606327581,1076.40139571981,
380.44826213456));
#124293=CARTESIAN_POINT('Ctrl Pts',(-84.9810339300332,1076.41380990982,
380.779769772346));
#124294=CARTESIAN_POINT('Ctrl Pts',(-84.9825257112795,1076.41829511191,
380.950241206266));
#124295=CARTESIAN_POINT('Ctrl Pts',(-85.0519167131888,1076.42348028237,
381.28106874482));
#124296=CARTESIAN_POINT('Ctrl Pts',(-85.1192376968099,1076.4241243296,381.438085739406));
#124297=CARTESIAN_POINT('Ctrl Pts',(-85.3111237528364,1076.42146587903,
381.716549588247));
#124298=CARTESIAN_POINT('Ctrl Pts',(-85.4337045468094,1076.41819268183,
381.835242468119));
#124299=CARTESIAN_POINT('Ctrl Pts',(-85.7177150601958,1076.40800779872,
382.017804202035));
#124300=CARTESIAN_POINT('Ctrl Pts',(-85.8762627837711,1076.40119785151,
382.079934047725));
#124301=CARTESIAN_POINT('Ctrl Pts',(-86.1161074105835,1076.38928422029,
382.122571135187));
#124302=CARTESIAN_POINT('Ctrl Pts',(-86.1909810984377,1076.38535383554,
382.129157075996));
#124303=CARTESIAN_POINT('Ctrl Pts',(-86.265985582796,1076.38119950511,382.1291268336));
#124304=CARTESIAN_POINT('Origin',(-86.2654713137621,1067.7251047501,380.853682816142));
#124305=CARTESIAN_POINT('',(-86.2654713137621,1076.36458696229,381.529126937278));
#124306=CARTESIAN_POINT('',(-86.2654713137623,1076.32506388483,380.178238695006));
#124307=CARTESIAN_POINT('Ctrl Pts',(-86.2654713137621,1076.36458696229,
381.529126937278));
#124308=CARTESIAN_POINT('Ctrl Pts',(-86.3176203844329,1076.36164319747,
381.529126937278));
#124309=CARTESIAN_POINT('Ctrl Pts',(-86.3697119936323,1076.35851489311,
381.523087338792));
#124310=CARTESIAN_POINT('Ctrl Pts',(-86.4636268773205,1076.3525165865,381.500911826086));
#124311=CARTESIAN_POINT('Ctrl Pts',(-86.5054630782866,1076.34970353828,
381.486592295606));
#124312=CARTESIAN_POINT('Ctrl Pts',(-86.5862544493745,1076.34397809118,
381.449769217969));
#124313=CARTESIAN_POINT('Ctrl Pts',(-86.6249698706937,1076.34107874961,
381.427252031763));
#124314=CARTESIAN_POINT('Ctrl Pts',(-86.7330705388248,1076.33249670945,
381.349107136058));
#124315=CARTESIAN_POINT('Ctrl Pts',(-86.7940420633252,1076.32696821287,
381.28346691746));
#124316=CARTESIAN_POINT('Ctrl Pts',(-86.8870760472062,1076.31694808952,
381.132415059668));
#124317=CARTESIAN_POINT('Ctrl Pts',(-86.9182729858075,1076.31255312352,
381.048481114142));
#124318=CARTESIAN_POINT('Ctrl Pts',(-86.9463994247123,1076.30556164688,
380.873509680982));
#124319=CARTESIAN_POINT('Ctrl Pts',(-86.9431418328645,1076.30302988497,
380.784194133374));
#124320=CARTESIAN_POINT('Ctrl Pts',(-86.9023852566707,1076.30022562937,
380.612097881493));
#124321=CARTESIAN_POINT('Ctrl Pts',(-86.8653797104945,1076.29997496699,
380.530985347912));
#124322=CARTESIAN_POINT('Ctrl Pts',(-86.7623125829652,1076.30180520775,
380.387685650732));
#124323=CARTESIAN_POINT('Ctrl Pts',(-86.6972952692519,1076.30386493615,
380.326876916281));
#124324=CARTESIAN_POINT('Ctrl Pts',(-86.5475324764006,1076.31000530059,
380.233637770325));
#124325=CARTESIAN_POINT('Ctrl Pts',(-86.464218835407,1076.31402749585,380.202144991004));
#124326=CARTESIAN_POINT('Ctrl Pts',(-86.340372603284,1076.32074018736,380.181364110388));
#124327=CARTESIAN_POINT('Ctrl Pts',(-86.3030552747707,1076.32285151909,
380.178250175801));
#124328=CARTESIAN_POINT('Ctrl Pts',(-86.2656782137016,1076.32505170487,
380.178238726578));
#124329=CARTESIAN_POINT('Ctrl Pts',(-86.2656092465274,1076.3250557646,380.178238705453));
#124330=CARTESIAN_POINT('Ctrl Pts',(-86.2655402798804,1076.32505982459,
380.178238695006));
#124331=CARTESIAN_POINT('Ctrl Pts',(-86.2654713137625,1076.32506388483,
380.178238695006));
#124332=CARTESIAN_POINT('',(-86.2654713137621,1082.7251047501,380.178238695006));
#124333=CARTESIAN_POINT('',(-86.2654713137621,1067.7251047501,380.178238695006));
#124334=CARTESIAN_POINT('Origin',(-86.2654713137621,1082.7251047501,380.853682816142));
#124335=CARTESIAN_POINT('Ctrl Pts',(-86.2654713137625,1076.32506388483,
380.178238695006));
#124336=CARTESIAN_POINT('Ctrl Pts',(-86.1770509574414,1076.33026945905,
380.178238695006));
#124337=CARTESIAN_POINT('Ctrl Pts',(-86.0895006637669,1076.33589992213,
380.195600640667));
#124338=CARTESIAN_POINT('Ctrl Pts',(-85.9669065670266,1076.34448117668,
380.246195871646));
#124339=CARTESIAN_POINT('Ctrl Pts',(-85.9277742439781,1076.34734529568,
380.267046474723));
#124340=CARTESIAN_POINT('Ctrl Pts',(-85.8159507223342,1076.35592662903,
380.341549771814));
#124341=CARTESIAN_POINT('Ctrl Pts',(-85.7516777695141,1076.36143430001,
380.406051840836));
#124342=CARTESIAN_POINT('Ctrl Pts',(-85.6524526681669,1076.37131553153,
380.556200724508));
#124343=CARTESIAN_POINT('Ctrl Pts',(-85.6183599087259,1076.37559710457,
380.640266770774));
#124344=CARTESIAN_POINT('Ctrl Pts',(-85.5850873944973,1076.3824166311,380.816788623762));
#124345=CARTESIAN_POINT('Ctrl Pts',(-85.5862070859935,1076.38488938295,
380.907467173279));
#124346=CARTESIAN_POINT('Ctrl Pts',(-85.6238764233128,1076.38772183095,
381.083147878936));
#124347=CARTESIAN_POINT('Ctrl Pts',(-85.6600581347183,1076.38805288534,
381.166371898665));
#124348=CARTESIAN_POINT('Ctrl Pts',(-85.7628554500964,1076.38651252053,
381.313761929224));
#124349=CARTESIAN_POINT('Ctrl Pts',(-85.8284231525437,1076.38465683894,
381.376442053706));
#124350=CARTESIAN_POINT('Ctrl Pts',(-85.9802096773907,1076.37895394214,
381.472487243089));
#124351=CARTESIAN_POINT('Ctrl Pts',(-86.0649071745352,1076.37516222332,
381.504878057641));
#124352=CARTESIAN_POINT('Ctrl Pts',(-86.1905403956323,1076.36871995438,
381.526012303071));
#124353=CARTESIAN_POINT('Ctrl Pts',(-86.2280206704145,1076.36670101505,
381.529126937278));
#124354=CARTESIAN_POINT('Ctrl Pts',(-86.2654713137621,1076.36458696229,
381.529126937278));
#124355=CARTESIAN_POINT('Origin',(-87.6738908373841,1067.7251047501,367.075634650624));
#124356=CARTESIAN_POINT('',(-87.6738908374021,1075.59148954561,365.976803514631));
#124357=CARTESIAN_POINT('',(-87.6738908373841,1067.7251047501,365.976803514631));
#124358=CARTESIAN_POINT('Ctrl Pts',(-87.6734743951659,1075.7170825134,368.174465707703));
#124359=CARTESIAN_POINT('Ctrl Pts',(-87.819343312233,1075.70465571775,368.174520990065));
#124360=CARTESIAN_POINT('Ctrl Pts',(-87.9636575725919,1075.6906511942,368.145532263478));
#124361=CARTESIAN_POINT('Ctrl Pts',(-88.1639583242107,1075.66858130876,
368.061723796441));
#124362=CARTESIAN_POINT('Ctrl Pts',(-88.2270334907758,1075.66117542291,
368.027773599668));
#124363=CARTESIAN_POINT('Ctrl Pts',(-88.4086864406982,1075.63838489597,
367.905823706016));
#124364=CARTESIAN_POINT('Ctrl Pts',(-88.5132999336648,1075.62309825929,
367.799900398979));
#124365=CARTESIAN_POINT('Ctrl Pts',(-88.6729366183675,1075.59481458622,
367.555450155456));
#124366=CARTESIAN_POINT('Ctrl Pts',(-88.7273878484798,1075.58204853035,
367.419926572265));
#124367=CARTESIAN_POINT('Ctrl Pts',(-88.7804597333168,1075.56065085913,
367.136108631691));
#124368=CARTESIAN_POINT('Ctrl Pts',(-88.7788827440092,1075.55220640037,
366.990645907562));
#124369=CARTESIAN_POINT('Ctrl Pts',(-88.7197058693303,1075.54090098764,
366.709236914304));
#124370=CARTESIAN_POINT('Ctrl Pts',(-88.6630334350074,1075.53812041122,
366.576030986879));
#124371=CARTESIAN_POINT('Ctrl Pts',(-88.5018533127044,1075.5386369226,366.339176513656));
#124372=CARTESIAN_POINT('Ctrl Pts',(-88.3990911692971,1075.54191181696,
366.237815058458));
#124373=CARTESIAN_POINT('Ctrl Pts',(-88.160345480136,1075.55407916221,366.07998436106));
#124374=CARTESIAN_POINT('Ctrl Pts',(-88.0266449019473,1075.56286283703,
366.02518536982));
#124375=CARTESIAN_POINT('Ctrl Pts',(-87.7451843872829,1075.58475377391,
365.969720362314));
#124376=CARTESIAN_POINT('Ctrl Pts',(-87.6000649909103,1075.59767257472,
365.96991986028));
#124377=CARTESIAN_POINT('Ctrl Pts',(-87.3175958345444,1075.62587011806,
366.026189090554));
#124378=CARTESIAN_POINT('Ctrl Pts',(-87.1829606302508,1075.64089300229,
366.082032503143));
#124379=CARTESIAN_POINT('Ctrl Pts',(-86.9415902402265,1075.6711193491,366.243468766865));
#124380=CARTESIAN_POINT('Ctrl Pts',(-86.8375236448611,1075.68603306015,
366.348108637216));
#124381=CARTESIAN_POINT('Ctrl Pts',(-86.6768162114639,1075.71350487496,
366.591463032114));
#124382=CARTESIAN_POINT('Ctrl Pts',(-86.6214830441957,1075.72581151788,
366.727644750228));
#124383=CARTESIAN_POINT('Ctrl Pts',(-86.5671441103932,1075.74631830682,
367.014025689984));
#124384=CARTESIAN_POINT('Ctrl Pts',(-86.5687179818675,1075.75431392225,
367.161369995145));
#124385=CARTESIAN_POINT('Ctrl Pts',(-86.6292282425146,1075.76490486689,
367.445891003711));
#124386=CARTESIAN_POINT('Ctrl Pts',(-86.6870868365479,1075.76743884215,
367.580267337248));
#124387=CARTESIAN_POINT('Ctrl Pts',(-86.8507785005654,1075.76677452854,
367.817567181624));
#124388=CARTESIAN_POINT('Ctrl Pts',(-86.9544469095452,1075.76364524551,
367.918455254543));
#124389=CARTESIAN_POINT('Ctrl Pts',(-87.1968443215546,1075.75198819898,
368.07621785947));
#124390=CARTESIAN_POINT('Ctrl Pts',(-87.3337235930814,1075.74347543984,
368.130599225017));
#124391=CARTESIAN_POINT('Ctrl Pts',(-87.5419143744327,1075.7279425631,368.168499682902));
#124392=CARTESIAN_POINT('Ctrl Pts',(-87.6076419361123,1075.72269088105,
368.174440758085));
#124393=CARTESIAN_POINT('Ctrl Pts',(-87.673474395166,1075.7170825134,368.174465707703));
#124394=CARTESIAN_POINT('Origin',(-87.6738908373841,1067.7251047501,367.075634650624));
#124395=CARTESIAN_POINT('',(-87.6738908373841,1075.68376086233,367.574465786616));
#124396=CARTESIAN_POINT('',(-87.6738908373842,1075.62676689012,366.576803514631));
#124397=CARTESIAN_POINT('Ctrl Pts',(-87.6738908373841,1075.68376086233,
367.574465786616));
#124398=CARTESIAN_POINT('Ctrl Pts',(-87.6769953171298,1075.68349322266,
367.574465786616));
#124399=CARTESIAN_POINT('Ctrl Pts',(-87.6801009614361,1075.68322380588,
367.574436805534));
#124400=CARTESIAN_POINT('Ctrl Pts',(-87.7496697673629,1075.67715100789,
367.573137261163));
#124401=CARTESIAN_POINT('Ctrl Pts',(-87.8151691130928,1075.67066331402,
367.558625056895));
#124402=CARTESIAN_POINT('Ctrl Pts',(-87.9055907621926,1075.66053419269,
367.518584251856));
#124403=CARTESIAN_POINT('Ctrl Pts',(-87.9339536640393,1075.65715335191,
367.502549366014));
#124404=CARTESIAN_POINT('Ctrl Pts',(-88.0151640038816,1075.64682142456,
367.445523969457));
#124405=CARTESIAN_POINT('Ctrl Pts',(-88.061552503808,1075.63995957008,367.396588511813));
#124406=CARTESIAN_POINT('Ctrl Pts',(-88.1319807875865,1075.62729936569,
367.283863784303));
#124407=CARTESIAN_POINT('Ctrl Pts',(-88.1555546455449,1075.62161404733,
367.221313695564));
#124408=CARTESIAN_POINT('Ctrl Pts',(-88.1767238053739,1075.61223872528,
367.09150150772));
#124409=CARTESIAN_POINT('Ctrl Pts',(-88.1744934763366,1075.60861202125,
367.025583724268));
#124410=CARTESIAN_POINT('Ctrl Pts',(-88.1447600013157,1075.60387016661,
366.898589417079));
#124411=CARTESIAN_POINT('Ctrl Pts',(-88.1176848205915,1075.60278928111,
366.8387486077));
#124412=CARTESIAN_POINT('Ctrl Pts',(-88.0421128711325,1075.60332914552,
366.73290012093));
#124413=CARTESIAN_POINT('Ctrl Pts',(-87.9944058423625,1075.6049400738,366.687927485667));
#124414=CARTESIAN_POINT('Ctrl Pts',(-87.884326747752,1075.6106538794,366.618699183331));
#124415=CARTESIAN_POINT('Ctrl Pts',(-87.822999222578,1075.61470748199,366.595193289664));
#124416=CARTESIAN_POINT('Ctrl Pts',(-87.7309262673952,1075.62189435976,
366.579259278205));
#124417=CARTESIAN_POINT('Ctrl Pts',(-87.7025481394435,1075.62424984986,
366.576817171752));
#124418=CARTESIAN_POINT('Ctrl Pts',(-87.6741295580651,1075.62674591951,
366.576803571751));
#124419=CARTESIAN_POINT('Ctrl Pts',(-87.674049983502,1075.62675290873,366.576803533669));
#124420=CARTESIAN_POINT('Ctrl Pts',(-87.6739704099395,1075.62675989893,
366.576803514631));
#124421=CARTESIAN_POINT('Ctrl Pts',(-87.6738908373843,1075.62676689012,
366.576803514631));
#124422=CARTESIAN_POINT('',(-87.6738908373841,1082.7251047501,366.576803514631));
#124423=CARTESIAN_POINT('',(-87.6738908373841,1067.7251047501,366.576803514631));
#124424=CARTESIAN_POINT('Origin',(-87.6738908373841,1082.7251047501,367.075634650624));
#124425=CARTESIAN_POINT('Ctrl Pts',(-87.6738908373843,1075.62676689012,
366.576803514631));
#124426=CARTESIAN_POINT('Ctrl Pts',(-87.6084744953582,1075.63251432502,
366.576803514631));
#124427=CARTESIAN_POINT('Ctrl Pts',(-87.5437388459447,1075.63892740047,
366.589670546865));
#124428=CARTESIAN_POINT('Ctrl Pts',(-87.4218180103966,1075.65246164864,
366.640058854636));
#124429=CARTESIAN_POINT('Ctrl Pts',(-87.3659830474847,1075.65946279612,
366.677563307127));
#124430=CARTESIAN_POINT('Ctrl Pts',(-87.272497503493,1075.6729528367,366.772120662268));
#124431=CARTESIAN_POINT('Ctrl Pts',(-87.2356857889018,1075.67931362939,
366.828194063365));
#124432=CARTESIAN_POINT('Ctrl Pts',(-87.1862113655451,1075.69055153046,
366.951500387343));
#124433=CARTESIAN_POINT('Ctrl Pts',(-87.1740123991004,1075.69531957854,
367.017500520854));
#124434=CARTESIAN_POINT('Ctrl Pts',(-87.1762354342323,1075.70257536774,
367.149793398211));
#124435=CARTESIAN_POINT('Ctrl Pts',(-87.1903430344116,1075.70501561211,
367.214750349486));
#124436=CARTESIAN_POINT('Ctrl Pts',(-87.2426809623601,1075.70727323407,
367.334701272723));
#124437=CARTESIAN_POINT('Ctrl Pts',(-87.2800698378778,1075.70710257816,
367.388622980891));
#124438=CARTESIAN_POINT('Ctrl Pts',(-87.3735040727621,1075.7041932488,367.479169595807));
#124439=CARTESIAN_POINT('Ctrl Pts',(-87.428652808903,1075.70147855512,367.51486012164));
#124440=CARTESIAN_POINT('Ctrl Pts',(-87.5479317826372,1075.69392442781,
367.562446644088));
#124441=CARTESIAN_POINT('Ctrl Pts',(-87.6106698370051,1075.68921119508,
367.574465786616));
#124442=CARTESIAN_POINT('Ctrl Pts',(-87.6738908373841,1075.68376086233,
367.574465786616));
#124443=CARTESIAN_POINT('Origin',(-86.223297681347,1067.7251047501,353.164138162982));
#124444=CARTESIAN_POINT('',(-86.2232976813637,1074.70656460683,352.073597414254));
#124445=CARTESIAN_POINT('',(-86.223297681347,1067.7251047501,352.073597414254));
#124446=CARTESIAN_POINT('Ctrl Pts',(-86.2233677532852,1074.89498441646,
354.254678909459));
#124447=CARTESIAN_POINT('Ctrl Pts',(-86.368344875043,1074.88010584553,354.254669594055));
#124448=CARTESIAN_POINT('Ctrl Pts',(-86.5116511349023,1074.86288057737,
354.22575525816));
#124449=CARTESIAN_POINT('Ctrl Pts',(-86.7104163792378,1074.83515588272,
354.142417373206));
#124450=CARTESIAN_POINT('Ctrl Pts',(-86.7730009159911,1074.82576075823,
354.10866651405));
#124451=CARTESIAN_POINT('Ctrl Pts',(-86.8909172515992,1074.8066630244,354.029372714505));
#124452=CARTESIAN_POINT('Ctrl Pts',(-86.9459561835566,1074.79700205051,
353.983961631481));
#124453=CARTESIAN_POINT('Ctrl Pts',(-87.0995725072276,1074.76758689865,
353.829646561973));
#124454=CARTESIAN_POINT('Ctrl Pts',(-87.1810712521107,1074.74825609641,
353.705899263475));
#124455=CARTESIAN_POINT('Ctrl Pts',(-87.2890357889482,1074.71331643717,
353.436335052299));
#124456=CARTESIAN_POINT('Ctrl Pts',(-87.31566387096,1074.6979657045,353.293605735661));
#124457=CARTESIAN_POINT('Ctrl Pts',(-87.3118383319029,1074.6731550123,353.007029673786));
#124458=CARTESIAN_POINT('Ctrl Pts',(-87.2819977757527,1074.6638825771,352.866020866224));
#124459=CARTESIAN_POINT('Ctrl Pts',(-87.1698735233297,1074.65271742962,
352.604358888485));
#124460=CARTESIAN_POINT('Ctrl Pts',(-87.0891892390927,1074.65087475215,
352.486187985245));
#124461=CARTESIAN_POINT('Ctrl Pts',(-86.8872485135896,1074.65485404087,
352.28751481358));
#124462=CARTESIAN_POINT('Ctrl Pts',(-86.7681391494087,1074.66061843664,
352.208957451225));
#124463=CARTESIAN_POINT('Ctrl Pts',(-86.5060753862408,1074.67901964644,
352.101358585668));
#124464=CARTESIAN_POINT('Ctrl Pts',(-86.3656006334892,1074.69151155488,
352.073688597946));
#124465=CARTESIAN_POINT('Ctrl Pts',(-86.0809227651831,1074.72162523263,
352.07350573436));
#124466=CARTESIAN_POINT('Ctrl Pts',(-85.9394289842916,1074.73900736629,
352.101567128908));
#124467=CARTESIAN_POINT('Ctrl Pts',(-85.7412472838941,1074.76692708733,
352.183298954599));
#124468=CARTESIAN_POINT('Ctrl Pts',(-85.6778517635491,1074.7765025099,352.217089791856));
#124469=CARTESIAN_POINT('Ctrl Pts',(-85.5588289393753,1074.79581686684,
352.296462570153));
#124470=CARTESIAN_POINT('Ctrl Pts',(-85.5034449821349,1074.80551182402,
352.341828958228));
#124471=CARTESIAN_POINT('Ctrl Pts',(-85.3502759860123,1074.83462368291,
352.494710311079));
#124472=CARTESIAN_POINT('Ctrl Pts',(-85.2690056712539,1074.85349436744,
352.616680404154));
#124473=CARTESIAN_POINT('Ctrl Pts',(-85.1593032350647,1074.88769575649,
352.884772454204));
#124474=CARTESIAN_POINT('Ctrl Pts',(-85.1316110871613,1074.90272070902,
353.028172840797));
#124475=CARTESIAN_POINT('Ctrl Pts',(-85.1339738033433,1074.92701700662,
353.317706236598));
#124476=CARTESIAN_POINT('Ctrl Pts',(-85.1639327013078,1074.93605189535,
353.460901381754));
#124477=CARTESIAN_POINT('Ctrl Pts',(-85.2770016280364,1074.94676759518,
353.724376683253));
#124478=CARTESIAN_POINT('Ctrl Pts',(-85.3577098365307,1074.94850940341,
353.842463017781));
#124479=CARTESIAN_POINT('Ctrl Pts',(-85.5599368404702,1074.94469892628,
354.04126579189));
#124480=CARTESIAN_POINT('Ctrl Pts',(-85.6794317190385,1074.93917903281,
354.119930596787));
#124481=CARTESIAN_POINT('Ctrl Pts',(-85.9417525597329,1074.92149346684,
354.227210035181));
#124482=CARTESIAN_POINT('Ctrl Pts',(-86.082003853221,1074.90949217319,354.254687992699));
#124483=CARTESIAN_POINT('Ctrl Pts',(-86.2233677532852,1074.89498441646,
354.254678909459));
#124484=CARTESIAN_POINT('Origin',(-86.223297681347,1067.7251047501,353.164138162982));
#124485=CARTESIAN_POINT('',(-86.223297681347,1074.84430822541,353.654678911711));
#124486=CARTESIAN_POINT('',(-86.223297681347,1074.75955377087,352.673597414254));
#124487=CARTESIAN_POINT('Ctrl Pts',(-86.223297681347,1074.84430822541,353.654678911711));
#124488=CARTESIAN_POINT('Ctrl Pts',(-86.2235616057638,1074.84428090512,
353.654678911711));
#124489=CARTESIAN_POINT('Ctrl Pts',(-86.2238255387521,1074.84425356549,
353.654678698713));
#124490=CARTESIAN_POINT('Ctrl Pts',(-86.2895776205274,1074.8374380034,353.654572565875));
#124491=CARTESIAN_POINT('Ctrl Pts',(-86.3542861322824,1074.82959371022,
353.641356063634));
#124492=CARTESIAN_POINT('Ctrl Pts',(-86.4439064652634,1074.81701539543,
353.603440338078));
#124493=CARTESIAN_POINT('Ctrl Pts',(-86.4720819309782,1074.81276372674,
353.588118861306));
#124494=CARTESIAN_POINT('Ctrl Pts',(-86.5250816008154,1074.80414390752,
353.552189237157));
#124495=CARTESIAN_POINT('Ctrl Pts',(-86.549780679976,1074.79979483259,353.531651378652));
#124496=CARTESIAN_POINT('Ctrl Pts',(-86.6184848412624,1074.78660945671,
353.462092690839));
#124497=CARTESIAN_POINT('Ctrl Pts',(-86.6548482908479,1074.77798532736,
353.406480662891));
#124498=CARTESIAN_POINT('Ctrl Pts',(-86.7031609604075,1074.76236519994,
353.284902225443));
#124499=CARTESIAN_POINT('Ctrl Pts',(-86.7149612752407,1074.75549914626,
353.220242998242));
#124500=CARTESIAN_POINT('Ctrl Pts',(-86.7125683266654,1074.74449113462,
353.090998295684));
#124501=CARTESIAN_POINT('Ctrl Pts',(-86.6988418164033,1074.74041282319,
353.027698486224));
#124502=CARTESIAN_POINT('Ctrl Pts',(-86.647870655823,1074.73553498482,352.910308239208));
#124503=CARTESIAN_POINT('Ctrl Pts',(-86.6113299191538,1074.73475915941,
352.857335800884));
#124504=CARTESIAN_POINT('Ctrl Pts',(-86.5200480541649,1074.73660923987,
352.768378295057));
#124505=CARTESIAN_POINT('Ctrl Pts',(-86.466260113021,1074.7392118728,352.733278000128));
#124506=CARTESIAN_POINT('Ctrl Pts',(-86.3487726254677,1074.74742840115,
352.685726662078));
#124507=CARTESIAN_POINT('Ctrl Pts',(-86.2862830539244,1074.75294285452,
352.673599117021));
#124508=CARTESIAN_POINT('Ctrl Pts',(-86.2233109440985,1074.7595523788,352.673597414443));
#124509=CARTESIAN_POINT('Ctrl Pts',(-86.223306523178,1074.75955284282,352.673597414323));
#124510=CARTESIAN_POINT('Ctrl Pts',(-86.2233021022608,1074.75955330684,
352.673597414254));
#124511=CARTESIAN_POINT('Ctrl Pts',(-86.223297681347,1074.75955377087,352.673597414254));
#124512=CARTESIAN_POINT('',(-86.223297681347,1082.7251047501,352.673597414254));
#124513=CARTESIAN_POINT('',(-86.223297681347,1067.7251047501,352.673597414254));
#124514=CARTESIAN_POINT('Origin',(-86.223297681347,1082.7251047501,353.164138162982));
#124515=CARTESIAN_POINT('Ctrl Pts',(-86.223297681347,1074.75955377087,352.673597414254));
#124516=CARTESIAN_POINT('Ctrl Pts',(-86.1588957466318,1074.76631351889,
352.673597414254));
#124517=CARTESIAN_POINT('Ctrl Pts',(-86.0952156099574,1074.7740892792,352.686278215375));
#124518=CARTESIAN_POINT('Ctrl Pts',(-86.0061506826996,1074.78659502971,
352.723103946718));
#124519=CARTESIAN_POINT('Ctrl Pts',(-85.9777275016174,1074.79087817074,
352.738276741612));
#124520=CARTESIAN_POINT('Ctrl Pts',(-85.9243073248254,1074.79953640906,
352.773926837269));
#124521=CARTESIAN_POINT('Ctrl Pts',(-85.8994258824298,1074.8038919747,352.794317643984));
#124522=CARTESIAN_POINT('Ctrl Pts',(-85.8304291692944,1074.81702219254,
352.863202457608));
#124523=CARTESIAN_POINT('Ctrl Pts',(-85.7938052904732,1074.82556721703,
352.91825082026));
#124524=CARTESIAN_POINT('Ctrl Pts',(-85.744424273489,1074.84109704224,353.039360492071));
#124525=CARTESIAN_POINT('Ctrl Pts',(-85.7320488061634,1074.84793826289,
353.104205426397));
#124526=CARTESIAN_POINT('Ctrl Pts',(-85.7335174022278,1074.85892494984,
353.234245441724));
#124527=CARTESIAN_POINT('Ctrl Pts',(-85.7469894804082,1074.86299706639,
353.298126973912));
#124528=CARTESIAN_POINT('Ctrl Pts',(-85.7976627926436,1074.86786162508,
353.416181240793));
#124529=CARTESIAN_POINT('Ctrl Pts',(-85.8339757250197,1074.86865593611,
353.469300526993));
#124530=CARTESIAN_POINT('Ctrl Pts',(-85.9249247406229,1074.86691646873,
353.558687620525));
#124531=CARTESIAN_POINT('Ctrl Pts',(-85.9786346967291,1074.86440039348,
353.594046282404));
#124532=CARTESIAN_POINT('Ctrl Pts',(-86.0965964857103,1074.85635183583,
353.642310203414));
#124533=CARTESIAN_POINT('Ctrl Pts',(-86.1596982074619,1074.85089176023,
353.654678911711));
#124534=CARTESIAN_POINT('Ctrl Pts',(-86.223297681347,1074.84430822541,353.654678911711));
#124535=CARTESIAN_POINT('Origin',(-88.5622696992325,1067.7251047501,411.301056626764));
#124536=CARTESIAN_POINT('',(-88.5622696992586,1076.66670986628,409.822753494571));
#124537=CARTESIAN_POINT('',(-88.5622696992325,1067.7251047501,409.822753494571));
#124538=CARTESIAN_POINT('Ctrl Pts',(-88.5617321436617,1076.67820104542,
412.779359661222));
#124539=CARTESIAN_POINT('Ctrl Pts',(-88.6593215347776,1076.67579673124,
412.779395147668));
#124540=CARTESIAN_POINT('Ctrl Pts',(-88.7566727307759,1076.67328588799,
412.769767089839));
#124541=CARTESIAN_POINT('Ctrl Pts',(-89.042583966656,1076.66557155864,412.712549655407));
#124542=CARTESIAN_POINT('Ctrl Pts',(-89.2234665533449,1076.66022627971,
412.637407100015));
#124543=CARTESIAN_POINT('Ctrl Pts',(-89.5459795296261,1076.6498915022,412.421493205337));
#124544=CARTESIAN_POINT('Ctrl Pts',(-89.6844588836696,1076.64500852948,
412.282771260311));
#124545=CARTESIAN_POINT('Ctrl Pts',(-89.8998609967692,1076.63669979489,
411.959768945481));
#124546=CARTESIAN_POINT('Ctrl Pts',(-89.9747075202018,1076.63336149731,
411.778637893389));
#124547=CARTESIAN_POINT('Ctrl Pts',(-90.0500502281694,1076.6289920861,411.398152893131));
#124548=CARTESIAN_POINT('Ctrl Pts',(-90.0499578729967,1076.62800326179,
411.202532384846));
#124549=CARTESIAN_POINT('Ctrl Pts',(-89.9744103265577,1076.6286195008,410.822940806752));
#124550=CARTESIAN_POINT('Ctrl Pts',(-89.8998750714784,1076.63021145483,
410.642618530076));
#124551=CARTESIAN_POINT('Ctrl Pts',(-89.6857907183491,1076.63563055537,
410.321087709615));
#124552=CARTESIAN_POINT('Ctrl Pts',(-89.5483835651257,1076.6393976063,410.182930557444));
#124553=CARTESIAN_POINT('Ctrl Pts',(-89.2281854038617,1076.64831647696,
409.967179654828));
#124554=CARTESIAN_POINT('Ctrl Pts',(-89.0484431140305,1076.65337636157,
409.891695090916));
#124555=CARTESIAN_POINT('Ctrl Pts',(-88.6699221160384,1076.66382623327,
409.814059840246));
#124556=CARTESIAN_POINT('Ctrl Pts',(-88.4747593446922,1076.66911090161,
409.812737768367));
#124557=CARTESIAN_POINT('Ctrl Pts',(-88.0920481922756,1076.67915233789,
409.885849219094));
#124558=CARTESIAN_POINT('Ctrl Pts',(-87.9084634367413,1076.68379948386,
409.960733286966));
#124559=CARTESIAN_POINT('Ctrl Pts',(-87.5824741873546,1076.69184601093,
410.177061009378));
#124560=CARTESIAN_POINT('Ctrl Pts',(-87.4429740478766,1076.69518140116,
410.315890982764));
#124561=CARTESIAN_POINT('Ctrl Pts',(-87.2256775268126,1076.70046426318,
410.639973285762));
#124562=CARTESIAN_POINT('Ctrl Pts',(-87.1501329207538,1076.70236580788,
410.82211529469));
#124563=CARTESIAN_POINT('Ctrl Pts',(-87.0740410935017,1076.70479706172,
411.206062452591));
#124564=CARTESIAN_POINT('Ctrl Pts',(-87.0745786619321,1076.70530259369,
411.404134500205));
#124565=CARTESIAN_POINT('Ctrl Pts',(-87.1528946154287,1076.7049395419,411.788341793998));
#124566=CARTESIAN_POINT('Ctrl Pts',(-87.2298311414188,1076.70407471558,
411.970675986506));
#124567=CARTESIAN_POINT('Ctrl Pts',(-87.4498085532559,1076.70090442615,
412.293961508813));
#124568=CARTESIAN_POINT('Ctrl Pts',(-87.5903808308169,1076.69862961784,
412.431921643145));
#124569=CARTESIAN_POINT('Ctrl Pts',(-87.9169957376771,1076.69260314726,
412.645328977771));
#124570=CARTESIAN_POINT('Ctrl Pts',(-88.0998395526459,1076.68890193453,
412.718658746031));
#124571=CARTESIAN_POINT('Ctrl Pts',(-88.380707200547,1076.68256419721,412.770963442842));
#124572=CARTESIAN_POINT('Ctrl Pts',(-88.4711236397969,1076.68043337116,
412.779326713237));
#124573=CARTESIAN_POINT('Ctrl Pts',(-88.5617321436617,1076.67820104542,
412.779359661222));
#124574=CARTESIAN_POINT('Origin',(-88.5622696992325,1067.7251047501,411.301056626764));
#124575=CARTESIAN_POINT('',(-88.5622696992324,1076.67614304338,412.179359758958));
#124576=CARTESIAN_POINT('',(-88.5622696992325,1076.6693343871,410.422753494571));
#124577=CARTESIAN_POINT('Ctrl Pts',(-88.5622696992324,1076.67614304338,
412.179359758958));
#124578=CARTESIAN_POINT('Ctrl Pts',(-88.5713478733904,1076.67591538937,
412.179359758958));
#124579=CARTESIAN_POINT('Ctrl Pts',(-88.5804283472778,1076.67568649302,
412.179219010571));
#124580=CARTESIAN_POINT('Ctrl Pts',(-88.6474792402766,1076.67398748811,
412.177138610937));
#124581=CARTESIAN_POINT('Ctrl Pts',(-88.7051293905032,1076.67247775111,
412.169602100923));
#124582=CARTESIAN_POINT('Ctrl Pts',(-88.8737893149981,1076.66791373208,
412.130296477369));
#124583=CARTESIAN_POINT('Ctrl Pts',(-88.9797364074945,1076.6648459483,412.082341167464));
#124584=CARTESIAN_POINT('Ctrl Pts',(-89.1671040340671,1076.65906117588,
411.948255948921));
#124585=CARTESIAN_POINT('Ctrl Pts',(-89.2467038093409,1076.65640251678,
411.863413100359));
#124586=CARTESIAN_POINT('Ctrl Pts',(-89.368581097211,1076.65197505532,411.667862894601));
#124587=CARTESIAN_POINT('Ctrl Pts',(-89.4096903733426,1076.6502514299,411.559061855057));
#124588=CARTESIAN_POINT('Ctrl Pts',(-89.4475377483728,1076.64808248081,
411.331937846654));
#124589=CARTESIAN_POINT('Ctrl Pts',(-89.4439674757885,1076.64765798086,
411.215831833517));
#124590=CARTESIAN_POINT('Ctrl Pts',(-89.3923040979717,1076.6482028578,410.991770890877));
#124591=CARTESIAN_POINT('Ctrl Pts',(-89.3447778078736,1076.64916448576,
410.88597406025));
#124592=CARTESIAN_POINT('Ctrl Pts',(-89.2117409049548,1076.65229599655,
410.698740149001));
#124593=CARTESIAN_POINT('Ctrl Pts',(-89.1275355879964,1076.65443295928,
410.619097196889));
#124594=CARTESIAN_POINT('Ctrl Pts',(-88.9332206535198,1076.65949516651,
410.49669052188));
#124595=CARTESIAN_POINT('Ctrl Pts',(-88.8249678993894,1076.66236952584,
410.455127182263));
#124596=CARTESIAN_POINT('Ctrl Pts',(-88.6624094006598,1076.6666814505,410.427042847244));
#124597=CARTESIAN_POINT('Ctrl Pts',(-88.612385243038,1076.66800807202,410.422753494571));
#124598=CARTESIAN_POINT('Ctrl Pts',(-88.5622696992325,1076.6693343871,410.422753494571));
#124599=CARTESIAN_POINT('',(-88.5622696992325,1082.7251047501,410.422753494571));
#124600=CARTESIAN_POINT('',(-88.5622696992325,1067.7251047501,410.422753494571));
#124601=CARTESIAN_POINT('Origin',(-88.5622696992325,1082.7251047501,411.301056626764));
#124602=CARTESIAN_POINT('Ctrl Pts',(-88.5622696992325,1076.6693343871,410.422753494571));
#124603=CARTESIAN_POINT('Ctrl Pts',(-88.5621479139323,1076.66933761017,
410.422753494571));
#124604=CARTESIAN_POINT('Ctrl Pts',(-88.5620261280924,1076.66934083323,
410.422753519901));
#124605=CARTESIAN_POINT('Ctrl Pts',(-88.5619043417208,1076.6693440563,410.422753570562));
#124606=CARTESIAN_POINT('Ctrl Pts',(-88.5044934230413,1076.67086343007,
410.422777452422));
#124607=CARTESIAN_POINT('Ctrl Pts',(-88.447222416631,1076.67237543949,410.428430336649));
#124608=CARTESIAN_POINT('Ctrl Pts',(-88.2762036933014,1076.67687629903,
410.46244962376));
#124609=CARTESIAN_POINT('Ctrl Pts',(-88.167193098939,1076.67972253554,410.507953514121));
#124610=CARTESIAN_POINT('Ctrl Pts',(-87.9738090385764,1076.68478130384,
410.638714698088));
#124611=CARTESIAN_POINT('Ctrl Pts',(-87.8912507914937,1076.68694853699,
410.722507068956));
#124612=CARTESIAN_POINT('Ctrl Pts',(-87.763563118689,1076.69043999321,410.917539359605));
#124613=CARTESIAN_POINT('Ctrl Pts',(-87.7197486379689,1076.69173149826,
411.026870139116));
#124614=CARTESIAN_POINT('Ctrl Pts',(-87.6773361005266,1076.69336831006,
411.256548822462));
#124615=CARTESIAN_POINT('Ctrl Pts',(-87.6792766294144,1076.69369681906,
411.37462478389));
#124616=CARTESIAN_POINT('Ctrl Pts',(-87.7292636477229,1076.69336814375,
411.603004899497));
#124617=CARTESIAN_POINT('Ctrl Pts',(-87.7767813386656,1076.69271443728,
411.711030619459));
#124618=CARTESIAN_POINT('Ctrl Pts',(-87.9111132566874,1076.6904414756,411.901882998739));
#124619=CARTESIAN_POINT('Ctrl Pts',(-87.9964854077183,1076.68884491687,
411.98287954438));
#124620=CARTESIAN_POINT('Ctrl Pts',(-88.1938844886558,1076.68478930375,
412.106846868462));
#124621=CARTESIAN_POINT('Ctrl Pts',(-88.3039599660869,1076.6823672592,412.148569736987));
#124622=CARTESIAN_POINT('Ctrl Pts',(-88.466341671572,1076.67851541078,412.175425510553));
#124623=CARTESIAN_POINT('Ctrl Pts',(-88.51427354557,1076.67734664628,412.179359758958));
#124624=CARTESIAN_POINT('Ctrl Pts',(-88.5622696992324,1076.67614304338,
412.179359758958));
#124625=CARTESIAN_POINT('Origin',(-93.4799432334773,1067.7251047501,399.745687154642));
#124626=CARTESIAN_POINT('',(-93.4799432334936,1076.32318567709,398.470243033506));
#124627=CARTESIAN_POINT('',(-93.4799432334773,1067.7251047501,398.470243033506));
#124628=CARTESIAN_POINT('Ctrl Pts',(-93.4801333950918,1076.36560796598,
401.021131261602));
#124629=CARTESIAN_POINT('Ctrl Pts',(-93.5629569069197,1076.36054728635,
401.021118913078));
#124630=CARTESIAN_POINT('Ctrl Pts',(-93.6455745583778,1076.35532421901,
401.013039155634));
#124631=CARTESIAN_POINT('Ctrl Pts',(-93.8095771701939,1076.34459454335,
400.980683159562));
#124632=CARTESIAN_POINT('Ctrl Pts',(-93.8905125998491,1076.33911044844,
400.9561853359));
#124633=CARTESIAN_POINT('Ctrl Pts',(-94.1232432929026,1076.32276821168,
400.859692860781));
#124634=CARTESIAN_POINT('Ctrl Pts',(-94.2639251192673,1076.31209976449,
400.765607436634));
#124635=CARTESIAN_POINT('Ctrl Pts',(-94.5007585398004,1076.29253532213,
400.52846982775));
#124636=CARTESIAN_POINT('Ctrl Pts',(-94.5946705888021,1076.28383022148,
400.387746201942));
#124637=CARTESIAN_POINT('Ctrl Pts',(-94.7225496399746,1076.26979329303,
400.07831192922));
#124638=CARTESIAN_POINT('Ctrl Pts',(-94.75542733347,1076.26459362006,399.912686407884));
#124639=CARTESIAN_POINT('Ctrl Pts',(-94.7553474338139,1076.25858411173,
399.578625581044));
#124640=CARTESIAN_POINT('Ctrl Pts',(-94.7226047752679,1076.25782102401,
399.413476123076));
#124641=CARTESIAN_POINT('Ctrl Pts',(-94.5955203019502,1076.2608791342,399.105405733507));
#124642=CARTESIAN_POINT('Ctrl Pts',(-94.5025336228493,1076.26466104138,
398.965461683089));
#124643=CARTESIAN_POINT('Ctrl Pts',(-94.2680295445492,1076.27618487448,
398.729115270103));
#124644=CARTESIAN_POINT('Ctrl Pts',(-94.1287405064727,1076.28381516539,
398.635049761835));
#124645=CARTESIAN_POINT('Ctrl Pts',(-93.8216056398943,1076.30176140672,
398.505575588351));
#124646=CARTESIAN_POINT('Ctrl Pts',(-93.6566292623946,1076.31190817482,
398.471575353977));
#124647=CARTESIAN_POINT('Ctrl Pts',(-93.4063476511197,1076.32788248785,
398.469633711281));
#124648=CARTESIAN_POINT('Ctrl Pts',(-93.3229984130479,1076.33329885397,
398.477185653582));
#124649=CARTESIAN_POINT('Ctrl Pts',(-93.1590300742001,1076.34413759169,
398.508458706518));
#124650=CARTESIAN_POINT('Ctrl Pts',(-93.0787977205017,1076.34953425454,
398.532096181547));
#124651=CARTESIAN_POINT('Ctrl Pts',(-92.8446604858417,1076.36557149516,
398.626856400855));
#124652=CARTESIAN_POINT('Ctrl Pts',(-92.7020073105663,1076.37574404396,
398.720887726704));
#124653=CARTESIAN_POINT('Ctrl Pts',(-92.4621703824325,1076.39385563328,
398.958730167123));
#124654=CARTESIAN_POINT('Ctrl Pts',(-92.3671563759896,1076.40163019714,
399.100001437337));
#124655=CARTESIAN_POINT('Ctrl Pts',(-92.2374009785951,1076.41398301362,
399.411854727107));
#124656=CARTESIAN_POINT('Ctrl Pts',(-92.2041160776654,1076.41843466233,
399.57940203307));
#124657=CARTESIAN_POINT('Ctrl Pts',(-92.2048899521654,1076.42353646164,
399.918302816354));
#124658=CARTESIAN_POINT('Ctrl Pts',(-92.2391437461501,1076.42412648457,
400.086242677537));
#124659=CARTESIAN_POINT('Ctrl Pts',(-92.3712558622388,1076.42133698604,
400.398581387896));
#124660=CARTESIAN_POINT('Ctrl Pts',(-92.4676687942551,1076.41799107729,
400.53987567314));
#124661=CARTESIAN_POINT('Ctrl Pts',(-92.7095487807018,1076.40766356967,
400.776087030306));
#124662=CARTESIAN_POINT('Ctrl Pts',(-92.8524308286309,1076.40079297176,
400.868816421315));
#124663=CARTESIAN_POINT('Ctrl Pts',(-93.1590792330014,1076.38455917893,
400.990609035014));
#124664=CARTESIAN_POINT('Ctrl Pts',(-93.3189077425315,1076.37545917075,
401.021155299449));
#124665=CARTESIAN_POINT('Ctrl Pts',(-93.4801333950918,1076.36560796598,
401.021131261602));
#124666=CARTESIAN_POINT('Origin',(-93.4799432334773,1067.7251047501,399.745687154642));
#124667=CARTESIAN_POINT('',(-93.4799432334773,1076.35619778296,400.421131275778));
#124668=CARTESIAN_POINT('',(-93.4799432334773,1076.33373423278,399.070243033506));
#124669=CARTESIAN_POINT('Ctrl Pts',(-93.4799432334773,1076.35619778296,
400.421131275778));
#124670=CARTESIAN_POINT('Ctrl Pts',(-93.4883532932941,1076.35567851875,
400.421131275778));
#124671=CARTESIAN_POINT('Ctrl Pts',(-93.4967694338094,1076.35515585416,
400.420974204448));
#124672=CARTESIAN_POINT('Ctrl Pts',(-93.5953782260296,1076.34899626522,
400.417286217715));
#124673=CARTESIAN_POINT('Ctrl Pts',(-93.6839797165283,1076.34310966564,
400.395870128729));
#124674=CARTESIAN_POINT('Ctrl Pts',(-93.8469288872262,1076.33156782656,
400.319772606978));
#124675=CARTESIAN_POINT('Ctrl Pts',(-93.9197814455157,1076.32602460709,
400.266074232109));
#124676=CARTESIAN_POINT('Ctrl Pts',(-94.0395870715425,1076.31610126246,
400.1341101629));
#124677=CARTESIAN_POINT('Ctrl Pts',(-94.0856782668617,1076.31180516189,
400.057409911078));
#124678=CARTESIAN_POINT('Ctrl Pts',(-94.1455327743756,1076.30504731657,
399.890727925973));
#124679=CARTESIAN_POINT('Ctrl Pts',(-94.1587945357534,1076.30264794552,
399.802401964556));
#124680=CARTESIAN_POINT('Ctrl Pts',(-94.1505032189142,1076.30012159766,
399.625819649506));
#124681=CARTESIAN_POINT('Ctrl Pts',(-94.1291125066518,1076.3000145825,399.53929278628));
#124682=CARTESIAN_POINT('Ctrl Pts',(-94.0542779032438,1076.30212357938,
399.379423555318));
#124683=CARTESIAN_POINT('Ctrl Pts',(-94.0015873571222,1076.30431699002,
399.307636848827));
#124684=CARTESIAN_POINT('Ctrl Pts',(-93.871542184645,1076.31069679075,399.188304816762));
#124685=CARTESIAN_POINT('Ctrl Pts',(-93.795413342083,1076.31482310402,399.141956126631));
#124686=CARTESIAN_POINT('Ctrl Pts',(-93.6380415729123,1076.32393226757,
399.084226239711));
#124687=CARTESIAN_POINT('Ctrl Pts',(-93.5593007106689,1076.32871601054,
399.07024530662));
#124688=CARTESIAN_POINT('Ctrl Pts',(-93.479962584241,1076.33373300911,399.070243033671));
#124689=CARTESIAN_POINT('Ctrl Pts',(-93.4799561339841,1076.333733417,399.070243033486));
#124690=CARTESIAN_POINT('Ctrl Pts',(-93.4799496837297,1076.33373382489,
399.070243033506));
#124691=CARTESIAN_POINT('Ctrl Pts',(-93.4799432334775,1076.33373423278,
399.070243033506));
#124692=CARTESIAN_POINT('',(-93.4799432334773,1082.7251047501,399.070243033506));
#124693=CARTESIAN_POINT('',(-93.4799432334773,1067.7251047501,399.070243033506));
#124694=CARTESIAN_POINT('Origin',(-93.4799432334773,1082.7251047501,399.745687154642));
#124695=CARTESIAN_POINT('Ctrl Pts',(-93.4799432334775,1076.33373423278,
399.070243033506));
#124696=CARTESIAN_POINT('Ctrl Pts',(-93.435721437085,1076.33653064493,399.070243033506));
#124697=CARTESIAN_POINT('Ctrl Pts',(-93.3916084193459,1076.33938105541,
399.074585875597));
#124698=CARTESIAN_POINT('Ctrl Pts',(-93.3049435932713,1076.34510035486,
399.091815221194));
#124699=CARTESIAN_POINT('Ctrl Pts',(-93.2625942045437,1076.34795567402,
399.104646568976));
#124700=CARTESIAN_POINT('Ctrl Pts',(-93.1387348822979,1076.35649513563,
399.155872324731));
#124701=CARTESIAN_POINT('Ctrl Pts',(-93.0633358533861,1076.36195946124,
399.20647345938));
#124702=CARTESIAN_POINT('Ctrl Pts',(-92.9368881130846,1076.37174713727,
399.334139596107));
#124703=CARTESIAN_POINT('Ctrl Pts',(-92.8870437902805,1076.37597700716,
399.409885692517));
#124704=CARTESIAN_POINT('Ctrl Pts',(-92.8198410747591,1076.38268695544,
399.576626213071));
#124705=CARTESIAN_POINT('Ctrl Pts',(-92.8032084878391,1076.38509827905,
399.665965229687));
#124706=CARTESIAN_POINT('Ctrl Pts',(-92.8059480411021,1076.38779313137,
399.846089904278));
#124707=CARTESIAN_POINT('Ctrl Pts',(-92.8253479181109,1076.38804668744,
399.935044626837));
#124708=CARTESIAN_POINT('Ctrl Pts',(-92.8978823718494,1076.38634035124,
400.100002885482));
#124709=CARTESIAN_POINT('Ctrl Pts',(-92.950244411421,1076.38439963927,400.174343344076));
#124710=CARTESIAN_POINT('Ctrl Pts',(-93.0808636745382,1076.37853760764,
400.29798447593));
#124711=CARTESIAN_POINT('Ctrl Pts',(-93.1577576535785,1076.37467765188,
400.346088105425));
#124712=CARTESIAN_POINT('Ctrl Pts',(-93.31798331091,1076.36591425995,400.40646485887));
#124713=CARTESIAN_POINT('Ctrl Pts',(-93.3986794334962,1076.36121527194,
400.421131275778));
#124714=CARTESIAN_POINT('Ctrl Pts',(-93.4799432334773,1076.35619778296,
400.421131275778));
#124715=CARTESIAN_POINT('Origin',(-99.1956712429286,1067.7251047501,372.652457095519));
#124716=CARTESIAN_POINT('',(-99.1956712429516,1074.73259927686,371.56191634679));
#124717=CARTESIAN_POINT('',(-99.1956712429286,1067.7251047501,371.56191634679));
#124718=CARTESIAN_POINT('Ctrl Pts',(-99.1952613378211,1074.86968995685,
373.742997767211));
#124719=CARTESIAN_POINT('Ctrl Pts',(-99.3408017340122,1074.85243551291,
373.743052471958));
#124720=CARTESIAN_POINT('Ctrl Pts',(-99.4847391278243,1074.83348174949,
373.713974810929));
#124721=CARTESIAN_POINT('Ctrl Pts',(-99.6843997937052,1074.80431537499,
373.629961568344));
#124722=CARTESIAN_POINT('Ctrl Pts',(-99.7472934042108,1074.79462839847,
373.595899336245));
#124723=CARTESIAN_POINT('Ctrl Pts',(-99.9280501618477,1074.76519211283,
373.473711540432));
#124724=CARTESIAN_POINT('Ctrl Pts',(-100.031958218192,1074.74591713644,
373.367679291368));
#124725=CARTESIAN_POINT('Ctrl Pts',(-100.189659947538,1074.7112567494,373.123497891547));
#124726=CARTESIAN_POINT('Ctrl Pts',(-100.243105198812,1074.69611853186,
372.988482528436));
#124727=CARTESIAN_POINT('Ctrl Pts',(-100.294165847614,1074.6718263573,372.706443612323));
#124728=CARTESIAN_POINT('Ctrl Pts',(-100.291844411895,1074.66285387972,
372.562331202692));
#124729=CARTESIAN_POINT('Ctrl Pts',(-100.231839953063,1074.65233192603,
372.284067747315));
#124730=CARTESIAN_POINT('Ctrl Pts',(-100.175253863595,1074.65082544753,
372.152661609642));
#124731=CARTESIAN_POINT('Ctrl Pts',(-100.01507247592,1074.65546506098,371.91905605327));
#124732=CARTESIAN_POINT('Ctrl Pts',(-99.9132074593707,1074.66154741341,
371.819176381304));
#124733=CARTESIAN_POINT('Ctrl Pts',(-99.6766085323472,1074.68052379203,
371.663437476209));
#124734=CARTESIAN_POINT('Ctrl Pts',(-99.5440372268615,1074.69326789544,
371.609400162372));
#124735=CARTESIAN_POINT('Ctrl Pts',(-99.2646770342454,1074.72378710895,
371.554738587819));
#124736=CARTESIAN_POINT('Ctrl Pts',(-99.1204299995402,1074.74131861624,
371.555197654905));
#124737=CARTESIAN_POINT('Ctrl Pts',(-98.9101695674117,1074.76938287174,
371.597506382811));
#124738=CARTESIAN_POINT('Ctrl Pts',(-98.8413848604377,1074.77899988353,
371.618577184547));
#124739=CARTESIAN_POINT('Ctrl Pts',(-98.709181303031,1074.79836792181,371.67382322579));
#124740=CARTESIAN_POINT('Ctrl Pts',(-98.6460451247645,1074.80807485702,
371.707835919492));
#124741=CARTESIAN_POINT('Ctrl Pts',(-98.4662524538523,1074.83716615011,
371.828863517514));
#124742=CARTESIAN_POINT('Ctrl Pts',(-98.3630814106523,1074.85595247211,
371.933263557887));
#124743=CARTESIAN_POINT('Ctrl Pts',(-98.2042354166269,1074.88983619223,
372.175804495964));
#124744=CARTESIAN_POINT('Ctrl Pts',(-98.1497567703304,1074.90463482366,
372.311365818768));
#124745=CARTESIAN_POINT('Ctrl Pts',(-98.0970469897061,1074.9283709619,372.595967805245));
#124746=CARTESIAN_POINT('Ctrl Pts',(-98.0992031312702,1074.93708574653,
372.742087826904));
#124747=CARTESIAN_POINT('Ctrl Pts',(-98.1599660416553,1074.94714886773,
373.022134517035));
#124748=CARTESIAN_POINT('Ctrl Pts',(-98.2167003806437,1074.94855697519,
373.153437943663));
#124749=CARTESIAN_POINT('Ctrl Pts',(-98.377342780694,1074.94408613779,373.387126542476));
#124750=CARTESIAN_POINT('Ctrl Pts',(-98.4796569838478,1074.93824599315,
373.48711237768));
#124751=CARTESIAN_POINT('Ctrl Pts',(-98.7192730786927,1074.91977646349,
373.644076669666));
#124752=CARTESIAN_POINT('Ctrl Pts',(-98.8548463810203,1074.90718271451,
373.698386081222));
#124753=CARTESIAN_POINT('Ctrl Pts',(-99.0623199847187,1074.88505662857,
373.73686213158));
#124754=CARTESIAN_POINT('Ctrl Pts',(-99.1287448150628,1074.87757577854,
373.742972765427));
#124755=CARTESIAN_POINT('Ctrl Pts',(-99.1952613378212,1074.86968995685,
373.742997767211));
#124756=CARTESIAN_POINT('Origin',(-99.1956712429286,1067.7251047501,372.652457095519));
#124757=CARTESIAN_POINT('',(-99.1956712429286,1074.8328201009,373.142997844247));
#124758=CARTESIAN_POINT('',(-99.1956712429286,1074.77118038462,372.16191634679));
#124759=CARTESIAN_POINT('Ctrl Pts',(-99.1956712429286,1074.8328201009,373.142997844247));
#124760=CARTESIAN_POINT('Ctrl Pts',(-99.2307558172767,1074.82863383938,
373.142997844247));
#124761=CARTESIAN_POINT('Ctrl Pts',(-99.2658013664893,1074.82421250411,
373.13923374202));
#124762=CARTESIAN_POINT('Ctrl Pts',(-99.3315287933037,1074.81545469225,
373.124898801776));
#124763=CARTESIAN_POINT('Ctrl Pts',(-99.3621030623619,1074.81117487194,
373.115012649334));
#124764=CARTESIAN_POINT('Ctrl Pts',(-99.4209335720955,1074.80251702725,
373.089399514846));
#124765=CARTESIAN_POINT('Ctrl Pts',(-99.4490523457672,1074.79815824675,
373.07371702756));
#124766=CARTESIAN_POINT('Ctrl Pts',(-99.5295155813452,1074.78498078999,
373.017850813383));
#124767=CARTESIAN_POINT('Ctrl Pts',(-99.5755408836341,1074.77640830922,
372.969759798282));
#124768=CARTESIAN_POINT('Ctrl Pts',(-99.6450929902016,1074.7610483231,372.85936697056));
#124769=CARTESIAN_POINT('Ctrl Pts',(-99.6684363547394,1074.7543712077,372.798445232698));
#124770=CARTESIAN_POINT('Ctrl Pts',(-99.6900123648613,1074.7437156369,372.671474620523));
#124771=CARTESIAN_POINT('Ctrl Pts',(-99.6882828172453,1074.73981601127,
372.606732697218));
#124772=CARTESIAN_POINT('Ctrl Pts',(-99.6600111766514,1074.73531901636,
372.481929375305));
#124773=CARTESIAN_POINT('Ctrl Pts',(-99.6339517209293,1074.73474154548,
372.423098988367));
#124774=CARTESIAN_POINT('Ctrl Pts',(-99.5608011538376,1074.73698123031,
372.318740912569));
#124775=CARTESIAN_POINT('Ctrl Pts',(-99.5144777954332,1074.7397717411,372.274260968877));
#124776=CARTESIAN_POINT('Ctrl Pts',(-99.4072144933072,1074.74838106255,
372.205274422036));
#124777=CARTESIAN_POINT('Ctrl Pts',(-99.347252102839,1074.75413301401,372.181586395893));
#124778=CARTESIAN_POINT('Ctrl Pts',(-99.2552154208791,1074.76417188024,
372.164631224256));
#124779=CARTESIAN_POINT('Ctrl Pts',(-99.2254770900566,1074.76758801247,
372.161918025972));
#124780=CARTESIAN_POINT('Ctrl Pts',(-99.1956988915339,1074.7711770522,372.161916347568));
#124781=CARTESIAN_POINT('Ctrl Pts',(-99.1956896753178,1074.77117816299,
372.161916347048));
#124782=CARTESIAN_POINT('Ctrl Pts',(-99.195680459116,1074.7711792738,372.16191634679));
#124783=CARTESIAN_POINT('Ctrl Pts',(-99.1956712429286,1074.77118038462,
372.16191634679));
#124784=CARTESIAN_POINT('',(-99.1956712429286,1082.7251047501,372.16191634679));
#124785=CARTESIAN_POINT('',(-99.1956712429286,1067.7251047501,372.16191634679));
#124786=CARTESIAN_POINT('Origin',(-99.1956712429286,1082.7251047501,372.652457095519));
#124787=CARTESIAN_POINT('Ctrl Pts',(-99.1956712429286,1074.77118038462,
372.16191634679));
#124788=CARTESIAN_POINT('Ctrl Pts',(-99.1297340660699,1074.77912774276,
372.16191634679));
#124789=CARTESIAN_POINT('Ctrl Pts',(-99.0645312222755,1074.7878101565,372.1752096209));
#124790=CARTESIAN_POINT('Ctrl Pts',(-98.9743517036196,1074.80104262714,
372.213502073698));
#124791=CARTESIAN_POINT('Ctrl Pts',(-98.9460644227095,1074.80540462821,
372.228947359956));
#124792=CARTESIAN_POINT('Ctrl Pts',(-98.8653599029516,1074.8185211102,372.283926582666));
#124793=CARTESIAN_POINT('Ctrl Pts',(-98.8191031316056,1074.82701527461,
372.33131186045));
#124794=CARTESIAN_POINT('Ctrl Pts',(-98.7481151465056,1074.84235637596,
372.441305120991));
#124795=CARTESIAN_POINT('Ctrl Pts',(-98.7239595772774,1074.84906341277,
372.502763622427));
#124796=CARTESIAN_POINT('Ctrl Pts',(-98.7013740385812,1074.85972531503,
372.630836062828));
#124797=CARTESIAN_POINT('Ctrl Pts',(-98.7028062655346,1074.86361216937,
372.696083679091));
#124798=CARTESIAN_POINT('Ctrl Pts',(-98.7307701748566,1074.86808704829,
372.821447784717));
#124799=CARTESIAN_POINT('Ctrl Pts',(-98.7566336507401,1074.8686798691,372.880361708791));
#124800=CARTESIAN_POINT('Ctrl Pts',(-98.8294783216542,1074.86654297423,
372.985020790852));
#124801=CARTESIAN_POINT('Ctrl Pts',(-98.8757212820671,1074.86383445787,
373.029699944009));
#124802=CARTESIAN_POINT('Ctrl Pts',(-98.9829389375818,1074.85541703767,
373.099089660562));
#124803=CARTESIAN_POINT('Ctrl Pts',(-99.042938015002,1074.84977184277,373.12296932195));
#124804=CARTESIAN_POINT('Ctrl Pts',(-99.1354780105686,1074.83982609407,
373.140230847772));
#124805=CARTESIAN_POINT('Ctrl Pts',(-99.1655889700239,1074.83640949208,
373.142997844247));
#124806=CARTESIAN_POINT('Ctrl Pts',(-99.1956712429286,1074.8328201009,373.142997844247));
#124807=CARTESIAN_POINT('Origin',(-97.7222027015963,1067.7251047501,386.561549283282));
#124808=CARTESIAN_POINT('',(-97.7222027016186,1075.61311396869,385.46271814729));
#124809=CARTESIAN_POINT('',(-97.7222027015963,1067.7251047501,385.46271814729));
#124810=CARTESIAN_POINT('Ctrl Pts',(-97.7213988942016,1075.69623611514,
387.660380125278));
#124811=CARTESIAN_POINT('Ctrl Pts',(-97.7927939677333,1075.68940709858,
387.660432351595));
#124812=CARTESIAN_POINT('Ctrl Pts',(-97.8640028065381,1075.68231205992,
387.653526301707));
#124813=CARTESIAN_POINT('Ctrl Pts',(-98.0042962639257,1075.66775644269,
387.625965942542));
#124814=CARTESIAN_POINT('Ctrl Pts',(-98.0730487518634,1075.66032808101,
387.605323305624));
#124815=CARTESIAN_POINT('Ctrl Pts',(-98.2758843532508,1075.6374862955,387.52210313036));
#124816=CARTESIAN_POINT('Ctrl Pts',(-98.3998385255858,1075.62218947111,
387.439084648386));
#124817=CARTESIAN_POINT('Ctrl Pts',(-98.6053228124055,1075.59396881424,
387.231195397763));
#124818=CARTESIAN_POINT('Ctrl Pts',(-98.6857602946434,1075.58127100407,
387.1092371073));
#124819=CARTESIAN_POINT('Ctrl Pts',(-98.7944472760788,1075.56005240322,
386.841647480565));
#124820=CARTESIAN_POINT('Ctrl Pts',(-98.8219370424237,1075.55171700464,
386.698755938379));
#124821=CARTESIAN_POINT('Ctrl Pts',(-98.8200911789728,1075.54065643482,
386.411143056393));
#124822=CARTESIAN_POINT('Ctrl Pts',(-98.7911263244649,1075.53800826563,
386.269295043914));
#124823=CARTESIAN_POINT('Ctrl Pts',(-98.6804305013425,1075.5387916389,386.005053410384));
#124824=CARTESIAN_POINT('Ctrl Pts',(-98.5999634160729,1075.54219713368,
385.885244836217));
#124825=CARTESIAN_POINT('Ctrl Pts',(-98.3975468297286,1075.55460304053,
385.682995241437));
#124826=CARTESIAN_POINT('Ctrl Pts',(-98.2775037975997,1075.5634916692,385.602639121292));
#124827=CARTESIAN_POINT('Ctrl Pts',(-98.0128524825785,1075.58555280984,
385.492138136355));
#124828=CARTESIAN_POINT('Ctrl Pts',(-97.8706550702968,1075.59853521395,
385.463366061341));
#124829=CARTESIAN_POINT('Ctrl Pts',(-97.5826998525611,1075.62681310325,
385.462088309446));
#124830=CARTESIAN_POINT('Ctrl Pts',(-97.4396440456053,1075.64185219423,
385.489908949946));
#124831=CARTESIAN_POINT('Ctrl Pts',(-97.1706666046853,1075.67209073474,
385.599963242149));
#124832=CARTESIAN_POINT('Ctrl Pts',(-97.0475985821659,1075.68699859297,
385.681895667295));
#124833=CARTESIAN_POINT('Ctrl Pts',(-96.841400767303,1075.71438832665,385.888646192269));
#124834=CARTESIAN_POINT('Ctrl Pts',(-96.7600209710137,1075.72662181786,
386.011188802362));
#124835=CARTESIAN_POINT('Ctrl Pts',(-96.6498379179535,1075.74692429867,
386.28104276992));
#124836=CARTESIAN_POINT('Ctrl Pts',(-96.6220888699548,1075.75479732189,
386.42563596903));
#124837=CARTESIAN_POINT('Ctrl Pts',(-96.624747375387,1075.76518408089,386.717694008871));
#124838=CARTESIAN_POINT('Ctrl Pts',(-96.6552215892545,1075.76758459124,
386.862159174312));
#124839=CARTESIAN_POINT('Ctrl Pts',(-96.7698335321823,1075.76655483237,
387.128091212793));
#124840=CARTESIAN_POINT('Ctrl Pts',(-96.8517548533546,1075.76324894579,
387.247307224677));
#124841=CARTESIAN_POINT('Ctrl Pts',(-97.0585089197345,1075.75126299893,
387.449365585822));
#124842=CARTESIAN_POINT('Ctrl Pts',(-97.1819905856914,1075.7426053114,387.52943428261));
#124843=CARTESIAN_POINT('Ctrl Pts',(-97.4460777276447,1075.72150585643,
387.634096632222));
#124844=CARTESIAN_POINT('Ctrl Pts',(-97.5831723197036,1075.70945763757,
387.660279010949));
#124845=CARTESIAN_POINT('Ctrl Pts',(-97.7213988942016,1075.69623611513,
387.660380125278));
#124846=CARTESIAN_POINT('Origin',(-97.7222027015963,1067.7251047501,386.561549283282));
#124847=CARTESIAN_POINT('',(-97.7222027015962,1075.6741872497,387.060380419275));
#124848=CARTESIAN_POINT('',(-97.7222027015963,1075.63649232378,386.06271814729));
#124849=CARTESIAN_POINT('Ctrl Pts',(-97.7222027015961,1075.6741872497,387.060380419275));
#124850=CARTESIAN_POINT('Ctrl Pts',(-97.7249263879499,1075.67392467079,
387.060380419275));
#124851=CARTESIAN_POINT('Ctrl Pts',(-97.7276509946975,1075.67366113051,
387.060358111756));
#124852=CARTESIAN_POINT('Ctrl Pts',(-97.762899977707,1075.67024032216,387.05978046529));
#124853=CARTESIAN_POINT('Ctrl Pts',(-97.7952848834862,1075.66697284493,
387.056067683896));
#124854=CARTESIAN_POINT('Ctrl Pts',(-97.8589146873207,1075.66030116281,
387.042385392596));
#124855=CARTESIAN_POINT('Ctrl Pts',(-97.8900104669429,1075.65691209393,
387.032435413474));
#124856=CARTESIAN_POINT('Ctrl Pts',(-97.9812941539065,1075.64656074511,
386.993028306789));
#124857=CARTESIAN_POINT('Ctrl Pts',(-98.036754080926,1075.63969324207,386.954445759814));
#124858=CARTESIAN_POINT('Ctrl Pts',(-98.128239041283,1075.62710710462,386.858642086529));
#124859=CARTESIAN_POINT('Ctrl Pts',(-98.1637678945812,1075.62148792769,
386.802725766566));
#124860=CARTESIAN_POINT('Ctrl Pts',(-98.211006819578,1075.61217335651,386.680571496346));
#124861=CARTESIAN_POINT('Ctrl Pts',(-98.2223941639612,1075.60855815078,
386.615582502864));
#124862=CARTESIAN_POINT('Ctrl Pts',(-98.2194229250556,1075.60384387592,
386.485153884733));
#124863=CARTESIAN_POINT('Ctrl Pts',(-98.2052336626134,1075.60277834611,
386.421012651017));
#124864=CARTESIAN_POINT('Ctrl Pts',(-98.1530459549406,1075.60334973963,
386.301881037638));
#124865=CARTESIAN_POINT('Ctrl Pts',(-98.1156137934597,1075.60497579798,
386.24806332025));
#124866=CARTESIAN_POINT('Ctrl Pts',(-98.0221507717359,1075.61071633582,
386.157690755954));
#124867=CARTESIAN_POINT('Ctrl Pts',(-97.9669908054845,1075.61478079353,
386.122079993755));
#124868=CARTESIAN_POINT('Ctrl Pts',(-97.8478871855469,1075.62465919293,
386.074690770394));
#124869=CARTESIAN_POINT('Ctrl Pts',(-97.7853021333535,1075.63033249837,
386.06271814729));
#124870=CARTESIAN_POINT('Ctrl Pts',(-97.7222027015964,1075.63649232378,
386.06271814729));
#124871=CARTESIAN_POINT('',(-97.7222027015963,1082.7251047501,386.06271814729));
#124872=CARTESIAN_POINT('',(-97.7222027015963,1067.7251047501,386.06271814729));
#124873=CARTESIAN_POINT('Origin',(-97.7222027015963,1082.7251047501,386.561549283282));
#124874=CARTESIAN_POINT('Ctrl Pts',(-97.7222027015964,1075.63649232378,
386.06271814729));
#124875=CARTESIAN_POINT('Ctrl Pts',(-97.7221511724957,1075.6364973541,386.06271814729));
#124876=CARTESIAN_POINT('Ctrl Pts',(-97.722099643052,1075.63650238475,386.062718155274));
#124877=CARTESIAN_POINT('Ctrl Pts',(-97.7220481132671,1075.63650741572,
386.062718171243));
#124878=CARTESIAN_POINT('Ctrl Pts',(-97.6893287168738,1075.63970188354,
386.062728311021));
#124879=CARTESIAN_POINT('Ctrl Pts',(-97.656698034032,1075.64300505106,386.065957603219));
#124880=CARTESIAN_POINT('Ctrl Pts',(-97.592592556617,1075.64972746131,386.078744203233));
#124881=CARTESIAN_POINT('Ctrl Pts',(-97.5612650171618,1075.65313098461,
386.088264651513));
#124882=CARTESIAN_POINT('Ctrl Pts',(-97.4695991206023,1075.6634566299,386.126283525766));
#124883=CARTESIAN_POINT('Ctrl Pts',(-97.413798364603,1075.67026241494,386.163856256138));
#124884=CARTESIAN_POINT('Ctrl Pts',(-97.3203918518557,1075.68281384094,
386.25858229628));
#124885=CARTESIAN_POINT('Ctrl Pts',(-97.2836336377487,1075.68844110033,
386.314739948528));
#124886=CARTESIAN_POINT('Ctrl Pts',(-97.2343187412388,1075.69777017507,
386.438203499131));
#124887=CARTESIAN_POINT('Ctrl Pts',(-97.222225460169,1075.70138131606,386.504250147017));
#124888=CARTESIAN_POINT('Ctrl Pts',(-97.2246604112321,1075.70603775601,
386.635792573754));
#124889=CARTESIAN_POINT('Ctrl Pts',(-97.2385639595588,1075.70709399248,
386.699965336072));
#124890=CARTESIAN_POINT('Ctrl Pts',(-97.2902347119164,1075.70660095883,
386.819358321241));
#124891=CARTESIAN_POINT('Ctrl Pts',(-97.327476342736,1075.70505768393,386.873391808103));
#124892=CARTESIAN_POINT('Ctrl Pts',(-97.420701095975,1075.6995360576,386.964267241999));
#124893=CARTESIAN_POINT('Ctrl Pts',(-97.4758256104629,1075.69560341623,
387.000146838782));
#124894=CARTESIAN_POINT('Ctrl Pts',(-97.5954245965813,1075.6859325459,387.04820135808));
#124895=CARTESIAN_POINT('Ctrl Pts',(-97.6585624263007,1075.68032253532,
387.060380419275));
#124896=CARTESIAN_POINT('Ctrl Pts',(-97.7222027015961,1075.6741872497,387.060380419275));
#124897=CARTESIAN_POINT('Origin',(-9.69136378659147,1067.7251047501,441.167646863288));
#124898=CARTESIAN_POINT('',(-9.69136378659147,1078.73142393294,440.067288797613));
#124899=CARTESIAN_POINT('Origin',(-9.69136378659147,1078.73142393294,441.167646863288));
#124900=CARTESIAN_POINT('',(-9.69136378659147,1076.73142393294,440.067288797613));
#124901=CARTESIAN_POINT('',(-9.69136378659147,1067.7251047501,440.067288797613));
#124902=CARTESIAN_POINT('Origin',(-9.69136378659147,1076.73142393294,441.167646863288));
#124903=CARTESIAN_POINT('Origin',(-9.69136378659147,1067.7251047501,441.167646863288));
#124904=CARTESIAN_POINT('',(-9.69136378659147,1076.73142393294,440.667288797613));
#124905=CARTESIAN_POINT('Origin',(-9.69136378659147,1076.73142393294,441.167646863288));
#124906=CARTESIAN_POINT('',(-9.69136378659147,1082.7251047501,440.667288797613));
#124907=CARTESIAN_POINT('',(-9.69136378659147,1067.7251047501,440.667288797613));
#124908=CARTESIAN_POINT('Origin',(-9.69136378659147,1082.7251047501,441.167646863288));
#124909=CARTESIAN_POINT('Origin',(-16.2097648263481,1067.7251047501,446.721728083052));
#124910=CARTESIAN_POINT('',(-16.2097648263481,1078.73142393294,445.507696516315));
#124911=CARTESIAN_POINT('Origin',(-16.2097648263481,1078.73142393294,446.721728083052));
#124912=CARTESIAN_POINT('',(-16.2097648263481,1076.73142393294,445.507696516315));
#124913=CARTESIAN_POINT('',(-16.2097648263481,1067.7251047501,445.507696516315));
#124914=CARTESIAN_POINT('Origin',(-16.2097648263481,1076.73142393294,446.721728083052));
#124915=CARTESIAN_POINT('Origin',(-16.2097648263481,1067.7251047501,446.721728083052));
#124916=CARTESIAN_POINT('',(-16.2097648263481,1076.73142393294,446.107696516315));
#124917=CARTESIAN_POINT('Origin',(-16.2097648263481,1076.73142393294,446.721728083052));
#124918=CARTESIAN_POINT('',(-16.2097648263481,1082.7251047501,446.107696516315));
#124919=CARTESIAN_POINT('',(-16.2097648263481,1067.7251047501,446.107696516315));
#124920=CARTESIAN_POINT('Origin',(-16.2097648263481,1082.7251047501,446.721728083052));
#124921=CARTESIAN_POINT('Origin',(-23.3029185074263,1067.7251047501,450.258118980149));
#124922=CARTESIAN_POINT('',(-23.3029185074263,1078.73142393294,448.929311016575));
#124923=CARTESIAN_POINT('Origin',(-23.3029185074263,1078.73142393294,450.258118980149));
#124924=CARTESIAN_POINT('',(-23.3029185074263,1076.73142393294,448.929311016575));
#124925=CARTESIAN_POINT('',(-23.3029185074263,1067.7251047501,448.929311016575));
#124926=CARTESIAN_POINT('Origin',(-23.3029185074263,1076.73142393294,450.258118980149));
#124927=CARTESIAN_POINT('Origin',(-23.3029185074263,1067.7251047501,450.258118980149));
#124928=CARTESIAN_POINT('',(-23.3029185074263,1076.73142393294,449.529311016575));
#124929=CARTESIAN_POINT('Origin',(-23.3029185074263,1076.73142393294,450.258118980149));
#124930=CARTESIAN_POINT('',(-23.3029185074263,1082.7251047501,449.529311016575));
#124931=CARTESIAN_POINT('',(-23.3029185074263,1067.7251047501,449.529311016575));
#124932=CARTESIAN_POINT('Origin',(-23.3029185074263,1082.7251047501,450.258118980149));
#124933=CARTESIAN_POINT('Origin',(-32.1589076220707,1067.7251047501,452.997442536411));
#124934=CARTESIAN_POINT('',(-32.1589076220707,1078.73142393294,451.536325534594));
#124935=CARTESIAN_POINT('Origin',(-32.1589076220707,1078.73142393294,452.997442536411));
#124936=CARTESIAN_POINT('',(-32.1589076220707,1076.73142393294,451.536325534594));
#124937=CARTESIAN_POINT('',(-32.1589076220707,1067.7251047501,451.536325534594));
#124938=CARTESIAN_POINT('Origin',(-32.1589076220707,1076.73142393294,452.997442536411));
#124939=CARTESIAN_POINT('Origin',(-32.1589076220707,1067.7251047501,452.997442536411));
#124940=CARTESIAN_POINT('',(-32.1589076220707,1076.73142393294,452.136325534594));
#124941=CARTESIAN_POINT('Origin',(-32.1589076220707,1076.73142393294,452.997442536411));
#124942=CARTESIAN_POINT('',(-32.1589076220707,1082.7251047501,452.136325534594));
#124943=CARTESIAN_POINT('',(-32.1589076220707,1067.7251047501,452.136325534594));
#124944=CARTESIAN_POINT('Origin',(-32.1589076220707,1082.7251047501,452.997442536411));
#124945=CARTESIAN_POINT('Origin',(-41.0676411737315,1067.7251047501,453.455473148425));
#124946=CARTESIAN_POINT('',(-41.0676411737315,1078.73142393294,451.8349911058));
#124947=CARTESIAN_POINT('Origin',(-41.0676411737315,1078.73142393294,453.455473148425));
#124948=CARTESIAN_POINT('',(-41.0676411737315,1076.73142393294,451.8349911058));
#124949=CARTESIAN_POINT('',(-41.0676411737315,1067.7251047501,451.8349911058));
#124950=CARTESIAN_POINT('Origin',(-41.0676411737315,1076.73142393294,453.455473148425));
#124951=CARTESIAN_POINT('Origin',(-41.0676411737315,1067.7251047501,453.455473148425));
#124952=CARTESIAN_POINT('',(-41.0676411737315,1076.73142393294,452.4349911058));
#124953=CARTESIAN_POINT('Origin',(-41.0676411737315,1076.73142393294,453.455473148425));
#124954=CARTESIAN_POINT('',(-41.0676411737315,1082.7251047501,452.4349911058));
#124955=CARTESIAN_POINT('',(-41.0676411737315,1067.7251047501,452.4349911058));
#124956=CARTESIAN_POINT('Origin',(-41.0676411737315,1082.7251047501,453.455473148425));
#124957=CARTESIAN_POINT('Origin',(-51.2135807025652,1067.7251047501,452.701475992022));
#124958=CARTESIAN_POINT('',(-51.2135807025652,1078.73142393294,451.000475768939));
#124959=CARTESIAN_POINT('Origin',(-51.2135807025652,1078.73142393294,452.701475992022));
#124960=CARTESIAN_POINT('',(-51.2135807025652,1076.73142393294,451.000475768939));
#124961=CARTESIAN_POINT('',(-51.2135807025652,1067.7251047501,451.000475768939));
#124962=CARTESIAN_POINT('Origin',(-51.2135807025652,1076.73142393294,452.701475992022));
#124963=CARTESIAN_POINT('Origin',(-51.2135807025652,1067.7251047501,452.701475992022));
#124964=CARTESIAN_POINT('',(-51.2135807025652,1076.73142393294,451.600475768939));
#124965=CARTESIAN_POINT('Origin',(-51.2135807025652,1076.73142393294,452.701475992022));
#124966=CARTESIAN_POINT('',(-51.2135807025652,1082.7251047501,451.600475768939));
#124967=CARTESIAN_POINT('',(-51.2135807025652,1067.7251047501,451.600475768939));
#124968=CARTESIAN_POINT('Origin',(-51.2135807025652,1082.7251047501,452.701475992022));
#124969=CARTESIAN_POINT('Origin',(-60.6270981054984,1067.7251047501,449.74779979654));
#124970=CARTESIAN_POINT('',(-60.6270981054984,1078.73142393294,448.026525164496));
#124971=CARTESIAN_POINT('Origin',(-60.6270981054984,1078.73142393294,449.74779979654));
#124972=CARTESIAN_POINT('',(-60.6270981054984,1076.73142393294,448.026525164496));
#124973=CARTESIAN_POINT('',(-60.6270981054984,1067.7251047501,448.026525164496));
#124974=CARTESIAN_POINT('Origin',(-60.6270981054984,1076.73142393294,449.74779979654));
#124975=CARTESIAN_POINT('Origin',(-60.6270981054984,1067.7251047501,449.74779979654));
#124976=CARTESIAN_POINT('',(-60.6270981054984,1076.73142393294,448.626525164496));
#124977=CARTESIAN_POINT('Origin',(-60.6270981054984,1076.73142393294,449.74779979654));
#124978=CARTESIAN_POINT('',(-60.6270981054984,1082.7251047501,448.626525164496));
#124979=CARTESIAN_POINT('',(-60.6270981054984,1067.7251047501,448.626525164496));
#124980=CARTESIAN_POINT('Origin',(-60.6270981054984,1082.7251047501,449.74779979654));
#124981=CARTESIAN_POINT('Origin',(-71.0377028430569,1067.7251047501,445.125673808251));
#124982=CARTESIAN_POINT('',(-71.0377028430569,1078.73142393294,443.343681153846));
#124983=CARTESIAN_POINT('Origin',(-71.0377028430569,1078.73142393294,445.125673808251));
#124984=CARTESIAN_POINT('',(-71.0377028430569,1076.73142393294,443.343681153846));
#124985=CARTESIAN_POINT('',(-71.0377028430569,1067.7251047501,443.343681153846));
#124986=CARTESIAN_POINT('Origin',(-71.0377028430569,1076.73142393294,445.125673808251));
#124987=CARTESIAN_POINT('Origin',(-71.0377028430569,1067.7251047501,445.125673808251));
#124988=CARTESIAN_POINT('',(-71.0377028430569,1076.73142393294,443.943681153846));
#124989=CARTESIAN_POINT('Origin',(-71.0377028430569,1076.73142393294,445.125673808251));
#124990=CARTESIAN_POINT('',(-71.0377028430569,1082.7251047501,443.943681153846));
#124991=CARTESIAN_POINT('',(-71.0377028430569,1067.7251047501,443.943681153846));
#124992=CARTESIAN_POINT('Origin',(-71.0377028430569,1082.7251047501,445.125673808251));
#124993=CARTESIAN_POINT('Origin',(-80.1058740725522,1067.7251047501,438.515078960781));
#124994=CARTESIAN_POINT('',(-80.1058740725522,1078.73142393294,436.85419815086));
#124995=CARTESIAN_POINT('Origin',(-80.1058740725522,1078.73142393294,438.515078960781));
#124996=CARTESIAN_POINT('',(-80.1058740725522,1076.73142393294,436.85419815086));
#124997=CARTESIAN_POINT('',(-80.1058740725522,1067.7251047501,436.85419815086));
#124998=CARTESIAN_POINT('Origin',(-80.1058740725522,1076.73142393294,438.515078960781));
#124999=CARTESIAN_POINT('Origin',(-80.1058740725522,1067.7251047501,438.515078960781));
#125000=CARTESIAN_POINT('',(-80.1058740725522,1076.73142393294,437.45419815086));
#125001=CARTESIAN_POINT('Origin',(-80.1058740725522,1076.73142393294,438.515078960781));
#125002=CARTESIAN_POINT('',(-80.1058740725522,1082.7251047501,437.45419815086));
#125003=CARTESIAN_POINT('',(-80.1058740725522,1067.7251047501,437.45419815086));
#125004=CARTESIAN_POINT('Origin',(-80.1058740725522,1082.7251047501,438.515078960781));
#125005=CARTESIAN_POINT('Origin',(-6.03918543247926,1067.7251047501,442.820994209267));
#125006=CARTESIAN_POINT('',(-6.03918543247926,1078.73142393294,441.720636143593));
#125007=CARTESIAN_POINT('Origin',(-6.03918543247926,1078.73142393294,442.820994209267));
#125008=CARTESIAN_POINT('',(-6.03918543247926,1076.73142393294,441.720636143593));
#125009=CARTESIAN_POINT('',(-6.03918543247926,1067.7251047501,441.720636143593));
#125010=CARTESIAN_POINT('Origin',(-6.03918543247926,1076.73142393294,442.820994209267));
#125011=CARTESIAN_POINT('Origin',(-6.03918543247926,1067.7251047501,442.820994209267));
#125012=CARTESIAN_POINT('',(-6.03918543247926,1076.73142393294,442.320636143593));
#125013=CARTESIAN_POINT('Origin',(-6.03918543247926,1076.73142393294,442.820994209267));
#125014=CARTESIAN_POINT('',(-6.03918543247926,1082.7251047501,442.320636143593));
#125015=CARTESIAN_POINT('',(-6.03918543247926,1067.7251047501,442.320636143593));
#125016=CARTESIAN_POINT('Origin',(-6.03918543247926,1082.7251047501,442.820994209267));
#125017=CARTESIAN_POINT('Origin',(-11.2603853527976,1067.7251047501,449.608957210264));
#125018=CARTESIAN_POINT('',(-11.2603853527976,1078.73142393294,448.394925643527));
#125019=CARTESIAN_POINT('Origin',(-11.2603853527976,1078.73142393294,449.608957210264));
#125020=CARTESIAN_POINT('',(-11.2603853527976,1076.73142393294,448.394925643527));
#125021=CARTESIAN_POINT('',(-11.2603853527976,1067.7251047501,448.394925643527));
#125022=CARTESIAN_POINT('Origin',(-11.2603853527976,1076.73142393294,449.608957210264));
#125023=CARTESIAN_POINT('Origin',(-11.2603853527976,1067.7251047501,449.608957210264));
#125024=CARTESIAN_POINT('',(-11.2603853527976,1076.73142393294,448.994925643527));
#125025=CARTESIAN_POINT('Origin',(-11.2603853527976,1076.73142393294,449.608957210264));
#125026=CARTESIAN_POINT('',(-11.2603853527976,1082.7251047501,448.994925643527));
#125027=CARTESIAN_POINT('',(-11.2603853527976,1067.7251047501,448.994925643527));
#125028=CARTESIAN_POINT('Origin',(-11.2603853527976,1082.7251047501,449.608957210264));
#125029=CARTESIAN_POINT('Origin',(-17.4632795967725,1067.7251047501,454.54281905658));
#125030=CARTESIAN_POINT('',(-17.4632795967725,1078.73142393294,453.214011093006));
#125031=CARTESIAN_POINT('Origin',(-17.4632795967725,1078.73142393294,454.54281905658));
#125032=CARTESIAN_POINT('',(-17.4632795967725,1076.73142393294,453.214011093006));
#125033=CARTESIAN_POINT('',(-17.4632795967725,1067.7251047501,453.214011093006));
#125034=CARTESIAN_POINT('Origin',(-17.4632795967725,1076.73142393294,454.54281905658));
#125035=CARTESIAN_POINT('Origin',(-17.4632795967725,1067.7251047501,454.54281905658));
#125036=CARTESIAN_POINT('',(-17.4632795967725,1076.73142393294,453.814011093006));
#125037=CARTESIAN_POINT('Origin',(-17.4632795967725,1076.73142393294,454.54281905658));
#125038=CARTESIAN_POINT('',(-17.4632795967725,1082.7251047501,453.814011093006));
#125039=CARTESIAN_POINT('',(-17.4632795967725,1067.7251047501,453.814011093006));
#125040=CARTESIAN_POINT('Origin',(-17.4632795967725,1082.7251047501,454.54281905658));
#125041=CARTESIAN_POINT('Origin',(-25.5562067091073,1067.7251047501,459.06354549146));
#125042=CARTESIAN_POINT('',(-25.5562067091073,1078.73142393294,457.602428489643));
#125043=CARTESIAN_POINT('Origin',(-25.5562067091073,1078.73142393294,459.06354549146));
#125044=CARTESIAN_POINT('',(-25.5562067091073,1076.73142393294,457.602428489643));
#125045=CARTESIAN_POINT('',(-25.5562067091073,1067.7251047501,457.602428489643));
#125046=CARTESIAN_POINT('Origin',(-25.5562067091073,1076.73142393294,459.06354549146));
#125047=CARTESIAN_POINT('Origin',(-25.5562067091073,1067.7251047501,459.06354549146));
#125048=CARTESIAN_POINT('',(-25.5562067091073,1076.73142393294,458.202428489643));
#125049=CARTESIAN_POINT('Origin',(-25.5562067091073,1076.73142393294,459.06354549146));
#125050=CARTESIAN_POINT('',(-25.5562067091073,1082.7251047501,458.202428489643));
#125051=CARTESIAN_POINT('',(-25.5562067091073,1067.7251047501,458.202428489643));
#125052=CARTESIAN_POINT('Origin',(-25.5562067091073,1082.7251047501,459.06354549146));
#125053=CARTESIAN_POINT('Origin',(-34.1750331392509,1067.7251047501,461.363796891435));
#125054=CARTESIAN_POINT('',(-34.1750331392509,1078.73142393294,459.743314848811));
#125055=CARTESIAN_POINT('Origin',(-34.1750331392509,1078.73142393294,461.363796891435));
#125056=CARTESIAN_POINT('',(-34.1750331392509,1076.73142393294,459.743314848811));
#125057=CARTESIAN_POINT('',(-34.1750331392509,1067.7251047501,459.743314848811));
#125058=CARTESIAN_POINT('Origin',(-34.1750331392509,1076.73142393294,461.363796891435));
#125059=CARTESIAN_POINT('Origin',(-34.1750331392509,1067.7251047501,461.363796891435));
#125060=CARTESIAN_POINT('',(-34.1750331392509,1076.73142393294,460.343314848811));
#125061=CARTESIAN_POINT('Origin',(-34.1750331392509,1076.73142393294,461.363796891435));
#125062=CARTESIAN_POINT('',(-34.1750331392509,1082.7251047501,460.343314848811));
#125063=CARTESIAN_POINT('',(-34.1750331392509,1067.7251047501,460.343314848811));
#125064=CARTESIAN_POINT('Origin',(-34.1750331392509,1082.7251047501,461.363796891435));
#125065=CARTESIAN_POINT('Origin',(-44.2560243702294,1067.7251047501,462.735735824314));
#125066=CARTESIAN_POINT('',(-44.2560243702294,1078.73142393294,461.034735601231));
#125067=CARTESIAN_POINT('Origin',(-44.2560243702294,1078.73142393294,462.735735824314));
#125068=CARTESIAN_POINT('',(-44.2560243702294,1076.73142393294,461.034735601231));
#125069=CARTESIAN_POINT('',(-44.2560243702294,1067.7251047501,461.034735601231));
#125070=CARTESIAN_POINT('Origin',(-44.2560243702294,1076.73142393294,462.735735824314));
#125071=CARTESIAN_POINT('Origin',(-44.2560243702294,1067.7251047501,462.735735824314));
#125072=CARTESIAN_POINT('',(-44.2560243702294,1076.73142393294,461.634735601231));
#125073=CARTESIAN_POINT('Origin',(-44.2560243702294,1076.73142393294,462.735735824314));
#125074=CARTESIAN_POINT('',(-44.2560243702294,1082.7251047501,461.634735601231));
#125075=CARTESIAN_POINT('',(-44.2560243702294,1067.7251047501,461.634735601231));
#125076=CARTESIAN_POINT('Origin',(-44.2560243702294,1082.7251047501,462.735735824314));
#125077=CARTESIAN_POINT('Origin',(-54.0779376443053,1067.7251047501,461.803784860145));
#125078=CARTESIAN_POINT('',(-54.0779376443053,1078.73142393294,460.082510228102));
#125079=CARTESIAN_POINT('Origin',(-54.0779376443053,1078.73142393294,461.803784860145));
#125080=CARTESIAN_POINT('',(-54.0779376443053,1076.73142393294,460.082510228102));
#125081=CARTESIAN_POINT('',(-54.0779376443053,1067.7251047501,460.082510228102));
#125082=CARTESIAN_POINT('Origin',(-54.0779376443053,1076.73142393294,461.803784860145));
#125083=CARTESIAN_POINT('Origin',(-54.0779376443053,1067.7251047501,461.803784860145));
#125084=CARTESIAN_POINT('',(-54.0779376443053,1076.73142393294,460.682510228102));
#125085=CARTESIAN_POINT('Origin',(-54.0779376443053,1076.73142393294,461.803784860145));
#125086=CARTESIAN_POINT('',(-54.0779376443053,1082.7251047501,460.682510228102));
#125087=CARTESIAN_POINT('',(-54.0779376443053,1067.7251047501,460.682510228102));
#125088=CARTESIAN_POINT('Origin',(-54.0779376443053,1082.7251047501,461.803784860145));
#125089=CARTESIAN_POINT('Origin',(-65.222039719934,1067.7251047501,459.447149847832));
#125090=CARTESIAN_POINT('',(-65.222039719934,1078.73142393294,457.665157193427));
#125091=CARTESIAN_POINT('Origin',(-65.222039719934,1078.73142393294,459.447149847832));
#125092=CARTESIAN_POINT('',(-65.222039719934,1076.73142393294,457.665157193427));
#125093=CARTESIAN_POINT('',(-65.222039719934,1067.7251047501,457.665157193427));
#125094=CARTESIAN_POINT('Origin',(-65.222039719934,1076.73142393294,459.447149847832));
#125095=CARTESIAN_POINT('Origin',(-65.222039719934,1067.7251047501,459.447149847832));
#125096=CARTESIAN_POINT('',(-65.222039719934,1076.73142393294,458.265157193427));
#125097=CARTESIAN_POINT('Origin',(-65.222039719934,1076.73142393294,459.447149847832));
#125098=CARTESIAN_POINT('',(-65.222039719934,1082.7251047501,458.265157193427));
#125099=CARTESIAN_POINT('',(-65.222039719934,1067.7251047501,458.265157193427));
#125100=CARTESIAN_POINT('Origin',(-65.222039719934,1082.7251047501,459.447149847832));
#125101=CARTESIAN_POINT('Origin',(-75.4664696031568,1067.7251047501,454.866391171305));
#125102=CARTESIAN_POINT('',(-75.4664696031568,1078.73142393294,453.205510361384));
#125103=CARTESIAN_POINT('Origin',(-75.4664696031568,1078.73142393294,454.866391171305));
#125104=CARTESIAN_POINT('',(-75.4664696031568,1076.73142393294,453.205510361384));
#125105=CARTESIAN_POINT('',(-75.4664696031568,1067.7251047501,453.205510361384));
#125106=CARTESIAN_POINT('Origin',(-75.4664696031568,1076.73142393294,454.866391171305));
#125107=CARTESIAN_POINT('Origin',(-75.4664696031568,1067.7251047501,454.866391171305));
#125108=CARTESIAN_POINT('',(-75.4664696031568,1076.73142393294,453.805510361384));
#125109=CARTESIAN_POINT('Origin',(-75.4664696031568,1076.73142393294,454.866391171305));
#125110=CARTESIAN_POINT('',(-75.4664696031568,1082.7251047501,453.805510361384));
#125111=CARTESIAN_POINT('',(-75.4664696031568,1067.7251047501,453.805510361384));
#125112=CARTESIAN_POINT('Origin',(-75.4664696031568,1082.7251047501,454.866391171305));
#125113=CARTESIAN_POINT('Origin',(-2.12306569574067,1067.7251047501,443.678881372145));
#125114=CARTESIAN_POINT('',(-2.12306569574067,1078.73142393294,442.578523306471));
#125115=CARTESIAN_POINT('Origin',(-2.12306569574067,1078.73142393294,443.678881372145));
#125116=CARTESIAN_POINT('',(-2.12306569574067,1076.73142393294,442.578523306471));
#125117=CARTESIAN_POINT('',(-2.12306569574067,1067.7251047501,442.578523306471));
#125118=CARTESIAN_POINT('Origin',(-2.12306569574067,1076.73142393294,443.678881372145));
#125119=CARTESIAN_POINT('Origin',(-2.12306569574067,1067.7251047501,443.678881372145));
#125120=CARTESIAN_POINT('',(-2.12306569574067,1076.73142393294,443.178523306471));
#125121=CARTESIAN_POINT('Origin',(-2.12306569574067,1076.73142393294,443.678881372145));
#125122=CARTESIAN_POINT('',(-2.12306569574067,1082.7251047501,443.178523306471));
#125123=CARTESIAN_POINT('',(-2.12306569574067,1067.7251047501,443.178523306471));
#125124=CARTESIAN_POINT('Origin',(-2.12306569574067,1082.7251047501,443.678881372145));
#125125=CARTESIAN_POINT('Origin',(-5.818873006006,1067.7251047501,451.404059598971));
#125126=CARTESIAN_POINT('',(-5.818873006006,1078.73142393294,450.190028032234));
#125127=CARTESIAN_POINT('Origin',(-5.818873006006,1078.73142393294,451.404059598971));
#125128=CARTESIAN_POINT('',(-5.818873006006,1076.73142393294,450.190028032234));
#125129=CARTESIAN_POINT('',(-5.818873006006,1067.7251047501,450.190028032234));
#125130=CARTESIAN_POINT('Origin',(-5.818873006006,1076.73142393294,451.404059598971));
#125131=CARTESIAN_POINT('Origin',(-5.818873006006,1067.7251047501,451.404059598971));
#125132=CARTESIAN_POINT('',(-5.818873006006,1076.73142393294,450.790028032234));
#125133=CARTESIAN_POINT('Origin',(-5.818873006006,1076.73142393294,451.404059598971));
#125134=CARTESIAN_POINT('',(-5.818873006006,1082.7251047501,450.790028032234));
#125135=CARTESIAN_POINT('',(-5.818873006006,1067.7251047501,450.790028032234));
#125136=CARTESIAN_POINT('Origin',(-5.818873006006,1082.7251047501,451.404059598971));
#125137=CARTESIAN_POINT('Origin',(-10.8604115696268,1067.7251047501,457.519758956525));
#125138=CARTESIAN_POINT('',(-10.8604115696268,1078.73142393294,456.190950992952));
#125139=CARTESIAN_POINT('Origin',(-10.8604115696268,1078.73142393294,457.519758956525));
#125140=CARTESIAN_POINT('',(-10.8604115696268,1076.73142393294,456.190950992952));
#125141=CARTESIAN_POINT('',(-10.8604115696268,1067.7251047501,456.190950992952));
#125142=CARTESIAN_POINT('Origin',(-10.8604115696268,1076.73142393294,457.519758956525));
#125143=CARTESIAN_POINT('Origin',(-10.8604115696268,1067.7251047501,457.519758956525));
#125144=CARTESIAN_POINT('',(-10.8604115696268,1076.73142393294,456.790950992952));
#125145=CARTESIAN_POINT('Origin',(-10.8604115696268,1076.73142393294,457.519758956525));
#125146=CARTESIAN_POINT('',(-10.8604115696268,1082.7251047501,456.790950992952));
#125147=CARTESIAN_POINT('',(-10.8604115696268,1067.7251047501,456.790950992952));
#125148=CARTESIAN_POINT('Origin',(-10.8604115696268,1082.7251047501,457.519758956525));
#125149=CARTESIAN_POINT('Origin',(-17.8365769306701,1067.7251047501,463.624310831968));
#125150=CARTESIAN_POINT('',(-17.8365769306701,1078.73142393294,462.163193830151));
#125151=CARTESIAN_POINT('Origin',(-17.8365769306701,1078.73142393294,463.624310831968));
#125152=CARTESIAN_POINT('',(-17.8365769306701,1076.73142393294,462.163193830151));
#125153=CARTESIAN_POINT('',(-17.8365769306701,1067.7251047501,462.163193830151));
#125154=CARTESIAN_POINT('Origin',(-17.8365769306701,1076.73142393294,463.624310831968));
#125155=CARTESIAN_POINT('Origin',(-17.8365769306701,1067.7251047501,463.624310831968));
#125156=CARTESIAN_POINT('',(-17.8365769306701,1076.73142393294,462.763193830151));
#125157=CARTESIAN_POINT('Origin',(-17.8365769306701,1076.73142393294,463.624310831968));
#125158=CARTESIAN_POINT('',(-17.8365769306701,1082.7251047501,462.763193830151));
#125159=CARTESIAN_POINT('',(-17.8365769306701,1067.7251047501,462.763193830151));
#125160=CARTESIAN_POINT('Origin',(-17.8365769306701,1082.7251047501,463.624310831968));
#125161=CARTESIAN_POINT('Origin',(-25.7888121665815,1067.7251047501,467.666250995894));
#125162=CARTESIAN_POINT('',(-25.7888121665815,1078.73142393294,466.04576895327));
#125163=CARTESIAN_POINT('Origin',(-25.7888121665815,1078.73142393294,467.666250995894));
#125164=CARTESIAN_POINT('',(-25.7888121665815,1076.73142393294,466.04576895327));
#125165=CARTESIAN_POINT('',(-25.7888121665815,1067.7251047501,466.04576895327));
#125166=CARTESIAN_POINT('Origin',(-25.7888121665815,1076.73142393294,467.666250995894));
#125167=CARTESIAN_POINT('Origin',(-25.7888121665815,1067.7251047501,467.666250995894));
#125168=CARTESIAN_POINT('',(-25.7888121665815,1076.73142393294,466.64576895327));
#125169=CARTESIAN_POINT('Origin',(-25.7888121665815,1076.73142393294,467.666250995894));
#125170=CARTESIAN_POINT('',(-25.7888121665815,1082.7251047501,466.64576895327));
#125171=CARTESIAN_POINT('',(-25.7888121665815,1067.7251047501,466.64576895327));
#125172=CARTESIAN_POINT('Origin',(-25.7888121665815,1082.7251047501,467.666250995894));
#125173=CARTESIAN_POINT('Origin',(-35.3642674089481,1067.7251047501,471.104165703395));
#125174=CARTESIAN_POINT('',(-35.3642674089481,1078.73142393294,469.403165480312));
#125175=CARTESIAN_POINT('Origin',(-35.3642674089481,1078.73142393294,471.104165703395));
#125176=CARTESIAN_POINT('',(-35.3642674089481,1076.73142393294,469.403165480312));
#125177=CARTESIAN_POINT('',(-35.3642674089481,1067.7251047501,469.403165480312));
#125178=CARTESIAN_POINT('Origin',(-35.3642674089481,1076.73142393294,471.104165703395));
#125179=CARTESIAN_POINT('Origin',(-35.3642674089481,1067.7251047501,471.104165703395));
#125180=CARTESIAN_POINT('',(-35.3642674089481,1076.73142393294,470.003165480312));
#125181=CARTESIAN_POINT('Origin',(-35.3642674089481,1076.73142393294,471.104165703395));
#125182=CARTESIAN_POINT('',(-35.3642674089481,1082.7251047501,470.003165480312));
#125183=CARTESIAN_POINT('',(-35.3642674089481,1067.7251047501,470.003165480312));
#125184=CARTESIAN_POINT('Origin',(-35.3642674089481,1082.7251047501,471.104165703395));
#125185=CARTESIAN_POINT('Origin',(-45.1653118133206,1067.7251047501,472.23467069967));
#125186=CARTESIAN_POINT('',(-45.1653118133206,1078.73142393294,470.513396067626));
#125187=CARTESIAN_POINT('Origin',(-45.1653118133206,1078.73142393294,472.23467069967));
#125188=CARTESIAN_POINT('',(-45.1653118133206,1076.73142393294,470.513396067626));
#125189=CARTESIAN_POINT('',(-45.1653118133206,1067.7251047501,470.513396067626));
#125190=CARTESIAN_POINT('Origin',(-45.1653118133206,1076.73142393294,472.23467069967));
#125191=CARTESIAN_POINT('Origin',(-45.1653118133206,1067.7251047501,472.23467069967));
#125192=CARTESIAN_POINT('',(-45.1653118133206,1076.73142393294,471.113396067626));
#125193=CARTESIAN_POINT('Origin',(-45.1653118133206,1076.73142393294,472.23467069967));
#125194=CARTESIAN_POINT('',(-45.1653118133206,1082.7251047501,471.113396067626));
#125195=CARTESIAN_POINT('',(-45.1653118133206,1067.7251047501,471.113396067626));
#125196=CARTESIAN_POINT('Origin',(-45.1653118133206,1082.7251047501,472.23467069967));
#125197=CARTESIAN_POINT('Origin',(-56.5558604909797,1067.7251047501,472.24652292176));
#125198=CARTESIAN_POINT('',(-56.5558604909797,1078.73142393294,470.464530267355));
#125199=CARTESIAN_POINT('Origin',(-56.5558604909797,1078.73142393294,472.24652292176));
#125200=CARTESIAN_POINT('',(-56.5558604909797,1076.73142393294,470.464530267355));
#125201=CARTESIAN_POINT('',(-56.5558604909797,1067.7251047501,470.464530267355));
#125202=CARTESIAN_POINT('Origin',(-56.5558604909797,1076.73142393294,472.24652292176));
#125203=CARTESIAN_POINT('Origin',(-56.5558604909797,1067.7251047501,472.24652292176));
#125204=CARTESIAN_POINT('',(-56.5558604909797,1076.73142393294,471.064530267355));
#125205=CARTESIAN_POINT('Origin',(-56.5558604909797,1076.73142393294,472.24652292176));
#125206=CARTESIAN_POINT('',(-56.5558604909797,1082.7251047501,471.064530267355));
#125207=CARTESIAN_POINT('',(-56.5558604909797,1067.7251047501,471.064530267355));
#125208=CARTESIAN_POINT('Origin',(-56.5558604909797,1082.7251047501,472.24652292176));
#125209=CARTESIAN_POINT('Origin',(-67.5288182838046,1067.7251047501,469.89580155126));
#125210=CARTESIAN_POINT('',(-67.5288182838046,1078.73142393294,468.234920741339));
#125211=CARTESIAN_POINT('Origin',(-67.5288182838046,1078.73142393294,469.89580155126));
#125212=CARTESIAN_POINT('',(-67.5288182838046,1076.73142393294,468.234920741339));
#125213=CARTESIAN_POINT('',(-67.5288182838046,1067.7251047501,468.234920741339));
#125214=CARTESIAN_POINT('Origin',(-67.5288182838046,1076.73142393294,469.89580155126));
#125215=CARTESIAN_POINT('Origin',(-67.5288182838046,1067.7251047501,469.89580155126));
#125216=CARTESIAN_POINT('',(-67.5288182838046,1076.73142393294,468.834920741339));
#125217=CARTESIAN_POINT('Origin',(-67.5288182838046,1076.73142393294,469.89580155126));
#125218=CARTESIAN_POINT('',(-67.5288182838046,1082.7251047501,468.834920741339));
#125219=CARTESIAN_POINT('',(-67.5288182838046,1067.7251047501,468.834920741339));
#125220=CARTESIAN_POINT('Origin',(-67.5288182838046,1082.7251047501,469.89580155126));
#125221=CARTESIAN_POINT('Origin',(1.88584219950125,1067.7251047501,443.703814566305));
#125222=CARTESIAN_POINT('',(1.88584219950125,1078.73142393294,442.60345650063));
#125223=CARTESIAN_POINT('Origin',(1.88584219950125,1078.73142393294,443.703814566305));
#125224=CARTESIAN_POINT('',(1.88584219950125,1076.73142393294,442.60345650063));
#125225=CARTESIAN_POINT('',(1.88584219950125,1067.7251047501,442.60345650063));
#125226=CARTESIAN_POINT('Origin',(1.88584219950125,1076.73142393294,443.703814566305));
#125227=CARTESIAN_POINT('Origin',(1.88584219950125,1067.7251047501,443.703814566305));
#125228=CARTESIAN_POINT('',(1.88584219950125,1076.73142393294,443.20345650063));
#125229=CARTESIAN_POINT('Origin',(1.88584219950125,1076.73142393294,443.703814566305));
#125230=CARTESIAN_POINT('',(1.88584219950125,1082.7251047501,443.20345650063));
#125231=CARTESIAN_POINT('',(1.88584219950125,1067.7251047501,443.20345650063));
#125232=CARTESIAN_POINT('Origin',(1.88584219950125,1082.7251047501,443.703814566305));
#125233=CARTESIAN_POINT('Origin',(-0.123047986801322,1067.7251047501,452.02858066093));
#125234=CARTESIAN_POINT('',(-0.123047986801322,1078.73142393294,450.814549094193));
#125235=CARTESIAN_POINT('Origin',(-0.123047986801322,1078.73142393294,452.02858066093));
#125236=CARTESIAN_POINT('',(-0.123047986801322,1076.73142393294,450.814549094193));
#125237=CARTESIAN_POINT('',(-0.123047986801322,1067.7251047501,450.814549094193));
#125238=CARTESIAN_POINT('Origin',(-0.123047986801322,1076.73142393294,452.02858066093));
#125239=CARTESIAN_POINT('Origin',(-0.123047986801322,1067.7251047501,452.02858066093));
#125240=CARTESIAN_POINT('',(-0.123047986801322,1076.73142393294,451.414549094192));
#125241=CARTESIAN_POINT('Origin',(-0.123047986801322,1076.73142393294,452.02858066093));
#125242=CARTESIAN_POINT('',(-0.123047986801322,1082.7251047501,451.414549094192));
#125243=CARTESIAN_POINT('',(-0.123047986801322,1067.7251047501,451.414549094192));
#125244=CARTESIAN_POINT('Origin',(-0.123047986801322,1082.7251047501,452.02858066093));
#125245=CARTESIAN_POINT('Origin',(-3.78289144285191,1067.7251047501,459.058832121416));
#125246=CARTESIAN_POINT('',(-3.78289144285191,1078.73142393294,457.730024157842));
#125247=CARTESIAN_POINT('Origin',(-3.78289144285191,1078.73142393294,459.058832121416));
#125248=CARTESIAN_POINT('',(-3.78289144285191,1076.73142393294,457.730024157842));
#125249=CARTESIAN_POINT('',(-3.78289144285191,1067.7251047501,457.730024157842));
#125250=CARTESIAN_POINT('Origin',(-3.78289144285191,1076.73142393294,459.058832121416));
#125251=CARTESIAN_POINT('Origin',(-3.78289144285191,1067.7251047501,459.058832121416));
#125252=CARTESIAN_POINT('',(-3.78289144285191,1076.73142393294,458.330024157842));
#125253=CARTESIAN_POINT('Origin',(-3.78289144285191,1076.73142393294,459.058832121416));
#125254=CARTESIAN_POINT('',(-3.78289144285191,1082.7251047501,458.330024157842));
#125255=CARTESIAN_POINT('',(-3.78289144285191,1067.7251047501,458.330024157842));
#125256=CARTESIAN_POINT('Origin',(-3.78289144285191,1082.7251047501,459.058832121416));
#125257=CARTESIAN_POINT('Origin',(-9.33740315097062,1067.7251047501,466.480411227574));
#125258=CARTESIAN_POINT('',(-9.33740315097062,1078.73142393294,465.019294225757));
#125259=CARTESIAN_POINT('Origin',(-9.33740315097062,1078.73142393294,466.480411227574));
#125260=CARTESIAN_POINT('',(-9.33740315097062,1076.73142393294,465.019294225757));
#125261=CARTESIAN_POINT('',(-9.33740315097062,1067.7251047501,465.019294225757));
#125262=CARTESIAN_POINT('Origin',(-9.33740315097062,1076.73142393294,466.480411227574));
#125263=CARTESIAN_POINT('Origin',(-9.33740315097062,1067.7251047501,466.480411227574));
#125264=CARTESIAN_POINT('',(-9.33740315097062,1076.73142393294,465.619294225757));
#125265=CARTESIAN_POINT('Origin',(-9.33740315097062,1076.73142393294,466.480411227574));
#125266=CARTESIAN_POINT('',(-9.33740315097062,1082.7251047501,465.619294225757));
#125267=CARTESIAN_POINT('',(-9.33740315097062,1067.7251047501,465.619294225757));
#125268=CARTESIAN_POINT('Origin',(-9.33740315097062,1082.7251047501,466.480411227574));
#125269=CARTESIAN_POINT('Origin',(-16.2754963537821,1067.7251047501,472.087387974907));
#125270=CARTESIAN_POINT('',(-16.2754963537821,1078.73142393294,470.466905932282));
#125271=CARTESIAN_POINT('Origin',(-16.2754963537821,1078.73142393294,472.087387974907));
#125272=CARTESIAN_POINT('',(-16.2754963537821,1076.73142393294,470.466905932282));
#125273=CARTESIAN_POINT('',(-16.2754963537821,1067.7251047501,470.466905932282));
#125274=CARTESIAN_POINT('Origin',(-16.2754963537821,1076.73142393294,472.087387974907));
#125275=CARTESIAN_POINT('Origin',(-16.2754963537821,1067.7251047501,472.087387974907));
#125276=CARTESIAN_POINT('',(-16.2754963537821,1076.73142393294,471.066905932282));
#125277=CARTESIAN_POINT('Origin',(-16.2754963537821,1076.73142393294,472.087387974907));
#125278=CARTESIAN_POINT('',(-16.2754963537821,1082.7251047501,471.066905932282));
#125279=CARTESIAN_POINT('',(-16.2754963537821,1067.7251047501,471.066905932282));
#125280=CARTESIAN_POINT('Origin',(-16.2754963537821,1082.7251047501,472.087387974907));
#125281=CARTESIAN_POINT('Origin',(-24.9269222653132,1067.7251047501,477.441025087366));
#125282=CARTESIAN_POINT('',(-24.9269222653132,1078.73142393294,475.740024864283));
#125283=CARTESIAN_POINT('Origin',(-24.9269222653132,1078.73142393294,477.441025087366));
#125284=CARTESIAN_POINT('',(-24.9269222653132,1076.73142393294,475.740024864283));
#125285=CARTESIAN_POINT('',(-24.9269222653132,1067.7251047501,475.740024864283));
#125286=CARTESIAN_POINT('Origin',(-24.9269222653132,1076.73142393294,477.441025087366));
#125287=CARTESIAN_POINT('Origin',(-24.9269222653132,1067.7251047501,477.441025087366));
#125288=CARTESIAN_POINT('',(-24.9269222653132,1076.73142393294,476.340024864283));
#125289=CARTESIAN_POINT('Origin',(-24.9269222653132,1076.73142393294,477.441025087366));
#125290=CARTESIAN_POINT('',(-24.9269222653132,1082.7251047501,476.340024864283));
#125291=CARTESIAN_POINT('',(-24.9269222653132,1067.7251047501,476.340024864283));
#125292=CARTESIAN_POINT('Origin',(-24.9269222653132,1082.7251047501,477.441025087366));
#125293=CARTESIAN_POINT('Origin',(-34.2787451288822,1067.7251047501,480.584577550983));
#125294=CARTESIAN_POINT('',(-34.2787451288822,1078.73142393294,478.863302918939));
#125295=CARTESIAN_POINT('Origin',(-34.2787451288822,1078.73142393294,480.584577550983));
#125296=CARTESIAN_POINT('',(-34.2787451288822,1076.73142393294,478.863302918939));
#125297=CARTESIAN_POINT('',(-34.2787451288822,1067.7251047501,478.863302918939));
#125298=CARTESIAN_POINT('Origin',(-34.2787451288822,1076.73142393294,480.584577550983));
#125299=CARTESIAN_POINT('Origin',(-34.2787451288822,1067.7251047501,480.584577550983));
#125300=CARTESIAN_POINT('',(-34.2787451288822,1076.73142393294,479.463302918939));
#125301=CARTESIAN_POINT('Origin',(-34.2787451288822,1076.73142393294,480.584577550983));
#125302=CARTESIAN_POINT('',(-34.2787451288822,1082.7251047501,479.463302918939));
#125303=CARTESIAN_POINT('',(-34.2787451288822,1067.7251047501,479.463302918939));
#125304=CARTESIAN_POINT('Origin',(-34.2787451288822,1082.7251047501,480.584577550983));
#125305=CARTESIAN_POINT('Origin',(-45.4179187734414,1067.7251047501,482.964399008498));
#125306=CARTESIAN_POINT('',(-45.4179187734414,1078.73142393294,481.182406354093));
#125307=CARTESIAN_POINT('Origin',(-45.4179187734414,1078.73142393294,482.964399008498));
#125308=CARTESIAN_POINT('',(-45.4179187734414,1076.73142393294,481.182406354093));
#125309=CARTESIAN_POINT('',(-45.4179187734414,1067.7251047501,481.182406354093));
#125310=CARTESIAN_POINT('Origin',(-45.4179187734414,1076.73142393294,482.964399008498));
#125311=CARTESIAN_POINT('Origin',(-45.4179187734414,1067.7251047501,482.964399008498));
#125312=CARTESIAN_POINT('',(-45.4179187734414,1076.73142393294,481.782406354093));
#125313=CARTESIAN_POINT('Origin',(-45.4179187734414,1076.73142393294,482.964399008498));
#125314=CARTESIAN_POINT('',(-45.4179187734414,1082.7251047501,481.782406354093));
#125315=CARTESIAN_POINT('',(-45.4179187734414,1067.7251047501,481.782406354093));
#125316=CARTESIAN_POINT('Origin',(-45.4179187734414,1082.7251047501,482.964399008498));
#125317=CARTESIAN_POINT('Origin',(-56.6398335662286,1067.7251047501,482.946452747927));
#125318=CARTESIAN_POINT('',(-56.6398335662286,1078.73142393294,481.285571938007));
#125319=CARTESIAN_POINT('Origin',(-56.6398335662286,1078.73142393294,482.946452747927));
#125320=CARTESIAN_POINT('',(-56.6398335662286,1076.73142393294,481.285571938007));
#125321=CARTESIAN_POINT('',(-56.6398335662286,1067.7251047501,481.285571938007));
#125322=CARTESIAN_POINT('Origin',(-56.6398335662286,1076.73142393294,482.946452747927));
#125323=CARTESIAN_POINT('Origin',(-56.6398335662286,1067.7251047501,482.946452747927));
#125324=CARTESIAN_POINT('',(-56.6398335662286,1076.73142393294,481.885571938007));
#125325=CARTESIAN_POINT('Origin',(-56.6398335662286,1076.73142393294,482.946452747927));
#125326=CARTESIAN_POINT('',(-56.6398335662286,1082.7251047501,481.885571938007));
#125327=CARTESIAN_POINT('',(-56.6398335662286,1067.7251047501,481.885571938007));
#125328=CARTESIAN_POINT('Origin',(-56.6398335662286,1082.7251047501,482.946452747927));
#125329=CARTESIAN_POINT('Origin',(5.81232974134988,1067.7251047501,442.894704091518));
#125330=CARTESIAN_POINT('',(5.81232974134988,1078.73142393294,441.794346025843));
#125331=CARTESIAN_POINT('Origin',(5.81232974134988,1078.73142393294,442.894704091518));
#125332=CARTESIAN_POINT('',(5.81232974134988,1076.73142393294,441.794346025843));
#125333=CARTESIAN_POINT('',(5.81232974134988,1067.7251047501,441.794346025843));
#125334=CARTESIAN_POINT('Origin',(5.81232974134988,1076.73142393294,442.894704091518));
#125335=CARTESIAN_POINT('Origin',(5.81232974134988,1067.7251047501,442.894704091518));
#125336=CARTESIAN_POINT('',(5.81232974134988,1076.73142393294,442.394346025843));
#125337=CARTESIAN_POINT('Origin',(5.81232974134988,1076.73142393294,442.894704091518));
#125338=CARTESIAN_POINT('',(5.81232974134988,1082.7251047501,442.394346025843));
#125339=CARTESIAN_POINT('',(5.81232974134988,1067.7251047501,442.394346025843));
#125340=CARTESIAN_POINT('Origin',(5.81232974134988,1082.7251047501,442.894704091518));
#125341=CARTESIAN_POINT('Origin',(5.57815481987611,1067.7251047501,451.455225828947));
#125342=CARTESIAN_POINT('',(5.57815481987611,1078.73142393294,450.24119426221));
#125343=CARTESIAN_POINT('Origin',(5.57815481987611,1078.73142393294,451.455225828947));
#125344=CARTESIAN_POINT('',(5.57815481987611,1076.73142393294,450.24119426221));
#125345=CARTESIAN_POINT('',(5.57815481987611,1067.7251047501,450.24119426221));
#125346=CARTESIAN_POINT('Origin',(5.57815481987611,1076.73142393294,451.455225828947));
#125347=CARTESIAN_POINT('Origin',(5.57815481987611,1067.7251047501,451.455225828947));
#125348=CARTESIAN_POINT('',(5.57815481987611,1076.73142393294,450.84119426221));
#125349=CARTESIAN_POINT('Origin',(5.57815481987611,1076.73142393294,451.455225828947));
#125350=CARTESIAN_POINT('',(5.57815481987611,1082.7251047501,450.84119426221));
#125351=CARTESIAN_POINT('',(5.57815481987611,1067.7251047501,450.84119426221));
#125352=CARTESIAN_POINT('Origin',(5.57815481987611,1082.7251047501,451.455225828947));
#125353=CARTESIAN_POINT('Origin',(3.45995919230269,1067.7251047501,459.092773668652));
#125354=CARTESIAN_POINT('',(3.45995919230269,1078.73142393294,457.763965705079));
#125355=CARTESIAN_POINT('Origin',(3.45995919230269,1078.73142393294,459.092773668652));
#125356=CARTESIAN_POINT('',(3.45995919230269,1076.73142393294,457.763965705079));
#125357=CARTESIAN_POINT('',(3.45995919230269,1067.7251047501,457.763965705079));
#125358=CARTESIAN_POINT('Origin',(3.45995919230269,1076.73142393294,459.092773668652));
#125359=CARTESIAN_POINT('Origin',(3.45995919230269,1067.7251047501,459.092773668652));
#125360=CARTESIAN_POINT('',(3.45995919230269,1076.73142393294,458.363965705079));
#125361=CARTESIAN_POINT('Origin',(3.45995919230269,1076.73142393294,459.092773668652));
#125362=CARTESIAN_POINT('',(3.45995919230269,1082.7251047501,458.363965705079));
#125363=CARTESIAN_POINT('',(3.45995919230269,1067.7251047501,458.363965705079));
#125364=CARTESIAN_POINT('Origin',(3.45995919230269,1082.7251047501,459.092773668652));
#125365=CARTESIAN_POINT('Origin',(-0.430140047742333,1067.7251047501,467.507021385899));
#125366=CARTESIAN_POINT('',(-0.430140047742334,1078.73142393294,466.045904384082));
#125367=CARTESIAN_POINT('Origin',(-0.430140047742333,1078.73142393294,467.507021385899));
#125368=CARTESIAN_POINT('',(-0.430140047742334,1076.73142393294,466.045904384082));
#125369=CARTESIAN_POINT('',(-0.430140047742334,1067.7251047501,466.045904384082));
#125370=CARTESIAN_POINT('Origin',(-0.430140047742333,1076.73142393294,467.507021385899));
#125371=CARTESIAN_POINT('Origin',(-0.430140047742333,1067.7251047501,467.507021385899));
#125372=CARTESIAN_POINT('',(-0.430140047742333,1076.73142393294,466.645904384082));
#125373=CARTESIAN_POINT('Origin',(-0.430140047742333,1076.73142393294,467.507021385899));
#125374=CARTESIAN_POINT('',(-0.430140047742333,1082.7251047501,466.645904384082));
#125375=CARTESIAN_POINT('',(-0.430140047742333,1067.7251047501,466.645904384082));
#125376=CARTESIAN_POINT('Origin',(-0.430140047742333,1082.7251047501,467.507021385899));
#125377=CARTESIAN_POINT('Origin',(-6.05086325182613,1067.7251047501,474.433982927521));
#125378=CARTESIAN_POINT('',(-6.05086325182613,1078.73142393294,472.813500884896));
#125379=CARTESIAN_POINT('Origin',(-6.05086325182613,1078.73142393294,474.433982927521));
#125380=CARTESIAN_POINT('',(-6.05086325182613,1076.73142393294,472.813500884896));
#125381=CARTESIAN_POINT('',(-6.05086325182613,1067.7251047501,472.813500884896));
#125382=CARTESIAN_POINT('Origin',(-6.05086325182613,1076.73142393294,474.433982927521));
#125383=CARTESIAN_POINT('Origin',(-6.05086325182613,1067.7251047501,474.433982927521));
#125384=CARTESIAN_POINT('',(-6.05086325182613,1076.73142393294,473.413500884896));
#125385=CARTESIAN_POINT('Origin',(-6.05086325182613,1076.73142393294,474.433982927521));
#125386=CARTESIAN_POINT('',(-6.05086325182613,1082.7251047501,473.413500884896));
#125387=CARTESIAN_POINT('',(-6.05086325182613,1067.7251047501,473.413500884896));
#125388=CARTESIAN_POINT('Origin',(-6.05086325182613,1082.7251047501,474.433982927521));
#125389=CARTESIAN_POINT('Origin',(-13.4001510060405,1067.7251047501,481.469362813523));
#125390=CARTESIAN_POINT('',(-13.4001510060405,1078.73142393294,479.76836259044));
#125391=CARTESIAN_POINT('Origin',(-13.4001510060405,1078.73142393294,481.469362813523));
#125392=CARTESIAN_POINT('',(-13.4001510060405,1076.73142393294,479.76836259044));
#125393=CARTESIAN_POINT('',(-13.4001510060405,1067.7251047501,479.76836259044));
#125394=CARTESIAN_POINT('Origin',(-13.4001510060405,1076.73142393294,481.469362813523));
#125395=CARTESIAN_POINT('Origin',(-13.4001510060405,1067.7251047501,481.469362813523));
#125396=CARTESIAN_POINT('',(-13.4001510060405,1076.73142393294,480.36836259044));
#125397=CARTESIAN_POINT('Origin',(-13.4001510060405,1076.73142393294,481.469362813523));
#125398=CARTESIAN_POINT('',(-13.4001510060405,1082.7251047501,480.36836259044));
#125399=CARTESIAN_POINT('',(-13.4001510060405,1067.7251047501,480.36836259044));
#125400=CARTESIAN_POINT('Origin',(-13.4001510060405,1082.7251047501,481.469362813523));
#125401=CARTESIAN_POINT('Origin',(-21.8940327946431,1067.7251047501,486.488574417384));
#125402=CARTESIAN_POINT('',(-21.8940327946431,1078.73142393294,484.76729978534));
#125403=CARTESIAN_POINT('Origin',(-21.8940327946431,1078.73142393294,486.488574417384));
#125404=CARTESIAN_POINT('',(-21.8940327946431,1076.73142393294,484.76729978534));
#125405=CARTESIAN_POINT('',(-21.8940327946431,1067.7251047501,484.76729978534));
#125406=CARTESIAN_POINT('Origin',(-21.8940327946431,1076.73142393294,486.488574417384));
#125407=CARTESIAN_POINT('Origin',(-21.8940327946431,1067.7251047501,486.488574417384));
#125408=CARTESIAN_POINT('',(-21.8940327946431,1076.73142393294,485.36729978534));
#125409=CARTESIAN_POINT('Origin',(-21.8940327946431,1076.73142393294,486.488574417384));
#125410=CARTESIAN_POINT('',(-21.8940327946431,1082.7251047501,485.36729978534));
#125411=CARTESIAN_POINT('',(-21.8940327946431,1067.7251047501,485.36729978534));
#125412=CARTESIAN_POINT('Origin',(-21.8940327946431,1082.7251047501,486.488574417384));
#125413=CARTESIAN_POINT('Origin',(-32.2949960661494,1067.7251047501,491.13235549298));
#125414=CARTESIAN_POINT('',(-32.2949960661494,1078.73142393294,489.350362838575));
#125415=CARTESIAN_POINT('Origin',(-32.2949960661494,1078.73142393294,491.13235549298));
#125416=CARTESIAN_POINT('',(-32.2949960661494,1076.73142393294,489.350362838575));
#125417=CARTESIAN_POINT('',(-32.2949960661494,1067.7251047501,489.350362838575));
#125418=CARTESIAN_POINT('Origin',(-32.2949960661494,1076.73142393294,491.13235549298));
#125419=CARTESIAN_POINT('Origin',(-32.2949960661494,1067.7251047501,491.13235549298));
#125420=CARTESIAN_POINT('',(-32.2949960661494,1076.73142393294,489.950362838575));
#125421=CARTESIAN_POINT('Origin',(-32.2949960661494,1076.73142393294,491.13235549298));
#125422=CARTESIAN_POINT('',(-32.2949960661494,1082.7251047501,489.950362838575));
#125423=CARTESIAN_POINT('',(-32.2949960661494,1067.7251047501,489.950362838575));
#125424=CARTESIAN_POINT('Origin',(-32.2949960661494,1082.7251047501,491.13235549298));
#125425=CARTESIAN_POINT('Origin',(-43.2754163337326,1067.7251047501,493.447968680042));
#125426=CARTESIAN_POINT('',(-43.2754163337326,1078.73142393294,491.787087870121));
#125427=CARTESIAN_POINT('Origin',(-43.2754163337326,1078.73142393294,493.447968680042));
#125428=CARTESIAN_POINT('',(-43.2754163337326,1076.73142393294,491.787087870121));
#125429=CARTESIAN_POINT('',(-43.2754163337326,1067.7251047501,491.787087870121));
#125430=CARTESIAN_POINT('Origin',(-43.2754163337326,1076.73142393294,493.447968680042));
#125431=CARTESIAN_POINT('Origin',(-43.2754163337326,1067.7251047501,493.447968680042));
#125432=CARTESIAN_POINT('',(-43.2754163337326,1076.73142393294,492.387087870121));
#125433=CARTESIAN_POINT('Origin',(-43.2754163337326,1076.73142393294,493.447968680042));
#125434=CARTESIAN_POINT('',(-43.2754163337326,1082.7251047501,492.387087870121));
#125435=CARTESIAN_POINT('',(-43.2754163337326,1067.7251047501,492.387087870121));
#125436=CARTESIAN_POINT('Origin',(-43.2754163337326,1082.7251047501,493.447968680042));
#125437=CARTESIAN_POINT('Origin',(9.48479058284935,1067.7251047501,441.286911958076));
#125438=CARTESIAN_POINT('',(9.48479058284935,1078.73142393294,440.186553892402));
#125439=CARTESIAN_POINT('Origin',(9.48479058284935,1078.73142393294,441.286911958076));
#125440=CARTESIAN_POINT('',(9.48479058284935,1076.73142393294,440.186553892402));
#125441=CARTESIAN_POINT('',(9.48479058284935,1067.7251047501,440.186553892402));
#125442=CARTESIAN_POINT('Origin',(9.48479058284935,1076.73142393294,441.286911958076));
#125443=CARTESIAN_POINT('Origin',(9.48479058284935,1067.7251047501,441.286911958076));
#125444=CARTESIAN_POINT('',(9.48479058284935,1076.73142393294,440.786553892401));
#125445=CARTESIAN_POINT('Origin',(9.48479058284935,1076.73142393294,441.286911958076));
#125446=CARTESIAN_POINT('',(9.48479058284935,1082.7251047501,440.786553892401));
#125447=CARTESIAN_POINT('',(9.48479058284935,1067.7251047501,440.786553892401));
#125448=CARTESIAN_POINT('Origin',(9.48479058284935,1082.7251047501,441.286911958076));
#125449=CARTESIAN_POINT('Origin',(11.0355654939687,1067.7251047501,449.709053460442));
#125450=CARTESIAN_POINT('',(11.0355654939687,1078.73142393294,448.495021893705));
#125451=CARTESIAN_POINT('Origin',(11.0355654939687,1078.73142393294,449.709053460442));
#125452=CARTESIAN_POINT('',(11.0355654939687,1076.73142393294,448.495021893705));
#125453=CARTESIAN_POINT('',(11.0355654939687,1067.7251047501,448.495021893705));
#125454=CARTESIAN_POINT('Origin',(11.0355654939687,1076.73142393294,449.709053460442));
#125455=CARTESIAN_POINT('Origin',(11.0355654939687,1067.7251047501,449.709053460442));
#125456=CARTESIAN_POINT('',(11.0355654939687,1076.73142393294,449.095021893705));
#125457=CARTESIAN_POINT('Origin',(11.0355654939687,1076.73142393294,449.709053460442));
#125458=CARTESIAN_POINT('',(11.0355654939687,1082.7251047501,449.095021893705));
#125459=CARTESIAN_POINT('',(11.0355654939687,1067.7251047501,449.095021893705));
#125460=CARTESIAN_POINT('Origin',(11.0355654939687,1082.7251047501,449.709053460442));
#125461=CARTESIAN_POINT('Origin',(10.5515930080276,1067.7251047501,457.620100189752));
#125462=CARTESIAN_POINT('',(10.5515930080276,1078.73142393294,456.291292226178));
#125463=CARTESIAN_POINT('Origin',(10.5515930080276,1078.73142393294,457.620100189752));
#125464=CARTESIAN_POINT('',(10.5515930080276,1076.73142393294,456.291292226178));
#125465=CARTESIAN_POINT('',(10.5515930080276,1067.7251047501,456.291292226178));
#125466=CARTESIAN_POINT('Origin',(10.5515930080276,1076.73142393294,457.620100189752));
#125467=CARTESIAN_POINT('Origin',(10.5515930080276,1067.7251047501,457.620100189752));
#125468=CARTESIAN_POINT('',(10.5515930080276,1076.73142393294,456.891292226178));
#125469=CARTESIAN_POINT('Origin',(10.5515930080276,1076.73142393294,457.620100189752));
#125470=CARTESIAN_POINT('',(10.5515930080276,1082.7251047501,456.891292226178));
#125471=CARTESIAN_POINT('',(10.5515930080276,1067.7251047501,456.891292226178));
#125472=CARTESIAN_POINT('Origin',(10.5515930080276,1082.7251047501,457.620100189752));
#125473=CARTESIAN_POINT('Origin',(8.49592223961343,1067.7251047501,466.659273516803));
#125474=CARTESIAN_POINT('',(8.49592223961343,1078.73142393294,465.198156514986));
#125475=CARTESIAN_POINT('Origin',(8.49592223961343,1078.73142393294,466.659273516803));
#125476=CARTESIAN_POINT('',(8.49592223961343,1076.73142393294,465.198156514986));
#125477=CARTESIAN_POINT('',(8.49592223961343,1067.7251047501,465.198156514986));
#125478=CARTESIAN_POINT('Origin',(8.49592223961343,1076.73142393294,466.659273516803));
#125479=CARTESIAN_POINT('Origin',(8.49592223961343,1067.7251047501,466.659273516803));
#125480=CARTESIAN_POINT('',(8.49592223961343,1076.73142393294,465.798156514986));
#125481=CARTESIAN_POINT('Origin',(8.49592223961343,1076.73142393294,466.659273516803));
#125482=CARTESIAN_POINT('',(8.49592223961343,1082.7251047501,465.798156514986));
#125483=CARTESIAN_POINT('',(8.49592223961343,1067.7251047501,465.798156514986));
#125484=CARTESIAN_POINT('Origin',(8.49592223961343,1082.7251047501,466.659273516803));
#125485=CARTESIAN_POINT('Origin',(4.43822160949819,1067.7251047501,474.603478394095));
#125486=CARTESIAN_POINT('',(4.43822160949819,1078.73142393294,472.982996351471));
#125487=CARTESIAN_POINT('Origin',(4.43822160949819,1078.73142393294,474.603478394095));
#125488=CARTESIAN_POINT('',(4.43822160949819,1076.73142393294,472.982996351471));
#125489=CARTESIAN_POINT('',(4.43822160949819,1067.7251047501,472.982996351471));
#125490=CARTESIAN_POINT('Origin',(4.43822160949819,1076.73142393294,474.603478394095));
#125491=CARTESIAN_POINT('Origin',(4.43822160949819,1067.7251047501,474.603478394095));
#125492=CARTESIAN_POINT('',(4.43822160949819,1076.73142393294,473.582996351471));
#125493=CARTESIAN_POINT('Origin',(4.43822160949819,1076.73142393294,474.603478394095));
#125494=CARTESIAN_POINT('',(4.43822160949819,1082.7251047501,473.582996351471));
#125495=CARTESIAN_POINT('',(4.43822160949819,1067.7251047501,473.582996351471));
#125496=CARTESIAN_POINT('Origin',(4.43822160949819,1082.7251047501,474.603478394095));
#125497=CARTESIAN_POINT('Origin',(-1.28772884674494,1067.7251047501,483.013121193124));
#125498=CARTESIAN_POINT('',(-1.28772884674494,1078.73142393294,481.312120970041));
#125499=CARTESIAN_POINT('Origin',(-1.28772884674494,1078.73142393294,483.013121193124));
#125500=CARTESIAN_POINT('',(-1.28772884674494,1076.73142393294,481.312120970041));
#125501=CARTESIAN_POINT('',(-1.28772884674494,1067.7251047501,481.312120970041));
#125502=CARTESIAN_POINT('Origin',(-1.28772884674494,1076.73142393294,483.013121193124));
#125503=CARTESIAN_POINT('Origin',(-1.28772884674494,1067.7251047501,483.013121193124));
#125504=CARTESIAN_POINT('',(-1.28772884674494,1076.73142393294,481.912120970041));
#125505=CARTESIAN_POINT('Origin',(-1.28772884674494,1076.73142393294,483.013121193124));
#125506=CARTESIAN_POINT('',(-1.28772884674494,1082.7251047501,481.912120970041));
#125507=CARTESIAN_POINT('',(-1.28772884674494,1067.7251047501,481.912120970041));
#125508=CARTESIAN_POINT('Origin',(-1.28772884674494,1082.7251047501,483.013121193124));
#125509=CARTESIAN_POINT('Origin',(-8.5524461680524,1067.7251047501,489.68862830529));
#125510=CARTESIAN_POINT('',(-8.5524461680524,1078.73142393294,487.967353673247));
#125511=CARTESIAN_POINT('Origin',(-8.5524461680524,1078.73142393294,489.68862830529));
#125512=CARTESIAN_POINT('',(-8.5524461680524,1076.73142393294,487.967353673247));
#125513=CARTESIAN_POINT('',(-8.5524461680524,1067.7251047501,487.967353673247));
#125514=CARTESIAN_POINT('Origin',(-8.5524461680524,1076.73142393294,489.68862830529));
#125515=CARTESIAN_POINT('Origin',(-8.5524461680524,1067.7251047501,489.68862830529));
#125516=CARTESIAN_POINT('',(-8.5524461680524,1076.73142393294,488.567353673247));
#125517=CARTESIAN_POINT('Origin',(-8.5524461680524,1076.73142393294,489.68862830529));
#125518=CARTESIAN_POINT('',(-8.5524461680524,1082.7251047501,488.567353673247));
#125519=CARTESIAN_POINT('',(-8.5524461680524,1067.7251047501,488.567353673247));
#125520=CARTESIAN_POINT('Origin',(-8.5524461680524,1082.7251047501,489.68862830529));
#125521=CARTESIAN_POINT('Origin',(-17.760627062182,1067.7251047501,496.39341348263));
#125522=CARTESIAN_POINT('',(-17.760627062182,1078.73142393294,494.611420828225));
#125523=CARTESIAN_POINT('Origin',(-17.760627062182,1078.73142393294,496.39341348263));
#125524=CARTESIAN_POINT('',(-17.760627062182,1076.73142393294,494.611420828225));
#125525=CARTESIAN_POINT('',(-17.760627062182,1067.7251047501,494.611420828225));
#125526=CARTESIAN_POINT('Origin',(-17.760627062182,1076.73142393294,496.39341348263));
#125527=CARTESIAN_POINT('Origin',(-17.760627062182,1067.7251047501,496.39341348263));
#125528=CARTESIAN_POINT('',(-17.760627062182,1076.73142393294,495.211420828225));
#125529=CARTESIAN_POINT('Origin',(-17.760627062182,1076.73142393294,496.39341348263));
#125530=CARTESIAN_POINT('',(-17.760627062182,1082.7251047501,495.211420828225));
#125531=CARTESIAN_POINT('',(-17.760627062182,1067.7251047501,495.211420828225));
#125532=CARTESIAN_POINT('Origin',(-17.760627062182,1082.7251047501,496.39341348263));
#125533=CARTESIAN_POINT('Origin',(-28.0196557489654,1067.7251047501,500.941382709505));
#125534=CARTESIAN_POINT('',(-28.0196557489654,1078.73142393294,499.280501899584));
#125535=CARTESIAN_POINT('Origin',(-28.0196557489654,1078.73142393294,500.941382709505));
#125536=CARTESIAN_POINT('',(-28.0196557489654,1076.73142393294,499.280501899584));
#125537=CARTESIAN_POINT('',(-28.0196557489654,1067.7251047501,499.280501899584));
#125538=CARTESIAN_POINT('Origin',(-28.0196557489654,1076.73142393294,500.941382709505));
#125539=CARTESIAN_POINT('Origin',(-28.0196557489654,1067.7251047501,500.941382709505));
#125540=CARTESIAN_POINT('',(-28.0196557489654,1076.73142393294,499.880501899584));
#125541=CARTESIAN_POINT('Origin',(-28.0196557489654,1076.73142393294,500.941382709505));
#125542=CARTESIAN_POINT('',(-28.0196557489654,1082.7251047501,499.880501899584));
#125543=CARTESIAN_POINT('',(-28.0196557489654,1067.7251047501,499.880501899584));
#125544=CARTESIAN_POINT('Origin',(-28.0196557489654,1082.7251047501,500.941382709505));
#125545=CARTESIAN_POINT('Origin',(12.7427205628033,1067.7251047501,438.950706397253));
#125546=CARTESIAN_POINT('',(12.7427205628033,1078.73142393294,437.850348331578));
#125547=CARTESIAN_POINT('Origin',(12.7427205628033,1078.73142393294,438.950706397253));
#125548=CARTESIAN_POINT('',(12.7427205628033,1076.73142393294,437.850348331578));
#125549=CARTESIAN_POINT('',(12.7427205628033,1067.7251047501,437.850348331578));
#125550=CARTESIAN_POINT('Origin',(12.7427205628033,1076.73142393294,438.950706397253));
#125551=CARTESIAN_POINT('Origin',(12.7427205628033,1067.7251047501,438.950706397253));
#125552=CARTESIAN_POINT('',(12.7427205628033,1076.73142393294,438.450348331578));
#125553=CARTESIAN_POINT('Origin',(12.7427205628033,1076.73142393294,438.950706397253));
#125554=CARTESIAN_POINT('',(12.7427205628033,1082.7251047501,438.450348331578));
#125555=CARTESIAN_POINT('',(12.7427205628033,1067.7251047501,438.450348331578));
#125556=CARTESIAN_POINT('Origin',(12.7427205628033,1082.7251047501,438.950706397253));
#125557=CARTESIAN_POINT('Origin',(16.0106690014563,1067.7251047501,446.866379666985));
#125558=CARTESIAN_POINT('',(16.0106690014563,1078.73142393294,445.652348100247));
#125559=CARTESIAN_POINT('Origin',(16.0106690014563,1078.73142393294,446.866379666985));
#125560=CARTESIAN_POINT('',(16.0106690014563,1076.73142393294,445.652348100247));
#125561=CARTESIAN_POINT('',(16.0106690014563,1067.7251047501,445.652348100247));
#125562=CARTESIAN_POINT('Origin',(16.0106690014563,1076.73142393294,446.866379666985));
#125563=CARTESIAN_POINT('Origin',(16.0106690014563,1067.7251047501,446.866379666985));
#125564=CARTESIAN_POINT('',(16.0106690014563,1076.73142393294,446.252348100247));
#125565=CARTESIAN_POINT('Origin',(16.0106690014563,1076.73142393294,446.866379666985));
#125566=CARTESIAN_POINT('',(16.0106690014563,1082.7251047501,446.252348100247));
#125567=CARTESIAN_POINT('',(16.0106690014563,1067.7251047501,446.252348100247));
#125568=CARTESIAN_POINT('Origin',(16.0106690014563,1082.7251047501,446.866379666985));
#125569=CARTESIAN_POINT('Origin',(17.1820715771408,1067.7251047501,454.705174582413));
#125570=CARTESIAN_POINT('',(17.1820715771408,1078.73142393294,453.376366618839));
#125571=CARTESIAN_POINT('Origin',(17.1820715771408,1078.73142393294,454.705174582413));
#125572=CARTESIAN_POINT('',(17.1820715771408,1076.73142393294,453.376366618839));
#125573=CARTESIAN_POINT('',(17.1820715771408,1067.7251047501,453.376366618839));
#125574=CARTESIAN_POINT('Origin',(17.1820715771408,1076.73142393294,454.705174582413));
#125575=CARTESIAN_POINT('Origin',(17.1820715771408,1067.7251047501,454.705174582413));
#125576=CARTESIAN_POINT('',(17.1820715771408,1076.73142393294,453.976366618839));
#125577=CARTESIAN_POINT('Origin',(17.1820715771408,1076.73142393294,454.705174582413));
#125578=CARTESIAN_POINT('',(17.1820715771408,1082.7251047501,453.976366618839));
#125579=CARTESIAN_POINT('',(17.1820715771408,1067.7251047501,453.976366618839));
#125580=CARTESIAN_POINT('Origin',(17.1820715771408,1082.7251047501,454.705174582413));
#125581=CARTESIAN_POINT('Origin',(17.05067195714,1067.7251047501,463.974218270111));
#125582=CARTESIAN_POINT('',(17.05067195714,1078.73142393294,462.513101268294));
#125583=CARTESIAN_POINT('Origin',(17.05067195714,1078.73142393294,463.974218270111));
#125584=CARTESIAN_POINT('',(17.05067195714,1076.73142393294,462.513101268294));
#125585=CARTESIAN_POINT('',(17.05067195714,1067.7251047501,462.513101268294));
#125586=CARTESIAN_POINT('Origin',(17.05067195714,1076.73142393294,463.974218270111));
#125587=CARTESIAN_POINT('Origin',(17.05067195714,1067.7251047501,463.974218270111));
#125588=CARTESIAN_POINT('',(17.05067195714,1076.73142393294,463.113101268294));
#125589=CARTESIAN_POINT('Origin',(17.05067195714,1076.73142393294,463.974218270111));
#125590=CARTESIAN_POINT('',(17.05067195714,1082.7251047501,463.113101268294));
#125591=CARTESIAN_POINT('',(17.05067195714,1067.7251047501,463.113101268294));
#125592=CARTESIAN_POINT('Origin',(17.05067195714,1082.7251047501,463.974218270111));
#125593=CARTESIAN_POINT('Origin',(14.7333348895372,1067.7251047501,472.588466609411));
#125594=CARTESIAN_POINT('',(14.7333348895372,1078.73142393294,470.967984566787));
#125595=CARTESIAN_POINT('Origin',(14.7333348895372,1078.73142393294,472.588466609411));
#125596=CARTESIAN_POINT('',(14.7333348895372,1076.73142393294,470.967984566787));
#125597=CARTESIAN_POINT('',(14.7333348895372,1067.7251047501,470.967984566787));
#125598=CARTESIAN_POINT('Origin',(14.7333348895372,1076.73142393294,472.588466609411));
#125599=CARTESIAN_POINT('Origin',(14.7333348895372,1067.7251047501,472.588466609411));
#125600=CARTESIAN_POINT('',(14.7333348895372,1076.73142393294,471.567984566787));
#125601=CARTESIAN_POINT('Origin',(14.7333348895372,1076.73142393294,472.588466609411));
#125602=CARTESIAN_POINT('',(14.7333348895372,1082.7251047501,471.567984566787));
#125603=CARTESIAN_POINT('',(14.7333348895372,1067.7251047501,471.567984566787));
#125604=CARTESIAN_POINT('Origin',(14.7333348895372,1082.7251047501,472.588466609411));
#125605=CARTESIAN_POINT('Origin',(10.8809732423619,1067.7251047501,482.004830577206));
#125606=CARTESIAN_POINT('',(10.8809732423619,1078.73142393294,480.303830354124));
#125607=CARTESIAN_POINT('Origin',(10.8809732423619,1078.73142393294,482.004830577206));
#125608=CARTESIAN_POINT('',(10.8809732423619,1076.73142393294,480.303830354124));
#125609=CARTESIAN_POINT('',(10.8809732423619,1067.7251047501,480.303830354124));
#125610=CARTESIAN_POINT('Origin',(10.8809732423619,1076.73142393294,482.004830577206));
#125611=CARTESIAN_POINT('Origin',(10.8809732423619,1067.7251047501,482.004830577206));
#125612=CARTESIAN_POINT('',(10.8809732423619,1076.73142393294,480.903830354123));
#125613=CARTESIAN_POINT('Origin',(10.8809732423619,1076.73142393294,482.004830577206));
#125614=CARTESIAN_POINT('',(10.8809732423619,1082.7251047501,480.903830354123));
#125615=CARTESIAN_POINT('',(10.8809732423619,1067.7251047501,480.903830354123));
#125616=CARTESIAN_POINT('Origin',(10.8809732423619,1082.7251047501,482.004830577206));
#125617=CARTESIAN_POINT('Origin',(5.16292339527213,1067.7251047501,490.044881504239));
#125618=CARTESIAN_POINT('',(5.16292339527213,1078.73142393294,488.323606872196));
#125619=CARTESIAN_POINT('Origin',(5.16292339527213,1078.73142393294,490.044881504239));
#125620=CARTESIAN_POINT('',(5.16292339527213,1076.73142393294,488.323606872196));
#125621=CARTESIAN_POINT('',(5.16292339527213,1067.7251047501,488.323606872196));
#125622=CARTESIAN_POINT('Origin',(5.16292339527213,1076.73142393294,490.044881504239));
#125623=CARTESIAN_POINT('Origin',(5.16292339527213,1067.7251047501,490.044881504239));
#125624=CARTESIAN_POINT('',(5.16292339527213,1076.73142393294,488.923606872196));
#125625=CARTESIAN_POINT('Origin',(5.16292339527213,1076.73142393294,490.044881504239));
#125626=CARTESIAN_POINT('',(5.16292339527213,1082.7251047501,488.923606872196));
#125627=CARTESIAN_POINT('',(5.16292339527213,1067.7251047501,488.923606872196));
#125628=CARTESIAN_POINT('Origin',(5.16292339527213,1082.7251047501,490.044881504239));
#125629=CARTESIAN_POINT('Origin',(-2.45003343065298,1067.7251047501,498.517639497944));
#125630=CARTESIAN_POINT('',(-2.45003343065298,1078.73142393294,496.735646843539));
#125631=CARTESIAN_POINT('Origin',(-2.45003343065298,1078.73142393294,498.517639497944));
#125632=CARTESIAN_POINT('',(-2.45003343065298,1076.73142393294,496.735646843539));
#125633=CARTESIAN_POINT('',(-2.45003343065298,1067.7251047501,496.735646843539));
#125634=CARTESIAN_POINT('Origin',(-2.45003343065298,1076.73142393294,498.517639497944));
#125635=CARTESIAN_POINT('Origin',(-2.45003343065298,1067.7251047501,498.517639497944));
#125636=CARTESIAN_POINT('',(-2.45003343065298,1076.73142393294,497.335646843539));
#125637=CARTESIAN_POINT('Origin',(-2.45003343065298,1076.73142393294,498.517639497944));
#125638=CARTESIAN_POINT('',(-2.45003343065298,1082.7251047501,497.335646843539));
#125639=CARTESIAN_POINT('',(-2.45003343065298,1067.7251047501,497.335646843539));
#125640=CARTESIAN_POINT('Origin',(-2.45003343065298,1082.7251047501,498.517639497944));
#125641=CARTESIAN_POINT('Origin',(-11.5393017547428,1067.7251047501,505.09919668584));
#125642=CARTESIAN_POINT('',(-11.5393017547428,1078.73142393294,503.438315875919));
#125643=CARTESIAN_POINT('Origin',(-11.5393017547428,1078.73142393294,505.09919668584));
#125644=CARTESIAN_POINT('',(-11.5393017547428,1076.73142393294,503.438315875919));
#125645=CARTESIAN_POINT('',(-11.5393017547428,1067.7251047501,503.438315875919));
#125646=CARTESIAN_POINT('Origin',(-11.5393017547428,1076.73142393294,505.09919668584));
#125647=CARTESIAN_POINT('Origin',(-11.5393017547428,1067.7251047501,505.09919668584));
#125648=CARTESIAN_POINT('',(-11.5393017547428,1076.73142393294,504.038315875919));
#125649=CARTESIAN_POINT('Origin',(-11.5393017547428,1076.73142393294,505.09919668584));
#125650=CARTESIAN_POINT('',(-11.5393017547428,1082.7251047501,504.038315875919));
#125651=CARTESIAN_POINT('',(-11.5393017547428,1067.7251047501,504.038315875919));
#125652=CARTESIAN_POINT('Origin',(-11.5393017547428,1082.7251047501,505.09919668584));
#125653=CARTESIAN_POINT('Origin',(15.4437325078056,1067.7251047501,435.988190802415));
#125654=CARTESIAN_POINT('',(15.4437325078056,1078.73142393294,434.88783273674));
#125655=CARTESIAN_POINT('Origin',(15.4437325078056,1078.73142393294,435.988190802415));
#125656=CARTESIAN_POINT('',(15.4437325078056,1076.73142393294,434.88783273674));
#125657=CARTESIAN_POINT('',(15.4437325078056,1067.7251047501,434.88783273674));
#125658=CARTESIAN_POINT('Origin',(15.4437325078056,1076.73142393294,435.988190802415));
#125659=CARTESIAN_POINT('Origin',(15.4437325078056,1067.7251047501,435.988190802415));
#125660=CARTESIAN_POINT('',(15.4437325078056,1076.73142393294,435.48783273674));
#125661=CARTESIAN_POINT('Origin',(15.4437325078056,1076.73142393294,435.988190802415));
#125662=CARTESIAN_POINT('',(15.4437325078056,1082.7251047501,435.48783273674));
#125663=CARTESIAN_POINT('',(15.4437325078056,1067.7251047501,435.48783273674));
#125664=CARTESIAN_POINT('Origin',(15.4437325078056,1082.7251047501,435.988190802415));
#125665=CARTESIAN_POINT('Origin',(20.2860294458665,1067.7251047501,443.05144293401));
#125666=CARTESIAN_POINT('',(20.2860294458665,1078.73142393294,441.837411367273));
#125667=CARTESIAN_POINT('Origin',(20.2860294458665,1078.73142393294,443.05144293401));
#125668=CARTESIAN_POINT('',(20.2860294458665,1076.73142393294,441.837411367273));
#125669=CARTESIAN_POINT('',(20.2860294458665,1067.7251047501,441.837411367273));
#125670=CARTESIAN_POINT('Origin',(20.2860294458665,1076.73142393294,443.05144293401));
#125671=CARTESIAN_POINT('Origin',(20.2860294458665,1067.7251047501,443.05144293401));
#125672=CARTESIAN_POINT('',(20.2860294458665,1076.73142393294,442.437411367273));
#125673=CARTESIAN_POINT('Origin',(20.2860294458665,1076.73142393294,443.05144293401));
#125674=CARTESIAN_POINT('',(20.2860294458665,1082.7251047501,442.437411367273));
#125675=CARTESIAN_POINT('',(20.2860294458665,1067.7251047501,442.437411367273));
#125676=CARTESIAN_POINT('Origin',(20.2860294458665,1082.7251047501,443.05144293401));
#125677=CARTESIAN_POINT('Origin',(23.0616111696061,1067.7251047501,450.475393083042));
#125678=CARTESIAN_POINT('',(23.0616111696061,1078.73142393294,449.146585119468));
#125679=CARTESIAN_POINT('Origin',(23.0616111696061,1078.73142393294,450.475393083042));
#125680=CARTESIAN_POINT('',(23.0616111696061,1076.73142393294,449.146585119468));
#125681=CARTESIAN_POINT('',(23.0616111696061,1067.7251047501,449.146585119468));
#125682=CARTESIAN_POINT('Origin',(23.0616111696061,1076.73142393294,450.475393083042));
#125683=CARTESIAN_POINT('Origin',(23.0616111696061,1067.7251047501,450.475393083042));
#125684=CARTESIAN_POINT('',(23.0616111696061,1076.73142393294,449.746585119468));
#125685=CARTESIAN_POINT('Origin',(23.0616111696061,1076.73142393294,450.475393083042));
#125686=CARTESIAN_POINT('',(23.0616111696061,1082.7251047501,449.746585119468));
#125687=CARTESIAN_POINT('',(23.0616111696061,1067.7251047501,449.746585119468));
#125688=CARTESIAN_POINT('Origin',(23.0616111696061,1082.7251047501,450.475393083042));
#125689=CARTESIAN_POINT('Origin',(24.8602254919379,1067.7251047501,459.569205444427));
#125690=CARTESIAN_POINT('',(24.8602254919379,1078.73142393294,458.108088442611));
#125691=CARTESIAN_POINT('Origin',(24.8602254919379,1078.73142393294,459.569205444427));
#125692=CARTESIAN_POINT('',(24.8602254919379,1076.73142393294,458.108088442611));
#125693=CARTESIAN_POINT('',(24.8602254919379,1067.7251047501,458.108088442611));
#125694=CARTESIAN_POINT('Origin',(24.8602254919379,1076.73142393294,459.569205444427));
#125695=CARTESIAN_POINT('Origin',(24.8602254919379,1067.7251047501,459.569205444427));
#125696=CARTESIAN_POINT('',(24.8602254919379,1076.73142393294,458.708088442611));
#125697=CARTESIAN_POINT('Origin',(24.8602254919379,1076.73142393294,459.569205444427));
#125698=CARTESIAN_POINT('',(24.8602254919379,1082.7251047501,458.708088442611));
#125699=CARTESIAN_POINT('',(24.8602254919379,1067.7251047501,458.708088442611));
#125700=CARTESIAN_POINT('Origin',(24.8602254919379,1082.7251047501,459.569205444427));
#125701=CARTESIAN_POINT('Origin',(24.3845307365188,1067.7251047501,468.477013257559));
#125702=CARTESIAN_POINT('',(24.3845307365188,1078.73142393294,466.856531214935));
#125703=CARTESIAN_POINT('Origin',(24.3845307365188,1078.73142393294,468.477013257559));
#125704=CARTESIAN_POINT('',(24.3845307365188,1076.73142393294,466.856531214935));
#125705=CARTESIAN_POINT('',(24.3845307365188,1067.7251047501,466.856531214935));
#125706=CARTESIAN_POINT('Origin',(24.3845307365188,1076.73142393294,468.477013257559));
#125707=CARTESIAN_POINT('Origin',(24.3845307365188,1067.7251047501,468.477013257559));
#125708=CARTESIAN_POINT('',(24.3845307365188,1076.73142393294,467.456531214935));
#125709=CARTESIAN_POINT('Origin',(24.3845307365188,1076.73142393294,468.477013257559));
#125710=CARTESIAN_POINT('',(24.3845307365188,1082.7251047501,467.456531214935));
#125711=CARTESIAN_POINT('',(24.3845307365188,1067.7251047501,467.456531214935));
#125712=CARTESIAN_POINT('Origin',(24.3845307365188,1082.7251047501,468.477013257559));
#125713=CARTESIAN_POINT('Origin',(22.5741245880751,1067.7251047501,478.488558104));
#125714=CARTESIAN_POINT('',(22.5741245880751,1078.73142393294,476.787557880917));
#125715=CARTESIAN_POINT('Origin',(22.5741245880751,1078.73142393294,478.488558104));
#125716=CARTESIAN_POINT('',(22.5741245880751,1076.73142393294,476.787557880917));
#125717=CARTESIAN_POINT('',(22.5741245880751,1067.7251047501,476.787557880917));
#125718=CARTESIAN_POINT('Origin',(22.5741245880751,1076.73142393294,478.488558104));
#125719=CARTESIAN_POINT('Origin',(22.5741245880751,1067.7251047501,478.488558104));
#125720=CARTESIAN_POINT('',(22.5741245880751,1076.73142393294,477.387557880917));
#125721=CARTESIAN_POINT('Origin',(22.5741245880751,1076.73142393294,478.488558104));
#125722=CARTESIAN_POINT('',(22.5741245880751,1082.7251047501,477.387557880917));
#125723=CARTESIAN_POINT('',(22.5741245880751,1067.7251047501,477.387557880917));
#125724=CARTESIAN_POINT('Origin',(22.5741245880751,1082.7251047501,478.488558104));
#125725=CARTESIAN_POINT('Origin',(18.6526484317682,1067.7251047501,487.541764039943));
#125726=CARTESIAN_POINT('',(18.6526484317682,1078.73142393294,485.8204894079));
#125727=CARTESIAN_POINT('Origin',(18.6526484317682,1078.73142393294,487.541764039943));
#125728=CARTESIAN_POINT('',(18.6526484317682,1076.73142393294,485.8204894079));
#125729=CARTESIAN_POINT('',(18.6526484317682,1067.7251047501,485.8204894079));
#125730=CARTESIAN_POINT('Origin',(18.6526484317682,1076.73142393294,487.541764039943));
#125731=CARTESIAN_POINT('Origin',(18.6526484317682,1067.7251047501,487.541764039943));
#125732=CARTESIAN_POINT('',(18.6526484317682,1076.73142393294,486.4204894079));
#125733=CARTESIAN_POINT('Origin',(18.6526484317682,1076.73142393294,487.541764039943));
#125734=CARTESIAN_POINT('',(18.6526484317682,1082.7251047501,486.4204894079));
#125735=CARTESIAN_POINT('',(18.6526484317682,1067.7251047501,486.4204894079));
#125736=CARTESIAN_POINT('Origin',(18.6526484317682,1082.7251047501,487.541764039943));
#125737=CARTESIAN_POINT('Origin',(12.9676384183603,1067.7251047501,497.412194668885));
#125738=CARTESIAN_POINT('',(12.9676384183603,1078.73142393294,495.63020201448));
#125739=CARTESIAN_POINT('Origin',(12.9676384183603,1078.73142393294,497.412194668885));
#125740=CARTESIAN_POINT('',(12.9676384183603,1076.73142393294,495.63020201448));
#125741=CARTESIAN_POINT('',(12.9676384183603,1067.7251047501,495.63020201448));
#125742=CARTESIAN_POINT('Origin',(12.9676384183603,1076.73142393294,497.412194668885));
#125743=CARTESIAN_POINT('Origin',(12.9676384183603,1067.7251047501,497.412194668885));
#125744=CARTESIAN_POINT('',(12.9676384183603,1076.73142393294,496.23020201448));
#125745=CARTESIAN_POINT('Origin',(12.9676384183603,1076.73142393294,497.412194668885));
#125746=CARTESIAN_POINT('',(12.9676384183603,1082.7251047501,496.23020201448));
#125747=CARTESIAN_POINT('',(12.9676384183603,1067.7251047501,496.23020201448));
#125748=CARTESIAN_POINT('Origin',(12.9676384183603,1082.7251047501,497.412194668885));
#125749=CARTESIAN_POINT('Origin',(5.4453750978754,1067.7251047501,505.739694186875));
#125750=CARTESIAN_POINT('',(5.4453750978754,1078.73142393294,504.078813376954));
#125751=CARTESIAN_POINT('Origin',(5.4453750978754,1078.73142393294,505.739694186875));
#125752=CARTESIAN_POINT('',(5.4453750978754,1076.73142393294,504.078813376954));
#125753=CARTESIAN_POINT('',(5.4453750978754,1067.7251047501,504.078813376954));
#125754=CARTESIAN_POINT('Origin',(5.4453750978754,1076.73142393294,505.739694186875));
#125755=CARTESIAN_POINT('Origin',(5.4453750978754,1067.7251047501,505.739694186875));
#125756=CARTESIAN_POINT('',(5.4453750978754,1076.73142393294,504.678813376955));
#125757=CARTESIAN_POINT('Origin',(5.4453750978754,1076.73142393294,505.739694186875));
#125758=CARTESIAN_POINT('',(5.4453750978754,1082.7251047501,504.678813376955));
#125759=CARTESIAN_POINT('',(5.4453750978754,1067.7251047501,504.678813376955));
#125760=CARTESIAN_POINT('Origin',(5.4453750978754,1082.7251047501,505.739694186875));
#125761=CARTESIAN_POINT('Origin',(17.4697792349661,1067.7251047501,432.528841320783));
#125762=CARTESIAN_POINT('',(17.4697792349661,1078.73142393294,431.428483255108));
#125763=CARTESIAN_POINT('Origin',(17.4697792349661,1078.73142393294,432.528841320783));
#125764=CARTESIAN_POINT('',(17.4697792349661,1076.73142393294,431.428483255108));
#125765=CARTESIAN_POINT('',(17.4697792349661,1067.7251047501,431.428483255108));
#125766=CARTESIAN_POINT('Origin',(17.4697792349661,1076.73142393294,432.528841320783));
#125767=CARTESIAN_POINT('Origin',(17.4697792349661,1067.7251047501,432.528841320783));
#125768=CARTESIAN_POINT('',(17.4697792349661,1076.73142393294,432.028483255108));
#125769=CARTESIAN_POINT('Origin',(17.4697792349661,1076.73142393294,432.528841320783));
#125770=CARTESIAN_POINT('',(17.4697792349661,1082.7251047501,432.028483255108));
#125771=CARTESIAN_POINT('',(17.4697792349661,1067.7251047501,432.028483255108));
#125772=CARTESIAN_POINT('Origin',(17.4697792349661,1082.7251047501,432.528841320783));
#125773=CARTESIAN_POINT('Origin',(23.6747930603231,1067.7251047501,438.430974302847));
#125774=CARTESIAN_POINT('',(23.6747930603231,1078.73142393294,437.21694273611));
#125775=CARTESIAN_POINT('Origin',(23.6747930603231,1078.73142393294,438.430974302847));
#125776=CARTESIAN_POINT('',(23.6747930603231,1076.73142393294,437.21694273611));
#125777=CARTESIAN_POINT('',(23.6747930603231,1067.7251047501,437.21694273611));
#125778=CARTESIAN_POINT('Origin',(23.6747930603231,1076.73142393294,438.430974302847));
#125779=CARTESIAN_POINT('Origin',(23.6747930603231,1067.7251047501,438.430974302847));
#125780=CARTESIAN_POINT('',(23.6747930603231,1076.73142393294,437.81694273611));
#125781=CARTESIAN_POINT('Origin',(23.6747930603231,1076.73142393294,438.430974302847));
#125782=CARTESIAN_POINT('',(23.6747930603231,1082.7251047501,437.81694273611));
#125783=CARTESIAN_POINT('',(23.6747930603231,1067.7251047501,437.81694273611));
#125784=CARTESIAN_POINT('Origin',(23.6747930603231,1082.7251047501,438.430974302847));
#125785=CARTESIAN_POINT('Origin',(27.9332476920715,1067.7251047501,445.115617439904));
#125786=CARTESIAN_POINT('',(27.9332476920715,1078.73142393294,443.786809476331));
#125787=CARTESIAN_POINT('Origin',(27.9332476920715,1078.73142393294,445.115617439904));
#125788=CARTESIAN_POINT('',(27.9332476920715,1076.73142393294,443.786809476331));
#125789=CARTESIAN_POINT('',(27.9332476920715,1067.7251047501,443.786809476331));
#125790=CARTESIAN_POINT('Origin',(27.9332476920715,1076.73142393294,445.115617439904));
#125791=CARTESIAN_POINT('Origin',(27.9332476920715,1067.7251047501,445.115617439904));
#125792=CARTESIAN_POINT('',(27.9332476920715,1076.73142393294,444.386809476331));
#125793=CARTESIAN_POINT('Origin',(27.9332476920715,1076.73142393294,445.115617439904));
#125794=CARTESIAN_POINT('',(27.9332476920715,1082.7251047501,444.386809476331));
#125795=CARTESIAN_POINT('',(27.9332476920715,1067.7251047501,444.386809476331));
#125796=CARTESIAN_POINT('Origin',(27.9332476920715,1082.7251047501,445.115617439904));
#125797=CARTESIAN_POINT('Origin',(31.583267880141,1067.7251047501,453.636755237832));
#125798=CARTESIAN_POINT('',(31.583267880141,1078.73142393294,452.175638236015));
#125799=CARTESIAN_POINT('Origin',(31.583267880141,1078.73142393294,453.636755237832));
#125800=CARTESIAN_POINT('',(31.583267880141,1076.73142393294,452.175638236015));
#125801=CARTESIAN_POINT('',(31.583267880141,1067.7251047501,452.175638236015));
#125802=CARTESIAN_POINT('Origin',(31.583267880141,1076.73142393294,453.636755237832));
#125803=CARTESIAN_POINT('Origin',(31.583267880141,1067.7251047501,453.636755237832));
#125804=CARTESIAN_POINT('',(31.583267880141,1076.73142393294,452.775638236015));
#125805=CARTESIAN_POINT('Origin',(31.583267880141,1076.73142393294,453.636755237832));
#125806=CARTESIAN_POINT('',(31.583267880141,1082.7251047501,452.775638236015));
#125807=CARTESIAN_POINT('',(31.583267880141,1067.7251047501,452.775638236015));
#125808=CARTESIAN_POINT('Origin',(31.583267880141,1082.7251047501,453.636755237832));
#125809=CARTESIAN_POINT('Origin',(32.9700055803541,1067.7251047501,462.448808578957));
#125810=CARTESIAN_POINT('',(32.9700055803541,1078.73142393294,460.828326536333));
#125811=CARTESIAN_POINT('Origin',(32.9700055803541,1078.73142393294,462.448808578957));
#125812=CARTESIAN_POINT('',(32.9700055803541,1076.73142393294,460.828326536333));
#125813=CARTESIAN_POINT('',(32.9700055803541,1067.7251047501,460.828326536333));
#125814=CARTESIAN_POINT('Origin',(32.9700055803541,1076.73142393294,462.448808578957));
#125815=CARTESIAN_POINT('Origin',(32.9700055803541,1067.7251047501,462.448808578957));
#125816=CARTESIAN_POINT('',(32.9700055803541,1076.73142393294,461.428326536333));
#125817=CARTESIAN_POINT('Origin',(32.9700055803541,1076.73142393294,462.448808578957));
#125818=CARTESIAN_POINT('',(32.9700055803541,1082.7251047501,461.428326536333));
#125819=CARTESIAN_POINT('',(32.9700055803541,1067.7251047501,461.428326536333));
#125820=CARTESIAN_POINT('Origin',(32.9700055803541,1082.7251047501,462.448808578957));
#125821=CARTESIAN_POINT('Origin',(33.2806783666214,1067.7251047501,472.617981753532));
#125822=CARTESIAN_POINT('',(33.2806783666214,1078.73142393294,470.916981530449));
#125823=CARTESIAN_POINT('Origin',(33.2806783666214,1078.73142393294,472.617981753532));
#125824=CARTESIAN_POINT('',(33.2806783666214,1076.73142393294,470.916981530449));
#125825=CARTESIAN_POINT('',(33.2806783666214,1067.7251047501,470.916981530449));
#125826=CARTESIAN_POINT('Origin',(33.2806783666214,1076.73142393294,472.617981753532));
#125827=CARTESIAN_POINT('Origin',(33.2806783666214,1067.7251047501,472.617981753532));
#125828=CARTESIAN_POINT('',(33.2806783666214,1076.73142393294,471.516981530449));
#125829=CARTESIAN_POINT('Origin',(33.2806783666214,1076.73142393294,472.617981753532));
#125830=CARTESIAN_POINT('',(33.2806783666214,1082.7251047501,471.516981530449));
#125831=CARTESIAN_POINT('',(33.2806783666214,1067.7251047501,471.516981530449));
#125832=CARTESIAN_POINT('Origin',(33.2806783666214,1082.7251047501,472.617981753532));
#125833=CARTESIAN_POINT('Origin',(31.3271632264583,1067.7251047501,482.288674156883));
#125834=CARTESIAN_POINT('',(31.3271632264583,1078.73142393294,480.56739952484));
#125835=CARTESIAN_POINT('Origin',(31.3271632264583,1078.73142393294,482.288674156883));
#125836=CARTESIAN_POINT('',(31.3271632264583,1076.73142393294,480.56739952484));
#125837=CARTESIAN_POINT('',(31.3271632264583,1067.7251047501,480.56739952484));
#125838=CARTESIAN_POINT('Origin',(31.3271632264583,1076.73142393294,482.288674156883));
#125839=CARTESIAN_POINT('Origin',(31.3271632264583,1067.7251047501,482.288674156883));
#125840=CARTESIAN_POINT('',(31.3271632264583,1076.73142393294,481.16739952484));
#125841=CARTESIAN_POINT('Origin',(31.3271632264583,1076.73142393294,482.288674156883));
#125842=CARTESIAN_POINT('',(31.3271632264583,1082.7251047501,481.16739952484));
#125843=CARTESIAN_POINT('',(31.3271632264583,1067.7251047501,481.16739952484));
#125844=CARTESIAN_POINT('Origin',(31.3271632264583,1082.7251047501,482.288674156883));
#125845=CARTESIAN_POINT('Origin',(27.8185622428584,1067.7251047501,493.125392238995));
#125846=CARTESIAN_POINT('',(27.8185622428584,1078.73142393294,491.34339958459));
#125847=CARTESIAN_POINT('Origin',(27.8185622428584,1078.73142393294,493.125392238995));
#125848=CARTESIAN_POINT('',(27.8185622428584,1076.73142393294,491.34339958459));
#125849=CARTESIAN_POINT('',(27.8185622428584,1067.7251047501,491.34339958459));
#125850=CARTESIAN_POINT('Origin',(27.8185622428584,1076.73142393294,493.125392238995));
#125851=CARTESIAN_POINT('Origin',(27.8185622428584,1067.7251047501,493.125392238995));
#125852=CARTESIAN_POINT('',(27.8185622428584,1076.73142393294,491.94339958459));
#125853=CARTESIAN_POINT('Origin',(27.8185622428584,1076.73142393294,493.125392238995));
#125854=CARTESIAN_POINT('',(27.8185622428584,1082.7251047501,491.94339958459));
#125855=CARTESIAN_POINT('',(27.8185622428584,1067.7251047501,491.94339958459));
#125856=CARTESIAN_POINT('Origin',(27.8185622428584,1082.7251047501,493.125392238995));
#125857=CARTESIAN_POINT('Origin',(22.1920629289076,1067.7251047501,502.834882398368));
#125858=CARTESIAN_POINT('',(22.1920629289076,1078.73142393294,501.174001588447));
#125859=CARTESIAN_POINT('Origin',(22.1920629289076,1078.73142393294,502.834882398368));
#125860=CARTESIAN_POINT('',(22.1920629289076,1076.73142393294,501.174001588447));
#125861=CARTESIAN_POINT('',(22.1920629289076,1067.7251047501,501.174001588447));
#125862=CARTESIAN_POINT('Origin',(22.1920629289076,1076.73142393294,502.834882398368));
#125863=CARTESIAN_POINT('Origin',(22.1920629289076,1067.7251047501,502.834882398368));
#125864=CARTESIAN_POINT('',(22.1920629289076,1076.73142393294,501.774001588447));
#125865=CARTESIAN_POINT('Origin',(22.1920629289076,1076.73142393294,502.834882398368));
#125866=CARTESIAN_POINT('',(22.1920629289076,1082.7251047501,501.774001588447));
#125867=CARTESIAN_POINT('',(22.1920629289076,1067.7251047501,501.774001588447));
#125868=CARTESIAN_POINT('Origin',(22.1920629289076,1082.7251047501,502.834882398368));
#125869=CARTESIAN_POINT('Origin',(18.7323127802571,1067.7251047501,428.723848124506));
#125870=CARTESIAN_POINT('',(18.7323127802571,1078.73142393294,427.623490058831));
#125871=CARTESIAN_POINT('Origin',(18.7323127802571,1078.73142393294,428.723848124506));
#125872=CARTESIAN_POINT('',(18.7323127802571,1076.73142393294,427.623490058831));
#125873=CARTESIAN_POINT('',(18.7323127802571,1067.7251047501,427.623490058831));
#125874=CARTESIAN_POINT('Origin',(18.7323127802571,1076.73142393294,428.723848124506));
#125875=CARTESIAN_POINT('Origin',(18.7323127802571,1067.7251047501,428.723848124506));
#125876=CARTESIAN_POINT('',(18.7323127802571,1076.73142393294,428.223490058831));
#125877=CARTESIAN_POINT('Origin',(18.7323127802571,1076.73142393294,428.723848124506));
#125878=CARTESIAN_POINT('',(18.7323127802571,1082.7251047501,428.223490058831));
#125879=CARTESIAN_POINT('',(18.7323127802571,1067.7251047501,428.223490058831));
#125880=CARTESIAN_POINT('Origin',(18.7323127802571,1082.7251047501,428.723848124506));
#125881=CARTESIAN_POINT('Origin',(26.0288546137823,1067.7251047501,433.206910424145));
#125882=CARTESIAN_POINT('',(26.0288546137823,1078.73142393294,431.992878857408));
#125883=CARTESIAN_POINT('Origin',(26.0288546137823,1078.73142393294,433.206910424145));
#125884=CARTESIAN_POINT('',(26.0288546137823,1076.73142393294,431.992878857408));
#125885=CARTESIAN_POINT('',(26.0288546137823,1067.7251047501,431.992878857408));
#125886=CARTESIAN_POINT('Origin',(26.0288546137823,1076.73142393294,433.206910424145));
#125887=CARTESIAN_POINT('Origin',(26.0288546137823,1067.7251047501,433.206910424145));
#125888=CARTESIAN_POINT('',(26.0288546137823,1076.73142393294,432.592878857408));
#125889=CARTESIAN_POINT('Origin',(26.0288546137823,1076.73142393294,433.206910424145));
#125890=CARTESIAN_POINT('',(26.0288546137823,1082.7251047501,432.592878857408));
#125891=CARTESIAN_POINT('',(26.0288546137823,1067.7251047501,432.592878857408));
#125892=CARTESIAN_POINT('Origin',(26.0288546137823,1082.7251047501,433.206910424145));
#125893=CARTESIAN_POINT('Origin',(31.5840672517996,1067.7251047501,438.860095567662));
#125894=CARTESIAN_POINT('',(31.5840672517996,1078.73142393294,437.531287604089));
#125895=CARTESIAN_POINT('Origin',(31.5840672517996,1078.73142393294,438.860095567662));
#125896=CARTESIAN_POINT('',(31.5840672517996,1076.73142393294,437.531287604089));
#125897=CARTESIAN_POINT('',(31.5840672517996,1067.7251047501,437.531287604089));
#125898=CARTESIAN_POINT('Origin',(31.5840672517996,1076.73142393294,438.860095567662));
#125899=CARTESIAN_POINT('Origin',(31.5840672517996,1067.7251047501,438.860095567662));
#125900=CARTESIAN_POINT('',(31.5840672517996,1076.73142393294,438.131287604089));
#125901=CARTESIAN_POINT('Origin',(31.5840672517996,1076.73142393294,438.860095567662));
#125902=CARTESIAN_POINT('',(31.5840672517996,1082.7251047501,438.131287604089));
#125903=CARTESIAN_POINT('',(31.5840672517996,1067.7251047501,438.131287604089));
#125904=CARTESIAN_POINT('Origin',(31.5840672517996,1082.7251047501,438.860095567662));
#125905=CARTESIAN_POINT('Origin',(36.9259699086481,1067.7251047501,446.436144191407));
#125906=CARTESIAN_POINT('',(36.9259699086481,1078.73142393294,444.97502718959));
#125907=CARTESIAN_POINT('Origin',(36.9259699086481,1078.73142393294,446.436144191407));
#125908=CARTESIAN_POINT('',(36.9259699086481,1076.73142393294,444.97502718959));
#125909=CARTESIAN_POINT('',(36.9259699086481,1067.7251047501,444.97502718959));
#125910=CARTESIAN_POINT('Origin',(36.9259699086481,1076.73142393294,446.436144191407));
#125911=CARTESIAN_POINT('Origin',(36.9259699086481,1067.7251047501,446.436144191407));
#125912=CARTESIAN_POINT('',(36.9259699086481,1076.73142393294,445.57502718959));
#125913=CARTESIAN_POINT('Origin',(36.9259699086481,1076.73142393294,446.436144191407));
#125914=CARTESIAN_POINT('',(36.9259699086481,1082.7251047501,445.57502718959));
#125915=CARTESIAN_POINT('',(36.9259699086481,1067.7251047501,445.57502718959));
#125916=CARTESIAN_POINT('Origin',(36.9259699086481,1082.7251047501,446.436144191407));
#125917=CARTESIAN_POINT('Origin',(40.1145329726883,1067.7251047501,454.767314044595));
#125918=CARTESIAN_POINT('',(40.1145329726883,1078.73142393294,453.14683200197));
#125919=CARTESIAN_POINT('Origin',(40.1145329726883,1078.73142393294,454.767314044595));
#125920=CARTESIAN_POINT('',(40.1145329726883,1076.73142393294,453.14683200197));
#125921=CARTESIAN_POINT('',(40.1145329726883,1067.7251047501,453.14683200197));
#125922=CARTESIAN_POINT('Origin',(40.1145329726883,1076.73142393294,454.767314044595));
#125923=CARTESIAN_POINT('Origin',(40.1145329726883,1067.7251047501,454.767314044595));
#125924=CARTESIAN_POINT('',(40.1145329726883,1076.73142393294,453.74683200197));
#125925=CARTESIAN_POINT('Origin',(40.1145329726883,1076.73142393294,454.767314044595));
#125926=CARTESIAN_POINT('',(40.1145329726883,1082.7251047501,453.74683200197));
#125927=CARTESIAN_POINT('',(40.1145329726883,1067.7251047501,453.74683200197));
#125928=CARTESIAN_POINT('Origin',(40.1145329726883,1082.7251047501,454.767314044595));
#125929=CARTESIAN_POINT('Origin',(42.5327068021333,1067.7251047501,464.649673882468));
#125930=CARTESIAN_POINT('',(42.5327068021333,1078.73142393294,462.948673659385));
#125931=CARTESIAN_POINT('Origin',(42.5327068021333,1078.73142393294,464.649673882468));
#125932=CARTESIAN_POINT('',(42.5327068021333,1076.73142393294,462.948673659385));
#125933=CARTESIAN_POINT('',(42.5327068021333,1067.7251047501,462.948673659385));
#125934=CARTESIAN_POINT('Origin',(42.5327068021333,1076.73142393294,464.649673882468));
#125935=CARTESIAN_POINT('Origin',(42.5327068021333,1067.7251047501,464.649673882468));
#125936=CARTESIAN_POINT('',(42.5327068021333,1076.73142393294,463.548673659385));
#125937=CARTESIAN_POINT('Origin',(42.5327068021333,1076.73142393294,464.649673882468));
#125938=CARTESIAN_POINT('',(42.5327068021333,1082.7251047501,463.548673659385));
#125939=CARTESIAN_POINT('',(42.5327068021333,1067.7251047501,463.548673659385));
#125940=CARTESIAN_POINT('Origin',(42.5327068021333,1082.7251047501,464.649673882468));
#125941=CARTESIAN_POINT('Origin',(42.6325306637449,1067.7251047501,474.51519709007));
#125942=CARTESIAN_POINT('',(42.6325306637449,1078.73142393294,472.793922458026));
#125943=CARTESIAN_POINT('Origin',(42.6325306637449,1078.73142393294,474.51519709007));
#125944=CARTESIAN_POINT('',(42.6325306637449,1076.73142393294,472.793922458026));
#125945=CARTESIAN_POINT('',(42.6325306637449,1067.7251047501,472.793922458026));
#125946=CARTESIAN_POINT('Origin',(42.6325306637449,1076.73142393294,474.51519709007));
#125947=CARTESIAN_POINT('Origin',(42.6325306637449,1067.7251047501,474.51519709007));
#125948=CARTESIAN_POINT('',(42.6325306637449,1076.73142393294,473.393922458026));
#125949=CARTESIAN_POINT('Origin',(42.6325306637449,1076.73142393294,474.51519709007));
#125950=CARTESIAN_POINT('',(42.6325306637449,1082.7251047501,473.393922458026));
#125951=CARTESIAN_POINT('',(42.6325306637449,1067.7251047501,473.393922458026));
#125952=CARTESIAN_POINT('Origin',(42.6325306637449,1082.7251047501,474.51519709007));
#125953=CARTESIAN_POINT('Origin',(41.4536814090717,1067.7251047501,485.844586044821));
#125954=CARTESIAN_POINT('',(41.4536814090717,1078.73142393294,484.062593390416));
#125955=CARTESIAN_POINT('Origin',(41.4536814090717,1078.73142393294,485.844586044821));
#125956=CARTESIAN_POINT('',(41.4536814090717,1076.73142393294,484.062593390416));
#125957=CARTESIAN_POINT('',(41.4536814090717,1067.7251047501,484.062593390416));
#125958=CARTESIAN_POINT('Origin',(41.4536814090717,1076.73142393294,485.844586044821));
#125959=CARTESIAN_POINT('Origin',(41.4536814090717,1067.7251047501,485.844586044821));
#125960=CARTESIAN_POINT('',(41.4536814090717,1076.73142393294,484.662593390416));
#125961=CARTESIAN_POINT('Origin',(41.4536814090717,1076.73142393294,485.844586044821));
#125962=CARTESIAN_POINT('',(41.4536814090717,1082.7251047501,484.662593390416));
#125963=CARTESIAN_POINT('',(41.4536814090717,1067.7251047501,484.662593390416));
#125964=CARTESIAN_POINT('Origin',(41.4536814090717,1082.7251047501,485.844586044821));
#125965=CARTESIAN_POINT('Origin',(37.9688511206139,1067.7251047501,496.511715534309));
#125966=CARTESIAN_POINT('',(37.9688511206139,1078.73142393294,494.850834724388));
#125967=CARTESIAN_POINT('Origin',(37.9688511206139,1078.73142393294,496.511715534309));
#125968=CARTESIAN_POINT('',(37.9688511206139,1076.73142393294,494.850834724388));
#125969=CARTESIAN_POINT('',(37.9688511206139,1067.7251047501,494.850834724388));
#125970=CARTESIAN_POINT('Origin',(37.9688511206139,1076.73142393294,496.511715534309));
#125971=CARTESIAN_POINT('Origin',(37.9688511206139,1067.7251047501,496.511715534309));
#125972=CARTESIAN_POINT('',(37.9688511206139,1076.73142393294,495.450834724388));
#125973=CARTESIAN_POINT('Origin',(37.9688511206139,1076.73142393294,496.511715534309));
#125974=CARTESIAN_POINT('',(37.9688511206139,1082.7251047501,495.450834724388));
#125975=CARTESIAN_POINT('',(37.9688511206139,1067.7251047501,495.450834724388));
#125976=CARTESIAN_POINT('Origin',(37.9688511206139,1082.7251047501,496.511715534309));
#125977=CARTESIAN_POINT('Origin',(19.1761543694413,1067.7251047501,424.739507674643));
#125978=CARTESIAN_POINT('',(19.1761543694413,1078.73142393294,423.639149608968));
#125979=CARTESIAN_POINT('Origin',(19.1761543694413,1078.73142393294,424.739507674643));
#125980=CARTESIAN_POINT('',(19.1761543694413,1076.73142393294,423.639149608968));
#125981=CARTESIAN_POINT('',(19.1761543694413,1067.7251047501,423.639149608968));
#125982=CARTESIAN_POINT('Origin',(19.1761543694413,1076.73142393294,424.739507674643));
#125983=CARTESIAN_POINT('Origin',(19.1761543694413,1067.7251047501,424.739507674643));
#125984=CARTESIAN_POINT('',(19.1761543694413,1076.73142393294,424.239149608968));
#125985=CARTESIAN_POINT('Origin',(19.1761543694413,1076.73142393294,424.739507674643));
#125986=CARTESIAN_POINT('',(19.1761543694413,1082.7251047501,424.239149608968));
#125987=CARTESIAN_POINT('',(19.1761543694413,1067.7251047501,424.239149608968));
#125988=CARTESIAN_POINT('Origin',(19.1761543694413,1082.7251047501,424.739507674643));
#125989=CARTESIAN_POINT('Origin',(27.2453303203172,1067.7251047501,427.607567957245));
#125990=CARTESIAN_POINT('',(27.2453303203172,1078.73142393294,426.393536390508));
#125991=CARTESIAN_POINT('Origin',(27.2453303203172,1078.73142393294,427.607567957245));
#125992=CARTESIAN_POINT('',(27.2453303203172,1076.73142393294,426.393536390508));
#125993=CARTESIAN_POINT('',(27.2453303203172,1067.7251047501,426.393536390508));
#125994=CARTESIAN_POINT('Origin',(27.2453303203172,1076.73142393294,427.607567957245));
#125995=CARTESIAN_POINT('Origin',(27.2453303203172,1067.7251047501,427.607567957245));
#125996=CARTESIAN_POINT('',(27.2453303203172,1076.73142393294,426.993536390508));
#125997=CARTESIAN_POINT('Origin',(27.2453303203172,1076.73142393294,427.607567957245));
#125998=CARTESIAN_POINT('',(27.2453303203172,1082.7251047501,426.993536390508));
#125999=CARTESIAN_POINT('',(27.2453303203172,1067.7251047501,426.993536390508));
#126000=CARTESIAN_POINT('Origin',(27.2453303203172,1082.7251047501,427.607567957245));
#126001=CARTESIAN_POINT('Origin',(33.8545115154544,1067.7251047501,431.982223789457));
#126002=CARTESIAN_POINT('',(33.8545115154544,1078.73142393294,430.653415825884));
#126003=CARTESIAN_POINT('Origin',(33.8545115154544,1078.73142393294,431.982223789457));
#126004=CARTESIAN_POINT('',(33.8545115154544,1076.73142393294,430.653415825884));
#126005=CARTESIAN_POINT('',(33.8545115154544,1067.7251047501,430.653415825884));
#126006=CARTESIAN_POINT('Origin',(33.8545115154544,1076.73142393294,431.982223789457));
#126007=CARTESIAN_POINT('Origin',(33.8545115154544,1067.7251047501,431.982223789457));
#126008=CARTESIAN_POINT('',(33.8545115154544,1076.73142393294,431.253415825884));
#126009=CARTESIAN_POINT('Origin',(33.8545115154544,1076.73142393294,431.982223789457));
#126010=CARTESIAN_POINT('',(33.8545115154544,1082.7251047501,431.253415825884));
#126011=CARTESIAN_POINT('',(33.8545115154544,1067.7251047501,431.253415825884));
#126012=CARTESIAN_POINT('Origin',(33.8545115154544,1082.7251047501,431.982223789457));
#126013=CARTESIAN_POINT('Origin',(40.6548298616846,1067.7251047501,438.282073560247));
#126014=CARTESIAN_POINT('',(40.6548298616846,1078.73142393294,436.82095655843));
#126015=CARTESIAN_POINT('Origin',(40.6548298616846,1078.73142393294,438.282073560247));
#126016=CARTESIAN_POINT('',(40.6548298616846,1076.73142393294,436.82095655843));
#126017=CARTESIAN_POINT('',(40.6548298616846,1067.7251047501,436.82095655843));
#126018=CARTESIAN_POINT('Origin',(40.6548298616846,1076.73142393294,438.282073560247));
#126019=CARTESIAN_POINT('Origin',(40.6548298616846,1067.7251047501,438.282073560247));
#126020=CARTESIAN_POINT('',(40.6548298616846,1076.73142393294,437.42095655843));
#126021=CARTESIAN_POINT('Origin',(40.6548298616846,1076.73142393294,438.282073560247));
#126022=CARTESIAN_POINT('',(40.6548298616846,1082.7251047501,437.42095655843));
#126023=CARTESIAN_POINT('',(40.6548298616846,1067.7251047501,437.42095655843));
#126024=CARTESIAN_POINT('Origin',(40.6548298616846,1082.7251047501,438.282073560247));
#126025=CARTESIAN_POINT('Origin',(45.5058627832302,1067.7251047501,445.768247825525));
#126026=CARTESIAN_POINT('',(45.5058627832302,1078.73142393294,444.1477657829));
#126027=CARTESIAN_POINT('Origin',(45.5058627832302,1078.73142393294,445.768247825525));
#126028=CARTESIAN_POINT('',(45.5058627832302,1076.73142393294,444.1477657829));
#126029=CARTESIAN_POINT('',(45.5058627832302,1067.7251047501,444.1477657829));
#126030=CARTESIAN_POINT('Origin',(45.5058627832302,1076.73142393294,445.768247825525));
#126031=CARTESIAN_POINT('Origin',(45.5058627832302,1067.7251047501,445.768247825525));
#126032=CARTESIAN_POINT('',(45.5058627832302,1076.73142393294,444.7477657829));
#126033=CARTESIAN_POINT('Origin',(45.5058627832302,1076.73142393294,445.768247825525));
#126034=CARTESIAN_POINT('',(45.5058627832302,1082.7251047501,444.7477657829));
#126035=CARTESIAN_POINT('',(45.5058627832302,1067.7251047501,444.7477657829));
#126036=CARTESIAN_POINT('Origin',(45.5058627832302,1082.7251047501,445.768247825525));
#126037=CARTESIAN_POINT('Origin',(49.9258518558208,1067.7251047501,454.931887780957));
#126038=CARTESIAN_POINT('',(49.9258518558208,1078.73142393294,453.230887557874));
#126039=CARTESIAN_POINT('Origin',(49.9258518558208,1078.73142393294,454.931887780957));
#126040=CARTESIAN_POINT('',(49.9258518558208,1076.73142393294,453.230887557874));
#126041=CARTESIAN_POINT('',(49.9258518558208,1067.7251047501,453.230887557874));
#126042=CARTESIAN_POINT('Origin',(49.9258518558208,1076.73142393294,454.931887780957));
#126043=CARTESIAN_POINT('Origin',(49.9258518558208,1067.7251047501,454.931887780957));
#126044=CARTESIAN_POINT('',(49.9258518558208,1076.73142393294,453.830887557874));
#126045=CARTESIAN_POINT('Origin',(49.9258518558208,1076.73142393294,454.931887780957));
#126046=CARTESIAN_POINT('',(49.9258518558208,1082.7251047501,453.830887557874));
#126047=CARTESIAN_POINT('',(49.9258518558208,1067.7251047501,453.830887557874));
#126048=CARTESIAN_POINT('Origin',(49.9258518558208,1082.7251047501,454.931887780957));
#126049=CARTESIAN_POINT('Origin',(52.0746519374465,1067.7251047501,464.561071088605));
#126050=CARTESIAN_POINT('',(52.0746519374465,1078.73142393294,462.839796456561));
#126051=CARTESIAN_POINT('Origin',(52.0746519374465,1078.73142393294,464.561071088605));
#126052=CARTESIAN_POINT('',(52.0746519374465,1076.73142393294,462.839796456561));
#126053=CARTESIAN_POINT('',(52.0746519374465,1067.7251047501,462.839796456561));
#126054=CARTESIAN_POINT('Origin',(52.0746519374465,1076.73142393294,464.561071088605));
#126055=CARTESIAN_POINT('Origin',(52.0746519374465,1067.7251047501,464.561071088605));
#126056=CARTESIAN_POINT('',(52.0746519374465,1076.73142393294,463.439796456561));
#126057=CARTESIAN_POINT('Origin',(52.0746519374465,1076.73142393294,464.561071088605));
#126058=CARTESIAN_POINT('',(52.0746519374465,1082.7251047501,463.439796456561));
#126059=CARTESIAN_POINT('',(52.0746519374465,1067.7251047501,463.439796456561));
#126060=CARTESIAN_POINT('Origin',(52.0746519374465,1082.7251047501,464.561071088605));
#126061=CARTESIAN_POINT('Origin',(53.2770757808756,1067.7251047501,475.887982254234));
#126062=CARTESIAN_POINT('',(53.2770757808756,1078.73142393294,474.105989599829));
#126063=CARTESIAN_POINT('Origin',(53.2770757808756,1078.73142393294,475.887982254234));
#126064=CARTESIAN_POINT('',(53.2770757808756,1076.73142393294,474.105989599829));
#126065=CARTESIAN_POINT('',(53.2770757808756,1067.7251047501,474.105989599829));
#126066=CARTESIAN_POINT('Origin',(53.2770757808756,1076.73142393294,475.887982254234));
#126067=CARTESIAN_POINT('Origin',(53.2770757808756,1067.7251047501,475.887982254234));
#126068=CARTESIAN_POINT('',(53.2770757808756,1076.73142393294,474.705989599829));
#126069=CARTESIAN_POINT('Origin',(53.2770757808756,1076.73142393294,475.887982254234));
#126070=CARTESIAN_POINT('',(53.2770757808756,1082.7251047501,474.705989599829));
#126071=CARTESIAN_POINT('',(53.2770757808756,1067.7251047501,474.705989599829));
#126072=CARTESIAN_POINT('Origin',(53.2770757808756,1082.7251047501,475.887982254234));
#126073=CARTESIAN_POINT('Origin',(52.0862183235875,1067.7251047501,487.046546328579));
#126074=CARTESIAN_POINT('',(52.0862183235875,1078.73142393294,485.385665518658));
#126075=CARTESIAN_POINT('Origin',(52.0862183235875,1078.73142393294,487.046546328579));
#126076=CARTESIAN_POINT('',(52.0862183235875,1076.73142393294,485.385665518658));
#126077=CARTESIAN_POINT('',(52.0862183235875,1067.7251047501,485.385665518658));
#126078=CARTESIAN_POINT('Origin',(52.0862183235875,1076.73142393294,487.046546328579));
#126079=CARTESIAN_POINT('Origin',(52.0862183235875,1067.7251047501,487.046546328579));
#126080=CARTESIAN_POINT('',(52.0862183235875,1076.73142393294,485.985665518658));
#126081=CARTESIAN_POINT('Origin',(52.0862183235875,1076.73142393294,487.046546328579));
#126082=CARTESIAN_POINT('',(52.0862183235875,1082.7251047501,485.985665518658));
#126083=CARTESIAN_POINT('',(52.0862183235875,1067.7251047501,485.985665518658));
#126084=CARTESIAN_POINT('Origin',(52.0862183235875,1082.7251047501,487.046546328579));
#126085=CARTESIAN_POINT('Origin',(18.7819059952831,1067.7251047501,420.74995476784));
#126086=CARTESIAN_POINT('',(18.7819059952831,1078.73142393294,419.649596702165));
#126087=CARTESIAN_POINT('Origin',(18.7819059952831,1078.73142393294,420.74995476784));
#126088=CARTESIAN_POINT('',(18.7819059952831,1076.73142393294,419.649596702165));
#126089=CARTESIAN_POINT('',(18.7819059952831,1067.7251047501,419.649596702165));
#126090=CARTESIAN_POINT('Origin',(18.7819059952831,1076.73142393294,420.74995476784));
#126091=CARTESIAN_POINT('Origin',(18.7819059952831,1067.7251047501,420.74995476784));
#126092=CARTESIAN_POINT('',(18.7819059952831,1076.73142393294,420.249596702165));
#126093=CARTESIAN_POINT('Origin',(18.7819059952831,1076.73142393294,420.74995476784));
#126094=CARTESIAN_POINT('',(18.7819059952831,1082.7251047501,420.249596702165));
#126095=CARTESIAN_POINT('',(18.7819059952831,1067.7251047501,420.249596702165));
#126096=CARTESIAN_POINT('Origin',(18.7819059952831,1082.7251047501,420.74995476784));
#126097=CARTESIAN_POINT('Origin',(27.2710543542544,1067.7251047501,421.877665036574));
#126098=CARTESIAN_POINT('',(27.2710543542544,1078.73142393294,420.663633469837));
#126099=CARTESIAN_POINT('Origin',(27.2710543542544,1078.73142393294,421.877665036574));
#126100=CARTESIAN_POINT('',(27.2710543542544,1076.73142393294,420.663633469837));
#126101=CARTESIAN_POINT('',(27.2710543542544,1067.7251047501,420.663633469837));
#126102=CARTESIAN_POINT('Origin',(27.2710543542544,1076.73142393294,421.877665036574));
#126103=CARTESIAN_POINT('Origin',(27.2710543542544,1067.7251047501,421.877665036574));
#126104=CARTESIAN_POINT('',(27.2710543542544,1076.73142393294,421.263633469837));
#126105=CARTESIAN_POINT('Origin',(27.2710543542544,1076.73142393294,421.877665036574));
#126106=CARTESIAN_POINT('',(27.2710543542544,1082.7251047501,421.263633469837));
#126107=CARTESIAN_POINT('',(27.2710543542544,1067.7251047501,421.263633469837));
#126108=CARTESIAN_POINT('Origin',(27.2710543542544,1082.7251047501,421.877665036574));
#126109=CARTESIAN_POINT('Origin',(34.6453511739137,1067.7251047501,424.782598105687));
#126110=CARTESIAN_POINT('',(34.6453511739137,1078.73142393294,423.453790142114));
#126111=CARTESIAN_POINT('Origin',(34.6453511739137,1078.73142393294,424.782598105687));
#126112=CARTESIAN_POINT('',(34.6453511739137,1076.73142393294,423.453790142114));
#126113=CARTESIAN_POINT('',(34.6453511739137,1067.7251047501,423.453790142114));
#126114=CARTESIAN_POINT('Origin',(34.6453511739137,1076.73142393294,424.782598105687));
#126115=CARTESIAN_POINT('Origin',(34.6453511739137,1067.7251047501,424.782598105687));
#126116=CARTESIAN_POINT('',(34.6453511739137,1076.73142393294,424.053790142114));
#126117=CARTESIAN_POINT('Origin',(34.6453511739137,1076.73142393294,424.782598105687));
#126118=CARTESIAN_POINT('',(34.6453511739137,1082.7251047501,424.053790142114));
#126119=CARTESIAN_POINT('',(34.6453511739137,1067.7251047501,424.053790142114));
#126120=CARTESIAN_POINT('Origin',(34.6453511739137,1082.7251047501,424.782598105687));
#126121=CARTESIAN_POINT('Origin',(42.6068786662477,1067.7251047501,429.530915358505));
#126122=CARTESIAN_POINT('',(42.6068786662477,1078.73142393294,428.069798356688));
#126123=CARTESIAN_POINT('Origin',(42.6068786662477,1078.73142393294,429.530915358505));
#126124=CARTESIAN_POINT('',(42.6068786662477,1076.73142393294,428.069798356688));
#126125=CARTESIAN_POINT('',(42.6068786662477,1067.7251047501,428.069798356688));
#126126=CARTESIAN_POINT('Origin',(42.6068786662477,1076.73142393294,429.530915358505));
#126127=CARTESIAN_POINT('Origin',(42.6068786662477,1067.7251047501,429.530915358505));
#126128=CARTESIAN_POINT('',(42.6068786662477,1076.73142393294,428.669798356688));
#126129=CARTESIAN_POINT('Origin',(42.6068786662477,1076.73142393294,429.530915358505));
#126130=CARTESIAN_POINT('',(42.6068786662477,1082.7251047501,428.669798356688));
#126131=CARTESIAN_POINT('',(42.6068786662477,1067.7251047501,428.669798356688));
#126132=CARTESIAN_POINT('Origin',(42.6068786662477,1082.7251047501,429.530915358505));
#126133=CARTESIAN_POINT('Origin',(48.9083680287886,1067.7251047501,435.84491229783));
#126134=CARTESIAN_POINT('',(48.9083680287886,1078.73142393294,434.224430255206));
#126135=CARTESIAN_POINT('Origin',(48.9083680287886,1078.73142393294,435.84491229783));
#126136=CARTESIAN_POINT('',(48.9083680287886,1076.73142393294,434.224430255206));
#126137=CARTESIAN_POINT('',(48.9083680287886,1067.7251047501,434.224430255206));
#126138=CARTESIAN_POINT('Origin',(48.9083680287886,1076.73142393294,435.84491229783));
#126139=CARTESIAN_POINT('Origin',(48.9083680287886,1067.7251047501,435.84491229783));
#126140=CARTESIAN_POINT('',(48.9083680287886,1076.73142393294,434.824430255206));
#126141=CARTESIAN_POINT('Origin',(48.9083680287886,1076.73142393294,435.84491229783));
#126142=CARTESIAN_POINT('',(48.9083680287886,1082.7251047501,434.824430255206));
#126143=CARTESIAN_POINT('',(48.9083680287886,1067.7251047501,434.824430255206));
#126144=CARTESIAN_POINT('Origin',(48.9083680287886,1082.7251047501,435.84491229783));
#126145=CARTESIAN_POINT('Origin',(55.1369976125917,1067.7251047501,443.889337332746));
#126146=CARTESIAN_POINT('',(55.1369976125917,1078.73142393294,442.188337109664));
#126147=CARTESIAN_POINT('Origin',(55.1369976125917,1078.73142393294,443.889337332746));
#126148=CARTESIAN_POINT('',(55.1369976125917,1076.73142393294,442.188337109664));
#126149=CARTESIAN_POINT('',(55.1369976125917,1067.7251047501,442.188337109664));
#126150=CARTESIAN_POINT('Origin',(55.1369976125917,1076.73142393294,443.889337332746));
#126151=CARTESIAN_POINT('Origin',(55.1369976125917,1067.7251047501,443.889337332746));
#126152=CARTESIAN_POINT('',(55.1369976125917,1076.73142393294,442.788337109663));
#126153=CARTESIAN_POINT('Origin',(55.1369976125917,1076.73142393294,443.889337332746));
#126154=CARTESIAN_POINT('',(55.1369976125917,1082.7251047501,442.788337109663));
#126155=CARTESIAN_POINT('',(55.1369976125917,1067.7251047501,442.788337109663));
#126156=CARTESIAN_POINT('Origin',(55.1369976125917,1082.7251047501,443.889337332746));
#126157=CARTESIAN_POINT('Origin',(59.2408610395779,1067.7251047501,452.861339223948));
#126158=CARTESIAN_POINT('',(59.2408610395779,1078.73142393294,451.140064591905));
#126159=CARTESIAN_POINT('Origin',(59.2408610395779,1078.73142393294,452.861339223948));
#126160=CARTESIAN_POINT('',(59.2408610395779,1076.73142393294,451.140064591905));
#126161=CARTESIAN_POINT('',(59.2408610395779,1067.7251047501,451.140064591905));
#126162=CARTESIAN_POINT('Origin',(59.2408610395779,1076.73142393294,452.861339223948));
#126163=CARTESIAN_POINT('Origin',(59.2408610395779,1067.7251047501,452.861339223948));
#126164=CARTESIAN_POINT('',(59.2408610395779,1076.73142393294,451.740064591905));
#126165=CARTESIAN_POINT('Origin',(59.2408610395779,1076.73142393294,452.861339223948));
#126166=CARTESIAN_POINT('',(59.2408610395779,1082.7251047501,451.740064591905));
#126167=CARTESIAN_POINT('',(59.2408610395779,1067.7251047501,451.740064591905));
#126168=CARTESIAN_POINT('Origin',(59.2408610395779,1082.7251047501,452.861339223948));
#126169=CARTESIAN_POINT('Origin',(62.7720062892815,1067.7251047501,463.690732229966));
#126170=CARTESIAN_POINT('',(62.7720062892815,1078.73142393294,461.908739575561));
#126171=CARTESIAN_POINT('Origin',(62.7720062892815,1078.73142393294,463.690732229966));
#126172=CARTESIAN_POINT('',(62.7720062892815,1076.73142393294,461.908739575561));
#126173=CARTESIAN_POINT('',(62.7720062892815,1067.7251047501,461.908739575561));
#126174=CARTESIAN_POINT('Origin',(62.7720062892815,1076.73142393294,463.690732229966));
#126175=CARTESIAN_POINT('Origin',(62.7720062892815,1067.7251047501,463.690732229966));
#126176=CARTESIAN_POINT('',(62.7720062892815,1076.73142393294,462.508739575561));
#126177=CARTESIAN_POINT('Origin',(62.7720062892815,1076.73142393294,463.690732229966));
#126178=CARTESIAN_POINT('',(62.7720062892815,1082.7251047501,462.508739575561));
#126179=CARTESIAN_POINT('',(62.7720062892815,1067.7251047501,462.508739575561));
#126180=CARTESIAN_POINT('Origin',(62.7720062892815,1082.7251047501,463.690732229966));
#126181=CARTESIAN_POINT('Origin',(63.9271678484146,1067.7251047501,474.853048094389));
#126182=CARTESIAN_POINT('',(63.9271678484146,1078.73142393294,473.192167284468));
#126183=CARTESIAN_POINT('Origin',(63.9271678484146,1078.73142393294,474.853048094389));
#126184=CARTESIAN_POINT('',(63.9271678484146,1076.73142393294,473.192167284468));
#126185=CARTESIAN_POINT('',(63.9271678484146,1067.7251047501,473.192167284468));
#126186=CARTESIAN_POINT('Origin',(63.9271678484146,1076.73142393294,474.853048094389));
#126187=CARTESIAN_POINT('Origin',(63.9271678484146,1067.7251047501,474.853048094389));
#126188=CARTESIAN_POINT('',(63.9271678484146,1076.73142393294,473.792167284468));
#126189=CARTESIAN_POINT('Origin',(63.9271678484146,1076.73142393294,474.853048094389));
#126190=CARTESIAN_POINT('',(63.9271678484146,1082.7251047501,473.792167284468));
#126191=CARTESIAN_POINT('',(63.9271678484146,1067.7251047501,473.792167284468));
#126192=CARTESIAN_POINT('Origin',(63.9271678484146,1082.7251047501,474.853048094389));
#126193=CARTESIAN_POINT('Origin',(17.5667982035468,1067.7251047501,416.929552010124));
#126194=CARTESIAN_POINT('',(17.5667982035468,1078.73142393294,415.829193944449));
#126195=CARTESIAN_POINT('Origin',(17.5667982035468,1078.73142393294,416.929552010124));
#126196=CARTESIAN_POINT('',(17.5667982035468,1076.73142393294,415.829193944449));
#126197=CARTESIAN_POINT('',(17.5667982035468,1067.7251047501,415.829193944449));
#126198=CARTESIAN_POINT('Origin',(17.5667982035468,1076.73142393294,416.929552010124));
#126199=CARTESIAN_POINT('Origin',(17.5667982035468,1067.7251047501,416.929552010124));
#126200=CARTESIAN_POINT('',(17.5667982035468,1076.73142393294,416.429193944449));
#126201=CARTESIAN_POINT('Origin',(17.5667982035468,1076.73142393294,416.929552010124));
#126202=CARTESIAN_POINT('',(17.5667982035468,1082.7251047501,416.429193944449));
#126203=CARTESIAN_POINT('',(17.5667982035468,1067.7251047501,416.429193944449));
#126204=CARTESIAN_POINT('Origin',(17.5667982035468,1082.7251047501,416.929552010124));
#126205=CARTESIAN_POINT('Origin',(26.104902451873,1067.7251047501,416.267625914893));
#126206=CARTESIAN_POINT('',(26.104902451873,1078.73142393294,415.053594348156));
#126207=CARTESIAN_POINT('Origin',(26.104902451873,1078.73142393294,416.267625914893));
#126208=CARTESIAN_POINT('',(26.104902451873,1076.73142393294,415.053594348156));
#126209=CARTESIAN_POINT('',(26.104902451873,1067.7251047501,415.053594348156));
#126210=CARTESIAN_POINT('Origin',(26.104902451873,1076.73142393294,416.267625914893));
#126211=CARTESIAN_POINT('Origin',(26.104902451873,1067.7251047501,416.267625914893));
#126212=CARTESIAN_POINT('',(26.104902451873,1076.73142393294,415.653594348156));
#126213=CARTESIAN_POINT('Origin',(26.104902451873,1076.73142393294,416.267625914893));
#126214=CARTESIAN_POINT('',(26.104902451873,1082.7251047501,415.653594348156));
#126215=CARTESIAN_POINT('',(26.104902451873,1067.7251047501,415.653594348156));
#126216=CARTESIAN_POINT('Origin',(26.104902451873,1082.7251047501,416.267625914893));
#126217=CARTESIAN_POINT('Origin',(33.9220227392334,1067.7251047501,417.57587670637));
#126218=CARTESIAN_POINT('',(33.9220227392334,1078.73142393294,416.247068742797));
#126219=CARTESIAN_POINT('Origin',(33.9220227392334,1078.73142393294,417.57587670637));
#126220=CARTESIAN_POINT('',(33.9220227392334,1076.73142393294,416.247068742797));
#126221=CARTESIAN_POINT('',(33.9220227392334,1067.7251047501,416.247068742797));
#126222=CARTESIAN_POINT('Origin',(33.9220227392334,1076.73142393294,417.57587670637));
#126223=CARTESIAN_POINT('Origin',(33.9220227392334,1067.7251047501,417.57587670637));
#126224=CARTESIAN_POINT('',(33.9220227392334,1076.73142393294,416.847068742797));
#126225=CARTESIAN_POINT('Origin',(33.9220227392334,1076.73142393294,417.57587670637));
#126226=CARTESIAN_POINT('',(33.9220227392334,1082.7251047501,416.847068742797));
#126227=CARTESIAN_POINT('',(33.9220227392334,1067.7251047501,416.847068742797));
#126228=CARTESIAN_POINT('Origin',(33.9220227392334,1082.7251047501,417.57587670637));
#126229=CARTESIAN_POINT('Origin',(42.6968024226085,1067.7251047501,420.565137192314));
#126230=CARTESIAN_POINT('',(42.6968024226085,1078.73142393294,419.104020190497));
#126231=CARTESIAN_POINT('Origin',(42.6968024226085,1078.73142393294,420.565137192314));
#126232=CARTESIAN_POINT('',(42.6968024226085,1076.73142393294,419.104020190497));
#126233=CARTESIAN_POINT('',(42.6968024226085,1067.7251047501,419.104020190497));
#126234=CARTESIAN_POINT('Origin',(42.6968024226085,1076.73142393294,420.565137192314));
#126235=CARTESIAN_POINT('Origin',(42.6968024226085,1067.7251047501,420.565137192314));
#126236=CARTESIAN_POINT('',(42.6968024226085,1076.73142393294,419.704020190497));
#126237=CARTESIAN_POINT('Origin',(42.6968024226085,1076.73142393294,420.565137192314));
#126238=CARTESIAN_POINT('',(42.6968024226085,1082.7251047501,419.704020190497));
#126239=CARTESIAN_POINT('',(42.6968024226085,1067.7251047501,419.704020190497));
#126240=CARTESIAN_POINT('Origin',(42.6968024226085,1082.7251047501,420.565137192314));
#126241=CARTESIAN_POINT('Origin',(50.1733429031008,1067.7251047501,425.431004841519));
#126242=CARTESIAN_POINT('',(50.1733429031008,1078.73142393294,423.810522798895));
#126243=CARTESIAN_POINT('Origin',(50.1733429031008,1078.73142393294,425.431004841519));
#126244=CARTESIAN_POINT('',(50.1733429031008,1076.73142393294,423.810522798895));
#126245=CARTESIAN_POINT('',(50.1733429031008,1067.7251047501,423.810522798895));
#126246=CARTESIAN_POINT('Origin',(50.1733429031008,1076.73142393294,425.431004841519));
#126247=CARTESIAN_POINT('Origin',(50.1733429031008,1067.7251047501,425.431004841519));
#126248=CARTESIAN_POINT('',(50.1733429031008,1076.73142393294,424.410522798895));
#126249=CARTESIAN_POINT('Origin',(50.1733429031008,1076.73142393294,425.431004841519));
#126250=CARTESIAN_POINT('',(50.1733429031008,1082.7251047501,424.410522798895));
#126251=CARTESIAN_POINT('',(50.1733429031008,1067.7251047501,424.410522798895));
#126252=CARTESIAN_POINT('Origin',(50.1733429031008,1082.7251047501,425.431004841519));
#126253=CARTESIAN_POINT('Origin',(57.9383919970236,1067.7251047501,432.00463498046));
#126254=CARTESIAN_POINT('',(57.9383919970236,1078.73142393294,430.303634757377));
#126255=CARTESIAN_POINT('Origin',(57.9383919970236,1078.73142393294,432.00463498046));
#126256=CARTESIAN_POINT('',(57.9383919970236,1076.73142393294,430.303634757377));
#126257=CARTESIAN_POINT('',(57.9383919970236,1067.7251047501,430.303634757377));
#126258=CARTESIAN_POINT('Origin',(57.9383919970236,1076.73142393294,432.00463498046));
#126259=CARTESIAN_POINT('Origin',(57.9383919970236,1067.7251047501,432.00463498046));
#126260=CARTESIAN_POINT('',(57.9383919970236,1076.73142393294,430.903634757377));
#126261=CARTESIAN_POINT('Origin',(57.9383919970236,1076.73142393294,432.00463498046));
#126262=CARTESIAN_POINT('',(57.9383919970236,1082.7251047501,430.903634757377));
#126263=CARTESIAN_POINT('',(57.9383919970236,1067.7251047501,430.903634757377));
#126264=CARTESIAN_POINT('Origin',(57.9383919970236,1082.7251047501,432.00463498046));
#126265=CARTESIAN_POINT('Origin',(63.8179602450892,1067.7251047501,439.927335920128));
#126266=CARTESIAN_POINT('',(63.8179602450892,1078.73142393294,438.206061288084));
#126267=CARTESIAN_POINT('Origin',(63.8179602450892,1078.73142393294,439.927335920128));
#126268=CARTESIAN_POINT('',(63.8179602450892,1076.73142393294,438.206061288084));
#126269=CARTESIAN_POINT('',(63.8179602450892,1067.7251047501,438.206061288084));
#126270=CARTESIAN_POINT('Origin',(63.8179602450892,1076.73142393294,439.927335920128));
#126271=CARTESIAN_POINT('Origin',(63.8179602450892,1067.7251047501,439.927335920128));
#126272=CARTESIAN_POINT('',(63.8179602450892,1076.73142393294,438.806061288084));
#126273=CARTESIAN_POINT('Origin',(63.8179602450892,1076.73142393294,439.927335920128));
#126274=CARTESIAN_POINT('',(63.8179602450892,1082.7251047501,438.806061288084));
#126275=CARTESIAN_POINT('',(63.8179602450892,1067.7251047501,438.806061288084));
#126276=CARTESIAN_POINT('Origin',(63.8179602450892,1082.7251047501,439.927335920128));
#126277=CARTESIAN_POINT('Origin',(69.5234989093405,1067.7251047501,449.785914326979));
#126278=CARTESIAN_POINT('',(69.5234989093405,1078.73142393294,448.003921672574));
#126279=CARTESIAN_POINT('Origin',(69.5234989093405,1078.73142393294,449.785914326979));
#126280=CARTESIAN_POINT('',(69.5234989093405,1076.73142393294,448.003921672574));
#126281=CARTESIAN_POINT('',(69.5234989093405,1067.7251047501,448.003921672574));
#126282=CARTESIAN_POINT('Origin',(69.5234989093405,1076.73142393294,449.785914326979));
#126283=CARTESIAN_POINT('Origin',(69.5234989093405,1067.7251047501,449.785914326979));
#126284=CARTESIAN_POINT('',(69.5234989093405,1076.73142393294,448.603921672574));
#126285=CARTESIAN_POINT('Origin',(69.5234989093405,1076.73142393294,449.785914326979));
#126286=CARTESIAN_POINT('',(69.5234989093405,1082.7251047501,448.603921672574));
#126287=CARTESIAN_POINT('',(69.5234989093405,1067.7251047501,448.603921672574));
#126288=CARTESIAN_POINT('Origin',(69.5234989093405,1082.7251047501,449.785914326979));
#126289=CARTESIAN_POINT('Origin',(72.9741933816806,1067.7251047501,460.46413521547));
#126290=CARTESIAN_POINT('',(72.9741933816806,1078.73142393294,458.803254405549));
#126291=CARTESIAN_POINT('Origin',(72.9741933816806,1078.73142393294,460.46413521547));
#126292=CARTESIAN_POINT('',(72.9741933816806,1076.73142393294,458.803254405549));
#126293=CARTESIAN_POINT('',(72.9741933816806,1067.7251047501,458.803254405549));
#126294=CARTESIAN_POINT('Origin',(72.9741933816806,1076.73142393294,460.46413521547));
#126295=CARTESIAN_POINT('Origin',(72.9741933816806,1067.7251047501,460.46413521547));
#126296=CARTESIAN_POINT('',(72.9741933816806,1076.73142393294,459.403254405549));
#126297=CARTESIAN_POINT('Origin',(72.9741933816806,1076.73142393294,460.46413521547));
#126298=CARTESIAN_POINT('',(72.9741933816806,1082.7251047501,459.403254405549));
#126299=CARTESIAN_POINT('',(72.9741933816806,1067.7251047501,459.403254405549));
#126300=CARTESIAN_POINT('Origin',(72.9741933816806,1082.7251047501,460.46413521547));
#126301=CARTESIAN_POINT('Origin',(15.5839370354653,1067.7251047501,413.445269334333));
#126302=CARTESIAN_POINT('',(15.5839370354653,1078.73142393294,412.344911268658));
#126303=CARTESIAN_POINT('Origin',(15.5839370354653,1078.73142393294,413.445269334333));
#126304=CARTESIAN_POINT('',(15.5839370354653,1076.73142393294,412.344911268658));
#126305=CARTESIAN_POINT('',(15.5839370354653,1067.7251047501,412.344911268658));
#126306=CARTESIAN_POINT('Origin',(15.5839370354653,1076.73142393294,413.445269334333));
#126307=CARTESIAN_POINT('Origin',(15.5839370354653,1067.7251047501,413.445269334333));
#126308=CARTESIAN_POINT('',(15.5839370354653,1076.73142393294,412.944911268658));
#126309=CARTESIAN_POINT('Origin',(15.5839370354653,1076.73142393294,413.445269334333));
#126310=CARTESIAN_POINT('',(15.5839370354653,1082.7251047501,412.944911268658));
#126311=CARTESIAN_POINT('',(15.5839370354653,1067.7251047501,412.944911268658));
#126312=CARTESIAN_POINT('Origin',(15.5839370354653,1082.7251047501,413.445269334333));
#126313=CARTESIAN_POINT('Origin',(23.7978410471248,1067.7251047501,411.022636221772));
#126314=CARTESIAN_POINT('',(23.7978410471248,1078.73142393294,409.808604655035));
#126315=CARTESIAN_POINT('Origin',(23.7978410471248,1078.73142393294,411.022636221772));
#126316=CARTESIAN_POINT('',(23.7978410471248,1076.73142393294,409.808604655035));
#126317=CARTESIAN_POINT('',(23.7978410471248,1067.7251047501,409.808604655035));
#126318=CARTESIAN_POINT('Origin',(23.7978410471248,1076.73142393294,411.022636221772));
#126319=CARTESIAN_POINT('Origin',(23.7978410471248,1067.7251047501,411.022636221772));
#126320=CARTESIAN_POINT('',(23.7978410471248,1076.73142393294,410.408604655034));
#126321=CARTESIAN_POINT('Origin',(23.7978410471248,1076.73142393294,411.022636221772));
#126322=CARTESIAN_POINT('',(23.7978410471248,1082.7251047501,410.408604655034));
#126323=CARTESIAN_POINT('',(23.7978410471248,1067.7251047501,410.408604655034));
#126324=CARTESIAN_POINT('Origin',(23.7978410471248,1082.7251047501,411.022636221772));
#126325=CARTESIAN_POINT('Origin',(31.7161391349238,1067.7251047501,410.677027898342));
#126326=CARTESIAN_POINT('',(31.7161391349238,1078.73142393294,409.348219934769));
#126327=CARTESIAN_POINT('Origin',(31.7161391349238,1078.73142393294,410.677027898342));
#126328=CARTESIAN_POINT('',(31.7161391349238,1076.73142393294,409.348219934769));
#126329=CARTESIAN_POINT('',(31.7161391349238,1067.7251047501,409.348219934769));
#126330=CARTESIAN_POINT('Origin',(31.7161391349238,1076.73142393294,410.677027898342));
#126331=CARTESIAN_POINT('Origin',(31.7161391349238,1067.7251047501,410.677027898342));
#126332=CARTESIAN_POINT('',(31.7161391349238,1076.73142393294,409.948219934769));
#126333=CARTESIAN_POINT('Origin',(31.7161391349238,1076.73142393294,410.677027898342));
#126334=CARTESIAN_POINT('',(31.7161391349238,1082.7251047501,409.948219934769));
#126335=CARTESIAN_POINT('',(31.7161391349238,1067.7251047501,409.948219934769));
#126336=CARTESIAN_POINT('Origin',(31.7161391349238,1082.7251047501,410.677027898342));
#126337=CARTESIAN_POINT('Origin',(40.920671031112,1067.7251047501,411.776586590112));
#126338=CARTESIAN_POINT('',(40.920671031112,1078.73142393294,410.315469588295));
#126339=CARTESIAN_POINT('Origin',(40.920671031112,1078.73142393294,411.776586590112));
#126340=CARTESIAN_POINT('',(40.920671031112,1076.73142393294,410.315469588295));
#126341=CARTESIAN_POINT('',(40.920671031112,1067.7251047501,410.315469588295));
#126342=CARTESIAN_POINT('Origin',(40.920671031112,1076.73142393294,411.776586590112));
#126343=CARTESIAN_POINT('Origin',(40.920671031112,1067.7251047501,411.776586590112));
#126344=CARTESIAN_POINT('',(40.920671031112,1076.73142393294,410.915469588295));
#126345=CARTESIAN_POINT('Origin',(40.920671031112,1076.73142393294,411.776586590112));
#126346=CARTESIAN_POINT('',(40.920671031112,1082.7251047501,410.915469588295));
#126347=CARTESIAN_POINT('',(40.920671031112,1067.7251047501,410.915469588295));
#126348=CARTESIAN_POINT('Origin',(40.920671031112,1082.7251047501,411.776586590112));
#126349=CARTESIAN_POINT('Origin',(49.2455019341365,1067.7251047501,414.981663183905));
#126350=CARTESIAN_POINT('',(49.2455019341365,1078.73142393294,413.36118114128));
#126351=CARTESIAN_POINT('Origin',(49.2455019341365,1078.73142393294,414.981663183905));
#126352=CARTESIAN_POINT('',(49.2455019341365,1076.73142393294,413.36118114128));
#126353=CARTESIAN_POINT('',(49.2455019341365,1067.7251047501,413.36118114128));
#126354=CARTESIAN_POINT('Origin',(49.2455019341365,1076.73142393294,414.981663183905));
#126355=CARTESIAN_POINT('Origin',(49.2455019341365,1067.7251047501,414.981663183905));
#126356=CARTESIAN_POINT('',(49.2455019341365,1076.73142393294,413.96118114128));
#126357=CARTESIAN_POINT('Origin',(49.2455019341365,1076.73142393294,414.981663183905));
#126358=CARTESIAN_POINT('',(49.2455019341365,1082.7251047501,413.96118114128));
#126359=CARTESIAN_POINT('',(49.2455019341365,1067.7251047501,413.96118114128));
#126360=CARTESIAN_POINT('Origin',(49.2455019341365,1082.7251047501,414.981663183905));
#126361=CARTESIAN_POINT('Origin',(58.207600631935,1067.7251047501,419.79719924602));
#126362=CARTESIAN_POINT('',(58.207600631935,1078.73142393294,418.096199022937));
#126363=CARTESIAN_POINT('Origin',(58.207600631935,1078.73142393294,419.79719924602));
#126364=CARTESIAN_POINT('',(58.207600631935,1076.73142393294,418.096199022937));
#126365=CARTESIAN_POINT('',(58.207600631935,1067.7251047501,418.096199022937));
#126366=CARTESIAN_POINT('Origin',(58.207600631935,1076.73142393294,419.79719924602));
#126367=CARTESIAN_POINT('Origin',(58.207600631935,1067.7251047501,419.79719924602));
#126368=CARTESIAN_POINT('',(58.207600631935,1076.73142393294,418.696199022937));
#126369=CARTESIAN_POINT('Origin',(58.207600631935,1076.73142393294,419.79719924602));
#126370=CARTESIAN_POINT('',(58.207600631935,1082.7251047501,418.696199022937));
#126371=CARTESIAN_POINT('',(58.207600631935,1067.7251047501,418.696199022937));
#126372=CARTESIAN_POINT('Origin',(58.207600631935,1082.7251047501,419.79719924602));
#126373=CARTESIAN_POINT('Origin',(65.6059083553409,1067.7251047501,426.324339185754));
#126374=CARTESIAN_POINT('',(65.6059083553409,1078.73142393294,424.603064553711));
#126375=CARTESIAN_POINT('Origin',(65.6059083553409,1078.73142393294,426.324339185754));
#126376=CARTESIAN_POINT('',(65.6059083553409,1076.73142393294,424.603064553711));
#126377=CARTESIAN_POINT('',(65.6059083553409,1067.7251047501,424.603064553711));
#126378=CARTESIAN_POINT('Origin',(65.6059083553409,1076.73142393294,426.324339185754));
#126379=CARTESIAN_POINT('Origin',(65.6059083553409,1067.7251047501,426.324339185754));
#126380=CARTESIAN_POINT('',(65.6059083553409,1076.73142393294,425.203064553711));
#126381=CARTESIAN_POINT('Origin',(65.6059083553409,1076.73142393294,426.324339185754));
#126382=CARTESIAN_POINT('',(65.6059083553409,1082.7251047501,425.203064553711));
#126383=CARTESIAN_POINT('',(65.6059083553409,1067.7251047501,425.203064553711));
#126384=CARTESIAN_POINT('Origin',(65.6059083553409,1082.7251047501,426.324339185754));
#126385=CARTESIAN_POINT('Origin',(73.2364810163002,1067.7251047501,434.781235810351));
#126386=CARTESIAN_POINT('',(73.2364810163002,1078.73142393294,432.999243155946));
#126387=CARTESIAN_POINT('Origin',(73.2364810163002,1078.73142393294,434.781235810351));
#126388=CARTESIAN_POINT('',(73.2364810163002,1076.73142393294,432.999243155946));
#126389=CARTESIAN_POINT('',(73.2364810163002,1067.7251047501,432.999243155946));
#126390=CARTESIAN_POINT('Origin',(73.2364810163002,1076.73142393294,434.781235810351));
#126391=CARTESIAN_POINT('Origin',(73.2364810163002,1067.7251047501,434.781235810351));
#126392=CARTESIAN_POINT('',(73.2364810163002,1076.73142393294,433.599243155946));
#126393=CARTESIAN_POINT('Origin',(73.2364810163002,1076.73142393294,434.781235810351));
#126394=CARTESIAN_POINT('',(73.2364810163002,1082.7251047501,433.599243155946));
#126395=CARTESIAN_POINT('',(73.2364810163002,1067.7251047501,433.599243155946));
#126396=CARTESIAN_POINT('Origin',(73.2364810163002,1082.7251047501,434.781235810351));
#126397=CARTESIAN_POINT('Origin',(78.8318964951367,1067.7251047501,444.508672230294));
#126398=CARTESIAN_POINT('',(78.8318964951367,1078.73142393294,442.847791420374));
#126399=CARTESIAN_POINT('Origin',(78.8318964951367,1078.73142393294,444.508672230294));
#126400=CARTESIAN_POINT('',(78.8318964951367,1076.73142393294,442.847791420374));
#126401=CARTESIAN_POINT('',(78.8318964951367,1067.7251047501,442.847791420374));
#126402=CARTESIAN_POINT('Origin',(78.8318964951367,1076.73142393294,444.508672230294));
#126403=CARTESIAN_POINT('Origin',(78.8318964951367,1067.7251047501,444.508672230294));
#126404=CARTESIAN_POINT('',(78.8318964951367,1076.73142393294,443.447791420374));
#126405=CARTESIAN_POINT('Origin',(78.8318964951367,1076.73142393294,444.508672230294));
#126406=CARTESIAN_POINT('',(78.8318964951367,1082.7251047501,443.447791420374));
#126407=CARTESIAN_POINT('',(78.8318964951367,1067.7251047501,443.447791420374));
#126408=CARTESIAN_POINT('Origin',(78.8318964951367,1082.7251047501,444.508672230294));
#126409=CARTESIAN_POINT('Origin',(12.9199830389075,1067.7251047501,410.449386612842));
#126410=CARTESIAN_POINT('',(12.9199830389075,1078.73142393294,409.349028547167));
#126411=CARTESIAN_POINT('Origin',(12.9199830389075,1078.73142393294,410.449386612842));
#126412=CARTESIAN_POINT('',(12.9199830389075,1076.73142393294,409.349028547167));
#126413=CARTESIAN_POINT('',(12.9199830389075,1067.7251047501,409.349028547167));
#126414=CARTESIAN_POINT('Origin',(12.9199830389075,1076.73142393294,410.449386612842));
#126415=CARTESIAN_POINT('Origin',(12.9199830389075,1067.7251047501,410.449386612842));
#126416=CARTESIAN_POINT('',(12.9199830389075,1076.73142393294,409.949028547167));
#126417=CARTESIAN_POINT('Origin',(12.9199830389075,1076.73142393294,410.449386612842));
#126418=CARTESIAN_POINT('',(12.9199830389075,1082.7251047501,409.949028547167));
#126419=CARTESIAN_POINT('',(12.9199830389075,1067.7251047501,409.949028547167));
#126420=CARTESIAN_POINT('Origin',(12.9199830389075,1082.7251047501,410.449386612842));
#126421=CARTESIAN_POINT('Origin',(20.4506997939064,1067.7251047501,406.371927175053));
#126422=CARTESIAN_POINT('',(20.4506997939064,1078.73142393294,405.157895608316));
#126423=CARTESIAN_POINT('Origin',(20.4506997939064,1078.73142393294,406.371927175053));
#126424=CARTESIAN_POINT('',(20.4506997939064,1076.73142393294,405.157895608316));
#126425=CARTESIAN_POINT('',(20.4506997939064,1067.7251047501,405.157895608316));
#126426=CARTESIAN_POINT('Origin',(20.4506997939064,1076.73142393294,406.371927175053));
#126427=CARTESIAN_POINT('Origin',(20.4506997939064,1067.7251047501,406.371927175053));
#126428=CARTESIAN_POINT('',(20.4506997939064,1076.73142393294,405.757895608316));
#126429=CARTESIAN_POINT('Origin',(20.4506997939064,1076.73142393294,406.371927175053));
#126430=CARTESIAN_POINT('',(20.4506997939064,1082.7251047501,405.757895608316));
#126431=CARTESIAN_POINT('',(20.4506997939064,1067.7251047501,405.757895608316));
#126432=CARTESIAN_POINT('Origin',(20.4506997939064,1082.7251047501,406.371927175053));
#126433=CARTESIAN_POINT('Origin',(28.1241080594971,1067.7251047501,404.387564478864));
#126434=CARTESIAN_POINT('',(28.1241080594971,1078.73142393294,403.058756515291));
#126435=CARTESIAN_POINT('Origin',(28.1241080594971,1078.73142393294,404.387564478864));
#126436=CARTESIAN_POINT('',(28.1241080594971,1076.73142393294,403.058756515291));
#126437=CARTESIAN_POINT('',(28.1241080594971,1067.7251047501,403.058756515291));
#126438=CARTESIAN_POINT('Origin',(28.1241080594971,1076.73142393294,404.387564478864));
#126439=CARTESIAN_POINT('Origin',(28.1241080594971,1067.7251047501,404.387564478864));
#126440=CARTESIAN_POINT('',(28.1241080594971,1076.73142393294,403.658756515291));
#126441=CARTESIAN_POINT('Origin',(28.1241080594971,1076.73142393294,404.387564478864));
#126442=CARTESIAN_POINT('',(28.1241080594971,1082.7251047501,403.658756515291));
#126443=CARTESIAN_POINT('',(28.1241080594971,1067.7251047501,403.658756515291));
#126444=CARTESIAN_POINT('Origin',(28.1241080594971,1082.7251047501,404.387564478864));
#126445=CARTESIAN_POINT('Origin',(37.3561099563906,1067.7251047501,403.549365385362));
#126446=CARTESIAN_POINT('',(37.3561099563906,1078.73142393294,402.088248383545));
#126447=CARTESIAN_POINT('Origin',(37.3561099563906,1078.73142393294,403.549365385362));
#126448=CARTESIAN_POINT('',(37.3561099563906,1076.73142393294,402.088248383545));
#126449=CARTESIAN_POINT('',(37.3561099563906,1067.7251047501,402.088248383545));
#126450=CARTESIAN_POINT('Origin',(37.3561099563906,1076.73142393294,403.549365385362));
#126451=CARTESIAN_POINT('Origin',(37.3561099563906,1067.7251047501,403.549365385362));
#126452=CARTESIAN_POINT('',(37.3561099563906,1076.73142393294,402.688248383545));
#126453=CARTESIAN_POINT('Origin',(37.3561099563906,1076.73142393294,403.549365385362));
#126454=CARTESIAN_POINT('',(37.3561099563906,1082.7251047501,402.688248383545));
#126455=CARTESIAN_POINT('',(37.3561099563906,1067.7251047501,402.688248383545));
#126456=CARTESIAN_POINT('Origin',(37.3561099563906,1082.7251047501,403.549365385362));
#126457=CARTESIAN_POINT('Origin',(46.1653962245145,1067.7251047501,404.953573696928));
#126458=CARTESIAN_POINT('',(46.1653962245145,1078.73142393294,403.333091654304));
#126459=CARTESIAN_POINT('Origin',(46.1653962245145,1078.73142393294,404.953573696928));
#126460=CARTESIAN_POINT('',(46.1653962245145,1076.73142393294,403.333091654304));
#126461=CARTESIAN_POINT('',(46.1653962245145,1067.7251047501,403.333091654304));
#126462=CARTESIAN_POINT('Origin',(46.1653962245145,1076.73142393294,404.953573696928));
#126463=CARTESIAN_POINT('Origin',(46.1653962245145,1067.7251047501,404.953573696928));
#126464=CARTESIAN_POINT('',(46.1653962245145,1076.73142393294,403.933091654304));
#126465=CARTESIAN_POINT('Origin',(46.1653962245145,1076.73142393294,404.953573696928));
#126466=CARTESIAN_POINT('',(46.1653962245145,1082.7251047501,403.933091654304));
#126467=CARTESIAN_POINT('',(46.1653962245145,1067.7251047501,403.933091654304));
#126468=CARTESIAN_POINT('Origin',(46.1653962245145,1082.7251047501,404.953573696928));
#126469=CARTESIAN_POINT('Origin',(55.9328578081739,1067.7251047501,407.800553648799));
#126470=CARTESIAN_POINT('',(55.9328578081739,1078.73142393294,406.099553425716));
#126471=CARTESIAN_POINT('Origin',(55.9328578081739,1078.73142393294,407.800553648799));
#126472=CARTESIAN_POINT('',(55.9328578081739,1076.73142393294,406.099553425716));
#126473=CARTESIAN_POINT('',(55.9328578081739,1067.7251047501,406.099553425716));
#126474=CARTESIAN_POINT('Origin',(55.9328578081739,1076.73142393294,407.800553648799));
#126475=CARTESIAN_POINT('Origin',(55.9328578081739,1067.7251047501,407.800553648799));
#126476=CARTESIAN_POINT('',(55.9328578081739,1076.73142393294,406.699553425716));
#126477=CARTESIAN_POINT('Origin',(55.9328578081739,1076.73142393294,407.800553648799));
#126478=CARTESIAN_POINT('',(55.9328578081739,1082.7251047501,406.699553425716));
#126479=CARTESIAN_POINT('',(55.9328578081739,1067.7251047501,406.699553425716));
#126480=CARTESIAN_POINT('Origin',(55.9328578081739,1082.7251047501,407.800553648799));
#126481=CARTESIAN_POINT('Origin',(64.5265634583882,1067.7251047501,412.64686525254));
#126482=CARTESIAN_POINT('',(64.5265634583882,1078.73142393294,410.925590620497));
#126483=CARTESIAN_POINT('Origin',(64.5265634583882,1078.73142393294,412.64686525254));
#126484=CARTESIAN_POINT('',(64.5265634583882,1076.73142393294,410.925590620497));
#126485=CARTESIAN_POINT('',(64.5265634583882,1067.7251047501,410.925590620497));
#126486=CARTESIAN_POINT('Origin',(64.5265634583882,1076.73142393294,412.64686525254));
#126487=CARTESIAN_POINT('Origin',(64.5265634583882,1067.7251047501,412.64686525254));
#126488=CARTESIAN_POINT('',(64.5265634583882,1076.73142393294,411.525590620497));
#126489=CARTESIAN_POINT('Origin',(64.5265634583882,1076.73142393294,412.64686525254));
#126490=CARTESIAN_POINT('',(64.5265634583882,1082.7251047501,411.525590620497));
#126491=CARTESIAN_POINT('',(64.5265634583882,1067.7251047501,411.525590620497));
#126492=CARTESIAN_POINT('Origin',(64.5265634583882,1082.7251047501,412.64686525254));
#126493=CARTESIAN_POINT('Origin',(73.7486774752213,1067.7251047501,419.332473131695));
#126494=CARTESIAN_POINT('',(73.7486774752213,1078.73142393294,417.55048047729));
#126495=CARTESIAN_POINT('Origin',(73.7486774752213,1078.73142393294,419.332473131695));
#126496=CARTESIAN_POINT('',(73.7486774752213,1076.73142393294,417.55048047729));
#126497=CARTESIAN_POINT('',(73.7486774752213,1067.7251047501,417.55048047729));
#126498=CARTESIAN_POINT('Origin',(73.7486774752213,1076.73142393294,419.332473131695));
#126499=CARTESIAN_POINT('Origin',(73.7486774752213,1067.7251047501,419.332473131695));
#126500=CARTESIAN_POINT('',(73.7486774752213,1076.73142393294,418.15048047729));
#126501=CARTESIAN_POINT('Origin',(73.7486774752213,1076.73142393294,419.332473131695));
#126502=CARTESIAN_POINT('',(73.7486774752213,1082.7251047501,418.15048047729));
#126503=CARTESIAN_POINT('',(73.7486774752213,1067.7251047501,418.15048047729));
#126504=CARTESIAN_POINT('Origin',(73.7486774752213,1082.7251047501,419.332473131695));
#126505=CARTESIAN_POINT('Origin',(81.2442674543467,1067.7251047501,427.683989434121));
#126506=CARTESIAN_POINT('',(81.2442674543467,1078.73142393294,426.0231086242));
#126507=CARTESIAN_POINT('Origin',(81.2442674543467,1078.73142393294,427.683989434121));
#126508=CARTESIAN_POINT('',(81.2442674543467,1076.73142393294,426.0231086242));
#126509=CARTESIAN_POINT('',(81.2442674543467,1067.7251047501,426.0231086242));
#126510=CARTESIAN_POINT('Origin',(81.2442674543467,1076.73142393294,427.683989434121));
#126511=CARTESIAN_POINT('Origin',(81.2442674543467,1067.7251047501,427.683989434121));
#126512=CARTESIAN_POINT('',(81.2442674543467,1076.73142393294,426.6231086242));
#126513=CARTESIAN_POINT('Origin',(81.2442674543467,1076.73142393294,427.683989434121));
#126514=CARTESIAN_POINT('',(81.2442674543467,1082.7251047501,426.6231086242));
#126515=CARTESIAN_POINT('',(81.2442674543467,1067.7251047501,426.6231086242));
#126516=CARTESIAN_POINT('Origin',(81.2442674543467,1082.7251047501,427.683989434121));
#126517=CARTESIAN_POINT('Origin',(9.69136378659227,1067.7251047501,408.072838296421));
#126518=CARTESIAN_POINT('',(9.69136378659227,1078.73142393294,406.972480230746));
#126519=CARTESIAN_POINT('Origin',(9.69136378659227,1078.73142393294,408.072838296421));
#126520=CARTESIAN_POINT('',(9.69136378659227,1076.73142393294,406.972480230746));
#126521=CARTESIAN_POINT('',(9.69136378659227,1067.7251047501,406.972480230746));
#126522=CARTESIAN_POINT('Origin',(9.69136378659227,1076.73142393294,408.072838296421));
#126523=CARTESIAN_POINT('Origin',(9.69136378659227,1067.7251047501,408.072838296421));
#126524=CARTESIAN_POINT('',(9.69136378659227,1076.73142393294,407.572480230746));
#126525=CARTESIAN_POINT('Origin',(9.69136378659227,1076.73142393294,408.072838296421));
#126526=CARTESIAN_POINT('',(9.69136378659227,1082.7251047501,407.572480230746));
#126527=CARTESIAN_POINT('',(9.69136378659227,1067.7251047501,407.572480230746));
#126528=CARTESIAN_POINT('Origin',(9.69136378659227,1082.7251047501,408.072838296421));
#126529=CARTESIAN_POINT('Origin',(16.2097648263488,1067.7251047501,402.518757076657));
#126530=CARTESIAN_POINT('',(16.2097648263488,1078.73142393294,401.30472550992));
#126531=CARTESIAN_POINT('Origin',(16.2097648263488,1078.73142393294,402.518757076657));
#126532=CARTESIAN_POINT('',(16.2097648263488,1076.73142393294,401.30472550992));
#126533=CARTESIAN_POINT('',(16.2097648263488,1067.7251047501,401.30472550992));
#126534=CARTESIAN_POINT('Origin',(16.2097648263488,1076.73142393294,402.518757076657));
#126535=CARTESIAN_POINT('Origin',(16.2097648263488,1067.7251047501,402.518757076657));
#126536=CARTESIAN_POINT('',(16.2097648263488,1076.73142393294,401.90472550992));
#126537=CARTESIAN_POINT('Origin',(16.2097648263488,1076.73142393294,402.518757076657));
#126538=CARTESIAN_POINT('',(16.2097648263488,1082.7251047501,401.90472550992));
#126539=CARTESIAN_POINT('',(16.2097648263488,1067.7251047501,401.90472550992));
#126540=CARTESIAN_POINT('Origin',(16.2097648263488,1082.7251047501,402.518757076657));
#126541=CARTESIAN_POINT('Origin',(23.302918507427,1067.7251047501,398.98236617956));
#126542=CARTESIAN_POINT('',(23.302918507427,1078.73142393294,397.653558215986));
#126543=CARTESIAN_POINT('Origin',(23.302918507427,1078.73142393294,398.98236617956));
#126544=CARTESIAN_POINT('',(23.302918507427,1076.73142393294,397.653558215986));
#126545=CARTESIAN_POINT('',(23.302918507427,1067.7251047501,397.653558215986));
#126546=CARTESIAN_POINT('Origin',(23.302918507427,1076.73142393294,398.98236617956));
#126547=CARTESIAN_POINT('Origin',(23.302918507427,1067.7251047501,398.98236617956));
#126548=CARTESIAN_POINT('',(23.302918507427,1076.73142393294,398.253558215986));
#126549=CARTESIAN_POINT('Origin',(23.302918507427,1076.73142393294,398.98236617956));
#126550=CARTESIAN_POINT('',(23.302918507427,1082.7251047501,398.253558215986));
#126551=CARTESIAN_POINT('',(23.302918507427,1067.7251047501,398.253558215986));
#126552=CARTESIAN_POINT('Origin',(23.302918507427,1082.7251047501,398.98236617956));
#126553=CARTESIAN_POINT('Origin',(32.1589076220714,1067.7251047501,396.243042623298));
#126554=CARTESIAN_POINT('',(32.1589076220714,1078.73142393294,394.781925621481));
#126555=CARTESIAN_POINT('Origin',(32.1589076220714,1078.73142393294,396.243042623298));
#126556=CARTESIAN_POINT('',(32.1589076220714,1076.73142393294,394.781925621481));
#126557=CARTESIAN_POINT('',(32.1589076220714,1067.7251047501,394.781925621481));
#126558=CARTESIAN_POINT('Origin',(32.1589076220714,1076.73142393294,396.243042623298));
#126559=CARTESIAN_POINT('Origin',(32.1589076220714,1067.7251047501,396.243042623298));
#126560=CARTESIAN_POINT('',(32.1589076220714,1076.73142393294,395.381925621481));
#126561=CARTESIAN_POINT('Origin',(32.1589076220714,1076.73142393294,396.243042623298));
#126562=CARTESIAN_POINT('',(32.1589076220714,1082.7251047501,395.381925621481));
#126563=CARTESIAN_POINT('',(32.1589076220714,1067.7251047501,395.381925621481));
#126564=CARTESIAN_POINT('Origin',(32.1589076220714,1082.7251047501,396.243042623298));
#126565=CARTESIAN_POINT('Origin',(41.0676411737322,1067.7251047501,395.785012011284));
#126566=CARTESIAN_POINT('',(41.0676411737322,1078.73142393294,394.164529968659));
#126567=CARTESIAN_POINT('Origin',(41.0676411737322,1078.73142393294,395.785012011284));
#126568=CARTESIAN_POINT('',(41.0676411737322,1076.73142393294,394.164529968659));
#126569=CARTESIAN_POINT('',(41.0676411737322,1067.7251047501,394.164529968659));
#126570=CARTESIAN_POINT('Origin',(41.0676411737322,1076.73142393294,395.785012011284));
#126571=CARTESIAN_POINT('Origin',(41.0676411737322,1067.7251047501,395.785012011284));
#126572=CARTESIAN_POINT('',(41.0676411737322,1076.73142393294,394.764529968659));
#126573=CARTESIAN_POINT('Origin',(41.0676411737322,1076.73142393294,395.785012011284));
#126574=CARTESIAN_POINT('',(41.0676411737322,1082.7251047501,394.764529968659));
#126575=CARTESIAN_POINT('',(41.0676411737322,1067.7251047501,394.764529968659));
#126576=CARTESIAN_POINT('Origin',(41.0676411737322,1082.7251047501,395.785012011284));
#126577=CARTESIAN_POINT('Origin',(51.2135807025659,1067.7251047501,396.539009167687));
#126578=CARTESIAN_POINT('',(51.2135807025659,1078.73142393294,394.838008944604));
#126579=CARTESIAN_POINT('Origin',(51.2135807025659,1078.73142393294,396.539009167687));
#126580=CARTESIAN_POINT('',(51.2135807025659,1076.73142393294,394.838008944604));
#126581=CARTESIAN_POINT('',(51.2135807025659,1067.7251047501,394.838008944604));
#126582=CARTESIAN_POINT('Origin',(51.2135807025659,1076.73142393294,396.539009167687));
#126583=CARTESIAN_POINT('Origin',(51.2135807025659,1067.7251047501,396.539009167687));
#126584=CARTESIAN_POINT('',(51.2135807025659,1076.73142393294,395.438008944604));
#126585=CARTESIAN_POINT('Origin',(51.2135807025659,1076.73142393294,396.539009167687));
#126586=CARTESIAN_POINT('',(51.2135807025659,1082.7251047501,395.438008944604));
#126587=CARTESIAN_POINT('',(51.2135807025659,1067.7251047501,395.438008944604));
#126588=CARTESIAN_POINT('Origin',(51.2135807025659,1082.7251047501,396.539009167687));
#126589=CARTESIAN_POINT('Origin',(60.6270981054991,1067.7251047501,399.492685363169));
#126590=CARTESIAN_POINT('',(60.6270981054991,1078.73142393294,397.771410731125));
#126591=CARTESIAN_POINT('Origin',(60.6270981054991,1078.73142393294,399.492685363169));
#126592=CARTESIAN_POINT('',(60.6270981054991,1076.73142393294,397.771410731125));
#126593=CARTESIAN_POINT('',(60.6270981054991,1067.7251047501,397.771410731125));
#126594=CARTESIAN_POINT('Origin',(60.6270981054991,1076.73142393294,399.492685363169));
#126595=CARTESIAN_POINT('Origin',(60.6270981054991,1067.7251047501,399.492685363169));
#126596=CARTESIAN_POINT('',(60.6270981054991,1076.73142393294,398.371410731125));
#126597=CARTESIAN_POINT('Origin',(60.6270981054991,1076.73142393294,399.492685363169));
#126598=CARTESIAN_POINT('',(60.6270981054991,1082.7251047501,398.371410731125));
#126599=CARTESIAN_POINT('',(60.6270981054991,1067.7251047501,398.371410731125));
#126600=CARTESIAN_POINT('Origin',(60.6270981054991,1082.7251047501,399.492685363169));
#126601=CARTESIAN_POINT('Origin',(71.0377028430577,1067.7251047501,404.114811351457));
#126602=CARTESIAN_POINT('',(71.0377028430577,1078.73142393294,402.332818697052));
#126603=CARTESIAN_POINT('Origin',(71.0377028430577,1078.73142393294,404.114811351457));
#126604=CARTESIAN_POINT('',(71.0377028430577,1076.73142393294,402.332818697052));
#126605=CARTESIAN_POINT('',(71.0377028430577,1067.7251047501,402.332818697052));
#126606=CARTESIAN_POINT('Origin',(71.0377028430577,1076.73142393294,404.114811351457));
#126607=CARTESIAN_POINT('Origin',(71.0377028430577,1067.7251047501,404.114811351457));
#126608=CARTESIAN_POINT('',(71.0377028430577,1076.73142393294,402.932818697052));
#126609=CARTESIAN_POINT('Origin',(71.0377028430577,1076.73142393294,404.114811351457));
#126610=CARTESIAN_POINT('',(71.0377028430577,1082.7251047501,402.932818697052));
#126611=CARTESIAN_POINT('',(71.0377028430577,1067.7251047501,402.932818697052));
#126612=CARTESIAN_POINT('Origin',(71.0377028430577,1082.7251047501,404.114811351457));
#126613=CARTESIAN_POINT('Origin',(80.105874072553,1067.7251047501,410.725406198927));
#126614=CARTESIAN_POINT('',(80.105874072553,1078.73142393294,409.064525389007));
#126615=CARTESIAN_POINT('Origin',(80.105874072553,1078.73142393294,410.725406198927));
#126616=CARTESIAN_POINT('',(80.105874072553,1076.73142393294,409.064525389007));
#126617=CARTESIAN_POINT('',(80.105874072553,1067.7251047501,409.064525389007));
#126618=CARTESIAN_POINT('Origin',(80.105874072553,1076.73142393294,410.725406198927));
#126619=CARTESIAN_POINT('Origin',(80.105874072553,1067.7251047501,410.725406198927));
#126620=CARTESIAN_POINT('',(80.105874072553,1076.73142393294,409.664525389007));
#126621=CARTESIAN_POINT('Origin',(80.105874072553,1076.73142393294,410.725406198927));
#126622=CARTESIAN_POINT('',(80.105874072553,1082.7251047501,409.664525389007));
#126623=CARTESIAN_POINT('',(80.105874072553,1067.7251047501,409.664525389007));
#126624=CARTESIAN_POINT('Origin',(80.105874072553,1082.7251047501,410.725406198927));
#126625=CARTESIAN_POINT('Origin',(6.03918543248003,1067.7251047501,406.419490950441));
#126626=CARTESIAN_POINT('',(6.03918543248003,1078.73142393294,405.319132884767));
#126627=CARTESIAN_POINT('Origin',(6.03918543248003,1078.73142393294,406.419490950441));
#126628=CARTESIAN_POINT('',(6.03918543248003,1076.73142393294,405.319132884767));
#126629=CARTESIAN_POINT('',(6.03918543248003,1067.7251047501,405.319132884767));
#126630=CARTESIAN_POINT('Origin',(6.03918543248003,1076.73142393294,406.419490950441));
#126631=CARTESIAN_POINT('Origin',(6.03918543248003,1067.7251047501,406.419490950441));
#126632=CARTESIAN_POINT('',(6.03918543248003,1076.73142393294,405.919132884767));
#126633=CARTESIAN_POINT('Origin',(6.03918543248003,1076.73142393294,406.419490950441));
#126634=CARTESIAN_POINT('',(6.03918543248003,1082.7251047501,405.919132884767));
#126635=CARTESIAN_POINT('',(6.03918543248003,1067.7251047501,405.919132884767));
#126636=CARTESIAN_POINT('Origin',(6.03918543248003,1082.7251047501,406.419490950441));
#126637=CARTESIAN_POINT('Origin',(11.2603853527983,1067.7251047501,399.631527949444));
#126638=CARTESIAN_POINT('',(11.2603853527983,1078.73142393294,398.417496382707));
#126639=CARTESIAN_POINT('Origin',(11.2603853527983,1078.73142393294,399.631527949444));
#126640=CARTESIAN_POINT('',(11.2603853527983,1076.73142393294,398.417496382707));
#126641=CARTESIAN_POINT('',(11.2603853527983,1067.7251047501,398.417496382707));
#126642=CARTESIAN_POINT('Origin',(11.2603853527983,1076.73142393294,399.631527949444));
#126643=CARTESIAN_POINT('Origin',(11.2603853527983,1067.7251047501,399.631527949444));
#126644=CARTESIAN_POINT('',(11.2603853527983,1076.73142393294,399.017496382707));
#126645=CARTESIAN_POINT('Origin',(11.2603853527983,1076.73142393294,399.631527949444));
#126646=CARTESIAN_POINT('',(11.2603853527983,1082.7251047501,399.017496382707));
#126647=CARTESIAN_POINT('',(11.2603853527983,1067.7251047501,399.017496382707));
#126648=CARTESIAN_POINT('Origin',(11.2603853527983,1082.7251047501,399.631527949444));
#126649=CARTESIAN_POINT('Origin',(17.4632795967732,1067.7251047501,394.697666103129));
#126650=CARTESIAN_POINT('',(17.4632795967732,1078.73142393294,393.368858139556));
#126651=CARTESIAN_POINT('Origin',(17.4632795967732,1078.73142393294,394.697666103129));
#126652=CARTESIAN_POINT('',(17.4632795967732,1076.73142393294,393.368858139556));
#126653=CARTESIAN_POINT('',(17.4632795967732,1067.7251047501,393.368858139556));
#126654=CARTESIAN_POINT('Origin',(17.4632795967732,1076.73142393294,394.697666103129));
#126655=CARTESIAN_POINT('Origin',(17.4632795967732,1067.7251047501,394.697666103129));
#126656=CARTESIAN_POINT('',(17.4632795967732,1076.73142393294,393.968858139556));
#126657=CARTESIAN_POINT('Origin',(17.4632795967732,1076.73142393294,394.697666103129));
#126658=CARTESIAN_POINT('',(17.4632795967732,1082.7251047501,393.968858139556));
#126659=CARTESIAN_POINT('',(17.4632795967732,1067.7251047501,393.968858139556));
#126660=CARTESIAN_POINT('Origin',(17.4632795967732,1082.7251047501,394.697666103129));
#126661=CARTESIAN_POINT('Origin',(25.5562067091079,1067.7251047501,390.176939668248));
#126662=CARTESIAN_POINT('',(25.5562067091079,1078.73142393294,388.715822666431));
#126663=CARTESIAN_POINT('Origin',(25.5562067091079,1078.73142393294,390.176939668248));
#126664=CARTESIAN_POINT('',(25.5562067091079,1076.73142393294,388.715822666431));
#126665=CARTESIAN_POINT('',(25.5562067091079,1067.7251047501,388.715822666431));
#126666=CARTESIAN_POINT('Origin',(25.5562067091079,1076.73142393294,390.176939668248));
#126667=CARTESIAN_POINT('Origin',(25.5562067091079,1067.7251047501,390.176939668248));
#126668=CARTESIAN_POINT('',(25.5562067091079,1076.73142393294,389.315822666431));
#126669=CARTESIAN_POINT('Origin',(25.5562067091079,1076.73142393294,390.176939668248));
#126670=CARTESIAN_POINT('',(25.5562067091079,1082.7251047501,389.315822666431));
#126671=CARTESIAN_POINT('',(25.5562067091079,1067.7251047501,389.315822666431));
#126672=CARTESIAN_POINT('Origin',(25.5562067091079,1082.7251047501,390.176939668248));
#126673=CARTESIAN_POINT('Origin',(34.1750331392515,1067.7251047501,387.876688268273));
#126674=CARTESIAN_POINT('',(34.1750331392515,1078.73142393294,386.256206225648));
#126675=CARTESIAN_POINT('Origin',(34.1750331392515,1078.73142393294,387.876688268273));
#126676=CARTESIAN_POINT('',(34.1750331392515,1076.73142393294,386.256206225648));
#126677=CARTESIAN_POINT('',(34.1750331392515,1067.7251047501,386.256206225648));
#126678=CARTESIAN_POINT('Origin',(34.1750331392515,1076.73142393294,387.876688268273));
#126679=CARTESIAN_POINT('Origin',(34.1750331392515,1067.7251047501,387.876688268273));
#126680=CARTESIAN_POINT('',(34.1750331392515,1076.73142393294,386.856206225649));
#126681=CARTESIAN_POINT('Origin',(34.1750331392515,1076.73142393294,387.876688268273));
#126682=CARTESIAN_POINT('',(34.1750331392515,1082.7251047501,386.856206225649));
#126683=CARTESIAN_POINT('',(34.1750331392515,1067.7251047501,386.856206225649));
#126684=CARTESIAN_POINT('Origin',(34.1750331392515,1082.7251047501,387.876688268273));
#126685=CARTESIAN_POINT('Origin',(44.25602437023,1067.7251047501,386.504749335394));
#126686=CARTESIAN_POINT('',(44.25602437023,1078.73142393294,384.803749112311));
#126687=CARTESIAN_POINT('Origin',(44.25602437023,1078.73142393294,386.504749335394));
#126688=CARTESIAN_POINT('',(44.25602437023,1076.73142393294,384.803749112311));
#126689=CARTESIAN_POINT('',(44.25602437023,1067.7251047501,384.803749112311));
#126690=CARTESIAN_POINT('Origin',(44.25602437023,1076.73142393294,386.504749335394));
#126691=CARTESIAN_POINT('Origin',(44.25602437023,1067.7251047501,386.504749335394));
#126692=CARTESIAN_POINT('',(44.25602437023,1076.73142393294,385.403749112311));
#126693=CARTESIAN_POINT('Origin',(44.25602437023,1076.73142393294,386.504749335394));
#126694=CARTESIAN_POINT('',(44.25602437023,1082.7251047501,385.403749112311));
#126695=CARTESIAN_POINT('',(44.25602437023,1067.7251047501,385.403749112311));
#126696=CARTESIAN_POINT('Origin',(44.25602437023,1082.7251047501,386.504749335394));
#126697=CARTESIAN_POINT('Origin',(54.0779376443059,1067.7251047501,387.436700299563));
#126698=CARTESIAN_POINT('',(54.0779376443059,1078.73142393294,385.71542566752));
#126699=CARTESIAN_POINT('Origin',(54.0779376443059,1078.73142393294,387.436700299563));
#126700=CARTESIAN_POINT('',(54.0779376443059,1076.73142393294,385.71542566752));
#126701=CARTESIAN_POINT('',(54.0779376443059,1067.7251047501,385.71542566752));
#126702=CARTESIAN_POINT('Origin',(54.0779376443059,1076.73142393294,387.436700299563));
#126703=CARTESIAN_POINT('Origin',(54.0779376443059,1067.7251047501,387.436700299563));
#126704=CARTESIAN_POINT('',(54.0779376443059,1076.73142393294,386.31542566752));
#126705=CARTESIAN_POINT('Origin',(54.0779376443059,1076.73142393294,387.436700299563));
#126706=CARTESIAN_POINT('',(54.0779376443059,1082.7251047501,386.31542566752));
#126707=CARTESIAN_POINT('',(54.0779376443059,1067.7251047501,386.31542566752));
#126708=CARTESIAN_POINT('Origin',(54.0779376443059,1082.7251047501,387.436700299563));
#126709=CARTESIAN_POINT('Origin',(65.2220397199346,1067.7251047501,389.793335311876));
#126710=CARTESIAN_POINT('',(65.2220397199346,1078.73142393294,388.011342657471));
#126711=CARTESIAN_POINT('Origin',(65.2220397199346,1078.73142393294,389.793335311876));
#126712=CARTESIAN_POINT('',(65.2220397199346,1076.73142393294,388.011342657471));
#126713=CARTESIAN_POINT('',(65.2220397199346,1067.7251047501,388.011342657471));
#126714=CARTESIAN_POINT('Origin',(65.2220397199346,1076.73142393294,389.793335311876));
#126715=CARTESIAN_POINT('Origin',(65.2220397199346,1067.7251047501,389.793335311876));
#126716=CARTESIAN_POINT('',(65.2220397199346,1076.73142393294,388.611342657471));
#126717=CARTESIAN_POINT('Origin',(65.2220397199346,1076.73142393294,389.793335311876));
#126718=CARTESIAN_POINT('',(65.2220397199346,1082.7251047501,388.611342657471));
#126719=CARTESIAN_POINT('',(65.2220397199346,1067.7251047501,388.611342657471));
#126720=CARTESIAN_POINT('Origin',(65.2220397199346,1082.7251047501,389.793335311876));
#126721=CARTESIAN_POINT('Origin',(75.4664696031574,1067.7251047501,394.374093988403));
#126722=CARTESIAN_POINT('',(75.4664696031574,1078.73142393294,392.713213178482));
#126723=CARTESIAN_POINT('Origin',(75.4664696031574,1078.73142393294,394.374093988403));
#126724=CARTESIAN_POINT('',(75.4664696031574,1076.73142393294,392.713213178482));
#126725=CARTESIAN_POINT('',(75.4664696031574,1067.7251047501,392.713213178482));
#126726=CARTESIAN_POINT('Origin',(75.4664696031574,1076.73142393294,394.374093988403));
#126727=CARTESIAN_POINT('Origin',(75.4664696031574,1067.7251047501,394.374093988403));
#126728=CARTESIAN_POINT('',(75.4664696031574,1076.73142393294,393.313213178482));
#126729=CARTESIAN_POINT('Origin',(75.4664696031574,1076.73142393294,394.374093988403));
#126730=CARTESIAN_POINT('',(75.4664696031574,1082.7251047501,393.313213178482));
#126731=CARTESIAN_POINT('',(75.4664696031574,1067.7251047501,393.313213178482));
#126732=CARTESIAN_POINT('Origin',(75.4664696031574,1082.7251047501,394.374093988403));
#126733=CARTESIAN_POINT('Origin',(2.12306569574147,1067.7251047501,405.561603787563));
#126734=CARTESIAN_POINT('',(2.12306569574147,1078.73142393294,404.461245721888));
#126735=CARTESIAN_POINT('Origin',(2.12306569574147,1078.73142393294,405.561603787563));
#126736=CARTESIAN_POINT('',(2.12306569574147,1076.73142393294,404.461245721888));
#126737=CARTESIAN_POINT('',(2.12306569574147,1067.7251047501,404.461245721888));
#126738=CARTESIAN_POINT('Origin',(2.12306569574147,1076.73142393294,405.561603787563));
#126739=CARTESIAN_POINT('Origin',(2.12306569574147,1067.7251047501,405.561603787563));
#126740=CARTESIAN_POINT('',(2.12306569574147,1076.73142393294,405.061245721888));
#126741=CARTESIAN_POINT('Origin',(2.12306569574147,1076.73142393294,405.561603787563));
#126742=CARTESIAN_POINT('',(2.12306569574147,1082.7251047501,405.061245721888));
#126743=CARTESIAN_POINT('',(2.12306569574147,1067.7251047501,405.061245721888));
#126744=CARTESIAN_POINT('Origin',(2.12306569574147,1082.7251047501,405.561603787563));
#126745=CARTESIAN_POINT('Origin',(5.81887300600675,1067.7251047501,397.836425560737));
#126746=CARTESIAN_POINT('',(5.81887300600675,1078.73142393294,396.622393994));
#126747=CARTESIAN_POINT('Origin',(5.81887300600675,1078.73142393294,397.836425560737));
#126748=CARTESIAN_POINT('',(5.81887300600675,1076.73142393294,396.622393994));
#126749=CARTESIAN_POINT('',(5.81887300600675,1067.7251047501,396.622393994));
#126750=CARTESIAN_POINT('Origin',(5.81887300600675,1076.73142393294,397.836425560737));
#126751=CARTESIAN_POINT('Origin',(5.81887300600675,1067.7251047501,397.836425560737));
#126752=CARTESIAN_POINT('',(5.81887300600675,1076.73142393294,397.222393994));
#126753=CARTESIAN_POINT('Origin',(5.81887300600675,1076.73142393294,397.836425560737));
#126754=CARTESIAN_POINT('',(5.81887300600675,1082.7251047501,397.222393994));
#126755=CARTESIAN_POINT('',(5.81887300600675,1067.7251047501,397.222393994));
#126756=CARTESIAN_POINT('Origin',(5.81887300600675,1082.7251047501,397.836425560737));
#126757=CARTESIAN_POINT('Origin',(10.8604115696276,1067.7251047501,391.720726203183));
#126758=CARTESIAN_POINT('',(10.8604115696276,1078.73142393294,390.39191823961));
#126759=CARTESIAN_POINT('Origin',(10.8604115696276,1078.73142393294,391.720726203183));
#126760=CARTESIAN_POINT('',(10.8604115696276,1076.73142393294,390.39191823961));
#126761=CARTESIAN_POINT('',(10.8604115696276,1067.7251047501,390.39191823961));
#126762=CARTESIAN_POINT('Origin',(10.8604115696276,1076.73142393294,391.720726203183));
#126763=CARTESIAN_POINT('Origin',(10.8604115696276,1067.7251047501,391.720726203183));
#126764=CARTESIAN_POINT('',(10.8604115696276,1076.73142393294,390.99191823961));
#126765=CARTESIAN_POINT('Origin',(10.8604115696276,1076.73142393294,391.720726203183));
#126766=CARTESIAN_POINT('',(10.8604115696276,1082.7251047501,390.99191823961));
#126767=CARTESIAN_POINT('',(10.8604115696276,1067.7251047501,390.99191823961));
#126768=CARTESIAN_POINT('Origin',(10.8604115696276,1082.7251047501,391.720726203183));
#126769=CARTESIAN_POINT('Origin',(17.8365769306708,1067.7251047501,385.61617432774));
#126770=CARTESIAN_POINT('',(17.8365769306708,1078.73142393294,384.155057325923));
#126771=CARTESIAN_POINT('Origin',(17.8365769306708,1078.73142393294,385.61617432774));
#126772=CARTESIAN_POINT('',(17.8365769306708,1076.73142393294,384.155057325923));
#126773=CARTESIAN_POINT('',(17.8365769306708,1067.7251047501,384.155057325923));
#126774=CARTESIAN_POINT('Origin',(17.8365769306708,1076.73142393294,385.61617432774));
#126775=CARTESIAN_POINT('Origin',(17.8365769306708,1067.7251047501,385.61617432774));
#126776=CARTESIAN_POINT('',(17.8365769306708,1076.73142393294,384.755057325923));
#126777=CARTESIAN_POINT('Origin',(17.8365769306708,1076.73142393294,385.61617432774));
#126778=CARTESIAN_POINT('',(17.8365769306708,1082.7251047501,384.755057325923));
#126779=CARTESIAN_POINT('',(17.8365769306708,1067.7251047501,384.755057325923));
#126780=CARTESIAN_POINT('Origin',(17.8365769306708,1082.7251047501,385.61617432774));
#126781=CARTESIAN_POINT('Origin',(25.7888121665822,1067.7251047501,381.574234163814));
#126782=CARTESIAN_POINT('',(25.7888121665822,1078.73142393294,379.953752121189));
#126783=CARTESIAN_POINT('Origin',(25.7888121665822,1078.73142393294,381.574234163814));
#126784=CARTESIAN_POINT('',(25.7888121665822,1076.73142393294,379.953752121189));
#126785=CARTESIAN_POINT('',(25.7888121665822,1067.7251047501,379.953752121189));
#126786=CARTESIAN_POINT('Origin',(25.7888121665822,1076.73142393294,381.574234163814));
#126787=CARTESIAN_POINT('Origin',(25.7888121665822,1067.7251047501,381.574234163814));
#126788=CARTESIAN_POINT('',(25.7888121665822,1076.73142393294,380.55375212119));
#126789=CARTESIAN_POINT('Origin',(25.7888121665822,1076.73142393294,381.574234163814));
#126790=CARTESIAN_POINT('',(25.7888121665822,1082.7251047501,380.55375212119));
#126791=CARTESIAN_POINT('',(25.7888121665822,1067.7251047501,380.55375212119));
#126792=CARTESIAN_POINT('Origin',(25.7888121665822,1082.7251047501,381.574234163814));
#126793=CARTESIAN_POINT('Origin',(35.3642674089487,1067.7251047501,378.136319456314));
#126794=CARTESIAN_POINT('',(35.3642674089487,1078.73142393294,376.435319233231));
#126795=CARTESIAN_POINT('Origin',(35.3642674089487,1078.73142393294,378.136319456314));
#126796=CARTESIAN_POINT('',(35.3642674089487,1076.73142393294,376.435319233231));
#126797=CARTESIAN_POINT('',(35.3642674089487,1067.7251047501,376.435319233231));
#126798=CARTESIAN_POINT('Origin',(35.3642674089487,1076.73142393294,378.136319456314));
#126799=CARTESIAN_POINT('Origin',(35.3642674089487,1067.7251047501,378.136319456314));
#126800=CARTESIAN_POINT('',(35.3642674089487,1076.73142393294,377.035319233231));
#126801=CARTESIAN_POINT('Origin',(35.3642674089487,1076.73142393294,378.136319456314));
#126802=CARTESIAN_POINT('',(35.3642674089487,1082.7251047501,377.035319233231));
#126803=CARTESIAN_POINT('',(35.3642674089487,1067.7251047501,377.035319233231));
#126804=CARTESIAN_POINT('Origin',(35.3642674089487,1082.7251047501,378.136319456314));
#126805=CARTESIAN_POINT('Origin',(45.1653118133212,1067.7251047501,377.005814460039));
#126806=CARTESIAN_POINT('',(45.1653118133212,1078.73142393294,375.284539827995));
#126807=CARTESIAN_POINT('Origin',(45.1653118133212,1078.73142393294,377.005814460039));
#126808=CARTESIAN_POINT('',(45.1653118133212,1076.73142393294,375.284539827995));
#126809=CARTESIAN_POINT('',(45.1653118133212,1067.7251047501,375.284539827995));
#126810=CARTESIAN_POINT('Origin',(45.1653118133212,1076.73142393294,377.005814460039));
#126811=CARTESIAN_POINT('Origin',(45.1653118133212,1067.7251047501,377.005814460039));
#126812=CARTESIAN_POINT('',(45.1653118133212,1076.73142393294,375.884539827995));
#126813=CARTESIAN_POINT('Origin',(45.1653118133212,1076.73142393294,377.005814460039));
#126814=CARTESIAN_POINT('',(45.1653118133212,1082.7251047501,375.884539827995));
#126815=CARTESIAN_POINT('',(45.1653118133212,1067.7251047501,375.884539827995));
#126816=CARTESIAN_POINT('Origin',(45.1653118133212,1082.7251047501,377.005814460039));
#126817=CARTESIAN_POINT('Origin',(56.5558604909803,1067.7251047501,376.993962237948));
#126818=CARTESIAN_POINT('',(56.5558604909803,1078.73142393294,375.211969583543));
#126819=CARTESIAN_POINT('Origin',(56.5558604909803,1078.73142393294,376.993962237948));
#126820=CARTESIAN_POINT('',(56.5558604909803,1076.73142393294,375.211969583543));
#126821=CARTESIAN_POINT('',(56.5558604909803,1067.7251047501,375.211969583543));
#126822=CARTESIAN_POINT('Origin',(56.5558604909803,1076.73142393294,376.993962237948));
#126823=CARTESIAN_POINT('Origin',(56.5558604909803,1067.7251047501,376.993962237948));
#126824=CARTESIAN_POINT('',(56.5558604909803,1076.73142393294,375.811969583543));
#126825=CARTESIAN_POINT('Origin',(56.5558604909803,1076.73142393294,376.993962237948));
#126826=CARTESIAN_POINT('',(56.5558604909803,1082.7251047501,375.811969583543));
#126827=CARTESIAN_POINT('',(56.5558604909803,1067.7251047501,375.811969583543));
#126828=CARTESIAN_POINT('Origin',(56.5558604909803,1082.7251047501,376.993962237948));
#126829=CARTESIAN_POINT('Origin',(67.5288182838053,1067.7251047501,379.344683608449));
#126830=CARTESIAN_POINT('',(67.5288182838053,1078.73142393294,377.683802798528));
#126831=CARTESIAN_POINT('Origin',(67.5288182838053,1078.73142393294,379.344683608449));
#126832=CARTESIAN_POINT('',(67.5288182838053,1076.73142393294,377.683802798528));
#126833=CARTESIAN_POINT('',(67.5288182838053,1067.7251047501,377.683802798528));
#126834=CARTESIAN_POINT('Origin',(67.5288182838053,1076.73142393294,379.344683608449));
#126835=CARTESIAN_POINT('Origin',(67.5288182838053,1067.7251047501,379.344683608449));
#126836=CARTESIAN_POINT('',(67.5288182838053,1076.73142393294,378.283802798528));
#126837=CARTESIAN_POINT('Origin',(67.5288182838053,1076.73142393294,379.344683608449));
#126838=CARTESIAN_POINT('',(67.5288182838053,1082.7251047501,378.283802798528));
#126839=CARTESIAN_POINT('',(67.5288182838053,1067.7251047501,378.283802798528));
#126840=CARTESIAN_POINT('Origin',(67.5288182838053,1082.7251047501,379.344683608449));
#126841=CARTESIAN_POINT('Origin',(-1.88584219950044,1067.7251047501,405.536670593404));
#126842=CARTESIAN_POINT('',(-1.88584219950044,1078.73142393294,404.436312527729));
#126843=CARTESIAN_POINT('Origin',(-1.88584219950044,1078.73142393294,405.536670593404));
#126844=CARTESIAN_POINT('',(-1.88584219950044,1076.73142393294,404.436312527729));
#126845=CARTESIAN_POINT('',(-1.88584219950044,1067.7251047501,404.436312527729));
#126846=CARTESIAN_POINT('Origin',(-1.88584219950044,1076.73142393294,405.536670593404));
#126847=CARTESIAN_POINT('Origin',(-1.88584219950044,1067.7251047501,405.536670593404));
#126848=CARTESIAN_POINT('',(-1.88584219950044,1076.73142393294,405.036312527729));
#126849=CARTESIAN_POINT('Origin',(-1.88584219950044,1076.73142393294,405.536670593404));
#126850=CARTESIAN_POINT('',(-1.88584219950044,1082.7251047501,405.036312527729));
#126851=CARTESIAN_POINT('',(-1.88584219950044,1067.7251047501,405.036312527729));
#126852=CARTESIAN_POINT('Origin',(-1.88584219950044,1082.7251047501,405.536670593404));
#126853=CARTESIAN_POINT('Origin',(0.123047986802127,1067.7251047501,397.211904498779));
#126854=CARTESIAN_POINT('',(0.123047986802127,1078.73142393294,395.997872932042));
#126855=CARTESIAN_POINT('Origin',(0.123047986802127,1078.73142393294,397.211904498779));
#126856=CARTESIAN_POINT('',(0.123047986802127,1076.73142393294,395.997872932042));
#126857=CARTESIAN_POINT('',(0.123047986802127,1067.7251047501,395.997872932042));
#126858=CARTESIAN_POINT('Origin',(0.123047986802127,1076.73142393294,397.211904498779));
#126859=CARTESIAN_POINT('Origin',(0.123047986802127,1067.7251047501,397.211904498779));
#126860=CARTESIAN_POINT('',(0.123047986802127,1076.73142393294,396.597872932042));
#126861=CARTESIAN_POINT('Origin',(0.123047986802127,1076.73142393294,397.211904498779));
#126862=CARTESIAN_POINT('',(0.123047986802127,1082.7251047501,396.597872932042));
#126863=CARTESIAN_POINT('',(0.123047986802127,1067.7251047501,396.597872932042));
#126864=CARTESIAN_POINT('Origin',(0.123047986802127,1082.7251047501,397.211904498779));
#126865=CARTESIAN_POINT('Origin',(3.7828914428526,1067.7251047501,390.181653038293));
#126866=CARTESIAN_POINT('',(3.7828914428526,1078.73142393294,388.85284507472));
#126867=CARTESIAN_POINT('Origin',(3.7828914428526,1078.73142393294,390.181653038293));
#126868=CARTESIAN_POINT('',(3.7828914428526,1076.73142393294,388.85284507472));
#126869=CARTESIAN_POINT('',(3.7828914428526,1067.7251047501,388.85284507472));
#126870=CARTESIAN_POINT('Origin',(3.7828914428526,1076.73142393294,390.181653038293));
#126871=CARTESIAN_POINT('Origin',(3.7828914428526,1067.7251047501,390.181653038293));
#126872=CARTESIAN_POINT('',(3.7828914428526,1076.73142393294,389.45284507472));
#126873=CARTESIAN_POINT('Origin',(3.7828914428526,1076.73142393294,390.181653038293));
#126874=CARTESIAN_POINT('',(3.7828914428526,1082.7251047501,389.45284507472));
#126875=CARTESIAN_POINT('',(3.7828914428526,1067.7251047501,389.45284507472));
#126876=CARTESIAN_POINT('Origin',(3.7828914428526,1082.7251047501,390.181653038293));
#126877=CARTESIAN_POINT('Origin',(9.33740315097129,1067.7251047501,382.760073932135));
#126878=CARTESIAN_POINT('',(9.33740315097129,1078.73142393294,381.298956930318));
#126879=CARTESIAN_POINT('Origin',(9.33740315097129,1078.73142393294,382.760073932135));
#126880=CARTESIAN_POINT('',(9.33740315097129,1076.73142393294,381.298956930318));
#126881=CARTESIAN_POINT('',(9.33740315097129,1067.7251047501,381.298956930318));
#126882=CARTESIAN_POINT('Origin',(9.33740315097129,1076.73142393294,382.760073932135));
#126883=CARTESIAN_POINT('Origin',(9.33740315097129,1067.7251047501,382.760073932135));
#126884=CARTESIAN_POINT('',(9.33740315097129,1076.73142393294,381.898956930318));
#126885=CARTESIAN_POINT('Origin',(9.33740315097129,1076.73142393294,382.760073932135));
#126886=CARTESIAN_POINT('',(9.33740315097129,1082.7251047501,381.898956930318));
#126887=CARTESIAN_POINT('',(9.33740315097129,1067.7251047501,381.898956930318));
#126888=CARTESIAN_POINT('Origin',(9.33740315097129,1082.7251047501,382.760073932135));
#126889=CARTESIAN_POINT('Origin',(16.2754963537827,1067.7251047501,377.153097184802));
#126890=CARTESIAN_POINT('',(16.2754963537827,1078.73142393294,375.532615142177));
#126891=CARTESIAN_POINT('Origin',(16.2754963537827,1078.73142393294,377.153097184802));
#126892=CARTESIAN_POINT('',(16.2754963537827,1076.73142393294,375.532615142177));
#126893=CARTESIAN_POINT('',(16.2754963537827,1067.7251047501,375.532615142177));
#126894=CARTESIAN_POINT('Origin',(16.2754963537827,1076.73142393294,377.153097184802));
#126895=CARTESIAN_POINT('Origin',(16.2754963537827,1067.7251047501,377.153097184802));
#126896=CARTESIAN_POINT('',(16.2754963537827,1076.73142393294,376.132615142177));
#126897=CARTESIAN_POINT('Origin',(16.2754963537827,1076.73142393294,377.153097184802));
#126898=CARTESIAN_POINT('',(16.2754963537827,1082.7251047501,376.132615142177));
#126899=CARTESIAN_POINT('',(16.2754963537827,1067.7251047501,376.132615142177));
#126900=CARTESIAN_POINT('Origin',(16.2754963537827,1082.7251047501,377.153097184802));
#126901=CARTESIAN_POINT('Origin',(24.9269222653138,1067.7251047501,371.799460072343));
#126902=CARTESIAN_POINT('',(24.9269222653138,1078.73142393294,370.09845984926));
#126903=CARTESIAN_POINT('Origin',(24.9269222653138,1078.73142393294,371.799460072343));
#126904=CARTESIAN_POINT('',(24.9269222653138,1076.73142393294,370.09845984926));
#126905=CARTESIAN_POINT('',(24.9269222653138,1067.7251047501,370.09845984926));
#126906=CARTESIAN_POINT('Origin',(24.9269222653138,1076.73142393294,371.799460072343));
#126907=CARTESIAN_POINT('Origin',(24.9269222653138,1067.7251047501,371.799460072343));
#126908=CARTESIAN_POINT('',(24.9269222653138,1076.73142393294,370.69845984926));
#126909=CARTESIAN_POINT('Origin',(24.9269222653138,1076.73142393294,371.799460072343));
#126910=CARTESIAN_POINT('',(24.9269222653138,1082.7251047501,370.69845984926));
#126911=CARTESIAN_POINT('',(24.9269222653138,1067.7251047501,370.69845984926));
#126912=CARTESIAN_POINT('Origin',(24.9269222653138,1082.7251047501,371.799460072343));
#126913=CARTESIAN_POINT('Origin',(34.2787451288828,1067.7251047501,368.655907608726));
#126914=CARTESIAN_POINT('',(34.2787451288828,1078.73142393294,366.934632976682));
#126915=CARTESIAN_POINT('Origin',(34.2787451288828,1078.73142393294,368.655907608726));
#126916=CARTESIAN_POINT('',(34.2787451288828,1076.73142393294,366.934632976682));
#126917=CARTESIAN_POINT('',(34.2787451288828,1067.7251047501,366.934632976682));
#126918=CARTESIAN_POINT('Origin',(34.2787451288828,1076.73142393294,368.655907608726));
#126919=CARTESIAN_POINT('Origin',(34.2787451288828,1067.7251047501,368.655907608726));
#126920=CARTESIAN_POINT('',(34.2787451288828,1076.73142393294,367.534632976682));
#126921=CARTESIAN_POINT('Origin',(34.2787451288828,1076.73142393294,368.655907608726));
#126922=CARTESIAN_POINT('',(34.2787451288828,1082.7251047501,367.534632976682));
#126923=CARTESIAN_POINT('',(34.2787451288828,1067.7251047501,367.534632976682));
#126924=CARTESIAN_POINT('Origin',(34.2787451288828,1082.7251047501,368.655907608726));
#126925=CARTESIAN_POINT('Origin',(45.4179187734419,1067.7251047501,366.27608615121));
#126926=CARTESIAN_POINT('',(45.4179187734419,1078.73142393294,364.494093496805));
#126927=CARTESIAN_POINT('Origin',(45.4179187734419,1078.73142393294,366.27608615121));
#126928=CARTESIAN_POINT('',(45.4179187734419,1076.73142393294,364.494093496805));
#126929=CARTESIAN_POINT('',(45.4179187734419,1067.7251047501,364.494093496805));
#126930=CARTESIAN_POINT('Origin',(45.4179187734419,1076.73142393294,366.27608615121));
#126931=CARTESIAN_POINT('Origin',(45.4179187734419,1067.7251047501,366.27608615121));
#126932=CARTESIAN_POINT('',(45.4179187734419,1076.73142393294,365.094093496805));
#126933=CARTESIAN_POINT('Origin',(45.4179187734419,1076.73142393294,366.27608615121));
#126934=CARTESIAN_POINT('',(45.4179187734419,1082.7251047501,365.094093496805));
#126935=CARTESIAN_POINT('',(45.4179187734419,1067.7251047501,365.094093496805));
#126936=CARTESIAN_POINT('Origin',(45.4179187734419,1082.7251047501,366.27608615121));
#126937=CARTESIAN_POINT('Origin',(56.6398335662292,1067.7251047501,366.294032411781));
#126938=CARTESIAN_POINT('',(56.6398335662292,1078.73142393294,364.63315160186));
#126939=CARTESIAN_POINT('Origin',(56.6398335662292,1078.73142393294,366.294032411781));
#126940=CARTESIAN_POINT('',(56.6398335662292,1076.73142393294,364.63315160186));
#126941=CARTESIAN_POINT('',(56.6398335662292,1067.7251047501,364.63315160186));
#126942=CARTESIAN_POINT('Origin',(56.6398335662292,1076.73142393294,366.294032411781));
#126943=CARTESIAN_POINT('Origin',(56.6398335662292,1067.7251047501,366.294032411781));
#126944=CARTESIAN_POINT('',(56.6398335662292,1076.73142393294,365.23315160186));
#126945=CARTESIAN_POINT('Origin',(56.6398335662292,1076.73142393294,366.294032411781));
#126946=CARTESIAN_POINT('',(56.6398335662292,1082.7251047501,365.23315160186));
#126947=CARTESIAN_POINT('',(56.6398335662292,1067.7251047501,365.23315160186));
#126948=CARTESIAN_POINT('Origin',(56.6398335662292,1082.7251047501,366.294032411781));
#126949=CARTESIAN_POINT('Origin',(-5.81232974134926,1067.7251047501,406.345781068191));
#126950=CARTESIAN_POINT('',(-5.81232974134926,1078.73142393294,405.245423002516));
#126951=CARTESIAN_POINT('Origin',(-5.81232974134926,1078.73142393294,406.345781068191));
#126952=CARTESIAN_POINT('',(-5.81232974134926,1076.73142393294,405.245423002516));
#126953=CARTESIAN_POINT('',(-5.81232974134926,1067.7251047501,405.245423002516));
#126954=CARTESIAN_POINT('Origin',(-5.81232974134926,1076.73142393294,406.345781068191));
#126955=CARTESIAN_POINT('Origin',(-5.81232974134926,1067.7251047501,406.345781068191));
#126956=CARTESIAN_POINT('',(-5.81232974134926,1076.73142393294,405.845423002516));
#126957=CARTESIAN_POINT('Origin',(-5.81232974134926,1076.73142393294,406.345781068191));
#126958=CARTESIAN_POINT('',(-5.81232974134926,1082.7251047501,405.845423002516));
#126959=CARTESIAN_POINT('',(-5.81232974134926,1067.7251047501,405.845423002516));
#126960=CARTESIAN_POINT('Origin',(-5.81232974134926,1082.7251047501,406.345781068191));
#126961=CARTESIAN_POINT('Origin',(-5.5781548198755,1067.7251047501,397.785259330762));
#126962=CARTESIAN_POINT('',(-5.5781548198755,1078.73142393294,396.571227764025));
#126963=CARTESIAN_POINT('Origin',(-5.5781548198755,1078.73142393294,397.785259330762));
#126964=CARTESIAN_POINT('',(-5.5781548198755,1076.73142393294,396.571227764025));
#126965=CARTESIAN_POINT('',(-5.5781548198755,1067.7251047501,396.571227764025));
#126966=CARTESIAN_POINT('Origin',(-5.5781548198755,1076.73142393294,397.785259330762));
#126967=CARTESIAN_POINT('Origin',(-5.5781548198755,1067.7251047501,397.785259330762));
#126968=CARTESIAN_POINT('',(-5.5781548198755,1076.73142393294,397.171227764025));
#126969=CARTESIAN_POINT('Origin',(-5.5781548198755,1076.73142393294,397.785259330762));
#126970=CARTESIAN_POINT('',(-5.5781548198755,1082.7251047501,397.171227764025));
#126971=CARTESIAN_POINT('',(-5.5781548198755,1067.7251047501,397.171227764025));
#126972=CARTESIAN_POINT('Origin',(-5.5781548198755,1082.7251047501,397.785259330762));
#126973=CARTESIAN_POINT('Origin',(-3.45995919230213,1067.7251047501,390.147711491056));
#126974=CARTESIAN_POINT('',(-3.45995919230213,1078.73142393294,388.818903527483));
#126975=CARTESIAN_POINT('Origin',(-3.45995919230213,1078.73142393294,390.147711491056));
#126976=CARTESIAN_POINT('',(-3.45995919230213,1076.73142393294,388.818903527483));
#126977=CARTESIAN_POINT('',(-3.45995919230213,1067.7251047501,388.818903527483));
#126978=CARTESIAN_POINT('Origin',(-3.45995919230213,1076.73142393294,390.147711491056));
#126979=CARTESIAN_POINT('Origin',(-3.45995919230213,1067.7251047501,390.147711491056));
#126980=CARTESIAN_POINT('',(-3.45995919230213,1076.73142393294,389.418903527483));
#126981=CARTESIAN_POINT('Origin',(-3.45995919230213,1076.73142393294,390.147711491056));
#126982=CARTESIAN_POINT('',(-3.45995919230213,1082.7251047501,389.418903527483));
#126983=CARTESIAN_POINT('',(-3.45995919230213,1067.7251047501,389.418903527483));
#126984=CARTESIAN_POINT('Origin',(-3.45995919230213,1082.7251047501,390.147711491056));
#126985=CARTESIAN_POINT('Origin',(0.430140047742833,1067.7251047501,381.733463773809));
#126986=CARTESIAN_POINT('',(0.430140047742833,1078.73142393294,380.272346771993));
#126987=CARTESIAN_POINT('Origin',(0.430140047742833,1078.73142393294,381.733463773809));
#126988=CARTESIAN_POINT('',(0.430140047742833,1076.73142393294,380.272346771993));
#126989=CARTESIAN_POINT('',(0.430140047742833,1067.7251047501,380.272346771993));
#126990=CARTESIAN_POINT('Origin',(0.430140047742833,1076.73142393294,381.733463773809));
#126991=CARTESIAN_POINT('Origin',(0.430140047742833,1067.7251047501,381.733463773809));
#126992=CARTESIAN_POINT('',(0.430140047742833,1076.73142393294,380.872346771993));
#126993=CARTESIAN_POINT('Origin',(0.430140047742833,1076.73142393294,381.733463773809));
#126994=CARTESIAN_POINT('',(0.430140047742833,1082.7251047501,380.872346771993));
#126995=CARTESIAN_POINT('',(0.430140047742833,1067.7251047501,380.872346771993));
#126996=CARTESIAN_POINT('Origin',(0.430140047742833,1082.7251047501,381.733463773809));
#126997=CARTESIAN_POINT('Origin',(6.05086325182658,1067.7251047501,374.806502232188));
#126998=CARTESIAN_POINT('',(6.05086325182658,1078.73142393294,373.186020189563));
#126999=CARTESIAN_POINT('Origin',(6.05086325182658,1078.73142393294,374.806502232188));
#127000=CARTESIAN_POINT('',(6.05086325182658,1076.73142393294,373.186020189563));
#127001=CARTESIAN_POINT('',(6.05086325182658,1067.7251047501,373.186020189563));
#127002=CARTESIAN_POINT('Origin',(6.05086325182658,1076.73142393294,374.806502232188));
#127003=CARTESIAN_POINT('Origin',(6.05086325182658,1067.7251047501,374.806502232188));
#127004=CARTESIAN_POINT('',(6.05086325182658,1076.73142393294,373.786020189563));
#127005=CARTESIAN_POINT('Origin',(6.05086325182658,1076.73142393294,374.806502232188));
#127006=CARTESIAN_POINT('',(6.05086325182658,1082.7251047501,373.786020189563));
#127007=CARTESIAN_POINT('',(6.05086325182658,1067.7251047501,373.786020189563));
#127008=CARTESIAN_POINT('Origin',(6.05086325182658,1082.7251047501,374.806502232188));
#127009=CARTESIAN_POINT('Origin',(13.4001510060409,1067.7251047501,367.771122346186));
#127010=CARTESIAN_POINT('',(13.4001510060409,1078.73142393294,366.070122123103));
#127011=CARTESIAN_POINT('Origin',(13.4001510060409,1078.73142393294,367.771122346186));
#127012=CARTESIAN_POINT('',(13.4001510060409,1076.73142393294,366.070122123103));
#127013=CARTESIAN_POINT('',(13.4001510060409,1067.7251047501,366.070122123103));
#127014=CARTESIAN_POINT('Origin',(13.4001510060409,1076.73142393294,367.771122346186));
#127015=CARTESIAN_POINT('Origin',(13.4001510060409,1067.7251047501,367.771122346186));
#127016=CARTESIAN_POINT('',(13.4001510060409,1076.73142393294,366.670122123103));
#127017=CARTESIAN_POINT('Origin',(13.4001510060409,1076.73142393294,367.771122346186));
#127018=CARTESIAN_POINT('',(13.4001510060409,1082.7251047501,366.670122123103));
#127019=CARTESIAN_POINT('',(13.4001510060409,1067.7251047501,366.670122123103));
#127020=CARTESIAN_POINT('Origin',(13.4001510060409,1082.7251047501,367.771122346186));
#127021=CARTESIAN_POINT('Origin',(21.8940327946435,1067.7251047501,362.751910742325));
#127022=CARTESIAN_POINT('',(21.8940327946435,1078.73142393294,361.030636110281));
#127023=CARTESIAN_POINT('Origin',(21.8940327946435,1078.73142393294,362.751910742325));
#127024=CARTESIAN_POINT('',(21.8940327946435,1076.73142393294,361.030636110281));
#127025=CARTESIAN_POINT('',(21.8940327946435,1067.7251047501,361.030636110281));
#127026=CARTESIAN_POINT('Origin',(21.8940327946435,1076.73142393294,362.751910742325));
#127027=CARTESIAN_POINT('Origin',(21.8940327946435,1067.7251047501,362.751910742325));
#127028=CARTESIAN_POINT('',(21.8940327946435,1076.73142393294,361.630636110281));
#127029=CARTESIAN_POINT('Origin',(21.8940327946435,1076.73142393294,362.751910742325));
#127030=CARTESIAN_POINT('',(21.8940327946435,1082.7251047501,361.630636110281));
#127031=CARTESIAN_POINT('',(21.8940327946435,1067.7251047501,361.630636110281));
#127032=CARTESIAN_POINT('Origin',(21.8940327946435,1082.7251047501,362.751910742325));
#127033=CARTESIAN_POINT('Origin',(32.2949960661498,1067.7251047501,358.108129666728));
#127034=CARTESIAN_POINT('',(32.2949960661498,1078.73142393294,356.326137012323));
#127035=CARTESIAN_POINT('Origin',(32.2949960661498,1078.73142393294,358.108129666728));
#127036=CARTESIAN_POINT('',(32.2949960661498,1076.73142393294,356.326137012323));
#127037=CARTESIAN_POINT('',(32.2949960661498,1067.7251047501,356.326137012323));
#127038=CARTESIAN_POINT('Origin',(32.2949960661498,1076.73142393294,358.108129666728));
#127039=CARTESIAN_POINT('Origin',(32.2949960661498,1067.7251047501,358.108129666728));
#127040=CARTESIAN_POINT('',(32.2949960661498,1076.73142393294,356.926137012323));
#127041=CARTESIAN_POINT('Origin',(32.2949960661498,1076.73142393294,358.108129666728));
#127042=CARTESIAN_POINT('',(32.2949960661498,1082.7251047501,356.926137012323));
#127043=CARTESIAN_POINT('',(32.2949960661498,1067.7251047501,356.926137012323));
#127044=CARTESIAN_POINT('Origin',(32.2949960661498,1082.7251047501,358.108129666728));
#127045=CARTESIAN_POINT('Origin',(43.2754163337329,1067.7251047501,355.792516479666));
#127046=CARTESIAN_POINT('',(43.2754163337329,1078.73142393294,354.131635669746));
#127047=CARTESIAN_POINT('Origin',(43.2754163337329,1078.73142393294,355.792516479666));
#127048=CARTESIAN_POINT('',(43.2754163337329,1076.73142393294,354.131635669746));
#127049=CARTESIAN_POINT('',(43.2754163337329,1067.7251047501,354.131635669746));
#127050=CARTESIAN_POINT('Origin',(43.2754163337329,1076.73142393294,355.792516479666));
#127051=CARTESIAN_POINT('Origin',(43.2754163337329,1067.7251047501,355.792516479666));
#127052=CARTESIAN_POINT('',(43.2754163337329,1076.73142393294,354.731635669746));
#127053=CARTESIAN_POINT('Origin',(43.2754163337329,1076.73142393294,355.792516479666));
#127054=CARTESIAN_POINT('',(43.2754163337329,1082.7251047501,354.731635669746));
#127055=CARTESIAN_POINT('',(43.2754163337329,1067.7251047501,354.731635669746));
#127056=CARTESIAN_POINT('Origin',(43.2754163337329,1082.7251047501,355.792516479666));
#127057=CARTESIAN_POINT('Origin',(-9.48479058284857,1067.7251047501,407.953573201632));
#127058=CARTESIAN_POINT('',(-9.48479058284857,1078.73142393294,406.853215135958));
#127059=CARTESIAN_POINT('Origin',(-9.48479058284857,1078.73142393294,407.953573201632));
#127060=CARTESIAN_POINT('',(-9.48479058284857,1076.73142393294,406.853215135958));
#127061=CARTESIAN_POINT('',(-9.48479058284857,1067.7251047501,406.853215135958));
#127062=CARTESIAN_POINT('Origin',(-9.48479058284857,1076.73142393294,407.953573201632));
#127063=CARTESIAN_POINT('Origin',(-9.48479058284857,1067.7251047501,407.953573201632));
#127064=CARTESIAN_POINT('',(-9.48479058284857,1076.73142393294,407.453215135958));
#127065=CARTESIAN_POINT('Origin',(-9.48479058284857,1076.73142393294,407.953573201632));
#127066=CARTESIAN_POINT('',(-9.48479058284857,1082.7251047501,407.453215135958));
#127067=CARTESIAN_POINT('',(-9.48479058284857,1067.7251047501,407.453215135958));
#127068=CARTESIAN_POINT('Origin',(-9.48479058284857,1082.7251047501,407.953573201632));
#127069=CARTESIAN_POINT('Origin',(-11.0355654939679,1067.7251047501,399.531431699266));
#127070=CARTESIAN_POINT('',(-11.0355654939679,1078.73142393294,398.317400132529));
#127071=CARTESIAN_POINT('Origin',(-11.0355654939679,1078.73142393294,399.531431699266));
#127072=CARTESIAN_POINT('',(-11.0355654939679,1076.73142393294,398.317400132529));
#127073=CARTESIAN_POINT('',(-11.0355654939679,1067.7251047501,398.317400132529));
#127074=CARTESIAN_POINT('Origin',(-11.0355654939679,1076.73142393294,399.531431699266));
#127075=CARTESIAN_POINT('Origin',(-11.0355654939679,1067.7251047501,399.531431699266));
#127076=CARTESIAN_POINT('',(-11.0355654939679,1076.73142393294,398.917400132529));
#127077=CARTESIAN_POINT('Origin',(-11.0355654939679,1076.73142393294,399.531431699266));
#127078=CARTESIAN_POINT('',(-11.0355654939679,1082.7251047501,398.917400132529));
#127079=CARTESIAN_POINT('',(-11.0355654939679,1067.7251047501,398.917400132529));
#127080=CARTESIAN_POINT('Origin',(-11.0355654939679,1082.7251047501,399.531431699266));
#127081=CARTESIAN_POINT('Origin',(-10.5515930080269,1067.7251047501,391.620384969957));
#127082=CARTESIAN_POINT('',(-10.5515930080269,1078.73142393294,390.291577006384));
#127083=CARTESIAN_POINT('Origin',(-10.5515930080269,1078.73142393294,391.620384969957));
#127084=CARTESIAN_POINT('',(-10.5515930080269,1076.73142393294,390.291577006384));
#127085=CARTESIAN_POINT('',(-10.5515930080269,1067.7251047501,390.291577006384));
#127086=CARTESIAN_POINT('Origin',(-10.5515930080269,1076.73142393294,391.620384969957));
#127087=CARTESIAN_POINT('Origin',(-10.5515930080269,1067.7251047501,391.620384969957));
#127088=CARTESIAN_POINT('',(-10.5515930080269,1076.73142393294,390.891577006384));
#127089=CARTESIAN_POINT('Origin',(-10.5515930080269,1076.73142393294,391.620384969957));
#127090=CARTESIAN_POINT('',(-10.5515930080269,1082.7251047501,390.891577006384));
#127091=CARTESIAN_POINT('',(-10.5515930080269,1067.7251047501,390.891577006384));
#127092=CARTESIAN_POINT('Origin',(-10.5515930080269,1082.7251047501,391.620384969957));
#127093=CARTESIAN_POINT('Origin',(-8.49592223961282,1067.7251047501,382.581211642906));
#127094=CARTESIAN_POINT('',(-8.49592223961282,1078.73142393294,381.120094641089));
#127095=CARTESIAN_POINT('Origin',(-8.49592223961282,1078.73142393294,382.581211642906));
#127096=CARTESIAN_POINT('',(-8.49592223961282,1076.73142393294,381.120094641089));
#127097=CARTESIAN_POINT('',(-8.49592223961282,1067.7251047501,381.120094641089));
#127098=CARTESIAN_POINT('Origin',(-8.49592223961282,1076.73142393294,382.581211642906));
#127099=CARTESIAN_POINT('Origin',(-8.49592223961282,1067.7251047501,382.581211642906));
#127100=CARTESIAN_POINT('',(-8.49592223961282,1076.73142393294,381.720094641089));
#127101=CARTESIAN_POINT('Origin',(-8.49592223961282,1076.73142393294,382.581211642906));
#127102=CARTESIAN_POINT('',(-8.49592223961282,1082.7251047501,381.720094641089));
#127103=CARTESIAN_POINT('',(-8.49592223961282,1067.7251047501,381.720094641089));
#127104=CARTESIAN_POINT('Origin',(-8.49592223961282,1082.7251047501,382.581211642906));
#127105=CARTESIAN_POINT('Origin',(-4.43822160949764,1067.7251047501,374.637006765614));
#127106=CARTESIAN_POINT('',(-4.43822160949764,1078.73142393294,373.016524722989));
#127107=CARTESIAN_POINT('Origin',(-4.43822160949764,1078.73142393294,374.637006765614));
#127108=CARTESIAN_POINT('',(-4.43822160949764,1076.73142393294,373.016524722989));
#127109=CARTESIAN_POINT('',(-4.43822160949764,1067.7251047501,373.016524722989));
#127110=CARTESIAN_POINT('Origin',(-4.43822160949764,1076.73142393294,374.637006765614));
#127111=CARTESIAN_POINT('Origin',(-4.43822160949764,1067.7251047501,374.637006765614));
#127112=CARTESIAN_POINT('',(-4.43822160949764,1076.73142393294,373.616524722989));
#127113=CARTESIAN_POINT('Origin',(-4.43822160949764,1076.73142393294,374.637006765614));
#127114=CARTESIAN_POINT('',(-4.43822160949764,1082.7251047501,373.616524722989));
#127115=CARTESIAN_POINT('',(-4.43822160949764,1067.7251047501,373.616524722989));
#127116=CARTESIAN_POINT('Origin',(-4.43822160949764,1082.7251047501,374.637006765614));
#127117=CARTESIAN_POINT('Origin',(1.28772884674538,1067.7251047501,366.227363966584));
#127118=CARTESIAN_POINT('',(1.28772884674538,1078.73142393294,364.526363743502));
#127119=CARTESIAN_POINT('Origin',(1.28772884674538,1078.73142393294,366.227363966584));
#127120=CARTESIAN_POINT('',(1.28772884674538,1076.73142393294,364.526363743502));
#127121=CARTESIAN_POINT('',(1.28772884674538,1067.7251047501,364.526363743502));
#127122=CARTESIAN_POINT('Origin',(1.28772884674538,1076.73142393294,366.227363966584));
#127123=CARTESIAN_POINT('Origin',(1.28772884674538,1067.7251047501,366.227363966584));
#127124=CARTESIAN_POINT('',(1.28772884674538,1076.73142393294,365.126363743502));
#127125=CARTESIAN_POINT('Origin',(1.28772884674538,1076.73142393294,366.227363966584));
#127126=CARTESIAN_POINT('',(1.28772884674538,1082.7251047501,365.126363743502));
#127127=CARTESIAN_POINT('',(1.28772884674538,1067.7251047501,365.126363743502));
#127128=CARTESIAN_POINT('Origin',(1.28772884674538,1082.7251047501,366.227363966584));
#127129=CARTESIAN_POINT('Origin',(8.55244616805279,1067.7251047501,359.551856854418));
#127130=CARTESIAN_POINT('',(8.55244616805279,1078.73142393294,357.830582222375));
#127131=CARTESIAN_POINT('Origin',(8.55244616805279,1078.73142393294,359.551856854418));
#127132=CARTESIAN_POINT('',(8.55244616805279,1076.73142393294,357.830582222375));
#127133=CARTESIAN_POINT('',(8.55244616805279,1067.7251047501,357.830582222375));
#127134=CARTESIAN_POINT('Origin',(8.55244616805279,1076.73142393294,359.551856854418));
#127135=CARTESIAN_POINT('Origin',(8.55244616805279,1067.7251047501,359.551856854418));
#127136=CARTESIAN_POINT('',(8.55244616805279,1076.73142393294,358.430582222375));
#127137=CARTESIAN_POINT('Origin',(8.55244616805279,1076.73142393294,359.551856854418));
#127138=CARTESIAN_POINT('',(8.55244616805279,1082.7251047501,358.430582222375));
#127139=CARTESIAN_POINT('',(8.55244616805279,1067.7251047501,358.430582222375));
#127140=CARTESIAN_POINT('Origin',(8.55244616805279,1082.7251047501,359.551856854418));
#127141=CARTESIAN_POINT('Origin',(17.7606270621823,1067.7251047501,352.847071677078));
#127142=CARTESIAN_POINT('',(17.7606270621823,1078.73142393294,351.065079022673));
#127143=CARTESIAN_POINT('Origin',(17.7606270621823,1078.73142393294,352.847071677078));
#127144=CARTESIAN_POINT('',(17.7606270621823,1076.73142393294,351.065079022673));
#127145=CARTESIAN_POINT('',(17.7606270621823,1067.7251047501,351.065079022673));
#127146=CARTESIAN_POINT('Origin',(17.7606270621823,1076.73142393294,352.847071677078));
#127147=CARTESIAN_POINT('Origin',(17.7606270621823,1067.7251047501,352.847071677078));
#127148=CARTESIAN_POINT('',(17.7606270621823,1076.73142393294,351.665079022673));
#127149=CARTESIAN_POINT('Origin',(17.7606270621823,1076.73142393294,352.847071677078));
#127150=CARTESIAN_POINT('',(17.7606270621823,1082.7251047501,351.665079022673));
#127151=CARTESIAN_POINT('',(17.7606270621823,1067.7251047501,351.665079022673));
#127152=CARTESIAN_POINT('Origin',(17.7606270621823,1082.7251047501,352.847071677078));
#127153=CARTESIAN_POINT('Origin',(28.0196557489657,1067.7251047501,348.299102450203));
#127154=CARTESIAN_POINT('',(28.0196557489657,1078.73142393294,346.638221640282));
#127155=CARTESIAN_POINT('Origin',(28.0196557489657,1078.73142393294,348.299102450203));
#127156=CARTESIAN_POINT('',(28.0196557489657,1076.73142393294,346.638221640282));
#127157=CARTESIAN_POINT('',(28.0196557489657,1067.7251047501,346.638221640282));
#127158=CARTESIAN_POINT('Origin',(28.0196557489657,1076.73142393294,348.299102450203));
#127159=CARTESIAN_POINT('Origin',(28.0196557489657,1067.7251047501,348.299102450203));
#127160=CARTESIAN_POINT('',(28.0196557489657,1076.73142393294,347.238221640282));
#127161=CARTESIAN_POINT('Origin',(28.0196557489657,1076.73142393294,348.299102450203));
#127162=CARTESIAN_POINT('',(28.0196557489657,1082.7251047501,347.238221640282));
#127163=CARTESIAN_POINT('',(28.0196557489657,1067.7251047501,347.238221640282));
#127164=CARTESIAN_POINT('Origin',(28.0196557489657,1082.7251047501,348.299102450203));
#127165=CARTESIAN_POINT('Origin',(-12.7427205628026,1067.7251047501,410.289778762456));
#127166=CARTESIAN_POINT('',(-12.7427205628026,1078.73142393294,409.189420696781));
#127167=CARTESIAN_POINT('Origin',(-12.7427205628026,1078.73142393294,410.289778762456));
#127168=CARTESIAN_POINT('',(-12.7427205628026,1076.73142393294,409.189420696781));
#127169=CARTESIAN_POINT('',(-12.7427205628026,1067.7251047501,409.189420696781));
#127170=CARTESIAN_POINT('Origin',(-12.7427205628026,1076.73142393294,410.289778762456));
#127171=CARTESIAN_POINT('Origin',(-12.7427205628026,1067.7251047501,410.289778762456));
#127172=CARTESIAN_POINT('',(-12.7427205628026,1076.73142393294,409.789420696781));
#127173=CARTESIAN_POINT('Origin',(-12.7427205628026,1076.73142393294,410.289778762456));
#127174=CARTESIAN_POINT('',(-12.7427205628026,1082.7251047501,409.789420696781));
#127175=CARTESIAN_POINT('',(-12.7427205628026,1067.7251047501,409.789420696781));
#127176=CARTESIAN_POINT('Origin',(-12.7427205628026,1082.7251047501,410.289778762456));
#127177=CARTESIAN_POINT('Origin',(-16.0106690014555,1067.7251047501,402.374105492724));
#127178=CARTESIAN_POINT('',(-16.0106690014555,1078.73142393294,401.160073925987));
#127179=CARTESIAN_POINT('Origin',(-16.0106690014555,1078.73142393294,402.374105492724));
#127180=CARTESIAN_POINT('',(-16.0106690014555,1076.73142393294,401.160073925987));
#127181=CARTESIAN_POINT('',(-16.0106690014555,1067.7251047501,401.160073925987));
#127182=CARTESIAN_POINT('Origin',(-16.0106690014555,1076.73142393294,402.374105492724));
#127183=CARTESIAN_POINT('Origin',(-16.0106690014555,1067.7251047501,402.374105492724));
#127184=CARTESIAN_POINT('',(-16.0106690014555,1076.73142393294,401.760073925987));
#127185=CARTESIAN_POINT('Origin',(-16.0106690014555,1076.73142393294,402.374105492724));
#127186=CARTESIAN_POINT('',(-16.0106690014555,1082.7251047501,401.760073925987));
#127187=CARTESIAN_POINT('',(-16.0106690014555,1067.7251047501,401.760073925987));
#127188=CARTESIAN_POINT('Origin',(-16.0106690014555,1082.7251047501,402.374105492724));
#127189=CARTESIAN_POINT('Origin',(-17.1820715771402,1067.7251047501,394.535310577296));
#127190=CARTESIAN_POINT('',(-17.1820715771402,1078.73142393294,393.206502613723));
#127191=CARTESIAN_POINT('Origin',(-17.1820715771402,1078.73142393294,394.535310577296));
#127192=CARTESIAN_POINT('',(-17.1820715771402,1076.73142393294,393.206502613723));
#127193=CARTESIAN_POINT('',(-17.1820715771402,1067.7251047501,393.206502613723));
#127194=CARTESIAN_POINT('Origin',(-17.1820715771402,1076.73142393294,394.535310577296));
#127195=CARTESIAN_POINT('Origin',(-17.1820715771402,1067.7251047501,394.535310577296));
#127196=CARTESIAN_POINT('',(-17.1820715771402,1076.73142393294,393.806502613723));
#127197=CARTESIAN_POINT('Origin',(-17.1820715771402,1076.73142393294,394.535310577296));
#127198=CARTESIAN_POINT('',(-17.1820715771402,1082.7251047501,393.806502613723));
#127199=CARTESIAN_POINT('',(-17.1820715771402,1067.7251047501,393.806502613723));
#127200=CARTESIAN_POINT('Origin',(-17.1820715771402,1082.7251047501,394.535310577296));
#127201=CARTESIAN_POINT('Origin',(-17.0506719571394,1067.7251047501,385.266266889598));
#127202=CARTESIAN_POINT('',(-17.0506719571394,1078.73142393294,383.805149887781));
#127203=CARTESIAN_POINT('Origin',(-17.0506719571394,1078.73142393294,385.266266889598));
#127204=CARTESIAN_POINT('',(-17.0506719571394,1076.73142393294,383.805149887781));
#127205=CARTESIAN_POINT('',(-17.0506719571394,1067.7251047501,383.805149887781));
#127206=CARTESIAN_POINT('Origin',(-17.0506719571394,1076.73142393294,385.266266889598));
#127207=CARTESIAN_POINT('Origin',(-17.0506719571394,1067.7251047501,385.266266889598));
#127208=CARTESIAN_POINT('',(-17.0506719571394,1076.73142393294,384.405149887781));
#127209=CARTESIAN_POINT('Origin',(-17.0506719571394,1076.73142393294,385.266266889598));
#127210=CARTESIAN_POINT('',(-17.0506719571394,1082.7251047501,384.405149887781));
#127211=CARTESIAN_POINT('',(-17.0506719571394,1067.7251047501,384.405149887781));
#127212=CARTESIAN_POINT('Origin',(-17.0506719571394,1082.7251047501,385.266266889598));
#127213=CARTESIAN_POINT('Origin',(-14.7333348895366,1067.7251047501,376.652018550297));
#127214=CARTESIAN_POINT('',(-14.7333348895366,1078.73142393294,375.031536507673));
#127215=CARTESIAN_POINT('Origin',(-14.7333348895366,1078.73142393294,376.652018550297));
#127216=CARTESIAN_POINT('',(-14.7333348895366,1076.73142393294,375.031536507673));
#127217=CARTESIAN_POINT('',(-14.7333348895366,1067.7251047501,375.031536507673));
#127218=CARTESIAN_POINT('Origin',(-14.7333348895366,1076.73142393294,376.652018550297));
#127219=CARTESIAN_POINT('Origin',(-14.7333348895366,1067.7251047501,376.652018550297));
#127220=CARTESIAN_POINT('',(-14.7333348895366,1076.73142393294,375.631536507673));
#127221=CARTESIAN_POINT('Origin',(-14.7333348895366,1076.73142393294,376.652018550297));
#127222=CARTESIAN_POINT('',(-14.7333348895366,1082.7251047501,375.631536507673));
#127223=CARTESIAN_POINT('',(-14.7333348895366,1067.7251047501,375.631536507673));
#127224=CARTESIAN_POINT('Origin',(-14.7333348895366,1082.7251047501,376.652018550297));
#127225=CARTESIAN_POINT('Origin',(-10.8809732423614,1067.7251047501,367.235654582502));
#127226=CARTESIAN_POINT('',(-10.8809732423614,1078.73142393294,365.53465435942));
#127227=CARTESIAN_POINT('Origin',(-10.8809732423614,1078.73142393294,367.235654582502));
#127228=CARTESIAN_POINT('',(-10.8809732423614,1076.73142393294,365.53465435942));
#127229=CARTESIAN_POINT('',(-10.8809732423614,1067.7251047501,365.53465435942));
#127230=CARTESIAN_POINT('Origin',(-10.8809732423614,1076.73142393294,367.235654582502));
#127231=CARTESIAN_POINT('Origin',(-10.8809732423614,1067.7251047501,367.235654582502));
#127232=CARTESIAN_POINT('',(-10.8809732423614,1076.73142393294,366.13465435942));
#127233=CARTESIAN_POINT('Origin',(-10.8809732423614,1076.73142393294,367.235654582502));
#127234=CARTESIAN_POINT('',(-10.8809732423614,1082.7251047501,366.13465435942));
#127235=CARTESIAN_POINT('',(-10.8809732423614,1067.7251047501,366.13465435942));
#127236=CARTESIAN_POINT('Origin',(-10.8809732423614,1082.7251047501,367.235654582502));
#127237=CARTESIAN_POINT('Origin',(-5.16292339527169,1067.7251047501,359.19560365547));
#127238=CARTESIAN_POINT('',(-5.16292339527169,1078.73142393294,357.474329023426));
#127239=CARTESIAN_POINT('Origin',(-5.16292339527169,1078.73142393294,359.19560365547));
#127240=CARTESIAN_POINT('',(-5.16292339527169,1076.73142393294,357.474329023426));
#127241=CARTESIAN_POINT('',(-5.16292339527169,1067.7251047501,357.474329023426));
#127242=CARTESIAN_POINT('Origin',(-5.16292339527169,1076.73142393294,359.19560365547));
#127243=CARTESIAN_POINT('Origin',(-5.16292339527169,1067.7251047501,359.19560365547));
#127244=CARTESIAN_POINT('',(-5.16292339527169,1076.73142393294,358.074329023426));
#127245=CARTESIAN_POINT('Origin',(-5.16292339527169,1076.73142393294,359.19560365547));
#127246=CARTESIAN_POINT('',(-5.16292339527169,1082.7251047501,358.074329023426));
#127247=CARTESIAN_POINT('',(-5.16292339527169,1067.7251047501,358.074329023426));
#127248=CARTESIAN_POINT('Origin',(-5.16292339527169,1082.7251047501,359.19560365547));
#127249=CARTESIAN_POINT('Origin',(2.45003343065336,1067.7251047501,350.722845661765));
#127250=CARTESIAN_POINT('',(2.45003343065336,1078.73142393294,348.94085300736));
#127251=CARTESIAN_POINT('Origin',(2.45003343065336,1078.73142393294,350.722845661765));
#127252=CARTESIAN_POINT('',(2.45003343065336,1076.73142393294,348.94085300736));
#127253=CARTESIAN_POINT('',(2.45003343065336,1067.7251047501,348.94085300736));
#127254=CARTESIAN_POINT('Origin',(2.45003343065336,1076.73142393294,350.722845661765));
#127255=CARTESIAN_POINT('Origin',(2.45003343065336,1067.7251047501,350.722845661765));
#127256=CARTESIAN_POINT('',(2.45003343065336,1076.73142393294,349.54085300736));
#127257=CARTESIAN_POINT('Origin',(2.45003343065336,1076.73142393294,350.722845661765));
#127258=CARTESIAN_POINT('',(2.45003343065336,1082.7251047501,349.54085300736));
#127259=CARTESIAN_POINT('',(2.45003343065336,1067.7251047501,349.54085300736));
#127260=CARTESIAN_POINT('Origin',(2.45003343065336,1082.7251047501,350.722845661765));
#127261=CARTESIAN_POINT('Origin',(11.539301754743,1067.7251047501,344.141288473869));
#127262=CARTESIAN_POINT('',(11.539301754743,1078.73142393294,342.480407663948));
#127263=CARTESIAN_POINT('Origin',(11.539301754743,1078.73142393294,344.141288473869));
#127264=CARTESIAN_POINT('',(11.539301754743,1076.73142393294,342.480407663948));
#127265=CARTESIAN_POINT('',(11.539301754743,1067.7251047501,342.480407663948));
#127266=CARTESIAN_POINT('Origin',(11.539301754743,1076.73142393294,344.141288473869));
#127267=CARTESIAN_POINT('Origin',(11.539301754743,1067.7251047501,344.141288473869));
#127268=CARTESIAN_POINT('',(11.539301754743,1076.73142393294,343.080407663948));
#127269=CARTESIAN_POINT('Origin',(11.539301754743,1076.73142393294,344.141288473869));
#127270=CARTESIAN_POINT('',(11.539301754743,1082.7251047501,343.080407663948));
#127271=CARTESIAN_POINT('',(11.539301754743,1067.7251047501,343.080407663948));
#127272=CARTESIAN_POINT('Origin',(11.539301754743,1082.7251047501,344.141288473869));
#127273=CARTESIAN_POINT('Origin',(-15.4437325078047,1067.7251047501,413.252294357294));
#127274=CARTESIAN_POINT('',(-15.4437325078047,1078.73142393294,412.151936291619));
#127275=CARTESIAN_POINT('Origin',(-15.4437325078047,1078.73142393294,413.252294357294));
#127276=CARTESIAN_POINT('',(-15.4437325078047,1076.73142393294,412.151936291619));
#127277=CARTESIAN_POINT('',(-15.4437325078047,1067.7251047501,412.151936291619));
#127278=CARTESIAN_POINT('Origin',(-15.4437325078047,1076.73142393294,413.252294357294));
#127279=CARTESIAN_POINT('Origin',(-15.4437325078047,1067.7251047501,413.252294357294));
#127280=CARTESIAN_POINT('',(-15.4437325078047,1076.73142393294,412.751936291619));
#127281=CARTESIAN_POINT('Origin',(-15.4437325078047,1076.73142393294,413.252294357294));
#127282=CARTESIAN_POINT('',(-15.4437325078047,1082.7251047501,412.751936291619));
#127283=CARTESIAN_POINT('',(-15.4437325078047,1067.7251047501,412.751936291619));
#127284=CARTESIAN_POINT('Origin',(-15.4437325078047,1082.7251047501,413.252294357294));
#127285=CARTESIAN_POINT('Origin',(-20.2860294458657,1067.7251047501,406.189042225699));
#127286=CARTESIAN_POINT('',(-20.2860294458657,1078.73142393294,404.975010658962));
#127287=CARTESIAN_POINT('Origin',(-20.2860294458657,1078.73142393294,406.189042225699));
#127288=CARTESIAN_POINT('',(-20.2860294458657,1076.73142393294,404.975010658962));
#127289=CARTESIAN_POINT('',(-20.2860294458657,1067.7251047501,404.975010658962));
#127290=CARTESIAN_POINT('Origin',(-20.2860294458657,1076.73142393294,406.189042225699));
#127291=CARTESIAN_POINT('Origin',(-20.2860294458657,1067.7251047501,406.189042225699));
#127292=CARTESIAN_POINT('',(-20.2860294458657,1076.73142393294,405.575010658962));
#127293=CARTESIAN_POINT('Origin',(-20.2860294458657,1076.73142393294,406.189042225699));
#127294=CARTESIAN_POINT('',(-20.2860294458657,1082.7251047501,405.575010658962));
#127295=CARTESIAN_POINT('',(-20.2860294458657,1067.7251047501,405.575010658962));
#127296=CARTESIAN_POINT('Origin',(-20.2860294458657,1082.7251047501,406.189042225699));
#127297=CARTESIAN_POINT('Origin',(-23.0616111696053,1067.7251047501,398.765092076667));
#127298=CARTESIAN_POINT('',(-23.0616111696053,1078.73142393294,397.436284113094));
#127299=CARTESIAN_POINT('Origin',(-23.0616111696053,1078.73142393294,398.765092076667));
#127300=CARTESIAN_POINT('',(-23.0616111696053,1076.73142393294,397.436284113094));
#127301=CARTESIAN_POINT('',(-23.0616111696053,1067.7251047501,397.436284113094));
#127302=CARTESIAN_POINT('Origin',(-23.0616111696053,1076.73142393294,398.765092076667));
#127303=CARTESIAN_POINT('Origin',(-23.0616111696053,1067.7251047501,398.765092076667));
#127304=CARTESIAN_POINT('',(-23.0616111696053,1076.73142393294,398.036284113094));
#127305=CARTESIAN_POINT('Origin',(-23.0616111696053,1076.73142393294,398.765092076667));
#127306=CARTESIAN_POINT('',(-23.0616111696053,1082.7251047501,398.036284113094));
#127307=CARTESIAN_POINT('',(-23.0616111696053,1067.7251047501,398.036284113094));
#127308=CARTESIAN_POINT('Origin',(-23.0616111696053,1082.7251047501,398.765092076667));
#127309=CARTESIAN_POINT('Origin',(-24.8602254919372,1067.7251047501,389.671279715281));
#127310=CARTESIAN_POINT('',(-24.8602254919372,1078.73142393294,388.210162713464));
#127311=CARTESIAN_POINT('Origin',(-24.8602254919372,1078.73142393294,389.671279715281));
#127312=CARTESIAN_POINT('',(-24.8602254919372,1076.73142393294,388.210162713464));
#127313=CARTESIAN_POINT('',(-24.8602254919372,1067.7251047501,388.210162713464));
#127314=CARTESIAN_POINT('Origin',(-24.8602254919372,1076.73142393294,389.671279715281));
#127315=CARTESIAN_POINT('Origin',(-24.8602254919372,1067.7251047501,389.671279715281));
#127316=CARTESIAN_POINT('',(-24.8602254919372,1076.73142393294,388.810162713464));
#127317=CARTESIAN_POINT('Origin',(-24.8602254919372,1076.73142393294,389.671279715281));
#127318=CARTESIAN_POINT('',(-24.8602254919372,1082.7251047501,388.810162713464));
#127319=CARTESIAN_POINT('',(-24.8602254919372,1067.7251047501,388.810162713464));
#127320=CARTESIAN_POINT('Origin',(-24.8602254919372,1082.7251047501,389.671279715281));
#127321=CARTESIAN_POINT('Origin',(-24.3845307365182,1067.7251047501,380.763471902149));
#127322=CARTESIAN_POINT('',(-24.3845307365182,1078.73142393294,379.142989859525));
#127323=CARTESIAN_POINT('Origin',(-24.3845307365182,1078.73142393294,380.763471902149));
#127324=CARTESIAN_POINT('',(-24.3845307365182,1076.73142393294,379.142989859525));
#127325=CARTESIAN_POINT('',(-24.3845307365182,1067.7251047501,379.142989859525));
#127326=CARTESIAN_POINT('Origin',(-24.3845307365182,1076.73142393294,380.763471902149));
#127327=CARTESIAN_POINT('Origin',(-24.3845307365182,1067.7251047501,380.763471902149));
#127328=CARTESIAN_POINT('',(-24.3845307365182,1076.73142393294,379.742989859525));
#127329=CARTESIAN_POINT('Origin',(-24.3845307365182,1076.73142393294,380.763471902149));
#127330=CARTESIAN_POINT('',(-24.3845307365182,1082.7251047501,379.742989859525));
#127331=CARTESIAN_POINT('',(-24.3845307365182,1067.7251047501,379.742989859525));
#127332=CARTESIAN_POINT('Origin',(-24.3845307365182,1082.7251047501,380.763471902149));
#127333=CARTESIAN_POINT('Origin',(-22.5741245880745,1067.7251047501,370.751927055709));
#127334=CARTESIAN_POINT('',(-22.5741245880745,1078.73142393294,369.050926832626));
#127335=CARTESIAN_POINT('Origin',(-22.5741245880745,1078.73142393294,370.751927055709));
#127336=CARTESIAN_POINT('',(-22.5741245880745,1076.73142393294,369.050926832626));
#127337=CARTESIAN_POINT('',(-22.5741245880745,1067.7251047501,369.050926832626));
#127338=CARTESIAN_POINT('Origin',(-22.5741245880745,1076.73142393294,370.751927055709));
#127339=CARTESIAN_POINT('Origin',(-22.5741245880745,1067.7251047501,370.751927055709));
#127340=CARTESIAN_POINT('',(-22.5741245880745,1076.73142393294,369.650926832626));
#127341=CARTESIAN_POINT('Origin',(-22.5741245880745,1076.73142393294,370.751927055709));
#127342=CARTESIAN_POINT('',(-22.5741245880745,1082.7251047501,369.650926832626));
#127343=CARTESIAN_POINT('',(-22.5741245880745,1067.7251047501,369.650926832626));
#127344=CARTESIAN_POINT('Origin',(-22.5741245880745,1082.7251047501,370.751927055709));
#127345=CARTESIAN_POINT('Origin',(-18.6526484317677,1067.7251047501,361.698721119765));
#127346=CARTESIAN_POINT('',(-18.6526484317677,1078.73142393294,359.977446487722));
#127347=CARTESIAN_POINT('Origin',(-18.6526484317677,1078.73142393294,361.698721119765));
#127348=CARTESIAN_POINT('',(-18.6526484317677,1076.73142393294,359.977446487722));
#127349=CARTESIAN_POINT('',(-18.6526484317677,1067.7251047501,359.977446487722));
#127350=CARTESIAN_POINT('Origin',(-18.6526484317677,1076.73142393294,361.698721119765));
#127351=CARTESIAN_POINT('Origin',(-18.6526484317677,1067.7251047501,361.698721119765));
#127352=CARTESIAN_POINT('',(-18.6526484317677,1076.73142393294,360.577446487722));
#127353=CARTESIAN_POINT('Origin',(-18.6526484317677,1076.73142393294,361.698721119765));
#127354=CARTESIAN_POINT('',(-18.6526484317677,1082.7251047501,360.577446487722));
#127355=CARTESIAN_POINT('',(-18.6526484317677,1067.7251047501,360.577446487722));
#127356=CARTESIAN_POINT('Origin',(-18.6526484317677,1082.7251047501,361.698721119765));
#127357=CARTESIAN_POINT('Origin',(-12.9676384183599,1067.7251047501,351.828290490824));
#127358=CARTESIAN_POINT('',(-12.9676384183599,1078.73142393294,350.046297836419));
#127359=CARTESIAN_POINT('Origin',(-12.9676384183599,1078.73142393294,351.828290490824));
#127360=CARTESIAN_POINT('',(-12.9676384183599,1076.73142393294,350.046297836419));
#127361=CARTESIAN_POINT('',(-12.9676384183599,1067.7251047501,350.046297836419));
#127362=CARTESIAN_POINT('Origin',(-12.9676384183599,1076.73142393294,351.828290490824));
#127363=CARTESIAN_POINT('Origin',(-12.9676384183599,1067.7251047501,351.828290490824));
#127364=CARTESIAN_POINT('',(-12.9676384183599,1076.73142393294,350.646297836419));
#127365=CARTESIAN_POINT('Origin',(-12.9676384183599,1076.73142393294,351.828290490824));
#127366=CARTESIAN_POINT('',(-12.9676384183599,1082.7251047501,350.646297836419));
#127367=CARTESIAN_POINT('',(-12.9676384183599,1067.7251047501,350.646297836419));
#127368=CARTESIAN_POINT('Origin',(-12.9676384183599,1082.7251047501,351.828290490824));
#127369=CARTESIAN_POINT('Origin',(-5.44537509787502,1067.7251047501,343.500790972833));
#127370=CARTESIAN_POINT('',(-5.44537509787502,1078.73142393294,341.839910162913));
#127371=CARTESIAN_POINT('Origin',(-5.44537509787502,1078.73142393294,343.500790972833));
#127372=CARTESIAN_POINT('',(-5.44537509787502,1076.73142393294,341.839910162913));
#127373=CARTESIAN_POINT('',(-5.44537509787502,1067.7251047501,341.839910162913));
#127374=CARTESIAN_POINT('Origin',(-5.44537509787502,1076.73142393294,343.500790972833));
#127375=CARTESIAN_POINT('Origin',(-5.44537509787502,1067.7251047501,343.500790972833));
#127376=CARTESIAN_POINT('',(-5.44537509787502,1076.73142393294,342.439910162913));
#127377=CARTESIAN_POINT('Origin',(-5.44537509787502,1076.73142393294,343.500790972833));
#127378=CARTESIAN_POINT('',(-5.44537509787502,1082.7251047501,342.439910162913));
#127379=CARTESIAN_POINT('',(-5.44537509787502,1067.7251047501,342.439910162913));
#127380=CARTESIAN_POINT('Origin',(-5.44537509787502,1082.7251047501,343.500790972833));
#127381=CARTESIAN_POINT('Origin',(-17.4697792349653,1067.7251047501,416.711643838926));
#127382=CARTESIAN_POINT('',(-17.4697792349653,1078.73142393294,415.611285773251));
#127383=CARTESIAN_POINT('Origin',(-17.4697792349653,1078.73142393294,416.711643838926));
#127384=CARTESIAN_POINT('',(-17.4697792349653,1076.73142393294,415.611285773251));
#127385=CARTESIAN_POINT('',(-17.4697792349653,1067.7251047501,415.611285773251));
#127386=CARTESIAN_POINT('Origin',(-17.4697792349653,1076.73142393294,416.711643838926));
#127387=CARTESIAN_POINT('Origin',(-17.4697792349653,1067.7251047501,416.711643838926));
#127388=CARTESIAN_POINT('',(-17.4697792349653,1076.73142393294,416.211285773251));
#127389=CARTESIAN_POINT('Origin',(-17.4697792349653,1076.73142393294,416.711643838926));
#127390=CARTESIAN_POINT('',(-17.4697792349653,1082.7251047501,416.211285773251));
#127391=CARTESIAN_POINT('',(-17.4697792349653,1067.7251047501,416.211285773251));
#127392=CARTESIAN_POINT('Origin',(-17.4697792349653,1082.7251047501,416.711643838926));
#127393=CARTESIAN_POINT('Origin',(-23.6747930603223,1067.7251047501,410.809510856862));
#127394=CARTESIAN_POINT('',(-23.6747930603223,1078.73142393294,409.595479290125));
#127395=CARTESIAN_POINT('Origin',(-23.6747930603223,1078.73142393294,410.809510856862));
#127396=CARTESIAN_POINT('',(-23.6747930603223,1076.73142393294,409.595479290125));
#127397=CARTESIAN_POINT('',(-23.6747930603223,1067.7251047501,409.595479290125));
#127398=CARTESIAN_POINT('Origin',(-23.6747930603223,1076.73142393294,410.809510856862));
#127399=CARTESIAN_POINT('Origin',(-23.6747930603223,1067.7251047501,410.809510856862));
#127400=CARTESIAN_POINT('',(-23.6747930603223,1076.73142393294,410.195479290125));
#127401=CARTESIAN_POINT('Origin',(-23.6747930603223,1076.73142393294,410.809510856862));
#127402=CARTESIAN_POINT('',(-23.6747930603223,1082.7251047501,410.195479290125));
#127403=CARTESIAN_POINT('',(-23.6747930603223,1067.7251047501,410.195479290125));
#127404=CARTESIAN_POINT('Origin',(-23.6747930603223,1082.7251047501,410.809510856862));
#127405=CARTESIAN_POINT('Origin',(-27.9332476920707,1067.7251047501,404.124867719805));
#127406=CARTESIAN_POINT('',(-27.9332476920707,1078.73142393294,402.796059756232));
#127407=CARTESIAN_POINT('Origin',(-27.9332476920707,1078.73142393294,404.124867719805));
#127408=CARTESIAN_POINT('',(-27.9332476920707,1076.73142393294,402.796059756232));
#127409=CARTESIAN_POINT('',(-27.9332476920707,1067.7251047501,402.796059756232));
#127410=CARTESIAN_POINT('Origin',(-27.9332476920707,1076.73142393294,404.124867719805));
#127411=CARTESIAN_POINT('Origin',(-27.9332476920707,1067.7251047501,404.124867719805));
#127412=CARTESIAN_POINT('',(-27.9332476920707,1076.73142393294,403.396059756232));
#127413=CARTESIAN_POINT('Origin',(-27.9332476920707,1076.73142393294,404.124867719805));
#127414=CARTESIAN_POINT('',(-27.9332476920707,1082.7251047501,403.396059756232));
#127415=CARTESIAN_POINT('',(-27.9332476920707,1067.7251047501,403.396059756232));
#127416=CARTESIAN_POINT('Origin',(-27.9332476920707,1082.7251047501,404.124867719805));
#127417=CARTESIAN_POINT('Origin',(-31.5832678801404,1067.7251047501,395.603729921877));
#127418=CARTESIAN_POINT('',(-31.5832678801404,1078.73142393294,394.14261292006));
#127419=CARTESIAN_POINT('Origin',(-31.5832678801404,1078.73142393294,395.603729921877));
#127420=CARTESIAN_POINT('',(-31.5832678801404,1076.73142393294,394.14261292006));
#127421=CARTESIAN_POINT('',(-31.5832678801404,1067.7251047501,394.14261292006));
#127422=CARTESIAN_POINT('Origin',(-31.5832678801404,1076.73142393294,395.603729921877));
#127423=CARTESIAN_POINT('Origin',(-31.5832678801404,1067.7251047501,395.603729921877));
#127424=CARTESIAN_POINT('',(-31.5832678801404,1076.73142393294,394.74261292006));
#127425=CARTESIAN_POINT('Origin',(-31.5832678801404,1076.73142393294,395.603729921877));
#127426=CARTESIAN_POINT('',(-31.5832678801404,1082.7251047501,394.74261292006));
#127427=CARTESIAN_POINT('',(-31.5832678801404,1067.7251047501,394.74261292006));
#127428=CARTESIAN_POINT('Origin',(-31.5832678801404,1082.7251047501,395.603729921877));
#127429=CARTESIAN_POINT('Origin',(-32.9700055803535,1067.7251047501,386.791676580752));
#127430=CARTESIAN_POINT('',(-32.9700055803535,1078.73142393294,385.171194538127));
#127431=CARTESIAN_POINT('Origin',(-32.9700055803535,1078.73142393294,386.791676580752));
#127432=CARTESIAN_POINT('',(-32.9700055803535,1076.73142393294,385.171194538127));
#127433=CARTESIAN_POINT('',(-32.9700055803535,1067.7251047501,385.171194538127));
#127434=CARTESIAN_POINT('Origin',(-32.9700055803535,1076.73142393294,386.791676580752));
#127435=CARTESIAN_POINT('Origin',(-32.9700055803535,1067.7251047501,386.791676580752));
#127436=CARTESIAN_POINT('',(-32.9700055803535,1076.73142393294,385.771194538127));
#127437=CARTESIAN_POINT('Origin',(-32.9700055803535,1076.73142393294,386.791676580752));
#127438=CARTESIAN_POINT('',(-32.9700055803535,1082.7251047501,385.771194538127));
#127439=CARTESIAN_POINT('',(-32.9700055803535,1067.7251047501,385.771194538127));
#127440=CARTESIAN_POINT('Origin',(-32.9700055803535,1082.7251047501,386.791676580752));
#127441=CARTESIAN_POINT('Origin',(-33.2806783666209,1067.7251047501,376.622503406177));
#127442=CARTESIAN_POINT('',(-33.2806783666209,1078.73142393294,374.921503183094));
#127443=CARTESIAN_POINT('Origin',(-33.2806783666209,1078.73142393294,376.622503406177));
#127444=CARTESIAN_POINT('',(-33.2806783666209,1076.73142393294,374.921503183094));
#127445=CARTESIAN_POINT('',(-33.2806783666209,1067.7251047501,374.921503183094));
#127446=CARTESIAN_POINT('Origin',(-33.2806783666209,1076.73142393294,376.622503406177));
#127447=CARTESIAN_POINT('Origin',(-33.2806783666209,1067.7251047501,376.622503406177));
#127448=CARTESIAN_POINT('',(-33.2806783666209,1076.73142393294,375.521503183094));
#127449=CARTESIAN_POINT('Origin',(-33.2806783666209,1076.73142393294,376.622503406177));
#127450=CARTESIAN_POINT('',(-33.2806783666209,1082.7251047501,375.521503183094));
#127451=CARTESIAN_POINT('',(-33.2806783666209,1067.7251047501,375.521503183094));
#127452=CARTESIAN_POINT('Origin',(-33.2806783666209,1082.7251047501,376.622503406177));
#127453=CARTESIAN_POINT('Origin',(-31.3271632264578,1067.7251047501,366.951811002826));
#127454=CARTESIAN_POINT('',(-31.3271632264578,1078.73142393294,365.230536370782));
#127455=CARTESIAN_POINT('Origin',(-31.3271632264578,1078.73142393294,366.951811002826));
#127456=CARTESIAN_POINT('',(-31.3271632264578,1076.73142393294,365.230536370782));
#127457=CARTESIAN_POINT('',(-31.3271632264578,1067.7251047501,365.230536370782));
#127458=CARTESIAN_POINT('Origin',(-31.3271632264578,1076.73142393294,366.951811002826));
#127459=CARTESIAN_POINT('Origin',(-31.3271632264578,1067.7251047501,366.951811002826));
#127460=CARTESIAN_POINT('',(-31.3271632264578,1076.73142393294,365.830536370782));
#127461=CARTESIAN_POINT('Origin',(-31.3271632264578,1076.73142393294,366.951811002826));
#127462=CARTESIAN_POINT('',(-31.3271632264578,1082.7251047501,365.830536370782));
#127463=CARTESIAN_POINT('',(-31.3271632264578,1067.7251047501,365.830536370782));
#127464=CARTESIAN_POINT('Origin',(-31.3271632264578,1082.7251047501,366.951811002826));
#127465=CARTESIAN_POINT('Origin',(-27.818562242858,1067.7251047501,356.115092920714));
#127466=CARTESIAN_POINT('',(-27.818562242858,1078.73142393294,354.333100266309));
#127467=CARTESIAN_POINT('Origin',(-27.818562242858,1078.73142393294,356.115092920714));
#127468=CARTESIAN_POINT('',(-27.818562242858,1076.73142393294,354.333100266309));
#127469=CARTESIAN_POINT('',(-27.818562242858,1067.7251047501,354.333100266309));
#127470=CARTESIAN_POINT('Origin',(-27.818562242858,1076.73142393294,356.115092920714));
#127471=CARTESIAN_POINT('Origin',(-27.818562242858,1067.7251047501,356.115092920714));
#127472=CARTESIAN_POINT('',(-27.818562242858,1076.73142393294,354.933100266309));
#127473=CARTESIAN_POINT('Origin',(-27.818562242858,1076.73142393294,356.115092920714));
#127474=CARTESIAN_POINT('',(-27.818562242858,1082.7251047501,354.933100266309));
#127475=CARTESIAN_POINT('',(-27.818562242858,1067.7251047501,354.933100266309));
#127476=CARTESIAN_POINT('Origin',(-27.818562242858,1082.7251047501,356.115092920714));
#127477=CARTESIAN_POINT('Origin',(-22.1920629289073,1067.7251047501,346.405602761341));
#127478=CARTESIAN_POINT('',(-22.1920629289073,1078.73142393294,344.74472195142));
#127479=CARTESIAN_POINT('Origin',(-22.1920629289073,1078.73142393294,346.405602761341));
#127480=CARTESIAN_POINT('',(-22.1920629289073,1076.73142393294,344.74472195142));
#127481=CARTESIAN_POINT('',(-22.1920629289073,1067.7251047501,344.74472195142));
#127482=CARTESIAN_POINT('Origin',(-22.1920629289073,1076.73142393294,346.405602761341));
#127483=CARTESIAN_POINT('Origin',(-22.1920629289073,1067.7251047501,346.405602761341));
#127484=CARTESIAN_POINT('',(-22.1920629289073,1076.73142393294,345.34472195142));
#127485=CARTESIAN_POINT('Origin',(-22.1920629289073,1076.73142393294,346.405602761341));
#127486=CARTESIAN_POINT('',(-22.1920629289073,1082.7251047501,345.34472195142));
#127487=CARTESIAN_POINT('',(-22.1920629289073,1067.7251047501,345.34472195142));
#127488=CARTESIAN_POINT('Origin',(-22.1920629289073,1082.7251047501,346.405602761341));
#127489=CARTESIAN_POINT('Origin',(-18.7323127802563,1067.7251047501,420.516637035203));
#127490=CARTESIAN_POINT('',(-18.7323127802563,1078.73142393294,419.416278969528));
#127491=CARTESIAN_POINT('Origin',(-18.7323127802563,1078.73142393294,420.516637035203));
#127492=CARTESIAN_POINT('',(-18.7323127802563,1076.73142393294,419.416278969528));
#127493=CARTESIAN_POINT('',(-18.7323127802563,1067.7251047501,419.416278969528));
#127494=CARTESIAN_POINT('Origin',(-18.7323127802563,1076.73142393294,420.516637035203));
#127495=CARTESIAN_POINT('Origin',(-18.7323127802563,1067.7251047501,420.516637035203));
#127496=CARTESIAN_POINT('',(-18.7323127802563,1076.73142393294,420.016278969528));
#127497=CARTESIAN_POINT('Origin',(-18.7323127802563,1076.73142393294,420.516637035203));
#127498=CARTESIAN_POINT('',(-18.7323127802563,1082.7251047501,420.016278969528));
#127499=CARTESIAN_POINT('',(-18.7323127802563,1067.7251047501,420.016278969528));
#127500=CARTESIAN_POINT('Origin',(-18.7323127802563,1082.7251047501,420.516637035203));
#127501=CARTESIAN_POINT('Origin',(-26.0288546137815,1067.7251047501,416.033574735563));
#127502=CARTESIAN_POINT('',(-26.0288546137815,1078.73142393294,414.819543168826));
#127503=CARTESIAN_POINT('Origin',(-26.0288546137815,1078.73142393294,416.033574735563));
#127504=CARTESIAN_POINT('',(-26.0288546137815,1076.73142393294,414.819543168826));
#127505=CARTESIAN_POINT('',(-26.0288546137815,1067.7251047501,414.819543168826));
#127506=CARTESIAN_POINT('Origin',(-26.0288546137815,1076.73142393294,416.033574735563));
#127507=CARTESIAN_POINT('Origin',(-26.0288546137815,1067.7251047501,416.033574735563));
#127508=CARTESIAN_POINT('',(-26.0288546137815,1076.73142393294,415.419543168826));
#127509=CARTESIAN_POINT('Origin',(-26.0288546137815,1076.73142393294,416.033574735563));
#127510=CARTESIAN_POINT('',(-26.0288546137815,1082.7251047501,415.419543168826));
#127511=CARTESIAN_POINT('',(-26.0288546137815,1067.7251047501,415.419543168826));
#127512=CARTESIAN_POINT('Origin',(-26.0288546137815,1082.7251047501,416.033574735563));
#127513=CARTESIAN_POINT('Origin',(-31.5840672517988,1067.7251047501,410.380389592047));
#127514=CARTESIAN_POINT('',(-31.5840672517988,1078.73142393294,409.051581628474));
#127515=CARTESIAN_POINT('Origin',(-31.5840672517988,1078.73142393294,410.380389592047));
#127516=CARTESIAN_POINT('',(-31.5840672517988,1076.73142393294,409.051581628474));
#127517=CARTESIAN_POINT('',(-31.5840672517988,1067.7251047501,409.051581628474));
#127518=CARTESIAN_POINT('Origin',(-31.5840672517988,1076.73142393294,410.380389592047));
#127519=CARTESIAN_POINT('Origin',(-31.5840672517988,1067.7251047501,410.380389592047));
#127520=CARTESIAN_POINT('',(-31.5840672517988,1076.73142393294,409.651581628474));
#127521=CARTESIAN_POINT('Origin',(-31.5840672517988,1076.73142393294,410.380389592047));
#127522=CARTESIAN_POINT('',(-31.5840672517988,1082.7251047501,409.651581628474));
#127523=CARTESIAN_POINT('',(-31.5840672517988,1067.7251047501,409.651581628474));
#127524=CARTESIAN_POINT('Origin',(-31.5840672517988,1082.7251047501,410.380389592047));
#127525=CARTESIAN_POINT('Origin',(-36.9259699086473,1067.7251047501,402.804340968302));
#127526=CARTESIAN_POINT('',(-36.9259699086473,1078.73142393294,401.343223966485));
#127527=CARTESIAN_POINT('Origin',(-36.9259699086473,1078.73142393294,402.804340968302));
#127528=CARTESIAN_POINT('',(-36.9259699086473,1076.73142393294,401.343223966485));
#127529=CARTESIAN_POINT('',(-36.9259699086473,1067.7251047501,401.343223966485));
#127530=CARTESIAN_POINT('Origin',(-36.9259699086473,1076.73142393294,402.804340968302));
#127531=CARTESIAN_POINT('Origin',(-36.9259699086473,1067.7251047501,402.804340968302));
#127532=CARTESIAN_POINT('',(-36.9259699086473,1076.73142393294,401.943223966485));
#127533=CARTESIAN_POINT('Origin',(-36.9259699086473,1076.73142393294,402.804340968302));
#127534=CARTESIAN_POINT('',(-36.9259699086473,1082.7251047501,401.943223966485));
#127535=CARTESIAN_POINT('',(-36.9259699086473,1067.7251047501,401.943223966485));
#127536=CARTESIAN_POINT('Origin',(-36.9259699086473,1082.7251047501,402.804340968302));
#127537=CARTESIAN_POINT('Origin',(-40.1145329726876,1067.7251047501,394.473171115114));
#127538=CARTESIAN_POINT('',(-40.1145329726876,1078.73142393294,392.85268907249));
#127539=CARTESIAN_POINT('Origin',(-40.1145329726876,1078.73142393294,394.473171115114));
#127540=CARTESIAN_POINT('',(-40.1145329726876,1076.73142393294,392.85268907249));
#127541=CARTESIAN_POINT('',(-40.1145329726876,1067.7251047501,392.85268907249));
#127542=CARTESIAN_POINT('Origin',(-40.1145329726876,1076.73142393294,394.473171115114));
#127543=CARTESIAN_POINT('Origin',(-40.1145329726876,1067.7251047501,394.473171115114));
#127544=CARTESIAN_POINT('',(-40.1145329726876,1076.73142393294,393.45268907249));
#127545=CARTESIAN_POINT('Origin',(-40.1145329726876,1076.73142393294,394.473171115114));
#127546=CARTESIAN_POINT('',(-40.1145329726876,1082.7251047501,393.45268907249));
#127547=CARTESIAN_POINT('',(-40.1145329726876,1067.7251047501,393.45268907249));
#127548=CARTESIAN_POINT('Origin',(-40.1145329726876,1082.7251047501,394.473171115114));
#127549=CARTESIAN_POINT('Origin',(-42.5327068021327,1067.7251047501,384.590811277241));
#127550=CARTESIAN_POINT('',(-42.5327068021327,1078.73142393294,382.889811054159));
#127551=CARTESIAN_POINT('Origin',(-42.5327068021327,1078.73142393294,384.590811277241));
#127552=CARTESIAN_POINT('',(-42.5327068021327,1076.73142393294,382.889811054159));
#127553=CARTESIAN_POINT('',(-42.5327068021327,1067.7251047501,382.889811054159));
#127554=CARTESIAN_POINT('Origin',(-42.5327068021327,1076.73142393294,384.590811277241));
#127555=CARTESIAN_POINT('Origin',(-42.5327068021327,1067.7251047501,384.590811277241));
#127556=CARTESIAN_POINT('',(-42.5327068021327,1076.73142393294,383.489811054159));
#127557=CARTESIAN_POINT('Origin',(-42.5327068021327,1076.73142393294,384.590811277241));
#127558=CARTESIAN_POINT('',(-42.5327068021327,1082.7251047501,383.489811054159));
#127559=CARTESIAN_POINT('',(-42.5327068021327,1067.7251047501,383.489811054159));
#127560=CARTESIAN_POINT('Origin',(-42.5327068021327,1082.7251047501,384.590811277241));
#127561=CARTESIAN_POINT('Origin',(-42.6325306637444,1067.7251047501,374.725288069639));
#127562=CARTESIAN_POINT('',(-42.6325306637444,1078.73142393294,373.004013437596));
#127563=CARTESIAN_POINT('Origin',(-42.6325306637444,1078.73142393294,374.725288069639));
#127564=CARTESIAN_POINT('',(-42.6325306637444,1076.73142393294,373.004013437596));
#127565=CARTESIAN_POINT('',(-42.6325306637444,1067.7251047501,373.004013437596));
#127566=CARTESIAN_POINT('Origin',(-42.6325306637444,1076.73142393294,374.725288069639));
#127567=CARTESIAN_POINT('Origin',(-42.6325306637444,1067.7251047501,374.725288069639));
#127568=CARTESIAN_POINT('',(-42.6325306637444,1076.73142393294,373.604013437596));
#127569=CARTESIAN_POINT('Origin',(-42.6325306637444,1076.73142393294,374.725288069639));
#127570=CARTESIAN_POINT('',(-42.6325306637444,1082.7251047501,373.604013437596));
#127571=CARTESIAN_POINT('',(-42.6325306637444,1067.7251047501,373.604013437596));
#127572=CARTESIAN_POINT('Origin',(-42.6325306637444,1082.7251047501,374.725288069639));
#127573=CARTESIAN_POINT('Origin',(-41.4536814090712,1067.7251047501,363.395899114888));
#127574=CARTESIAN_POINT('',(-41.4536814090712,1078.73142393294,361.613906460483));
#127575=CARTESIAN_POINT('Origin',(-41.4536814090712,1078.73142393294,363.395899114888));
#127576=CARTESIAN_POINT('',(-41.4536814090712,1076.73142393294,361.613906460483));
#127577=CARTESIAN_POINT('',(-41.4536814090712,1067.7251047501,361.613906460483));
#127578=CARTESIAN_POINT('Origin',(-41.4536814090712,1076.73142393294,363.395899114888));
#127579=CARTESIAN_POINT('Origin',(-41.4536814090712,1067.7251047501,363.395899114888));
#127580=CARTESIAN_POINT('',(-41.4536814090712,1076.73142393294,362.213906460483));
#127581=CARTESIAN_POINT('Origin',(-41.4536814090712,1076.73142393294,363.395899114888));
#127582=CARTESIAN_POINT('',(-41.4536814090712,1082.7251047501,362.213906460483));
#127583=CARTESIAN_POINT('',(-41.4536814090712,1067.7251047501,362.213906460483));
#127584=CARTESIAN_POINT('Origin',(-41.4536814090712,1082.7251047501,363.395899114888));
#127585=CARTESIAN_POINT('Origin',(-37.9688511206135,1067.7251047501,352.7287696254));
#127586=CARTESIAN_POINT('',(-37.9688511206135,1078.73142393294,351.067888815479));
#127587=CARTESIAN_POINT('Origin',(-37.9688511206135,1078.73142393294,352.7287696254));
#127588=CARTESIAN_POINT('',(-37.9688511206135,1076.73142393294,351.067888815479));
#127589=CARTESIAN_POINT('',(-37.9688511206135,1067.7251047501,351.067888815479));
#127590=CARTESIAN_POINT('Origin',(-37.9688511206135,1076.73142393294,352.7287696254));
#127591=CARTESIAN_POINT('Origin',(-37.9688511206135,1067.7251047501,352.7287696254));
#127592=CARTESIAN_POINT('',(-37.9688511206135,1076.73142393294,351.667888815479));
#127593=CARTESIAN_POINT('Origin',(-37.9688511206135,1076.73142393294,352.7287696254));
#127594=CARTESIAN_POINT('',(-37.9688511206135,1082.7251047501,351.667888815479));
#127595=CARTESIAN_POINT('',(-37.9688511206135,1067.7251047501,351.667888815479));
#127596=CARTESIAN_POINT('Origin',(-37.9688511206135,1082.7251047501,352.7287696254));
#127597=CARTESIAN_POINT('Origin',(-19.1761543694403,1067.7251047501,424.500977485066));
#127598=CARTESIAN_POINT('',(-19.1761543694403,1078.73142393294,423.400619419391));
#127599=CARTESIAN_POINT('Origin',(-19.1761543694403,1078.73142393294,424.500977485066));
#127600=CARTESIAN_POINT('',(-19.1761543694403,1076.73142393294,423.400619419391));
#127601=CARTESIAN_POINT('',(-19.1761543694403,1067.7251047501,423.400619419391));
#127602=CARTESIAN_POINT('Origin',(-19.1761543694403,1076.73142393294,424.500977485066));
#127603=CARTESIAN_POINT('Origin',(-19.1761543694403,1067.7251047501,424.500977485066));
#127604=CARTESIAN_POINT('',(-19.1761543694403,1076.73142393294,424.000619419391));
#127605=CARTESIAN_POINT('Origin',(-19.1761543694403,1076.73142393294,424.500977485066));
#127606=CARTESIAN_POINT('',(-19.1761543694403,1082.7251047501,424.000619419391));
#127607=CARTESIAN_POINT('',(-19.1761543694403,1067.7251047501,424.000619419391));
#127608=CARTESIAN_POINT('Origin',(-19.1761543694403,1082.7251047501,424.500977485066));
#127609=CARTESIAN_POINT('Origin',(-27.2453303203163,1067.7251047501,421.632917202464));
#127610=CARTESIAN_POINT('',(-27.2453303203163,1078.73142393294,420.418885635727));
#127611=CARTESIAN_POINT('Origin',(-27.2453303203163,1078.73142393294,421.632917202464));
#127612=CARTESIAN_POINT('',(-27.2453303203163,1076.73142393294,420.418885635727));
#127613=CARTESIAN_POINT('',(-27.2453303203163,1067.7251047501,420.418885635727));
#127614=CARTESIAN_POINT('Origin',(-27.2453303203163,1076.73142393294,421.632917202464));
#127615=CARTESIAN_POINT('Origin',(-27.2453303203163,1067.7251047501,421.632917202464));
#127616=CARTESIAN_POINT('',(-27.2453303203163,1076.73142393294,421.018885635727));
#127617=CARTESIAN_POINT('Origin',(-27.2453303203163,1076.73142393294,421.632917202464));
#127618=CARTESIAN_POINT('',(-27.2453303203163,1082.7251047501,421.018885635727));
#127619=CARTESIAN_POINT('',(-27.2453303203163,1067.7251047501,421.018885635727));
#127620=CARTESIAN_POINT('Origin',(-27.2453303203163,1082.7251047501,421.632917202464));
#127621=CARTESIAN_POINT('Origin',(-33.8545115154534,1067.7251047501,417.258261370252));
#127622=CARTESIAN_POINT('',(-33.8545115154534,1078.73142393294,415.929453406678));
#127623=CARTESIAN_POINT('Origin',(-33.8545115154534,1078.73142393294,417.258261370252));
#127624=CARTESIAN_POINT('',(-33.8545115154534,1076.73142393294,415.929453406678));
#127625=CARTESIAN_POINT('',(-33.8545115154534,1067.7251047501,415.929453406678));
#127626=CARTESIAN_POINT('Origin',(-33.8545115154534,1076.73142393294,417.258261370252));
#127627=CARTESIAN_POINT('Origin',(-33.8545115154534,1067.7251047501,417.258261370252));
#127628=CARTESIAN_POINT('',(-33.8545115154534,1076.73142393294,416.529453406679));
#127629=CARTESIAN_POINT('Origin',(-33.8545115154534,1076.73142393294,417.258261370252));
#127630=CARTESIAN_POINT('',(-33.8545115154534,1082.7251047501,416.529453406679));
#127631=CARTESIAN_POINT('',(-33.8545115154534,1067.7251047501,416.529453406679));
#127632=CARTESIAN_POINT('Origin',(-33.8545115154534,1082.7251047501,417.258261370252));
#127633=CARTESIAN_POINT('Origin',(-40.6548298616837,1067.7251047501,410.958411599462));
#127634=CARTESIAN_POINT('',(-40.6548298616837,1078.73142393294,409.497294597646));
#127635=CARTESIAN_POINT('Origin',(-40.6548298616837,1078.73142393294,410.958411599462));
#127636=CARTESIAN_POINT('',(-40.6548298616837,1076.73142393294,409.497294597646));
#127637=CARTESIAN_POINT('',(-40.6548298616837,1067.7251047501,409.497294597646));
#127638=CARTESIAN_POINT('Origin',(-40.6548298616837,1076.73142393294,410.958411599462));
#127639=CARTESIAN_POINT('Origin',(-40.6548298616837,1067.7251047501,410.958411599462));
#127640=CARTESIAN_POINT('',(-40.6548298616837,1076.73142393294,410.097294597645));
#127641=CARTESIAN_POINT('Origin',(-40.6548298616837,1076.73142393294,410.958411599462));
#127642=CARTESIAN_POINT('',(-40.6548298616837,1082.7251047501,410.097294597645));
#127643=CARTESIAN_POINT('',(-40.6548298616837,1067.7251047501,410.097294597645));
#127644=CARTESIAN_POINT('Origin',(-40.6548298616837,1082.7251047501,410.958411599462));
#127645=CARTESIAN_POINT('Origin',(-45.5058627832294,1067.7251047501,403.472237334184));
#127646=CARTESIAN_POINT('',(-45.5058627832294,1078.73142393294,401.85175529156));
#127647=CARTESIAN_POINT('Origin',(-45.5058627832294,1078.73142393294,403.472237334184));
#127648=CARTESIAN_POINT('',(-45.5058627832294,1076.73142393294,401.85175529156));
#127649=CARTESIAN_POINT('',(-45.5058627832294,1067.7251047501,401.85175529156));
#127650=CARTESIAN_POINT('Origin',(-45.5058627832294,1076.73142393294,403.472237334184));
#127651=CARTESIAN_POINT('Origin',(-45.5058627832294,1067.7251047501,403.472237334184));
#127652=CARTESIAN_POINT('',(-45.5058627832294,1076.73142393294,402.45175529156));
#127653=CARTESIAN_POINT('Origin',(-45.5058627832294,1076.73142393294,403.472237334184));
#127654=CARTESIAN_POINT('',(-45.5058627832294,1082.7251047501,402.45175529156));
#127655=CARTESIAN_POINT('',(-45.5058627832294,1067.7251047501,402.45175529156));
#127656=CARTESIAN_POINT('Origin',(-45.5058627832294,1082.7251047501,403.472237334184));
#127657=CARTESIAN_POINT('Origin',(-49.92585185582,1067.7251047501,394.308597378752));
#127658=CARTESIAN_POINT('',(-49.92585185582,1078.73142393294,392.607597155669));
#127659=CARTESIAN_POINT('Origin',(-49.92585185582,1078.73142393294,394.308597378752));
#127660=CARTESIAN_POINT('',(-49.92585185582,1076.73142393294,392.607597155669));
#127661=CARTESIAN_POINT('',(-49.92585185582,1067.7251047501,392.607597155669));
#127662=CARTESIAN_POINT('Origin',(-49.92585185582,1076.73142393294,394.308597378752));
#127663=CARTESIAN_POINT('Origin',(-49.92585185582,1067.7251047501,394.308597378752));
#127664=CARTESIAN_POINT('',(-49.92585185582,1076.73142393294,393.207597155669));
#127665=CARTESIAN_POINT('Origin',(-49.92585185582,1076.73142393294,394.308597378752));
#127666=CARTESIAN_POINT('',(-49.92585185582,1082.7251047501,393.207597155669));
#127667=CARTESIAN_POINT('',(-49.92585185582,1067.7251047501,393.207597155669));
#127668=CARTESIAN_POINT('Origin',(-49.92585185582,1082.7251047501,394.308597378752));
#127669=CARTESIAN_POINT('Origin',(-52.0746519374459,1067.7251047501,384.679414071104));
#127670=CARTESIAN_POINT('',(-52.0746519374459,1078.73142393294,382.958139439061));
#127671=CARTESIAN_POINT('Origin',(-52.0746519374459,1078.73142393294,384.679414071104));
#127672=CARTESIAN_POINT('',(-52.0746519374459,1076.73142393294,382.958139439061));
#127673=CARTESIAN_POINT('',(-52.0746519374459,1067.7251047501,382.958139439061));
#127674=CARTESIAN_POINT('Origin',(-52.0746519374459,1076.73142393294,384.679414071104));
#127675=CARTESIAN_POINT('Origin',(-52.0746519374459,1067.7251047501,384.679414071104));
#127676=CARTESIAN_POINT('',(-52.0746519374459,1076.73142393294,383.558139439061));
#127677=CARTESIAN_POINT('Origin',(-52.0746519374459,1076.73142393294,384.679414071104));
#127678=CARTESIAN_POINT('',(-52.0746519374459,1082.7251047501,383.558139439061));
#127679=CARTESIAN_POINT('',(-52.0746519374459,1067.7251047501,383.558139439061));
#127680=CARTESIAN_POINT('Origin',(-52.0746519374459,1082.7251047501,384.679414071104));
#127681=CARTESIAN_POINT('Origin',(-53.277075780875,1067.7251047501,373.352502905475));
#127682=CARTESIAN_POINT('',(-53.277075780875,1078.73142393294,371.57051025107));
#127683=CARTESIAN_POINT('Origin',(-53.277075780875,1078.73142393294,373.352502905475));
#127684=CARTESIAN_POINT('',(-53.277075780875,1076.73142393294,371.57051025107));
#127685=CARTESIAN_POINT('',(-53.277075780875,1067.7251047501,371.57051025107));
#127686=CARTESIAN_POINT('Origin',(-53.277075780875,1076.73142393294,373.352502905475));
#127687=CARTESIAN_POINT('Origin',(-53.277075780875,1067.7251047501,373.352502905475));
#127688=CARTESIAN_POINT('',(-53.277075780875,1076.73142393294,372.17051025107));
#127689=CARTESIAN_POINT('Origin',(-53.277075780875,1076.73142393294,373.352502905475));
#127690=CARTESIAN_POINT('',(-53.277075780875,1082.7251047501,372.17051025107));
#127691=CARTESIAN_POINT('',(-53.277075780875,1067.7251047501,372.17051025107));
#127692=CARTESIAN_POINT('Origin',(-53.277075780875,1082.7251047501,373.352502905475));
#127693=CARTESIAN_POINT('Origin',(-52.086218323587,1067.7251047501,362.19393883113));
#127694=CARTESIAN_POINT('',(-52.086218323587,1078.73142393294,360.53305802121));
#127695=CARTESIAN_POINT('Origin',(-52.086218323587,1078.73142393294,362.19393883113));
#127696=CARTESIAN_POINT('',(-52.086218323587,1076.73142393294,360.53305802121));
#127697=CARTESIAN_POINT('',(-52.086218323587,1067.7251047501,360.53305802121));
#127698=CARTESIAN_POINT('Origin',(-52.086218323587,1076.73142393294,362.19393883113));
#127699=CARTESIAN_POINT('Origin',(-52.086218323587,1067.7251047501,362.19393883113));
#127700=CARTESIAN_POINT('',(-52.086218323587,1076.73142393294,361.133058021209));
#127701=CARTESIAN_POINT('Origin',(-52.086218323587,1076.73142393294,362.19393883113));
#127702=CARTESIAN_POINT('',(-52.086218323587,1082.7251047501,361.133058021209));
#127703=CARTESIAN_POINT('',(-52.086218323587,1067.7251047501,361.133058021209));
#127704=CARTESIAN_POINT('Origin',(-52.086218323587,1082.7251047501,362.19393883113));
#127705=CARTESIAN_POINT('Origin',(-18.7819059952821,1067.7251047501,428.490530391869));
#127706=CARTESIAN_POINT('',(-18.7819059952821,1078.73142393294,427.390172326194));
#127707=CARTESIAN_POINT('Origin',(-18.7819059952821,1078.73142393294,428.490530391869));
#127708=CARTESIAN_POINT('',(-18.7819059952821,1076.73142393294,427.390172326194));
#127709=CARTESIAN_POINT('',(-18.7819059952821,1067.7251047501,427.390172326194));
#127710=CARTESIAN_POINT('Origin',(-18.7819059952821,1076.73142393294,428.490530391869));
#127711=CARTESIAN_POINT('Origin',(-18.7819059952821,1067.7251047501,428.490530391869));
#127712=CARTESIAN_POINT('',(-18.7819059952821,1076.73142393294,427.990172326194));
#127713=CARTESIAN_POINT('Origin',(-18.7819059952821,1076.73142393294,428.490530391869));
#127714=CARTESIAN_POINT('',(-18.7819059952821,1082.7251047501,427.990172326194));
#127715=CARTESIAN_POINT('',(-18.7819059952821,1067.7251047501,427.990172326194));
#127716=CARTESIAN_POINT('Origin',(-18.7819059952821,1082.7251047501,428.490530391869));
#127717=CARTESIAN_POINT('Origin',(-27.2710543542534,1067.7251047501,427.362820123134));
#127718=CARTESIAN_POINT('',(-27.2710543542534,1078.73142393294,426.148788556397));
#127719=CARTESIAN_POINT('Origin',(-27.2710543542534,1078.73142393294,427.362820123134));
#127720=CARTESIAN_POINT('',(-27.2710543542534,1076.73142393294,426.148788556397));
#127721=CARTESIAN_POINT('',(-27.2710543542534,1067.7251047501,426.148788556397));
#127722=CARTESIAN_POINT('Origin',(-27.2710543542534,1076.73142393294,427.362820123134));
#127723=CARTESIAN_POINT('Origin',(-27.2710543542534,1067.7251047501,427.362820123134));
#127724=CARTESIAN_POINT('',(-27.2710543542534,1076.73142393294,426.748788556397));
#127725=CARTESIAN_POINT('Origin',(-27.2710543542534,1076.73142393294,427.362820123134));
#127726=CARTESIAN_POINT('',(-27.2710543542534,1082.7251047501,426.748788556397));
#127727=CARTESIAN_POINT('',(-27.2710543542534,1067.7251047501,426.748788556397));
#127728=CARTESIAN_POINT('Origin',(-27.2710543542534,1082.7251047501,427.362820123134));
#127729=CARTESIAN_POINT('Origin',(-34.6453511739129,1067.7251047501,424.457887054022));
#127730=CARTESIAN_POINT('',(-34.6453511739129,1078.73142393294,423.129079090448));
#127731=CARTESIAN_POINT('Origin',(-34.6453511739129,1078.73142393294,424.457887054022));
#127732=CARTESIAN_POINT('',(-34.6453511739129,1076.73142393294,423.129079090448));
#127733=CARTESIAN_POINT('',(-34.6453511739129,1067.7251047501,423.129079090448));
#127734=CARTESIAN_POINT('Origin',(-34.6453511739129,1076.73142393294,424.457887054022));
#127735=CARTESIAN_POINT('Origin',(-34.6453511739129,1067.7251047501,424.457887054022));
#127736=CARTESIAN_POINT('',(-34.6453511739129,1076.73142393294,423.729079090448));
#127737=CARTESIAN_POINT('Origin',(-34.6453511739129,1076.73142393294,424.457887054022));
#127738=CARTESIAN_POINT('',(-34.6453511739129,1082.7251047501,423.729079090448));
#127739=CARTESIAN_POINT('',(-34.6453511739129,1067.7251047501,423.729079090448));
#127740=CARTESIAN_POINT('Origin',(-34.6453511739129,1082.7251047501,424.457887054022));
#127741=CARTESIAN_POINT('Origin',(-42.6068786662468,1067.7251047501,419.709569801204));
#127742=CARTESIAN_POINT('',(-42.6068786662468,1078.73142393294,418.248452799388));
#127743=CARTESIAN_POINT('Origin',(-42.6068786662468,1078.73142393294,419.709569801204));
#127744=CARTESIAN_POINT('',(-42.6068786662468,1076.73142393294,418.248452799388));
#127745=CARTESIAN_POINT('',(-42.6068786662468,1067.7251047501,418.248452799388));
#127746=CARTESIAN_POINT('Origin',(-42.6068786662468,1076.73142393294,419.709569801204));
#127747=CARTESIAN_POINT('Origin',(-42.6068786662468,1067.7251047501,419.709569801204));
#127748=CARTESIAN_POINT('',(-42.6068786662468,1076.73142393294,418.848452799388));
#127749=CARTESIAN_POINT('Origin',(-42.6068786662468,1076.73142393294,419.709569801204));
#127750=CARTESIAN_POINT('',(-42.6068786662468,1082.7251047501,418.848452799388));
#127751=CARTESIAN_POINT('',(-42.6068786662468,1067.7251047501,418.848452799388));
#127752=CARTESIAN_POINT('Origin',(-42.6068786662468,1082.7251047501,419.709569801204));
#127753=CARTESIAN_POINT('Origin',(-48.9083680287877,1067.7251047501,413.395572861879));
#127754=CARTESIAN_POINT('',(-48.9083680287877,1078.73142393294,411.775090819254));
#127755=CARTESIAN_POINT('Origin',(-48.9083680287877,1078.73142393294,413.395572861879));
#127756=CARTESIAN_POINT('',(-48.9083680287877,1076.73142393294,411.775090819254));
#127757=CARTESIAN_POINT('',(-48.9083680287877,1067.7251047501,411.775090819254));
#127758=CARTESIAN_POINT('Origin',(-48.9083680287877,1076.73142393294,413.395572861879));
#127759=CARTESIAN_POINT('Origin',(-48.9083680287877,1067.7251047501,413.395572861879));
#127760=CARTESIAN_POINT('',(-48.9083680287877,1076.73142393294,412.375090819254));
#127761=CARTESIAN_POINT('Origin',(-48.9083680287877,1076.73142393294,413.395572861879));
#127762=CARTESIAN_POINT('',(-48.9083680287877,1082.7251047501,412.375090819254));
#127763=CARTESIAN_POINT('',(-48.9083680287877,1067.7251047501,412.375090819254));
#127764=CARTESIAN_POINT('Origin',(-48.9083680287877,1082.7251047501,413.395572861879));
#127765=CARTESIAN_POINT('Origin',(-55.136997612591,1067.7251047501,405.351147826963));
#127766=CARTESIAN_POINT('',(-55.136997612591,1078.73142393294,403.65014760388));
#127767=CARTESIAN_POINT('Origin',(-55.136997612591,1078.73142393294,405.351147826963));
#127768=CARTESIAN_POINT('',(-55.136997612591,1076.73142393294,403.65014760388));
#127769=CARTESIAN_POINT('',(-55.136997612591,1067.7251047501,403.65014760388));
#127770=CARTESIAN_POINT('Origin',(-55.136997612591,1076.73142393294,405.351147826963));
#127771=CARTESIAN_POINT('Origin',(-55.136997612591,1067.7251047501,405.351147826963));
#127772=CARTESIAN_POINT('',(-55.136997612591,1076.73142393294,404.25014760388));
#127773=CARTESIAN_POINT('Origin',(-55.136997612591,1076.73142393294,405.351147826963));
#127774=CARTESIAN_POINT('',(-55.136997612591,1082.7251047501,404.25014760388));
#127775=CARTESIAN_POINT('',(-55.136997612591,1067.7251047501,404.25014760388));
#127776=CARTESIAN_POINT('Origin',(-55.136997612591,1082.7251047501,405.351147826963));
#127777=CARTESIAN_POINT('Origin',(-59.2408610395772,1067.7251047501,396.379145935761));
#127778=CARTESIAN_POINT('',(-59.2408610395772,1078.73142393294,394.657871303717));
#127779=CARTESIAN_POINT('Origin',(-59.2408610395772,1078.73142393294,396.379145935761));
#127780=CARTESIAN_POINT('',(-59.2408610395772,1076.73142393294,394.657871303717));
#127781=CARTESIAN_POINT('',(-59.2408610395772,1067.7251047501,394.657871303717));
#127782=CARTESIAN_POINT('Origin',(-59.2408610395772,1076.73142393294,396.379145935761));
#127783=CARTESIAN_POINT('Origin',(-59.2408610395772,1067.7251047501,396.379145935761));
#127784=CARTESIAN_POINT('',(-59.2408610395772,1076.73142393294,395.257871303717));
#127785=CARTESIAN_POINT('Origin',(-59.2408610395772,1076.73142393294,396.379145935761));
#127786=CARTESIAN_POINT('',(-59.2408610395772,1082.7251047501,395.257871303717));
#127787=CARTESIAN_POINT('',(-59.2408610395772,1067.7251047501,395.257871303717));
#127788=CARTESIAN_POINT('Origin',(-59.2408610395772,1082.7251047501,396.379145935761));
#127789=CARTESIAN_POINT('Origin',(-62.7720062892809,1067.7251047501,385.549752929743));
#127790=CARTESIAN_POINT('',(-62.7720062892809,1078.73142393294,383.767760275338));
#127791=CARTESIAN_POINT('Origin',(-62.7720062892809,1078.73142393294,385.549752929743));
#127792=CARTESIAN_POINT('',(-62.7720062892809,1076.73142393294,383.767760275338));
#127793=CARTESIAN_POINT('',(-62.7720062892809,1067.7251047501,383.767760275338));
#127794=CARTESIAN_POINT('Origin',(-62.7720062892809,1076.73142393294,385.549752929743));
#127795=CARTESIAN_POINT('Origin',(-62.7720062892809,1067.7251047501,385.549752929743));
#127796=CARTESIAN_POINT('',(-62.7720062892809,1076.73142393294,384.367760275338));
#127797=CARTESIAN_POINT('Origin',(-62.7720062892809,1076.73142393294,385.549752929743));
#127798=CARTESIAN_POINT('',(-62.7720062892809,1082.7251047501,384.367760275338));
#127799=CARTESIAN_POINT('',(-62.7720062892809,1067.7251047501,384.367760275338));
#127800=CARTESIAN_POINT('Origin',(-62.7720062892809,1082.7251047501,385.549752929743));
#127801=CARTESIAN_POINT('Origin',(-63.9271678484141,1067.7251047501,374.38743706532));
#127802=CARTESIAN_POINT('',(-63.9271678484141,1078.73142393294,372.726556255399));
#127803=CARTESIAN_POINT('Origin',(-63.9271678484141,1078.73142393294,374.38743706532));
#127804=CARTESIAN_POINT('',(-63.9271678484141,1076.73142393294,372.726556255399));
#127805=CARTESIAN_POINT('',(-63.9271678484141,1067.7251047501,372.726556255399));
#127806=CARTESIAN_POINT('Origin',(-63.9271678484141,1076.73142393294,374.38743706532));
#127807=CARTESIAN_POINT('Origin',(-63.9271678484141,1067.7251047501,374.38743706532));
#127808=CARTESIAN_POINT('',(-63.9271678484141,1076.73142393294,373.326556255399));
#127809=CARTESIAN_POINT('Origin',(-63.9271678484141,1076.73142393294,374.38743706532));
#127810=CARTESIAN_POINT('',(-63.9271678484141,1082.7251047501,373.326556255399));
#127811=CARTESIAN_POINT('',(-63.9271678484141,1067.7251047501,373.326556255399));
#127812=CARTESIAN_POINT('Origin',(-63.9271678484141,1082.7251047501,374.38743706532));
#127813=CARTESIAN_POINT('Origin',(-17.5667982035458,1067.7251047501,432.310933149585));
#127814=CARTESIAN_POINT('',(-17.5667982035458,1078.73142393294,431.21057508391));
#127815=CARTESIAN_POINT('Origin',(-17.5667982035458,1078.73142393294,432.310933149585));
#127816=CARTESIAN_POINT('',(-17.5667982035458,1076.73142393294,431.21057508391));
#127817=CARTESIAN_POINT('',(-17.5667982035458,1067.7251047501,431.21057508391));
#127818=CARTESIAN_POINT('Origin',(-17.5667982035458,1076.73142393294,432.310933149585));
#127819=CARTESIAN_POINT('Origin',(-17.5667982035458,1067.7251047501,432.310933149585));
#127820=CARTESIAN_POINT('',(-17.5667982035458,1076.73142393294,431.81057508391));
#127821=CARTESIAN_POINT('Origin',(-17.5667982035458,1076.73142393294,432.310933149585));
#127822=CARTESIAN_POINT('',(-17.5667982035458,1082.7251047501,431.81057508391));
#127823=CARTESIAN_POINT('',(-17.5667982035458,1067.7251047501,431.81057508391));
#127824=CARTESIAN_POINT('Origin',(-17.5667982035458,1082.7251047501,432.310933149585));
#127825=CARTESIAN_POINT('Origin',(-26.104902451872,1067.7251047501,432.972859244816));
#127826=CARTESIAN_POINT('',(-26.104902451872,1078.73142393294,431.758827678079));
#127827=CARTESIAN_POINT('Origin',(-26.104902451872,1078.73142393294,432.972859244816));
#127828=CARTESIAN_POINT('',(-26.104902451872,1076.73142393294,431.758827678079));
#127829=CARTESIAN_POINT('',(-26.104902451872,1067.7251047501,431.758827678079));
#127830=CARTESIAN_POINT('Origin',(-26.104902451872,1076.73142393294,432.972859244816));
#127831=CARTESIAN_POINT('Origin',(-26.104902451872,1067.7251047501,432.972859244816));
#127832=CARTESIAN_POINT('',(-26.104902451872,1076.73142393294,432.358827678079));
#127833=CARTESIAN_POINT('Origin',(-26.104902451872,1076.73142393294,432.972859244816));
#127834=CARTESIAN_POINT('',(-26.104902451872,1082.7251047501,432.358827678079));
#127835=CARTESIAN_POINT('',(-26.104902451872,1067.7251047501,432.358827678079));
#127836=CARTESIAN_POINT('Origin',(-26.104902451872,1082.7251047501,432.972859244816));
#127837=CARTESIAN_POINT('Origin',(-33.9220227392324,1067.7251047501,431.664608453338));
#127838=CARTESIAN_POINT('',(-33.9220227392324,1078.73142393294,430.335800489765));
#127839=CARTESIAN_POINT('Origin',(-33.9220227392324,1078.73142393294,431.664608453338));
#127840=CARTESIAN_POINT('',(-33.9220227392324,1076.73142393294,430.335800489765));
#127841=CARTESIAN_POINT('',(-33.9220227392324,1067.7251047501,430.335800489765));
#127842=CARTESIAN_POINT('Origin',(-33.9220227392324,1076.73142393294,431.664608453338));
#127843=CARTESIAN_POINT('Origin',(-33.9220227392324,1067.7251047501,431.664608453338));
#127844=CARTESIAN_POINT('',(-33.9220227392324,1076.73142393294,430.935800489765));
#127845=CARTESIAN_POINT('Origin',(-33.9220227392324,1076.73142393294,431.664608453338));
#127846=CARTESIAN_POINT('',(-33.9220227392324,1082.7251047501,430.935800489765));
#127847=CARTESIAN_POINT('',(-33.9220227392324,1067.7251047501,430.935800489765));
#127848=CARTESIAN_POINT('Origin',(-33.9220227392324,1082.7251047501,431.664608453338));
#127849=CARTESIAN_POINT('Origin',(-42.6968024226075,1067.7251047501,428.675347967396));
#127850=CARTESIAN_POINT('',(-42.6968024226075,1078.73142393294,427.214230965579));
#127851=CARTESIAN_POINT('Origin',(-42.6968024226075,1078.73142393294,428.675347967396));
#127852=CARTESIAN_POINT('',(-42.6968024226075,1076.73142393294,427.214230965579));
#127853=CARTESIAN_POINT('',(-42.6968024226075,1067.7251047501,427.214230965579));
#127854=CARTESIAN_POINT('Origin',(-42.6968024226075,1076.73142393294,428.675347967396));
#127855=CARTESIAN_POINT('Origin',(-42.6968024226075,1067.7251047501,428.675347967396));
#127856=CARTESIAN_POINT('',(-42.6968024226075,1076.73142393294,427.814230965579));
#127857=CARTESIAN_POINT('Origin',(-42.6968024226075,1076.73142393294,428.675347967396));
#127858=CARTESIAN_POINT('',(-42.6968024226075,1082.7251047501,427.814230965579));
#127859=CARTESIAN_POINT('',(-42.6968024226075,1067.7251047501,427.814230965579));
#127860=CARTESIAN_POINT('Origin',(-42.6968024226075,1082.7251047501,428.675347967396));
#127861=CARTESIAN_POINT('Origin',(-50.1733429030999,1067.7251047501,423.80948031819));
#127862=CARTESIAN_POINT('',(-50.1733429030999,1078.73142393294,422.188998275565));
#127863=CARTESIAN_POINT('Origin',(-50.1733429030999,1078.73142393294,423.80948031819));
#127864=CARTESIAN_POINT('',(-50.1733429030999,1076.73142393294,422.188998275565));
#127865=CARTESIAN_POINT('',(-50.1733429030999,1067.7251047501,422.188998275565));
#127866=CARTESIAN_POINT('Origin',(-50.1733429030999,1076.73142393294,423.80948031819));
#127867=CARTESIAN_POINT('Origin',(-50.1733429030999,1067.7251047501,423.80948031819));
#127868=CARTESIAN_POINT('',(-50.1733429030999,1076.73142393294,422.788998275565));
#127869=CARTESIAN_POINT('Origin',(-50.1733429030999,1076.73142393294,423.80948031819));
#127870=CARTESIAN_POINT('',(-50.1733429030999,1082.7251047501,422.788998275565));
#127871=CARTESIAN_POINT('',(-50.1733429030999,1067.7251047501,422.788998275565));
#127872=CARTESIAN_POINT('Origin',(-50.1733429030999,1082.7251047501,423.80948031819));
#127873=CARTESIAN_POINT('Origin',(-57.9383919970227,1067.7251047501,417.23585017925));
#127874=CARTESIAN_POINT('',(-57.9383919970227,1078.73142393294,415.534849956167));
#127875=CARTESIAN_POINT('Origin',(-57.9383919970227,1078.73142393294,417.23585017925));
#127876=CARTESIAN_POINT('',(-57.9383919970227,1076.73142393294,415.534849956167));
#127877=CARTESIAN_POINT('',(-57.9383919970227,1067.7251047501,415.534849956167));
#127878=CARTESIAN_POINT('Origin',(-57.9383919970227,1076.73142393294,417.23585017925));
#127879=CARTESIAN_POINT('Origin',(-57.9383919970227,1067.7251047501,417.23585017925));
#127880=CARTESIAN_POINT('',(-57.9383919970227,1076.73142393294,416.134849956167));
#127881=CARTESIAN_POINT('Origin',(-57.9383919970227,1076.73142393294,417.23585017925));
#127882=CARTESIAN_POINT('',(-57.9383919970227,1082.7251047501,416.134849956167));
#127883=CARTESIAN_POINT('',(-57.9383919970227,1067.7251047501,416.134849956167));
#127884=CARTESIAN_POINT('Origin',(-57.9383919970227,1082.7251047501,417.23585017925));
#127885=CARTESIAN_POINT('Origin',(-63.8179602450884,1067.7251047501,409.313149239581));
#127886=CARTESIAN_POINT('',(-63.8179602450884,1078.73142393294,407.591874607538));
#127887=CARTESIAN_POINT('Origin',(-63.8179602450884,1078.73142393294,409.313149239581));
#127888=CARTESIAN_POINT('',(-63.8179602450884,1076.73142393294,407.591874607538));
#127889=CARTESIAN_POINT('',(-63.8179602450884,1067.7251047501,407.591874607538));
#127890=CARTESIAN_POINT('Origin',(-63.8179602450884,1076.73142393294,409.313149239581));
#127891=CARTESIAN_POINT('Origin',(-63.8179602450884,1067.7251047501,409.313149239581));
#127892=CARTESIAN_POINT('',(-63.8179602450884,1076.73142393294,408.191874607538));
#127893=CARTESIAN_POINT('Origin',(-63.8179602450884,1076.73142393294,409.313149239581));
#127894=CARTESIAN_POINT('',(-63.8179602450884,1082.7251047501,408.191874607538));
#127895=CARTESIAN_POINT('',(-63.8179602450884,1067.7251047501,408.191874607538));
#127896=CARTESIAN_POINT('Origin',(-63.8179602450884,1082.7251047501,409.313149239581));
#127897=CARTESIAN_POINT('Origin',(-69.5234989093398,1067.7251047501,399.45457083273));
#127898=CARTESIAN_POINT('',(-69.5234989093398,1078.73142393294,397.672578178326));
#127899=CARTESIAN_POINT('Origin',(-69.5234989093398,1078.73142393294,399.45457083273));
#127900=CARTESIAN_POINT('',(-69.5234989093398,1076.73142393294,397.672578178326));
#127901=CARTESIAN_POINT('',(-69.5234989093398,1067.7251047501,397.672578178326));
#127902=CARTESIAN_POINT('Origin',(-69.5234989093398,1076.73142393294,399.45457083273));
#127903=CARTESIAN_POINT('Origin',(-69.5234989093398,1067.7251047501,399.45457083273));
#127904=CARTESIAN_POINT('',(-69.5234989093398,1076.73142393294,398.272578178326));
#127905=CARTESIAN_POINT('Origin',(-69.5234989093398,1076.73142393294,399.45457083273));
#127906=CARTESIAN_POINT('',(-69.5234989093398,1082.7251047501,398.272578178326));
#127907=CARTESIAN_POINT('',(-69.5234989093398,1067.7251047501,398.272578178326));
#127908=CARTESIAN_POINT('Origin',(-69.5234989093398,1082.7251047501,399.45457083273));
#127909=CARTESIAN_POINT('Origin',(-72.9741933816799,1067.7251047501,388.776349944239));
#127910=CARTESIAN_POINT('',(-72.9741933816799,1078.73142393294,387.115469134319));
#127911=CARTESIAN_POINT('Origin',(-72.9741933816799,1078.73142393294,388.776349944239));
#127912=CARTESIAN_POINT('',(-72.9741933816799,1076.73142393294,387.115469134319));
#127913=CARTESIAN_POINT('',(-72.9741933816799,1067.7251047501,387.115469134319));
#127914=CARTESIAN_POINT('Origin',(-72.9741933816799,1076.73142393294,388.776349944239));
#127915=CARTESIAN_POINT('Origin',(-72.9741933816799,1067.7251047501,388.776349944239));
#127916=CARTESIAN_POINT('',(-72.9741933816799,1076.73142393294,387.715469134319));
#127917=CARTESIAN_POINT('Origin',(-72.9741933816799,1076.73142393294,388.776349944239));
#127918=CARTESIAN_POINT('',(-72.9741933816799,1082.7251047501,387.715469134319));
#127919=CARTESIAN_POINT('',(-72.9741933816799,1067.7251047501,387.715469134319));
#127920=CARTESIAN_POINT('Origin',(-72.9741933816799,1082.7251047501,388.776349944239));
#127921=CARTESIAN_POINT('Origin',(-15.5839370354643,1067.7251047501,435.795215825376));
#127922=CARTESIAN_POINT('',(-15.5839370354643,1078.73142393294,434.694857759701));
#127923=CARTESIAN_POINT('Origin',(-15.5839370354643,1078.73142393294,435.795215825376));
#127924=CARTESIAN_POINT('',(-15.5839370354643,1076.73142393294,434.694857759701));
#127925=CARTESIAN_POINT('',(-15.5839370354643,1067.7251047501,434.694857759701));
#127926=CARTESIAN_POINT('Origin',(-15.5839370354643,1076.73142393294,435.795215825376));
#127927=CARTESIAN_POINT('Origin',(-15.5839370354643,1067.7251047501,435.795215825376));
#127928=CARTESIAN_POINT('',(-15.5839370354643,1076.73142393294,435.294857759701));
#127929=CARTESIAN_POINT('Origin',(-15.5839370354643,1076.73142393294,435.795215825376));
#127930=CARTESIAN_POINT('',(-15.5839370354643,1082.7251047501,435.294857759701));
#127931=CARTESIAN_POINT('',(-15.5839370354643,1067.7251047501,435.294857759701));
#127932=CARTESIAN_POINT('Origin',(-15.5839370354643,1082.7251047501,435.795215825376));
#127933=CARTESIAN_POINT('Origin',(-23.7978410471238,1067.7251047501,438.217848937937));
#127934=CARTESIAN_POINT('',(-23.7978410471238,1078.73142393294,437.0038173712));
#127935=CARTESIAN_POINT('Origin',(-23.7978410471238,1078.73142393294,438.217848937937));
#127936=CARTESIAN_POINT('',(-23.7978410471238,1076.73142393294,437.0038173712));
#127937=CARTESIAN_POINT('',(-23.7978410471238,1067.7251047501,437.0038173712));
#127938=CARTESIAN_POINT('Origin',(-23.7978410471238,1076.73142393294,438.217848937937));
#127939=CARTESIAN_POINT('Origin',(-23.7978410471238,1067.7251047501,438.217848937937));
#127940=CARTESIAN_POINT('',(-23.7978410471238,1076.73142393294,437.6038173712));
#127941=CARTESIAN_POINT('Origin',(-23.7978410471238,1076.73142393294,438.217848937937));
#127942=CARTESIAN_POINT('',(-23.7978410471238,1082.7251047501,437.6038173712));
#127943=CARTESIAN_POINT('',(-23.7978410471238,1067.7251047501,437.6038173712));
#127944=CARTESIAN_POINT('Origin',(-23.7978410471238,1082.7251047501,438.217848937937));
#127945=CARTESIAN_POINT('Origin',(-31.7161391349227,1067.7251047501,438.563457261366));
#127946=CARTESIAN_POINT('',(-31.7161391349227,1078.73142393294,437.234649297793));
#127947=CARTESIAN_POINT('Origin',(-31.7161391349227,1078.73142393294,438.563457261366));
#127948=CARTESIAN_POINT('',(-31.7161391349227,1076.73142393294,437.234649297793));
#127949=CARTESIAN_POINT('',(-31.7161391349227,1067.7251047501,437.234649297793));
#127950=CARTESIAN_POINT('Origin',(-31.7161391349227,1076.73142393294,438.563457261366));
#127951=CARTESIAN_POINT('Origin',(-31.7161391349227,1067.7251047501,438.563457261366));
#127952=CARTESIAN_POINT('',(-31.7161391349227,1076.73142393294,437.834649297793));
#127953=CARTESIAN_POINT('Origin',(-31.7161391349227,1076.73142393294,438.563457261366));
#127954=CARTESIAN_POINT('',(-31.7161391349227,1082.7251047501,437.834649297793));
#127955=CARTESIAN_POINT('',(-31.7161391349227,1067.7251047501,437.834649297793));
#127956=CARTESIAN_POINT('Origin',(-31.7161391349227,1082.7251047501,438.563457261366));
#127957=CARTESIAN_POINT('Origin',(-40.9206710311109,1067.7251047501,437.463898569597));
#127958=CARTESIAN_POINT('',(-40.9206710311109,1078.73142393294,436.00278156778));
#127959=CARTESIAN_POINT('Origin',(-40.9206710311109,1078.73142393294,437.463898569597));
#127960=CARTESIAN_POINT('',(-40.9206710311109,1076.73142393294,436.00278156778));
#127961=CARTESIAN_POINT('',(-40.9206710311109,1067.7251047501,436.00278156778));
#127962=CARTESIAN_POINT('Origin',(-40.9206710311109,1076.73142393294,437.463898569597));
#127963=CARTESIAN_POINT('Origin',(-40.9206710311109,1067.7251047501,437.463898569597));
#127964=CARTESIAN_POINT('',(-40.9206710311109,1076.73142393294,436.60278156778));
#127965=CARTESIAN_POINT('Origin',(-40.9206710311109,1076.73142393294,437.463898569597));
#127966=CARTESIAN_POINT('',(-40.9206710311109,1082.7251047501,436.60278156778));
#127967=CARTESIAN_POINT('',(-40.9206710311109,1067.7251047501,436.60278156778));
#127968=CARTESIAN_POINT('Origin',(-40.9206710311109,1082.7251047501,437.463898569597));
#127969=CARTESIAN_POINT('Origin',(-49.2455019341356,1067.7251047501,434.258821975804));
#127970=CARTESIAN_POINT('',(-49.2455019341356,1078.73142393294,432.63833993318));
#127971=CARTESIAN_POINT('Origin',(-49.2455019341356,1078.73142393294,434.258821975804));
#127972=CARTESIAN_POINT('',(-49.2455019341356,1076.73142393294,432.63833993318));
#127973=CARTESIAN_POINT('',(-49.2455019341356,1067.7251047501,432.63833993318));
#127974=CARTESIAN_POINT('Origin',(-49.2455019341356,1076.73142393294,434.258821975804));
#127975=CARTESIAN_POINT('Origin',(-49.2455019341356,1067.7251047501,434.258821975804));
#127976=CARTESIAN_POINT('',(-49.2455019341356,1076.73142393294,433.23833993318));
#127977=CARTESIAN_POINT('Origin',(-49.2455019341356,1076.73142393294,434.258821975804));
#127978=CARTESIAN_POINT('',(-49.2455019341356,1082.7251047501,433.23833993318));
#127979=CARTESIAN_POINT('',(-49.2455019341356,1067.7251047501,433.23833993318));
#127980=CARTESIAN_POINT('Origin',(-49.2455019341356,1082.7251047501,434.258821975804));
#127981=CARTESIAN_POINT('Origin',(-58.207600631934,1067.7251047501,429.443285913689));
#127982=CARTESIAN_POINT('',(-58.207600631934,1078.73142393294,427.742285690606));
#127983=CARTESIAN_POINT('Origin',(-58.207600631934,1078.73142393294,429.443285913689));
#127984=CARTESIAN_POINT('',(-58.207600631934,1076.73142393294,427.742285690606));
#127985=CARTESIAN_POINT('',(-58.207600631934,1067.7251047501,427.742285690606));
#127986=CARTESIAN_POINT('Origin',(-58.207600631934,1076.73142393294,429.443285913689));
#127987=CARTESIAN_POINT('Origin',(-58.207600631934,1067.7251047501,429.443285913689));
#127988=CARTESIAN_POINT('',(-58.207600631934,1076.73142393294,428.342285690606));
#127989=CARTESIAN_POINT('Origin',(-58.207600631934,1076.73142393294,429.443285913689));
#127990=CARTESIAN_POINT('',(-58.207600631934,1082.7251047501,428.342285690606));
#127991=CARTESIAN_POINT('',(-58.207600631934,1067.7251047501,428.342285690606));
#127992=CARTESIAN_POINT('Origin',(-58.207600631934,1082.7251047501,429.443285913689));
#127993=CARTESIAN_POINT('Origin',(-65.60590835534,1067.7251047501,422.916145973955));
#127994=CARTESIAN_POINT('',(-65.60590835534,1078.73142393294,421.194871341911));
#127995=CARTESIAN_POINT('Origin',(-65.60590835534,1078.73142393294,422.916145973955));
#127996=CARTESIAN_POINT('',(-65.60590835534,1076.73142393294,421.194871341911));
#127997=CARTESIAN_POINT('',(-65.60590835534,1067.7251047501,421.194871341911));
#127998=CARTESIAN_POINT('Origin',(-65.60590835534,1076.73142393294,422.916145973955));
#127999=CARTESIAN_POINT('Origin',(-65.60590835534,1067.7251047501,422.916145973955));
#128000=CARTESIAN_POINT('',(-65.60590835534,1076.73142393294,421.794871341911));
#128001=CARTESIAN_POINT('Origin',(-65.60590835534,1076.73142393294,422.916145973955));
#128002=CARTESIAN_POINT('',(-65.60590835534,1082.7251047501,421.794871341911));
#128003=CARTESIAN_POINT('',(-65.60590835534,1067.7251047501,421.794871341911));
#128004=CARTESIAN_POINT('Origin',(-65.60590835534,1082.7251047501,422.916145973955));
#128005=CARTESIAN_POINT('Origin',(-73.2364810162993,1067.7251047501,414.459249349358));
#128006=CARTESIAN_POINT('',(-73.2364810162993,1078.73142393294,412.677256694953));
#128007=CARTESIAN_POINT('Origin',(-73.2364810162993,1078.73142393294,414.459249349358));
#128008=CARTESIAN_POINT('',(-73.2364810162993,1076.73142393294,412.677256694953));
#128009=CARTESIAN_POINT('',(-73.2364810162993,1067.7251047501,412.677256694953));
#128010=CARTESIAN_POINT('Origin',(-73.2364810162993,1076.73142393294,414.459249349358));
#128011=CARTESIAN_POINT('Origin',(-73.2364810162993,1067.7251047501,414.459249349358));
#128012=CARTESIAN_POINT('',(-73.2364810162993,1076.73142393294,413.277256694953));
#128013=CARTESIAN_POINT('Origin',(-73.2364810162993,1076.73142393294,414.459249349358));
#128014=CARTESIAN_POINT('',(-73.2364810162993,1082.7251047501,413.277256694953));
#128015=CARTESIAN_POINT('',(-73.2364810162993,1067.7251047501,413.277256694953));
#128016=CARTESIAN_POINT('Origin',(-73.2364810162993,1082.7251047501,414.459249349358));
#128017=CARTESIAN_POINT('Origin',(-78.8318964951359,1067.7251047501,404.731812929415));
#128018=CARTESIAN_POINT('',(-78.8318964951359,1078.73142393294,403.070932119494));
#128019=CARTESIAN_POINT('Origin',(-78.8318964951359,1078.73142393294,404.731812929415));
#128020=CARTESIAN_POINT('',(-78.8318964951359,1076.73142393294,403.070932119494));
#128021=CARTESIAN_POINT('',(-78.8318964951359,1067.7251047501,403.070932119494));
#128022=CARTESIAN_POINT('Origin',(-78.8318964951359,1076.73142393294,404.731812929415));
#128023=CARTESIAN_POINT('Origin',(-78.8318964951359,1067.7251047501,404.731812929415));
#128024=CARTESIAN_POINT('',(-78.8318964951359,1076.73142393294,403.670932119494));
#128025=CARTESIAN_POINT('Origin',(-78.8318964951359,1076.73142393294,404.731812929415));
#128026=CARTESIAN_POINT('',(-78.8318964951359,1082.7251047501,403.670932119494));
#128027=CARTESIAN_POINT('',(-78.8318964951359,1067.7251047501,403.670932119494));
#128028=CARTESIAN_POINT('Origin',(-78.8318964951359,1082.7251047501,404.731812929415));
#128029=CARTESIAN_POINT('Origin',(-12.9199830389064,1067.7251047501,438.791098546867));
#128030=CARTESIAN_POINT('',(-12.9199830389064,1078.73142393294,437.690740481192));
#128031=CARTESIAN_POINT('Origin',(-12.9199830389064,1078.73142393294,438.791098546867));
#128032=CARTESIAN_POINT('',(-12.9199830389064,1076.73142393294,437.690740481192));
#128033=CARTESIAN_POINT('',(-12.9199830389064,1067.7251047501,437.690740481192));
#128034=CARTESIAN_POINT('Origin',(-12.9199830389064,1076.73142393294,438.791098546867));
#128035=CARTESIAN_POINT('Origin',(-12.9199830389064,1067.7251047501,438.791098546867));
#128036=CARTESIAN_POINT('',(-12.9199830389064,1076.73142393294,438.290740481192));
#128037=CARTESIAN_POINT('Origin',(-12.9199830389064,1076.73142393294,438.791098546867));
#128038=CARTESIAN_POINT('',(-12.9199830389064,1082.7251047501,438.290740481192));
#128039=CARTESIAN_POINT('',(-12.9199830389064,1067.7251047501,438.290740481192));
#128040=CARTESIAN_POINT('Origin',(-12.9199830389064,1082.7251047501,438.791098546867));
#128041=CARTESIAN_POINT('Origin',(-20.4506997939053,1067.7251047501,442.868557984656));
#128042=CARTESIAN_POINT('',(-20.4506997939053,1078.73142393294,441.654526417919));
#128043=CARTESIAN_POINT('Origin',(-20.4506997939053,1078.73142393294,442.868557984656));
#128044=CARTESIAN_POINT('',(-20.4506997939053,1076.73142393294,441.654526417919));
#128045=CARTESIAN_POINT('',(-20.4506997939053,1067.7251047501,441.654526417919));
#128046=CARTESIAN_POINT('Origin',(-20.4506997939053,1076.73142393294,442.868557984656));
#128047=CARTESIAN_POINT('Origin',(-20.4506997939053,1067.7251047501,442.868557984656));
#128048=CARTESIAN_POINT('',(-20.4506997939053,1076.73142393294,442.254526417919));
#128049=CARTESIAN_POINT('Origin',(-20.4506997939053,1076.73142393294,442.868557984656));
#128050=CARTESIAN_POINT('',(-20.4506997939053,1082.7251047501,442.254526417919));
#128051=CARTESIAN_POINT('',(-20.4506997939053,1067.7251047501,442.254526417919));
#128052=CARTESIAN_POINT('Origin',(-20.4506997939053,1082.7251047501,442.868557984656));
#128053=CARTESIAN_POINT('Origin',(-28.1241080594961,1067.7251047501,444.852920680845));
#128054=CARTESIAN_POINT('',(-28.1241080594961,1078.73142393294,443.524112717272));
#128055=CARTESIAN_POINT('Origin',(-28.1241080594961,1078.73142393294,444.852920680845));
#128056=CARTESIAN_POINT('',(-28.1241080594961,1076.73142393294,443.524112717272));
#128057=CARTESIAN_POINT('',(-28.1241080594961,1067.7251047501,443.524112717272));
#128058=CARTESIAN_POINT('Origin',(-28.1241080594961,1076.73142393294,444.852920680845));
#128059=CARTESIAN_POINT('Origin',(-28.1241080594961,1067.7251047501,444.852920680845));
#128060=CARTESIAN_POINT('',(-28.1241080594961,1076.73142393294,444.124112717272));
#128061=CARTESIAN_POINT('Origin',(-28.1241080594961,1076.73142393294,444.852920680845));
#128062=CARTESIAN_POINT('',(-28.1241080594961,1082.7251047501,444.124112717272));
#128063=CARTESIAN_POINT('',(-28.1241080594961,1067.7251047501,444.124112717272));
#128064=CARTESIAN_POINT('Origin',(-28.1241080594961,1082.7251047501,444.852920680845));
#128065=CARTESIAN_POINT('Origin',(-37.3561099563896,1067.7251047501,445.691119774347));
#128066=CARTESIAN_POINT('',(-37.3561099563896,1078.73142393294,444.23000277253));
#128067=CARTESIAN_POINT('Origin',(-37.3561099563896,1078.73142393294,445.691119774347));
#128068=CARTESIAN_POINT('',(-37.3561099563896,1076.73142393294,444.23000277253));
#128069=CARTESIAN_POINT('',(-37.3561099563896,1067.7251047501,444.23000277253));
#128070=CARTESIAN_POINT('Origin',(-37.3561099563896,1076.73142393294,445.691119774347));
#128071=CARTESIAN_POINT('Origin',(-37.3561099563896,1067.7251047501,445.691119774347));
#128072=CARTESIAN_POINT('',(-37.3561099563896,1076.73142393294,444.83000277253));
#128073=CARTESIAN_POINT('Origin',(-37.3561099563896,1076.73142393294,445.691119774347));
#128074=CARTESIAN_POINT('',(-37.3561099563896,1082.7251047501,444.83000277253));
#128075=CARTESIAN_POINT('',(-37.3561099563896,1067.7251047501,444.83000277253));
#128076=CARTESIAN_POINT('Origin',(-37.3561099563896,1082.7251047501,445.691119774347));
#128077=CARTESIAN_POINT('Origin',(-46.1653962245135,1067.7251047501,444.286911462781));
#128078=CARTESIAN_POINT('',(-46.1653962245135,1078.73142393294,442.666429420156));
#128079=CARTESIAN_POINT('Origin',(-46.1653962245135,1078.73142393294,444.286911462781));
#128080=CARTESIAN_POINT('',(-46.1653962245135,1076.73142393294,442.666429420156));
#128081=CARTESIAN_POINT('',(-46.1653962245135,1067.7251047501,442.666429420156));
#128082=CARTESIAN_POINT('Origin',(-46.1653962245135,1076.73142393294,444.286911462781));
#128083=CARTESIAN_POINT('Origin',(-46.1653962245135,1067.7251047501,444.286911462781));
#128084=CARTESIAN_POINT('',(-46.1653962245135,1076.73142393294,443.266429420156));
#128085=CARTESIAN_POINT('Origin',(-46.1653962245135,1076.73142393294,444.286911462781));
#128086=CARTESIAN_POINT('',(-46.1653962245135,1082.7251047501,443.266429420156));
#128087=CARTESIAN_POINT('',(-46.1653962245135,1067.7251047501,443.266429420156));
#128088=CARTESIAN_POINT('Origin',(-46.1653962245135,1082.7251047501,444.286911462781));
#128089=CARTESIAN_POINT('Origin',(-55.9328578081729,1067.7251047501,441.43993151091));
#128090=CARTESIAN_POINT('',(-55.9328578081729,1078.73142393294,439.738931287827));
#128091=CARTESIAN_POINT('Origin',(-55.9328578081729,1078.73142393294,441.43993151091));
#128092=CARTESIAN_POINT('',(-55.9328578081729,1076.73142393294,439.738931287827));
#128093=CARTESIAN_POINT('',(-55.9328578081729,1067.7251047501,439.738931287827));
#128094=CARTESIAN_POINT('Origin',(-55.9328578081729,1076.73142393294,441.43993151091));
#128095=CARTESIAN_POINT('Origin',(-55.9328578081729,1067.7251047501,441.43993151091));
#128096=CARTESIAN_POINT('',(-55.9328578081729,1076.73142393294,440.338931287827));
#128097=CARTESIAN_POINT('Origin',(-55.9328578081729,1076.73142393294,441.43993151091));
#128098=CARTESIAN_POINT('',(-55.9328578081729,1082.7251047501,440.338931287827));
#128099=CARTESIAN_POINT('',(-55.9328578081729,1067.7251047501,440.338931287827));
#128100=CARTESIAN_POINT('Origin',(-55.9328578081729,1082.7251047501,441.43993151091));
#128101=CARTESIAN_POINT('Origin',(-64.5265634583872,1067.7251047501,436.593619907169));
#128102=CARTESIAN_POINT('',(-64.5265634583872,1078.73142393294,434.872345275125));
#128103=CARTESIAN_POINT('Origin',(-64.5265634583872,1078.73142393294,436.593619907169));
#128104=CARTESIAN_POINT('',(-64.5265634583872,1076.73142393294,434.872345275125));
#128105=CARTESIAN_POINT('',(-64.5265634583872,1067.7251047501,434.872345275125));
#128106=CARTESIAN_POINT('Origin',(-64.5265634583872,1076.73142393294,436.593619907169));
#128107=CARTESIAN_POINT('Origin',(-64.5265634583872,1067.7251047501,436.593619907169));
#128108=CARTESIAN_POINT('',(-64.5265634583872,1076.73142393294,435.472345275125));
#128109=CARTESIAN_POINT('Origin',(-64.5265634583872,1076.73142393294,436.593619907169));
#128110=CARTESIAN_POINT('',(-64.5265634583872,1082.7251047501,435.472345275125));
#128111=CARTESIAN_POINT('',(-64.5265634583872,1067.7251047501,435.472345275125));
#128112=CARTESIAN_POINT('Origin',(-64.5265634583872,1082.7251047501,436.593619907169));
#128113=CARTESIAN_POINT('Origin',(-73.7486774752203,1067.7251047501,429.908012028014));
#128114=CARTESIAN_POINT('',(-73.7486774752203,1078.73142393294,428.126019373609));
#128115=CARTESIAN_POINT('Origin',(-73.7486774752203,1078.73142393294,429.908012028014));
#128116=CARTESIAN_POINT('',(-73.7486774752203,1076.73142393294,428.126019373609));
#128117=CARTESIAN_POINT('',(-73.7486774752203,1067.7251047501,428.126019373609));
#128118=CARTESIAN_POINT('Origin',(-73.7486774752203,1076.73142393294,429.908012028014));
#128119=CARTESIAN_POINT('Origin',(-73.7486774752203,1067.7251047501,429.908012028014));
#128120=CARTESIAN_POINT('',(-73.7486774752203,1076.73142393294,428.726019373609));
#128121=CARTESIAN_POINT('Origin',(-73.7486774752203,1076.73142393294,429.908012028014));
#128122=CARTESIAN_POINT('',(-73.7486774752203,1082.7251047501,428.726019373609));
#128123=CARTESIAN_POINT('',(-73.7486774752203,1067.7251047501,428.726019373609));
#128124=CARTESIAN_POINT('Origin',(-73.7486774752203,1082.7251047501,429.908012028014));
#128125=CARTESIAN_POINT('Origin',(-81.2442674543458,1067.7251047501,421.556495725588));
#128126=CARTESIAN_POINT('',(-81.2442674543458,1078.73142393294,419.895614915668));
#128127=CARTESIAN_POINT('Origin',(-81.2442674543458,1078.73142393294,421.556495725588));
#128128=CARTESIAN_POINT('',(-81.2442674543458,1076.73142393294,419.895614915668));
#128129=CARTESIAN_POINT('',(-81.2442674543458,1067.7251047501,419.895614915668));
#128130=CARTESIAN_POINT('Origin',(-81.2442674543458,1076.73142393294,421.556495725588));
#128131=CARTESIAN_POINT('Origin',(-81.2442674543458,1067.7251047501,421.556495725588));
#128132=CARTESIAN_POINT('',(-81.2442674543458,1076.73142393294,420.495614915667));
#128133=CARTESIAN_POINT('Origin',(-81.2442674543458,1076.73142393294,421.556495725588));
#128134=CARTESIAN_POINT('',(-81.2442674543458,1082.7251047501,420.495614915667));
#128135=CARTESIAN_POINT('',(-81.2442674543458,1067.7251047501,420.495614915667));
#128136=CARTESIAN_POINT('Origin',(-81.2442674543458,1082.7251047501,421.556495725588));
#128137=CARTESIAN_POINT('Origin',(0.,1074.88309437944,424.620242579854));
#128138=CARTESIAN_POINT('',(-1.56039672537847E-14,1074.88309437944,552.036304620344));
#128139=CARTESIAN_POINT('Origin',(-1.55427349138273E-14,1074.88309437944,
551.536304620344));
#128140=CARTESIAN_POINT('Origin',(0.,1074.88309437944,424.620242579854));
#128141=CARTESIAN_POINT('Origin',(0.,1074.39201604106,424.620242579854));
#128142=CARTESIAN_POINT('Origin',(0.,1118.16413742548,424.620242579854));
#128143=CARTESIAN_POINT('',(-1.56039672537847E-14,1075.04643807976,552.036304620344));
#128144=CARTESIAN_POINT('',(-1.56039672537847E-14,1118.16413742548,552.036304620344));
#128145=CARTESIAN_POINT('Origin',(0.,1075.04643807976,424.620242579854));
#128146=CARTESIAN_POINT('Origin',(0.,1122.00270384563,424.620242579854));
#128147=CARTESIAN_POINT('',(-1.45329701922362E-15,1121.50270384563,436.487313315967));
#128148=CARTESIAN_POINT('Origin',(0.,1121.50270384563,424.620242579854));
#128149=CARTESIAN_POINT('',(-1.51452935918098E-15,1122.00270384563,436.987313315967));
#128150=CARTESIAN_POINT('Origin',(-1.45329701922361E-15,1122.00270384563,
436.487313315967));
#128151=CARTESIAN_POINT('',(1.51452935918099E-15,1122.00270384563,412.253171843741));
#128152=CARTESIAN_POINT('Origin',(0.,1122.00270384563,424.620242579854));
#128153=CARTESIAN_POINT('Origin',(0.,1122.00270384563,424.620242579854));
#128154=CARTESIAN_POINT('Origin',(0.,1133.64517683891,424.620242579854));
#128155=CARTESIAN_POINT('',(-1.45329701922361E-15,1134.14517683891,412.753171843741));
#128156=CARTESIAN_POINT('Origin',(0.,1134.14517683891,424.620242579854));
#128157=CARTESIAN_POINT('',(-1.51452935918099E-15,1133.64517683891,412.253171843741));
#128158=CARTESIAN_POINT('Origin',(-1.45329701922361E-15,1133.64517683891,
412.753171843741));
#128159=CARTESIAN_POINT('Origin',(0.,1133.64517683891,424.620242579854));
#128160=CARTESIAN_POINT('Origin',(0.,1134.14517683891,424.620242579854));
#128161=CARTESIAN_POINT('',(-1.51452935918099E-15,1134.14517683891,412.253171843741));
#128162=CARTESIAN_POINT('Origin',(0.,1109.29344889777,424.620242579854));
#128163=CARTESIAN_POINT('',(0.,1118.15413742548,435.663222162066));
#128164=CARTESIAN_POINT('Origin',(0.,1118.15413742548,424.620242579854));
#128165=CARTESIAN_POINT('Origin',(0.,1117.65413742548,424.620242579854));
#128166=CARTESIAN_POINT('',(-2.03875185873375E-15,1117.69439144477,441.267914873231));
#128167=CARTESIAN_POINT('Origin',(0.,1117.69439144477,424.620242579854));
#128168=CARTESIAN_POINT('',(-1.97771828143355E-15,1118.15413742548,440.769537893495));
#128169=CARTESIAN_POINT('Origin',(-1.97771828143355E-15,1117.65413742548,
440.769537893495));
#128170=CARTESIAN_POINT('Origin',(0.,1118.15413742548,424.620242579854));
#128171=CARTESIAN_POINT('Origin',(0.,1075.18041267597,424.620242579854));
#128172=CARTESIAN_POINT('',(-1.59204083889156E-14,1075.18041267597,294.620242579854));
#128173=CARTESIAN_POINT('Origin',(0.,1075.18041267597,424.620242579854));
#128174=CARTESIAN_POINT('',(-1.57979437090009E-14,1074.18041267597,295.620242579854));
#128175=CARTESIAN_POINT('Origin',(-1.57979437090009E-14,1075.18041267597,
295.620242579854));
#128176=CARTESIAN_POINT('Origin',(0.,1074.18041267597,424.620242579854));
#128177=CARTESIAN_POINT('Origin',(0.,1075.04643807976,424.620242579854));
#128178=CARTESIAN_POINT('',(-1.5665199593742E-14,1074.18041267597,552.536304620344));
#128179=CARTESIAN_POINT('Origin',(-1.57264319336994E-14,1075.04643807976,
553.036304620344));
#128180=CARTESIAN_POINT('Origin',(0.,1074.18041267597,424.620242579854));
#128181=CARTESIAN_POINT('Origin',(0.,1094.6328882123,424.620242579854));
#128182=CARTESIAN_POINT('',(-2.2668647037689E-15,1094.6328882123,443.130597609134));
#128183=CARTESIAN_POINT('Origin',(0.,1094.6328882123,424.620242579854));
#128184=CARTESIAN_POINT('',(-2.2668647037689E-15,1094.6328882123,443.130597609134));
#128185=CARTESIAN_POINT('Origin',(0.,1093.6328882123,424.620242579854));
#128186=CARTESIAN_POINT('',(1.59204083889156E-14,1093.6328882123,294.620242579854));
#128187=CARTESIAN_POINT('',(-1.59204083889156E-14,1093.6328882123,554.620242579854));
#128188=CARTESIAN_POINT('Origin',(0.,1093.6328882123,424.620242579854));
#128189=CARTESIAN_POINT('Origin',(0.,1093.6328882123,424.620242579854));
#128190=CARTESIAN_POINT('',(-1.57979437090009E-14,1094.6328882123,553.620242579854));
#128191=CARTESIAN_POINT('Origin',(-1.57979437090009E-14,1093.6328882123,
553.620242579854));
#128192=CARTESIAN_POINT('Origin',(0.,1094.6328882123,424.620242579854));
#128193=CARTESIAN_POINT('Origin',(0.,1118.15413742548,424.620242579854));
#128194=CARTESIAN_POINT('',(-1.59204083889156E-14,1118.15413742548,294.620242579854));
#128195=CARTESIAN_POINT('Origin',(-89.3961860936676,1067.7251047501,430.005244031937));
#128196=CARTESIAN_POINT('',(-89.3961860936676,1076.67140064346,430.88354716413));
#128197=CARTESIAN_POINT('',(-89.3961860936687,1076.67415347727,429.126940899744));
#128198=CARTESIAN_POINT('Ctrl Pts',(-89.3961860936676,1076.67140064346,
430.88354716413));
#128199=CARTESIAN_POINT('Ctrl Pts',(-89.405023436492,1076.67116823115,430.88354716413));
#128200=CARTESIAN_POINT('Ctrl Pts',(-89.4138630014268,1076.67093534602,
430.883413784404));
#128201=CARTESIAN_POINT('Ctrl Pts',(-89.5390342024466,1076.66763180858,
430.879633183896));
#128202=CARTESIAN_POINT('Ctrl Pts',(-89.6535182774614,1076.66453579198,
430.853031166677));
#128203=CARTESIAN_POINT('Ctrl Pts',(-89.8643186271013,1076.65875455185,
430.75725940252));
#128204=CARTESIAN_POINT('Ctrl Pts',(-89.9587775668252,1076.65612353728,
430.689473083606));
#128205=CARTESIAN_POINT('Ctrl Pts',(-90.1161258498771,1076.65176824399,
430.521339609659));
#128206=CARTESIAN_POINT('Ctrl Pts',(-90.1775034223224,1076.65008833703,
430.422634332581));
#128207=CARTESIAN_POINT('Ctrl Pts',(-90.2586432415134,1076.64801435652,
430.207265590749));
#128208=CARTESIAN_POINT('Ctrl Pts',(-90.2776597841645,1076.64764053423,
430.092708970466));
#128209=CARTESIAN_POINT('Ctrl Pts',(-90.2704609974862,1076.64828460326,
429.862893265806));
#128210=CARTESIAN_POINT('Ctrl Pts',(-90.2443592853713,1076.64929444614,
429.749861592639));
#128211=CARTESIAN_POINT('Ctrl Pts',(-90.1501312341865,1076.65251178129,
429.540291536694));
#128212=CARTESIAN_POINT('Ctrl Pts',(-90.0829218230843,1076.65468593256,
429.445776131215));
#128213=CARTESIAN_POINT('Ctrl Pts',(-89.9159003371264,1076.65980500206,
429.287940991561));
#128214=CARTESIAN_POINT('Ctrl Pts',(-89.8176790713377,1076.66269844556,
429.226162629292));
#128215=CARTESIAN_POINT('Ctrl Pts',(-89.6605146832878,1076.66710802558,
429.165961206007));
#128216=CARTESIAN_POINT('Ctrl Pts',(-89.6090347504715,1076.66852301801,
429.151452089803));
#128217=CARTESIAN_POINT('Ctrl Pts',(-89.5036687283435,1076.67135652926,
429.131884096841));
#128218=CARTESIAN_POINT('Ctrl Pts',(-89.4499887326727,1076.67276900264,
429.12694142144));
#128219=CARTESIAN_POINT('Ctrl Pts',(-89.396194610801,1076.67415325811,429.126940899785));
#128220=CARTESIAN_POINT('',(-89.3961860936676,1082.7251047501,429.126940899744));
#128221=CARTESIAN_POINT('',(-89.3961860936676,1067.7251047501,429.126940899744));
#128222=CARTESIAN_POINT('Origin',(-89.3961860936676,1082.7251047501,430.005244031937));
#128223=CARTESIAN_POINT('Ctrl Pts',(-89.3961860936707,1076.67415347727,
429.126940899744));
#128224=CARTESIAN_POINT('Ctrl Pts',(-89.2796210199493,1076.67715297711,
429.126940899743));
#128225=CARTESIAN_POINT('Ctrl Pts',(-89.1642164309715,1076.67997334784,
429.150143740078));
#128226=CARTESIAN_POINT('Ctrl Pts',(-88.9493848859387,1076.68498184303,
429.240178986333));
#128227=CARTESIAN_POINT('Ctrl Pts',(-88.8520628226455,1076.68712361318,
429.306038141905));
#128228=CARTESIAN_POINT('Ctrl Pts',(-88.6884166218447,1076.6905664082,429.472203861829));
#128229=CARTESIAN_POINT('Ctrl Pts',(-88.6238554495119,1076.69183261313,
429.570989421663));
#128230=CARTESIAN_POINT('Ctrl Pts',(-88.5370000408771,1076.69341471635,
429.788484763094));
#128231=CARTESIAN_POINT('Ctrl Pts',(-88.5157580119964,1076.6937126517,429.905083111817));
#128232=CARTESIAN_POINT('Ctrl Pts',(-88.5203404525082,1076.69331570962,
430.139583869797));
#128233=CARTESIAN_POINT('Ctrl Pts',(-88.5460623157962,1076.69262548977,
430.255126137273));
#128234=CARTESIAN_POINT('Ctrl Pts',(-88.6410887384043,1076.69027838736,
430.468755941952));
#128235=CARTESIAN_POINT('Ctrl Pts',(-88.7092298410642,1076.68864710353,
430.564800713523));
#128236=CARTESIAN_POINT('Ctrl Pts',(-88.8788436280051,1076.68453246604,
430.724487658119));
#128237=CARTESIAN_POINT('Ctrl Pts',(-88.9785650294521,1076.68208877619,
430.7866172519));
#128238=CARTESIAN_POINT('Ctrl Pts',(-89.1408075113255,1076.67800408912,
430.847528149199));
#128239=CARTESIAN_POINT('Ctrl Pts',(-89.1959526202103,1076.67660009373,
430.862312884638));
#128240=CARTESIAN_POINT('Ctrl Pts',(-89.2997610432547,1076.67392404207,
430.879571908049));
#128241=CARTESIAN_POINT('Ctrl Pts',(-89.3479404563299,1076.67266945018,
430.88354716413));
#128242=CARTESIAN_POINT('Ctrl Pts',(-89.3961860936676,1076.67140064346,
430.88354716413));
#128243=CARTESIAN_POINT('Origin',(-89.3961860936676,1067.7251047501,430.005244031937));
#128244=CARTESIAN_POINT('',(-89.3961860936954,1076.6748778677,428.526940899743));
#128245=CARTESIAN_POINT('',(-89.3961860936676,1067.7251047501,428.526940899744));
#128246=CARTESIAN_POINT('Ctrl Pts',(-89.396310882001,1076.6702336653,431.483547158863));
#128247=CARTESIAN_POINT('Ctrl Pts',(-89.5922242330258,1076.66503522431,
431.483530621186));
#128248=CARTESIAN_POINT('Ctrl Pts',(-89.786193582667,1076.65963369298,431.444568941278));
#128249=CARTESIAN_POINT('Ctrl Pts',(-90.1458826936886,1076.64929134132,
431.294031807984));
#128250=CARTESIAN_POINT('Ctrl Pts',(-90.3083768514711,1076.64445312791,
431.184623642052));
#128251=CARTESIAN_POINT('Ctrl Pts',(-90.5817833137706,1076.63627341402,
430.90932457426));
#128252=CARTESIAN_POINT('Ctrl Pts',(-90.6900606418802,1076.63301783246,
430.746123907287));
#128253=CARTESIAN_POINT('Ctrl Pts',(-90.8372870058146,1076.62883349518,
430.387498136413));
#128254=CARTESIAN_POINT('Ctrl Pts',(-90.8749203854877,1076.62794565169,
430.195609537752));
#128255=CARTESIAN_POINT('Ctrl Pts',(-90.8740514734311,1076.62876031399,
429.808623023054));
#128256=CARTESIAN_POINT('Ctrl Pts',(-90.8357080596201,1076.63044894684,
429.61728140158));
#128257=CARTESIAN_POINT('Ctrl Pts',(-90.6876309142824,1076.63603781517,
429.260360231857));
#128258=CARTESIAN_POINT('Ctrl Pts',(-90.5793801275754,1076.63987714276,
429.098204129196));
#128259=CARTESIAN_POINT('Ctrl Pts',(-90.3065942273166,1076.64890226726,
428.824617633557));
#128260=CARTESIAN_POINT('Ctrl Pts',(-90.1446436506629,1076.65399508226,
428.715854129427));
#128261=CARTESIAN_POINT('Ctrl Pts',(-89.8772431317426,1076.66184606648,
428.604067161451));
#128262=CARTESIAN_POINT('Ctrl Pts',(-89.7846756756862,1076.66448013638,
428.575632748052));
#128263=CARTESIAN_POINT('Ctrl Pts',(-89.5953138101581,1076.66968566528,
428.537231028037));
#128264=CARTESIAN_POINT('Ctrl Pts',(-89.4989728558646,1076.67224455488,
428.527357176248));
#128265=CARTESIAN_POINT('Ctrl Pts',(-89.2067578975014,1076.67973121083,
428.5261371014));
#128266=CARTESIAN_POINT('Ctrl Pts',(-89.0129151656653,1076.68431790559,
428.564149733114));
#128267=CARTESIAN_POINT('Ctrl Pts',(-88.652142016831,1076.69224877693,428.713083425865));
#128268=CARTESIAN_POINT('Ctrl Pts',(-88.4886162547277,1076.69552734412,
428.822194499984));
#128269=CARTESIAN_POINT('Ctrl Pts',(-88.2125818772706,1076.70070586114,
429.098194867347));
#128270=CARTESIAN_POINT('Ctrl Pts',(-88.1030544639645,1076.70255649978,
429.262631847192));
#128271=CARTESIAN_POINT('Ctrl Pts',(-87.9539426673206,1076.70488424405,
429.625695227485));
#128272=CARTESIAN_POINT('Ctrl Pts',(-87.9162748479842,1076.70533563943,
429.820887429998));
#128273=CARTESIAN_POINT('Ctrl Pts',(-87.9195938260601,1076.70485327614,
430.214251499443));
#128274=CARTESIAN_POINT('Ctrl Pts',(-87.9604298910247,1076.70392505077,
430.408493855319));
#128275=CARTESIAN_POINT('Ctrl Pts',(-88.1151305771591,1076.70061930047,
430.76838028918));
#128276=CARTESIAN_POINT('Ctrl Pts',(-88.2269711146128,1076.69827684766,
430.930668302977));
#128277=CARTESIAN_POINT('Ctrl Pts',(-88.5069220174034,1076.6921230587,431.202126228349));
#128278=CARTESIAN_POINT('Ctrl Pts',(-88.6721722242147,1076.68836681521,
431.308744036377));
#128279=CARTESIAN_POINT('Ctrl Pts',(-88.9391143575598,1076.68192578571,
431.414135149626));
#128280=CARTESIAN_POINT('Ctrl Pts',(-89.0278915873782,1076.67973295163,
431.43990320465));
#128281=CARTESIAN_POINT('Ctrl Pts',(-89.2100593557822,1076.67511974181,
431.474743718238));
#128282=CARTESIAN_POINT('Ctrl Pts',(-89.3030821256448,1076.67270743334,
431.483555028603));
#128283=CARTESIAN_POINT('Ctrl Pts',(-89.396310882001,1076.6702336653,431.483547158863));
#128284=CARTESIAN_POINT('Ctrl Pts',(-90.9758547056989,1076.62738724384,
428.575583521194));
#128285=CARTESIAN_POINT('Ctrl Pts',(-90.9317360093904,1076.62738724384,
429.590347144532));
#128286=CARTESIAN_POINT('Ctrl Pts',(-90.8706467446144,1076.62738724384,
430.604230654776));
#128287=CARTESIAN_POINT('Ctrl Pts',(-90.7926040105104,1076.62738724384,
431.616950261709));
#128288=CARTESIAN_POINT('Ctrl Pts',(-89.9667063292985,1076.66219983996,
428.531708957971));
#128289=CARTESIAN_POINT('Ctrl Pts',(-89.9230770190023,1076.66219983996,
429.535216330228));
#128290=CARTESIAN_POINT('Ctrl Pts',(-89.8626653860283,1076.66219983996,
430.537853352032));
#128291=CARTESIAN_POINT('Ctrl Pts',(-89.7854883398441,1076.66219983996,
431.539339381107));
#128292=CARTESIAN_POINT('Ctrl Pts',(-88.9650760950845,1076.68827166653,
428.488161259669));
#128293=CARTESIAN_POINT('Ctrl Pts',(-88.9219325248811,1076.68827166653,
429.480496239767));
#128294=CARTESIAN_POINT('Ctrl Pts',(-88.8621934753611,1076.68827166653,
430.471970559324));
#128295=CARTESIAN_POINT('Ctrl Pts',(-88.785875667733,1076.68827166653,431.462306700548));
#128296=CARTESIAN_POINT('Ctrl Pts',(-87.9709679881959,1076.70560884642,
428.44494059955));
#128297=CARTESIAN_POINT('Ctrl Pts',(-87.9283065102335,1076.70560884642,
429.426187090864));
#128298=CARTESIAN_POINT('Ctrl Pts',(-87.8692349931434,1076.70560884642,
430.406582538776));
#128299=CARTESIAN_POINT('Ctrl Pts',(-87.7937699712892,1076.70560884642,
431.385852526519));
#128300=CARTESIAN_POINT('Origin',(0.,1082.7251047501,424.620242579854));
#128301=CARTESIAN_POINT('Origin',(0.,1074.18041267597,296.704180539364));
#128302=CARTESIAN_POINT('Origin',(0.,1094.6328882123,294.620242579854));
#128303=CARTESIAN_POINT('Origin',(0.,1118.15413742548,408.009704071406));
#128304=CARTESIAN_POINT('Origin',(0.,1134.14517683891,424.620242579854));
#128305=CARTESIAN_POINT('Origin',(0.,1121.50270384563,431.789154132961));
#128306=CARTESIAN_POINT('Origin',(0.,1078.73142393294,424.620242579854));
#128307=CARTESIAN_POINT('Origin',(0.,1078.73142393294,424.620242579854));
#128308=CARTESIAN_POINT('Ctrl Pts',(-1.04233045748865E-14,1078.73142393294,
509.732983511718));
#128309=CARTESIAN_POINT('Ctrl Pts',(170.225481863728,1078.73142393294,509.732983511718));
#128310=CARTESIAN_POINT('Ctrl Pts',(170.225481863728,1078.73142393294,339.50750164799));
#128311=CARTESIAN_POINT('Ctrl Pts',(2.08466091497731E-14,1078.73142393294,
339.50750164799));
#128312=CARTESIAN_POINT('Ctrl Pts',(-1.27558853978063E-14,1078.73142393294,
528.779951376607));
#128313=CARTESIAN_POINT('Ctrl Pts',(208.319417593505,1078.73142393294,528.779951376607));
#128314=CARTESIAN_POINT('Ctrl Pts',(208.319417593505,1078.73142393294,320.460533783101));
#128315=CARTESIAN_POINT('Ctrl Pts',(2.55117707956127E-14,1078.73142393294,
320.460533783101));
#128316=CARTESIAN_POINT('Ctrl Pts',(-1.55312192834318E-14,1074.39201604106,
551.442272362198));
#128317=CARTESIAN_POINT('Ctrl Pts',(253.644059564688,1074.39201604106,551.442272362198));
#128318=CARTESIAN_POINT('Ctrl Pts',(253.644059564688,1074.39201604106,297.79821279751));
#128319=CARTESIAN_POINT('Ctrl Pts',(3.10624385668636E-14,1074.39201604106,
297.79821279751));
#128320=CARTESIAN_POINT('Origin',(0.,1082.7251047501,424.620242579854));
#128321=CARTESIAN_POINT('Origin',(0.,1076.73142393294,424.620242579854));
#128322=CARTESIAN_POINT('Origin',(0.,1082.7251047501,424.620242579854));
#128323=CARTESIAN_POINT('Origin',(0.,1076.73142393294,424.620242579854));
#128324=CARTESIAN_POINT('Origin',(0.,1082.7251047501,424.620242579854));
#128325=CARTESIAN_POINT('Origin',(0.,1076.73142393294,424.620242579854));
#128326=CARTESIAN_POINT('Origin',(0.,1082.7251047501,424.620242579854));
#128327=CARTESIAN_POINT('Origin',(0.,1076.73142393294,424.620242579854));
#128328=CARTESIAN_POINT('Origin',(0.,1082.7251047501,424.620242579854));
#128329=CARTESIAN_POINT('Origin',(0.,1076.73142393294,424.620242579854));
#128330=CARTESIAN_POINT('Origin',(0.,1082.7251047501,424.620242579854));
#128331=CARTESIAN_POINT('Origin',(0.,1076.73142393294,424.620242579854));
#128332=CARTESIAN_POINT('Origin',(0.,1082.7251047501,424.620242579854));
#128333=CARTESIAN_POINT('Origin',(0.,1076.73142393294,424.620242579854));
#128334=CARTESIAN_POINT('Origin',(0.,1082.7251047501,424.620242579854));
#128335=CARTESIAN_POINT('Origin',(0.,1076.73142393294,424.620242579854));
#128336=CARTESIAN_POINT('Origin',(0.,1082.7251047501,424.620242579854));
#128337=CARTESIAN_POINT('Origin',(0.,1076.73142393294,424.620242579854));
#128338=CARTESIAN_POINT('Origin',(0.,1082.7251047501,424.620242579854));
#128339=CARTESIAN_POINT('Origin',(0.,1076.73142393294,424.620242579854));
#128340=CARTESIAN_POINT('Origin',(0.,1082.7251047501,424.620242579854));
#128341=CARTESIAN_POINT('Origin',(0.,1076.73142393294,424.620242579854));
#128342=CARTESIAN_POINT('Origin',(0.,1082.7251047501,424.620242579854));
#128343=CARTESIAN_POINT('Origin',(0.,1076.73142393294,424.620242579854));
#128344=CARTESIAN_POINT('Origin',(0.,1082.7251047501,424.620242579854));
#128345=CARTESIAN_POINT('Origin',(0.,1076.73142393294,424.620242579854));
#128346=CARTESIAN_POINT('Origin',(0.,1082.7251047501,424.620242579854));
#128347=CARTESIAN_POINT('Origin',(0.,1076.73142393294,424.620242579854));
#128348=CARTESIAN_POINT('Origin',(0.,1082.7251047501,424.620242579854));
#128349=CARTESIAN_POINT('Origin',(0.,1076.73142393294,424.620242579854));
#128350=CARTESIAN_POINT('Origin',(0.,1082.7251047501,424.620242579854));
#128351=CARTESIAN_POINT('Origin',(0.,1076.73142393294,424.620242579854));
#128352=CARTESIAN_POINT('Origin',(0.,1082.7251047501,424.620242579854));
#128353=CARTESIAN_POINT('Origin',(0.,1076.73142393294,424.620242579854));
#128354=CARTESIAN_POINT('Origin',(0.,1082.7251047501,424.620242579854));
#128355=CARTESIAN_POINT('Origin',(0.,1076.73142393294,424.620242579854));
#128356=CARTESIAN_POINT('Origin',(0.,1082.7251047501,424.620242579854));
#128357=CARTESIAN_POINT('Origin',(0.,1076.73142393294,424.620242579854));
#128358=CARTESIAN_POINT('Origin',(0.,1082.7251047501,424.620242579854));
#128359=CARTESIAN_POINT('Origin',(0.,1076.73142393294,424.620242579854));
#128360=CARTESIAN_POINT('Origin',(0.,1082.7251047501,424.620242579854));
#128361=CARTESIAN_POINT('Origin',(0.,1076.73142393294,424.620242579854));
#128362=CARTESIAN_POINT('Origin',(0.,1082.7251047501,424.620242579854));
#128363=CARTESIAN_POINT('Origin',(0.,1076.73142393294,424.620242579854));
#128364=CARTESIAN_POINT('Origin',(0.,1082.7251047501,424.620242579854));
#128365=CARTESIAN_POINT('Origin',(0.,1076.73142393294,424.620242579854));
#128366=CARTESIAN_POINT('Origin',(0.,1082.7251047501,424.620242579854));
#128367=CARTESIAN_POINT('Origin',(0.,1076.73142393294,424.620242579854));
#128368=CARTESIAN_POINT('Origin',(0.,1082.7251047501,424.620242579854));
#128369=CARTESIAN_POINT('Origin',(0.,1076.73142393294,424.620242579854));
#128370=CARTESIAN_POINT('Origin',(0.,1082.7251047501,424.620242579854));
#128371=CARTESIAN_POINT('Origin',(0.,1076.73142393294,424.620242579854));
#128372=CARTESIAN_POINT('Origin',(0.,1082.7251047501,424.620242579854));
#128373=CARTESIAN_POINT('Origin',(0.,1076.73142393294,424.620242579854));
#128374=CARTESIAN_POINT('Origin',(0.,1082.7251047501,424.620242579854));
#128375=CARTESIAN_POINT('Origin',(0.,1076.73142393294,424.620242579854));
#128376=CARTESIAN_POINT('Origin',(0.,1082.7251047501,424.620242579854));
#128377=CARTESIAN_POINT('Origin',(0.,1076.73142393294,424.620242579854));
#128378=CARTESIAN_POINT('Origin',(0.,1082.7251047501,424.620242579854));
#128379=CARTESIAN_POINT('Origin',(0.,1076.73142393294,424.620242579854));
#128380=CARTESIAN_POINT('Origin',(0.,1082.7251047501,424.620242579854));
#128381=CARTESIAN_POINT('Origin',(0.,1076.73142393294,424.620242579854));
#128382=CARTESIAN_POINT('Origin',(0.,1082.7251047501,424.620242579854));
#128383=CARTESIAN_POINT('Origin',(0.,1076.73142393294,424.620242579854));
#128384=CARTESIAN_POINT('Origin',(0.,1082.7251047501,424.620242579854));
#128385=CARTESIAN_POINT('Origin',(0.,1076.73142393294,424.620242579854));
#128386=CARTESIAN_POINT('Origin',(0.,1082.7251047501,424.620242579854));
#128387=CARTESIAN_POINT('Origin',(0.,1076.73142393294,424.620242579854));
#128388=CARTESIAN_POINT('Origin',(0.,1082.7251047501,424.620242579854));
#128389=CARTESIAN_POINT('Origin',(0.,1076.73142393294,424.620242579854));
#128390=CARTESIAN_POINT('Origin',(0.,1082.7251047501,424.620242579854));
#128391=CARTESIAN_POINT('Origin',(0.,1076.73142393294,424.620242579854));
#128392=CARTESIAN_POINT('Origin',(0.,1082.7251047501,424.620242579854));
#128393=CARTESIAN_POINT('Origin',(0.,1076.73142393294,424.620242579854));
#128394=CARTESIAN_POINT('Origin',(0.,1082.7251047501,424.620242579854));
#128395=CARTESIAN_POINT('Origin',(0.,1076.73142393294,424.620242579854));
#128396=CARTESIAN_POINT('Origin',(0.,1082.7251047501,424.620242579854));
#128397=CARTESIAN_POINT('Origin',(0.,1076.73142393294,424.620242579854));
#128398=CARTESIAN_POINT('Origin',(0.,1082.7251047501,424.620242579854));
#128399=CARTESIAN_POINT('Origin',(0.,1076.73142393294,424.620242579854));
#128400=CARTESIAN_POINT('Origin',(0.,1082.7251047501,424.620242579854));
#128401=CARTESIAN_POINT('Origin',(0.,1076.73142393294,424.620242579854));
#128402=CARTESIAN_POINT('Origin',(0.,1082.7251047501,424.620242579854));
#128403=CARTESIAN_POINT('Origin',(0.,1076.73142393294,424.620242579854));
#128404=CARTESIAN_POINT('Origin',(0.,1082.7251047501,424.620242579854));
#128405=CARTESIAN_POINT('Origin',(0.,1076.73142393294,424.620242579854));
#128406=CARTESIAN_POINT('Origin',(0.,1082.7251047501,424.620242579854));
#128407=CARTESIAN_POINT('Origin',(0.,1076.73142393294,424.620242579854));
#128408=CARTESIAN_POINT('Origin',(0.,1082.7251047501,424.620242579854));
#128409=CARTESIAN_POINT('Origin',(0.,1076.73142393294,424.620242579854));
#128410=CARTESIAN_POINT('Origin',(0.,1082.7251047501,424.620242579854));
#128411=CARTESIAN_POINT('Origin',(0.,1076.73142393294,424.620242579854));
#128412=CARTESIAN_POINT('Origin',(0.,1082.7251047501,424.620242579854));
#128413=CARTESIAN_POINT('Origin',(0.,1076.73142393294,424.620242579854));
#128414=CARTESIAN_POINT('Origin',(0.,1082.7251047501,424.620242579854));
#128415=CARTESIAN_POINT('Origin',(0.,1076.73142393294,424.620242579854));
#128416=CARTESIAN_POINT('Origin',(0.,1082.7251047501,424.620242579854));
#128417=CARTESIAN_POINT('Origin',(0.,1076.73142393294,424.620242579854));
#128418=CARTESIAN_POINT('Origin',(0.,1082.7251047501,424.620242579854));
#128419=CARTESIAN_POINT('Origin',(0.,1076.73142393294,424.620242579854));
#128420=CARTESIAN_POINT('Origin',(0.,1082.7251047501,424.620242579854));
#128421=CARTESIAN_POINT('Origin',(0.,1076.73142393294,424.620242579854));
#128422=CARTESIAN_POINT('Origin',(0.,1082.7251047501,424.620242579854));
#128423=CARTESIAN_POINT('Origin',(0.,1076.73142393294,424.620242579854));
#128424=CARTESIAN_POINT('Origin',(0.,1082.7251047501,424.620242579854));
#128425=CARTESIAN_POINT('Origin',(0.,1076.73142393294,424.620242579854));
#128426=CARTESIAN_POINT('Origin',(0.,1082.7251047501,424.620242579854));
#128427=CARTESIAN_POINT('Origin',(0.,1076.73142393294,424.620242579854));
#128428=CARTESIAN_POINT('Origin',(0.,1082.7251047501,424.620242579854));
#128429=CARTESIAN_POINT('Origin',(0.,1076.73142393294,424.620242579854));
#128430=CARTESIAN_POINT('Origin',(0.,1082.7251047501,424.620242579854));
#128431=CARTESIAN_POINT('Origin',(0.,1076.73142393294,424.620242579854));
#128432=CARTESIAN_POINT('Origin',(0.,1082.7251047501,424.620242579854));
#128433=CARTESIAN_POINT('Origin',(0.,1076.73142393294,424.620242579854));
#128434=CARTESIAN_POINT('Origin',(0.,1082.7251047501,424.620242579854));
#128435=CARTESIAN_POINT('Origin',(0.,1076.73142393294,424.620242579854));
#128436=CARTESIAN_POINT('Origin',(0.,1082.7251047501,424.620242579854));
#128437=CARTESIAN_POINT('Origin',(0.,1076.73142393294,424.620242579854));
#128438=CARTESIAN_POINT('Origin',(0.,1082.7251047501,424.620242579854));
#128439=CARTESIAN_POINT('Origin',(0.,1076.73142393294,424.620242579854));
#128440=CARTESIAN_POINT('Origin',(0.,1082.7251047501,424.620242579854));
#128441=CARTESIAN_POINT('Origin',(0.,1076.73142393294,424.620242579854));
#128442=CARTESIAN_POINT('Origin',(0.,1082.7251047501,424.620242579854));
#128443=CARTESIAN_POINT('Origin',(0.,1076.73142393294,424.620242579854));
#128444=CARTESIAN_POINT('Origin',(0.,1082.7251047501,424.620242579854));
#128445=CARTESIAN_POINT('Origin',(0.,1076.73142393294,424.620242579854));
#128446=CARTESIAN_POINT('Origin',(0.,1082.7251047501,424.620242579854));
#128447=CARTESIAN_POINT('Origin',(0.,1076.73142393294,424.620242579854));
#128448=CARTESIAN_POINT('Origin',(0.,1082.7251047501,424.620242579854));
#128449=CARTESIAN_POINT('Origin',(0.,1076.73142393294,424.620242579854));
#128450=CARTESIAN_POINT('Origin',(0.,1082.7251047501,424.620242579854));
#128451=CARTESIAN_POINT('Origin',(0.,1076.73142393294,424.620242579854));
#128452=CARTESIAN_POINT('Origin',(0.,1082.7251047501,424.620242579854));
#128453=CARTESIAN_POINT('Origin',(0.,1076.73142393294,424.620242579854));
#128454=CARTESIAN_POINT('Origin',(0.,1082.7251047501,424.620242579854));
#128455=CARTESIAN_POINT('Origin',(0.,1076.73142393294,424.620242579854));
#128456=CARTESIAN_POINT('Origin',(0.,1082.7251047501,424.620242579854));
#128457=CARTESIAN_POINT('Origin',(0.,1076.73142393294,424.620242579854));
#128458=CARTESIAN_POINT('Origin',(0.,1082.7251047501,424.620242579854));
#128459=CARTESIAN_POINT('Origin',(0.,1076.73142393294,424.620242579854));
#128460=CARTESIAN_POINT('Origin',(0.,1082.7251047501,424.620242579854));
#128461=CARTESIAN_POINT('Origin',(0.,1076.73142393294,424.620242579854));
#128462=CARTESIAN_POINT('Origin',(0.,1082.7251047501,424.620242579854));
#128463=CARTESIAN_POINT('Origin',(0.,1076.73142393294,424.620242579854));
#128464=CARTESIAN_POINT('Origin',(0.,1082.7251047501,424.620242579854));
#128465=CARTESIAN_POINT('Origin',(0.,1076.73142393294,424.620242579854));
#128466=CARTESIAN_POINT('Origin',(0.,1082.7251047501,424.620242579854));
#128467=CARTESIAN_POINT('Origin',(0.,1076.73142393294,424.620242579854));
#128468=CARTESIAN_POINT('Origin',(0.,1082.7251047501,424.620242579854));
#128469=CARTESIAN_POINT('Origin',(0.,1076.73142393294,424.620242579854));
#128470=CARTESIAN_POINT('Origin',(0.,1082.7251047501,424.620242579854));
#128471=CARTESIAN_POINT('Origin',(0.,1076.73142393294,424.620242579854));
#128472=CARTESIAN_POINT('Origin',(0.,1082.7251047501,424.620242579854));
#128473=CARTESIAN_POINT('Origin',(0.,1076.73142393294,424.620242579854));
#128474=CARTESIAN_POINT('Origin',(0.,1082.7251047501,424.620242579854));
#128475=CARTESIAN_POINT('Origin',(0.,1076.73142393294,424.620242579854));
#128476=CARTESIAN_POINT('Origin',(0.,1082.7251047501,424.620242579854));
#128477=CARTESIAN_POINT('Origin',(0.,1076.73142393294,424.620242579854));
#128478=CARTESIAN_POINT('Origin',(0.,1082.7251047501,424.620242579854));
#128479=CARTESIAN_POINT('Origin',(0.,1076.73142393294,424.620242579854));
#128480=CARTESIAN_POINT('Origin',(0.,1082.7251047501,424.620242579854));
#128481=CARTESIAN_POINT('Origin',(0.,1076.73142393294,424.620242579854));
#128482=CARTESIAN_POINT('Origin',(0.,1082.7251047501,424.620242579854));
#128483=CARTESIAN_POINT('Origin',(0.,1076.73142393294,424.620242579854));
#128484=CARTESIAN_POINT('Origin',(0.,1082.7251047501,424.620242579854));
#128485=CARTESIAN_POINT('Origin',(0.,1076.73142393294,424.620242579854));
#128486=CARTESIAN_POINT('Origin',(0.,1082.7251047501,424.620242579854));
#128487=CARTESIAN_POINT('Origin',(0.,1076.73142393294,424.620242579854));
#128488=CARTESIAN_POINT('Origin',(0.,1082.7251047501,424.620242579854));
#128489=CARTESIAN_POINT('Origin',(0.,1076.73142393294,424.620242579854));
#128490=CARTESIAN_POINT('Origin',(0.,1082.7251047501,424.620242579854));
#128491=CARTESIAN_POINT('Origin',(0.,1076.73142393294,424.620242579854));
#128492=CARTESIAN_POINT('Origin',(0.,1082.7251047501,424.620242579854));
#128493=CARTESIAN_POINT('Origin',(0.,1076.73142393294,424.620242579854));
#128494=CARTESIAN_POINT('Origin',(0.,1082.7251047501,424.620242579854));
#128495=CARTESIAN_POINT('Origin',(0.,1076.73142393294,424.620242579854));
#128496=CARTESIAN_POINT('Origin',(0.,1082.7251047501,424.620242579854));
#128497=CARTESIAN_POINT('Origin',(0.,1076.73142393294,424.620242579854));
#128498=CARTESIAN_POINT('Origin',(0.,1082.7251047501,424.620242579854));
#128499=CARTESIAN_POINT('Origin',(0.,1076.73142393294,424.620242579854));
#128500=CARTESIAN_POINT('Origin',(0.,1082.7251047501,424.620242579854));
#128501=CARTESIAN_POINT('Origin',(0.,1076.73142393294,424.620242579854));
#128502=CARTESIAN_POINT('Origin',(0.,1082.7251047501,424.620242579854));
#128503=CARTESIAN_POINT('Origin',(0.,1076.73142393294,424.620242579854));
#128504=CARTESIAN_POINT('Origin',(0.,1082.7251047501,424.620242579854));
#128505=CARTESIAN_POINT('Origin',(0.,1076.73142393294,424.620242579854));
#128506=CARTESIAN_POINT('Origin',(0.,1082.7251047501,424.620242579854));
#128507=CARTESIAN_POINT('Origin',(0.,1076.73142393294,424.620242579854));
#128508=CARTESIAN_POINT('Origin',(0.,1082.7251047501,424.620242579854));
#128509=CARTESIAN_POINT('Origin',(0.,1076.73142393294,424.620242579854));
#128510=CARTESIAN_POINT('Origin',(0.,1082.7251047501,424.620242579854));
#128511=CARTESIAN_POINT('Origin',(0.,1076.73142393294,424.620242579854));
#128512=CARTESIAN_POINT('Origin',(0.,1082.7251047501,424.620242579854));
#128513=CARTESIAN_POINT('Origin',(0.,1076.73142393294,424.620242579854));
#128514=CARTESIAN_POINT('Origin',(0.,1082.7251047501,424.620242579854));
#128515=CARTESIAN_POINT('Origin',(0.,1076.73142393294,424.620242579854));
#128516=CARTESIAN_POINT('Origin',(0.,1082.7251047501,424.620242579854));
#128517=CARTESIAN_POINT('Origin',(0.,1076.73142393294,424.620242579854));
#128518=CARTESIAN_POINT('Origin',(0.,1082.7251047501,424.620242579854));
#128519=CARTESIAN_POINT('Origin',(0.,1076.73142393294,424.620242579854));
#128520=CARTESIAN_POINT('Origin',(0.,1082.7251047501,424.620242579854));
#128521=CARTESIAN_POINT('Origin',(0.,1076.73142393294,424.620242579854));
#128522=CARTESIAN_POINT('Origin',(0.,1082.7251047501,424.620242579854));
#128523=CARTESIAN_POINT('Origin',(0.,1076.73142393294,424.620242579854));
#128524=CARTESIAN_POINT('Origin',(0.,1082.7251047501,424.620242579854));
#128525=CARTESIAN_POINT('Origin',(0.,1076.73142393294,424.620242579854));
#128526=CARTESIAN_POINT('Origin',(0.,1082.7251047501,424.620242579854));
#128527=CARTESIAN_POINT('Origin',(0.,1076.73142393294,424.620242579854));
#128528=CARTESIAN_POINT('Origin',(0.,1082.7251047501,424.620242579854));
#128529=CARTESIAN_POINT('Origin',(0.,1076.73142393294,424.620242579854));
#128530=CARTESIAN_POINT('Origin',(0.,1082.7251047501,424.620242579854));
#128531=CARTESIAN_POINT('Origin',(0.,1076.73142393294,424.620242579854));
#128532=CARTESIAN_POINT('Origin',(0.,1082.7251047501,424.620242579854));
#128533=CARTESIAN_POINT('Origin',(0.,1076.73142393294,424.620242579854));
#128534=CARTESIAN_POINT('Origin',(0.,1082.7251047501,424.620242579854));
#128535=CARTESIAN_POINT('Origin',(0.,1076.73142393294,424.620242579854));
#128536=CARTESIAN_POINT('Origin',(0.,1082.7251047501,424.620242579854));
#128537=CARTESIAN_POINT('Origin',(0.,1076.73142393294,424.620242579854));
#128538=CARTESIAN_POINT('Origin',(0.,1082.7251047501,424.620242579854));
#128539=CARTESIAN_POINT('Origin',(0.,1076.73142393294,424.620242579854));
#128540=CARTESIAN_POINT('Origin',(0.,1082.7251047501,424.620242579854));
#128541=CARTESIAN_POINT('Origin',(0.,1076.73142393294,424.620242579854));
#128542=CARTESIAN_POINT('Origin',(0.,1082.7251047501,424.620242579854));
#128543=CARTESIAN_POINT('Origin',(0.,1076.73142393294,424.620242579854));
#128544=CARTESIAN_POINT('Origin',(0.,1082.7251047501,424.620242579854));
#128545=CARTESIAN_POINT('Origin',(0.,1076.73142393294,424.620242579854));
#128546=CARTESIAN_POINT('Origin',(0.,1082.7251047501,424.620242579854));
#128547=CARTESIAN_POINT('Origin',(0.,1076.73142393294,424.620242579854));
#128548=CARTESIAN_POINT('Origin',(0.,1082.7251047501,424.620242579854));
#128549=CARTESIAN_POINT('Origin',(0.,1076.73142393294,424.620242579854));
#128550=CARTESIAN_POINT('Origin',(0.,1082.7251047501,424.620242579854));
#128551=CARTESIAN_POINT('Origin',(0.,1076.73142393294,424.620242579854));
#128552=CARTESIAN_POINT('Origin',(0.,1082.7251047501,424.620242579854));
#128553=CARTESIAN_POINT('Origin',(0.,1076.73142393294,424.620242579854));
#128554=CARTESIAN_POINT('Origin',(0.,1082.7251047501,424.620242579854));
#128555=CARTESIAN_POINT('Origin',(0.,1076.73142393294,424.620242579854));
#128556=CARTESIAN_POINT('Origin',(0.,1082.7251047501,424.620242579854));
#128557=CARTESIAN_POINT('Origin',(0.,1076.73142393294,424.620242579854));
#128558=CARTESIAN_POINT('Origin',(0.,1082.7251047501,424.620242579854));
#128559=CARTESIAN_POINT('Origin',(0.,1076.73142393294,424.620242579854));
#128560=CARTESIAN_POINT('Origin',(0.,1082.7251047501,424.620242579854));
#128561=CARTESIAN_POINT('Origin',(0.,1076.73142393294,424.620242579854));
#128562=CARTESIAN_POINT('Origin',(0.,1082.7251047501,424.620242579854));
#128563=CARTESIAN_POINT('Origin',(0.,1076.73142393294,424.620242579854));
#128564=CARTESIAN_POINT('Origin',(0.,1082.7251047501,424.620242579854));
#128565=CARTESIAN_POINT('Origin',(0.,1076.73142393294,424.620242579854));
#128566=CARTESIAN_POINT('Origin',(0.,1082.7251047501,424.620242579854));
#128567=CARTESIAN_POINT('Origin',(0.,1076.73142393294,424.620242579854));
#128568=CARTESIAN_POINT('Origin',(0.,1082.7251047501,424.620242579854));
#128569=CARTESIAN_POINT('Origin',(0.,1076.73142393294,424.620242579854));
#128570=CARTESIAN_POINT('Origin',(0.,1082.7251047501,424.620242579854));
#128571=CARTESIAN_POINT('Origin',(0.,1076.73142393294,424.620242579854));
#128572=CARTESIAN_POINT('Origin',(0.,1082.7251047501,424.620242579854));
#128573=CARTESIAN_POINT('Origin',(0.,1076.73142393294,424.620242579854));
#128574=CARTESIAN_POINT('Origin',(0.,1082.7251047501,424.620242579854));
#128575=CARTESIAN_POINT('Origin',(0.,1076.73142393294,424.620242579854));
#128576=CARTESIAN_POINT('Origin',(0.,1082.7251047501,424.620242579854));
#128577=CARTESIAN_POINT('Origin',(0.,1076.73142393294,424.620242579854));
#128578=CARTESIAN_POINT('Origin',(0.,1082.7251047501,424.620242579854));
#128579=CARTESIAN_POINT('Origin',(0.,1076.73142393294,424.620242579854));
#128580=CARTESIAN_POINT('Origin',(0.,1082.7251047501,424.620242579854));
#128581=CARTESIAN_POINT('Origin',(0.,1076.73142393294,424.620242579854));
#128582=CARTESIAN_POINT('Origin',(0.,1082.7251047501,424.620242579854));
#128583=CARTESIAN_POINT('Origin',(0.,1076.73142393294,424.620242579854));
#128584=CARTESIAN_POINT('Origin',(0.,1082.7251047501,424.620242579854));
#128585=CARTESIAN_POINT('Origin',(0.,1076.73142393294,424.620242579854));
#128586=CARTESIAN_POINT('Origin',(0.,1082.7251047501,424.620242579854));
#128587=CARTESIAN_POINT('Origin',(0.,1076.73142393294,424.620242579854));
#128588=CARTESIAN_POINT('Origin',(0.,1082.7251047501,424.620242579854));
#128589=CARTESIAN_POINT('Origin',(0.,1076.73142393294,424.620242579854));
#128590=CARTESIAN_POINT('Origin',(0.,1082.7251047501,424.620242579854));
#128591=CARTESIAN_POINT('Origin',(0.,1076.73142393294,424.620242579854));
#128592=CARTESIAN_POINT('Origin',(0.,1082.7251047501,424.620242579854));
#128593=CARTESIAN_POINT('Origin',(0.,1076.73142393294,424.620242579854));
#128594=CARTESIAN_POINT('Origin',(0.,1082.7251047501,424.620242579854));
#128595=CARTESIAN_POINT('Origin',(0.,1076.73142393294,424.620242579854));
#128596=CARTESIAN_POINT('Origin',(0.,1082.7251047501,424.620242579854));
#128597=CARTESIAN_POINT('Origin',(0.,1076.73142393294,424.620242579854));
#128598=CARTESIAN_POINT('Origin',(0.,1082.7251047501,424.620242579854));
#128599=CARTESIAN_POINT('Origin',(0.,1076.73142393294,424.620242579854));
#128600=CARTESIAN_POINT('Origin',(0.,1082.7251047501,424.620242579854));
#128601=CARTESIAN_POINT('Origin',(0.,1076.73142393294,424.620242579854));
#128602=CARTESIAN_POINT('Origin',(0.,1082.7251047501,424.620242579854));
#128603=CARTESIAN_POINT('Origin',(0.,1076.73142393294,424.620242579854));
#128604=CARTESIAN_POINT('Origin',(0.,1082.7251047501,424.620242579854));
#128605=CARTESIAN_POINT('Origin',(0.,1076.73142393294,424.620242579854));
#128606=CARTESIAN_POINT('Origin',(0.,1082.7251047501,424.620242579854));
#128607=CARTESIAN_POINT('Origin',(0.,1076.73142393294,424.620242579854));
#128608=CARTESIAN_POINT('Origin',(0.,1082.7251047501,424.620242579854));
#128609=CARTESIAN_POINT('Origin',(0.,1076.73142393294,424.620242579854));
#128610=CARTESIAN_POINT('Origin',(0.,1082.7251047501,424.620242579854));
#128611=CARTESIAN_POINT('Origin',(0.,1076.73142393294,424.620242579854));
#128612=CARTESIAN_POINT('Origin',(0.,1082.7251047501,424.620242579854));
#128613=CARTESIAN_POINT('Origin',(0.,1076.73142393294,424.620242579854));
#128614=CARTESIAN_POINT('Origin',(0.,1082.7251047501,424.620242579854));
#128615=CARTESIAN_POINT('Origin',(0.,1076.73142393294,424.620242579854));
#128616=CARTESIAN_POINT('Origin',(0.,1082.7251047501,424.620242579854));
#128617=CARTESIAN_POINT('Origin',(0.,1076.73142393294,424.620242579854));
#128618=CARTESIAN_POINT('Origin',(0.,1082.7251047501,424.620242579854));
#128619=CARTESIAN_POINT('Origin',(0.,1076.73142393294,424.620242579854));
#128620=CARTESIAN_POINT('Origin',(0.,1082.7251047501,424.620242579854));
#128621=CARTESIAN_POINT('Origin',(0.,1076.73142393294,424.620242579854));
#128622=CARTESIAN_POINT('Origin',(0.,1082.7251047501,424.620242579854));
#128623=CARTESIAN_POINT('Origin',(0.,1076.73142393294,424.620242579854));
#128624=CARTESIAN_POINT('Origin',(0.,1082.7251047501,424.620242579854));
#128625=CARTESIAN_POINT('Origin',(0.,1076.73142393294,424.620242579854));
#128626=CARTESIAN_POINT('Origin',(0.,1082.7251047501,424.620242579854));
#128627=CARTESIAN_POINT('Origin',(0.,1076.73142393294,424.620242579854));
#128628=CARTESIAN_POINT('Origin',(0.,1082.7251047501,424.620242579854));
#128629=CARTESIAN_POINT('Origin',(0.,1076.73142393294,424.620242579854));
#128630=CARTESIAN_POINT('Origin',(0.,1082.7251047501,424.620242579854));
#128631=CARTESIAN_POINT('Origin',(0.,1076.73142393294,424.620242579854));
#128632=CARTESIAN_POINT('Origin',(0.,1082.7251047501,424.620242579854));
#128633=CARTESIAN_POINT('Origin',(0.,1076.73142393294,424.620242579854));
#128634=CARTESIAN_POINT('Origin',(0.,1082.7251047501,424.620242579854));
#128635=CARTESIAN_POINT('Origin',(0.,1076.73142393294,424.620242579854));
#128636=CARTESIAN_POINT('Origin',(0.,1082.7251047501,424.620242579854));
#128637=CARTESIAN_POINT('Origin',(0.,1076.73142393294,424.620242579854));
#128638=CARTESIAN_POINT('Origin',(0.,1082.7251047501,424.620242579854));
#128639=CARTESIAN_POINT('Origin',(0.,1076.73142393294,424.620242579854));
#128640=CARTESIAN_POINT('Origin',(0.,1082.7251047501,424.620242579854));
#128641=CARTESIAN_POINT('Origin',(0.,1076.73142393294,424.620242579854));
#128642=CARTESIAN_POINT('Origin',(0.,1082.7251047501,424.620242579854));
#128643=CARTESIAN_POINT('Origin',(0.,1076.73142393294,424.620242579854));
#128644=CARTESIAN_POINT('Origin',(0.,1082.7251047501,424.620242579854));
#128645=CARTESIAN_POINT('Origin',(0.,1076.73142393294,424.620242579854));
#128646=CARTESIAN_POINT('Origin',(0.,1082.7251047501,424.620242579854));
#128647=CARTESIAN_POINT('Origin',(0.,1076.73142393294,424.620242579854));
#128648=CARTESIAN_POINT('Origin',(0.,1082.7251047501,424.620242579854));
#128649=CARTESIAN_POINT('Origin',(0.,1076.73142393294,424.620242579854));
#128650=CARTESIAN_POINT('Origin',(0.,1082.7251047501,424.620242579854));
#128651=CARTESIAN_POINT('Origin',(0.,1076.73142393294,424.620242579854));
#128652=CARTESIAN_POINT('Origin',(0.,1082.7251047501,424.620242579854));
#128653=CARTESIAN_POINT('Origin',(0.,1076.73142393294,424.620242579854));
#128654=CARTESIAN_POINT('Origin',(0.,1082.7251047501,424.620242579854));
#128655=CARTESIAN_POINT('Origin',(0.,1076.73142393294,424.620242579854));
#128656=CARTESIAN_POINT('Origin',(0.,1082.7251047501,424.620242579854));
#128657=CARTESIAN_POINT('Origin',(0.,1076.73142393294,424.620242579854));
#128658=CARTESIAN_POINT('Origin',(0.,1082.7251047501,424.620242579854));
#128659=CARTESIAN_POINT('Origin',(0.,1076.73142393294,424.620242579854));
#128660=CARTESIAN_POINT('Origin',(0.,1082.7251047501,424.620242579854));
#128661=CARTESIAN_POINT('Origin',(0.,1076.73142393294,424.620242579854));
#128662=CARTESIAN_POINT('Origin',(0.,1082.7251047501,424.620242579854));
#128663=CARTESIAN_POINT('Origin',(0.,1076.73142393294,424.620242579854));
#128664=CARTESIAN_POINT('Origin',(0.,1082.7251047501,424.620242579854));
#128665=CARTESIAN_POINT('Origin',(0.,1076.73142393294,424.620242579854));
#128666=CARTESIAN_POINT('Origin',(0.,1082.7251047501,424.620242579854));
#128667=CARTESIAN_POINT('Origin',(0.,1076.73142393294,424.620242579854));
#128668=CARTESIAN_POINT('Origin',(0.,1082.7251047501,424.620242579854));
#128669=CARTESIAN_POINT('Origin',(0.,1076.73142393294,424.620242579854));
#128670=CARTESIAN_POINT('Origin',(0.,1082.7251047501,424.620242579854));
#128671=CARTESIAN_POINT('Origin',(0.,1076.73142393294,424.620242579854));
#128672=CARTESIAN_POINT('Origin',(0.,1082.7251047501,424.620242579854));
#128673=CARTESIAN_POINT('Origin',(0.,1076.73142393294,424.620242579854));
#128674=CARTESIAN_POINT('Origin',(0.,1082.7251047501,424.620242579854));
#128675=CARTESIAN_POINT('Origin',(0.,1076.73142393294,424.620242579854));
#128676=CARTESIAN_POINT('Origin',(0.,1082.7251047501,424.620242579854));
#128677=CARTESIAN_POINT('Origin',(0.,1076.73142393294,424.620242579854));
#128678=CARTESIAN_POINT('Origin',(0.,1082.7251047501,424.620242579854));
#128679=CARTESIAN_POINT('Origin',(0.,1076.73142393294,424.620242579854));
#128680=CARTESIAN_POINT('Origin',(0.,1082.7251047501,424.620242579854));
#128681=CARTESIAN_POINT('Origin',(0.,1076.73142393294,424.620242579854));
#128682=CARTESIAN_POINT('Origin',(0.,1082.7251047501,424.620242579854));
#128683=CARTESIAN_POINT('Origin',(0.,1076.73142393294,424.620242579854));
#128684=CARTESIAN_POINT('Origin',(0.,1082.7251047501,424.620242579854));
#128685=CARTESIAN_POINT('Origin',(0.,1076.73142393294,424.620242579854));
#128686=CARTESIAN_POINT('Origin',(0.,1082.7251047501,424.620242579854));
#128687=CARTESIAN_POINT('Origin',(0.,1076.73142393294,424.620242579854));
#128688=CARTESIAN_POINT('Origin',(0.,1082.7251047501,424.620242579854));
#128689=CARTESIAN_POINT('Origin',(0.,1076.73142393294,424.620242579854));
#128690=CARTESIAN_POINT('Origin',(0.,1082.7251047501,424.620242579854));
#128691=CARTESIAN_POINT('Origin',(0.,1076.73142393294,424.620242579854));
#128692=CARTESIAN_POINT('Origin',(0.,1082.7251047501,424.620242579854));
#128693=CARTESIAN_POINT('Origin',(0.,1076.73142393294,424.620242579854));
#128694=CARTESIAN_POINT('Origin',(0.,1082.7251047501,424.620242579854));
#128695=CARTESIAN_POINT('Origin',(0.,1076.73142393294,424.620242579854));
#128696=CARTESIAN_POINT('Origin',(0.,1082.7251047501,424.620242579854));
#128697=CARTESIAN_POINT('Origin',(0.,1076.73142393294,424.620242579854));
#128698=CARTESIAN_POINT('Origin',(0.,1082.7251047501,424.620242579854));
#128699=CARTESIAN_POINT('Origin',(0.,1076.73142393294,424.620242579854));
#128700=CARTESIAN_POINT('Origin',(0.,1082.7251047501,424.620242579854));
#128701=CARTESIAN_POINT('Origin',(0.,1076.73142393294,424.620242579854));
#128702=CARTESIAN_POINT('Origin',(0.,1082.7251047501,424.620242579854));
#128703=CARTESIAN_POINT('Origin',(0.,1076.73142393294,424.620242579854));
#128704=CARTESIAN_POINT('Origin',(0.,1082.7251047501,424.620242579854));
#128705=CARTESIAN_POINT('Origin',(0.,1076.73142393294,424.620242579854));
#128706=CARTESIAN_POINT('Origin',(0.,1082.7251047501,424.620242579854));
#128707=CARTESIAN_POINT('Origin',(0.,1076.73142393294,424.620242579854));
#128708=CARTESIAN_POINT('Origin',(0.,1082.7251047501,424.620242579854));
#128709=CARTESIAN_POINT('Origin',(0.,1076.73142393294,424.620242579854));
#128710=CARTESIAN_POINT('Origin',(0.,1082.7251047501,424.620242579854));
#128711=CARTESIAN_POINT('Origin',(0.,1076.73142393294,424.620242579854));
#128712=CARTESIAN_POINT('Origin',(0.,1082.7251047501,424.620242579854));
#128713=CARTESIAN_POINT('Origin',(0.,1076.73142393294,424.620242579854));
#128714=CARTESIAN_POINT('Origin',(0.,1082.7251047501,424.620242579854));
#128715=CARTESIAN_POINT('Origin',(0.,1076.73142393294,424.620242579854));
#128716=CARTESIAN_POINT('Origin',(0.,1082.7251047501,424.620242579854));
#128717=CARTESIAN_POINT('Origin',(0.,1076.73142393294,424.620242579854));
#128718=CARTESIAN_POINT('Origin',(0.,1082.7251047501,424.620242579854));
#128719=CARTESIAN_POINT('Origin',(0.,1076.73142393294,424.620242579854));
#128720=CARTESIAN_POINT('Origin',(0.,1082.7251047501,424.620242579854));
#128721=CARTESIAN_POINT('Origin',(0.,1076.73142393294,424.620242579854));
#128722=CARTESIAN_POINT('Origin',(0.,1082.7251047501,424.620242579854));
#128723=CARTESIAN_POINT('Origin',(0.,1076.73142393294,424.620242579854));
#128724=CARTESIAN_POINT('Origin',(0.,1082.7251047501,424.620242579854));
#128725=CARTESIAN_POINT('Origin',(0.,1076.73142393294,424.620242579854));
#128726=CARTESIAN_POINT('Origin',(0.,1082.7251047501,424.620242579854));
#128727=CARTESIAN_POINT('Origin',(0.,1076.73142393294,424.620242579854));
#128728=CARTESIAN_POINT('Origin',(0.,1082.7251047501,424.620242579854));
#128729=CARTESIAN_POINT('Origin',(0.,1076.73142393294,424.620242579854));
#128730=CARTESIAN_POINT('Origin',(0.,1082.7251047501,424.620242579854));
#128731=CARTESIAN_POINT('Origin',(0.,1076.73142393294,424.620242579854));
#128732=CARTESIAN_POINT('Origin',(0.,1082.7251047501,424.620242579854));
#128733=CARTESIAN_POINT('Origin',(0.,1076.73142393294,424.620242579854));
#128734=CARTESIAN_POINT('Origin',(0.,1082.7251047501,424.620242579854));
#128735=CARTESIAN_POINT('Origin',(0.,1076.73142393294,424.620242579854));
#128736=CARTESIAN_POINT('Origin',(0.,1082.7251047501,424.620242579854));
#128737=CARTESIAN_POINT('Origin',(0.,1076.73142393294,424.620242579854));
#128738=CARTESIAN_POINT('Origin',(0.,1082.7251047501,424.620242579854));
#128739=CARTESIAN_POINT('Origin',(0.,1076.73142393294,424.620242579854));
#128740=CARTESIAN_POINT('Origin',(0.,1082.7251047501,424.620242579854));
#128741=CARTESIAN_POINT('Origin',(0.,1076.73142393294,424.620242579854));
#128742=CARTESIAN_POINT('Origin',(0.,1082.7251047501,424.620242579854));
#128743=CARTESIAN_POINT('Origin',(0.,1076.73142393294,424.620242579854));
#128744=CARTESIAN_POINT('Origin',(0.,1082.7251047501,424.620242579854));
#128745=CARTESIAN_POINT('Origin',(0.,1076.73142393294,424.620242579854));
#128746=CARTESIAN_POINT('Origin',(0.,1082.7251047501,424.620242579854));
#128747=CARTESIAN_POINT('Origin',(0.,1076.73142393294,424.620242579854));
#128748=CARTESIAN_POINT('Origin',(0.,1082.7251047501,424.620242579854));
#128749=CARTESIAN_POINT('Origin',(0.,1076.73142393294,424.620242579854));
#128750=CARTESIAN_POINT('Origin',(0.,1082.7251047501,424.620242579854));
#128751=CARTESIAN_POINT('Origin',(0.,1076.73142393294,424.620242579854));
#128752=CARTESIAN_POINT('Origin',(0.,1082.7251047501,424.620242579854));
#128753=CARTESIAN_POINT('Origin',(0.,1076.73142393294,424.620242579854));
#128754=CARTESIAN_POINT('Origin',(0.,1082.7251047501,424.620242579854));
#128755=CARTESIAN_POINT('Origin',(0.,1076.73142393294,424.620242579854));
#128756=CARTESIAN_POINT('Origin',(0.,1082.7251047501,424.620242579854));
#128757=CARTESIAN_POINT('Origin',(0.,1076.73142393294,424.620242579854));
#128758=CARTESIAN_POINT('Origin',(0.,1082.7251047501,424.620242579854));
#128759=CARTESIAN_POINT('Origin',(0.,1076.73142393294,424.620242579854));
#128760=CARTESIAN_POINT('Origin',(0.,1082.7251047501,424.620242579854));
#128761=CARTESIAN_POINT('Origin',(0.,1076.73142393294,424.620242579854));
#128762=CARTESIAN_POINT('Origin',(0.,1082.7251047501,424.620242579854));
#128763=CARTESIAN_POINT('Origin',(0.,1076.73142393294,424.620242579854));
#128764=CARTESIAN_POINT('Origin',(0.,1082.7251047501,424.620242579854));
#128765=CARTESIAN_POINT('Origin',(0.,1076.73142393294,424.620242579854));
#128766=CARTESIAN_POINT('Origin',(0.,1082.7251047501,424.620242579854));
#128767=CARTESIAN_POINT('Origin',(0.,1076.73142393294,424.620242579854));
#128768=CARTESIAN_POINT('Origin',(0.,1082.7251047501,424.620242579854));
#128769=CARTESIAN_POINT('Origin',(0.,1076.73142393294,424.620242579854));
#128770=CARTESIAN_POINT('Origin',(0.,1082.7251047501,424.620242579854));
#128771=CARTESIAN_POINT('Origin',(0.,1076.73142393294,424.620242579854));
#128772=CARTESIAN_POINT('Origin',(0.,1082.7251047501,424.620242579854));
#128773=CARTESIAN_POINT('Origin',(0.,1076.73142393294,424.620242579854));
#128774=CARTESIAN_POINT('Origin',(0.,1082.7251047501,424.620242579854));
#128775=CARTESIAN_POINT('Origin',(0.,1076.73142393294,424.620242579854));
#128776=CARTESIAN_POINT('Origin',(0.,1082.7251047501,424.620242579854));
#128777=CARTESIAN_POINT('Origin',(0.,1076.73142393294,424.620242579854));
#128778=CARTESIAN_POINT('Origin',(0.,1082.7251047501,424.620242579854));
#128779=CARTESIAN_POINT('Origin',(0.,1076.73142393294,424.620242579854));
#128780=CARTESIAN_POINT('Origin',(0.,1082.7251047501,424.620242579854));
#128781=CARTESIAN_POINT('Origin',(0.,1076.73142393294,424.620242579854));
#128782=CARTESIAN_POINT('Origin',(0.,1082.7251047501,424.620242579854));
#128783=CARTESIAN_POINT('Origin',(0.,1076.73142393294,424.620242579854));
#128784=CARTESIAN_POINT('Origin',(0.,1082.7251047501,424.620242579854));
#128785=CARTESIAN_POINT('Origin',(0.,1076.73142393294,424.620242579854));
#128786=CARTESIAN_POINT('Origin',(0.,1082.7251047501,424.620242579854));
#128787=CARTESIAN_POINT('Origin',(0.,1076.73142393294,424.620242579854));
#128788=CARTESIAN_POINT('Origin',(0.,1082.7251047501,424.620242579854));
#128789=CARTESIAN_POINT('Origin',(0.,1076.73142393294,424.620242579854));
#128790=CARTESIAN_POINT('Origin',(0.,1082.7251047501,424.620242579854));
#128791=CARTESIAN_POINT('Origin',(0.,1076.73142393294,424.620242579854));
#128792=CARTESIAN_POINT('Origin',(0.,1082.7251047501,424.620242579854));
#128793=CARTESIAN_POINT('Origin',(0.,1076.73142393294,424.620242579854));
#128794=CARTESIAN_POINT('Origin',(0.,1082.7251047501,424.620242579854));
#128795=CARTESIAN_POINT('Origin',(0.,1076.73142393294,424.620242579854));
#128796=CARTESIAN_POINT('Origin',(0.,1082.7251047501,424.620242579854));
#128797=CARTESIAN_POINT('Origin',(0.,1076.73142393294,424.620242579854));
#128798=CARTESIAN_POINT('Origin',(0.,1082.7251047501,424.620242579854));
#128799=CARTESIAN_POINT('Origin',(0.,1076.73142393294,424.620242579854));
#128800=CARTESIAN_POINT('Origin',(0.,1082.7251047501,424.620242579854));
#128801=CARTESIAN_POINT('Origin',(0.,1076.73142393294,424.620242579854));
#128802=CARTESIAN_POINT('Origin',(0.,1082.7251047501,424.620242579854));
#128803=CARTESIAN_POINT('Origin',(0.,1076.73142393294,424.620242579854));
#128804=CARTESIAN_POINT('Origin',(0.,1082.7251047501,424.620242579854));
#128805=CARTESIAN_POINT('Origin',(0.,1076.73142393294,424.620242579854));
#128806=CARTESIAN_POINT('Origin',(0.,1082.7251047501,424.620242579854));
#128807=CARTESIAN_POINT('Origin',(0.,1076.73142393294,424.620242579854));
#128808=CARTESIAN_POINT('Origin',(0.,1082.7251047501,424.620242579854));
#128809=CARTESIAN_POINT('Origin',(0.,1076.73142393294,424.620242579854));
#128810=CARTESIAN_POINT('Origin',(0.,1082.7251047501,424.620242579854));
#128811=CARTESIAN_POINT('Origin',(0.,1076.73142393294,424.620242579854));
#128812=CARTESIAN_POINT('Origin',(0.,1082.7251047501,424.620242579854));
#128813=CARTESIAN_POINT('Origin',(0.,1076.73142393294,424.620242579854));
#128814=CARTESIAN_POINT('Origin',(0.,1082.7251047501,424.620242579854));
#128815=CARTESIAN_POINT('Origin',(0.,1076.73142393294,424.620242579854));
#128816=CARTESIAN_POINT('Origin',(0.,1082.7251047501,424.620242579854));
#128817=CARTESIAN_POINT('Origin',(0.,1076.73142393294,424.620242579854));
#128818=CARTESIAN_POINT('Origin',(0.,1082.7251047501,424.620242579854));
#128819=CARTESIAN_POINT('Origin',(0.,1076.73142393294,424.620242579854));
#128820=CARTESIAN_POINT('Origin',(0.,1082.7251047501,424.620242579854));
#128821=CARTESIAN_POINT('Origin',(0.,1076.73142393294,424.620242579854));
#128822=CARTESIAN_POINT('Origin',(0.,1082.7251047501,424.620242579854));
#128823=CARTESIAN_POINT('Origin',(0.,1076.73142393294,424.620242579854));
#128824=CARTESIAN_POINT('Origin',(0.,1082.7251047501,424.620242579854));
#128825=CARTESIAN_POINT('Origin',(0.,1076.73142393294,424.620242579854));
#128826=CARTESIAN_POINT('Origin',(0.,1082.7251047501,424.620242579854));
#128827=CARTESIAN_POINT('Origin',(0.,1076.73142393294,424.620242579854));
#128828=CARTESIAN_POINT('Origin',(0.,1082.7251047501,424.620242579854));
#128829=CARTESIAN_POINT('Origin',(0.,1076.73142393294,424.620242579854));
#128830=CARTESIAN_POINT('Origin',(0.,1082.7251047501,424.620242579854));
#128831=CARTESIAN_POINT('Origin',(0.,1076.73142393294,424.620242579854));
#128832=CARTESIAN_POINT('Origin',(0.,1082.7251047501,424.620242579854));
#128833=CARTESIAN_POINT('Origin',(0.,1076.73142393294,424.620242579854));
#128834=CARTESIAN_POINT('Origin',(0.,1082.7251047501,424.620242579854));
#128835=CARTESIAN_POINT('Origin',(0.,1076.73142393294,424.620242579854));
#128836=CARTESIAN_POINT('Origin',(0.,1082.7251047501,424.620242579854));
#128837=CARTESIAN_POINT('Origin',(0.,1076.73142393294,424.620242579854));
#128838=CARTESIAN_POINT('Origin',(0.,1082.7251047501,424.620242579854));
#128839=CARTESIAN_POINT('Origin',(0.,1076.73142393294,424.620242579854));
#128840=CARTESIAN_POINT('Origin',(0.,1082.7251047501,424.620242579854));
#128841=CARTESIAN_POINT('Origin',(0.,1076.73142393294,424.620242579854));
#128842=CARTESIAN_POINT('Origin',(0.,1082.7251047501,424.620242579854));
#128843=CARTESIAN_POINT('Origin',(0.,1076.73142393294,424.620242579854));
#128844=CARTESIAN_POINT('Origin',(0.,1082.7251047501,424.620242579854));
#128845=CARTESIAN_POINT('Origin',(0.,1076.73142393294,424.620242579854));
#128846=CARTESIAN_POINT('Origin',(0.,1082.7251047501,424.620242579854));
#128847=CARTESIAN_POINT('Origin',(0.,1076.73142393294,424.620242579854));
#128848=CARTESIAN_POINT('Origin',(0.,1082.7251047501,424.620242579854));
#128849=CARTESIAN_POINT('Origin',(0.,1076.73142393294,424.620242579854));
#128850=CARTESIAN_POINT('Origin',(0.,1082.7251047501,424.620242579854));
#128851=CARTESIAN_POINT('Origin',(0.,1076.73142393294,424.620242579854));
#128852=CARTESIAN_POINT('Origin',(0.,1082.7251047501,424.620242579854));
#128853=CARTESIAN_POINT('Origin',(0.,1076.73142393294,424.620242579854));
#128854=CARTESIAN_POINT('Origin',(0.,1082.7251047501,424.620242579854));
#128855=CARTESIAN_POINT('Origin',(0.,1076.73142393294,424.620242579854));
#128856=CARTESIAN_POINT('Origin',(0.,1082.7251047501,424.620242579854));
#128857=CARTESIAN_POINT('Origin',(0.,1076.73142393294,424.620242579854));
#128858=CARTESIAN_POINT('Origin',(0.,1082.7251047501,424.620242579854));
#128859=CARTESIAN_POINT('Origin',(0.,1076.73142393294,424.620242579854));
#128860=CARTESIAN_POINT('Origin',(0.,1082.7251047501,424.620242579854));
#128861=CARTESIAN_POINT('Ctrl Pts',(-98.3487995443478,1075.53620292392,
385.104677429649));
#128862=CARTESIAN_POINT('Ctrl Pts',(-98.629240211509,1075.53620292392,385.802655627705));
#128863=CARTESIAN_POINT('Ctrl Pts',(-98.9022349770337,1075.53620292392,
386.50357958275));
#128864=CARTESIAN_POINT('Ctrl Pts',(-99.1677529050815,1075.53620292392,
387.207369865892));
#128865=CARTESIAN_POINT('Ctrl Pts',(-97.654964079969,1075.61786654403,385.383453587804));
#128866=CARTESIAN_POINT('Ctrl Pts',(-97.9334262818979,1075.61786654403,
386.076507658373));
#128867=CARTESIAN_POINT('Ctrl Pts',(-98.2044951118669,1075.61786654403,
386.772486704074));
#128868=CARTESIAN_POINT('Ctrl Pts',(-98.4681398522829,1075.61786654403,
387.471311856374));
#128869=CARTESIAN_POINT('Ctrl Pts',(-96.9644573915014,1075.69533882439,
385.660892277053));
#128870=CARTESIAN_POINT('Ctrl Pts',(-97.240950620171,1075.69533882439,386.349045844348));
#128871=CARTESIAN_POINT('Ctrl Pts',(-97.5101027545383,1075.69533882439,
387.040103704622));
#128872=CARTESIAN_POINT('Ctrl Pts',(-97.7718832942109,1075.69533882439,
387.733987547012));
#128873=CARTESIAN_POINT('Ctrl Pts',(-96.2772807018516,1075.76862178799,
385.936993006044));
#128874=CARTESIAN_POINT('Ctrl Pts',(-96.5518144527218,1075.76862178799,
386.620269702957));
#128875=CARTESIAN_POINT('Ctrl Pts',(-96.8190591348362,1075.76862178799,
387.306430110437));
#128876=CARTESIAN_POINT('Ctrl Pts',(-97.0789844639553,1075.76862178799,
387.995396472602));
#128877=CARTESIAN_POINT('Origin',(0.,1082.7251047501,424.620242579854));
#128878=CARTESIAN_POINT('Ctrl Pts',(-99.649831526399,1074.6499846452,371.148967657458));
#128879=CARTESIAN_POINT('Ctrl Pts',(-100.003261188269,1074.6499846452,371.807624222369));
#128880=CARTESIAN_POINT('Ctrl Pts',(-100.350143399903,1074.6499846452,372.469752403044));
#128881=CARTESIAN_POINT('Ctrl Pts',(-100.690444064651,1074.6499846452,373.135287115859));
#128882=CARTESIAN_POINT('Ctrl Pts',(-98.9960442017051,1074.75386596962,
371.499784525324));
#128883=CARTESIAN_POINT('Ctrl Pts',(-99.3471550655449,1074.75386596962,
372.154119745113));
#128884=CARTESIAN_POINT('Ctrl Pts',(-99.6917614359683,1074.75386596962,
372.811903803923));
#128885=CARTESIAN_POINT('Ctrl Pts',(-100.029829440031,1074.75386596962,
373.473072045138));
#128886=CARTESIAN_POINT('Ctrl Pts',(-98.3451877959452,1074.85385082036,
371.849028686346));
#128887=CARTESIAN_POINT('Ctrl Pts',(-98.6939902568916,1074.85385082036,
372.499061933538));
#128888=CARTESIAN_POINT('Ctrl Pts',(-99.0363309886679,1074.85385082036,
373.152521345119));
#128889=CARTESIAN_POINT('Ctrl Pts',(-99.3721763410299,1074.85385082036,
373.809342689561));
#128890=CARTESIAN_POINT('Ctrl Pts',(-97.6972633477068,1074.94994100663,
372.196699583225));
#128891=CARTESIAN_POINT('Ctrl Pts',(-98.0437678045809,1074.94994100663,
372.842450237212));
#128892=CARTESIAN_POINT('Ctrl Pts',(-98.383853103888,1074.94994100663,373.4916044831));
#128893=CARTESIAN_POINT('Ctrl Pts',(-98.7174858170808,1074.94994100663,
374.144098512532));
#128894=CARTESIAN_POINT('Origin',(0.,1082.7251047501,424.620242579854));
#128895=CARTESIAN_POINT('Ctrl Pts',(-94.3883656101975,1076.25696242948,
398.145298833932));
#128896=CARTESIAN_POINT('Ctrl Pts',(-94.6250421977941,1076.25696242948,
398.989097275803));
#128897=CARTESIAN_POINT('Ctrl Pts',(-94.8503832990042,1076.25696242948,
399.835993376708));
#128898=CARTESIAN_POINT('Ctrl Pts',(-95.064348397423,1076.25696242948,400.685834864445));
#128899=CARTESIAN_POINT('Ctrl Pts',(-93.5499215982822,1076.31899804589,
398.380473560245));
#128900=CARTESIAN_POINT('Ctrl Pts',(-93.7844958074093,1076.31899804589,
399.216776610643));
#128901=CARTESIAN_POINT('Ctrl Pts',(-94.0078352223339,1076.31899804589,
400.056149803825));
#128902=CARTESIAN_POINT('Ctrl Pts',(-94.2198996865552,1076.31899804589,
400.898442220214));
#128903=CARTESIAN_POINT('Ctrl Pts',(-92.7165113242668,1076.37494427844,
398.614236376025));
#128904=CARTESIAN_POINT('Ctrl Pts',(-92.9489957769028,1076.37494427844,
399.443089034776));
#128905=CARTESIAN_POINT('Ctrl Pts',(-93.1703455229981,1076.37494427844,
400.274984485262));
#128906=CARTESIAN_POINT('Ctrl Pts',(-93.380520763795,1076.37494427844,401.109773152406));
#128907=CARTESIAN_POINT('Ctrl Pts',(-91.8881370161384,1076.42480467903,
398.846586656342));
#128908=CARTESIAN_POINT('Ctrl Pts',(-92.1185443398482,1076.42480467903,
399.668033943192));
#128909=CARTESIAN_POINT('Ctrl Pts',(-92.3379164398894,1076.42480467903,
400.492496836));
#128910=CARTESIAN_POINT('Ctrl Pts',(-92.5462138730855,1076.42480467903,
401.319827096063));
#128911=CARTESIAN_POINT('Origin',(0.,1082.7251047501,424.620242579854));
#128912=CARTESIAN_POINT('Ctrl Pts',(-89.8068600050043,1076.62748242345,
409.571133399922));
#128913=CARTESIAN_POINT('Ctrl Pts',(-89.9752215487277,1076.62748242345,
410.575845466703));
#128914=CARTESIAN_POINT('Ctrl Pts',(-90.1267006838473,1076.62748242345,
411.583241127883));
#128915=CARTESIAN_POINT('Ctrl Pts',(-90.2612547574608,1076.62748242345,
412.593036724929));
#128916=CARTESIAN_POINT('Ctrl Pts',(-88.8113461800284,1076.66225518595,
409.73795357648));
#128917=CARTESIAN_POINT('Ctrl Pts',(-88.977841427075,1076.66225518595,410.731528356505));
#128918=CARTESIAN_POINT('Ctrl Pts',(-89.1276414079163,1076.66225518595,
411.727756983141));
#128919=CARTESIAN_POINT('Ctrl Pts',(-89.2607039424593,1076.66225518595,
412.726358942227));
#128920=CARTESIAN_POINT('Ctrl Pts',(-87.8232439306037,1076.68829918657,
409.903531780993));
#128921=CARTESIAN_POINT('Ctrl Pts',(-87.9878867755057,1076.68829918657,
410.886052191082));
#128922=CARTESIAN_POINT('Ctrl Pts',(-88.1360201033303,1076.68829918657,
411.871196921468));
#128923=CARTESIAN_POINT('Ctrl Pts',(-88.267602203274,1076.68829918657,412.858688578948));
#128924=CARTESIAN_POINT('Ctrl Pts',(-86.8425571826817,1076.70562053557,
410.06786735558));
#128925=CARTESIAN_POINT('Ctrl Pts',(-87.0053615273314,1076.70562053557,
411.039416356477));
#128926=CARTESIAN_POINT('Ctrl Pts',(-87.1518407100228,1076.70562053557,
412.013560372944));
#128927=CARTESIAN_POINT('Ctrl Pts',(-87.2819534857204,1076.70562053557,
412.990025109318));
#128928=CARTESIAN_POINT('Origin',(0.,1082.7251047501,424.620242579854));
#128929=CARTESIAN_POINT('Ctrl Pts',(-86.3584302894826,1074.64930692473,
351.59570928573));
#128930=CARTESIAN_POINT('Ctrl Pts',(-86.8398187017703,1074.64930692473,
352.164996698732));
#128931=CARTESIAN_POINT('Ctrl Pts',(-87.315554525217,1074.64930692473,352.739016200472));
#128932=CARTESIAN_POINT('Ctrl Pts',(-87.7855912457502,1074.64930692473,
353.317711667395));
#128933=CARTESIAN_POINT('Ctrl Pts',(-85.7921843593031,1074.75314553403,
352.074525825614));
#128934=CARTESIAN_POINT('Ctrl Pts',(-86.2704163428741,1074.75314553403,
352.640080462562));
#128935=CARTESIAN_POINT('Ctrl Pts',(-86.743032801217,1074.75314553403,353.210336160286));
#128936=CARTESIAN_POINT('Ctrl Pts',(-87.2099875252486,1074.75314553403,
353.785237163231));
#128937=CARTESIAN_POINT('Ctrl Pts',(-85.2284753922116,1074.85309213932,
352.551197114076));
#128938=CARTESIAN_POINT('Ctrl Pts',(-85.7035650888773,1074.85309213932,
353.113035699));
#128939=CARTESIAN_POINT('Ctrl Pts',(-86.1730761578708,1074.85309213932,
353.679544455756));
#128940=CARTESIAN_POINT('Ctrl Pts',(-86.6369626937321,1074.85309213932,
354.250667995136));
#128941=CARTESIAN_POINT('Ctrl Pts',(-84.6673042866797,1074.94914854672,
353.025722391367));
#128942=CARTESIAN_POINT('Ctrl Pts',(-85.1392658432598,1074.94914854672,
353.583861654224));
#128943=CARTESIAN_POINT('Ctrl Pts',(-85.6056855036081,1074.94914854672,
354.146640339031));
#128944=CARTESIAN_POINT('Ctrl Pts',(-86.0665176645205,1074.94914854672,
354.714003421281));
#128945=CARTESIAN_POINT('Origin',(0.,1082.7251047501,424.620242579854));
#128946=CARTESIAN_POINT('Ctrl Pts',(-87.9863052406897,1075.53617638582,
365.523475655949));
#128947=CARTESIAN_POINT('Ctrl Pts',(-88.4058111505509,1075.53617638582,
366.148057624754));
#128948=CARTESIAN_POINT('Ctrl Pts',(-88.8186430196475,1075.53617638582,
366.777070893312));
#128949=CARTESIAN_POINT('Ctrl Pts',(-89.2247540438749,1075.53617638582,
367.410444148325));
#128950=CARTESIAN_POINT('Ctrl Pts',(-87.3640928236274,1075.6180360885,365.94139003578));
#128951=CARTESIAN_POINT('Ctrl Pts',(-87.780632115156,1075.6180360885,366.561555150674));
#128952=CARTESIAN_POINT('Ctrl Pts',(-88.1905445627084,1075.6180360885,367.186120228515));
#128953=CARTESIAN_POINT('Ctrl Pts',(-88.5937836931645,1075.6180360885,367.815014460311));
#128954=CARTESIAN_POINT('Ctrl Pts',(-86.7448726917102,1075.69568439305,
366.357294621277));
#128955=CARTESIAN_POINT('Ctrl Pts',(-87.1584596316867,1075.69568439305,
366.973064123375));
#128956=CARTESIAN_POINT('Ctrl Pts',(-87.5654666975011,1075.69568439305,
367.593202402318));
#128957=CARTESIAN_POINT('Ctrl Pts',(-87.965847745426,1075.69568439305,368.217639150992));
#128958=CARTESIAN_POINT('Ctrl Pts',(-86.1286459468542,1075.76912333699,
366.771188672327));
#128959=CARTESIAN_POINT('Ctrl Pts',(-86.5392948073127,1075.76912333699,
367.382583810569));
#128960=CARTESIAN_POINT('Ctrl Pts',(-86.9434105363655,1075.76912333699,
367.998316690309));
#128961=CARTESIAN_POINT('Ctrl Pts',(-87.3409473180852,1075.76912333699,
368.618317503889));
#128962=CARTESIAN_POINT('Origin',(0.,1082.7251047501,424.620242579854));
#128963=CARTESIAN_POINT('Ctrl Pts',(-86.8150232951319,1076.25735809069,
379.099381006362));
#128964=CARTESIAN_POINT('Ctrl Pts',(-87.2224634623205,1076.25735809069,
379.876429734861));
#128965=CARTESIAN_POINT('Ctrl Pts',(-87.6194349295328,1076.25735809069,
380.658878372485));
#128966=CARTESIAN_POINT('Ctrl Pts',(-88.0058661457325,1076.25735809069,
381.446585888919));
#128967=CARTESIAN_POINT('Ctrl Pts',(-86.0454051748305,1076.31924104508,
379.502924985146));
#128968=CARTESIAN_POINT('Ctrl Pts',(-86.4492333711446,1076.31924104508,
380.273085150362));
#128969=CARTESIAN_POINT('Ctrl Pts',(-86.8426856728622,1076.31924104508,
381.048597354327));
#128970=CARTESIAN_POINT('Ctrl Pts',(-87.2256911632491,1076.31924104508,
381.829321816963));
#128971=CARTESIAN_POINT('Ctrl Pts',(-85.2803982612145,1076.37505949439,
379.904051109354));
#128972=CARTESIAN_POINT('Ctrl Pts',(-85.6806361279641,1076.37505949439,
380.667363984471));
#128973=CARTESIAN_POINT('Ctrl Pts',(-86.0705903494486,1076.37505949439,
381.435981314777));
#128974=CARTESIAN_POINT('Ctrl Pts',(-86.4501906394357,1076.37505949439,
382.209764562942));
#128975=CARTESIAN_POINT('Ctrl Pts',(-84.5200045910798,1076.42481696877,
380.302758311009));
#128976=CARTESIAN_POINT('Ctrl Pts',(-84.9166737791338,1076.42481696877,
381.059265187439));
#128977=CARTESIAN_POINT('Ctrl Pts',(-85.3031510149603,1076.42481696877,
381.821029222443));
#128978=CARTESIAN_POINT('Ctrl Pts',(-85.6793666390268,1076.42481696877,
382.587913113945));
#128979=CARTESIAN_POINT('Origin',(0.,1082.7251047501,424.620242579854));
#128980=CARTESIAN_POINT('Ctrl Pts',(-84.7179661437949,1076.62733369941,
391.222638015823));
#128981=CARTESIAN_POINT('Ctrl Pts',(-85.0910907886886,1076.62733369941,
392.169123892465));
#128982=CARTESIAN_POINT('Ctrl Pts',(-85.4483030389599,1076.62733369941,
393.121729227095));
#128983=CARTESIAN_POINT('Ctrl Pts',(-85.7895025866761,1076.62733369941,
394.080186520848));
#128984=CARTESIAN_POINT('Ctrl Pts',(-83.7798178484809,1076.66209686976,
391.59247581075));
#128985=CARTESIAN_POINT('Ctrl Pts',(-84.1488105923685,1076.66209686976,
392.528480509052));
#128986=CARTESIAN_POINT('Ctrl Pts',(-84.502067152024,1076.66209686976,393.470536899799));
#128987=CARTESIAN_POINT('Ctrl Pts',(-84.8394883303031,1076.66209686976,
394.418380446348));
#128988=CARTESIAN_POINT('Ctrl Pts',(-82.8486469713158,1076.68814855513,
391.95956296065));
#128989=CARTESIAN_POINT('Ctrl Pts',(-83.2135385449476,1076.68814855513,
392.885164433709));
#128990=CARTESIAN_POINT('Ctrl Pts',(-83.5628688341843,1076.68814855513,
393.81675033767));
#128991=CARTESIAN_POINT('Ctrl Pts',(-83.8965397444081,1076.68814855513,
394.754059076083));
#128992=CARTESIAN_POINT('Ctrl Pts',(-81.924457204617,1076.70549484766,392.323898009936));
#128993=CARTESIAN_POINT('Ctrl Pts',(-82.2852783550056,1076.70549484766,
393.239174252098));
#128994=CARTESIAN_POINT('Ctrl Pts',(-82.6307118095888,1076.70549484766,
394.160368167888));
#128995=CARTESIAN_POINT('Ctrl Pts',(-82.96066056801,1076.70549484766,395.087221079007));
#128996=CARTESIAN_POINT('Origin',(0.,1082.7251047501,424.620242579854));
#128997=CARTESIAN_POINT('Ctrl Pts',(-69.2937118359578,1074.64931581022,
335.240557572053));
#128998=CARTESIAN_POINT('Ctrl Pts',(-69.8828803090973,1074.64931581022,
335.697324346259));
#128999=CARTESIAN_POINT('Ctrl Pts',(-70.4675037924513,1074.64931581022,
336.15989407989));
#129000=CARTESIAN_POINT('Ctrl Pts',(-71.0475251325708,1074.64931581022,
336.628221551608));
#129001=CARTESIAN_POINT('Ctrl Pts',(-68.8381453304565,1074.75343131481,
335.828177857977));
#129002=CARTESIAN_POINT('Ctrl Pts',(-69.4234403580071,1074.75343131481,
336.281941652004));
#129003=CARTESIAN_POINT('Ctrl Pts',(-70.0042202764792,1074.75343131481,
336.741470254319));
#129004=CARTESIAN_POINT('Ctrl Pts',(-70.5804283081752,1074.75343131481,
337.206718740888));
#129005=CARTESIAN_POINT('Ctrl Pts',(-68.3846253564385,1074.85363401426,
336.413158390099));
#129006=CARTESIAN_POINT('Ctrl Pts',(-68.9660643389952,1074.85363401426,
336.86393269417));
#129007=CARTESIAN_POINT('Ctrl Pts',(-69.5430179589482,1074.85363401426,
337.320433826776));
#129008=CARTESIAN_POINT('Ctrl Pts',(-70.1154298126631,1074.85363401426,
337.782617159852));
#129009=CARTESIAN_POINT('Ctrl Pts',(-67.933152640622,1074.94992572917,336.995498231047));
#129010=CARTESIAN_POINT('Ctrl Pts',(-68.5107529849589,1074.94992572917,
337.443296540175));
#129011=CARTESIAN_POINT('Ctrl Pts',(-69.0838975788868,1074.94992572917,
337.896783869531));
#129012=CARTESIAN_POINT('Ctrl Pts',(-69.6525303911459,1074.94992572917,
338.355915885685));
#129013=CARTESIAN_POINT('Origin',(0.,1082.7251047501,424.620242579854));
#129014=CARTESIAN_POINT('Ctrl Pts',(-73.7691873467676,1075.53681660702,
348.522397650382));
#129015=CARTESIAN_POINT('Ctrl Pts',(-74.3105270143456,1075.53681660702,
349.047171872212));
#129016=CARTESIAN_POINT('Ctrl Pts',(-74.8462364222988,1075.53681660702,
349.5776924183));
#129017=CARTESIAN_POINT('Ctrl Pts',(-75.3762545767591,1075.53681660702,
350.113898885561));
#129018=CARTESIAN_POINT('Ctrl Pts',(-73.2488932306589,1075.61843552384,
349.059115789613));
#129019=CARTESIAN_POINT('Ctrl Pts',(-73.7864148292844,1075.61843552384,
349.580188778588));
#129020=CARTESIAN_POINT('Ctrl Pts',(-74.3183458785092,1075.61843552384,
350.106967562993));
#129021=CARTESIAN_POINT('Ctrl Pts',(-74.8446258146548,1075.61843552384,
350.639392165767));
#129022=CARTESIAN_POINT('Ctrl Pts',(-72.7310946383515,1075.6958655393,349.593259629329));
#129023=CARTESIAN_POINT('Ctrl Pts',(-73.2648164809012,1075.6958655393,350.110649137936));
#129024=CARTESIAN_POINT('Ctrl Pts',(-73.7929872938091,1075.6958655393,350.633704107536));
#129025=CARTESIAN_POINT('Ctrl Pts',(-74.3155469415234,1075.6958655393,351.162364985049));
#129026=CARTESIAN_POINT('Ctrl Pts',(-72.2157924863696,1075.76910867463,
350.124828224073));
#129027=CARTESIAN_POINT('Ctrl Pts',(-72.7457328924458,1075.76910867463,
350.63855201132));
#129028=CARTESIAN_POINT('Ctrl Pts',(-73.2701615981042,1075.76910867463,
351.157901119585));
#129029=CARTESIAN_POINT('Ctrl Pts',(-73.7890188938555,1075.76910867463,
351.682816417725));
#129030=CARTESIAN_POINT('Origin',(0.,1082.7251047501,424.620242579854));
#129031=CARTESIAN_POINT('Ctrl Pts',(-75.4581277762219,1076.25692467333,
362.040205265552));
#129032=CARTESIAN_POINT('Ctrl Pts',(-76.0168599993451,1076.25692467333,
362.713916712436));
#129033=CARTESIAN_POINT('Ctrl Pts',(-76.5665200306141,1076.25692467333,
363.395050077384));
#129034=CARTESIAN_POINT('Ctrl Pts',(-77.1070092920242,1076.25692467333,
364.08348320349));
#129035=CARTESIAN_POINT('Ctrl Pts',(-74.7894053761516,1076.31881801516,
362.594799899458));
#129036=CARTESIAN_POINT('Ctrl Pts',(-75.3431860219661,1076.31881801516,
363.262540804149));
#129037=CARTESIAN_POINT('Ctrl Pts',(-75.8879748751902,1076.31881801516,
363.937637852639));
#129038=CARTESIAN_POINT('Ctrl Pts',(-76.4236742314337,1076.31881801516,
364.619969970597));
#129039=CARTESIAN_POINT('Ctrl Pts',(-74.124688384805,1076.37465035438,363.146072709264));
#129040=CARTESIAN_POINT('Ctrl Pts',(-74.6735471114934,1076.37465035438,
363.807878833181));
#129041=CARTESIAN_POINT('Ctrl Pts',(-75.2134939632922,1076.37465035438,
364.476975720596));
#129042=CARTESIAN_POINT('Ctrl Pts',(-75.744432104193,1076.37465035438,365.15324337327));
#129043=CARTESIAN_POINT('Ctrl Pts',(-73.4639785708834,1076.42442521807,
363.694022228125));
#129044=CARTESIAN_POINT('Ctrl Pts',(-74.0079450497246,1076.42442521807,
364.349929348478));
#129045=CARTESIAN_POINT('Ctrl Pts',(-74.5430790896012,1076.42442521807,
365.013062246167));
#129046=CARTESIAN_POINT('Ctrl Pts',(-75.0692847176521,1076.42442521807,
365.683301992556));
#129047=CARTESIAN_POINT('Origin',(0.,1082.7251047501,424.620242579854));
#129048=CARTESIAN_POINT('Ctrl Pts',(-75.9265346513598,1076.62732561046,
374.343629244776));
#129049=CARTESIAN_POINT('Ctrl Pts',(-76.4886562467854,1076.62732561046,
375.192531785385));
#129050=CARTESIAN_POINT('Ctrl Pts',(-77.0364633027961,1076.62732561046,
376.050741340727));
#129051=CARTESIAN_POINT('Ctrl Pts',(-77.56980176015,1076.62732561046,376.91801655737));
#129052=CARTESIAN_POINT('Ctrl Pts',(-75.0834901232,1076.6621832391,374.901871813875));
#129053=CARTESIAN_POINT('Ctrl Pts',(-75.639370244056,1076.6621832391,375.741348629405));
#129054=CARTESIAN_POINT('Ctrl Pts',(-76.1810947659015,1076.6621832391,376.590029119935));
#129055=CARTESIAN_POINT('Ctrl Pts',(-76.7085113400799,1076.6621832391,377.447674611882));
#129056=CARTESIAN_POINT('Ctrl Pts',(-74.2467324701365,1076.68828265731,
375.455951374748));
#129057=CARTESIAN_POINT('Ctrl Pts',(-74.796417661261,1076.68828265731,376.286072756096));
#129058=CARTESIAN_POINT('Ctrl Pts',(-75.3321050085058,1076.68828265731,
377.125295243352));
#129059=CARTESIAN_POINT('Ctrl Pts',(-75.8536438610429,1076.68828265731,
377.973382822797));
#129060=CARTESIAN_POINT('Ctrl Pts',(-73.4162650279748,1076.70563000628,
376.00586571851));
#129061=CARTESIAN_POINT('Ctrl Pts',(-73.9598018589024,1076.70563000628,
376.82670199387));
#129062=CARTESIAN_POINT('Ctrl Pts',(-74.4894974151786,1076.70563000628,
377.656537577094));
#129063=CARTESIAN_POINT('Ctrl Pts',(-75.0052027310409,1076.70563000628,
378.495139094332));
#129064=CARTESIAN_POINT('Origin',(0.,1082.7251047501,424.620242579854));
#129065=CARTESIAN_POINT('Ctrl Pts',(-49.1887364726124,1074.64986286691,
322.787383952035));
#129066=CARTESIAN_POINT('Ctrl Pts',(-49.861949754311,1074.64986286691,323.112568879077));
#129067=CARTESIAN_POINT('Ctrl Pts',(-50.5319053641702,1074.64986286691,
323.444413481638));
#129068=CARTESIAN_POINT('Ctrl Pts',(-51.1985374242161,1074.64986286691,
323.782885128825));
#129069=CARTESIAN_POINT('Ctrl Pts',(-48.8659612240735,1074.75376552472,
323.455608602841));
#129070=CARTESIAN_POINT('Ctrl Pts',(-49.5347568971914,1074.75376552472,
323.778659674591));
#129071=CARTESIAN_POINT('Ctrl Pts',(-50.2003162752302,1074.75376552472,
324.108326721237));
#129072=CARTESIAN_POINT('Ctrl Pts',(-50.8625739125059,1074.75376552472,
324.444577326009));
#129073=CARTESIAN_POINT('Ctrl Pts',(-48.544633221678,1074.85377033612,324.12083709594));
#129074=CARTESIAN_POINT('Ctrl Pts',(-49.2090310937035,1074.85377033612,
324.441763880088));
#129075=CARTESIAN_POINT('Ctrl Pts',(-49.8702139515621,1074.85377033612,
324.769263134453));
#129076=CARTESIAN_POINT('Ctrl Pts',(-50.5281167799212,1074.85377033612,
325.103302655427));
#129077=CARTESIAN_POINT('Ctrl Pts',(-48.2247529783561,1074.94987911127,
324.783068369438));
#129078=CARTESIAN_POINT('Ctrl Pts',(-48.8847728637976,1074.94987911127,
325.101880437067));
#129079=CARTESIAN_POINT('Ctrl Pts',(-49.5415989201024,1074.94987911127,
325.427221666245));
#129080=CARTESIAN_POINT('Ctrl Pts',(-50.19516656035,1074.94987911127,325.759060065568));
#129081=CARTESIAN_POINT('Origin',(0.,1082.7251047501,424.620242579854));
#129082=CARTESIAN_POINT('Ctrl Pts',(-56.3385706144534,1075.53620324036,
334.843123513399));
#129083=CARTESIAN_POINT('Ctrl Pts',(-56.9759578646755,1075.53620324036,
335.243108353399));
#129084=CARTESIAN_POINT('Ctrl Pts',(-57.6090494979524,1075.53620324036,
335.649858107977));
#129085=CARTESIAN_POINT('Ctrl Pts',(-58.2377737176665,1075.53620324036,
336.063326649126));
#129086=CARTESIAN_POINT('Ctrl Pts',(-55.9408904765946,1075.61791211129,
335.47683815503));
#129087=CARTESIAN_POINT('Ctrl Pts',(-56.5737785667072,1075.61791211129,
335.873999600247));
#129088=CARTESIAN_POINT('Ctrl Pts',(-57.2024013615799,1075.61791211129,
336.277878208172));
#129089=CARTESIAN_POINT('Ctrl Pts',(-57.8266875713899,1075.61791211129,
336.688428176403));
#129090=CARTESIAN_POINT('Ctrl Pts',(-55.5451193241529,1075.69542499513,
336.107510773953));
#129091=CARTESIAN_POINT('Ctrl Pts',(-56.1735298514906,1075.69542499513,
336.50186237754));
#129092=CARTESIAN_POINT('Ctrl Pts',(-56.7977052597404,1075.69542499513,
336.902883621188));
#129093=CARTESIAN_POINT('Ctrl Pts',(-57.4175747634414,1075.69542499513,
337.310529026537));
#129094=CARTESIAN_POINT('Ctrl Pts',(-55.1512578588289,1075.76874391824,
336.73514025199));
#129095=CARTESIAN_POINT('Ctrl Pts',(-55.7752124286652,1075.76874391824,
337.126695572081));
#129096=CARTESIAN_POINT('Ctrl Pts',(-56.3949619099586,1075.76874391824,
337.524873238893));
#129097=CARTESIAN_POINT('Ctrl Pts',(-57.0104360191766,1075.76874391824,
337.929628096546));
#129098=CARTESIAN_POINT('Origin',(0.,1082.7251047501,424.620242579854));
#129099=CARTESIAN_POINT('Ctrl Pts',(-60.8036583368741,1076.25693403304,
347.723691993978));
#129100=CARTESIAN_POINT('Ctrl Pts',(-61.4899622341832,1076.25693403304,
348.266366371038));
#129101=CARTESIAN_POINT('Ctrl Pts',(-62.1689399918952,1076.25693403304,
348.81817949476));
#129102=CARTESIAN_POINT('Ctrl Pts',(-62.8404699284279,1076.25693403304,
349.379032473106));
#129103=CARTESIAN_POINT('Ctrl Pts',(-60.2634899240499,1076.31897791375,
348.406826673992));
#129104=CARTESIAN_POINT('Ctrl Pts',(-60.9436968249437,1076.31897791375,
348.94468003263));
#129105=CARTESIAN_POINT('Ctrl Pts',(-61.6166426703044,1076.31897791375,
349.491590951002));
#129106=CARTESIAN_POINT('Ctrl Pts',(-62.2822068595465,1076.31897791375,
350.047461415607));
#129107=CARTESIAN_POINT('Ctrl Pts',(-59.7265648307342,1076.37493115239,
349.085859625763));
#129108=CARTESIAN_POINT('Ctrl Pts',(-60.4007113432535,1076.37493115239,
349.618920912699));
#129109=CARTESIAN_POINT('Ctrl Pts',(-61.0676614935213,1076.37493115239,
350.160959059907));
#129110=CARTESIAN_POINT('Ctrl Pts',(-61.7272957554581,1076.37493115239,
350.711876927153));
#129111=CARTESIAN_POINT('Ctrl Pts',(-59.1928844926034,1076.42479730197,
349.760789033635));
#129112=CARTESIAN_POINT('Ctrl Pts',(-59.8610072409942,1076.42479730197,
350.2890872084));
#129113=CARTESIAN_POINT('Ctrl Pts',(-60.5219979294594,1076.42479730197,
350.826282031662));
#129114=CARTESIAN_POINT('Ctrl Pts',(-61.175738099932,1076.42479730197,351.372277231172));
#129115=CARTESIAN_POINT('Origin',(0.,1082.7251047501,424.620242579854));
#129116=CARTESIAN_POINT('Ctrl Pts',(-63.8042737731188,1076.62756831568,
359.656342770107));
#129117=CARTESIAN_POINT('Ctrl Pts',(-64.5322278769664,1076.62756831568,
360.371302664328));
#129118=CARTESIAN_POINT('Ctrl Pts',(-65.2480630511544,1076.62756831568,
361.098396077204));
#129119=CARTESIAN_POINT('Ctrl Pts',(-65.9515770830636,1076.62756831568,
361.837417615835));
#129120=CARTESIAN_POINT('Ctrl Pts',(-63.0975147104926,1076.66230088097,
360.375946994384));
#129121=CARTESIAN_POINT('Ctrl Pts',(-63.8174052767486,1076.66230088097,
361.082987287695));
#129122=CARTESIAN_POINT('Ctrl Pts',(-64.5253111545621,1076.66230088097,
361.802026696842));
#129123=CARTESIAN_POINT('Ctrl Pts',(-65.2210323712204,1076.66230088097,
362.532862104058));
#129124=CARTESIAN_POINT('Ctrl Pts',(-62.3960136094621,1076.68831765292,
361.090197694985));
#129125=CARTESIAN_POINT('Ctrl Pts',(-63.1079006271289,1076.68831765292,
361.789377305565));
#129126=CARTESIAN_POINT('Ctrl Pts',(-63.8079361988774,1076.68831765292,
362.500422629057));
#129127=CARTESIAN_POINT('Ctrl Pts',(-64.4959225752375,1076.68831765292,
363.223132805903));
#129128=CARTESIAN_POINT('Ctrl Pts',(-61.6997732531278,1076.7056247282,361.799092038227));
#129129=CARTESIAN_POINT('Ctrl Pts',(-62.4037167429603,1076.7056247282,362.490469915442));
#129130=CARTESIAN_POINT('Ctrl Pts',(-63.0959410301775,1076.7056247282,363.193581103069));
#129131=CARTESIAN_POINT('Ctrl Pts',(-63.7762505718791,1076.7056247282,363.908226982823));
#129132=CARTESIAN_POINT('Origin',(0.,1082.7251047501,424.620242579854));
#129133=CARTESIAN_POINT('Ctrl Pts',(-26.9425711955054,1074.64941712613,
314.782722615003));
#129134=CARTESIAN_POINT('Ctrl Pts',(-27.6676358963114,1074.64941712613,
314.960577207214));
#129135=CARTESIAN_POINT('Ctrl Pts',(-28.3909040175034,1074.64941712613,
315.145602343865));
#129136=CARTESIAN_POINT('Ctrl Pts',(-29.1123046476605,1074.64941712613,
315.337779884526));
#129137=CARTESIAN_POINT('Ctrl Pts',(-26.7656745127426,1074.75339142399,
315.503882180053));
#129138=CARTESIAN_POINT('Ctrl Pts',(-27.4859786604659,1074.75339142399,
315.680569033404));
#129139=CARTESIAN_POINT('Ctrl Pts',(-28.2044980243675,1074.75339142399,
315.864379351593));
#129140=CARTESIAN_POINT('Ctrl Pts',(-28.9211621586091,1074.75339142399,
316.055295113295));
#129141=CARTESIAN_POINT('Ctrl Pts',(-26.5895714430747,1074.85346333329,
316.221806400802));
#129142=CARTESIAN_POINT('Ctrl Pts',(-27.3051363950251,1074.85346333329,
316.39733075413));
#129143=CARTESIAN_POINT('Ctrl Pts',(-28.0189283060266,1074.85346333329,
316.579931703908));
#129144=CARTESIAN_POINT('Ctrl Pts',(-28.7308771937348,1074.85346333329,
316.76959134738));
#129145=CARTESIAN_POINT('Ctrl Pts',(-26.4142622679364,1074.9496346674,316.936494129919));
#129146=CARTESIAN_POINT('Ctrl Pts',(-27.1251093889977,1074.9496346674,317.110861223917));
#129147=CARTESIAN_POINT('Ctrl Pts',(-27.8341951590444,1074.9496346674,317.292258257267));
#129148=CARTESIAN_POINT('Ctrl Pts',(-28.5414500571367,1074.9496346674,317.480667445246));
#129149=CARTESIAN_POINT('Origin',(0.,1082.7251047501,424.620242579854));
#129150=CARTESIAN_POINT('Ctrl Pts',(-36.4456850718535,1075.53624331041,
325.093362237882));
#129151=CARTESIAN_POINT('Ctrl Pts',(-37.152037505206,1075.53624331041,325.352020986627));
#129152=CARTESIAN_POINT('Ctrl Pts',(-37.8555964276979,1075.53624331041,
325.61818437815));
#129153=CARTESIAN_POINT('Ctrl Pts',(-38.5562821088095,1075.53624331041,
325.891822249598));
#129154=CARTESIAN_POINT('Ctrl Pts',(-36.1881437694065,1075.61803963491,
325.796663118116));
#129155=CARTESIAN_POINT('Ctrl Pts',(-36.8895048045918,1075.61803963491,
326.053494069937));
#129156=CARTESIAN_POINT('Ctrl Pts',(-37.5880920690975,1075.61803963491,
326.317776633418));
#129157=CARTESIAN_POINT('Ctrl Pts',(-38.2838263958152,1075.61803963491,
326.589480858848));
#129158=CARTESIAN_POINT('Ctrl Pts',(-35.9318400894039,1075.69563084465,
326.4965842649));
#129159=CARTESIAN_POINT('Ctrl Pts',(-36.6282337127353,1075.69563084465,
326.751596203331));
#129160=CARTESIAN_POINT('Ctrl Pts',(-37.3218732107063,1075.69563084465,
327.014006977145));
#129161=CARTESIAN_POINT('Ctrl Pts',(-38.0126799769119,1075.69563084465,
327.28378684875));
#129162=CARTESIAN_POINT('Ctrl Pts',(-35.6767744872628,1075.76901897262,
327.193124434569));
#129163=CARTESIAN_POINT('Ctrl Pts',(-36.3682246938802,1075.76901897262,
327.446326146375));
#129164=CARTESIAN_POINT('Ctrl Pts',(-37.0569403255594,1075.76901897262,
327.706874172223));
#129165=CARTESIAN_POINT('Ctrl Pts',(-37.7428433338905,1075.76901897262,
327.974738985617));
#129166=CARTESIAN_POINT('Origin',(0.,1082.7251047501,424.620242579854));
#129167=CARTESIAN_POINT('Ctrl Pts',(-43.4792032208331,1076.25720649399,
336.762554668715));
#129168=CARTESIAN_POINT('Ctrl Pts',(-44.2653215602855,1076.25720649399,
337.151590618207));
#129169=CARTESIAN_POINT('Ctrl Pts',(-45.0461479884214,1076.25720649399,
337.551141744779));
#129170=CARTESIAN_POINT('Ctrl Pts',(-45.8215418613918,1076.25720649399,
337.96113608057));
#129171=CARTESIAN_POINT('Ctrl Pts',(-43.093582895018,1076.3191283065,337.541771115382));
#129172=CARTESIAN_POINT('Ctrl Pts',(-43.8727290917508,1076.3191283065,337.927356675757));
#129173=CARTESIAN_POINT('Ctrl Pts',(-44.6466303115269,1076.3191283065,338.323364153316));
#129174=CARTESIAN_POINT('Ctrl Pts',(-45.4151471578782,1076.3191283065,338.729722218484));
#129175=CARTESIAN_POINT('Ctrl Pts',(-42.7102740907138,1076.37497993555,
338.316316709769));
#129176=CARTESIAN_POINT('Ctrl Pts',(-43.4824899377986,1076.37497993555,
338.698472563673));
#129177=CARTESIAN_POINT('Ctrl Pts',(-44.2495074609481,1076.37497993555,
339.090957633891));
#129178=CARTESIAN_POINT('Ctrl Pts',(-45.0111885035979,1076.37497993555,
339.493701225312));
#129179=CARTESIAN_POINT('Ctrl Pts',(-42.3292778294105,1076.42476491624,
339.086189387768));
#129180=CARTESIAN_POINT('Ctrl Pts',(-43.0946051383877,1076.42476491624,
339.464936226988));
#129181=CARTESIAN_POINT('Ctrl Pts',(-43.8547804949884,1076.42476491624,
339.853920140925));
#129182=CARTESIAN_POINT('Ctrl Pts',(-44.6096669750714,1076.42476491624,
340.253071065104));
#129183=CARTESIAN_POINT('Origin',(0.,1082.7251047501,424.620242579854));
#129184=CARTESIAN_POINT('Ctrl Pts',(-48.9068694848042,1076.62734888474,
347.80506396164));
#129185=CARTESIAN_POINT('Ctrl Pts',(-49.7666339575146,1076.62734888474,
348.352460838284));
#129186=CARTESIAN_POINT('Ctrl Pts',(-50.6170879148582,1076.62734888474,
348.914213769326));
#129187=CARTESIAN_POINT('Ctrl Pts',(-51.4579916683211,1076.62734888474,
349.490164432584));
#129188=CARTESIAN_POINT('Ctrl Pts',(-48.3647367445688,1076.66214464411,
348.656560361116));
#129189=CARTESIAN_POINT('Ctrl Pts',(-49.2149707264819,1076.66214464411,
349.197889342353));
#129190=CARTESIAN_POINT('Ctrl Pts',(-50.0559974001086,1076.66214464411,
349.753415241098));
#129191=CARTESIAN_POINT('Ctrl Pts',(-50.8875797338825,1076.66214464411,
350.32298149017));
#129192=CARTESIAN_POINT('Ctrl Pts',(-47.8266401655489,1076.68821130439,
349.501717396655));
#129193=CARTESIAN_POINT('Ctrl Pts',(-48.6674146108693,1076.68821130439,
350.037023657776));
#129194=CARTESIAN_POINT('Ctrl Pts',(-49.4990841866101,1076.68821130439,
350.586368884283));
#129195=CARTESIAN_POINT('Ctrl Pts',(-50.3214144983718,1076.68821130439,
351.149598250933));
#129196=CARTESIAN_POINT('Ctrl Pts',(-47.2925818857626,1076.70555497619,
350.340531710195));
#129197=CARTESIAN_POINT('Ctrl Pts',(-48.1239677862803,1076.70555497619,
350.86986045042));
#129198=CARTESIAN_POINT('Ctrl Pts',(-48.9463504871448,1076.70555497619,
351.413071389307));
#129199=CARTESIAN_POINT('Ctrl Pts',(-49.759498211332,1076.70555497619,351.970011430476));
#129200=CARTESIAN_POINT('Origin',(0.,1082.7251047501,424.620242579854));
#129201=CARTESIAN_POINT('Ctrl Pts',(-3.52018246155676,1074.6501598088,311.586656837294));
#129202=CARTESIAN_POINT('Ctrl Pts',(-4.26598294102489,1074.6501598088,311.609883153175));
#129203=CARTESIAN_POINT('Ctrl Pts',(-5.0115170308526,1074.6501598088,311.64048932623));
#129204=CARTESIAN_POINT('Ctrl Pts',(-5.75671170754627,1074.6501598088,311.678472358649));
#129205=CARTESIAN_POINT('Ctrl Pts',(-3.49714761316157,1074.75376387604,
312.326309267126));
#129206=CARTESIAN_POINT('Ctrl Pts',(-4.23806783395981,1074.75376387604,
312.349383598083));
#129207=CARTESIAN_POINT('Ctrl Pts',(-4.97872340827869,1074.75376387604,
312.379789494998));
#129208=CARTESIAN_POINT('Ctrl Pts',(-5.71904179046491,1074.75376387604,
312.417523979677));
#129209=CARTESIAN_POINT('Ctrl Pts',(-3.47421575892244,1074.85349191521,
313.062654539192));
#129210=CARTESIAN_POINT('Ctrl Pts',(-4.21027754182053,1074.85349191521,
313.085577564784));
#129211=CARTESIAN_POINT('Ctrl Pts',(-4.94607641360625,1074.85349191521,
313.11578408104));
#129212=CARTESIAN_POINT('Ctrl Pts',(-5.68154030433007,1074.85349191521,
313.153271129294));
#129213=CARTESIAN_POINT('Ctrl Pts',(-3.45138693524003,1074.94934572131,
313.795691484659));
#129214=CARTESIAN_POINT('Ctrl Pts',(-4.18261210871973,1074.94934572131,
313.818463884687));
#129215=CARTESIAN_POINT('Ctrl Pts',(-4.9135760986572,1074.94934572131,313.848471916081));
#129216=CARTESIAN_POINT('Ctrl Pts',(-5.64420730866941,1074.94934572131,
313.885712639618));
#129217=CARTESIAN_POINT('Origin',(0.,1082.7251047501,424.620242579854));
#129218=CARTESIAN_POINT('Ctrl Pts',(-14.9526527161707,1075.53640608928,
319.691742708466));
#129219=CARTESIAN_POINT('Ctrl Pts',(-15.6983726462263,1075.53640608928,
319.798010225406));
#129220=CARTESIAN_POINT('Ctrl Pts',(-16.4429173934917,1075.53640608928,
319.912221076722));
#129221=CARTESIAN_POINT('Ctrl Pts',(-17.1862023488174,1075.53640608928,
320.034362283631));
#129222=CARTESIAN_POINT('Ctrl Pts',(-14.8472166832474,1075.61802125527,
320.431627796218));
#129223=CARTESIAN_POINT('Ctrl Pts',(-15.5876782987691,1075.61802125527,
320.537145986225));
#129224=CARTESIAN_POINT('Ctrl Pts',(-16.326973018098,1075.61802125527,320.650551499564));
#129225=CARTESIAN_POINT('Ctrl Pts',(-17.0650168286911,1075.61802125527,
320.771831448972));
#129226=CARTESIAN_POINT('Ctrl Pts',(-14.7422862420094,1075.69544934262,
321.167964953172));
#129227=CARTESIAN_POINT('Ctrl Pts',(-15.4775147579075,1075.69544934262,
321.272737409452));
#129228=CARTESIAN_POINT('Ctrl Pts',(-16.2115846244738,1075.69544934262,
321.385341446608));
#129229=CARTESIAN_POINT('Ctrl Pts',(-16.9444124229112,1075.69544934262,
321.505764268456));
#129230=CARTESIAN_POINT('Ctrl Pts',(-14.6378615781037,1075.76869237125,
321.900752876572));
#129231=CARTESIAN_POINT('Ctrl Pts',(-15.367882218547,1075.76869237125,322.00478319365));
#129232=CARTESIAN_POINT('Ctrl Pts',(-16.0967524167687,1075.76869237125,
322.116589617835));
#129233=CARTESIAN_POINT('Ctrl Pts',(-16.8243893448556,1075.76869237125,
322.236159443582));
#129234=CARTESIAN_POINT('Origin',(0.,1082.7251047501,424.620242579854));
#129235=CARTESIAN_POINT('Ctrl Pts',(-24.2635631860074,1076.2570261591,329.640295684007));
#129236=CARTESIAN_POINT('Ctrl Pts',(-25.1128615239931,1076.2570261591,329.857257311813));
#129237=CARTESIAN_POINT('Ctrl Pts',(-25.9591735823918,1076.2570261591,330.085590214949));
#129238=CARTESIAN_POINT('Ctrl Pts',(-26.8023471182513,1076.2570261591,330.325253318642));
#129239=CARTESIAN_POINT('Ctrl Pts',(-24.0482616346989,1076.31899119494,
330.483095636887));
#129240=CARTESIAN_POINT('Ctrl Pts',(-24.8900237650678,1076.31899119494,
330.698132066211));
#129241=CARTESIAN_POINT('Ctrl Pts',(-25.7288261144568,1076.31899119494,
330.924438868403));
#129242=CARTESIAN_POINT('Ctrl Pts',(-26.5645177908342,1076.31899119494,
331.161975333167));
#129243=CARTESIAN_POINT('Ctrl Pts',(-23.8342513036848,1076.37487987957,
331.320841095749));
#129244=CARTESIAN_POINT('Ctrl Pts',(-24.6685224230654,1076.37487987957,
331.533963872513));
#129245=CARTESIAN_POINT('Ctrl Pts',(-25.4998601011541,1076.37487987957,
331.758256724825));
#129246=CARTESIAN_POINT('Ctrl Pts',(-26.3281147887377,1076.37487987957,
331.993679304677));
#129247=CARTESIAN_POINT('Ctrl Pts',(-23.6215327638613,1076.42469575349,
332.153529825814));
#129248=CARTESIAN_POINT('Ctrl Pts',(-24.4483580888651,1076.42469575349,
332.364750501048));
#129249=CARTESIAN_POINT('Ctrl Pts',(-25.2722761532755,1076.42469575349,
332.587041559914));
#129250=CARTESIAN_POINT('Ctrl Pts',(-26.0931387425927,1076.42469575349,
332.820363014507));
#129251=CARTESIAN_POINT('Origin',(0.,1082.7251047501,424.620242579854));
#129252=CARTESIAN_POINT('Ctrl Pts',(-31.8715411090461,1076.62737351001,
339.317673442166));
#129253=CARTESIAN_POINT('Ctrl Pts',(-32.8252407714822,1076.62737351001,
339.67400360085));
#129254=CARTESIAN_POINT('Ctrl Pts',(-33.7728311362533,1076.62737351001,
340.046275985955));
#129255=CARTESIAN_POINT('Ctrl Pts',(-34.7140457315322,1076.62737351001,
340.434385910786));
#129256=CARTESIAN_POINT('Ctrl Pts',(-31.5180618270612,1076.66218303982,
340.263742877186));
#129257=CARTESIAN_POINT('Ctrl Pts',(-32.4611842453422,1076.66218303982,
340.616121067303));
#129258=CARTESIAN_POINT('Ctrl Pts',(-33.398265122649,1076.66218303982,340.9842646726));
#129259=CARTESIAN_POINT('Ctrl Pts',(-34.3290409425265,1076.66218303982,
341.368070167436));
#129260=CARTESIAN_POINT('Ctrl Pts',(-31.1672155499358,1076.68825449303,
341.20276520776));
#129261=CARTESIAN_POINT('Ctrl Pts',(-32.099839512089,1076.68825449303,341.551220866827));
#129262=CARTESIAN_POINT('Ctrl Pts',(-33.0264891852509,1076.68825449303,
341.915266446869));
#129263=CARTESIAN_POINT('Ctrl Pts',(-33.9469039863248,1076.68825449303,
342.294799574649));
#129264=CARTESIAN_POINT('Ctrl Pts',(-30.8190036731312,1076.7055939897,342.134736699005));
#129265=CARTESIAN_POINT('Ctrl Pts',(-31.7412080089404,1076.7055939897,342.479299280142));
#129266=CARTESIAN_POINT('Ctrl Pts',(-32.6575048027661,1076.7055939897,342.83927760578));
#129267=CARTESIAN_POINT('Ctrl Pts',(-33.5676363828443,1076.7055939897,343.214570446438));
#129268=CARTESIAN_POINT('Origin',(0.,1082.7251047501,424.620242579854));
#129269=CARTESIAN_POINT('Ctrl Pts',(20.0601507246982,1074.64981245085,313.322737267786));
#129270=CARTESIAN_POINT('Ctrl Pts',(19.3253404299007,1074.64981245085,313.190295797275));
#129271=CARTESIAN_POINT('Ctrl Pts',(18.5892545990681,1074.64981245085,313.065137648924));
#129272=CARTESIAN_POINT('Ctrl Pts',(17.8519654215009,1074.64981245085,312.947275097222));
#129273=CARTESIAN_POINT('Ctrl Pts',(19.9285675901508,1074.75367623909,314.052785352531));
#129274=CARTESIAN_POINT('Ctrl Pts',(19.1985772313156,1074.75367623909,313.921212622444));
#129275=CARTESIAN_POINT('Ctrl Pts',(18.4673197032334,1074.75367623909,313.796875440081));
#129276=CARTESIAN_POINT('Ctrl Pts',(17.734866721684,1074.75367623909,313.67978599942));
#129277=CARTESIAN_POINT('Ctrl Pts',(19.7975742137943,1074.85364519094,314.779561347436));
#129278=CARTESIAN_POINT('Ctrl Pts',(19.0723821878739,1074.85364519094,314.648853464061));
#129279=CARTESIAN_POINT('Ctrl Pts',(18.3459313219943,1074.85364519094,314.525333568101));
#129280=CARTESIAN_POINT('Ctrl Pts',(17.6182928605373,1074.85364519094,314.409013773381));
#129281=CARTESIAN_POINT('Ctrl Pts',(19.667170804569,1074.94972111449,315.50306409326));
#129282=CARTESIAN_POINT('Ctrl Pts',(18.9467555008622,1074.94972111449,315.373217161506));
#129283=CARTESIAN_POINT('Ctrl Pts',(18.2250896489708,1074.94972111449,315.25051087106));
#129284=CARTESIAN_POINT('Ctrl Pts',(17.5022440240014,1074.94972111449,315.134957255955));
#129285=CARTESIAN_POINT('Origin',(0.,1082.7251047501,424.620242579854));
#129286=CARTESIAN_POINT('Ctrl Pts',(7.18925503840259,1075.53658218756,318.877419242361));
#129287=CARTESIAN_POINT('Ctrl Pts',(6.43791533520909,1075.53658218756,318.826337073603));
#129288=CARTESIAN_POINT('Ctrl Pts',(5.68607388927085,1075.53658218756,318.783265299441));
#129289=CARTESIAN_POINT('Ctrl Pts',(4.93381610082962,1075.53658218756,318.748208812317));
#129290=CARTESIAN_POINT('Ctrl Pts',(7.13853586903372,1075.61823151961,319.623419785915));
#129291=CARTESIAN_POINT('Ctrl Pts',(6.39249676033246,1075.61823151961,319.572697994575));
#129292=CARTESIAN_POINT('Ctrl Pts',(5.64595944860998,1075.61823151961,319.529930085639));
#129293=CARTESIAN_POINT('Ctrl Pts',(4.89900873162153,1075.61823151961,319.495120917034));
#129294=CARTESIAN_POINT('Ctrl Pts',(7.08806003205873,1075.69568964953,320.365841286272));
#129295=CARTESIAN_POINT('Ctrl Pts',(6.34729608749738,1075.69568964953,320.315478143388));
#129296=CARTESIAN_POINT('Ctrl Pts',(5.60603746265602,1075.69568964953,320.273012641843));
#129297=CARTESIAN_POINT('Ctrl Pts',(4.86436835569387,1075.69568964953,320.23844960521));
#129298=CARTESIAN_POINT('Ctrl Pts',(7.03782761687019,1075.76895860023,321.104682428605));
#129299=CARTESIAN_POINT('Ctrl Pts',(6.30231339675412,1075.76895860023,321.054676204581));
#129300=CARTESIAN_POINT('Ctrl Pts',(5.56630800211068,1075.76895860023,321.012511652053));
#129301=CARTESIAN_POINT('Ctrl Pts',(4.82989503439467,1075.76895860023,320.978193560413));
#129302=CARTESIAN_POINT('Origin',(0.,1082.7251047501,424.620242579854));
#129303=CARTESIAN_POINT('Ctrl Pts',(-3.98735671405646,1076.25744174455,
326.677056081815));
#129304=CARTESIAN_POINT('Ctrl Pts',(-4.86288710452009,1076.25744174455,
326.712699724886));
#129305=CARTESIAN_POINT('Ctrl Pts',(-5.73786088507023,1076.25744174455,
326.760079227486));
#129306=CARTESIAN_POINT('Ctrl Pts',(-6.61212075197863,1076.25744174455,
326.819186071675));
#129307=CARTESIAN_POINT('Ctrl Pts',(-3.95209372041479,1076.31916993005,
327.543236413901));
#129308=CARTESIAN_POINT('Ctrl Pts',(-4.81988118121196,1076.31916993005,
327.578564835223));
#129309=CARTESIAN_POINT('Ctrl Pts',(-5.68711695458773,1076.31916993005,
327.625525327631));
#129310=CARTESIAN_POINT('Ctrl Pts',(-6.5536451279611,1076.31916993005,327.684109448517));
#129311=CARTESIAN_POINT('Ctrl Pts',(-3.91704149820492,1076.37486284266,
328.404239475144));
#129312=CARTESIAN_POINT('Ctrl Pts',(-4.77713230981848,1076.37486284266,
328.439254558837));
#129313=CARTESIAN_POINT('Ctrl Pts',(-5.63667632708034,1076.37486284266,
328.485798545532));
#129314=CARTESIAN_POINT('Ctrl Pts',(-6.49551902024172,1076.37486284266,
328.5438630675));
#129315=CARTESIAN_POINT('Ctrl Pts',(-3.88220014030112,1076.42452398704,
329.260062984234));
#129316=CARTESIAN_POINT('Ctrl Pts',(-4.73464060360691,1076.42452398704,
329.29476661525));
#129317=CARTESIAN_POINT('Ctrl Pts',(-5.5865391361954,1076.42452398704,329.340896601812));
#129318=CARTESIAN_POINT('Ctrl Pts',(-6.43774258283125,1076.42452398704,
329.398444650623));
#129319=CARTESIAN_POINT('Origin',(0.,1082.7251047501,424.620242579854));
#129320=CARTESIAN_POINT('Ctrl Pts',(-13.4363545933944,1076.62739445405,
334.555392974316));
#129321=CARTESIAN_POINT('Ctrl Pts',(-14.4438874283289,1076.62739445405,
334.705702095954));
#129322=CARTESIAN_POINT('Ctrl Pts',(-15.4487564642742,1076.62739445405,
334.872894996872));
#129323=CARTESIAN_POINT('Ctrl Pts',(-16.4506787909077,1076.62739445405,
335.056924605664));
#129324=CARTESIAN_POINT('Ctrl Pts',(-13.2875689926388,1076.6621457791,335.552713539383));
#129325=CARTESIAN_POINT('Ctrl Pts',(-14.2839450530862,1076.6621457791,335.701358233903));
#129326=CARTESIAN_POINT('Ctrl Pts',(-15.2776868117514,1076.6621457791,335.866699747524));
#129327=CARTESIAN_POINT('Ctrl Pts',(-16.2685144910799,1076.6621457791,336.04869153008));
#129328=CARTESIAN_POINT('Ctrl Pts',(-13.1398899312993,1076.68818647194,
336.542616891292));
#129329=CARTESIAN_POINT('Ctrl Pts',(-14.125192191759,1076.68818647194,336.68960953727));
#129330=CARTESIAN_POINT('Ctrl Pts',(-15.1078894282686,1076.68818647194,
336.853113432622));
#129331=CARTESIAN_POINT('Ctrl Pts',(-16.0877049727428,1076.68818647194,
337.033082544543));
#129332=CARTESIAN_POINT('Ctrl Pts',(-12.993317994907,1076.70552262381,337.525099105185));
#129333=CARTESIAN_POINT('Ctrl Pts',(-13.9676294737846,1076.70552262381,
337.670452087752));
#129334=CARTESIAN_POINT('Ctrl Pts',(-14.9393649870532,1076.70552262381,
337.832132141148));
#129335=CARTESIAN_POINT('Ctrl Pts',(-15.9082509527858,1076.70552262381,
338.010093746053));
#129336=CARTESIAN_POINT('Origin',(0.,1082.7251047501,424.620242579854));
#129337=CARTESIAN_POINT('Ctrl Pts',(42.762254864373,1074.64941228744,319.922676659465));
#129338=CARTESIAN_POINT('Ctrl Pts',(42.0709027679261,1074.64941228744,319.640303575722));
#129339=CARTESIAN_POINT('Ctrl Pts',(41.3767877733801,1074.64941228744,319.364791953408));
#129340=CARTESIAN_POINT('Ctrl Pts',(40.6799779767329,1074.64941228744,319.096168821529));
#129341=CARTESIAN_POINT('Ctrl Pts',(42.4815009844214,1074.75338301753,320.61006435562));
#129342=CARTESIAN_POINT('Ctrl Pts',(41.7946879326087,1074.75338301753,320.329545181104));
#129343=CARTESIAN_POINT('Ctrl Pts',(41.1051301223943,1074.75338301753,320.055842419366));
#129344=CARTESIAN_POINT('Ctrl Pts',(40.4128952026945,1074.75338301753,319.788982921953));
#129345=CARTESIAN_POINT('Ctrl Pts',(42.2020066081244,1074.85345163594,321.294368328354));
#129346=CARTESIAN_POINT('Ctrl Pts',(41.5197122381168,1074.85345163594,321.015694746152));
#129347=CARTESIAN_POINT('Ctrl Pts',(40.8346911680273,1074.85345163594,320.743792730171));
#129348=CARTESIAN_POINT('Ctrl Pts',(40.1470106016967,1074.85345163594,320.478688955298));
#129349=CARTESIAN_POINT('Ctrl Pts',(41.9237721821172,1074.94961995582,321.97558748414));
#129350=CARTESIAN_POINT('Ctrl Pts',(41.2459761238645,1074.94961995582,321.698751174391));
#129351=CARTESIAN_POINT('Ctrl Pts',(40.5654713424437,1074.94961995582,321.428641786473));
#129352=CARTESIAN_POINT('Ctrl Pts',(39.8823245986259,1074.94961995582,321.165285819407));
#129353=CARTESIAN_POINT('Origin',(0.,1082.7251047501,424.620242579854));
#129354=CARTESIAN_POINT('Ctrl Pts',(29.0176251705041,1075.53651526506,322.682332980308));
#129355=CARTESIAN_POINT('Ctrl Pts',(28.2930779591799,1075.53651526506,322.476083514538));
#129356=CARTESIAN_POINT('Ctrl Pts',(27.5663730602314,1075.53651526506,322.27757030739));
#129357=CARTESIAN_POINT('Ctrl Pts',(26.8375930740242,1075.53651526506,322.086815922718));
#129358=CARTESIAN_POINT('Ctrl Pts',(28.8127959863172,1075.61821260512,323.401890791752));
#129359=CARTESIAN_POINT('Ctrl Pts',(28.0933631981523,1075.61821260512,323.197097196667));
#129360=CARTESIAN_POINT('Ctrl Pts',(27.3717879530167,1075.61821260512,322.999985251615));
#129361=CARTESIAN_POINT('Ctrl Pts',(26.6481522682177,1075.61821260512,322.810577361177));
#129362=CARTESIAN_POINT('Ctrl Pts',(28.6089500466826,1075.69571404777,324.117994499226));
#129363=CARTESIAN_POINT('Ctrl Pts',(27.8946071308361,1075.69571404777,323.914649786188));
#129364=CARTESIAN_POINT('Ctrl Pts',(27.1781369155606,1075.69571404777,323.718932376733));
#129365=CARTESIAN_POINT('Ctrl Pts',(26.4596208379039,1075.69571404777,323.530864516934));
#129366=CARTESIAN_POINT('Ctrl Pts',(28.4060877130153,1075.7690216193,324.830642833093));
#129367=CARTESIAN_POINT('Ctrl Pts',(27.6968101096221,1075.7690216193,324.628740010895));
#129368=CARTESIAN_POINT('Ctrl Pts',(26.9854202912027,1075.7690216193,324.434410408066));
#129369=CARTESIAN_POINT('Ctrl Pts',(26.2719991173455,1075.7690216193,324.247676112933));
#129370=CARTESIAN_POINT('Origin',(0.,1082.7251047501,424.620242579854));
#129371=CARTESIAN_POINT('Ctrl Pts',(16.464705126852,1076.25721586291,327.98535171322));
#129372=CARTESIAN_POINT('Ctrl Pts',(15.6016647874419,1076.25721586291,327.838306432023));
#129373=CARTESIAN_POINT('Ctrl Pts',(14.7367321236006,1076.25721586291,327.702835294166));
#129374=CARTESIAN_POINT('Ctrl Pts',(13.8700623477992,1076.25721586291,327.578962609995));
#129375=CARTESIAN_POINT('Ctrl Pts',(16.3187044751784,1076.31912596814,328.842260897578));
#129376=CARTESIAN_POINT('Ctrl Pts',(15.4633171396334,1076.31912596814,328.69651953933));
#129377=CARTESIAN_POINT('Ctrl Pts',(14.6060542598303,1076.31912596814,328.562249690793));
#129378=CARTESIAN_POINT('Ctrl Pts',(13.7470696718946,1076.31912596814,328.439475446738));
#129379=CARTESIAN_POINT('Ctrl Pts',(16.1735788380354,1076.37496806519,329.694034433709));
#129380=CARTESIAN_POINT('Ctrl Pts',(15.3257986401933,1076.37496806519,329.54958918371));
#129381=CARTESIAN_POINT('Ctrl Pts',(14.4761595776988,1076.37496806519,329.416513424896));
#129382=CARTESIAN_POINT('Ctrl Pts',(13.6248141185805,1076.37496806519,329.29483103776));
#129383=CARTESIAN_POINT('Ctrl Pts',(16.0293286020337,1076.42474568726,330.540670052514));
#129384=CARTESIAN_POINT('Ctrl Pts',(15.189109655467,1076.42474568726,330.397513092609));
#129385=CARTESIAN_POINT('Ctrl Pts',(14.3470484232417,1076.42474568726,330.265624220743));
#129386=CARTESIAN_POINT('Ctrl Pts',(13.5032960135423,1076.42474568726,330.14502710442));
#129387=CARTESIAN_POINT('Origin',(0.,1082.7251047501,424.620242579854));
#129388=CARTESIAN_POINT('Ctrl Pts',(5.58142985825276,1076.62751743038,333.733442928555));
#129389=CARTESIAN_POINT('Ctrl Pts',(4.56395251573579,1076.62751743038,333.670958844602));
#129390=CARTESIAN_POINT('Ctrl Pts',(3.5455694495139,1076.62751743038,333.625567945566));
#129391=CARTESIAN_POINT('Ctrl Pts',(2.52656779749708,1076.62751743038,333.597283029625));
#129392=CARTESIAN_POINT('Ctrl Pts',(5.51963911911433,1076.66223932963,334.739629993698));
#129393=CARTESIAN_POINT('Ctrl Pts',(4.51342603658942,1076.66223932963,334.677837656812));
#129394=CARTESIAN_POINT('Ctrl Pts',(3.50631725742049,1076.66223932963,334.632949270084));
#129395=CARTESIAN_POINT('Ctrl Pts',(2.49859674067911,1076.66223932963,334.604977490007));
#129396=CARTESIAN_POINT('Ctrl Pts',(5.45830781737085,1076.68825505249,335.738335679423));
#129397=CARTESIAN_POINT('Ctrl Pts',(4.46327524082663,1076.68825505249,335.677229946204));
#129398=CARTESIAN_POINT('Ctrl Pts',(3.46735692014434,1076.68825505249,335.632840335416));
#129399=CARTESIAN_POINT('Ctrl Pts',(2.470833659193,1076.68825505249,335.605179362921));
#129400=CARTESIAN_POINT('Ctrl Pts',(5.39743619607369,1076.70557068555,336.729556027934));
#129401=CARTESIAN_POINT('Ctrl Pts',(4.41350032719132,1076.70557068555,336.669131752261));
#129402=CARTESIAN_POINT('Ctrl Pts',(3.42868859208241,1076.70557068555,336.625237179069));
#129403=CARTESIAN_POINT('Ctrl Pts',(2.44327866306178,1076.70557068555,336.59788468464));
#129404=CARTESIAN_POINT('Origin',(0.,1082.7251047501,424.620242579854));
#129405=CARTESIAN_POINT('Ctrl Pts',(63.5947113611256,1074.64992056935,331.105097475553));
#129406=CARTESIAN_POINT('Ctrl Pts',(62.9766859027927,1074.64992056935,330.684811001178));
#129407=CARTESIAN_POINT('Ctrl Pts',(62.3545245459131,1074.64992056935,330.270671611968));
#129408=CARTESIAN_POINT('Ctrl Pts',(61.7282884292425,1074.64992056935,329.862720004706));
#129409=CARTESIAN_POINT('Ctrl Pts',(63.1774566783766,1074.7538085787,331.718664726155));
#129410=CARTESIAN_POINT('Ctrl Pts',(62.5634861801343,1074.7538085787,331.301135815984));
#129411=CARTESIAN_POINT('Ctrl Pts',(61.9454069196119,1074.7538085787,330.889713659005));
#129412=CARTESIAN_POINT('Ctrl Pts',(61.3232796344242,1074.7538085787,330.484438684985));
#129413=CARTESIAN_POINT('Ctrl Pts',(62.7620726301513,1074.85379973269,332.329481234516));
#129414=CARTESIAN_POINT('Ctrl Pts',(62.1521389128188,1074.85379973269,331.914697525846));
#129415=CARTESIAN_POINT('Ctrl Pts',(61.5381234478156,1074.85379973269,331.505980419214));
#129416=CARTESIAN_POINT('Ctrl Pts',(60.920086573414,1074.85379973269,331.103370078565));
#129417=CARTESIAN_POINT('Ctrl Pts',(62.3485598793522,1074.94989584082,332.937546025845));
#129418=CARTESIAN_POINT('Ctrl Pts',(61.7426447573065,1074.94989584082,332.525495151596));
#129419=CARTESIAN_POINT('Ctrl Pts',(61.132674780499,1074.94989584082,332.119470909108));
#129420=CARTESIAN_POINT('Ctrl Pts',(60.5187098896588,1074.94989584082,331.719513197707));
#129421=CARTESIAN_POINT('Origin',(0.,1082.7251047501,424.620242579854));
#129422=CARTESIAN_POINT('Ctrl Pts',(49.5794614304066,1075.53619414421,330.940680740174));
#129423=CARTESIAN_POINT('Ctrl Pts',(48.9146671134995,1075.53619414421,330.588841517755));
#129424=CARTESIAN_POINT('Ctrl Pts',(48.2461653747274,1075.53619414421,330.244098501171));
#129425=CARTESIAN_POINT('Ctrl Pts',(47.5740319583019,1075.53619414421,329.906490751336));
#129426=CARTESIAN_POINT('Ctrl Pts',(49.2289544664351,1075.61802890567,331.602957777061));
#129427=CARTESIAN_POINT('Ctrl Pts',(48.568859979477,1075.61802890567,331.253605917234));
#129428=CARTESIAN_POINT('Ctrl Pts',(47.9050842806437,1075.61802890567,330.911300095904));
#129429=CARTESIAN_POINT('Ctrl Pts',(47.2377025786657,1075.61802890567,330.576079097841));
#129430=CARTESIAN_POINT('Ctrl Pts',(48.8801326275998,1075.6956547724,332.262050798233));
#129431=CARTESIAN_POINT('Ctrl Pts',(48.2247153753147,1075.6956547724,331.915174342554));
#129432=CARTESIAN_POINT('Ctrl Pts',(47.565642995135,1075.6956547724,331.575293999225));
#129433=CARTESIAN_POINT('Ctrl Pts',(46.9029901628844,1075.6956547724,331.242448278195));
#129434=CARTESIAN_POINT('Ctrl Pts',(48.5329965342673,1075.76907378011,332.917958631515));
#129435=CARTESIAN_POINT('Ctrl Pts',(47.8822339130609,1075.76907378011,332.573545617141));
#129436=CARTESIAN_POINT('Ctrl Pts',(47.227842121885,1075.76907378011,332.236079030245));
#129437=CARTESIAN_POINT('Ctrl Pts',(46.5698953062317,1075.76907378011,331.905597107288));
#129438=CARTESIAN_POINT('Origin',(0.,1082.7251047501,424.620242579854));
#129439=CARTESIAN_POINT('Ctrl Pts',(36.19552153342,1076.25694505369,333.515806627299));
#129440=CARTESIAN_POINT('Ctrl Pts',(35.3812836960972,1076.25694505369,333.192312355412));
#129441=CARTESIAN_POINT('Ctrl Pts',(34.5627824799597,1076.25694505369,332.879762265261));
#129442=CARTESIAN_POINT('Ctrl Pts',(33.7401649782897,1076.25694505369,332.578212525388));
#129443=CARTESIAN_POINT('Ctrl Pts',(35.874500582732,1076.31888525212,334.3238190941));
#129444=CARTESIAN_POINT('Ctrl Pts',(35.0674842853553,1076.31888525212,334.003193918563));
#129445=CARTESIAN_POINT('Ctrl Pts',(34.2562424214086,1076.31888525212,333.693415859946));
#129446=CARTESIAN_POINT('Ctrl Pts',(33.4409207795923,1076.31888525212,333.394540588628));
#129447=CARTESIAN_POINT('Ctrl Pts',(35.5554039327238,1076.37475500685,335.126988079703));
#129448=CARTESIAN_POINT('Ctrl Pts',(34.7555658871084,1076.37475500685,334.809214802248));
#129449=CARTESIAN_POINT('Ctrl Pts',(33.9515398605094,1076.37475500685,334.502192158735));
#129450=CARTESIAN_POINT('Ctrl Pts',(33.143470344865,1076.37475500685,334.205975324365));
#129451=CARTESIAN_POINT('Ctrl Pts',(35.2382324337861,1076.4245578532,335.925311443665));
#129452=CARTESIAN_POINT('Ctrl Pts',(34.4455293326173,1076.4245578532,335.610372858426));
#129453=CARTESIAN_POINT('Ctrl Pts',(33.6486756092925,1076.4245578532,335.306089006244));
#129454=CARTESIAN_POINT('Ctrl Pts',(32.8478144668115,1076.4245578532,335.01251457013));
#129455=CARTESIAN_POINT('Origin',(0.,1082.7251047501,424.620242579854));
#129456=CARTESIAN_POINT('Ctrl Pts',(24.3576856453425,1076.62752897425,336.880828280042));
#129457=CARTESIAN_POINT('Ctrl Pts',(23.3746783538014,1076.62752897426,336.607931739924));
#129458=CARTESIAN_POINT('Ctrl Pts',(22.3872241095125,1076.62752897426,336.351592175542));
#129459=CARTESIAN_POINT('Ctrl Pts',(21.3956017636078,1076.62752897425,336.111881975646));
#129460=CARTESIAN_POINT('Ctrl Pts',(24.0878033771608,1076.66227769843,337.852977789029));
#129461=CARTESIAN_POINT('Ctrl Pts',(23.1156877705418,1076.66227769843,337.583104932618));
#129462=CARTESIAN_POINT('Ctrl Pts',(22.1391744832491,1076.66227769843,337.329605601256));
#129463=CARTESIAN_POINT('Ctrl Pts',(21.1585392767545,1076.66227769843,337.092551381628));
#129464=CARTESIAN_POINT('Ctrl Pts',(23.8199294505212,1076.68830582022,338.817893001901));
#129465=CARTESIAN_POINT('Ctrl Pts',(22.8586244778407,1076.68830582022,338.551021328313));
#129466=CARTESIAN_POINT('Ctrl Pts',(21.8929707299003,1076.68830582022,338.300341094244));
#129467=CARTESIAN_POINT('Ctrl Pts',(20.9232409015031,1076.68830582022,338.065923090283));
#129468=CARTESIAN_POINT('Ctrl Pts',(23.5540649287557,1076.70561944135,339.775570088405));
#129469=CARTESIAN_POINT('Ctrl Pts',(22.603489496117,1076.70561944135,339.511677084842));
#129470=CARTESIAN_POINT('Ctrl Pts',(21.6486138267775,1076.70561944135,339.263794801149));
#129471=CARTESIAN_POINT('Ctrl Pts',(20.689707571876,1076.70561944135,339.031993237788));
#129472=CARTESIAN_POINT('Origin',(0.,1082.7251047501,424.620242579854));
#129473=CARTESIAN_POINT('Ctrl Pts',(81.6513798708841,1074.64930297342,346.367961510039));
#129474=CARTESIAN_POINT('Ctrl Pts',(81.1354496615202,1074.64930297342,345.829620481053));
#129475=CARTESIAN_POINT('Ctrl Pts',(80.6142207985842,1074.64930297342,345.296408031023));
#129476=CARTESIAN_POINT('Ctrl Pts',(80.0877442598867,1074.64930297342,344.768376309793));
#129477=CARTESIAN_POINT('Ctrl Pts',(81.1145207771131,1074.75342815374,346.882471476277));
#129478=CARTESIAN_POINT('Ctrl Pts',(80.6019828169075,1074.75342815374,346.347670047937));
#129479=CARTESIAN_POINT('Ctrl Pts',(80.0841810418596,1074.75342815374,345.817963478067));
#129480=CARTESIAN_POINT('Ctrl Pts',(79.5611660946002,1074.75342815374,345.293403573624));
#129481=CARTESIAN_POINT('Ctrl Pts',(80.580073619499,1074.85363982574,347.394669913838));
#129482=CARTESIAN_POINT('Ctrl Pts',(80.0709126681616,1074.85363982574,346.863392183851));
#129483=CARTESIAN_POINT('Ctrl Pts',(79.5565225841924,1074.85363982574,346.337175743343));
#129484=CARTESIAN_POINT('Ctrl Pts',(79.0369536765479,1074.85363982574,345.816072057925));
#129485=CARTESIAN_POINT('Ctrl Pts',(80.0480392545915,1074.9499398105,347.90455600183));
#129486=CARTESIAN_POINT('Ctrl Pts',(79.5422400664198,1074.9499398105,347.376786062256));
#129487=CARTESIAN_POINT('Ctrl Pts',(79.0312462712518,1074.9499398105,346.854043994718));
#129488=CARTESIAN_POINT('Ctrl Pts',(78.5151078458766,1074.9499398105,346.336380925024));
#129489=CARTESIAN_POINT('Origin',(0.,1082.7251047501,424.620242579854));
#129490=CARTESIAN_POINT('Ctrl Pts',(67.9699229048373,1075.5361780923,343.293100500072));
#129491=CARTESIAN_POINT('Ctrl Pts',(67.3926691025201,1075.5361780923,342.810655212599));
#129492=CARTESIAN_POINT('Ctrl Pts',(66.8103116710274,1075.5361780923,342.334382990357));
#129493=CARTESIAN_POINT('Ctrl Pts',(66.2229166210398,1075.5361780923,341.864337819182));
#129494=CARTESIAN_POINT('Ctrl Pts',(67.490436446628,1075.61783741877,343.866814014015));
#129495=CARTESIAN_POINT('Ctrl Pts',(66.9172548187275,1075.61783741877,343.387772084561));
#129496=CARTESIAN_POINT('Ctrl Pts',(66.3390055646507,1075.61783741877,342.914859673117));
#129497=CARTESIAN_POINT('Ctrl Pts',(65.755754229413,1075.61783741877,342.448130384685));
#129498=CARTESIAN_POINT('Ctrl Pts',(67.013250246792,1075.69530593322,344.437775230594));
#129499=CARTESIAN_POINT('Ctrl Pts',(66.4441212577132,1075.69530593322,343.962120332102));
#129500=CARTESIAN_POINT('Ctrl Pts',(65.8699604727387,1075.69530593322,343.492551613311));
#129501=CARTESIAN_POINT('Ctrl Pts',(65.2908329734526,1075.69530593322,343.029122300212));
#129502=CARTESIAN_POINT('Ctrl Pts',(66.538365150332,1075.76858565825,345.005983138752));
#129503=CARTESIAN_POINT('Ctrl Pts',(65.9732692573033,1075.76858565825,344.533698938167));
#129504=CARTESIAN_POINT('Ctrl Pts',(65.4031772258775,1075.76858565825,344.067457787961));
#129505=CARTESIAN_POINT('Ctrl Pts',(64.8281536764424,1075.76858565825,343.607312536943));
#129506=CARTESIAN_POINT('Origin',(0.,1082.7251047501,424.620242579854));
#129507=CARTESIAN_POINT('Ctrl Pts',(54.3457421654589,1076.25743101328,343.039995893921));
#129508=CARTESIAN_POINT('Ctrl Pts',(53.6154830488532,1076.25743101328,342.553524287408));
#129509=CARTESIAN_POINT('Ctrl Pts',(52.8787582301574,1076.25743101328,342.076901225811));
#129510=CARTESIAN_POINT('Ctrl Pts',(52.1357005219295,1076.25743101328,341.610212632023));
#129511=CARTESIAN_POINT('Ctrl Pts',(53.8641626587902,1076.31928350271,343.762911312637));
#129512=CARTESIAN_POINT('Ctrl Pts',(53.1403746622963,1076.31928350271,343.280750526934));
#129513=CARTESIAN_POINT('Ctrl Pts',(52.4101782589021,1076.31928350271,342.808351014224));
#129514=CARTESIAN_POINT('Ctrl Pts',(51.6737050842604,1076.31928350271,342.345797936003));
#129515=CARTESIAN_POINT('Ctrl Pts',(53.3854673762382,1076.37507652506,344.481497124182));
#129516=CARTESIAN_POINT('Ctrl Pts',(52.6681117437203,1076.37507652506,344.003621341385));
#129517=CARTESIAN_POINT('Ctrl Pts',(51.9444046563461,1076.37507652506,343.535420082339));
#129518=CARTESIAN_POINT('Ctrl Pts',(51.2144765799112,1076.37507652506,343.076977751702));
#129519=CARTESIAN_POINT('Ctrl Pts',(52.9096575912514,1076.42481360611,345.19575141694));
#129520=CARTESIAN_POINT('Ctrl Pts',(52.1986955494624,1076.42481360611,344.722134807747));
#129521=CARTESIAN_POINT('Ctrl Pts',(51.4814386615631,1076.42481360611,344.258106495972));
#129522=CARTESIAN_POINT('Ctrl Pts',(50.7580162305439,1076.42481360611,343.803750133997));
#129523=CARTESIAN_POINT('Origin',(0.,1082.7251047501,424.620242579854));
#129524=CARTESIAN_POINT('Ctrl Pts',(42.0705803179982,1076.6273260991,343.857378571533));
#129525=CARTESIAN_POINT('Ctrl Pts',(41.1680830520137,1076.6273260991,343.387254286299));
#129526=CARTESIAN_POINT('Ctrl Pts',(40.2578330776796,1076.6273260991,342.932322266211));
#129527=CARTESIAN_POINT('Ctrl Pts',(39.3400861126556,1076.6273260991,342.492710315889));
#129528=CARTESIAN_POINT('Ctrl Pts',(41.6034762298823,1076.66218189567,344.754077967193));
#129529=CARTESIAN_POINT('Ctrl Pts',(40.7109992716585,1076.66218189567,344.289173409709));
#129530=CARTESIAN_POINT('Ctrl Pts',(39.8108556823802,1076.66218189567,343.839292439662));
#129531=CARTESIAN_POINT('Ctrl Pts',(38.9032983405081,1076.66218189567,343.404561442672));
#129532=CARTESIAN_POINT('Ctrl Pts',(41.1398553241158,1076.68828036131,345.644090700101));
#129533=CARTESIAN_POINT('Ctrl Pts',(40.257323952493,1076.68828036131,345.184366947001));
#129534=CARTESIAN_POINT('Ctrl Pts',(39.367211385235,1076.68828036131,344.739499361452));
#129535=CARTESIAN_POINT('Ctrl Pts',(38.4697676827748,1076.68828036131,344.309612920659));
#129536=CARTESIAN_POINT('Ctrl Pts',(40.6797194487766,1076.70562763633,346.527413222502));
#129537=CARTESIAN_POINT('Ctrl Pts',(39.8070589029502,1076.70562763633,346.072831329768));
#129538=CARTESIAN_POINT('Ctrl Pts',(38.9269019546913,1076.70562763633,345.632939443192));
#129539=CARTESIAN_POINT('Ctrl Pts',(38.0394958675885,1076.70562763633,345.20786114215));
#129540=CARTESIAN_POINT('Origin',(0.,1082.7251047501,424.620242579854));
#129541=CARTESIAN_POINT('Ctrl Pts',(96.1331826317623,1074.64932100267,365.048861852279));
#129542=CARTESIAN_POINT('Ctrl Pts',(95.7405047741856,1074.64932100267,364.415178836427));
#129543=CARTESIAN_POINT('Ctrl Pts',(95.3415807234807,1074.64932100267,363.78540930225));
#129544=CARTESIAN_POINT('Ctrl Pts',(94.9364494785642,1074.64932100267,363.159614816175));
#129545=CARTESIAN_POINT('Ctrl Pts',(95.5028901751477,1074.75315166316,365.439438663269));
#129546=CARTESIAN_POINT('Ctrl Pts',(95.1127868905201,1074.75315166316,364.809910358766));
#129547=CARTESIAN_POINT('Ctrl Pts',(94.7164783656206,1074.75315166316,364.184269877387));
#129548=CARTESIAN_POINT('Ctrl Pts',(94.3140033436712,1074.75315166316,363.562578381905));
#129549=CARTESIAN_POINT('Ctrl Pts',(94.8754214251531,1074.8530908892,365.828265692369));
#129550=CARTESIAN_POINT('Ctrl Pts',(94.4878811794024,1074.8530908892,365.20287348613));
#129551=CARTESIAN_POINT('Ctrl Pts',(94.0941764627675,1074.8530908892,364.581343559416));
#129552=CARTESIAN_POINT('Ctrl Pts',(93.6943457639214,1074.8530908892,363.963736673152));
#129553=CARTESIAN_POINT('Ctrl Pts',(94.2507773817279,1074.94914048649,366.215342319933));
#129554=CARTESIAN_POINT('Ctrl Pts',(93.8657886366974,1074.94914048649,365.594067592284));
#129555=CARTESIAN_POINT('Ctrl Pts',(93.4746760066368,1074.94914048649,364.976629715552));
#129556=CARTESIAN_POINT('Ctrl Pts',(93.0774777268163,1074.94914048649,364.363089050622));
#129557=CARTESIAN_POINT('Origin',(0.,1082.7251047501,424.620242579854));
#129558=CARTESIAN_POINT('Ctrl Pts',(83.3922632669072,1075.53677429,359.209329248305));
#129559=CARTESIAN_POINT('Ctrl Pts',(82.9269536714695,1075.53677429,358.616106828574));
#129560=CARTESIAN_POINT('Ctrl Pts',(82.4553408499488,1075.53677429,358.027883056991));
#129561=CARTESIAN_POINT('Ctrl Pts',(81.9774784970065,1075.53677429,357.444724904756));
#129562=CARTESIAN_POINT('Ctrl Pts',(82.8039693524285,1075.61841261373,359.670773041121));
#129563=CARTESIAN_POINT('Ctrl Pts',(82.3419423013495,1075.61841261373,359.081735531666));
#129564=CARTESIAN_POINT('Ctrl Pts',(81.8736564905372,1075.61841261373,358.497661407204));
#129565=CARTESIAN_POINT('Ctrl Pts',(81.399165235862,1075.61841261373,357.918617166484));
#129566=CARTESIAN_POINT('Ctrl Pts',(82.2184977300363,1075.69586019218,360.130003094967));
#129567=CARTESIAN_POINT('Ctrl Pts',(81.7597374755771,1075.69586019218,359.545130419022));
#129568=CARTESIAN_POINT('Ctrl Pts',(81.2947627144106,1075.69586019218,358.965186034087));
#129569=CARTESIAN_POINT('Ctrl Pts',(80.8236263854336,1075.69586019218,358.390235968727));
#129570=CARTESIAN_POINT('Ctrl Pts',(81.6358494364943,1075.76911904789,360.587018596629));
#129571=CARTESIAN_POINT('Ctrl Pts',(81.180340225131,1075.76911904789,360.006290670053));
#129572=CARTESIAN_POINT('Ctrl Pts',(80.7186605466846,1075.76911904789,359.430456109738));
#129573=CARTESIAN_POINT('Ctrl Pts',(80.2508629648956,1075.76911904789,358.859580476334));
#129574=CARTESIAN_POINT('Origin',(0.,1082.7251047501,424.620242579854));
#129575=CARTESIAN_POINT('Ctrl Pts',(70.1247710735795,1076.25692701636,356.116956881602));
#129576=CARTESIAN_POINT('Ctrl Pts',(69.5128940250494,1076.25692701636,355.490596590764));
#129577=CARTESIAN_POINT('Ctrl Pts',(68.892680340111,1076.25692701636,354.872490029181));
#129578=CARTESIAN_POINT('Ctrl Pts',(68.2642413448404,1076.25692701636,354.262748144708));
#129579=CARTESIAN_POINT('Ctrl Pts',(69.5016741105325,1076.31898349264,356.725646059818));
#129580=CARTESIAN_POINT('Ctrl Pts',(68.8952339243959,1076.31898349264,356.104851322906));
#129581=CARTESIAN_POINT('Ctrl Pts',(68.2805311774272,1076.31898349264,355.492236976348));
#129582=CARTESIAN_POINT('Ctrl Pts',(67.6576762065094,1076.31898349264,354.887912982168));
#129583=CARTESIAN_POINT('Ctrl Pts',(68.8823191228473,1076.37494694374,357.33067978785));
#129584=CARTESIAN_POINT('Ctrl Pts',(68.2812831483188,1076.37494694374,356.715417181229));
#129585=CARTESIAN_POINT('Ctrl Pts',(67.6720582436777,1076.37494694374,356.108262066495));
#129586=CARTESIAN_POINT('Ctrl Pts',(67.0547537625543,1076.37494694374,355.509323425758));
#129587=CARTESIAN_POINT('Ctrl Pts',(68.2667077672577,1076.42482092472,357.932056447273));
#129588=CARTESIAN_POINT('Ctrl Pts',(67.6710433390963,1076.42482092472,357.32229253251));
#129589=CARTESIAN_POINT('Ctrl Pts',(67.0672631664877,1076.42482092472,356.720563651793));
#129590=CARTESIAN_POINT('Ctrl Pts',(66.455475625753,1076.42482092472,356.126977813244));
#129591=CARTESIAN_POINT('Origin',(0.,1082.7251047501,424.620242579854));
#129592=CARTESIAN_POINT('Ctrl Pts',(57.9363124048121,1076.6273289632,354.363979478503));
#129593=CARTESIAN_POINT('Ctrl Pts',(57.1513185877894,1076.6273289632,353.716640081114));
#129594=CARTESIAN_POINT('Ctrl Pts',(56.3555866550415,1076.6273289632,353.082546807706));
#129595=CARTESIAN_POINT('Ctrl Pts',(55.5493400979898,1076.6273289632,352.461877751429));
#129596=CARTESIAN_POINT('Ctrl Pts',(57.2950021496325,1076.6620786573,355.141662077677));
#129597=CARTESIAN_POINT('Ctrl Pts',(56.518697608199,1076.6620786573,354.501488227712));
#129598=CARTESIAN_POINT('Ctrl Pts',(55.7317738136923,1076.6620786573,353.87441387736));
#129599=CARTESIAN_POINT('Ctrl Pts',(54.9344517836562,1076.6620786573,353.26061514842));
#129600=CARTESIAN_POINT('Ctrl Pts',(56.658459637728,1076.68812401525,355.913563089931));
#129601=CARTESIAN_POINT('Ctrl Pts',(55.8907797725189,1076.68812401525,355.280501515997));
#129602=CARTESIAN_POINT('Ctrl Pts',(55.1125986332183,1076.68812401525,354.660393907371));
#129603=CARTESIAN_POINT('Ctrl Pts',(54.3241347818846,1076.68812401525,354.053414429152));
#129604=CARTESIAN_POINT('Ctrl Pts',(56.0266873910628,1076.70547112168,356.679679457015));
#129605=CARTESIAN_POINT('Ctrl Pts',(55.2675675685421,1076.70547112168,356.053676859542));
#129606=CARTESIAN_POINT('Ctrl Pts',(54.4980635667746,1076.70547112168,355.440483783707));
#129607=CARTESIAN_POINT('Ctrl Pts',(53.7183915107343,1076.70547112168,354.840272452576));
#129608=CARTESIAN_POINT('Origin',(0.,1082.7251047501,424.620242579854));
#129609=CARTESIAN_POINT('Ctrl Pts',(106.417077534095,1074.64979188503,386.345144051125));
#129610=CARTESIAN_POINT('Ctrl Pts',(106.164069922499,1074.64979188503,385.641701560972));
#129611=CARTESIAN_POINT('Ctrl Pts',(105.904100089906,1074.64979188503,384.940802228243));
#129612=CARTESIAN_POINT('Ctrl Pts',(105.637193594043,1074.64979188503,384.242514958602));
#129613=CARTESIAN_POINT('Ctrl Pts',(105.718538992071,1074.75373114609,386.596387856552));
#129614=CARTESIAN_POINT('Ctrl Pts',(105.467192162487,1074.75373114609,385.897562874254));
#129615=CARTESIAN_POINT('Ctrl Pts',(105.208928813027,1074.75373114609,385.201264355693));
#129616=CARTESIAN_POINT('Ctrl Pts',(104.943774333653,1074.75373114609,384.507560754223));
#129617=CARTESIAN_POINT('Ctrl Pts',(105.023133571111,1074.85376994682,386.846504770316));
#129618=CARTESIAN_POINT('Ctrl Pts',(104.773440074514,1074.85376994682,386.15227658519));
#129619=CARTESIAN_POINT('Ctrl Pts',(104.516875554181,1074.85376994682,385.460558244988));
#129620=CARTESIAN_POINT('Ctrl Pts',(104.25346523306,1074.85376994682,384.771417752785));
#129621=CARTESIAN_POINT('Ctrl Pts',(104.330862382022,1074.94991009922,387.095494392893));
#129622=CARTESIAN_POINT('Ctrl Pts',(104.082814766745,1074.94991009922,386.405842286912));
#129623=CARTESIAN_POINT('Ctrl Pts',(103.827941418819,1074.94991009922,385.718683481943));
#129624=CARTESIAN_POINT('Ctrl Pts',(103.566267394931,1074.94991009922,385.034085532814));
#129625=CARTESIAN_POINT('Origin',(0.,1082.7251047501,424.620242579854));
#129626=CARTESIAN_POINT('Ctrl Pts',(95.1741262372256,1075.53621972965,377.974563935349));
#129627=CARTESIAN_POINT('Ctrl Pts',(94.8428820819214,1075.53621972965,377.298705549998));
#129628=CARTESIAN_POINT('Ctrl Pts',(94.504457797769,1075.53621972965,376.626413759651));
#129629=CARTESIAN_POINT('Ctrl Pts',(94.1588917817534,1075.53621972965,375.957764841274));
#129630=CARTESIAN_POINT('Ctrl Pts',(94.5012690776854,1075.61805523595,378.304337163415));
#129631=CARTESIAN_POINT('Ctrl Pts',(94.1723667353325,1075.61805523595,377.633256927036));
#129632=CARTESIAN_POINT('Ctrl Pts',(93.8363350258384,1075.61805523595,376.96571807073));
#129633=CARTESIAN_POINT('Ctrl Pts',(93.4932120747309,1075.61805523595,376.301796332204));
#129634=CARTESIAN_POINT('Ctrl Pts',(93.8316468671878,1075.69568168088,378.632524914424));
#129635=CARTESIAN_POINT('Ctrl Pts',(93.5050750788652,1075.69568168088,377.966199854729));
#129636=CARTESIAN_POINT('Ctrl Pts',(93.1714244410573,1075.69568168088,377.303391081404));
#129637=CARTESIAN_POINT('Ctrl Pts',(92.8307328091399,1075.69568168088,376.64417379549));
#129638=CARTESIAN_POINT('Ctrl Pts',(93.1652607966795,1075.76910110026,378.959126604684));
#129639=CARTESIAN_POINT('Ctrl Pts',(92.8410082993214,1075.76910110026,378.297533740928));
#129640=CARTESIAN_POINT('Ctrl Pts',(92.5097272259928,1075.76910110026,377.639432191111));
#129641=CARTESIAN_POINT('Ctrl Pts',(92.1714551632232,1075.76910110026,376.984896622203));
#129642=CARTESIAN_POINT('Origin',(0.,1082.7251047501,424.620242579854));
#129643=CARTESIAN_POINT('Ctrl Pts',(82.8314235492149,1076.25695287626,372.188689355832));
#129644=CARTESIAN_POINT('Ctrl Pts',(82.3633219523744,1076.25695287626,371.449181955273));
#129645=CARTESIAN_POINT('Ctrl Pts',(81.8853595906112,1076.25695287626,370.716009205381));
#129646=CARTESIAN_POINT('Ctrl Pts',(81.3976221753205,1076.25695287626,369.989302583579));
#129647=CARTESIAN_POINT('Ctrl Pts',(82.0971191044224,1076.3188643633,372.653497528022));
#129648=CARTESIAN_POINT('Ctrl Pts',(81.6331672501365,1076.3188643633,371.920545895164));
#129649=CARTESIAN_POINT('Ctrl Pts',(81.1594420470705,1076.3188643633,371.193872756));
#129650=CARTESIAN_POINT('Ctrl Pts',(80.6760284467838,1076.3188643633,370.473608422396));
#129651=CARTESIAN_POINT('Ctrl Pts',(81.3672143100217,1076.3747109331,373.115520760707));
#129652=CARTESIAN_POINT('Ctrl Pts',(80.907387334739,1076.3747109331,372.389085616086));
#129653=CARTESIAN_POINT('Ctrl Pts',(80.437873903057,1076.3747109331,371.668873144652));
#129654=CARTESIAN_POINT('Ctrl Pts',(79.958758211252,1076.3747109331,370.955012499705));
#129655=CARTESIAN_POINT('Ctrl Pts',(80.6417111094299,1076.42449611617,373.574757823721));
#129656=CARTESIAN_POINT('Ctrl Pts',(80.185984138616,1076.42449611617,372.85479987052));
#129657=CARTESIAN_POINT('Ctrl Pts',(79.7206570797905,1076.42449611617,372.141009106621));
#129658=CARTESIAN_POINT('Ctrl Pts',(79.2458133785017,1076.42449611617,371.433513533737));
#129659=CARTESIAN_POINT('Origin',(0.,1082.7251047501,424.620242579854));
#129660=CARTESIAN_POINT('Ctrl Pts',(71.2784833618073,1076.62751692106,367.955057389048));
#129661=CARTESIAN_POINT('Ctrl Pts',(70.6436506951664,1076.62751692106,367.15650869439));
#129662=CARTESIAN_POINT('Ctrl Pts',(69.9954894423832,1076.62751692106,366.368739995617));
#129663=CARTESIAN_POINT('Ctrl Pts',(69.3341826242336,1076.62751692106,365.591973734349));
#129664=CARTESIAN_POINT('Ctrl Pts',(70.4885383781271,1076.66227574332,368.583050251404));
#129665=CARTESIAN_POINT('Ctrl Pts',(69.860741255129,1076.66227574332,367.793351486007));
#129666=CARTESIAN_POINT('Ctrl Pts',(69.2197632602675,1076.66227574332,367.01431324701));
#129667=CARTESIAN_POINT('Ctrl Pts',(68.5657853859875,1076.66227574332,366.246155510821));
#129668=CARTESIAN_POINT('Ctrl Pts',(69.7044731636426,1076.68830990593,369.206368796987));
#129669=CARTESIAN_POINT('Ctrl Pts',(69.0836592168774,1076.68830990594,368.425454088489));
#129670=CARTESIAN_POINT('Ctrl Pts',(68.4498110130512,1076.68830990594,367.65508132615));
#129671=CARTESIAN_POINT('Ctrl Pts',(67.8031075313755,1076.68830990593,366.895468039513));
#129672=CARTESIAN_POINT('Ctrl Pts',(68.9262908321672,1076.70562551488,369.825010550368));
#129673=CARTESIAN_POINT('Ctrl Pts',(68.3124076664922,1076.70562551488,369.052813991523));
#129674=CARTESIAN_POINT('Ctrl Pts',(67.6856357584999,1076.70562551488,368.29104168831));
#129675=CARTESIAN_POINT('Ctrl Pts',(67.0461520892739,1076.70562551488,367.539908741765));
#129676=CARTESIAN_POINT('Origin',(0.,1082.7251047501,424.620242579854));
#129677=CARTESIAN_POINT('Ctrl Pts',(112.050974474796,1074.64949814216,409.302566991023));
#129678=CARTESIAN_POINT('Ctrl Pts',(111.949995186494,1074.64949814216,408.563889141998));
#129679=CARTESIAN_POINT('Ctrl Pts',(111.841716652463,1074.64949814216,407.826245908196));
#129680=CARTESIAN_POINT('Ctrl Pts',(111.726149460023,1074.64949814216,407.08970941532));
#129681=CARTESIAN_POINT('Ctrl Pts',(111.314975450695,1074.75351345269,409.403180076609));
#129682=CARTESIAN_POINT('Ctrl Pts',(111.214659437818,1074.75351345269,408.669354181604));
#129683=CARTESIAN_POINT('Ctrl Pts',(111.107092123798,1074.75351345269,407.936556106024));
#129684=CARTESIAN_POINT('Ctrl Pts',(110.992284026415,1074.75351345269,407.204857501819));
#129685=CARTESIAN_POINT('Ctrl Pts',(110.582279720134,1074.85362314365,409.503341592907));
#129686=CARTESIAN_POINT('Ctrl Pts',(110.482624005784,1074.85362314365,408.774345875495));
#129687=CARTESIAN_POINT('Ctrl Pts',(110.375764719695,1074.85362314365,408.046371212211));
#129688=CARTESIAN_POINT('Ctrl Pts',(110.261712310416,1074.85362314365,407.319488783379));
#129689=CARTESIAN_POINT('Ctrl Pts',(109.852888455028,1074.94982903064,409.603051379713));
#129690=CARTESIAN_POINT('Ctrl Pts',(109.753890061251,1074.94982903064,408.878864055743));
#129691=CARTESIAN_POINT('Ctrl Pts',(109.64773560988,1074.94982903064,408.155691051114));
#129692=CARTESIAN_POINT('Ctrl Pts',(109.534435480544,1074.94982903064,407.433603076653));
#129693=CARTESIAN_POINT('Origin',(0.,1082.7251047501,424.620242579854));
#129694=CARTESIAN_POINT('Ctrl Pts',(102.791080266267,1075.53629018843,398.778596009474));
#129695=CARTESIAN_POINT('Ctrl Pts',(102.607642971954,1075.53629018843,398.048932069828));
#129696=CARTESIAN_POINT('Ctrl Pts',(102.416447074636,1075.53629018843,397.321262615603));
#129697=CARTESIAN_POINT('Ctrl Pts',(102.217514250128,1075.53629018843,396.59567014245));
#129698=CARTESIAN_POINT('Ctrl Pts',(102.065499511081,1075.61799617016,398.961006792445));
#129699=CARTESIAN_POINT('Ctrl Pts',(101.883357062296,1075.61799617016,398.23649339807));
#129700=CARTESIAN_POINT('Ctrl Pts',(101.693510776862,1075.61799617016,397.51396041046));
#129701=CARTESIAN_POINT('Ctrl Pts',(101.495982177591,1075.61799617016,396.793489742946));
#129702=CARTESIAN_POINT('Ctrl Pts',(101.343401779889,1075.69550615652,399.142541944234));
#129703=CARTESIAN_POINT('Ctrl Pts',(101.162547960951,1075.69550615652,398.423154370835));
#129704=CARTESIAN_POINT('Ctrl Pts',(100.974044808825,1075.69550615652,397.705733193127));
#129705=CARTESIAN_POINT('Ctrl Pts',(100.777913694053,1075.69550615652,396.990359744918));
#129706=CARTESIAN_POINT('Ctrl Pts',(100.624788352975,1075.76882217388,399.323201142979));
#129707=CARTESIAN_POINT('Ctrl Pts',(100.445216945919,1075.76882217388,398.608914657173));
#129708=CARTESIAN_POINT('Ctrl Pts',(100.258050446143,1075.76882217388,397.896580623591));
#129709=CARTESIAN_POINT('Ctrl Pts',(100.063310072652,1075.76882217388,397.186279799312));
#129710=CARTESIAN_POINT('Origin',(0.,1082.7251047501,424.620242579854));
#129711=CARTESIAN_POINT('Ctrl Pts',(91.9219760284135,1076.25713903639,390.562197315818));
#129712=CARTESIAN_POINT('Ctrl Pts',(91.6173444167836,1076.25713903639,389.740002751079));
#129713=CARTESIAN_POINT('Ctrl Pts',(91.301709724956,1076.25713903639,388.921969095044));
#129714=CARTESIAN_POINT('Ctrl Pts',(90.9751287655975,1076.25713903639,388.108243589682));
#129715=CARTESIAN_POINT('Ctrl Pts',(91.1063834873439,1076.31909062344,390.864382809221));
#129716=CARTESIAN_POINT('Ctrl Pts',(90.8044547687648,1076.31909062344,390.049483298214));
#129717=CARTESIAN_POINT('Ctrl Pts',(90.4916205965896,1076.31909062344,389.238707777579));
#129718=CARTESIAN_POINT('Ctrl Pts',(90.1679372794056,1076.31909062344,388.432202182856));
#129719=CARTESIAN_POINT('Ctrl Pts',(90.2956818280571,1076.37496705179,391.16475618021));
#129720=CARTESIAN_POINT('Ctrl Pts',(89.9964397940304,1076.37496705179,390.357107976526));
#129721=CARTESIAN_POINT('Ctrl Pts',(89.6863893475696,1076.37496705179,389.55354706627));
#129722=CARTESIAN_POINT('Ctrl Pts',(89.3655862962055,1076.37496705179,388.754218086388));
#129723=CARTESIAN_POINT('Ctrl Pts',(89.4898732127801,1076.42477186091,391.463316627657));
#129724=CARTESIAN_POINT('Ctrl Pts',(89.1933016476416,1076.42477186091,390.662875965546));
#129725=CARTESIAN_POINT('Ctrl Pts',(88.8860181255329,1076.42477186091,389.866486121406));
#129726=CARTESIAN_POINT('Ctrl Pts',(88.5680779559518,1076.42477186091,389.074290441427));
#129727=CARTESIAN_POINT('Origin',(0.,1082.7251047501,424.620242579854));
#129728=CARTESIAN_POINT('Ctrl Pts',(81.5058918905999,1076.62736807858,384.010616614734));
#129729=CARTESIAN_POINT('Ctrl Pts',(81.0512512124329,1076.62736807858,383.098126211705));
#129730=CARTESIAN_POINT('Ctrl Pts',(80.5813525416058,1076.62736807858,382.193398561516));
#129731=CARTESIAN_POINT('Ctrl Pts',(80.0963283776399,1076.62736807858,381.296688774443));
#129732=CARTESIAN_POINT('Ctrl Pts',(80.6014836943623,1076.66219575471,384.46123040126));
#129733=CARTESIAN_POINT('Ctrl Pts',(80.1518878141374,1076.66219575471,383.558865202438));
#129734=CARTESIAN_POINT('Ctrl Pts',(79.687203247462,1076.66219575471,382.664176619158));
#129735=CARTESIAN_POINT('Ctrl Pts',(79.2075610236123,1076.66219575471,381.777416930934));
#129736=CARTESIAN_POINT('Ctrl Pts',(79.7038156058466,1076.68827669796,384.908485985732));
#129737=CARTESIAN_POINT('Ctrl Pts',(79.2592269271757,1076.68827669796,384.01617053297));
#129738=CARTESIAN_POINT('Ctrl Pts',(78.7997176065083,1076.68827669796,383.13144620039));
#129739=CARTESIAN_POINT('Ctrl Pts',(78.3254172138324,1076.68827669796,382.254562457841));
#129740=CARTESIAN_POINT('Ctrl Pts',(78.8128911989983,1076.70561703749,385.352381587462));
#129741=CARTESIAN_POINT('Ctrl Pts',(78.3732721055577,1076.70561703749,384.470040382601));
#129742=CARTESIAN_POINT('Ctrl Pts',(77.9188991521501,1076.70561703749,383.595205444841));
#129743=CARTESIAN_POINT('Ctrl Pts',(77.449900460438,1076.70561703749,382.728123455474));
#129744=CARTESIAN_POINT('Origin',(0.,1082.7251047501,424.620242579854));
#129745=CARTESIAN_POINT('Ctrl Pts',(112.785775301718,1074.64965137923,432.937298637013));
#129746=CARTESIAN_POINT('Ctrl Pts',(112.840648198164,1074.64965137923,432.193179308468));
#129747=CARTESIAN_POINT('Ctrl Pts',(112.888154506911,1074.64965137923,431.448553388621));
#129748=CARTESIAN_POINT('Ctrl Pts',(112.928289575393,1074.64965137923,430.70349380298));
#129749=CARTESIAN_POINT('Ctrl Pts',(112.045457486278,1074.75359102585,432.882706071996));
#129750=CARTESIAN_POINT('Ctrl Pts',(112.099970200931,1074.75359102585,432.143471089853));
#129751=CARTESIAN_POINT('Ctrl Pts',(112.147164681643,1074.75359102585,431.403732841637));
#129752=CARTESIAN_POINT('Ctrl Pts',(112.187036306387,1074.75359102585,430.663563774178));
#129753=CARTESIAN_POINT('Ctrl Pts',(111.308460068527,1074.85363044618,432.828358359964));
#129754=CARTESIAN_POINT('Ctrl Pts',(111.362614216836,1074.85363044618,432.093985817452));
#129755=CARTESIAN_POINT('Ctrl Pts',(111.409498268092,1074.85363044618,431.359113319182));
#129756=CARTESIAN_POINT('Ctrl Pts',(111.44910763067,1074.85363044618,430.623812835454));
#129757=CARTESIAN_POINT('Ctrl Pts',(110.574784225631,1074.94977145207,432.774255587723));
#129758=CARTESIAN_POINT('Ctrl Pts',(110.628581423621,1074.94977145207,432.044723570305));
#129759=CARTESIAN_POINT('Ctrl Pts',(110.675156444497,1074.94977145207,431.314694892525));
#129760=CARTESIAN_POINT('Ctrl Pts',(110.714504726896,1074.94977145207,430.5842410503));
#129761=CARTESIAN_POINT('Origin',(0.,1082.7251047501,424.620242579854));
#129762=CARTESIAN_POINT('Ctrl Pts',(105.917360566518,1075.53631386031,420.713368851864));
#129763=CARTESIAN_POINT('Ctrl Pts',(105.889707479413,1075.53631386031,419.963679406639));
#129764=CARTESIAN_POINT('Ctrl Pts',(105.854096729417,1075.53631386031,419.214325797191));
#129765=CARTESIAN_POINT('Ctrl Pts',(105.810532330478,1075.53631386031,418.465392488643));
#129766=CARTESIAN_POINT('Ctrl Pts',(105.169355002635,1075.61805795958,420.740959827227));
#129767=CARTESIAN_POINT('Ctrl Pts',(105.141897206112,1075.61805795958,419.996564810349));
#129768=CARTESIAN_POINT('Ctrl Pts',(105.106537945003,1075.61805795958,419.252503257522));
#129769=CARTESIAN_POINT('Ctrl Pts',(105.063281204908,1075.61805795958,418.50885903736));
#129770=CARTESIAN_POINT('Ctrl Pts',(104.424941823346,1075.69560206441,420.76841829369));
#129771=CARTESIAN_POINT('Ctrl Pts',(104.397678379499,1075.69560206441,420.029292278045));
#129772=CARTESIAN_POINT('Ctrl Pts',(104.362569399472,1075.69560206441,419.290497366114));
#129773=CARTESIAN_POINT('Ctrl Pts',(104.319618840655,1075.69560206441,418.552116832871));
#129774=CARTESIAN_POINT('Ctrl Pts',(103.684122349764,1075.76894820407,420.795744202522));
#129775=CARTESIAN_POINT('Ctrl Pts',(103.657052320342,1075.76894820407,420.061861751644));
#129776=CARTESIAN_POINT('Ctrl Pts',(103.622192413148,1075.76894820407,419.328308055539));
#129777=CARTESIAN_POINT('Ctrl Pts',(103.579546557497,1075.76894820407,418.595165798406));
#129778=CARTESIAN_POINT('Origin',(0.,1082.7251047501,424.620242579854));
#129779=CARTESIAN_POINT('Ctrl Pts',(96.9947980060726,1076.25705988878,410.413654841029));
#129780=CARTESIAN_POINT('Ctrl Pts',(96.8679299958094,1076.25705988878,409.547469571552));
#129781=CARTESIAN_POINT('Ctrl Pts',(96.7294712182359,1076.25705988878,408.683061346232));
#129782=CARTESIAN_POINT('Ctrl Pts',(96.5794465158489,1076.25705988878,407.820585258586));
#129783=CARTESIAN_POINT('Ctrl Pts',(96.1340987741442,1076.31902403782,410.539719324965));
#129784=CARTESIAN_POINT('Ctrl Pts',(96.0083565479565,1076.31902403782,409.681220292394));
#129785=CARTESIAN_POINT('Ctrl Pts',(95.8711264070311,1076.31902403782,408.824482535088));
#129786=CARTESIAN_POINT('Ctrl Pts',(95.7224329734211,1076.31902403782,407.969659770316));
#129787=CARTESIAN_POINT('Ctrl Pts',(95.2785615044095,1076.37491157774,410.665027749089));
#129788=CARTESIAN_POINT('Ctrl Pts',(95.1539383105136,1076.37491157774,409.814168855945));
#129789=CARTESIAN_POINT('Ctrl Pts',(95.0179294376044,1076.37491157774,408.965055563747));
#129790=CARTESIAN_POINT('Ctrl Pts',(94.8705592886128,1076.37491157774,408.117840221769));
#129791=CARTESIAN_POINT('Ctrl Pts',(94.4281884792105,1076.42472604926,410.789579779111));
#129792=CARTESIAN_POINT('Ctrl Pts',(94.3046775628379,1076.42472604926,409.946314907535));
#129793=CARTESIAN_POINT('Ctrl Pts',(94.1698825860548,1076.42472604926,409.104780057198));
#129794=CARTESIAN_POINT('Ctrl Pts',(94.023827733993,1076.42472604926,408.265126217639));
#129795=CARTESIAN_POINT('Origin',(0.,1082.7251047501,424.620242579854));
#129796=CARTESIAN_POINT('Ctrl Pts',(88.1662889859269,1076.62740160071,401.841294443769));
#129797=CARTESIAN_POINT('Ctrl Pts',(87.9114355350873,1076.62740160071,400.854880020173));
#129798=CARTESIAN_POINT('Ctrl Pts',(87.6400653482025,1076.62740160071,399.872881080177));
#129799=CARTESIAN_POINT('Ctrl Pts',(87.3522548453362,1076.62740160071,398.895574162713));
#129800=CARTESIAN_POINT('Ctrl Pts',(87.1890270721594,1076.66218602849,402.093783220433));
#129801=CARTESIAN_POINT('Ctrl Pts',(86.9369984943407,1076.66218602849,401.118302513777));
#129802=CARTESIAN_POINT('Ctrl Pts',(86.6686362569933,1076.66218602849,400.147188348159));
#129803=CARTESIAN_POINT('Ctrl Pts',(86.384015933118,1076.66218602849,399.180714197272));
#129804=CARTESIAN_POINT('Ctrl Pts',(86.2190403734841,1076.6882426219,402.3443923473));
#129805=CARTESIAN_POINT('Ctrl Pts',(85.9698156389513,1076.6882426219,401.379763961652));
#129806=CARTESIAN_POINT('Ctrl Pts',(85.7044389584957,1076.6882426219,400.419453538836));
#129807=CARTESIAN_POINT('Ctrl Pts',(85.4229850643604,1076.6882426219,399.463731510118));
#129808=CARTESIAN_POINT('Ctrl Pts',(85.2563327434172,1076.70557749024,402.59312082876));
#129809=CARTESIAN_POINT('Ctrl Pts',(85.0098908112967,1076.70557749024,401.639263325079));
#129810=CARTESIAN_POINT('Ctrl Pts',(84.7474772832261,1076.70557749024,400.689675570564));
#129811=CARTESIAN_POINT('Ctrl Pts',(84.4691660570007,1076.70557749024,399.744624976895));
#129812=CARTESIAN_POINT('Origin',(0.,1082.7251047501,424.620242579854));
#129813=CARTESIAN_POINT('Ctrl Pts',(108.594221951652,1074.64934918539,456.20485338271));
#129814=CARTESIAN_POINT('Ctrl Pts',(108.80254055405,1074.64934918539,455.488612277612));
#129815=CARTESIAN_POINT('Ctrl Pts',(109.003763162472,1074.64934918539,454.770345319861));
#129816=CARTESIAN_POINT('Ctrl Pts',(109.197870082341,1074.64934918539,454.050122809524));
#129817=CARTESIAN_POINT('Ctrl Pts',(107.880497720998,1074.75343155823,455.997266812811));
#129818=CARTESIAN_POINT('Ctrl Pts',(108.087447171046,1074.75343155823,455.285733127892));
#129819=CARTESIAN_POINT('Ctrl Pts',(108.2873472648,1074.75343155823,454.572186905025));
#129820=CARTESIAN_POINT('Ctrl Pts',(108.480178437124,1074.75343155823,453.856697982239));
#129821=CARTESIAN_POINT('Ctrl Pts',(107.169978746795,1074.85360355319,455.7906124912));
#129822=CARTESIAN_POINT('Ctrl Pts',(107.375565193204,1074.85360355319,455.083765085957));
#129823=CARTESIAN_POINT('Ctrl Pts',(107.574148711557,1074.85360355319,454.374918397678));
#129824=CARTESIAN_POINT('Ctrl Pts',(107.765709865577,1074.85360355319,453.664141804425));
#129825=CARTESIAN_POINT('Ctrl Pts',(106.462666166869,1074.94986698918,455.584890748814));
#129826=CARTESIAN_POINT('Ctrl Pts',(106.666895760533,1074.94986698918,454.88270847524));
#129827=CARTESIAN_POINT('Ctrl Pts',(106.86416864486,1074.94986698918,454.178540113725));
#129828=CARTESIAN_POINT('Ctrl Pts',(107.05446551185,1074.94986698918,453.472454584442));
#129829=CARTESIAN_POINT('Origin',(0.,1082.7251047501,424.620242579854));
#129830=CARTESIAN_POINT('Ctrl Pts',(104.415190336176,1075.53624138483,442.823528975234));
#129831=CARTESIAN_POINT('Ctrl Pts',(104.544378431635,1075.53624138483,442.082497972176));
#129832=CARTESIAN_POINT('Ctrl Pts',(104.665670898072,1075.53624138483,441.34013374278));
#129833=CARTESIAN_POINT('Ctrl Pts',(104.779053990598,1075.53624138483,440.596520411922));
#129834=CARTESIAN_POINT('Ctrl Pts',(103.677939602859,1075.61797203207,442.694999915424));
#129835=CARTESIAN_POINT('Ctrl Pts',(103.806215532015,1075.61797203207,441.959201155383));
#129836=CARTESIAN_POINT('Ctrl Pts',(103.926651581301,1075.61797203207,441.222078582595));
#129837=CARTESIAN_POINT('Ctrl Pts',(104.039234102877,1075.61797203207,440.483715727953));
#129838=CARTESIAN_POINT('Ctrl Pts',(102.944228902186,1075.69550432148,442.567088009382));
#129839=CARTESIAN_POINT('Ctrl Pts',(103.071597044958,1075.69550432148,441.836496368867));
#129840=CARTESIAN_POINT('Ctrl Pts',(103.191180789323,1075.69550432148,441.104590283998));
#129841=CARTESIAN_POINT('Ctrl Pts',(103.302966584025,1075.69550432148,440.371452694533));
#129842=CARTESIAN_POINT('Ctrl Pts',(102.214059535762,1075.76884028115,442.439793484022));
#129843=CARTESIAN_POINT('Ctrl Pts',(102.34052427368,1075.76884028115,441.714383830307));
#129844=CARTESIAN_POINT('Ctrl Pts',(102.459259826867,1075.76884028115,440.987669055412));
#129845=CARTESIAN_POINT('Ctrl Pts',(102.570252740182,1075.76884028115,440.259731510815));
#129846=CARTESIAN_POINT('Origin',(0.,1082.7251047501,424.620242579854));
#129847=CARTESIAN_POINT('Ctrl Pts',(97.8272190274779,1076.2571674599,430.893766563347));
#129848=CARTESIAN_POINT('Ctrl Pts',(97.8832329311818,1076.2571674599,430.020304623829));
#129849=CARTESIAN_POINT('Ctrl Pts',(97.9275442980839,1076.2571674599,429.146170869785));
#129850=CARTESIAN_POINT('Ctrl Pts',(97.9601451806249,1076.2571674599,428.271522083327));
#129851=CARTESIAN_POINT('Ctrl Pts',(96.9595108057009,1076.31909709904,430.838121637588));
#129852=CARTESIAN_POINT('Ctrl Pts',(97.0150278770789,1076.31909709904,429.972407133946));
#129853=CARTESIAN_POINT('Ctrl Pts',(97.0589462108583,1076.31909709904,429.106026774641));
#129854=CARTESIAN_POINT('Ctrl Pts',(97.0912579299732,1076.31909709904,428.239135951158));
#129855=CARTESIAN_POINT('Ctrl Pts',(96.0970043114389,1076.37495551961,430.782810291406));
#129856=CARTESIAN_POINT('Ctrl Pts',(96.1520275288957,1076.37495551961,429.924796779398));
#129857=CARTESIAN_POINT('Ctrl Pts',(96.1955551857029,1076.37495551961,429.066123334868));
#129858=CARTESIAN_POINT('Ctrl Pts',(96.2275794748654,1076.37495551961,428.206943967011));
#129859=CARTESIAN_POINT('Ctrl Pts',(95.2397018435956,1076.42474625764,430.727832672226));
#129860=CARTESIAN_POINT('Ctrl Pts',(95.2942341868524,1076.42474625764,429.877473687084));
#129861=CARTESIAN_POINT('Ctrl Pts',(95.3373735238793,1076.42474625764,429.026460656824));
#129862=CARTESIAN_POINT('Ctrl Pts',(95.3691121173291,1076.42474625764,428.174946216689));
#129863=CARTESIAN_POINT('Origin',(0.,1082.7251047501,424.620242579854));
#129864=CARTESIAN_POINT('Ctrl Pts',(90.9765429512604,1076.62736694439,420.667172948711));
#129865=CARTESIAN_POINT('Ctrl Pts',(90.9324560734266,1076.62736694439,419.652550867876));
#129866=CARTESIAN_POINT('Ctrl Pts',(90.8714034843986,1076.62736694439,418.638808197823));
#129867=CARTESIAN_POINT('Ctrl Pts',(90.7934022680253,1076.62736694439,417.62622860591));
#129868=CARTESIAN_POINT('Ctrl Pts',(89.967409109738,1076.66218229773,420.711021354171));
#129869=CARTESIAN_POINT('Ctrl Pts',(89.9238112542274,1076.66218229773,419.707653707116));
#129870=CARTESIAN_POINT('Ctrl Pts',(89.8634358752988,1076.66218229773,418.705155716205));
#129871=CARTESIAN_POINT('Ctrl Pts',(89.7862998673032,1076.66218229773,417.70380790229));
#129872=CARTESIAN_POINT('Ctrl Pts',(88.9657931412671,1076.68825720191,420.754543096574));
#129873=CARTESIAN_POINT('Ctrl Pts',(88.9226806649477,1076.68825720191,419.762346039708));
#129874=CARTESIAN_POINT('Ctrl Pts',(88.8629774510202,1076.68825720191,418.771008957019));
#129875=CARTESIAN_POINT('Ctrl Pts',(88.7867002057489,1076.68825720191,417.780809246293));
#129876=CARTESIAN_POINT('Ctrl Pts',(87.9716990307714,1076.70559777949,420.797738002768));
#129877=CARTESIAN_POINT('Ctrl Pts',(87.9290682885802,1076.70559777949,419.816627648059));
#129878=CARTESIAN_POINT('Ctrl Pts',(87.8700321918811,1076.70559777949,418.836367658269));
#129879=CARTESIAN_POINT('Ctrl Pts',(87.7946072602644,1076.70559777949,417.85723233157));
#129880=CARTESIAN_POINT('Origin',(0.,1082.7251047501,424.620242579854));
#129881=CARTESIAN_POINT('Ctrl Pts',(99.6541986370725,1074.64931753844,478.093455448501));
#129882=CARTESIAN_POINT('Ctrl Pts',(100.007599436641,1074.64931753844,477.434847678565));
#129883=CARTESIAN_POINT('Ctrl Pts',(100.354454045054,1074.64931753844,476.77276898205));
#129884=CARTESIAN_POINT('Ctrl Pts',(100.694728376414,1074.64931753844,476.107284422369));
#129885=CARTESIAN_POINT('Ctrl Pts',(99.0004381414725,1074.75320910968,477.742655636507));
#129886=CARTESIAN_POINT('Ctrl Pts',(99.3515205291227,1074.75320910968,477.088368524887));
#129887=CARTESIAN_POINT('Ctrl Pts',(99.6960996705322,1074.75320910968,476.430633256974));
#129888=CARTESIAN_POINT('Ctrl Pts',(100.034141703419,1074.75320910968,475.769514469349));
#129889=CARTESIAN_POINT('Ctrl Pts',(98.3496082045902,1074.85320468589,477.393428326146));
#129890=CARTESIAN_POINT('Ctrl Pts',(98.6983825728772,1074.85320468589,476.74344250498));
#129891=CARTESIAN_POINT('Ctrl Pts',(99.0406964473337,1074.85320468589,476.090031195739));
#129892=CARTESIAN_POINT('Ctrl Pts',(99.3765161882889,1074.85320468589,475.433258610078));
#129893=CARTESIAN_POINT('Ctrl Pts',(97.7017098648222,1074.94930607596,477.04577407461));
#129894=CARTESIAN_POINT('Ctrl Pts',(98.048186609984,1074.94930607596,476.400070169174));
#129895=CARTESIAN_POINT('Ctrl Pts',(98.3882454211516,1074.94930607596,475.750963341771));
#129896=CARTESIAN_POINT('Ctrl Pts',(98.7218528802625,1074.94930607596,475.098517381053));
#129897=CARTESIAN_POINT('Origin',(0.,1082.7251047501,424.620242579854));
#129898=CARTESIAN_POINT('Ctrl Pts',(98.3451399293708,1075.53671645102,464.132302641614));
#129899=CARTESIAN_POINT('Ctrl Pts',(98.6258712392865,1075.53671645102,463.43356509381));
#129900=CARTESIAN_POINT('Ctrl Pts',(98.8991401434067,1075.53671645102,462.731875465044));
#129901=CARTESIAN_POINT('Ctrl Pts',(99.164915605103,1075.53671645102,462.027313450004));
#129902=CARTESIAN_POINT('Ctrl Pts',(97.6512806020871,1075.61836636429,463.853531251042));
#129903=CARTESIAN_POINT('Ctrl Pts',(97.9300312545144,1075.61836636429,463.159723540801));
#129904=CARTESIAN_POINT('Ctrl Pts',(98.2013721510267,1075.61836636429,462.46298457756));
#129905=CARTESIAN_POINT('Ctrl Pts',(98.4652724739699,1075.61836636429,461.763393493733));
#129906=CARTESIAN_POINT('Ctrl Pts',(96.9607503923561,1075.69582454512,463.576097397768));
#129907=CARTESIAN_POINT('Ctrl Pts',(97.237529890434,1075.69582454512,462.887195871867));
#129908=CARTESIAN_POINT('Ctrl Pts',(97.5069520298648,1075.69582454512,462.195383820996));
#129909=CARTESIAN_POINT('Ctrl Pts',(97.7689862109179,1075.69582454512,461.500739817996));
#129910=CARTESIAN_POINT('Ctrl Pts',(96.2735505232669,1075.76909301678,463.300001573192));
#129911=CARTESIAN_POINT('Ctrl Pts',(96.5483683736258,1075.76909301678,462.615982569719));
#129912=CARTESIAN_POINT('Ctrl Pts',(96.8158810098999,1075.76909301678,461.929073669338));
#129913=CARTESIAN_POINT('Ctrl Pts',(97.0760580492314,1075.76909301678,461.239352888012));
#129914=CARTESIAN_POINT('Origin',(0.,1082.7251047501,424.620242579854));
#129915=CARTESIAN_POINT('Ctrl Pts',(94.3881599803209,1076.25694104584,451.097030807224));
#129916=CARTESIAN_POINT('Ctrl Pts',(94.6244864530644,1076.25694104584,450.254541124361));
#129917=CARTESIAN_POINT('Ctrl Pts',(94.8495125801886,1076.25694104584,449.408963032425));
#129918=CARTESIAN_POINT('Ctrl Pts',(95.0631980271476,1076.25694104584,448.560448096076));
#129919=CARTESIAN_POINT('Ctrl Pts',(93.5497242556542,1076.31897768791,450.861841508811));
#129920=CARTESIAN_POINT('Ctrl Pts',(93.7839514761455,1076.31897768791,450.026835534158));
#129921=CARTESIAN_POINT('Ctrl Pts',(94.0069787302753,1076.31897768791,449.188768584302));
#129922=CARTESIAN_POINT('Ctrl Pts',(94.2187660417838,1076.31897768791,448.347790877577));
#129923=CARTESIAN_POINT('Ctrl Pts',(92.7163221816138,1076.37492501907,450.628064197893));
#129924=CARTESIAN_POINT('Ctrl Pts',(92.9484627529684,1076.37492501907,449.8004970021));
#129925=CARTESIAN_POINT('Ctrl Pts',(93.1695031345806,1076.37492501907,448.969896100271));
#129926=CARTESIAN_POINT('Ctrl Pts',(93.379403706325,1076.37492501907,448.136410372497));
#129927=CARTESIAN_POINT('Ctrl Pts',(91.8879559861347,1076.42478659114,450.395699499429));
#129928=CARTESIAN_POINT('Ctrl Pts',(92.1180225170464,1076.42478659114,449.575526133259));
#129929=CARTESIAN_POINT('Ctrl Pts',(92.3370880319291,1076.42478659114,448.752346165445));
#129930=CARTESIAN_POINT('Ctrl Pts',(92.5451132646399,1076.42478659114,447.926307145921));
#129931=CARTESIAN_POINT('Origin',(0.,1082.7251047501,424.620242579854));
#129932=CARTESIAN_POINT('Ctrl Pts',(89.8103648304035,1076.62734440709,439.672670140951));
#129933=CARTESIAN_POINT('Ctrl Pts',(89.9786348315319,1076.62734440709,438.668686555578));
#129934=CARTESIAN_POINT('Ctrl Pts',(90.1300475661144,1076.62734440709,437.662022750337));
#129935=CARTESIAN_POINT('Ctrl Pts',(90.2645604650628,1076.62734440709,436.652961744751));
#129936=CARTESIAN_POINT('Ctrl Pts',(88.8148916651083,1076.66213832489,439.505826506167));
#129937=CARTESIAN_POINT('Ctrl Pts',(88.9812965332872,1076.66213832489,438.512971243449));
#129938=CARTESIAN_POINT('Ctrl Pts',(89.1310309836935,1076.66213832489,437.51746546887));
#129939=CARTESIAN_POINT('Ctrl Pts',(89.2640529190817,1076.66213832489,436.519589064918));
#129940=CARTESIAN_POINT('Ctrl Pts',(87.8268292096143,1076.68820444296,439.340224923707));
#129941=CARTESIAN_POINT('Ctrl Pts',(87.9913828296571,1076.68820444296,438.358415139856));
#129942=CARTESIAN_POINT('Ctrl Pts',(88.1394514897216,1076.68820444296,437.37398433099));
#129943=CARTESIAN_POINT('Ctrl Pts',(88.2709935608928,1076.68820444296,436.387209265918));
#129944=CARTESIAN_POINT('Ctrl Pts',(86.8461813891991,1076.70554887055,439.175866051459));
#129945=CARTESIAN_POINT('Ctrl Pts',(87.0088976532735,1076.70554887055,438.205018858802));
#129946=CARTESIAN_POINT('Ctrl Pts',(87.1553130234483,1076.70554887055,437.231579906705));
#129947=CARTESIAN_POINT('Ctrl Pts',(87.2853863356247,1076.70554887055,436.255822873657));
#129948=CARTESIAN_POINT('Origin',(0.,1082.7251047501,424.620242579854));
#129949=CARTESIAN_POINT('Ctrl Pts',(86.3565913854363,1074.65013798949,497.637758039474));
#129950=CARTESIAN_POINT('Ctrl Pts',(86.8384286186397,1074.65013798949,497.067897221832));
#129951=CARTESIAN_POINT('Ctrl Pts',(87.3146017276091,1074.65013798949,496.493295062873));
#129952=CARTESIAN_POINT('Ctrl Pts',(87.7850640597002,1074.65013798949,495.914007858744));
#129953=CARTESIAN_POINT('Ctrl Pts',(85.7902738736794,1074.75396819847,497.158916795206));
#129954=CARTESIAN_POINT('Ctrl Pts',(86.2689512686052,1074.75396819847,496.592793065319));
#129955=CARTESIAN_POINT('Ctrl Pts',(86.7420016840325,1074.75396819847,496.021959087338));
#129956=CARTESIAN_POINT('Ctrl Pts',(87.2093787732602,1074.75396819847,495.446470788223));
#129957=CARTESIAN_POINT('Ctrl Pts',(85.2264940110564,1074.85390548088,496.68222122195));
#129958=CARTESIAN_POINT('Ctrl Pts',(85.7020257268305,1074.85390548088,496.119817834058));
#129959=CARTESIAN_POINT('Ctrl Pts',(86.1719674413972,1074.85390548088,495.552735151966));
#129960=CARTESIAN_POINT('Ctrl Pts',(86.6362731126277,1074.85390548088,494.981028735103));
#129961=CARTESIAN_POINT('Ctrl Pts',(84.6652526963884,1074.94995164347,496.207672079691));
#129962=CARTESIAN_POINT('Ctrl Pts',(85.1376528971515,1074.94995164347,495.648972282103));
#129963=CARTESIAN_POINT('Ctrl Pts',(85.6044999084952,1074.94995164347,495.08562400483));
#129964=CARTESIAN_POINT('Ctrl Pts',(86.0657479914915,1074.94995164347,494.517682441429));
#129965=CARTESIAN_POINT('Origin',(0.,1082.7251047501,424.620242579854));
#129966=CARTESIAN_POINT('Ctrl Pts',(87.9839219813682,1075.53617027389,483.720658031948));
#129967=CARTESIAN_POINT('Ctrl Pts',(88.4030068095904,1075.53617027389,483.096758410468));
#129968=CARTESIAN_POINT('Ctrl Pts',(88.8154320139319,1075.53617027389,482.468436612539));
#129969=CARTESIAN_POINT('Ctrl Pts',(89.2211509359701,1075.53617027389,481.835763721363));
#129970=CARTESIAN_POINT('Ctrl Pts',(87.3617260771309,1075.61803025466,483.302717621872));
#129971=CARTESIAN_POINT('Ctrl Pts',(87.7778472631583,1075.61803025466,482.683230031367));
#129972=CARTESIAN_POINT('Ctrl Pts',(88.1873559201675,1075.61803025466,482.05935153672));
#129973=CARTESIAN_POINT('Ctrl Pts',(88.5902057196901,1075.61803025466,481.431152718451));
#129974=CARTESIAN_POINT('Ctrl Pts',(86.7425223803861,1075.69567883021,482.886787132494));
#129975=CARTESIAN_POINT('Ctrl Pts',(87.155694176695,1075.69567883021,482.271690355031));
#129976=CARTESIAN_POINT('Ctrl Pts',(87.5623003123638,1075.69567883021,481.652233795337));
#129977=CARTESIAN_POINT('Ctrl Pts',(87.9622947872917,1075.69567883021,481.028487533674));
#129978=CARTESIAN_POINT('Ctrl Pts',(86.1263119930219,1075.76911803806,482.472867303973));
#129979=CARTESIAN_POINT('Ctrl Pts',(86.5365486573371,1075.76911803806,481.862140113802));
#129980=CARTESIAN_POINT('Ctrl Pts',(86.9402663028226,1075.76911803806,481.247084112867));
#129981=CARTESIAN_POINT('Ctrl Pts',(87.3374192561581,1075.76911803806,480.627768883586));
#129982=CARTESIAN_POINT('Origin',(0.,1082.7251047501,424.620242579854));
#129983=CARTESIAN_POINT('Ctrl Pts',(86.8205627762618,1076.25692673602,470.143580773689));
#129984=CARTESIAN_POINT('Ctrl Pts',(87.2279599308813,1076.25692673602,469.366606772202));
#129985=CARTESIAN_POINT('Ctrl Pts',(87.6248910727604,1076.25692673602,468.584234284709));
#129986=CARTESIAN_POINT('Ctrl Pts',(88.0112846810161,1076.25692673602,467.796604282691));
#129987=CARTESIAN_POINT('Ctrl Pts',(86.0509918531742,1076.31883222028,469.740065335922));
#129988=CARTESIAN_POINT('Ctrl Pts',(86.4547778701287,1076.31883222028,468.969978373408));
#129989=CARTESIAN_POINT('Ctrl Pts',(86.8481906442906,1076.31883222028,468.194540776661));
#129990=CARTESIAN_POINT('Ctrl Pts',(87.2311592887328,1076.31883222028,467.413892267602));
#129991=CARTESIAN_POINT('Ctrl Pts',(85.286031300467,1076.37467429721,469.338967291492));
#129992=CARTESIAN_POINT('Ctrl Pts',(85.6862278134767,1076.37467429721,468.575726108856));
#129993=CARTESIAN_POINT('Ctrl Pts',(86.0761432978725,1076.37467429721,467.807181857088));
#129994=CARTESIAN_POINT('Ctrl Pts',(86.4557074968852,1076.37467429721,467.033473016034));
#129995=CARTESIAN_POINT('Ctrl Pts',(84.5256831543828,1076.42445649601,468.94028770808));
#129996=CARTESIAN_POINT('Ctrl Pts',(84.9223118067231,1076.42445649601,468.183851028003));
#129997=CARTESIAN_POINT('Ctrl Pts',(85.3087510886134,1076.42445649601,467.422158557096));
#129998=CARTESIAN_POINT('Ctrl Pts',(85.6849313696428,1076.42445649601,466.655347540621));
#129999=CARTESIAN_POINT('Origin',(0.,1082.7251047501,424.620242579854));
#130000=CARTESIAN_POINT('Ctrl Pts',(84.7123651370726,1076.62758566352,458.012113964912));
#130001=CARTESIAN_POINT('Ctrl Pts',(85.0860848089413,1076.62758566352,457.064018635447));
#130002=CARTESIAN_POINT('Ctrl Pts',(85.4438367859815,1076.62758566352,456.109783512525));
#130003=CARTESIAN_POINT('Ctrl Pts',(85.7855202534696,1076.62758566352,455.149677500182));
#130004=CARTESIAN_POINT('Ctrl Pts',(83.7741341029246,1076.66231053226,457.642282595299));
#130005=CARTESIAN_POINT('Ctrl Pts',(84.1437146459465,1076.66231053226,456.704687887084));
#130006=CARTESIAN_POINT('Ctrl Pts',(84.4975043441996,1076.66231053226,455.761021386639));
#130007=CARTESIAN_POINT('Ctrl Pts',(84.8354034995328,1076.66231053226,454.811549019754));
#130008=CARTESIAN_POINT('Ctrl Pts',(82.8428821294764,1076.68832201484,457.275202227821));
#130009=CARTESIAN_POINT('Ctrl Pts',(83.2083543326901,1076.68832201484,456.348030031658));
#130010=CARTESIAN_POINT('Ctrl Pts',(83.55821122569,1076.68832201484,455.414853538662));
#130011=CARTESIAN_POINT('Ctrl Pts',(83.8923542185919,1076.68832201484,454.475935718534));
#130012=CARTESIAN_POINT('Ctrl Pts',(81.9186129103161,1076.70562620542,456.910874318414));
#130013=CARTESIAN_POINT('Ctrl Pts',(82.2800075790548,1076.70562620542,455.994046483766));
#130014=CARTESIAN_POINT('Ctrl Pts',(82.6259611559338,1076.70562620542,455.071281341587));
#130015=CARTESIAN_POINT('Ctrl Pts',(82.956376151026,1076.70562620542,454.142838927651));
#130016=CARTESIAN_POINT('Origin',(0.,1082.7251047501,424.620242579854));
#130017=CARTESIAN_POINT('Ctrl Pts',(69.2883894728621,1074.6493363685,514.003867860922));
#130018=CARTESIAN_POINT('Ctrl Pts',(69.8780536973393,1074.6493363685,513.546772007903));
#130019=CARTESIAN_POINT('Ctrl Pts',(70.4631660048975,1074.6493363685,513.083863697306));
#130020=CARTESIAN_POINT('Ctrl Pts',(71.0436691030515,1074.6493363685,512.615188255759));
#130021=CARTESIAN_POINT('Ctrl Pts',(68.8328608071636,1074.75345063343,513.416225344342));
#130022=CARTESIAN_POINT('Ctrl Pts',(69.4186483510103,1074.75345063343,512.962134616216));
#130023=CARTESIAN_POINT('Ctrl Pts',(69.9999139040001,1074.75345063343,512.502269643857));
#130024=CARTESIAN_POINT('Ctrl Pts',(70.5766005503106,1074.75345063343,512.036675455896));
#130025=CARTESIAN_POINT('Ctrl Pts',(68.3793784899775,1074.85365214779,512.831222664682));
#130026=CARTESIAN_POINT('Ctrl Pts',(68.9613067682112,1074.85365214779,512.380123561678));
#130027=CARTESIAN_POINT('Ctrl Pts',(69.5387428472146,1074.85365214779,511.92328825612));
#130028=CARTESIAN_POINT('Ctrl Pts',(70.1116301861363,1074.85365214779,511.460761479985));
#130029=CARTESIAN_POINT('Ctrl Pts',(67.9279432479523,1074.94994273216,512.248860759335));
#130030=CARTESIAN_POINT('Ctrl Pts',(68.5060296817743,1074.94994273216,511.800739776888));
#130031=CARTESIAN_POINT('Ctrl Pts',(69.0796535735096,1074.94994273216,511.346920461842));
#130032=CARTESIAN_POINT('Ctrl Pts',(69.648758755585,1074.94994273216,510.887447250856));
#130033=CARTESIAN_POINT('Origin',(0.,1082.7251047501,424.620242579854));
#130034=CARTESIAN_POINT('Ctrl Pts',(73.7732679240495,1075.53618795423,500.72214962966));
#130035=CARTESIAN_POINT('Ctrl Pts',(74.3145652537746,1075.53618795423,500.197415434678));
#130036=CARTESIAN_POINT('Ctrl Pts',(74.8502334981649,1075.53618795423,499.666936116983));
#130037=CARTESIAN_POINT('Ctrl Pts',(75.3802116840874,1075.53618795423,499.13077205907));
#130038=CARTESIAN_POINT('Ctrl Pts',(73.2529980727088,1075.6178224785,500.185457559732));
#130039=CARTESIAN_POINT('Ctrl Pts',(73.7904780212985,1075.6178224785,499.664423937997));
#130040=CARTESIAN_POINT('Ctrl Pts',(74.3223685824477,1075.6178224785,499.13768570977));
#130041=CARTESIAN_POINT('Ctrl Pts',(74.8486092130231,1075.6178224785,498.605302831716));
#130042=CARTESIAN_POINT('Ctrl Pts',(72.7352233846767,1075.69526870155,499.651339412466));
#130043=CARTESIAN_POINT('Ctrl Pts',(73.2689042599175,1075.69526870155,499.13398861639));
#130044=CARTESIAN_POINT('Ctrl Pts',(73.7970352552249,1075.69526870155,498.610973535734));
#130045=CARTESIAN_POINT('Ctrl Pts',(74.319556255403,1075.69526870155,498.082353703368));
#130046=CARTESIAN_POINT('Ctrl Pts',(72.2199447762796,1075.76852864419,499.119796133112));
#130047=CARTESIAN_POINT('Ctrl Pts',(72.7498448926814,1075.76852864419,498.606110408591));
#130048=CARTESIAN_POINT('Ctrl Pts',(73.2742344461996,1075.76852864419,498.086800527018));
#130049=CARTESIAN_POINT('Ctrl Pts',(73.7930537475129,1075.76852864419,497.561925599512));
#130050=CARTESIAN_POINT('Origin',(0.,1082.7251047501,424.620242579854));
#130051=CARTESIAN_POINT('Ctrl Pts',(75.4567986547188,1076.25738960263,487.191656892968));
#130052=CARTESIAN_POINT('Ctrl Pts',(76.0156278790124,1076.25738960263,486.51774749324));
#130053=CARTESIAN_POINT('Ctrl Pts',(76.5653794102637,1076.25738960263,485.836412601389));
#130054=CARTESIAN_POINT('Ctrl Pts',(77.1059545926398,1076.25738960263,485.147774486581));
#130055=CARTESIAN_POINT('Ctrl Pts',(74.7879755561225,1076.3192607262,486.637045407316));
#130056=CARTESIAN_POINT('Ctrl Pts',(75.3418515104651,1076.3192607262,485.969109308615));
#130057=CARTESIAN_POINT('Ctrl Pts',(75.8867302333128,1076.3192607262,485.293813534798));
#130058=CARTESIAN_POINT('Ctrl Pts',(76.4225139432842,1076.3192607262,484.61127927128));
#130059=CARTESIAN_POINT('Ctrl Pts',(74.1231591212705,1076.3750692605,486.085756387255));
#130060=CARTESIAN_POINT('Ctrl Pts',(74.6721114788105,1076.3750692605,485.423757805816));
#130061=CARTESIAN_POINT('Ctrl Pts',(75.2121465843888,1076.3750692605,484.754464971983));
#130062=CARTESIAN_POINT('Ctrl Pts',(75.7431675258367,1076.3750692605,484.077997993913));
#130063=CARTESIAN_POINT('Ctrl Pts',(73.4623511196488,1076.42481873403,485.537791300105));
#130064=CARTESIAN_POINT('Ctrl Pts',(74.0064095666395,1076.42481873403,484.881694436359));
#130065=CARTESIAN_POINT('Ctrl Pts',(74.5416302589744,1076.42481873403,484.218368348484));
#130066=CARTESIAN_POINT('Ctrl Pts',(75.0679171484566,1076.42481873403,483.54793207387));
#130067=CARTESIAN_POINT('Origin',(0.,1082.7251047501,424.620242579854));
#130068=CARTESIAN_POINT('Ctrl Pts',(75.9228204664487,1076.62732636353,474.902424976691));
#130069=CARTESIAN_POINT('Ctrl Pts',(76.4850486031252,1076.62732636353,474.053497109058));
#130070=CARTESIAN_POINT('Ctrl Pts',(77.032960627269,1076.62732636353,473.195259720037));
#130071=CARTESIAN_POINT('Ctrl Pts',(77.5664024258491,1076.62732636353,472.327954208904));
#130072=CARTESIAN_POINT('Ctrl Pts',(75.0798167841509,1076.66218387772,474.344120310794));
#130073=CARTESIAN_POINT('Ctrl Pts',(75.6358022603651,1076.66218387772,473.504618453865));
#130074=CARTESIAN_POINT('Ctrl Pts',(76.1776305819925,1076.66218387772,472.655910443163));
#130075=CARTESIAN_POINT('Ctrl Pts',(76.7051493471851,1076.66218387772,471.798234997602));
#130076=CARTESIAN_POINT('Ctrl Pts',(74.2430996751547,1076.68828317563,473.789979118058));
#130077=CARTESIAN_POINT('Ctrl Pts',(74.7928890446091,1076.68828317564,472.959832978775));
#130078=CARTESIAN_POINT('Ctrl Pts',(75.3286790320175,1076.68828317564,472.120583282485));
#130079=CARTESIAN_POINT('Ctrl Pts',(75.8503189339542,1076.68828317563,471.27246608773));
#130080=CARTESIAN_POINT('Ctrl Pts',(73.4126724751064,1076.7056303985,473.240003607618));
#130081=CARTESIAN_POINT('Ctrl Pts',(73.9563123162048,1076.7056303985,472.419142855625));
#130082=CARTESIAN_POINT('Ctrl Pts',(74.486109361764,1076.7056303985,471.589280372132));
#130083=CARTESIAN_POINT('Ctrl Pts',(75.001914594013,1076.7056303985,470.750649575311));
#130084=CARTESIAN_POINT('Origin',(0.,1082.7251047501,424.620242579854));
#130085=CARTESIAN_POINT('Ctrl Pts',(49.1901626715064,1074.64938719149,526.456185081641));
#130086=CARTESIAN_POINT('Ctrl Pts',(49.8633080434734,1074.64938719149,526.131033376505));
#130087=CARTESIAN_POINT('Ctrl Pts',(50.5331965078962,1074.64938719149,525.799223538816));
#130088=CARTESIAN_POINT('Ctrl Pts',(51.1997622106805,1074.64938719149,525.460788187493));
#130089=CARTESIAN_POINT('Ctrl Pts',(48.8673986854593,1074.75329680596,525.787982885518));
#130090=CARTESIAN_POINT('Ctrl Pts',(49.536127176659,1074.75329680596,525.464964681365));
#130091=CARTESIAN_POINT('Ctrl Pts',(50.2016201306943,1074.75329680596,525.135332032367));
#130092=CARTESIAN_POINT('Ctrl Pts',(50.8638121255763,1074.75329680596,524.799117343409));
#130093=CARTESIAN_POINT('Ctrl Pts',(48.5460818056865,1074.85330894177,525.122776561402));
#130094=CARTESIAN_POINT('Ctrl Pts',(49.2104132191208,1074.85330894177,524.80188229272));
#130095=CARTESIAN_POINT('Ctrl Pts',(49.871530369957,1074.85330894177,524.474417071027));
#130096=CARTESIAN_POINT('Ctrl Pts',(50.529368266374,1074.85330894177,524.140413088137));
#130097=CARTESIAN_POINT('Ctrl Pts',(48.2262125450444,1074.94942540884,524.460567171033));
#130098=CARTESIAN_POINT('Ctrl Pts',(48.8861666907337,1074.94942540884,524.141787268921));
#130099=CARTESIAN_POINT('Ctrl Pts',(49.5429277525433,1074.94942540884,523.816479709689));
#130100=CARTESIAN_POINT('Ctrl Pts',(50.1964311668822,1074.94942540884,523.484676473041));
#130101=CARTESIAN_POINT('Origin',(0.,1082.7251047501,424.620242579854));
#130102=CARTESIAN_POINT('Ctrl Pts',(56.3423819173354,1075.53657255571,514.390977079417));
#130103=CARTESIAN_POINT('Ctrl Pts',(56.9789503748771,1075.53657255571,513.991450626266));
#130104=CARTESIAN_POINT('Ctrl Pts',(57.6112333937505,1075.53657255571,513.585176123069));
#130105=CARTESIAN_POINT('Ctrl Pts',(58.2391594429655,1075.53657255571,513.172199532181));
#130106=CARTESIAN_POINT('Ctrl Pts',(55.9446376610293,1075.61827500173,513.75724820931));
#130107=CARTESIAN_POINT('Ctrl Pts',(56.5767123176503,1075.61827500173,513.360542179198));
#130108=CARTESIAN_POINT('Ctrl Pts',(57.2045317882931,1075.61827500173,512.957135736324));
#130109=CARTESIAN_POINT('Ctrl Pts',(57.8280250469345,1075.61827500173,512.547074518578));
#130110=CARTESIAN_POINT('Ctrl Pts',(55.5488028719652,1075.6957808248,513.126561707506));
#130111=CARTESIAN_POINT('Ctrl Pts',(56.1764053012408,1075.6957808248,512.73266256031));
#130112=CARTESIAN_POINT('Ctrl Pts',(56.7997826519929,1075.6957808248,512.332110408945));
#130113=CARTESIAN_POINT('Ctrl Pts',(57.418864400741,1075.6957808248,511.92495056839));
#130114=CARTESIAN_POINT('Ctrl Pts',(55.154878252074,1075.76909205172,512.498918692396));
#130115=CARTESIAN_POINT('Ctrl Pts',(55.77803003551,1075.76909205172,512.107812883019));
#130116=CARTESIAN_POINT('Ctrl Pts',(56.3969867025886,1075.76909205172,511.710101249285));
#130117=CARTESIAN_POINT('Ctrl Pts',(57.0116782299466,1075.76909205172,511.305828784823));
#130118=CARTESIAN_POINT('Origin',(0.,1082.7251047501,424.620242579854));
#130119=CARTESIAN_POINT('Ctrl Pts',(60.797722754504,1076.25695168791,501.521170266194));
#130120=CARTESIAN_POINT('Ctrl Pts',(61.4850557949331,1076.25695168791,500.977766111143));
#130121=CARTESIAN_POINT('Ctrl Pts',(62.1650421640159,1076.25695168791,500.42519636708));
#130122=CARTESIAN_POINT('Ctrl Pts',(62.8375596476042,1076.25695168791,499.863560347527));
#130123=CARTESIAN_POINT('Ctrl Pts',(60.2576093626057,1076.31899406394,500.83799959777));
#130124=CARTESIAN_POINT('Ctrl Pts',(60.9388362897955,1076.31899406394,500.299422923883));
#130125=CARTESIAN_POINT('Ctrl Pts',(61.6127818118266,1076.31899406394,499.751762086029));
#130126=CARTESIAN_POINT('Ctrl Pts',(62.2793248002741,1076.31899406394,499.195115515452));
#130127=CARTESIAN_POINT('Ctrl Pts',(59.7207389454293,1076.37494586681,500.158930855427));
#130128=CARTESIAN_POINT('Ctrl Pts',(60.3958964219976,1076.37494586681,499.625152677309));
#130129=CARTESIAN_POINT('Ctrl Pts',(61.0638373677205,1076.37494586681,499.082371271375));
#130130=CARTESIAN_POINT('Ctrl Pts',(61.7244417333773,1076.37494586681,498.530684191884));
#130131=CARTESIAN_POINT('Ctrl Pts',(59.1871129384905,1076.42481064945,499.483965854899));
#130132=CARTESIAN_POINT('Ctrl Pts',(59.8562376432841,1076.42481064945,498.954957174325));
#130133=CARTESIAN_POINT('Ctrl Pts',(60.5182102994977,1076.42481064945,498.417025712973));
#130134=CARTESIAN_POINT('Ctrl Pts',(61.1729119305929,1076.42481064945,497.870268153419));
#130135=CARTESIAN_POINT('Origin',(0.,1082.7251047501,424.620242579854));
#130136=CARTESIAN_POINT('Ctrl Pts',(63.8090632272348,1076.62733705021,489.588846730312));
#130137=CARTESIAN_POINT('Ctrl Pts',(64.5369215796459,1076.62733705021,488.873978984009));
#130138=CARTESIAN_POINT('Ctrl Pts',(65.2526650562726,1076.62733705021,488.146981768371));
#130139=CARTESIAN_POINT('Ctrl Pts',(65.9560915528467,1076.62733705021,487.408060365382));
#130140=CARTESIAN_POINT('Ctrl Pts',(63.1023554131808,1076.66210456745,488.869296592774));
#130141=CARTESIAN_POINT('Ctrl Pts',(63.8221524783835,1076.66210456745,488.162346258149));
#130142=CARTESIAN_POINT('Ctrl Pts',(64.5299688443114,1076.66210456745,487.443400792327));
#130143=CARTESIAN_POINT('Ctrl Pts',(65.225604645072,1076.66210456745,486.712663203721));
#130144=CARTESIAN_POINT('Ctrl Pts',(62.4009044379396,1076.68815814051,488.15509882154));
#130145=CARTESIAN_POINT('Ctrl Pts',(63.112700179736,1076.68815814051,487.456007005007));
#130146=CARTESIAN_POINT('Ctrl Pts',(63.8126484006965,1076.68815814051,486.745053396143));
#130147=CARTESIAN_POINT('Ctrl Pts',(64.5005514566546,1076.68815814051,486.022438746702));
#130148=CARTESIAN_POINT('Ctrl Pts',(61.7047130837235,1076.7055038641,487.446256249381));
#130149=CARTESIAN_POINT('Ctrl Pts',(62.4085674976518,1076.7055038641,486.754964026185));
#130150=CARTESIAN_POINT('Ctrl Pts',(63.1007065705844,1076.7055038641,486.051942349721));
#130151=CARTESIAN_POINT('Ctrl Pts',(63.7809348634214,1076.7055038641,485.337389732007));
#130152=CARTESIAN_POINT('Origin',(0.,1082.7251047501,424.620242579854));
#130153=CARTESIAN_POINT('Ctrl Pts',(26.9469667224666,1074.64963445669,534.45508610748));
#130154=CARTESIAN_POINT('Ctrl Pts',(27.6711831580577,1074.64963445669,534.277406278721));
#130155=CARTESIAN_POINT('Ctrl Pts',(28.3936068826267,1074.64963445669,534.092572490392));
#130156=CARTESIAN_POINT('Ctrl Pts',(29.1141672297197,1074.64963445669,533.90060282267));
#130157=CARTESIAN_POINT('Ctrl Pts',(26.7700334311186,1074.75360709312,533.73391253087));
#130158=CARTESIAN_POINT('Ctrl Pts',(27.4894946748206,1074.75360709312,533.557399344622));
#130159=CARTESIAN_POINT('Ctrl Pts',(28.2071749784082,1074.75360709312,533.373779171571));
#130160=CARTESIAN_POINT('Ctrl Pts',(28.9230041394223,1074.75360709312,533.183069973182));
#130161=CARTESIAN_POINT('Ctrl Pts',(26.5938939510957,1074.85367705875,533.015974499974));
#130162=CARTESIAN_POINT('Ctrl Pts',(27.3086213370798,1074.85367705875,532.840622722093));
#130163=CARTESIAN_POINT('Ctrl Pts',(28.0215795010474,1074.85367705875,532.658210719436));
#130164=CARTESIAN_POINT('Ctrl Pts',(28.7326987024519,1074.85367705875,532.468756335282));
#130165=CARTESIAN_POINT('Ctrl Pts',(26.4185485639129,1074.94984616712,532.301273162236));
#130166=CARTESIAN_POINT('Ctrl Pts',(27.1285634339167,1074.94984616712,532.127077556726));
#130167=CARTESIAN_POINT('Ctrl Pts',(27.8368207471725,1074.94984616712,531.945868277644));
#130168=CARTESIAN_POINT('Ctrl Pts',(28.5432512229646,1074.94984616712,531.757663050624));
#130169=CARTESIAN_POINT('Origin',(0.,1082.7251047501,424.620242579854));
#130170=CARTESIAN_POINT('Ctrl Pts',(36.4415553305205,1075.53628600585,524.14821876446));
#130171=CARTESIAN_POINT('Ctrl Pts',(37.1487244658279,1075.53628600585,523.889293142135));
#130172=CARTESIAN_POINT('Ctrl Pts',(37.853093954926,1075.53628600585,523.622845611362));
#130173=CARTESIAN_POINT('Ctrl Pts',(38.5545837925167,1075.53628600585,523.348906436389));
#130174=CARTESIAN_POINT('Ctrl Pts',(36.1840447135347,1075.61808022474,523.44491424515));
#130175=CARTESIAN_POINT('Ctrl Pts',(36.8862167086625,1075.61808022474,523.187818294917));
#130176=CARTESIAN_POINT('Ctrl Pts',(37.5856088410019,1075.61808022474,522.92325358905));
#130177=CARTESIAN_POINT('Ctrl Pts',(38.2821416706041,1075.61808022474,522.651250177942));
#130178=CARTESIAN_POINT('Ctrl Pts',(35.9277715639648,1075.69566939527,522.744989456106));
#130179=CARTESIAN_POINT('Ctrl Pts',(36.6249704326731,1075.69566939527,522.489714385474));
#130180=CARTESIAN_POINT('Ctrl Pts',(37.3194091269444,1075.69566939527,522.227023456599));
#130181=CARTESIAN_POINT('Ctrl Pts',(38.0110087694628,1075.69566939527,521.95694650704));
#130182=CARTESIAN_POINT('Ctrl Pts',(35.6727363371673,1075.76905555037,522.048445640983));
#130183=CARTESIAN_POINT('Ctrl Pts',(36.3649861020524,1075.76905555037,521.794982654226));
#130184=CARTESIAN_POINT('Ctrl Pts',(37.0544952857479,1075.76905555037,521.534156451097));
#130185=CARTESIAN_POINT('Ctrl Pts',(37.7411855708526,1075.76905555037,521.265996657351));
#130186=CARTESIAN_POINT('Origin',(0.,1082.7251047501,424.620242579854));
#130187=CARTESIAN_POINT('Ctrl Pts',(43.4804114603392,1076.25699166103,512.48069772089));
#130188=CARTESIAN_POINT('Ctrl Pts',(44.2664168702271,1076.25699166103,512.09171910045));
#130189=CARTESIAN_POINT('Ctrl Pts',(45.0471320873662,1076.25699166103,511.692228648424));
#130190=CARTESIAN_POINT('Ctrl Pts',(45.8224165371904,1076.25699166103,511.282298296544));
#130191=CARTESIAN_POINT('Ctrl Pts',(43.0948065119335,1076.31892436805,511.701509458091));
#130192=CARTESIAN_POINT('Ctrl Pts',(43.8738412523786,1076.31892436805,511.315980484879));
#130193=CARTESIAN_POINT('Ctrl Pts',(44.6476327160179,1076.31892436805,510.920032903999));
#130194=CARTESIAN_POINT('Ctrl Pts',(45.4160415749672,1076.31892436805,510.513738009255));
#130195=CARTESIAN_POINT('Ctrl Pts',(42.7115128423091,1076.37478750376,510.926991574409));
#130196=CARTESIAN_POINT('Ctrl Pts',(43.4836186948302,1076.37478750376,510.544891571573));
#130197=CARTESIAN_POINT('Ctrl Pts',(44.2505279052787,1076.37478750376,510.152465626211));
#130198=CARTESIAN_POINT('Ctrl Pts',(45.01210238498,1076.37478750376,509.749784398027));
#130199=CARTESIAN_POINT('Ctrl Pts',(42.3305314727975,1076.42458460272,510.15714613364));
#130200=CARTESIAN_POINT('Ctrl Pts',(43.0957502373761,1076.42458460272,509.778454415191));
#130201=CARTESIAN_POINT('Ctrl Pts',(43.8558187132815,1076.42458460272,509.389528860335));
#130202=CARTESIAN_POINT('Ctrl Pts',(44.6106000435729,1076.42458460272,508.990439498502));
#130203=CARTESIAN_POINT('Origin',(0.,1082.7251047501,424.620242579854));
#130204=CARTESIAN_POINT('Ctrl Pts',(48.9116093958664,1076.62746842925,501.428290573206));
#130205=CARTESIAN_POINT('Ctrl Pts',(49.7696403684266,1076.62746842925,500.881893719285));
#130206=CARTESIAN_POINT('Ctrl Pts',(50.6183959633884,1076.62746842925,500.321197177589));
#130207=CARTESIAN_POINT('Ctrl Pts',(51.457637890193,1076.62746842925,499.746358365276));
#130208=CARTESIAN_POINT('Ctrl Pts',(48.3693760270001,1076.66224654234,500.576797704051));
#130209=CARTESIAN_POINT('Ctrl Pts',(49.2178948810554,1076.66224654234,500.036458197465));
#130210=CARTESIAN_POINT('Ctrl Pts',(50.0572411842092,1076.66224654234,499.481977529229));
#130211=CARTESIAN_POINT('Ctrl Pts',(50.8871792875885,1076.66224654234,498.913511371376));
#130212=CARTESIAN_POINT('Ctrl Pts',(47.8311799129396,1076.68829438222,499.731644713397));
#130213=CARTESIAN_POINT('Ctrl Pts',(48.6702574719552,1076.68829438222,499.197317453539));
#130214=CARTESIAN_POINT('Ctrl Pts',(49.5002645411595,1076.68829438222,498.649006377832));
#130215=CARTESIAN_POINT('Ctrl Pts',(50.3209680936961,1076.68829438222,498.086865426179));
#130216=CARTESIAN_POINT('Ctrl Pts',(47.2970231924259,1076.70561806076,498.892834959804));
#130217=CARTESIAN_POINT('Ctrl Pts',(48.1267303173858,1076.70561806076,498.364474822172));
#130218=CARTESIAN_POINT('Ctrl Pts',(48.9474682476122,1076.70561806076,497.822287033547));
#130219=CARTESIAN_POINT('Ctrl Pts',(49.759006558586,1076.70561806076,497.266423814698));
#130220=CARTESIAN_POINT('Origin',(0.,1082.7251047501,424.620242579854));
#130221=CARTESIAN_POINT('Ctrl Pts',(3.5173666145595,1074.64994371665,537.655460170167));
#130222=CARTESIAN_POINT('Ctrl Pts',(4.2639663124766,1074.64994371665,537.632227898775));
#130223=CARTESIAN_POINT('Ctrl Pts',(5.01029920227245,1074.64994371665,537.601600052411));
#130224=CARTESIAN_POINT('Ctrl Pts',(5.75629202757494,1074.64994371665,537.563579637354));
#130225=CARTESIAN_POINT('Ctrl Pts',(3.49435080813864,1074.75355117008,536.915816859735));
#130226=CARTESIAN_POINT('Ctrl Pts',(4.23606514834239,1074.75355117008,536.892736608169));
#130227=CARTESIAN_POINT('Ctrl Pts',(4.9775144262776,1074.75355117008,536.862309174403));
#130228=CARTESIAN_POINT('Ctrl Pts',(5.71862586492354,1074.75355117008,536.824537545045));
#130229=CARTESIAN_POINT('Ctrl Pts',(3.47143790807793,1074.85328274408,536.179480580978));
#130230=CARTESIAN_POINT('Ctrl Pts',(4.20828873357357,1074.85328274408,536.15655166954));
#130231=CARTESIAN_POINT('Ctrl Pts',(4.94487623484748,1074.85328274408,536.126323752305));
#130232=CARTESIAN_POINT('Ctrl Pts',(5.68112811208704,1074.85328274408,536.088799796296));
#130233=CARTESIAN_POINT('Ctrl Pts',(3.44862795074633,1074.94914023354,535.446452502662));
#130234=CARTESIAN_POINT('Ctrl Pts',(4.18063711225881,1074.94914023354,535.423674251413));
#130235=CARTESIAN_POINT('Ctrl Pts',(4.9123846797877,1074.94914023354,535.393644954323));
#130236=CARTESIAN_POINT('Ctrl Pts',(5.64379882858451,1074.94914023354,535.356367558921));
#130237=CARTESIAN_POINT('Origin',(0.,1082.7251047501,424.620242579854));
#130238=CARTESIAN_POINT('Ctrl Pts',(14.9520407112949,1075.53663732595,529.546690715972));
#130239=CARTESIAN_POINT('Ctrl Pts',(15.697740763202,1075.53663732595,529.440428303276));
#130240=CARTESIAN_POINT('Ctrl Pts',(16.4422656965068,1075.53663732595,529.326222824188));
#130241=CARTESIAN_POINT('Ctrl Pts',(17.185530905513,1075.53663732595,529.204087256694));
#130242=CARTESIAN_POINT('Ctrl Pts',(14.8466056747203,1075.61824626063,528.806796803797));
#130243=CARTESIAN_POINT('Ctrl Pts',(15.5870473867283,1075.61824626063,528.701283705632));
#130244=CARTESIAN_POINT('Ctrl Pts',(16.3263222665394,1075.61824626063,528.587883551991));
#130245=CARTESIAN_POINT('Ctrl Pts',(17.0643463050586,1075.61824626063,528.466609229344));
#130246=CARTESIAN_POINT('Ctrl Pts',(14.7416762402029,1075.69566794643,528.070450971049));
#130247=CARTESIAN_POINT('Ctrl Pts',(15.4768848280991,1075.69566794643,527.96568359416));
#130248=CARTESIAN_POINT('Ctrl Pts',(16.2109348304675,1075.69566794643,527.853084904116));
#130249=CARTESIAN_POINT('Ctrl Pts',(16.9437428319531,1075.69566794643,527.732667696313));
#130250=CARTESIAN_POINT('Ctrl Pts',(14.6372525933972,1075.76890440336,527.337654520564));
#130251=CARTESIAN_POINT('Ctrl Pts',(15.3672532822281,1075.76890440336,527.233629270376));
#130252=CARTESIAN_POINT('Ctrl Pts',(16.0961035924491,1075.76890440336,527.121828180663));
#130253=CARTESIAN_POINT('Ctrl Pts',(16.8237206995835,1075.76890440336,527.002263956182));
#130254=CARTESIAN_POINT('Origin',(0.,1082.7251047501,424.620242579854));
#130255=CARTESIAN_POINT('Ctrl Pts',(24.2670610153852,1076.25706953122,519.598667421324));
#130256=CARTESIAN_POINT('Ctrl Pts',(25.1150319980636,1076.25706953122,519.382010179321));
#130257=CARTESIAN_POINT('Ctrl Pts',(25.9600256331401,1076.25706953122,519.154016967454));
#130258=CARTESIAN_POINT('Ctrl Pts',(26.8018903847055,1076.25706953122,518.914728672612));
#130259=CARTESIAN_POINT('Ctrl Pts',(24.0517235332975,1076.31903292809,518.755861823849));
#130260=CARTESIAN_POINT('Ctrl Pts',(24.892169915606,1076.31903292809,518.541127123061));
#130261=CARTESIAN_POINT('Ctrl Pts',(25.7296653702625,1076.31903292809,518.315157043875));
#130262=CARTESIAN_POINT('Ctrl Pts',(26.5640597060347,1076.31903292809,518.07799211036));
#130263=CARTESIAN_POINT('Ctrl Pts',(23.837677515676,1076.37491973991,517.918110866517));
#130264=CARTESIAN_POINT('Ctrl Pts',(24.6706444256336,1076.37491973991,517.7052871767));
#130265=CARTESIAN_POINT('Ctrl Pts',(25.5006866694382,1076.37491973991,517.481328096663));
#130266=CARTESIAN_POINT('Ctrl Pts',(26.32765539247,1076.37491973991,517.246273789834));
#130267=CARTESIAN_POINT('Ctrl Pts',(23.6249235335358,1076.42473350737,517.085416784213));
#130268=CARTESIAN_POINT('Ctrl Pts',(24.4504561191147,1076.42473350737,516.874492570025));
#130269=CARTESIAN_POINT('Ctrl Pts',(25.2730901415187,1076.42473350737,516.652532350241));
#130270=CARTESIAN_POINT('Ctrl Pts',(26.0926780746722,1076.42473350737,516.419575929826));
#130271=CARTESIAN_POINT('Origin',(0.,1082.7251047501,424.620242579854));
#130272=CARTESIAN_POINT('Ctrl Pts',(31.867100541542,1076.6273958791,509.923777861397));
#130273=CARTESIAN_POINT('Ctrl Pts',(32.8224307605543,1076.6273958791,509.566892252387));
#130274=CARTESIAN_POINT('Ctrl Pts',(33.7716315198204,1076.6273958791,509.19401012103));
#130275=CARTESIAN_POINT('Ctrl Pts',(34.7144349873161,1076.6273958791,508.805236681924));
#130276=CARTESIAN_POINT('Ctrl Pts',(31.5136676399737,1076.66220181075,508.977690031747));
#130277=CARTESIAN_POINT('Ctrl Pts',(32.4584024447335,1076.66220181075,508.624762583792));
#130278=CARTESIAN_POINT('Ctrl Pts',(33.3970757706022,1076.66220181075,508.256016028355));
#130279=CARTESIAN_POINT('Ctrl Pts',(34.3294227560376,1076.66220181075,507.871554413115));
#130280=CARTESIAN_POINT('Ctrl Pts',(31.1628674174928,1076.68826959406,508.038649496315));
#130281=CARTESIAN_POINT('Ctrl Pts',(32.097085731964,1076.68826959406,507.689650725552));
#130282=CARTESIAN_POINT('Ctrl Pts',(33.0253100420179,1076.68826959406,507.325008940628));
#130283=CARTESIAN_POINT('Ctrl Pts',(33.9472784344677,1076.68826959406,506.944827030996));
#130284=CARTESIAN_POINT('Ctrl Pts',(30.8147012693935,1076.70560534914,507.1066599901));
#130285=CARTESIAN_POINT('Ctrl Pts',(31.7384820593689,1076.70560534914,506.761560397037));
#130286=CARTESIAN_POINT('Ctrl Pts',(32.6563358127511,1076.70560534914,506.400992560893));
#130287=CARTESIAN_POINT('Ctrl Pts',(33.5680035425704,1076.70560534914,506.025058221592));
#130288=CARTESIAN_POINT('Origin',(0.,1082.7251047501,424.620242579854));
#130289=CARTESIAN_POINT('Ctrl Pts',(-20.0609463067695,1074.64954802915,
535.919523414127));
#130290=CARTESIAN_POINT('Ctrl Pts',(-19.3257242373893,1074.64954802915,
536.05204224396));
#130291=CARTESIAN_POINT('Ctrl Pts',(-18.5892252109256,1074.64954802915,
536.177269699343));
#130292=CARTESIAN_POINT('Ctrl Pts',(-17.8515215358667,1074.64954802915,
536.295193485614));
#130293=CARTESIAN_POINT('Ctrl Pts',(-19.9293635146521,1074.75341498236,
535.189494535684));
#130294=CARTESIAN_POINT('Ctrl Pts',(-19.1989638784332,1074.75341498236,
535.321144154395));
#130295=CARTESIAN_POINT('Ctrl Pts',(-18.467295660886,1074.75341498236,535.44555022389));
#130296=CARTESIAN_POINT('Ctrl Pts',(-17.7344306962167,1074.75341498236,
535.562700530145));
#130297=CARTESIAN_POINT('Ctrl Pts',(-19.7983704549659,1074.85338735602,
534.462737526598));
#130298=CARTESIAN_POINT('Ctrl Pts',(-19.072771638556,1074.85338735602,534.593521829849));
#130299=CARTESIAN_POINT('Ctrl Pts',(-18.3459125790345,1074.85338735602,
534.71711019477));
#130300=CARTESIAN_POINT('Ctrl Pts',(-17.6178646384507,1074.85338735602,
534.833490487621));
#130301=CARTESIAN_POINT('Ctrl Pts',(-19.6679673366353,1074.94946695803,
533.739253545992));
#130302=CARTESIAN_POINT('Ctrl Pts',(-18.9471477190252,1074.94946695803,
533.869176430824));
#130303=CARTESIAN_POINT('Ctrl Pts',(-18.2250761589681,1074.94946695803,
533.991950773792));
#130304=CARTESIAN_POINT('Ctrl Pts',(-17.5018235484828,1074.94946695803,
534.107564521076));
#130305=CARTESIAN_POINT('Origin',(0.,1082.7251047501,424.620242579854));
#130306=CARTESIAN_POINT('Ctrl Pts',(-7.18812240170579,1075.53634869535,
530.365286015731));
#130307=CARTESIAN_POINT('Ctrl Pts',(-6.43769521904607,1075.53634869535,
530.416297034946));
#130308=CARTESIAN_POINT('Ctrl Pts',(-5.68676756649073,1075.53634869535,
530.459317276502));
#130309=CARTESIAN_POINT('Ctrl Pts',(-4.93542452985916,1075.53634869535,
530.494341865881));
#130310=CARTESIAN_POINT('Ctrl Pts',(-7.13741356032504,1075.61800315405,
529.619304195344));
#130311=CARTESIAN_POINT('Ctrl Pts',(-6.39228029043513,1075.61800315405,
529.669955355678));
#130312=CARTESIAN_POINT('Ctrl Pts',(-5.64665008123061,1075.61800315405,
529.712672109553));
#130313=CARTESIAN_POINT('Ctrl Pts',(-4.90060741829024,1075.61800315405,
529.747449616836));
#130314=CARTESIAN_POINT('Ctrl Pts',(-7.08694799094726,1075.69546670263,
528.876901168845));
#130315=CARTESIAN_POINT('Ctrl Pts',(-6.3470832366631,1075.69546670263,528.927194196695));
#130316=CARTESIAN_POINT('Ctrl Pts',(-5.60672505670767,1075.69546670263,
528.969608918849));
#130317=CARTESIAN_POINT('Ctrl Pts',(-4.86595733929864,1075.69546670263,
529.004140529394));
#130318=CARTESIAN_POINT('Ctrl Pts',(-7.03672578293973,1075.76874136376,
528.138078250924));
#130319=CARTESIAN_POINT('Ctrl Pts',(-6.3021041377675,1075.76874136376,528.188014873321));
#130320=CARTESIAN_POINT('Ctrl Pts',(-5.56699256362338,1075.76874136376,
528.230129020248));
#130321=CARTESIAN_POINT('Ctrl Pts',(-4.83147435424468,1075.76874136376,
528.264415919851));
#130322=CARTESIAN_POINT('Origin',(0.,1082.7251047501,424.620242579854));
#130323=CARTESIAN_POINT('Ctrl Pts',(3.98619775720727,1076.25727779325,522.565780470137));
#130324=CARTESIAN_POINT('Ctrl Pts',(4.86230647016848,1076.25727779325,522.530124505997));
#130325=CARTESIAN_POINT('Ctrl Pts',(5.73785795148452,1076.25727779325,522.482717457253));
#130326=CARTESIAN_POINT('Ctrl Pts',(6.61269459313368,1076.25727779325,522.42356785765));
#130327=CARTESIAN_POINT('Ctrl Pts',(3.95094675756026,1076.3190144058,521.69962220808));
#130328=CARTESIAN_POINT('Ctrl Pts',(4.81930780976492,1076.3190144058,521.664281559049));
#130329=CARTESIAN_POINT('Ctrl Pts',(5.68711655807104,1076.3190144058,521.617293743359));
#130330=CARTESIAN_POINT('Ctrl Pts',(6.55421678822626,1076.3190144058,521.558667219288));
#130331=CARTESIAN_POINT('Ctrl Pts',(3.91590644763562,1076.37471618392,520.838640838752));
#130332=CARTESIAN_POINT('Ctrl Pts',(4.7765661456427,1076.37471618392,520.803613620241));
#130333=CARTESIAN_POINT('Ctrl Pts',(5.6366784380455,1076.37471618392,520.757042531915));
#130334=CARTESIAN_POINT('Ctrl Pts',(6.49608849603066,1076.37471618392,520.698935957035));
#130335=CARTESIAN_POINT('Ctrl Pts',(3.88107692026826,1076.42438663189,519.982838643216));
#130336=CARTESIAN_POINT('Ctrl Pts',(4.73408159104051,1076.42438663189,519.948122969804));
#130337=CARTESIAN_POINT('Ctrl Pts',(5.58654372503737,1076.42438663189,519.901966102047));
#130338=CARTESIAN_POINT('Ctrl Pts',(6.4383098705505,1076.42438663189,519.84437634864));
#130339=CARTESIAN_POINT('Origin',(0.,1082.7251047501,424.620242579854));
#130340=CARTESIAN_POINT('Ctrl Pts',(13.4352335940896,1076.62753213844,514.681218805467));
#130341=CARTESIAN_POINT('Ctrl Pts',(14.4439034065725,1076.62753213844,514.530746146631));
#130342=CARTESIAN_POINT('Ctrl Pts',(15.4499032260186,1076.62753213844,514.36335088103));
#130343=CARTESIAN_POINT('Ctrl Pts',(16.4529491598105,1076.62753213844,514.179080247518));
#130344=CARTESIAN_POINT('Ctrl Pts',(13.2864477959342,1076.66226255021,513.683856598361));
#130345=CARTESIAN_POINT('Ctrl Pts',(14.2839472970061,1076.66226255021,513.535050318788));
#130346=CARTESIAN_POINT('Ctrl Pts',(15.2788063733432,1076.66226255021,513.369508838461));
#130347=CARTESIAN_POINT('Ctrl Pts',(16.2707442762401,1076.66226255021,513.187278873099));
#130348=CARTESIAN_POINT('Ctrl Pts',(13.1387686281562,1076.68828128334,512.693912514015));
#130349=CARTESIAN_POINT('Ctrl Pts',(14.1251808997112,1076.68828128334,512.546760219605));
#130350=CARTESIAN_POINT('Ctrl Pts',(15.1089820949122,1076.68828128334,512.383058736577));
#130351=CARTESIAN_POINT('Ctrl Pts',(16.0898945855816,1076.68828128334,512.202854261401));
#130352=CARTESIAN_POINT('Ctrl Pts',(12.9921966763696,1076.7055944302,511.711390478002));
#130353=CARTESIAN_POINT('Ctrl Pts',(13.9676048442678,1076.7055944302,511.565879768097));
#130354=CARTESIAN_POINT('Ctrl Pts',(14.9404310641548,1076.7055944302,511.404004487093));
#130355=CARTESIAN_POINT('Ctrl Pts',(15.9104008049853,1076.7055944302,511.22581031611));
#130356=CARTESIAN_POINT('Origin',(0.,1082.7251047501,424.620242579854));
#130357=CARTESIAN_POINT('Ctrl Pts',(-42.7617176792035,1074.64965272011,
529.316173097487));
#130358=CARTESIAN_POINT('Ctrl Pts',(-42.0711681572054,1074.64965272011,
529.598219243476));
#130359=CARTESIAN_POINT('Ctrl Pts',(-41.3778620576057,1074.64965272011,
529.87341975775));
#130360=CARTESIAN_POINT('Ctrl Pts',(-40.6818672413462,1074.64965272011,
530.141747703627));
#130361=CARTESIAN_POINT('Ctrl Pts',(-42.4809605599403,1074.75361908038,
528.628779572484));
#130362=CARTESIAN_POINT('Ctrl Pts',(-41.7949449225714,1074.75361908038,
528.908973911114));
#130363=CARTESIAN_POINT('Ctrl Pts',(-41.1061908062375,1074.75361908038,
529.182367563835));
#130364=CARTESIAN_POINT('Ctrl Pts',(-40.4147656263312,1074.75361908038,
529.448933770821));
#130365=CARTESIAN_POINT('Ctrl Pts',(-42.2014629878619,1074.8536832068,527.944469868049));
#130366=CARTESIAN_POINT('Ctrl Pts',(-41.5199608949733,1074.8536832068,528.222820706996));
#130367=CARTESIAN_POINT('Ctrl Pts',(-40.8357383405612,1074.8536832068,528.494415604201));
#130368=CARTESIAN_POINT('Ctrl Pts',(-40.148862296468,1074.8536832068,528.759227975899));
#130369=CARTESIAN_POINT('Ctrl Pts',(-41.923225409626,1074.94984691261,527.263245077761));
#130370=CARTESIAN_POINT('Ctrl Pts',(-41.2462165138558,1074.94984691261,
527.539760727644));
#130371=CARTESIAN_POINT('Ctrl Pts',(-40.5665050927797,1074.94984691261,
527.809564978243));
#130372=CARTESIAN_POINT('Ctrl Pts',(-39.8841576766896,1074.94984691261,
528.072631421062));
#130373=CARTESIAN_POINT('Origin',(0.,1082.7251047501,424.620242579854));
#130374=CARTESIAN_POINT('Ctrl Pts',(-29.0176510102205,1075.53628195624,
526.560366125851));
#130375=CARTESIAN_POINT('Ctrl Pts',(-28.2931960294411,1075.53628195624,
526.766585042148));
#130376=CARTESIAN_POINT('Ctrl Pts',(-27.5665839967992,1075.53628195624,
526.965069839135));
#130377=CARTESIAN_POINT('Ctrl Pts',(-26.8378974774944,1075.53628195624,
527.155797962909));
#130378=CARTESIAN_POINT('Ctrl Pts',(-28.8128258799699,1075.61798649467,
525.840807569036));
#130379=CARTESIAN_POINT('Ctrl Pts',(-28.0934845655498,1075.61798649467,
526.045570860397));
#130380=CARTESIAN_POINT('Ctrl Pts',(-27.3720014251182,1075.61798649467,
526.242654624806));
#130381=CARTESIAN_POINT('Ctrl Pts',(-26.6484584410766,1075.61798649467,
526.43203646756));
#130382=CARTESIAN_POINT('Ctrl Pts',(-28.6089839559804,1075.69549521486,
525.124703053615));
#130383=CARTESIAN_POINT('Ctrl Pts',(-27.8947317611819,1075.69549521486,
525.328017707364));
#130384=CARTESIAN_POINT('Ctrl Pts',(-27.1783528931352,1075.69549521486,
525.523707164464));
#130385=CARTESIAN_POINT('Ctrl Pts',(-26.4599287542417,1075.69549521486,
525.711749188647));
#130386=CARTESIAN_POINT('Ctrl Pts',(-28.4061255996499,1075.76881014303,
524.412053849191));
#130387=CARTESIAN_POINT('Ctrl Pts',(-27.6969379687123,1075.76881014303,
524.613926855221));
#130388=CARTESIAN_POINT('Ctrl Pts',(-26.9856387441757,1075.76881014303,
524.808228732752));
#130389=CARTESIAN_POINT('Ctrl Pts',(-26.2723087512395,1075.76881014303,
524.994937403189));
#130390=CARTESIAN_POINT('Origin',(0.,1082.7251047501,424.620242579854));
#130391=CARTESIAN_POINT('Ctrl Pts',(-16.4646989908154,1076.25701255651,
521.258029889561));
#130392=CARTESIAN_POINT('Ctrl Pts',(-15.6004015618574,1076.25701255651,
521.405284885795));
#130393=CARTESIAN_POINT('Ctrl Pts',(-14.7342065197343,1076.25701255651,
521.540932328162));
#130394=CARTESIAN_POINT('Ctrl Pts',(-13.8662697472228,1076.25701255651,
521.664947805186));
#130395=CARTESIAN_POINT('Ctrl Pts',(-16.3187084370332,1076.31893267559,
520.401153970147));
#130396=CARTESIAN_POINT('Ctrl Pts',(-15.4620746319505,1076.31893267559,
520.54710327361));
#130397=CARTESIAN_POINT('Ctrl Pts',(-14.603560039616,1076.31893267559,520.681547946024));
#130398=CARTESIAN_POINT('Ctrl Pts',(-13.743319160612,1076.31893267559,520.804463792367));
#130399=CARTESIAN_POINT('Ctrl Pts',(-16.173592779169,1076.37478542332,519.54941315862));
#130400=CARTESIAN_POINT('Ctrl Pts',(-15.3245766712008,1076.37478542332,
519.694064594101));
#130401=CARTESIAN_POINT('Ctrl Pts',(-14.4736965010593,1076.37478542332,
519.827313704553));
#130402=CARTESIAN_POINT('Ctrl Pts',(-13.6211053954157,1076.37478542332,
519.949136510109));
#130403=CARTESIAN_POINT('Ctrl Pts',(-16.0293524037607,1076.42457433234,
518.702809723722));
#130404=CARTESIAN_POINT('Ctrl Pts',(-15.1879080458553,1076.42457433234,
518.846171119467));
#130405=CARTESIAN_POINT('Ctrl Pts',(-14.3446162499757,1076.42457433234,
518.978231879131));
#130406=CARTESIAN_POINT('Ctrl Pts',(-13.4996287771691,1076.42457433234,
519.098968236707));
#130407=CARTESIAN_POINT('Origin',(0.,1082.7251047501,424.620242579854));
#130408=CARTESIAN_POINT('Ctrl Pts',(-5.58190196061815,1076.62744005165,
515.509263604268));
#130409=CARTESIAN_POINT('Ctrl Pts',(-4.56636243499452,1076.62744005165,
515.571632436116));
#130410=CARTESIAN_POINT('Ctrl Pts',(-3.54992031559118,1076.62744005165,
515.616973556448));
#130411=CARTESIAN_POINT('Ctrl Pts',(-2.53286108863103,1076.62744005165,
515.645274230384));
#130412=CARTESIAN_POINT('Ctrl Pts',(-5.52010923061872,1076.66217353754,
514.503104632702));
#130413=CARTESIAN_POINT('Ctrl Pts',(-4.51581192317688,1076.66217353754,
514.564783029568));
#130414=CARTESIAN_POINT('Ctrl Pts',(-3.51062201384234,1076.66217353754,
514.609622214962));
#130415=CARTESIAN_POINT('Ctrl Pts',(-2.50482182845053,1076.66217353754,
514.637609594987));
#130416=CARTESIAN_POINT('Ctrl Pts',(-5.45877592976358,1076.68820151705,
513.504426456294));
#130417=CARTESIAN_POINT('Ctrl Pts',(-4.46563725457555,1076.68820151705,
513.565419551563));
#130418=CARTESIAN_POINT('Ctrl Pts',(-3.47161589509213,1076.68820151705,
513.609760533908));
#130419=CARTESIAN_POINT('Ctrl Pts',(-2.47699104025874,1076.68820151705,
513.637436949361));
#130420=CARTESIAN_POINT('Ctrl Pts',(-5.39790230109045,1076.70553007605,
512.513233032379));
#130421=CARTESIAN_POINT('Ctrl Pts',(-4.41583862801136,1076.70553007605,
512.573545962152));
#130422=CARTESIAN_POINT('Ctrl Pts',(-3.43290211390516,1076.70553007605,
512.617392475312));
#130423=CARTESIAN_POINT('Ctrl Pts',(-2.44936883433722,1076.70553007605,
512.644760256767));
#130424=CARTESIAN_POINT('Origin',(0.,1082.7251047501,424.620242579854));
#130425=CARTESIAN_POINT('Ctrl Pts',(-63.5965651485269,1074.64936691183,
518.138908889593));
#130426=CARTESIAN_POINT('Ctrl Pts',(-62.9786024477089,1074.64936691183,
518.559149112349));
#130427=CARTESIAN_POINT('Ctrl Pts',(-62.3565048751138,1074.64936691183,
518.973243732692));
#130428=CARTESIAN_POINT('Ctrl Pts',(-61.7303335462127,1074.64936691183,
519.381152069561));
#130429=CARTESIAN_POINT('Ctrl Pts',(-63.1793148961809,1074.75326661151,
517.525342936374));
#130430=CARTESIAN_POINT('Ctrl Pts',(-62.5654065824553,1074.75326661151,
517.94282600804));
#130431=CARTESIAN_POINT('Ctrl Pts',(-61.9473905254034,1074.75326661151,
518.35420379793));
#130432=CARTESIAN_POINT('Ctrl Pts',(-61.3253274395243,1074.75326661151,
518.75943589189));
#130433=CARTESIAN_POINT('Ctrl Pts',(-62.7639351887473,1074.85326961418,
516.914527617015));
#130434=CARTESIAN_POINT('Ctrl Pts',(-62.1540630861798,1074.85326961418,
517.329265897978));
#130435=CARTESIAN_POINT('Ctrl Pts',(-61.5401102471193,1074.85326961418,
517.737939037045));
#130436=CARTESIAN_POINT('Ctrl Pts',(-60.9221369868903,1074.85326961418,
518.140506885771));
#130437=CARTESIAN_POINT('Ctrl Pts',(-62.3504266890833,1074.94937772924,
516.306463906247));
#130438=CARTESIAN_POINT('Ctrl Pts',(-61.7445726152988,1074.94937772924,
516.718469761274));
#130439=CARTESIAN_POINT('Ctrl Pts',(-61.1346646901937,1074.94937772924,
517.124450433464));
#130440=CARTESIAN_POINT('Ctrl Pts',(-60.5207628317164,1074.94937772924,
517.524366038881));
#130441=CARTESIAN_POINT('Origin',(0.,1082.7251047501,424.620242579854));
#130442=CARTESIAN_POINT('Ctrl Pts',(-49.5774617998323,1075.53622510687,
518.300541925841));
#130443=CARTESIAN_POINT('Ctrl Pts',(-48.911899503254,1075.53622510687,518.652770618153));
#130444=CARTESIAN_POINT('Ctrl Pts',(-48.2426214679627,1075.53622510687,
518.997886734541));
#130445=CARTESIAN_POINT('Ctrl Pts',(-47.569703700229,1075.53622510687,519.335851082043));
#130446=CARTESIAN_POINT('Ctrl Pts',(-49.2269716736319,1075.61805805635,
517.638264779164));
#130447=CARTESIAN_POINT('Ctrl Pts',(-48.5661146000491,1075.61805805635,
517.988003374679));
#130448=CARTESIAN_POINT('Ctrl Pts',(-47.9015680563376,1075.61805805635,
518.33067967695));
#130449=CARTESIAN_POINT('Ctrl Pts',(-47.2334075114381,1075.61805805635,
518.666254770092));
#130450=CARTESIAN_POINT('Ctrl Pts',(-48.8781665782885,1075.69568218855,
516.979171623546));
#130451=CARTESIAN_POINT('Ctrl Pts',(-48.2219921066762,1075.69568218855,
517.326432093757));
#130452=CARTESIAN_POINT('Ctrl Pts',(-47.5621543072295,1075.69568218855,
517.666680311663));
#130453=CARTESIAN_POINT('Ctrl Pts',(-46.8987281141425,1075.69568218855,
517.999877637121));
#130454=CARTESIAN_POINT('Ctrl Pts',(-48.5310471341285,1075.7690995391,516.32326363114));
#130455=CARTESIAN_POINT('Ctrl Pts',(-47.8795326351339,1075.7690995391,516.668057951947));
#130456=CARTESIAN_POINT('Ctrl Pts',(-47.2243808242627,1075.7690995391,517.005889819556));
#130457=CARTESIAN_POINT('Ctrl Pts',(-46.5656661035469,1075.7690995391,517.336720868239));
#130458=CARTESIAN_POINT('Origin',(0.,1082.7251047501,424.620242579854));
#130459=CARTESIAN_POINT('Ctrl Pts',(-36.1968662814073,1076.25723523531,
515.719760643928));
#130460=CARTESIAN_POINT('Ctrl Pts',(-35.3839173772627,1076.25723523531,
516.042772262456));
#130461=CARTESIAN_POINT('Ctrl Pts',(-34.5667178457009,1076.25723523531,
516.354873771694));
#130462=CARTESIAN_POINT('Ctrl Pts',(-33.7454140973306,1076.25723523531,
516.6560092551));
#130463=CARTESIAN_POINT('Ctrl Pts',(-35.8758056493458,1076.31916041081,
514.911721941828));
#130464=CARTESIAN_POINT('Ctrl Pts',(-35.0700674768422,1076.31916041081,
515.23186849702));
#130465=CARTESIAN_POINT('Ctrl Pts',(-34.2601163793322,1076.31916041081,
515.541201713914));
#130466=CARTESIAN_POINT('Ctrl Pts',(-33.4460974687851,1076.31916041081,
515.839666171937));
#130467=CARTESIAN_POINT('Ctrl Pts',(-35.5566697156339,1076.37501437569,
514.108527280388));
#130468=CARTESIAN_POINT('Ctrl Pts',(-34.7580990477857,1076.37501437569,
514.425825947764));
#130469=CARTESIAN_POINT('Ctrl Pts',(-33.9553529313231,1076.37501437569,
514.732407467707));
#130470=CARTESIAN_POINT('Ctrl Pts',(-33.148575187361,1076.37501437569,515.028216912643));
#130471=CARTESIAN_POINT('Ctrl Pts',(-35.2394593308914,1076.42480066596,
513.310178800431));
#130472=CARTESIAN_POINT('Ctrl Pts',(-34.448012921609,1076.42480066596,513.624646763099));
#130473=CARTESIAN_POINT('Ctrl Pts',(-33.6524283139854,1076.42480066596,
513.92849318882));
#130474=CARTESIAN_POINT('Ctrl Pts',(-32.8528480460696,1076.42480066596,
514.221663640044));
#130475=CARTESIAN_POINT('Origin',(0.,1082.7251047501,424.620242579854));
#130476=CARTESIAN_POINT('Ctrl Pts',(-24.3584940949169,1076.62734697186,
512.364914333088));
#130477=CARTESIAN_POINT('Ctrl Pts',(-23.3756297382246,1076.62734697186,
512.637763899338));
#130478=CARTESIAN_POINT('Ctrl Pts',(-22.3883200821596,1076.62734697186,
512.894062304522));
#130479=CARTESIAN_POINT('Ctrl Pts',(-21.3968438225608,1076.62734697186,
513.133737201227));
#130480=CARTESIAN_POINT('Ctrl Pts',(-24.0886312393208,1076.66212359129,
511.39280876735));
#130481=CARTESIAN_POINT('Ctrl Pts',(-23.116655839102,1076.66212359129,511.662635488148));
#130482=CARTESIAN_POINT('Ctrl Pts',(-22.1402843880881,1076.66212359129,
511.916094414863));
#130483=CARTESIAN_POINT('Ctrl Pts',(-21.1597924945025,1076.66212359129,
512.153114001606));
#130484=CARTESIAN_POINT('Ctrl Pts',(-23.8207763800282,1076.68818087236,
510.42793644747));
#130485=CARTESIAN_POINT('Ctrl Pts',(-22.8596089137046,1076.68818087236,
510.694762815213));
#130486=CARTESIAN_POINT('Ctrl Pts',(-21.8940942787144,1076.68818087236,
510.945403391459));
#130487=CARTESIAN_POINT('Ctrl Pts',(-20.9245050186402,1076.68818087236,
511.179787425878));
#130488=CARTESIAN_POINT('Ctrl Pts',(-23.5549305801114,1076.70552491543,
509.47030120287));
#130489=CARTESIAN_POINT('Ctrl Pts',(-22.6044899822098,1076.70552491543,
509.734149721862));
#130490=CARTESIAN_POINT('Ctrl Pts',(-21.6497507311271,1076.70552491543,
509.981993086825));
#130491=CARTESIAN_POINT('Ctrl Pts',(-20.6909823287917,1076.70552491543,
510.213761337017));
#130492=CARTESIAN_POINT('Origin',(0.,1082.7251047501,424.620242579854));
#130493=CARTESIAN_POINT('Ctrl Pts',(-81.6487557536238,1074.64931959703,
502.875090091892));
#130494=CARTESIAN_POINT('Ctrl Pts',(-81.1322577363025,1074.64931959703,
503.413988598556));
#130495=CARTESIAN_POINT('Ctrl Pts',(-80.6104499440739,1074.64931959703,
503.947747373989));
#130496=CARTESIAN_POINT('Ctrl Pts',(-80.0833835204045,1074.64931959703,
504.476314103383));
#130497=CARTESIAN_POINT('Ctrl Pts',(-81.1119145088187,1074.75344418584,
502.360563821863));
#130498=CARTESIAN_POINT('Ctrl Pts',(-80.5988124702359,1074.75344418584,
502.895919066386));
#130499=CARTESIAN_POINT('Ctrl Pts',(-80.0804355685597,1074.75344418584,
503.426168373453));
#130500=CARTESIAN_POINT('Ctrl Pts',(-79.5568346109878,1074.75344418584,
503.951259772227));
#130501=CARTESIAN_POINT('Ctrl Pts',(-80.5774851171265,1074.85365527957,
501.848349151023));
#130502=CARTESIAN_POINT('Ctrl Pts',(-80.0677638002541,1074.85365527957,
502.380177052129));
#130503=CARTESIAN_POINT('Ctrl Pts',(-79.5528023752549,1074.85365527957,
502.906932657731));
#130504=CARTESIAN_POINT('Ctrl Pts',(-79.0326513145686,1074.85365527957,
503.428564339414));
#130505=CARTESIAN_POINT('Ctrl Pts',(-80.045468435066,1074.94995469931,501.338446900288));
#130506=CARTESIAN_POINT('Ctrl Pts',(-79.5391125774579,1074.94995469931,
501.866763382355));
#130507=CARTESIAN_POINT('Ctrl Pts',(-79.0275512097863,1074.94995469931,
502.390041058989));
#130508=CARTESIAN_POINT('Ctrl Pts',(-78.5108344712444,1074.94995469931,
502.908228642658));
#130509=CARTESIAN_POINT('Origin',(0.,1082.7251047501,424.620242579854));
#130510=CARTESIAN_POINT('Ctrl Pts',(-67.9701058202362,1075.5367489508,505.940418806113));
#130511=CARTESIAN_POINT('Ctrl Pts',(-67.3934113371822,1075.5367489508,506.422439220457));
#130512=CARTESIAN_POINT('Ctrl Pts',(-66.8116221918185,1075.5367489508,506.898298019857));
#130513=CARTESIAN_POINT('Ctrl Pts',(-66.2248042139591,1075.5367489508,507.367941360586));
#130514=CARTESIAN_POINT('Ctrl Pts',(-67.4905656334257,1075.61839547079,
505.366691694342));
#130515=CARTESIAN_POINT('Ctrl Pts',(-66.9179398240452,1075.61839547079,
505.845311376015));
#130516=CARTESIAN_POINT('Ctrl Pts',(-66.3402552960289,1075.61839547079,
506.317812913943));
#130517=CARTESIAN_POINT('Ctrl Pts',(-65.7575774147506,1075.61839547079,
506.784142844273));
#130518=CARTESIAN_POINT('Ctrl Pts',(-67.01332620572,1075.6958504928,504.795717235868));
#130519=CARTESIAN_POINT('Ctrl Pts',(-66.4447495491506,1075.6958504928,505.270952501055));
#130520=CARTESIAN_POINT('Ctrl Pts',(-65.8711499451671,1075.6958504928,505.740112885127));
#130521=CARTESIAN_POINT('Ctrl Pts',(-65.2925922969317,1075.6958504928,506.203145302288));
#130522=CARTESIAN_POINT('Ctrl Pts',(-66.5383883823746,1075.76911603994,
504.227496441963));
#130523=CARTESIAN_POINT('Ctrl Pts',(-65.9738413505823,1075.76911603994,
504.699363612844));
#130524=CARTESIAN_POINT('Ctrl Pts',(-65.4043069700822,1075.76911603994,
505.165198956596));
#130525=CARTESIAN_POINT('Ctrl Pts',(-64.8298496840536,1075.76911603994,
505.624949763653));
#130526=CARTESIAN_POINT('Origin',(0.,1082.7251047501,424.620242579854));
#130527=CARTESIAN_POINT('Ctrl Pts',(-54.3493735289956,1076.25693128953,
506.206500653992));
#130528=CARTESIAN_POINT('Ctrl Pts',(-53.6191815405488,1076.25693128953,
506.692924202084));
#130529=CARTESIAN_POINT('Ctrl Pts',(-52.8825255487871,1076.25693128953,
507.169501748694));
#130530=CARTESIAN_POINT('Ctrl Pts',(-52.1395383098849,1076.25693128953,
507.636147407581));
#130531=CARTESIAN_POINT('Ctrl Pts',(-53.8678157746301,1076.31881191121,
505.483612924582));
#130532=CARTESIAN_POINT('Ctrl Pts',(-53.1440935868706,1076.31881191121,
505.96572656041));
#130533=CARTESIAN_POINT('Ctrl Pts',(-52.4139646695184,1076.31881191121,
506.43808143437));
#130534=CARTESIAN_POINT('Ctrl Pts',(-51.6775606024737,1076.31881191121,
506.900592421209));
#130535=CARTESIAN_POINT('Ctrl Pts',(-53.3891418081157,1076.37463393687,
504.765054177174));
#130536=CARTESIAN_POINT('Ctrl Pts',(-52.671850676921,1076.37463393687,505.242883710463));
#130537=CARTESIAN_POINT('Ctrl Pts',(-51.9482097468746,1076.37463393687,
505.711041199065));
#130538=CARTESIAN_POINT('Ctrl Pts',(-51.2183494286465,1076.37463393687,
506.169442274161));
#130539=CARTESIAN_POINT('Ctrl Pts',(-52.9133529026173,1076.42440089149,
504.050826322972));
#130540=CARTESIAN_POINT('Ctrl Pts',(-52.2024540667598,1076.42440089149,
504.52439757484));
#130541=CARTESIAN_POINT('Ctrl Pts',(-51.4852620196589,1076.42440089149,
504.988382976543));
#130542=CARTESIAN_POINT('Ctrl Pts',(-50.7619060098017,1076.42440089149,
505.442698911133));
#130543=CARTESIAN_POINT('Origin',(0.,1082.7251047501,424.620242579854));
#130544=CARTESIAN_POINT('Ctrl Pts',(-42.0660921733734,1076.62733098606,
505.385284537138));
#130545=CARTESIAN_POINT('Ctrl Pts',(-41.1625853458286,1076.62733098606,
505.855871818042));
#130546=CARTESIAN_POINT('Ctrl Pts',(-40.2513098605778,1076.62733098606,
506.311233176031));
#130547=CARTESIAN_POINT('Ctrl Pts',(-39.332522282548,1076.62733098606,506.751240406456));
#130548=CARTESIAN_POINT('Ctrl Pts',(-41.5990376134109,1076.66218595673,
504.488560378016));
#130549=CARTESIAN_POINT('Ctrl Pts',(-40.7055623091657,1076.66218595673,
504.953922787199));
#130550=CARTESIAN_POINT('Ctrl Pts',(-39.8044046016495,1076.66218595673,
505.404228324985));
#130551=CARTESIAN_POINT('Ctrl Pts',(-38.8958182071807,1076.66218595673,
505.839350210165));
#130552=CARTESIAN_POINT('Ctrl Pts',(-41.135465868248,1076.68828360045,503.598523069725));
#130553=CARTESIAN_POINT('Ctrl Pts',(-40.2519472824706,1076.68828360045,
504.058699568932));
#130554=CARTESIAN_POINT('Ctrl Pts',(-39.3608319046597,1076.68828360045,
504.503986987646));
#130555=CARTESIAN_POINT('Ctrl Pts',(-38.4623706237676,1076.68828360045,
504.934259957486));
#130556=CARTESIAN_POINT('Ctrl Pts',(-40.675378785767,1076.70563005751,502.715176160118));
#130557=CARTESIAN_POINT('Ctrl Pts',(-39.8017420739363,1076.70563005751,
503.170205731766));
#130558=CARTESIAN_POINT('Ctrl Pts',(-38.9205935377711,1076.70563005751,
503.610512752543));
#130559=CARTESIAN_POINT('Ctrl Pts',(-38.0321812601107,1076.70563005751,
504.035973256274));
#130560=CARTESIAN_POINT('Origin',(0.,1082.7251047501,424.620242579854));
#130561=CARTESIAN_POINT('Ctrl Pts',(-96.131601715426,1074.65015601416,484.182852263091));
#130562=CARTESIAN_POINT('Ctrl Pts',(-95.7386795646446,1074.65015601416,
484.817012450245));
#130563=CARTESIAN_POINT('Ctrl Pts',(-95.3395017199826,1074.65015601416,
485.447253680153));
#130564=CARTESIAN_POINT('Ctrl Pts',(-94.9341072652433,1074.65015601416,
486.073514245423));
#130565=CARTESIAN_POINT('Ctrl Pts',(-95.5012439298025,1074.7539752954,483.792286059305));
#130566=CARTESIAN_POINT('Ctrl Pts',(-95.1108982630542,1074.7539752954,484.422287907222));
#130567=CARTESIAN_POINT('Ctrl Pts',(-94.7143379224985,1074.7539752954,485.048396495429));
#130568=CARTESIAN_POINT('Ctrl Pts',(-94.3116017356569,1074.7539752954,485.670550521162));
#130569=CARTESIAN_POINT('Ctrl Pts',(-94.8737104720578,1074.85390243578,
483.40346979348));
#130570=CARTESIAN_POINT('Ctrl Pts',(-94.4859297453657,1074.85390243578,
484.029331933664));
#130571=CARTESIAN_POINT('Ctrl Pts',(-94.0919751811483,1074.85390243578,
484.651326396534));
#130572=CARTESIAN_POINT('Ctrl Pts',(-93.6918853517936,1074.85390243578,
485.269392282145));
#130573=CARTESIAN_POINT('Ctrl Pts',(-94.2490023424518,1074.94993924152,
483.01640408537));
#130574=CARTESIAN_POINT('Ctrl Pts',(-93.8637750077506,1074.94993924152,
483.638145155924));
#130575=CARTESIAN_POINT('Ctrl Pts',(-93.4724144879501,1074.94993924152,
484.256044016381));
#130576=CARTESIAN_POINT('Ctrl Pts',(-93.0749591014535,1074.94993924152,
484.870040167801));
#130577=CARTESIAN_POINT('Origin',(0.,1082.7251047501,424.620242579854));
#130578=CARTESIAN_POINT('Ctrl Pts',(-83.396532923316,1075.53617509883,490.034603122049));
#130579=CARTESIAN_POINT('Ctrl Pts',(-82.9312588738367,1075.53617509883,
490.62777933388));
#130580=CARTESIAN_POINT('Ctrl Pts',(-82.4596828994069,1075.53617509883,
491.215957928986));
#130581=CARTESIAN_POINT('Ctrl Pts',(-81.981858676633,1075.53617509883,491.799071958599));
#130582=CARTESIAN_POINT('Ctrl Pts',(-82.808284881169,1075.61782568845,489.573194617781));
#130583=CARTESIAN_POINT('Ctrl Pts',(-82.34629270132,1075.61782568845,490.162186785827));
#130584=CARTESIAN_POINT('Ctrl Pts',(-81.8780430479488,1075.61782568845,
490.746216588473));
#130585=CARTESIAN_POINT('Ctrl Pts',(-81.4035892190472,1075.61782568845,
491.325217549183));
#130586=CARTESIAN_POINT('Ctrl Pts',(-82.2228585576068,1075.69528637324,
489.113999405966));
#130587=CARTESIAN_POINT('Ctrl Pts',(-81.7641325048579,1075.69528637324,
489.698827600322));
#130588=CARTESIAN_POINT('Ctrl Pts',(-81.2991932167898,1075.69528637324,
490.278728511509));
#130589=CARTESIAN_POINT('Ctrl Pts',(-80.8280936145958,1075.69528637324,
490.853636132955));
#130590=CARTESIAN_POINT('Ctrl Pts',(-81.6402549890788,1075.76855917516,
488.65701829957));
#130591=CARTESIAN_POINT('Ctrl Pts',(-81.1847793151174,1075.76855917516,
489.237702597704));
#130592=CARTESIAN_POINT('Ctrl Pts',(-80.7231344307362,1075.76855917516,
489.813494525742));
#130593=CARTESIAN_POINT('Ctrl Pts',(-80.2553728821466,1075.76855917516,
490.384328544814));
#130594=CARTESIAN_POINT('Origin',(0.,1082.7251047501,424.620242579854));
#130595=CARTESIAN_POINT('Ctrl Pts',(-70.1200501589484,1076.25692209858,
493.128459381365));
#130596=CARTESIAN_POINT('Ctrl Pts',(-69.5084690741912,1076.25692209858,
493.754429496216));
#130597=CARTESIAN_POINT('Ctrl Pts',(-68.8885611520353,1076.25692209858,
494.372154496493));
#130598=CARTESIAN_POINT('Ctrl Pts',(-68.2604375400634,1076.25692209858,
494.981523626005));
#130599=CARTESIAN_POINT('Ctrl Pts',(-69.4969951628274,1076.31897891888,
492.519726406178));
#130600=CARTESIAN_POINT('Ctrl Pts',(-68.8908483104976,1076.31897891888,
493.140134434199));
#130601=CARTESIAN_POINT('Ctrl Pts',(-68.2764486092736,1076.31897891888,
493.752370609999));
#130602=CARTESIAN_POINT('Ctrl Pts',(-67.6539062191311,1076.31897891888,
494.356325161516));
#130603=CARTESIAN_POINT('Ctrl Pts',(-68.8776818901403,1076.37494270955,
491.914649144295));
#130604=CARTESIAN_POINT('Ctrl Pts',(-68.276936635246,1076.37494270955,492.529528488301));
#130605=CARTESIAN_POINT('Ctrl Pts',(-67.668012075628,1076.37494270955,493.136308802465));
#130606=CARTESIAN_POINT('Ctrl Pts',(-67.0510173895858,1076.37494270955,
493.734881292945));
#130607=CARTESIAN_POINT('Ctrl Pts',(-68.2621119975104,1076.42481702568,
491.313229214258));
#130608=CARTESIAN_POINT('Ctrl Pts',(-67.6667356906106,1076.42481702568,
491.922613291853));
#130609=CARTESIAN_POINT('Ctrl Pts',(-67.0632531786269,1076.42481702568,
492.523970721817));
#130610=CARTESIAN_POINT('Ctrl Pts',(-66.4517726641162,1076.42481702568,
493.117193682615));
#130611=CARTESIAN_POINT('Origin',(0.,1082.7251047501,424.620242579854));
#130612=CARTESIAN_POINT('Ctrl Pts',(-57.9374139544679,1076.6276306297,494.864246584548));
#130613=CARTESIAN_POINT('Ctrl Pts',(-57.1515529148392,1076.6276306297,495.51242655391));
#130614=CARTESIAN_POINT('Ctrl Pts',(-56.3549261816959,1076.6276306297,496.147328667886));
#130615=CARTESIAN_POINT('Ctrl Pts',(-55.5477580706169,1076.6276306297,496.768774149603));
#130616=CARTESIAN_POINT('Ctrl Pts',(-57.2959682255943,1076.66233473874,
494.086550217513));
#130617=CARTESIAN_POINT('Ctrl Pts',(-56.5188077332104,1076.66233473874,
494.727553955758));
#130618=CARTESIAN_POINT('Ctrl Pts',(-55.7310007381363,1076.66233473874,
495.355426842478));
#130619=CARTESIAN_POINT('Ctrl Pts',(-54.9327690724731,1076.66233473874,
495.969992080104));
#130620=CARTESIAN_POINT('Ctrl Pts',(-56.659292123221,1076.68833210733,493.314636601901));
#130621=CARTESIAN_POINT('Ctrl Pts',(-55.8907674830364,1076.68833210733,
493.948517469649));
#130622=CARTESIAN_POINT('Ctrl Pts',(-55.1117146447132,1076.68833210733,
494.569413396651));
#130623=CARTESIAN_POINT('Ctrl Pts',(-54.3223529753417,1076.68833210733,
495.177149549924));
#130624=CARTESIAN_POINT('Ctrl Pts',(-56.0273881706553,1076.70562882264,
492.548508796999));
#130625=CARTESIAN_POINT('Ctrl Pts',(-55.2674346533982,1076.70562882264,
493.1753201831));
#130626=CARTESIAN_POINT('Ctrl Pts',(-54.497070355813,1076.70562882264,493.789291445574));
#130627=CARTESIAN_POINT('Ctrl Pts',(-53.7165121984548,1076.70562882264,
494.390249701295));
#130628=CARTESIAN_POINT('Origin',(0.,1082.7251047501,424.620242579854));
#130629=CARTESIAN_POINT('Ctrl Pts',(-106.420074485931,1074.64935171829,
462.896296919825));
#130630=CARTESIAN_POINT('Ctrl Pts',(-106.167092369887,1074.64935171829,
463.599670767973));
#130631=CARTESIAN_POINT('Ctrl Pts',(-105.907149585896,1074.64935171829,
464.300502038928));
#130632=CARTESIAN_POINT('Ctrl Pts',(-105.640271682601,1074.64935171829,
464.998721851043));
#130633=CARTESIAN_POINT('Ctrl Pts',(-105.721561764291,1074.75329679414,
462.645063202692));
#130634=CARTESIAN_POINT('Ctrl Pts',(-105.470240154756,1074.75329679414,
463.343820294243));
#130635=CARTESIAN_POINT('Ctrl Pts',(-105.212003565226,1074.75329679414,
464.040051497392));
#130636=CARTESIAN_POINT('Ctrl Pts',(-104.946877376646,1074.75329679414,
464.733688382615));
#130637=CARTESIAN_POINT('Ctrl Pts',(-105.026181850047,1074.85334179708,
462.39495626081));
#130638=CARTESIAN_POINT('Ctrl Pts',(-104.776513299703,1074.85334179708,
463.08911730177));
#130639=CARTESIAN_POINT('Ctrl Pts',(-104.519975252404,1074.85334179708,
463.780769068272));
#130640=CARTESIAN_POINT('Ctrl Pts',(-104.256592922156,1074.85334179708,
464.469843580884));
#130641=CARTESIAN_POINT('Ctrl Pts',(-104.33393585384,1074.94948853882,462.145976493642));
#130642=CARTESIAN_POINT('Ctrl Pts',(-104.085912912726,1074.94948853882,
462.835562197359));
#130643=CARTESIAN_POINT('Ctrl Pts',(-103.831065752719,1074.94948853882,
463.522655165687));
#130644=CARTESIAN_POINT('Ctrl Pts',(-103.569419421632,1074.94948853882,
464.207187867256));
#130645=CARTESIAN_POINT('Origin',(0.,1082.7251047501,424.620242579854));
#130646=CARTESIAN_POINT('Ctrl Pts',(-95.1717412686241,1075.53619529415,
471.271295452212));
#130647=CARTESIAN_POINT('Ctrl Pts',(-94.8408681026697,1075.53619529415,
471.946302197056));
#130648=CARTESIAN_POINT('Ctrl Pts',(-94.5028326909729,1075.53619529415,
472.617750793729));
#130649=CARTESIAN_POINT('Ctrl Pts',(-94.1576732917246,1075.53619529415,
473.285565248982));
#130650=CARTESIAN_POINT('Ctrl Pts',(-94.498905235811,1075.61803121392,470.941486320606));
#130651=CARTESIAN_POINT('Ctrl Pts',(-94.1703712451766,1075.61803121392,
471.611720967617));
#130652=CARTESIAN_POINT('Ctrl Pts',(-93.8347256437568,1075.61803121392,
472.27842262151));
#130653=CARTESIAN_POINT('Ctrl Pts',(-93.4920064192681,1075.61803121392,
472.941515826288));
#130654=CARTESIAN_POINT('Ctrl Pts',(-93.8293040304781,1075.69565811578,
470.613262828874));
#130655=CARTESIAN_POINT('Ctrl Pts',(-93.5030979689936,1075.69565811578,
471.278748321106));
#130656=CARTESIAN_POINT('Ctrl Pts',(-93.1698306882401,1075.69565811578,
471.940725854334));
#130657=CARTESIAN_POINT('Ctrl Pts',(-92.8295399067608,1075.69565811578,
472.599120507228));
#130658=CARTESIAN_POINT('Ctrl Pts',(-93.1629388435215,1075.76907803551,
470.286625560767));
#130659=CARTESIAN_POINT('Ctrl Pts',(-92.8390494608762,1075.76907803551,
470.947384849718));
#130660=CARTESIAN_POINT('Ctrl Pts',(-92.5081490069488,1075.76907803551,
471.604661092798));
#130661=CARTESIAN_POINT('Ctrl Pts',(-92.1702749324093,1075.76907803551,
472.258379900757));
#130662=CARTESIAN_POINT('Origin',(0.,1082.7251047501,424.620242579854));
#130663=CARTESIAN_POINT('Ctrl Pts',(-82.8304831843315,1076.25730969014,
477.043914818581));
#130664=CARTESIAN_POINT('Ctrl Pts',(-82.3617874431307,1076.25730969014,
477.78446375482));
#130665=CARTESIAN_POINT('Ctrl Pts',(-81.8832030846018,1076.25730969014,
478.518660892212));
#130666=CARTESIAN_POINT('Ctrl Pts',(-81.394816175536,1076.25730969014,479.246374195538));
#130667=CARTESIAN_POINT('Ctrl Pts',(-82.0961025158692,1076.31920325934,
476.579122993375));
#130668=CARTESIAN_POINT('Ctrl Pts',(-81.6315622628231,1076.31920325934,
477.313106172638));
#130669=CARTESIAN_POINT('Ctrl Pts',(-81.1572210655994,1076.31920325934,
478.040793868532));
#130670=CARTESIAN_POINT('Ctrl Pts',(-80.6731642279151,1076.31920325934,
478.762055216471));
#130671=CARTESIAN_POINT('Ctrl Pts',(-81.3661224427135,1076.3750308618,476.117116318722));
#130672=CARTESIAN_POINT('Ctrl Pts',(-80.9057127770828,1076.3750308618,476.84457308469));
#130673=CARTESIAN_POINT('Ctrl Pts',(-80.4355893150649,1076.3750308618,477.565790345312));
#130674=CARTESIAN_POINT('Ctrl Pts',(-79.9558366018756,1076.3750308618,478.280638399618));
#130675=CARTESIAN_POINT('Ctrl Pts',(-80.6405449088662,1076.42479602894,
475.657896024986));
#130676=CARTESIAN_POINT('Ctrl Pts',(-80.1842409189113,1076.42479602894,
476.378865738722));
#130677=CARTESIAN_POINT('Ctrl Pts',(-79.718309754768,1076.42479602894,477.093651587527));
#130678=CARTESIAN_POINT('Ctrl Pts',(-79.242835207725,1076.42479602894,477.802125027034));
#130679=CARTESIAN_POINT('Origin',(0.,1082.7251047501,424.620242579854));
#130680=CARTESIAN_POINT('Ctrl Pts',(-71.2826353250197,1076.62733493393,
481.288691976922));
#130681=CARTESIAN_POINT('Ctrl Pts',(-70.6478912735919,1076.62733493393,
482.087129718276));
#130682=CARTESIAN_POINT('Ctrl Pts',(-69.9998230975193,1076.62733493393,
482.874791115581));
#130683=CARTESIAN_POINT('Ctrl Pts',(-69.3386137191451,1076.62733493393,
483.651453845209));
#130684=CARTESIAN_POINT('Ctrl Pts',(-70.4927453171238,1076.66212086289,
480.660743224219));
#130685=CARTESIAN_POINT('Ctrl Pts',(-69.8650349279827,1076.66212086289,
481.450333397145));
#130686=CARTESIAN_POINT('Ctrl Pts',(-69.2241480601543,1076.66212086289,
482.229266639767));
#130687=CARTESIAN_POINT('Ctrl Pts',(-68.5702656090004,1076.66212086289,
482.997323092047));
#130688=CARTESIAN_POINT('Ctrl Pts',(-69.7087339478242,1076.68818379331,
480.037467886469));
#130689=CARTESIAN_POINT('Ctrl Pts',(-69.0880048739874,1076.68818379331,
480.818276337675));
#130690=CARTESIAN_POINT('Ctrl Pts',(-68.4542458685872,1076.68818379331,
481.588546383604));
#130691=CARTESIAN_POINT('Ctrl Pts',(-67.8076358150905,1076.68818379331,
482.348060609473));
#130692=CARTESIAN_POINT('Ctrl Pts',(-68.9306043300403,1076.7055298294,479.418868438389));
#130693=CARTESIAN_POINT('Ctrl Pts',(-68.3168041968055,1076.7055298294,480.190961049452));
#130694=CARTESIAN_POINT('Ctrl Pts',(-67.6901195797166,1076.7055298294,480.952632891074));
#130695=CARTESIAN_POINT('Ctrl Pts',(-67.0507273654387,1076.7055298294,481.703668975384));
#130696=CARTESIAN_POINT('Origin',(0.,1082.7251047501,424.620242579854));
#130697=CARTESIAN_POINT('Ctrl Pts',(-112.051426574092,1074.64943926585,
439.937715424524));
#130698=CARTESIAN_POINT('Ctrl Pts',(-111.950523798461,1074.64943926585,
440.675846320489));
#130699=CARTESIAN_POINT('Ctrl Pts',(-111.842332607831,1074.64943926585,
441.412944181006));
#130700=CARTESIAN_POINT('Ctrl Pts',(-111.726863565238,1074.64943926585,
442.148937040966));
#130701=CARTESIAN_POINT('Ctrl Pts',(-111.315440883155,1074.75345395672,
439.83710589924));
#130702=CARTESIAN_POINT('Ctrl Pts',(-111.215200865699,1074.75345395672,
440.570388541202));
#130703=CARTESIAN_POINT('Ctrl Pts',(-111.107720305631,1074.75345395672,
441.302644932987));
#130704=CARTESIAN_POINT('Ctrl Pts',(-110.993009696604,1074.75345395672,
442.033803582172));
#130705=CARTESIAN_POINT('Ctrl Pts',(-110.582758353619,1074.85356318489,
439.736947917383));
#130706=CARTESIAN_POINT('Ctrl Pts',(-110.483178119828,1074.85356318489,
440.465404064685));
#130707=CARTESIAN_POINT('Ctrl Pts',(-110.376405000956,1074.85356318489,
441.192840716628));
#130708=CARTESIAN_POINT('Ctrl Pts',(-110.262449421587,1074.85356318489,
441.919186851356));
#130709=CARTESIAN_POINT('Ctrl Pts',(-109.853380157329,1074.94976876584,
439.637241639143));
#130710=CARTESIAN_POINT('Ctrl Pts',(-109.754456731637,1074.94976876584,
440.360893058848));
#130711=CARTESIAN_POINT('Ctrl Pts',(-109.648387863464,1074.94976876584,
441.083531707549));
#130712=CARTESIAN_POINT('Ctrl Pts',(-109.535183908635,1074.94976876584,
441.805087031833));
#130713=CARTESIAN_POINT('Origin',(0.,1082.7251047501,424.620242579854));
#130714=CARTESIAN_POINT('Ctrl Pts',(-102.790046090129,1075.53649189674,
450.458426927557));
#130715=CARTESIAN_POINT('Ctrl Pts',(-102.60642453742,1075.53649189674,451.188914318317));
#130716=CARTESIAN_POINT('Ctrl Pts',(-102.415026793123,1075.53649189674,
451.917402894861));
#130717=CARTESIAN_POINT('Ctrl Pts',(-102.215874605379,1075.53649189674,
452.643809880507));
#130718=CARTESIAN_POINT('Ctrl Pts',(-102.064433267001,1075.61819462687,
450.276030687822));
#130719=CARTESIAN_POINT('Ctrl Pts',(-101.882107930787,1075.61819462687,
451.001361440969));
#130720=CARTESIAN_POINT('Ctrl Pts',(-101.692061296475,1075.61819462687,
451.724707489879));
#130721=CARTESIAN_POINT('Ctrl Pts',(-101.494314958681,1075.61819462687,
452.445986642201));
#130722=CARTESIAN_POINT('Ctrl Pts',(-101.342303806185,1075.69570098791,
450.094510055804));
#130723=CARTESIAN_POINT('Ctrl Pts',(-101.161268463875,1075.69570098791,
450.814708926189));
#130724=CARTESIAN_POINT('Ctrl Pts',(-100.972566453436,1075.69570098791,
451.532937134578));
#130725=CARTESIAN_POINT('Ctrl Pts',(-100.776219216697,1075.69570098791,
452.249113070151));
#130726=CARTESIAN_POINT('Ctrl Pts',(-100.623658988146,1075.7690130065,449.913865353371));
#130727=CARTESIAN_POINT('Ctrl Pts',(-100.443907414862,1075.7690130065,450.628957104945));
#130728=CARTESIAN_POINT('Ctrl Pts',(-100.256543539801,1075.7690130065,451.342092169003));
#130729=CARTESIAN_POINT('Ctrl Pts',(-100.061588652741,1075.7690130065,452.053189513449));
#130730=CARTESIAN_POINT('Origin',(0.,1082.7251047501,424.620242579854));
#130731=CARTESIAN_POINT('Ctrl Pts',(-91.9241429483952,1076.25698153983,
458.678803283175));
#130732=CARTESIAN_POINT('Ctrl Pts',(-91.6195337915803,1076.25698153983,
459.500944180976));
#130733=CARTESIAN_POINT('Ctrl Pts',(-91.3039232474814,1076.25698153983,
460.318924852328));
#130734=CARTESIAN_POINT('Ctrl Pts',(-90.9773681143258,1076.25698153983,
461.132598090958));
#130735=CARTESIAN_POINT('Ctrl Pts',(-91.1085750045413,1076.31894086093,
458.376629453401));
#130736=CARTESIAN_POINT('Ctrl Pts',(-90.8066683963251,1076.31894086093,
459.191476165582));
#130737=CARTESIAN_POINT('Ctrl Pts',(-90.493858007161,1076.31894086093,460.002199561611));
#130738=CARTESIAN_POINT('Ctrl Pts',(-90.1702001313522,1076.31894086093,
460.808653741254));
#130739=CARTESIAN_POINT('Ctrl Pts',(-90.297897541255,1076.37482552263,458.076267582095));
#130740=CARTESIAN_POINT('Ctrl Pts',(-89.9986772760452,1076.37482552263,
458.883863847592));
#130741=CARTESIAN_POINT('Ctrl Pts',(-89.6886502509362,1076.37482552263,
459.687373485902));
#130742=CARTESIAN_POINT('Ctrl Pts',(-89.3678722593284,1076.37482552263,
460.486651895004));
#130743=CARTESIAN_POINT('Ctrl Pts',(-89.492112720497,1076.42463906393,457.77771847028));
#130744=CARTESIAN_POINT('Ctrl Pts',(-89.1955625855377,1076.42463906393,
458.578108047362));
#130745=CARTESIAN_POINT('Ctrl Pts',(-88.8883021261812,1076.42463906393,
459.374447464799));
#130746=CARTESIAN_POINT('Ctrl Pts',(-88.5703866379484,1076.42463906393,
460.16659341094));
#130747=CARTESIAN_POINT('Origin',(0.,1082.7251047501,424.620242579854));
#130748=CARTESIAN_POINT('Ctrl Pts',(-81.5036900617922,1076.62735149554,
465.235366130203));
#130749=CARTESIAN_POINT('Ctrl Pts',(-81.0498664378651,1076.62735149554,
466.14606876395));
#130750=CARTESIAN_POINT('Ctrl Pts',(-80.5808440211162,1076.62735149554,
467.049037833927));
#130751=CARTESIAN_POINT('Ctrl Pts',(-80.0967545534475,1076.62735149554,
467.944019708627));
#130752=CARTESIAN_POINT('Ctrl Pts',(-80.5993187014014,1076.66218157195,
464.784697522318));
#130753=CARTESIAN_POINT('Ctrl Pts',(-80.1505307401276,1076.66218157195,
465.685294927956));
#130754=CARTESIAN_POINT('Ctrl Pts',(-79.6867126330335,1076.66218157195,
466.578244582057));
#130755=CARTESIAN_POINT('Ctrl Pts',(-79.2079946602025,1076.66218157195,
467.463295667427));
#130756=CARTESIAN_POINT('Ctrl Pts',(-79.7016870849284,1076.6882651034,464.33738748055));
#130757=CARTESIAN_POINT('Ctrl Pts',(-79.2578972584977,1076.6882651034,465.227954966357));
#130758=CARTESIAN_POINT('Ctrl Pts',(-78.799244676422,1076.6882651034,466.110959873351));
#130759=CARTESIAN_POINT('Ctrl Pts',(-78.3258581678604,1076.6882651034,466.986154177682));
#130760=CARTESIAN_POINT('Ctrl Pts',(-78.8107987860875,1076.70560821884,
463.893437785763));
#130761=CARTESIAN_POINT('Ctrl Pts',(-78.3719695467908,1076.70560821884,
464.774050699948));
#130762=CARTESIAN_POINT('Ctrl Pts',(-77.9184436845319,1076.70560821884,
465.647185568199));
#130763=CARTESIAN_POINT('Ctrl Pts',(-77.450348588445,1076.70560821884,466.512597139021));
#130764=CARTESIAN_POINT('Origin',(0.,1082.7251047501,424.620242579854));
#130765=CARTESIAN_POINT('Ctrl Pts',(-112.787114881755,1074.64949257569,
416.305931144629));
#130766=CARTESIAN_POINT('Ctrl Pts',(-112.841951325419,1074.64949257569,
417.049810456757));
#130767=CARTESIAN_POINT('Ctrl Pts',(-112.88942602191,1074.64949257569,417.794195854089));
#130768=CARTESIAN_POINT('Ctrl Pts',(-112.929534324867,1074.64949257569,
418.539014483421));
#130769=CARTESIAN_POINT('Ctrl Pts',(-112.046792792878,1074.75343612786,
416.360505360981));
#130770=CARTESIAN_POINT('Ctrl Pts',(-112.10126929622,1074.75343612786,417.099501931967));
#130771=CARTESIAN_POINT('Ctrl Pts',(-112.148432374078,1074.75343612786,
417.839001266268));
#130772=CARTESIAN_POINT('Ctrl Pts',(-112.188277410591,1074.75343612786,
418.578930988884));
#130773=CARTESIAN_POINT('Ctrl Pts',(-111.309791102948,1074.85347945785,
416.414834807964));
#130774=CARTESIAN_POINT('Ctrl Pts',(-111.363909280326,1074.85347945785,
417.14897053726));
#130775=CARTESIAN_POINT('Ctrl Pts',(-111.410762137185,1074.85347945785,
417.883605722883));
#130776=CARTESIAN_POINT('Ctrl Pts',(-111.450345088023,1074.85347945785,
418.618668465888));
#130777=CARTESIAN_POINT('Ctrl Pts',(-110.576110989133,1074.9496243775,416.468919398801));
#130778=CARTESIAN_POINT('Ctrl Pts',(-110.629872455478,1074.9496243775,417.198216193623));
#130779=CARTESIAN_POINT('Ctrl Pts',(-110.676416489465,1074.9496243775,417.928009152689));
#130780=CARTESIAN_POINT('Ctrl Pts',(-110.715738535817,1074.9496243775,418.658226850962));
#130781=CARTESIAN_POINT('Origin',(0.,1082.7251047501,424.620242579854));
#130782=CARTESIAN_POINT('Ctrl Pts',(-105.916863873868,1075.53636233154,
428.528540576853));
#130783=CARTESIAN_POINT('Ctrl Pts',(-105.889193093616,1075.53636233154,
429.278432797824));
#130784=CARTESIAN_POINT('Ctrl Pts',(-105.853560308952,1075.53636233154,
430.027988879656));
#130785=CARTESIAN_POINT('Ctrl Pts',(-105.809969538517,1075.53636233154,
430.777124287901));
#130786=CARTESIAN_POINT('Ctrl Pts',(-105.168863810439,1075.61810436561,
428.500939616602));
#130787=CARTESIAN_POINT('Ctrl Pts',(-105.141388445201,1075.61810436561,
429.2455359913));
#130788=CARTESIAN_POINT('Ctrl Pts',(-105.106007304366,1075.61810436561,
429.989798600721));
#130789=CARTESIAN_POINT('Ctrl Pts',(-105.062724378195,1075.61810436561,
430.733643507413));
#130790=CARTESIAN_POINT('Ctrl Pts',(-104.424456094477,1075.69564644726,
428.47347121281));
#130791=CARTESIAN_POINT('Ctrl Pts',(-104.397175205751,1075.69564644726,
429.212797175083));
#130792=CARTESIAN_POINT('Ctrl Pts',(-104.3620445002,1075.69564644726,429.95179173454));
#130793=CARTESIAN_POINT('Ctrl Pts',(-104.31906793984,1075.69564644726,430.690371547858));
#130794=CARTESIAN_POINT('Ctrl Pts',(-103.683642047071,1075.7689906057,428.446135414225));
#130795=CARTESIAN_POINT('Ctrl Pts',(-103.656554696013,1075.7689906057,429.180216407274));
#130796=CARTESIAN_POINT('Ctrl Pts',(-103.621673216755,1075.7689906057,429.913968348564));
#130797=CARTESIAN_POINT('Ctrl Pts',(-103.579001543208,1075.7689906057,430.647308486031));
#130798=CARTESIAN_POINT('Origin',(0.,1082.7251047501,424.620242579854));
#130799=CARTESIAN_POINT('Ctrl Pts',(-96.9953277889122,1076.25703779475,
438.82535338608));
#130800=CARTESIAN_POINT('Ctrl Pts',(-96.8685997973428,1076.25703779475,
439.690677370524));
#130801=CARTESIAN_POINT('Ctrl Pts',(-96.7303041265953,1076.25703779475,
440.554228115619));
#130802=CARTESIAN_POINT('Ctrl Pts',(-96.580465540314,1076.25703779475,441.415850991338));
#130803=CARTESIAN_POINT('Ctrl Pts',(-96.1346410229007,1076.31900226003,
438.699304522085));
#130804=CARTESIAN_POINT('Ctrl Pts',(-96.0090375504984,1076.31900226003,
439.556950065528));
#130805=CARTESIAN_POINT('Ctrl Pts',(-95.8719690445673,1076.31900226003,
440.412838104439));
#130806=CARTESIAN_POINT('Ctrl Pts',(-95.7234600490115,1076.31900226003,
441.266815380898));
#130807=CARTESIAN_POINT('Ctrl Pts',(-95.2791160427069,1076.37489033703,
438.574011609342));
#130808=CARTESIAN_POINT('Ctrl Pts',(-95.1546303454073,1076.37489033703,
439.424024761602));
#130809=CARTESIAN_POINT('Ctrl Pts',(-95.0187816446325,1076.37489033703,
440.272296049779));
#130810=CARTESIAN_POINT('Ctrl Pts',(-94.8715942658647,1076.37489033703,
441.118673579832));
#130811=CARTESIAN_POINT('Ctrl Pts',(-94.4287551305539,1076.42470556629,
438.449474982086));
#130812=CARTESIAN_POINT('Ctrl Pts',(-94.3053804613106,1076.42470556629,
439.29190181334));
#130813=CARTESIAN_POINT('Ctrl Pts',(-94.1707442027782,1076.42470556629,
440.132602326552));
#130814=CARTESIAN_POINT('Ctrl Pts',(-94.0248704633352,1076.42470556629,
440.971425983329));
#130815=CARTESIAN_POINT('Origin',(0.,1082.7251047501,424.620242579854));
#130816=CARTESIAN_POINT('Ctrl Pts',(-88.1662720496537,1076.62742624042,
447.39639773452));
#130817=CARTESIAN_POINT('Ctrl Pts',(-87.9111819950692,1076.62742624042,
448.38384882084));
#130818=CARTESIAN_POINT('Ctrl Pts',(-87.6395405034666,1076.62742624042,
449.366875516236));
#130819=CARTESIAN_POINT('Ctrl Pts',(-87.3514242321929,1076.62742624042,
450.345200410149));
#130820=CARTESIAN_POINT('Ctrl Pts',(-87.1889865167269,1076.66220724281,
447.143933766033));
#130821=CARTESIAN_POINT('Ctrl Pts',(-86.936724026631,1076.66220724281,448.120439378095));
#130822=CARTESIAN_POINT('Ctrl Pts',(-86.6680935651391,1076.66220724281,
449.09256964172));
#130823=CARTESIAN_POINT('Ctrl Pts',(-86.383170939884,1076.66220724281,450.060050221327));
#130824=CARTESIAN_POINT('Ctrl Pts',(-86.2189765468992,1076.68826006274,
446.893349307138));
#130825=CARTESIAN_POINT('Ctrl Pts',(-85.9695205710223,1076.68826006274,
447.858990930328));
#130826=CARTESIAN_POINT('Ctrl Pts',(-85.7038787235315,1076.68826006274,
448.820305882463));
#130827=CARTESIAN_POINT('Ctrl Pts',(-85.4221259686714,1076.68826006274,
449.777022880047));
#130828=CARTESIAN_POINT('Ctrl Pts',(-85.2562459939478,1076.70559080985,
446.644645353388));
#130829=CARTESIAN_POINT('Ctrl Pts',(-85.0095754708705,1076.70559080985,
447.599504516253));
#130830=CARTESIAN_POINT('Ctrl Pts',(-84.7468998093977,1076.70559080985,
448.550085320147));
#130831=CARTESIAN_POINT('Ctrl Pts',(-84.4682931367152,1076.70559080985,
449.496119510755));
#130832=CARTESIAN_POINT('Origin',(0.,1082.7251047501,424.620242579854));
#130833=CARTESIAN_POINT('Ctrl Pts',(-108.594074399517,1074.64939441013,
393.036280926091));
#130834=CARTESIAN_POINT('Ctrl Pts',(-108.802630048851,1074.64939441013,
393.753350809485));
#130835=CARTESIAN_POINT('Ctrl Pts',(-109.004073252079,1074.64939441013,
394.47245115882));
#130836=CARTESIAN_POINT('Ctrl Pts',(-109.198384247329,1074.64939441013,
395.193511429301));
#130837=CARTESIAN_POINT('Ctrl Pts',(-107.880346429781,1074.75347617509,
393.243864599068));
#130838=CARTESIAN_POINT('Ctrl Pts',(-108.087531359755,1074.75347617509,
393.956221584131));
#130839=CARTESIAN_POINT('Ctrl Pts',(-108.287650589744,1074.75347617509,
394.67059569002));
#130840=CARTESIAN_POINT('Ctrl Pts',(-108.480684487759,1074.75347617509,
395.386916835592));
#130841=CARTESIAN_POINT('Ctrl Pts',(-107.169823753786,1074.85364752299,
393.450516030804));
#130842=CARTESIAN_POINT('Ctrl Pts',(-107.375644120187,1074.85364752299,
394.158181282776));
#130843=CARTESIAN_POINT('Ctrl Pts',(-107.574445322792,1074.85364752299,
394.867850370391));
#130844=CARTESIAN_POINT('Ctrl Pts',(-107.766207858911,1074.85364752299,
395.579453674075));
#130845=CARTESIAN_POINT('Ctrl Pts',(-106.462507509375,1074.94991027277,
393.656234890365));
#130846=CARTESIAN_POINT('Ctrl Pts',(-106.666969470178,1074.94991027277,
394.359229581998));
#130847=CARTESIAN_POINT('Ctrl Pts',(-106.864458593364,1074.94991027277,
395.064214884045));
#130848=CARTESIAN_POINT('Ctrl Pts',(-107.054955504962,1074.94991027277,
395.771121636418));
#130849=CARTESIAN_POINT('Origin',(0.,1082.7251047501,424.620242579854));
#130850=CARTESIAN_POINT('Ctrl Pts',(-104.413416366025,1075.53647952796,
406.419477816671));
#130851=CARTESIAN_POINT('Ctrl Pts',(-104.542624892593,1075.53647952796,
407.160716102985));
#130852=CARTESIAN_POINT('Ctrl Pts',(-104.663933237021,1075.53647952796,
407.903288204539));
#130853=CARTESIAN_POINT('Ctrl Pts',(-104.777327644461,1075.53647952796,
408.64710992296));
#130854=CARTESIAN_POINT('Ctrl Pts',(-103.676158825789,1075.61820324334,
406.547992441772));
#130855=CARTESIAN_POINT('Ctrl Pts',(-103.804455017872,1075.61820324334,
407.283996884248));
#130856=CARTESIAN_POINT('Ctrl Pts',(-103.924906810578,1075.61820324334,
408.021325723968));
#130857=CARTESIAN_POINT('Ctrl Pts',(-104.037500546181,1075.61820324334,
408.759895357077));
#130858=CARTESIAN_POINT('Ctrl Pts',(-102.942441438183,1075.69572847712,
406.675889967198));
#130859=CARTESIAN_POINT('Ctrl Pts',(-103.069829676616,1075.69572847712,
407.406685697633));
#130860=CARTESIAN_POINT('Ctrl Pts',(-103.189429030577,1075.69572847712,
408.138796452538));
#130861=CARTESIAN_POINT('Ctrl Pts',(-103.301225938997,1075.69572847712,
408.872139219722));
#130862=CARTESIAN_POINT('Ctrl Pts',(-102.212265504876,1075.76905725745,
406.803170166049));
#130863=CARTESIAN_POINT('Ctrl Pts',(-102.338750172103,1075.76905725745,
407.528782325481));
#130864=CARTESIAN_POINT('Ctrl Pts',(-102.45750120181,1075.76905725745,408.255700181846));
#130865=CARTESIAN_POINT('Ctrl Pts',(-102.568505129116,1075.76905725745,
408.983841311767));
#130866=CARTESIAN_POINT('Origin',(0.,1082.7251047501,424.620242579854));
#130867=CARTESIAN_POINT('Ctrl Pts',(-97.8296100732469,1076.25700990573,
418.349442191101));
#130868=CARTESIAN_POINT('Ctrl Pts',(-97.8855743077914,1076.25700990573,
419.2225299796));
#130869=CARTESIAN_POINT('Ctrl Pts',(-97.9298463187621,1076.25700990573,
420.096288682573));
#130870=CARTESIAN_POINT('Ctrl Pts',(-97.9624181728472,1076.25700990573,
420.970561727049));
#130871=CARTESIAN_POINT('Ctrl Pts',(-96.9619111406566,1076.31894843203,
418.405061004257));
#130872=CARTESIAN_POINT('Ctrl Pts',(-97.0173790008771,1076.31894843203,
419.270404947702));
#130873=CARTESIAN_POINT('Ctrl Pts',(-97.0612583416058,1076.31894843203,
420.13641385495));
#130874=CARTESIAN_POINT('Ctrl Pts',(-97.0935412998954,1076.31894843203,
421.002932541753));
#130875=CARTESIAN_POINT('Ctrl Pts',(-96.0994137067278,1076.37481601301,
418.460346405476));
#130876=CARTESIAN_POINT('Ctrl Pts',(-96.1543881681843,1076.37481601301,
419.317992925037));
#130877=CARTESIAN_POINT('Ctrl Pts',(-96.1978771925678,1076.37481601301,
420.176298493401));
#130878=CARTESIAN_POINT('Ctrl Pts',(-96.2298729868736,1076.37481601301,
421.035109306721));
#130879=CARTESIAN_POINT('Ctrl Pts',(-95.2421200702117,1076.42461618443,
418.515298247409));
#130880=CARTESIAN_POINT('Ctrl Pts',(-95.2966041097795,1076.42461618443,
419.365293784771));
#130881=CARTESIAN_POINT('Ctrl Pts',(-95.3397051727548,1076.42461618443,
420.215942491626));
#130882=CARTESIAN_POINT('Ctrl Pts',(-95.3714155356537,1076.42461618443,
421.067091936193));
#130899=UNCERTAINTY_MEASURE_WITH_UNIT(LENGTH_MEASURE(0.01),#130911,
'DISTANCE_ACCURACY_VALUE',
'Maximum model space distance between geometric entities at asserted c
onnectivities');
#130900=UNCERTAINTY_MEASURE_WITH_UNIT(LENGTH_MEASURE(0.01),#130911,
'DISTANCE_ACCURACY_VALUE',
'Maximum model space distance between geometric entities at asserted c
onnectivities');
#130909=(
GEOMETRIC_REPRESENTATION_CONTEXT(3)
GLOBAL_UNCERTAINTY_ASSIGNED_CONTEXT((#130899))
GLOBAL_UNIT_ASSIGNED_CONTEXT((#130911,#130913,#130914))
REPRESENTATION_CONTEXT('','3D')
);
#130910=(
GEOMETRIC_REPRESENTATION_CONTEXT(3)
GLOBAL_UNCERTAINTY_ASSIGNED_CONTEXT((#130900))
GLOBAL_UNIT_ASSIGNED_CONTEXT((#130911,#130913,#130914))
REPRESENTATION_CONTEXT('','3D')
);
#130911=(
LENGTH_UNIT()
NAMED_UNIT(*)
SI_UNIT(.MILLI.,.METRE.)
);
#130913=(
NAMED_UNIT(*)
PLANE_ANGLE_UNIT()
SI_UNIT($,.RADIAN.)
);
#130914=(
NAMED_UNIT(*)
SI_UNIT($,.STERADIAN.)
SOLID_ANGLE_UNIT()
);
#130923=SHAPE_DEFINITION_REPRESENTATION(#130932,#130949);
#130932=PRODUCT_DEFINITION_SHAPE('',$,#130959);
#130949=SHAPE_REPRESENTATION('',(#48902),#130909);
#130950=PRODUCT_DEFINITION_CONTEXT('part definition',#130979,'design');
#130959=PRODUCT_DEFINITION('Component8','Component8',#130968,#130950);
#130968=PRODUCT_DEFINITION_FORMATION('',$,#130989);
#130979=APPLICATION_CONTEXT(
'Core Data for Automotive Mechanical Design Process');
#130980=PRODUCT_CONTEXT('part definition',#130979,'mechanical');
#130989=PRODUCT('Component8','Component8',$,(#130980));
#130991=PRESENTATION_STYLE_ASSIGNMENT((#130993));
#130993=SURFACE_STYLE_USAGE(.BOTH.,#130995);
#130995=SURFACE_SIDE_STYLE('',(#130997));
#130997=SURFACE_STYLE_FILL_AREA(#130999);
#130999=FILL_AREA_STYLE('Opaque(202,209,238)',(#131001));
#131001=FILL_AREA_STYLE_COLOUR('Opaque(202,209,238)',#131003);
#131003=COLOUR_RGB('Opaque(202,209,238)', 0.40784314, 0.44705882, 0.49803922);
ENDSEC;
END-ISO-10303-21;
